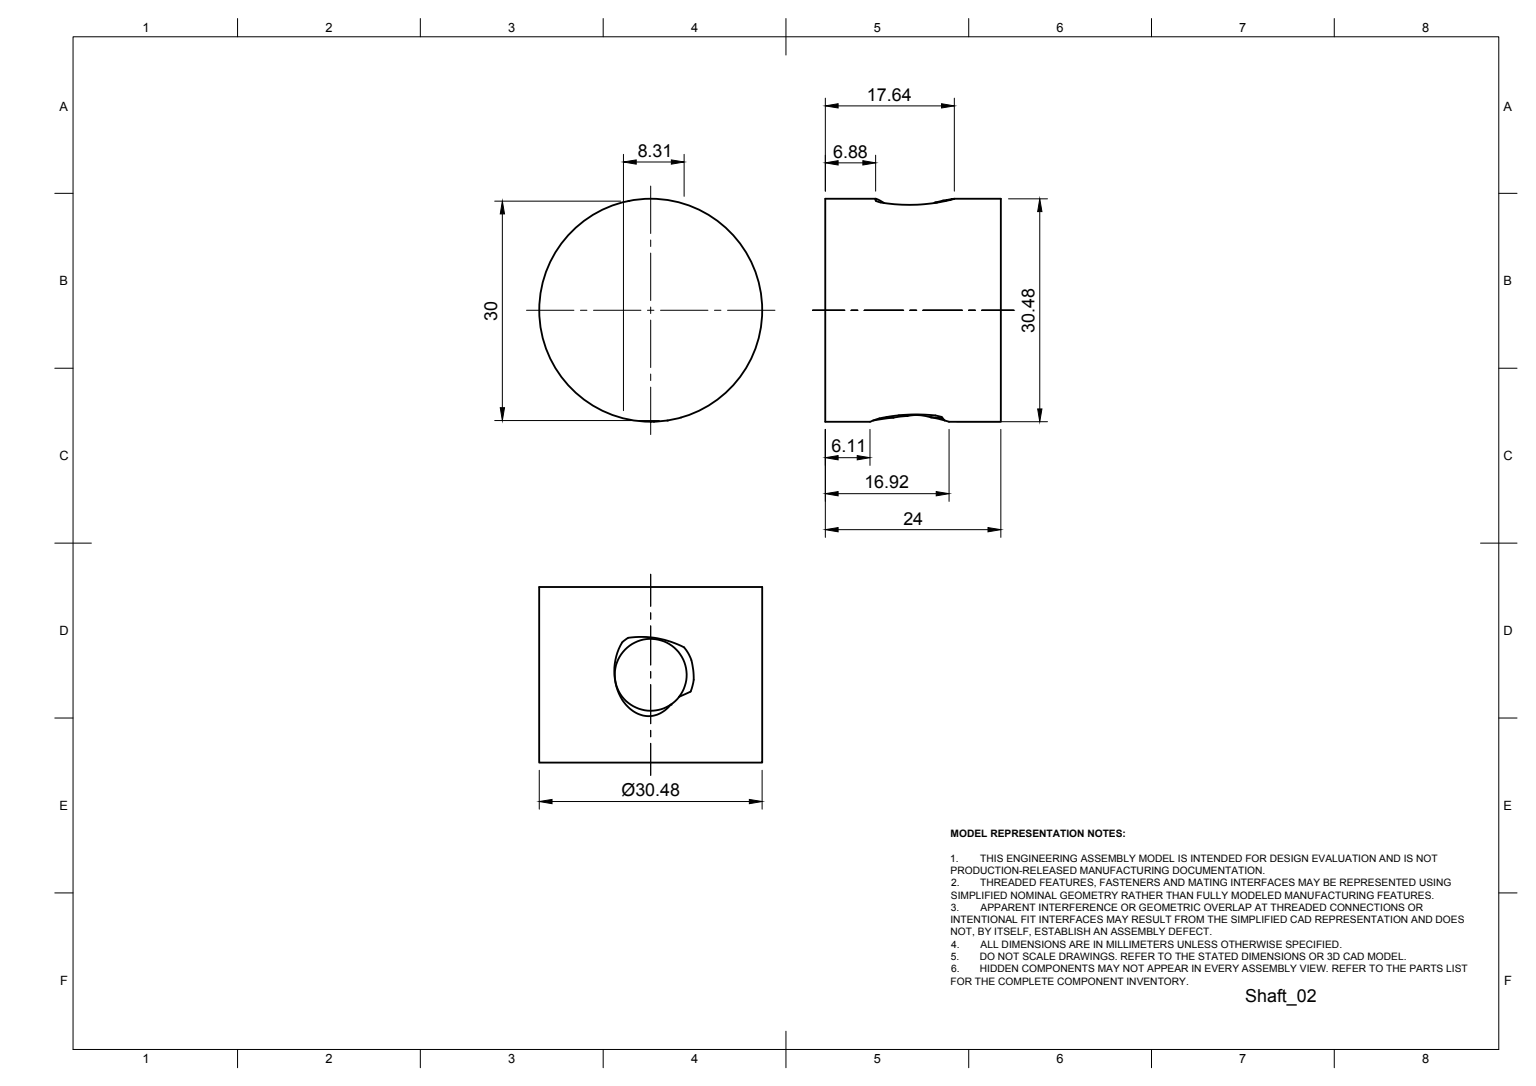
ISO-10303-21;
HEADER;
/* Generated by software containing ST-Developer
 * from STEP Tools, Inc. (www.steptools.com) 
 */

FILE_DESCRIPTION(
/* description */ (''),
/* implementation_level */ '2;1');

FILE_NAME(
/* name */ 'Shaft_02.step',
/* time_stamp */ '2026-10-06T13:41:14-07:00',
/* author */ (''),
/* organization */ (''),
/* preprocessor_version */ 'ST-DEVELOPER v20.2',
/* originating_system */ 'Autodesk Translation Framework v15.15.0.0',
/* authorisation */ '');

FILE_SCHEMA (('AUTOMOTIVE_DESIGN { 1 0 10303 214 3 1 1 }'));
ENDSEC;

DATA;
#10=MECHANICAL_DESIGN_GEOMETRIC_PRESENTATION_REPRESENTATION('',(#1967),#279266);
#53=B_SPLINE_SURFACE_WITH_KNOTS('',3,3,((#247756,#247757,#247758,#247759,
#247760,#247761,#247762,#247763,#247764,#247765,#247766,#247767,#247768,
#247769,#247770,#247771,#247772,#247773,#247774,#247775,#247776,#247777,
#247778,#247779,#247780,#247781,#247782,#247783,#247784,#247785,#247786,
#247787,#247788,#247789,#247790,#247791,#247792,#247793,#247794,#247795,
#247796,#247797,#247798,#247799,#247800,#247801,#247802,#247803,#247804,
#247805,#247806,#247807,#247808,#247809,#247810,#247811,#247812,#247813,
#247814,#247815,#247816,#247817,#247818,#247819,#247820,#247821,#247822,
#247823,#247824,#247825,#247826,#247827,#247828,#247829,#247830,#247831,
#247832,#247833,#247834,#247835,#247836,#247837,#247838,#247839,#247840,
#247841,#247842,#247843,#247844,#247845,#247846,#247847,#247848,#247849,
#247850,#247851,#247852,#247853,#247854,#247855,#247856,#247857,#247858,
#247859,#247860,#247861,#247862,#247863,#247864,#247865,#247866,#247867,
#247868,#247869,#247870,#247871,#247872,#247873,#247874,#247875,#247876,
#247877,#247878,#247879,#247880,#247881,#247882,#247883,#247884,#247885,
#247886,#247887,#247888,#247889,#247890,#247891,#247892,#247893,#247894,
#247895,#247896,#247897,#247898,#247899,#247900,#247901,#247902,#247903,
#247904,#247905,#247906,#247907,#247908,#247909,#247910,#247911,#247912,
#247913,#247914,#247915,#247916,#247917,#247918,#247919,#247920,#247921,
#247922,#247923,#247924,#247925,#247926,#247927,#247928,#247929,#247930,
#247931,#247932,#247933,#247934,#247935,#247936,#247937,#247938,#247939,
#247940,#247941,#247942,#247943,#247944,#247945,#247946,#247947,#247948,
#247949,#247950,#247951,#247952,#247953,#247954,#247955,#247956,#247957,
#247958,#247959,#247960,#247961,#247962,#247963,#247964,#247965,#247966,
#247967,#247968,#247969,#247970,#247971,#247972,#247973,#247974,#247975,
#247976,#247977,#247978,#247979,#247980,#247981,#247982,#247983,#247984,
#247985,#247986,#247987,#247988,#247989,#247990,#247991,#247992,#247993,
#247994,#247995,#247996,#247997,#247998,#247999,#248000,#248001,#248002,
#248003,#248004,#248005,#248006,#248007,#248008,#248009,#248010,#248011,
#248012,#248013,#248014,#248015,#248016,#248017,#248018,#248019,#248020,
#248021,#248022,#248023,#248024,#248025,#248026,#248027,#248028,#248029,
#248030,#248031,#248032,#248033,#248034,#248035,#248036,#248037,#248038,
#248039,#248040,#248041,#248042,#248043,#248044,#248045,#248046,#248047,
#248048,#248049,#248050,#248051,#248052,#248053,#248054,#248055,#248056,
#248057,#248058,#248059,#248060,#248061,#248062,#248063,#248064,#248065,
#248066,#248067,#248068,#248069,#248070,#248071,#248072,#248073,#248074,
#248075,#248076,#248077,#248078,#248079,#248080,#248081,#248082,#248083,
#248084,#248085,#248086,#248087,#248088,#248089,#248090,#248091,#248092,
#248093,#248094,#248095,#248096,#248097,#248098,#248099,#248100,#248101,
#248102,#248103,#248104,#248105,#248106,#248107,#248108,#248109,#248110,
#248111,#248112,#248113,#248114,#248115,#248116,#248117,#248118,#248119,
#248120,#248121,#248122,#248123,#248124,#248125,#248126,#248127,#248128,
#248129,#248130,#248131,#248132,#248133,#248134,#248135,#248136,#248137,
#248138,#248139,#248140,#248141,#248142,#248143,#248144,#248145,#248146,
#248147,#248148,#248149,#248150,#248151,#248152,#248153,#248154,#248155,
#248156,#248157,#248158,#248159,#248160,#248161,#248162,#248163,#248164,
#248165,#248166,#248167,#248168,#248169,#248170,#248171,#248172,#248173,
#248174,#248175,#248176,#248177,#248178,#248179,#248180,#248181,#248182,
#248183,#248184,#248185,#248186,#248187,#248188,#248189,#248190,#248191,
#248192,#248193,#248194,#248195,#248196,#248197,#248198,#248199,#248200,
#248201,#248202,#248203,#248204,#248205,#248206,#248207,#248208,#248209,
#248210,#248211,#248212,#248213,#248214,#248215,#248216,#248217,#248218,
#248219,#248220,#248221,#248222,#248223,#248224,#248225,#248226,#248227,
#248228,#248229,#248230,#248231,#248232,#248233,#248234,#248235,#248236,
#248237,#248238,#248239,#248240,#248241,#248242,#248243,#248244,#248245,
#248246,#248247,#248248,#248249,#248250,#248251,#248252,#248253,#248254,
#248255,#248256,#248257,#248258,#248259,#248260,#248261,#248262,#248263,
#248264,#248265,#248266,#248267,#248268,#248269,#248270,#248271,#248272,
#248273,#248274,#248275,#248276,#248277,#248278,#248279,#248280,#248281,
#248282,#248283,#248284,#248285,#248286,#248287,#248288,#248289,#248290,
#248291,#248292,#248293,#248294,#248295,#248296,#248297,#248298,#248299,
#248300,#248301,#248302,#248303,#248304,#248305,#248306,#248307,#248308,
#248309,#248310,#248311,#248312,#248313,#248314,#248315,#248316,#248317,
#248318,#248319,#248320,#248321,#248322,#248323,#248324,#248325,#248326,
#248327,#248328,#248329,#248330,#248331,#248332,#248333,#248334,#248335,
#248336,#248337,#248338,#248339,#248340,#248341,#248342,#248343,#248344,
#248345,#248346,#248347,#248348,#248349,#248350,#248351,#248352,#248353,
#248354,#248355,#248356,#248357,#248358,#248359,#248360,#248361,#248362,
#248363,#248364,#248365,#248366,#248367,#248368,#248369,#248370,#248371,
#248372,#248373,#248374,#248375,#248376,#248377,#248378,#248379,#248380,
#248381,#248382,#248383,#248384,#248385,#248386,#248387,#248388,#248389,
#248390,#248391,#248392,#248393,#248394,#248395,#248396,#248397,#248398,
#248399,#248400,#248401,#248402,#248403,#248404,#248405,#248406,#248407,
#248408,#248409,#248410,#248411,#248412,#248413,#248414,#248415,#248416,
#248417,#248418,#248419,#248420,#248421,#248422,#248423,#248424,#248425,
#248426,#248427,#248428,#248429,#248430,#248431,#248432,#248433,#248434,
#248435,#248436,#248437,#248438,#248439,#248440,#248441,#248442,#248443,
#248444,#248445,#248446,#248447,#248448,#248449,#248450,#248451,#248452,
#248453,#248454,#248455,#248456,#248457,#248458,#248459,#248460,#248461,
#248462,#248463,#248464,#248465,#248466,#248467,#248468,#248469,#248470,
#248471,#248472,#248473,#248474,#248475,#248476,#248477,#248478,#248479,
#248480,#248481,#248482,#248483,#248484,#248485,#248486,#248487,#248488,
#248489,#248490,#248491,#248492,#248493,#248494,#248495,#248496,#248497,
#248498,#248499,#248500,#248501,#248502,#248503,#248504,#248505,#248506,
#248507,#248508,#248509,#248510,#248511,#248512,#248513,#248514,#248515,
#248516,#248517,#248518,#248519,#248520,#248521,#248522,#248523,#248524,
#248525,#248526,#248527,#248528,#248529,#248530,#248531,#248532,#248533,
#248534,#248535,#248536,#248537,#248538,#248539,#248540,#248541,#248542,
#248543,#248544,#248545,#248546,#248547,#248548,#248549,#248550,#248551,
#248552,#248553,#248554,#248555,#248556,#248557,#248558,#248559,#248560,
#248561,#248562,#248563,#248564,#248565,#248566,#248567,#248568,#248569,
#248570,#248571,#248572,#248573,#248574,#248575,#248576,#248577,#248578,
#248579,#248580,#248581,#248582,#248583,#248584,#248585,#248586,#248587,
#248588,#248589,#248590,#248591,#248592,#248593,#248594,#248595,#248596,
#248597,#248598,#248599,#248600,#248601,#248602,#248603,#248604,#248605,
#248606,#248607,#248608,#248609,#248610,#248611,#248612,#248613,#248614,
#248615,#248616,#248617,#248618,#248619,#248620,#248621,#248622,#248623,
#248624,#248625,#248626,#248627,#248628,#248629,#248630,#248631,#248632,
#248633,#248634,#248635,#248636,#248637,#248638,#248639,#248640,#248641,
#248642,#248643,#248644,#248645,#248646,#248647,#248648,#248649,#248650,
#248651,#248652,#248653,#248654,#248655,#248656,#248657,#248658,#248659,
#248660,#248661,#248662,#248663,#248664,#248665,#248666,#248667,#248668,
#248669,#248670,#248671,#248672,#248673,#248674,#248675,#248676,#248677,
#248678,#248679,#248680,#248681,#248682,#248683,#248684,#248685,#248686,
#248687,#248688,#248689,#248690,#248691,#248692,#248693,#248694,#248695,
#248696,#248697,#248698,#248699,#248700,#248701,#248702,#248703,#248704,
#248705,#248706,#248707,#248708,#248709,#248710,#248711,#248712,#248713,
#248714,#248715,#248716,#248717,#248718,#248719,#248720,#248721,#248722,
#248723,#248724,#248725,#248726,#248727,#248728,#248729,#248730,#248731,
#248732,#248733,#248734,#248735,#248736,#248737,#248738,#248739,#248740,
#248741,#248742,#248743,#248744,#248745,#248746,#248747,#248748,#248749,
#248750,#248751,#248752,#248753,#248754,#248755,#248756,#248757,#248758,
#248759,#248760,#248761,#248762,#248763,#248764,#248765,#248766,#248767,
#248768,#248769,#248770,#248771,#248772,#248773,#248774,#248775,#248776,
#248777,#248778,#248779,#248780,#248781,#248782,#248783,#248784,#248785,
#248786,#248787,#248788,#248789,#248790,#248791,#248792,#248793,#248794,
#248795,#248796,#248797,#248798,#248799,#248800,#248801,#248802,#248803,
#248804,#248805,#248806,#248807,#248808,#248809,#248810,#248811,#248812,
#248813,#248814,#248815,#248816,#248817,#248818,#248819,#248820,#248821,
#248822,#248823,#248824,#248825,#248826,#248827,#248828,#248829,#248830,
#248831,#248832,#248833,#248834,#248835,#248836,#248837,#248838,#248839,
#248840,#248841,#248842,#248843,#248844,#248845,#248846,#248847,#248848,
#248849,#248850,#248851,#248852,#248853,#248854,#248855,#248856,#248857,
#248858,#248859,#248860,#248861,#248862,#248863,#248864,#248865,#248866,
#248867,#248868,#248869,#248870,#248871,#248872,#248873,#248874,#248875,
#248876,#248877,#248878,#248879,#248880,#248881,#248882,#248883,#248884,
#248885,#248886,#248887,#248888,#248889,#248890,#248891,#248892,#248893,
#248894,#248895,#248896,#248897,#248898,#248899,#248900,#248901,#248902,
#248903,#248904,#248905,#248906,#248907,#248908,#248909,#248910,#248911,
#248912,#248913,#248914,#248915,#248916,#248917,#248918,#248919,#248920,
#248921,#248922,#248923,#248924,#248925,#248926,#248927,#248928,#248929,
#248930,#248931,#248932,#248933,#248934,#248935,#248936,#248937,#248938,
#248939,#248940,#248941,#248942,#248943,#248944,#248945,#248946,#248947,
#248948,#248949,#248950,#248951,#248952,#248953,#248954,#248955,#248956,
#248957,#248958,#248959,#248960,#248961,#248962,#248963,#248964,#248965,
#248966,#248967,#248968,#248969,#248970,#248971,#248972,#248973,#248974,
#248975,#248976,#248977,#248978,#248979,#248980,#248981,#248982,#248983,
#248984,#248985,#248986,#248987,#248988,#248989,#248990,#248991,#248992,
#248993,#248994,#248995,#248996,#248997,#248998,#248999,#249000,#249001,
#249002,#249003,#249004,#249005,#249006,#249007,#249008,#249009,#249010,
#249011,#249012,#249013,#249014,#249015,#249016,#249017,#249018,#249019,
#249020,#249021,#249022,#249023,#249024,#249025,#249026,#249027,#249028,
#249029,#249030,#249031,#249032,#249033,#249034,#249035,#249036,#249037,
#249038,#249039,#249040,#249041,#249042,#249043,#249044,#249045,#249046,
#249047,#249048,#249049,#249050,#249051,#249052,#249053,#249054,#249055,
#249056,#249057,#249058,#249059,#249060,#249061,#249062,#249063,#249064,
#249065,#249066,#249067,#249068,#249069,#249070,#249071,#249072,#249073,
#249074,#249075,#249076,#249077,#249078,#249079,#249080,#249081,#249082,
#249083,#249084,#249085,#249086,#249087,#249088,#249089,#249090,#249091,
#249092,#249093,#249094,#249095,#249096,#249097,#249098,#249099,#249100,
#249101,#249102,#249103,#249104,#249105,#249106,#249107,#249108,#249109,
#249110,#249111,#249112,#249113,#249114,#249115,#249116,#249117,#249118,
#249119,#249120,#249121,#249122,#249123,#249124,#249125,#249126,#249127,
#249128,#249129,#249130,#249131,#249132,#249133,#249134,#249135,#249136,
#249137,#249138,#249139,#249140,#249141,#249142,#249143,#249144,#249145,
#249146,#249147,#249148,#249149,#249150,#249151,#249152,#249153,#249154,
#249155,#249156,#249157,#249158,#249159,#249160,#249161,#249162,#249163,
#249164,#249165,#249166,#249167,#249168,#249169,#249170,#249171,#249172,
#249173,#249174,#249175,#249176,#249177,#249178,#249179,#249180,#249181,
#249182,#249183,#249184,#249185,#249186,#249187,#249188,#249189,#249190,
#249191,#249192,#249193,#249194,#249195,#249196,#249197,#249198,#249199,
#249200,#249201,#249202,#249203,#249204,#249205,#249206,#249207,#249208,
#249209,#249210,#249211,#249212,#249213,#249214,#249215,#249216,#249217,
#249218,#249219,#249220,#249221,#249222,#249223,#249224,#249225,#249226,
#249227,#249228,#249229,#249230,#249231,#249232,#249233,#249234,#249235,
#249236,#249237,#249238,#249239,#249240,#249241,#249242,#249243,#249244,
#249245,#249246,#249247,#249248,#249249,#249250,#249251,#249252,#249253,
#249254,#249255,#249256,#249257,#249258,#249259,#249260,#249261,#249262,
#249263,#249264,#249265,#249266,#249267,#249268,#249269,#249270,#249271,
#249272,#249273,#249274,#249275,#249276,#249277,#249278,#249279,#249280,
#249281,#249282,#249283,#249284,#249285,#249286,#249287,#249288,#249289,
#249290,#249291,#249292,#249293,#249294,#249295,#249296,#249297,#249298,
#249299,#249300,#249301,#249302,#249303,#249304,#249305,#249306,#249307,
#249308,#249309,#249310,#249311,#249312,#249313,#249314,#249315,#249316,
#249317,#249318,#249319,#249320,#249321,#249322,#249323,#249324,#249325,
#249326,#249327,#249328,#249329,#249330,#249331,#249332,#249333,#249334,
#249335,#249336,#249337,#249338,#249339,#249340,#249341,#249342,#249343,
#249344,#249345,#249346,#249347,#249348,#249349,#249350,#249351,#249352,
#249353,#249354,#249355,#249356,#249357,#249358,#249359,#249360,#249361,
#249362,#249363,#249364,#249365,#249366,#249367,#249368,#249369,#249370,
#249371,#249372,#249373,#249374,#249375,#249376,#249377,#249378,#249379,
#249380,#249381,#249382,#249383,#249384,#249385,#249386,#249387,#249388,
#249389,#249390,#249391,#249392,#249393,#249394,#249395,#249396,#249397,
#249398,#249399,#249400,#249401,#249402,#249403,#249404,#249405,#249406,
#249407,#249408,#249409,#249410,#249411,#249412,#249413,#249414,#249415,
#249416,#249417,#249418,#249419,#249420,#249421,#249422,#249423,#249424,
#249425,#249426,#249427,#249428,#249429,#249430,#249431,#249432,#249433,
#249434,#249435,#249436,#249437,#249438,#249439,#249440,#249441,#249442,
#249443,#249444,#249445,#249446,#249447,#249448,#249449,#249450),(#249451,
#249452,#249453,#249454,#249455,#249456,#249457,#249458,#249459,#249460,
#249461,#249462,#249463,#249464,#249465,#249466,#249467,#249468,#249469,
#249470,#249471,#249472,#249473,#249474,#249475,#249476,#249477,#249478,
#249479,#249480,#249481,#249482,#249483,#249484,#249485,#249486,#249487,
#249488,#249489,#249490,#249491,#249492,#249493,#249494,#249495,#249496,
#249497,#249498,#249499,#249500,#249501,#249502,#249503,#249504,#249505,
#249506,#249507,#249508,#249509,#249510,#249511,#249512,#249513,#249514,
#249515,#249516,#249517,#249518,#249519,#249520,#249521,#249522,#249523,
#249524,#249525,#249526,#249527,#249528,#249529,#249530,#249531,#249532,
#249533,#249534,#249535,#249536,#249537,#249538,#249539,#249540,#249541,
#249542,#249543,#249544,#249545,#249546,#249547,#249548,#249549,#249550,
#249551,#249552,#249553,#249554,#249555,#249556,#249557,#249558,#249559,
#249560,#249561,#249562,#249563,#249564,#249565,#249566,#249567,#249568,
#249569,#249570,#249571,#249572,#249573,#249574,#249575,#249576,#249577,
#249578,#249579,#249580,#249581,#249582,#249583,#249584,#249585,#249586,
#249587,#249588,#249589,#249590,#249591,#249592,#249593,#249594,#249595,
#249596,#249597,#249598,#249599,#249600,#249601,#249602,#249603,#249604,
#249605,#249606,#249607,#249608,#249609,#249610,#249611,#249612,#249613,
#249614,#249615,#249616,#249617,#249618,#249619,#249620,#249621,#249622,
#249623,#249624,#249625,#249626,#249627,#249628,#249629,#249630,#249631,
#249632,#249633,#249634,#249635,#249636,#249637,#249638,#249639,#249640,
#249641,#249642,#249643,#249644,#249645,#249646,#249647,#249648,#249649,
#249650,#249651,#249652,#249653,#249654,#249655,#249656,#249657,#249658,
#249659,#249660,#249661,#249662,#249663,#249664,#249665,#249666,#249667,
#249668,#249669,#249670,#249671,#249672,#249673,#249674,#249675,#249676,
#249677,#249678,#249679,#249680,#249681,#249682,#249683,#249684,#249685,
#249686,#249687,#249688,#249689,#249690,#249691,#249692,#249693,#249694,
#249695,#249696,#249697,#249698,#249699,#249700,#249701,#249702,#249703,
#249704,#249705,#249706,#249707,#249708,#249709,#249710,#249711,#249712,
#249713,#249714,#249715,#249716,#249717,#249718,#249719,#249720,#249721,
#249722,#249723,#249724,#249725,#249726,#249727,#249728,#249729,#249730,
#249731,#249732,#249733,#249734,#249735,#249736,#249737,#249738,#249739,
#249740,#249741,#249742,#249743,#249744,#249745,#249746,#249747,#249748,
#249749,#249750,#249751,#249752,#249753,#249754,#249755,#249756,#249757,
#249758,#249759,#249760,#249761,#249762,#249763,#249764,#249765,#249766,
#249767,#249768,#249769,#249770,#249771,#249772,#249773,#249774,#249775,
#249776,#249777,#249778,#249779,#249780,#249781,#249782,#249783,#249784,
#249785,#249786,#249787,#249788,#249789,#249790,#249791,#249792,#249793,
#249794,#249795,#249796,#249797,#249798,#249799,#249800,#249801,#249802,
#249803,#249804,#249805,#249806,#249807,#249808,#249809,#249810,#249811,
#249812,#249813,#249814,#249815,#249816,#249817,#249818,#249819,#249820,
#249821,#249822,#249823,#249824,#249825,#249826,#249827,#249828,#249829,
#249830,#249831,#249832,#249833,#249834,#249835,#249836,#249837,#249838,
#249839,#249840,#249841,#249842,#249843,#249844,#249845,#249846,#249847,
#249848,#249849,#249850,#249851,#249852,#249853,#249854,#249855,#249856,
#249857,#249858,#249859,#249860,#249861,#249862,#249863,#249864,#249865,
#249866,#249867,#249868,#249869,#249870,#249871,#249872,#249873,#249874,
#249875,#249876,#249877,#249878,#249879,#249880,#249881,#249882,#249883,
#249884,#249885,#249886,#249887,#249888,#249889,#249890,#249891,#249892,
#249893,#249894,#249895,#249896,#249897,#249898,#249899,#249900,#249901,
#249902,#249903,#249904,#249905,#249906,#249907,#249908,#249909,#249910,
#249911,#249912,#249913,#249914,#249915,#249916,#249917,#249918,#249919,
#249920,#249921,#249922,#249923,#249924,#249925,#249926,#249927,#249928,
#249929,#249930,#249931,#249932,#249933,#249934,#249935,#249936,#249937,
#249938,#249939,#249940,#249941,#249942,#249943,#249944,#249945,#249946,
#249947,#249948,#249949,#249950,#249951,#249952,#249953,#249954,#249955,
#249956,#249957,#249958,#249959,#249960,#249961,#249962,#249963,#249964,
#249965,#249966,#249967,#249968,#249969,#249970,#249971,#249972,#249973,
#249974,#249975,#249976,#249977,#249978,#249979,#249980,#249981,#249982,
#249983,#249984,#249985,#249986,#249987,#249988,#249989,#249990,#249991,
#249992,#249993,#249994,#249995,#249996,#249997,#249998,#249999,#250000,
#250001,#250002,#250003,#250004,#250005,#250006,#250007,#250008,#250009,
#250010,#250011,#250012,#250013,#250014,#250015,#250016,#250017,#250018,
#250019,#250020,#250021,#250022,#250023,#250024,#250025,#250026,#250027,
#250028,#250029,#250030,#250031,#250032,#250033,#250034,#250035,#250036,
#250037,#250038,#250039,#250040,#250041,#250042,#250043,#250044,#250045,
#250046,#250047,#250048,#250049,#250050,#250051,#250052,#250053,#250054,
#250055,#250056,#250057,#250058,#250059,#250060,#250061,#250062,#250063,
#250064,#250065,#250066,#250067,#250068,#250069,#250070,#250071,#250072,
#250073,#250074,#250075,#250076,#250077,#250078,#250079,#250080,#250081,
#250082,#250083,#250084,#250085,#250086,#250087,#250088,#250089,#250090,
#250091,#250092,#250093,#250094,#250095,#250096,#250097,#250098,#250099,
#250100,#250101,#250102,#250103,#250104,#250105,#250106,#250107,#250108,
#250109,#250110,#250111,#250112,#250113,#250114,#250115,#250116,#250117,
#250118,#250119,#250120,#250121,#250122,#250123,#250124,#250125,#250126,
#250127,#250128,#250129,#250130,#250131,#250132,#250133,#250134,#250135,
#250136,#250137,#250138,#250139,#250140,#250141,#250142,#250143,#250144,
#250145,#250146,#250147,#250148,#250149,#250150,#250151,#250152,#250153,
#250154,#250155,#250156,#250157,#250158,#250159,#250160,#250161,#250162,
#250163,#250164,#250165,#250166,#250167,#250168,#250169,#250170,#250171,
#250172,#250173,#250174,#250175,#250176,#250177,#250178,#250179,#250180,
#250181,#250182,#250183,#250184,#250185,#250186,#250187,#250188,#250189,
#250190,#250191,#250192,#250193,#250194,#250195,#250196,#250197,#250198,
#250199,#250200,#250201,#250202,#250203,#250204,#250205,#250206,#250207,
#250208,#250209,#250210,#250211,#250212,#250213,#250214,#250215,#250216,
#250217,#250218,#250219,#250220,#250221,#250222,#250223,#250224,#250225,
#250226,#250227,#250228,#250229,#250230,#250231,#250232,#250233,#250234,
#250235,#250236,#250237,#250238,#250239,#250240,#250241,#250242,#250243,
#250244,#250245,#250246,#250247,#250248,#250249,#250250,#250251,#250252,
#250253,#250254,#250255,#250256,#250257,#250258,#250259,#250260,#250261,
#250262,#250263,#250264,#250265,#250266,#250267,#250268,#250269,#250270,
#250271,#250272,#250273,#250274,#250275,#250276,#250277,#250278,#250279,
#250280,#250281,#250282,#250283,#250284,#250285,#250286,#250287,#250288,
#250289,#250290,#250291,#250292,#250293,#250294,#250295,#250296,#250297,
#250298,#250299,#250300,#250301,#250302,#250303,#250304,#250305,#250306,
#250307,#250308,#250309,#250310,#250311,#250312,#250313,#250314,#250315,
#250316,#250317,#250318,#250319,#250320,#250321,#250322,#250323,#250324,
#250325,#250326,#250327,#250328,#250329,#250330,#250331,#250332,#250333,
#250334,#250335,#250336,#250337,#250338,#250339,#250340,#250341,#250342,
#250343,#250344,#250345,#250346,#250347,#250348,#250349,#250350,#250351,
#250352,#250353,#250354,#250355,#250356,#250357,#250358,#250359,#250360,
#250361,#250362,#250363,#250364,#250365,#250366,#250367,#250368,#250369,
#250370,#250371,#250372,#250373,#250374,#250375,#250376,#250377,#250378,
#250379,#250380,#250381,#250382,#250383,#250384,#250385,#250386,#250387,
#250388,#250389,#250390,#250391,#250392,#250393,#250394,#250395,#250396,
#250397,#250398,#250399,#250400,#250401,#250402,#250403,#250404,#250405,
#250406,#250407,#250408,#250409,#250410,#250411,#250412,#250413,#250414,
#250415,#250416,#250417,#250418,#250419,#250420,#250421,#250422,#250423,
#250424,#250425,#250426,#250427,#250428,#250429,#250430,#250431,#250432,
#250433,#250434,#250435,#250436,#250437,#250438,#250439,#250440,#250441,
#250442,#250443,#250444,#250445,#250446,#250447,#250448,#250449,#250450,
#250451,#250452,#250453,#250454,#250455,#250456,#250457,#250458,#250459,
#250460,#250461,#250462,#250463,#250464,#250465,#250466,#250467,#250468,
#250469,#250470,#250471,#250472,#250473,#250474,#250475,#250476,#250477,
#250478,#250479,#250480,#250481,#250482,#250483,#250484,#250485,#250486,
#250487,#250488,#250489,#250490,#250491,#250492,#250493,#250494,#250495,
#250496,#250497,#250498,#250499,#250500,#250501,#250502,#250503,#250504,
#250505,#250506,#250507,#250508,#250509,#250510,#250511,#250512,#250513,
#250514,#250515,#250516,#250517,#250518,#250519,#250520,#250521,#250522,
#250523,#250524,#250525,#250526,#250527,#250528,#250529,#250530,#250531,
#250532,#250533,#250534,#250535,#250536,#250537,#250538,#250539,#250540,
#250541,#250542,#250543,#250544,#250545,#250546,#250547,#250548,#250549,
#250550,#250551,#250552,#250553,#250554,#250555,#250556,#250557,#250558,
#250559,#250560,#250561,#250562,#250563,#250564,#250565,#250566,#250567,
#250568,#250569,#250570,#250571,#250572,#250573,#250574,#250575,#250576,
#250577,#250578,#250579,#250580,#250581,#250582,#250583,#250584,#250585,
#250586,#250587,#250588,#250589,#250590,#250591,#250592,#250593,#250594,
#250595,#250596,#250597,#250598,#250599,#250600,#250601,#250602,#250603,
#250604,#250605,#250606,#250607,#250608,#250609,#250610,#250611,#250612,
#250613,#250614,#250615,#250616,#250617,#250618,#250619,#250620,#250621,
#250622,#250623,#250624,#250625,#250626,#250627,#250628,#250629,#250630,
#250631,#250632,#250633,#250634,#250635,#250636,#250637,#250638,#250639,
#250640,#250641,#250642,#250643,#250644,#250645,#250646,#250647,#250648,
#250649,#250650,#250651,#250652,#250653,#250654,#250655,#250656,#250657,
#250658,#250659,#250660,#250661,#250662,#250663,#250664,#250665,#250666,
#250667,#250668,#250669,#250670,#250671,#250672,#250673,#250674,#250675,
#250676,#250677,#250678,#250679,#250680,#250681,#250682,#250683,#250684,
#250685,#250686,#250687,#250688,#250689,#250690,#250691,#250692,#250693,
#250694,#250695,#250696,#250697,#250698,#250699,#250700,#250701,#250702,
#250703,#250704,#250705,#250706,#250707,#250708,#250709,#250710,#250711,
#250712,#250713,#250714,#250715,#250716,#250717,#250718,#250719,#250720,
#250721,#250722,#250723,#250724,#250725,#250726,#250727,#250728,#250729,
#250730,#250731,#250732,#250733,#250734,#250735,#250736,#250737,#250738,
#250739,#250740,#250741,#250742,#250743,#250744,#250745,#250746,#250747,
#250748,#250749,#250750,#250751,#250752,#250753,#250754,#250755,#250756,
#250757,#250758,#250759,#250760,#250761,#250762,#250763,#250764,#250765,
#250766,#250767,#250768,#250769,#250770,#250771,#250772,#250773,#250774,
#250775,#250776,#250777,#250778,#250779,#250780,#250781,#250782,#250783,
#250784,#250785,#250786,#250787,#250788,#250789,#250790,#250791,#250792,
#250793,#250794,#250795,#250796,#250797,#250798,#250799,#250800,#250801,
#250802,#250803,#250804,#250805,#250806,#250807,#250808,#250809,#250810,
#250811,#250812,#250813,#250814,#250815,#250816,#250817,#250818,#250819,
#250820,#250821,#250822,#250823,#250824,#250825,#250826,#250827,#250828,
#250829,#250830,#250831,#250832,#250833,#250834,#250835,#250836,#250837,
#250838,#250839,#250840,#250841,#250842,#250843,#250844,#250845,#250846,
#250847,#250848,#250849,#250850,#250851,#250852,#250853,#250854,#250855,
#250856,#250857,#250858,#250859,#250860,#250861,#250862,#250863,#250864,
#250865,#250866,#250867,#250868,#250869,#250870,#250871,#250872,#250873,
#250874,#250875,#250876,#250877,#250878,#250879,#250880,#250881,#250882,
#250883,#250884,#250885,#250886,#250887,#250888,#250889,#250890,#250891,
#250892,#250893,#250894,#250895,#250896,#250897,#250898,#250899,#250900,
#250901,#250902,#250903,#250904,#250905,#250906,#250907,#250908,#250909,
#250910,#250911,#250912,#250913,#250914,#250915,#250916,#250917,#250918,
#250919,#250920,#250921,#250922,#250923,#250924,#250925,#250926,#250927,
#250928,#250929,#250930,#250931,#250932,#250933,#250934,#250935,#250936,
#250937,#250938,#250939,#250940,#250941,#250942,#250943,#250944,#250945,
#250946,#250947,#250948,#250949,#250950,#250951,#250952,#250953,#250954,
#250955,#250956,#250957,#250958,#250959,#250960,#250961,#250962,#250963,
#250964,#250965,#250966,#250967,#250968,#250969,#250970,#250971,#250972,
#250973,#250974,#250975,#250976,#250977,#250978,#250979,#250980,#250981,
#250982,#250983,#250984,#250985,#250986,#250987,#250988,#250989,#250990,
#250991,#250992,#250993,#250994,#250995,#250996,#250997,#250998,#250999,
#251000,#251001,#251002,#251003,#251004,#251005,#251006,#251007,#251008,
#251009,#251010,#251011,#251012,#251013,#251014,#251015,#251016,#251017,
#251018,#251019,#251020,#251021,#251022,#251023,#251024,#251025,#251026,
#251027,#251028,#251029,#251030,#251031,#251032,#251033,#251034,#251035,
#251036,#251037,#251038,#251039,#251040,#251041,#251042,#251043,#251044,
#251045,#251046,#251047,#251048,#251049,#251050,#251051,#251052,#251053,
#251054,#251055,#251056,#251057,#251058,#251059,#251060,#251061,#251062,
#251063,#251064,#251065,#251066,#251067,#251068,#251069,#251070,#251071,
#251072,#251073,#251074,#251075,#251076,#251077,#251078,#251079,#251080,
#251081,#251082,#251083,#251084,#251085,#251086,#251087,#251088,#251089,
#251090,#251091,#251092,#251093,#251094,#251095,#251096,#251097,#251098,
#251099,#251100,#251101,#251102,#251103,#251104,#251105,#251106,#251107,
#251108,#251109,#251110,#251111,#251112,#251113,#251114,#251115,#251116,
#251117,#251118,#251119,#251120,#251121,#251122,#251123,#251124,#251125,
#251126,#251127,#251128,#251129,#251130,#251131,#251132,#251133,#251134,
#251135,#251136,#251137,#251138,#251139,#251140,#251141,#251142,#251143,
#251144,#251145),(#251146,#251147,#251148,#251149,#251150,#251151,#251152,
#251153,#251154,#251155,#251156,#251157,#251158,#251159,#251160,#251161,
#251162,#251163,#251164,#251165,#251166,#251167,#251168,#251169,#251170,
#251171,#251172,#251173,#251174,#251175,#251176,#251177,#251178,#251179,
#251180,#251181,#251182,#251183,#251184,#251185,#251186,#251187,#251188,
#251189,#251190,#251191,#251192,#251193,#251194,#251195,#251196,#251197,
#251198,#251199,#251200,#251201,#251202,#251203,#251204,#251205,#251206,
#251207,#251208,#251209,#251210,#251211,#251212,#251213,#251214,#251215,
#251216,#251217,#251218,#251219,#251220,#251221,#251222,#251223,#251224,
#251225,#251226,#251227,#251228,#251229,#251230,#251231,#251232,#251233,
#251234,#251235,#251236,#251237,#251238,#251239,#251240,#251241,#251242,
#251243,#251244,#251245,#251246,#251247,#251248,#251249,#251250,#251251,
#251252,#251253,#251254,#251255,#251256,#251257,#251258,#251259,#251260,
#251261,#251262,#251263,#251264,#251265,#251266,#251267,#251268,#251269,
#251270,#251271,#251272,#251273,#251274,#251275,#251276,#251277,#251278,
#251279,#251280,#251281,#251282,#251283,#251284,#251285,#251286,#251287,
#251288,#251289,#251290,#251291,#251292,#251293,#251294,#251295,#251296,
#251297,#251298,#251299,#251300,#251301,#251302,#251303,#251304,#251305,
#251306,#251307,#251308,#251309,#251310,#251311,#251312,#251313,#251314,
#251315,#251316,#251317,#251318,#251319,#251320,#251321,#251322,#251323,
#251324,#251325,#251326,#251327,#251328,#251329,#251330,#251331,#251332,
#251333,#251334,#251335,#251336,#251337,#251338,#251339,#251340,#251341,
#251342,#251343,#251344,#251345,#251346,#251347,#251348,#251349,#251350,
#251351,#251352,#251353,#251354,#251355,#251356,#251357,#251358,#251359,
#251360,#251361,#251362,#251363,#251364,#251365,#251366,#251367,#251368,
#251369,#251370,#251371,#251372,#251373,#251374,#251375,#251376,#251377,
#251378,#251379,#251380,#251381,#251382,#251383,#251384,#251385,#251386,
#251387,#251388,#251389,#251390,#251391,#251392,#251393,#251394,#251395,
#251396,#251397,#251398,#251399,#251400,#251401,#251402,#251403,#251404,
#251405,#251406,#251407,#251408,#251409,#251410,#251411,#251412,#251413,
#251414,#251415,#251416,#251417,#251418,#251419,#251420,#251421,#251422,
#251423,#251424,#251425,#251426,#251427,#251428,#251429,#251430,#251431,
#251432,#251433,#251434,#251435,#251436,#251437,#251438,#251439,#251440,
#251441,#251442,#251443,#251444,#251445,#251446,#251447,#251448,#251449,
#251450,#251451,#251452,#251453,#251454,#251455,#251456,#251457,#251458,
#251459,#251460,#251461,#251462,#251463,#251464,#251465,#251466,#251467,
#251468,#251469,#251470,#251471,#251472,#251473,#251474,#251475,#251476,
#251477,#251478,#251479,#251480,#251481,#251482,#251483,#251484,#251485,
#251486,#251487,#251488,#251489,#251490,#251491,#251492,#251493,#251494,
#251495,#251496,#251497,#251498,#251499,#251500,#251501,#251502,#251503,
#251504,#251505,#251506,#251507,#251508,#251509,#251510,#251511,#251512,
#251513,#251514,#251515,#251516,#251517,#251518,#251519,#251520,#251521,
#251522,#251523,#251524,#251525,#251526,#251527,#251528,#251529,#251530,
#251531,#251532,#251533,#251534,#251535,#251536,#251537,#251538,#251539,
#251540,#251541,#251542,#251543,#251544,#251545,#251546,#251547,#251548,
#251549,#251550,#251551,#251552,#251553,#251554,#251555,#251556,#251557,
#251558,#251559,#251560,#251561,#251562,#251563,#251564,#251565,#251566,
#251567,#251568,#251569,#251570,#251571,#251572,#251573,#251574,#251575,
#251576,#251577,#251578,#251579,#251580,#251581,#251582,#251583,#251584,
#251585,#251586,#251587,#251588,#251589,#251590,#251591,#251592,#251593,
#251594,#251595,#251596,#251597,#251598,#251599,#251600,#251601,#251602,
#251603,#251604,#251605,#251606,#251607,#251608,#251609,#251610,#251611,
#251612,#251613,#251614,#251615,#251616,#251617,#251618,#251619,#251620,
#251621,#251622,#251623,#251624,#251625,#251626,#251627,#251628,#251629,
#251630,#251631,#251632,#251633,#251634,#251635,#251636,#251637,#251638,
#251639,#251640,#251641,#251642,#251643,#251644,#251645,#251646,#251647,
#251648,#251649,#251650,#251651,#251652,#251653,#251654,#251655,#251656,
#251657,#251658,#251659,#251660,#251661,#251662,#251663,#251664,#251665,
#251666,#251667,#251668,#251669,#251670,#251671,#251672,#251673,#251674,
#251675,#251676,#251677,#251678,#251679,#251680,#251681,#251682,#251683,
#251684,#251685,#251686,#251687,#251688,#251689,#251690,#251691,#251692,
#251693,#251694,#251695,#251696,#251697,#251698,#251699,#251700,#251701,
#251702,#251703,#251704,#251705,#251706,#251707,#251708,#251709,#251710,
#251711,#251712,#251713,#251714,#251715,#251716,#251717,#251718,#251719,
#251720,#251721,#251722,#251723,#251724,#251725,#251726,#251727,#251728,
#251729,#251730,#251731,#251732,#251733,#251734,#251735,#251736,#251737,
#251738,#251739,#251740,#251741,#251742,#251743,#251744,#251745,#251746,
#251747,#251748,#251749,#251750,#251751,#251752,#251753,#251754,#251755,
#251756,#251757,#251758,#251759,#251760,#251761,#251762,#251763,#251764,
#251765,#251766,#251767,#251768,#251769,#251770,#251771,#251772,#251773,
#251774,#251775,#251776,#251777,#251778,#251779,#251780,#251781,#251782,
#251783,#251784,#251785,#251786,#251787,#251788,#251789,#251790,#251791,
#251792,#251793,#251794,#251795,#251796,#251797,#251798,#251799,#251800,
#251801,#251802,#251803,#251804,#251805,#251806,#251807,#251808,#251809,
#251810,#251811,#251812,#251813,#251814,#251815,#251816,#251817,#251818,
#251819,#251820,#251821,#251822,#251823,#251824,#251825,#251826,#251827,
#251828,#251829,#251830,#251831,#251832,#251833,#251834,#251835,#251836,
#251837,#251838,#251839,#251840,#251841,#251842,#251843,#251844,#251845,
#251846,#251847,#251848,#251849,#251850,#251851,#251852,#251853,#251854,
#251855,#251856,#251857,#251858,#251859,#251860,#251861,#251862,#251863,
#251864,#251865,#251866,#251867,#251868,#251869,#251870,#251871,#251872,
#251873,#251874,#251875,#251876,#251877,#251878,#251879,#251880,#251881,
#251882,#251883,#251884,#251885,#251886,#251887,#251888,#251889,#251890,
#251891,#251892,#251893,#251894,#251895,#251896,#251897,#251898,#251899,
#251900,#251901,#251902,#251903,#251904,#251905,#251906,#251907,#251908,
#251909,#251910,#251911,#251912,#251913,#251914,#251915,#251916,#251917,
#251918,#251919,#251920,#251921,#251922,#251923,#251924,#251925,#251926,
#251927,#251928,#251929,#251930,#251931,#251932,#251933,#251934,#251935,
#251936,#251937,#251938,#251939,#251940,#251941,#251942,#251943,#251944,
#251945,#251946,#251947,#251948,#251949,#251950,#251951,#251952,#251953,
#251954,#251955,#251956,#251957,#251958,#251959,#251960,#251961,#251962,
#251963,#251964,#251965,#251966,#251967,#251968,#251969,#251970,#251971,
#251972,#251973,#251974,#251975,#251976,#251977,#251978,#251979,#251980,
#251981,#251982,#251983,#251984,#251985,#251986,#251987,#251988,#251989,
#251990,#251991,#251992,#251993,#251994,#251995,#251996,#251997,#251998,
#251999,#252000,#252001,#252002,#252003,#252004,#252005,#252006,#252007,
#252008,#252009,#252010,#252011,#252012,#252013,#252014,#252015,#252016,
#252017,#252018,#252019,#252020,#252021,#252022,#252023,#252024,#252025,
#252026,#252027,#252028,#252029,#252030,#252031,#252032,#252033,#252034,
#252035,#252036,#252037,#252038,#252039,#252040,#252041,#252042,#252043,
#252044,#252045,#252046,#252047,#252048,#252049,#252050,#252051,#252052,
#252053,#252054,#252055,#252056,#252057,#252058,#252059,#252060,#252061,
#252062,#252063,#252064,#252065,#252066,#252067,#252068,#252069,#252070,
#252071,#252072,#252073,#252074,#252075,#252076,#252077,#252078,#252079,
#252080,#252081,#252082,#252083,#252084,#252085,#252086,#252087,#252088,
#252089,#252090,#252091,#252092,#252093,#252094,#252095,#252096,#252097,
#252098,#252099,#252100,#252101,#252102,#252103,#252104,#252105,#252106,
#252107,#252108,#252109,#252110,#252111,#252112,#252113,#252114,#252115,
#252116,#252117,#252118,#252119,#252120,#252121,#252122,#252123,#252124,
#252125,#252126,#252127,#252128,#252129,#252130,#252131,#252132,#252133,
#252134,#252135,#252136,#252137,#252138,#252139,#252140,#252141,#252142,
#252143,#252144,#252145,#252146,#252147,#252148,#252149,#252150,#252151,
#252152,#252153,#252154,#252155,#252156,#252157,#252158,#252159,#252160,
#252161,#252162,#252163,#252164,#252165,#252166,#252167,#252168,#252169,
#252170,#252171,#252172,#252173,#252174,#252175,#252176,#252177,#252178,
#252179,#252180,#252181,#252182,#252183,#252184,#252185,#252186,#252187,
#252188,#252189,#252190,#252191,#252192,#252193,#252194,#252195,#252196,
#252197,#252198,#252199,#252200,#252201,#252202,#252203,#252204,#252205,
#252206,#252207,#252208,#252209,#252210,#252211,#252212,#252213,#252214,
#252215,#252216,#252217,#252218,#252219,#252220,#252221,#252222,#252223,
#252224,#252225,#252226,#252227,#252228,#252229,#252230,#252231,#252232,
#252233,#252234,#252235,#252236,#252237,#252238,#252239,#252240,#252241,
#252242,#252243,#252244,#252245,#252246,#252247,#252248,#252249,#252250,
#252251,#252252,#252253,#252254,#252255,#252256,#252257,#252258,#252259,
#252260,#252261,#252262,#252263,#252264,#252265,#252266,#252267,#252268,
#252269,#252270,#252271,#252272,#252273,#252274,#252275,#252276,#252277,
#252278,#252279,#252280,#252281,#252282,#252283,#252284,#252285,#252286,
#252287,#252288,#252289,#252290,#252291,#252292,#252293,#252294,#252295,
#252296,#252297,#252298,#252299,#252300,#252301,#252302,#252303,#252304,
#252305,#252306,#252307,#252308,#252309,#252310,#252311,#252312,#252313,
#252314,#252315,#252316,#252317,#252318,#252319,#252320,#252321,#252322,
#252323,#252324,#252325,#252326,#252327,#252328,#252329,#252330,#252331,
#252332,#252333,#252334,#252335,#252336,#252337,#252338,#252339,#252340,
#252341,#252342,#252343,#252344,#252345,#252346,#252347,#252348,#252349,
#252350,#252351,#252352,#252353,#252354,#252355,#252356,#252357,#252358,
#252359,#252360,#252361,#252362,#252363,#252364,#252365,#252366,#252367,
#252368,#252369,#252370,#252371,#252372,#252373,#252374,#252375,#252376,
#252377,#252378,#252379,#252380,#252381,#252382,#252383,#252384,#252385,
#252386,#252387,#252388,#252389,#252390,#252391,#252392,#252393,#252394,
#252395,#252396,#252397,#252398,#252399,#252400,#252401,#252402,#252403,
#252404,#252405,#252406,#252407,#252408,#252409,#252410,#252411,#252412,
#252413,#252414,#252415,#252416,#252417,#252418,#252419,#252420,#252421,
#252422,#252423,#252424,#252425,#252426,#252427,#252428,#252429,#252430,
#252431,#252432,#252433,#252434,#252435,#252436,#252437,#252438,#252439,
#252440,#252441,#252442,#252443,#252444,#252445,#252446,#252447,#252448,
#252449,#252450,#252451,#252452,#252453,#252454,#252455,#252456,#252457,
#252458,#252459,#252460,#252461,#252462,#252463,#252464,#252465,#252466,
#252467,#252468,#252469,#252470,#252471,#252472,#252473,#252474,#252475,
#252476,#252477,#252478,#252479,#252480,#252481,#252482,#252483,#252484,
#252485,#252486,#252487,#252488,#252489,#252490,#252491,#252492,#252493,
#252494,#252495,#252496,#252497,#252498,#252499,#252500,#252501,#252502,
#252503,#252504,#252505,#252506,#252507,#252508,#252509,#252510,#252511,
#252512,#252513,#252514,#252515,#252516,#252517,#252518,#252519,#252520,
#252521,#252522,#252523,#252524,#252525,#252526,#252527,#252528,#252529,
#252530,#252531,#252532,#252533,#252534,#252535,#252536,#252537,#252538,
#252539,#252540,#252541,#252542,#252543,#252544,#252545,#252546,#252547,
#252548,#252549,#252550,#252551,#252552,#252553,#252554,#252555,#252556,
#252557,#252558,#252559,#252560,#252561,#252562,#252563,#252564,#252565,
#252566,#252567,#252568,#252569,#252570,#252571,#252572,#252573,#252574,
#252575,#252576,#252577,#252578,#252579,#252580,#252581,#252582,#252583,
#252584,#252585,#252586,#252587,#252588,#252589,#252590,#252591,#252592,
#252593,#252594,#252595,#252596,#252597,#252598,#252599,#252600,#252601,
#252602,#252603,#252604,#252605,#252606,#252607,#252608,#252609,#252610,
#252611,#252612,#252613,#252614,#252615,#252616,#252617,#252618,#252619,
#252620,#252621,#252622,#252623,#252624,#252625,#252626,#252627,#252628,
#252629,#252630,#252631,#252632,#252633,#252634,#252635,#252636,#252637,
#252638,#252639,#252640,#252641,#252642,#252643,#252644,#252645,#252646,
#252647,#252648,#252649,#252650,#252651,#252652,#252653,#252654,#252655,
#252656,#252657,#252658,#252659,#252660,#252661,#252662,#252663,#252664,
#252665,#252666,#252667,#252668,#252669,#252670,#252671,#252672,#252673,
#252674,#252675,#252676,#252677,#252678,#252679,#252680,#252681,#252682,
#252683,#252684,#252685,#252686,#252687,#252688,#252689,#252690,#252691,
#252692,#252693,#252694,#252695,#252696,#252697,#252698,#252699,#252700,
#252701,#252702,#252703,#252704,#252705,#252706,#252707,#252708,#252709,
#252710,#252711,#252712,#252713,#252714,#252715,#252716,#252717,#252718,
#252719,#252720,#252721,#252722,#252723,#252724,#252725,#252726,#252727,
#252728,#252729,#252730,#252731,#252732,#252733,#252734,#252735,#252736,
#252737,#252738,#252739,#252740,#252741,#252742,#252743,#252744,#252745,
#252746,#252747,#252748,#252749,#252750,#252751,#252752,#252753,#252754,
#252755,#252756,#252757,#252758,#252759,#252760,#252761,#252762,#252763,
#252764,#252765,#252766,#252767,#252768,#252769,#252770,#252771,#252772,
#252773,#252774,#252775,#252776,#252777,#252778,#252779,#252780,#252781,
#252782,#252783,#252784,#252785,#252786,#252787,#252788,#252789,#252790,
#252791,#252792,#252793,#252794,#252795,#252796,#252797,#252798,#252799,
#252800,#252801,#252802,#252803,#252804,#252805,#252806,#252807,#252808,
#252809,#252810,#252811,#252812,#252813,#252814,#252815,#252816,#252817,
#252818,#252819,#252820,#252821,#252822,#252823,#252824,#252825,#252826,
#252827,#252828,#252829,#252830,#252831,#252832,#252833,#252834,#252835,
#252836,#252837,#252838,#252839,#252840),(#252841,#252842,#252843,#252844,
#252845,#252846,#252847,#252848,#252849,#252850,#252851,#252852,#252853,
#252854,#252855,#252856,#252857,#252858,#252859,#252860,#252861,#252862,
#252863,#252864,#252865,#252866,#252867,#252868,#252869,#252870,#252871,
#252872,#252873,#252874,#252875,#252876,#252877,#252878,#252879,#252880,
#252881,#252882,#252883,#252884,#252885,#252886,#252887,#252888,#252889,
#252890,#252891,#252892,#252893,#252894,#252895,#252896,#252897,#252898,
#252899,#252900,#252901,#252902,#252903,#252904,#252905,#252906,#252907,
#252908,#252909,#252910,#252911,#252912,#252913,#252914,#252915,#252916,
#252917,#252918,#252919,#252920,#252921,#252922,#252923,#252924,#252925,
#252926,#252927,#252928,#252929,#252930,#252931,#252932,#252933,#252934,
#252935,#252936,#252937,#252938,#252939,#252940,#252941,#252942,#252943,
#252944,#252945,#252946,#252947,#252948,#252949,#252950,#252951,#252952,
#252953,#252954,#252955,#252956,#252957,#252958,#252959,#252960,#252961,
#252962,#252963,#252964,#252965,#252966,#252967,#252968,#252969,#252970,
#252971,#252972,#252973,#252974,#252975,#252976,#252977,#252978,#252979,
#252980,#252981,#252982,#252983,#252984,#252985,#252986,#252987,#252988,
#252989,#252990,#252991,#252992,#252993,#252994,#252995,#252996,#252997,
#252998,#252999,#253000,#253001,#253002,#253003,#253004,#253005,#253006,
#253007,#253008,#253009,#253010,#253011,#253012,#253013,#253014,#253015,
#253016,#253017,#253018,#253019,#253020,#253021,#253022,#253023,#253024,
#253025,#253026,#253027,#253028,#253029,#253030,#253031,#253032,#253033,
#253034,#253035,#253036,#253037,#253038,#253039,#253040,#253041,#253042,
#253043,#253044,#253045,#253046,#253047,#253048,#253049,#253050,#253051,
#253052,#253053,#253054,#253055,#253056,#253057,#253058,#253059,#253060,
#253061,#253062,#253063,#253064,#253065,#253066,#253067,#253068,#253069,
#253070,#253071,#253072,#253073,#253074,#253075,#253076,#253077,#253078,
#253079,#253080,#253081,#253082,#253083,#253084,#253085,#253086,#253087,
#253088,#253089,#253090,#253091,#253092,#253093,#253094,#253095,#253096,
#253097,#253098,#253099,#253100,#253101,#253102,#253103,#253104,#253105,
#253106,#253107,#253108,#253109,#253110,#253111,#253112,#253113,#253114,
#253115,#253116,#253117,#253118,#253119,#253120,#253121,#253122,#253123,
#253124,#253125,#253126,#253127,#253128,#253129,#253130,#253131,#253132,
#253133,#253134,#253135,#253136,#253137,#253138,#253139,#253140,#253141,
#253142,#253143,#253144,#253145,#253146,#253147,#253148,#253149,#253150,
#253151,#253152,#253153,#253154,#253155,#253156,#253157,#253158,#253159,
#253160,#253161,#253162,#253163,#253164,#253165,#253166,#253167,#253168,
#253169,#253170,#253171,#253172,#253173,#253174,#253175,#253176,#253177,
#253178,#253179,#253180,#253181,#253182,#253183,#253184,#253185,#253186,
#253187,#253188,#253189,#253190,#253191,#253192,#253193,#253194,#253195,
#253196,#253197,#253198,#253199,#253200,#253201,#253202,#253203,#253204,
#253205,#253206,#253207,#253208,#253209,#253210,#253211,#253212,#253213,
#253214,#253215,#253216,#253217,#253218,#253219,#253220,#253221,#253222,
#253223,#253224,#253225,#253226,#253227,#253228,#253229,#253230,#253231,
#253232,#253233,#253234,#253235,#253236,#253237,#253238,#253239,#253240,
#253241,#253242,#253243,#253244,#253245,#253246,#253247,#253248,#253249,
#253250,#253251,#253252,#253253,#253254,#253255,#253256,#253257,#253258,
#253259,#253260,#253261,#253262,#253263,#253264,#253265,#253266,#253267,
#253268,#253269,#253270,#253271,#253272,#253273,#253274,#253275,#253276,
#253277,#253278,#253279,#253280,#253281,#253282,#253283,#253284,#253285,
#253286,#253287,#253288,#253289,#253290,#253291,#253292,#253293,#253294,
#253295,#253296,#253297,#253298,#253299,#253300,#253301,#253302,#253303,
#253304,#253305,#253306,#253307,#253308,#253309,#253310,#253311,#253312,
#253313,#253314,#253315,#253316,#253317,#253318,#253319,#253320,#253321,
#253322,#253323,#253324,#253325,#253326,#253327,#253328,#253329,#253330,
#253331,#253332,#253333,#253334,#253335,#253336,#253337,#253338,#253339,
#253340,#253341,#253342,#253343,#253344,#253345,#253346,#253347,#253348,
#253349,#253350,#253351,#253352,#253353,#253354,#253355,#253356,#253357,
#253358,#253359,#253360,#253361,#253362,#253363,#253364,#253365,#253366,
#253367,#253368,#253369,#253370,#253371,#253372,#253373,#253374,#253375,
#253376,#253377,#253378,#253379,#253380,#253381,#253382,#253383,#253384,
#253385,#253386,#253387,#253388,#253389,#253390,#253391,#253392,#253393,
#253394,#253395,#253396,#253397,#253398,#253399,#253400,#253401,#253402,
#253403,#253404,#253405,#253406,#253407,#253408,#253409,#253410,#253411,
#253412,#253413,#253414,#253415,#253416,#253417,#253418,#253419,#253420,
#253421,#253422,#253423,#253424,#253425,#253426,#253427,#253428,#253429,
#253430,#253431,#253432,#253433,#253434,#253435,#253436,#253437,#253438,
#253439,#253440,#253441,#253442,#253443,#253444,#253445,#253446,#253447,
#253448,#253449,#253450,#253451,#253452,#253453,#253454,#253455,#253456,
#253457,#253458,#253459,#253460,#253461,#253462,#253463,#253464,#253465,
#253466,#253467,#253468,#253469,#253470,#253471,#253472,#253473,#253474,
#253475,#253476,#253477,#253478,#253479,#253480,#253481,#253482,#253483,
#253484,#253485,#253486,#253487,#253488,#253489,#253490,#253491,#253492,
#253493,#253494,#253495,#253496,#253497,#253498,#253499,#253500,#253501,
#253502,#253503,#253504,#253505,#253506,#253507,#253508,#253509,#253510,
#253511,#253512,#253513,#253514,#253515,#253516,#253517,#253518,#253519,
#253520,#253521,#253522,#253523,#253524,#253525,#253526,#253527,#253528,
#253529,#253530,#253531,#253532,#253533,#253534,#253535,#253536,#253537,
#253538,#253539,#253540,#253541,#253542,#253543,#253544,#253545,#253546,
#253547,#253548,#253549,#253550,#253551,#253552,#253553,#253554,#253555,
#253556,#253557,#253558,#253559,#253560,#253561,#253562,#253563,#253564,
#253565,#253566,#253567,#253568,#253569,#253570,#253571,#253572,#253573,
#253574,#253575,#253576,#253577,#253578,#253579,#253580,#253581,#253582,
#253583,#253584,#253585,#253586,#253587,#253588,#253589,#253590,#253591,
#253592,#253593,#253594,#253595,#253596,#253597,#253598,#253599,#253600,
#253601,#253602,#253603,#253604,#253605,#253606,#253607,#253608,#253609,
#253610,#253611,#253612,#253613,#253614,#253615,#253616,#253617,#253618,
#253619,#253620,#253621,#253622,#253623,#253624,#253625,#253626,#253627,
#253628,#253629,#253630,#253631,#253632,#253633,#253634,#253635,#253636,
#253637,#253638,#253639,#253640,#253641,#253642,#253643,#253644,#253645,
#253646,#253647,#253648,#253649,#253650,#253651,#253652,#253653,#253654,
#253655,#253656,#253657,#253658,#253659,#253660,#253661,#253662,#253663,
#253664,#253665,#253666,#253667,#253668,#253669,#253670,#253671,#253672,
#253673,#253674,#253675,#253676,#253677,#253678,#253679,#253680,#253681,
#253682,#253683,#253684,#253685,#253686,#253687,#253688,#253689,#253690,
#253691,#253692,#253693,#253694,#253695,#253696,#253697,#253698,#253699,
#253700,#253701,#253702,#253703,#253704,#253705,#253706,#253707,#253708,
#253709,#253710,#253711,#253712,#253713,#253714,#253715,#253716,#253717,
#253718,#253719,#253720,#253721,#253722,#253723,#253724,#253725,#253726,
#253727,#253728,#253729,#253730,#253731,#253732,#253733,#253734,#253735,
#253736,#253737,#253738,#253739,#253740,#253741,#253742,#253743,#253744,
#253745,#253746,#253747,#253748,#253749,#253750,#253751,#253752,#253753,
#253754,#253755,#253756,#253757,#253758,#253759,#253760,#253761,#253762,
#253763,#253764,#253765,#253766,#253767,#253768,#253769,#253770,#253771,
#253772,#253773,#253774,#253775,#253776,#253777,#253778,#253779,#253780,
#253781,#253782,#253783,#253784,#253785,#253786,#253787,#253788,#253789,
#253790,#253791,#253792,#253793,#253794,#253795,#253796,#253797,#253798,
#253799,#253800,#253801,#253802,#253803,#253804,#253805,#253806,#253807,
#253808,#253809,#253810,#253811,#253812,#253813,#253814,#253815,#253816,
#253817,#253818,#253819,#253820,#253821,#253822,#253823,#253824,#253825,
#253826,#253827,#253828,#253829,#253830,#253831,#253832,#253833,#253834,
#253835,#253836,#253837,#253838,#253839,#253840,#253841,#253842,#253843,
#253844,#253845,#253846,#253847,#253848,#253849,#253850,#253851,#253852,
#253853,#253854,#253855,#253856,#253857,#253858,#253859,#253860,#253861,
#253862,#253863,#253864,#253865,#253866,#253867,#253868,#253869,#253870,
#253871,#253872,#253873,#253874,#253875,#253876,#253877,#253878,#253879,
#253880,#253881,#253882,#253883,#253884,#253885,#253886,#253887,#253888,
#253889,#253890,#253891,#253892,#253893,#253894,#253895,#253896,#253897,
#253898,#253899,#253900,#253901,#253902,#253903,#253904,#253905,#253906,
#253907,#253908,#253909,#253910,#253911,#253912,#253913,#253914,#253915,
#253916,#253917,#253918,#253919,#253920,#253921,#253922,#253923,#253924,
#253925,#253926,#253927,#253928,#253929,#253930,#253931,#253932,#253933,
#253934,#253935,#253936,#253937,#253938,#253939,#253940,#253941,#253942,
#253943,#253944,#253945,#253946,#253947,#253948,#253949,#253950,#253951,
#253952,#253953,#253954,#253955,#253956,#253957,#253958,#253959,#253960,
#253961,#253962,#253963,#253964,#253965,#253966,#253967,#253968,#253969,
#253970,#253971,#253972,#253973,#253974,#253975,#253976,#253977,#253978,
#253979,#253980,#253981,#253982,#253983,#253984,#253985,#253986,#253987,
#253988,#253989,#253990,#253991,#253992,#253993,#253994,#253995,#253996,
#253997,#253998,#253999,#254000,#254001,#254002,#254003,#254004,#254005,
#254006,#254007,#254008,#254009,#254010,#254011,#254012,#254013,#254014,
#254015,#254016,#254017,#254018,#254019,#254020,#254021,#254022,#254023,
#254024,#254025,#254026,#254027,#254028,#254029,#254030,#254031,#254032,
#254033,#254034,#254035,#254036,#254037,#254038,#254039,#254040,#254041,
#254042,#254043,#254044,#254045,#254046,#254047,#254048,#254049,#254050,
#254051,#254052,#254053,#254054,#254055,#254056,#254057,#254058,#254059,
#254060,#254061,#254062,#254063,#254064,#254065,#254066,#254067,#254068,
#254069,#254070,#254071,#254072,#254073,#254074,#254075,#254076,#254077,
#254078,#254079,#254080,#254081,#254082,#254083,#254084,#254085,#254086,
#254087,#254088,#254089,#254090,#254091,#254092,#254093,#254094,#254095,
#254096,#254097,#254098,#254099,#254100,#254101,#254102,#254103,#254104,
#254105,#254106,#254107,#254108,#254109,#254110,#254111,#254112,#254113,
#254114,#254115,#254116,#254117,#254118,#254119,#254120,#254121,#254122,
#254123,#254124,#254125,#254126,#254127,#254128,#254129,#254130,#254131,
#254132,#254133,#254134,#254135,#254136,#254137,#254138,#254139,#254140,
#254141,#254142,#254143,#254144,#254145,#254146,#254147,#254148,#254149,
#254150,#254151,#254152,#254153,#254154,#254155,#254156,#254157,#254158,
#254159,#254160,#254161,#254162,#254163,#254164,#254165,#254166,#254167,
#254168,#254169,#254170,#254171,#254172,#254173,#254174,#254175,#254176,
#254177,#254178,#254179,#254180,#254181,#254182,#254183,#254184,#254185,
#254186,#254187,#254188,#254189,#254190,#254191,#254192,#254193,#254194,
#254195,#254196,#254197,#254198,#254199,#254200,#254201,#254202,#254203,
#254204,#254205,#254206,#254207,#254208,#254209,#254210,#254211,#254212,
#254213,#254214,#254215,#254216,#254217,#254218,#254219,#254220,#254221,
#254222,#254223,#254224,#254225,#254226,#254227,#254228,#254229,#254230,
#254231,#254232,#254233,#254234,#254235,#254236,#254237,#254238,#254239,
#254240,#254241,#254242,#254243,#254244,#254245,#254246,#254247,#254248,
#254249,#254250,#254251,#254252,#254253,#254254,#254255,#254256,#254257,
#254258,#254259,#254260,#254261,#254262,#254263,#254264,#254265,#254266,
#254267,#254268,#254269,#254270,#254271,#254272,#254273,#254274,#254275,
#254276,#254277,#254278,#254279,#254280,#254281,#254282,#254283,#254284,
#254285,#254286,#254287,#254288,#254289,#254290,#254291,#254292,#254293,
#254294,#254295,#254296,#254297,#254298,#254299,#254300,#254301,#254302,
#254303,#254304,#254305,#254306,#254307,#254308,#254309,#254310,#254311,
#254312,#254313,#254314,#254315,#254316,#254317,#254318,#254319,#254320,
#254321,#254322,#254323,#254324,#254325,#254326,#254327,#254328,#254329,
#254330,#254331,#254332,#254333,#254334,#254335,#254336,#254337,#254338,
#254339,#254340,#254341,#254342,#254343,#254344,#254345,#254346,#254347,
#254348,#254349,#254350,#254351,#254352,#254353,#254354,#254355,#254356,
#254357,#254358,#254359,#254360,#254361,#254362,#254363,#254364,#254365,
#254366,#254367,#254368,#254369,#254370,#254371,#254372,#254373,#254374,
#254375,#254376,#254377,#254378,#254379,#254380,#254381,#254382,#254383,
#254384,#254385,#254386,#254387,#254388,#254389,#254390,#254391,#254392,
#254393,#254394,#254395,#254396,#254397,#254398,#254399,#254400,#254401,
#254402,#254403,#254404,#254405,#254406,#254407,#254408,#254409,#254410,
#254411,#254412,#254413,#254414,#254415,#254416,#254417,#254418,#254419,
#254420,#254421,#254422,#254423,#254424,#254425,#254426,#254427,#254428,
#254429,#254430,#254431,#254432,#254433,#254434,#254435,#254436,#254437,
#254438,#254439,#254440,#254441,#254442,#254443,#254444,#254445,#254446,
#254447,#254448,#254449,#254450,#254451,#254452,#254453,#254454,#254455,
#254456,#254457,#254458,#254459,#254460,#254461,#254462,#254463,#254464,
#254465,#254466,#254467,#254468,#254469,#254470,#254471,#254472,#254473,
#254474,#254475,#254476,#254477,#254478,#254479,#254480,#254481,#254482,
#254483,#254484,#254485,#254486,#254487,#254488,#254489,#254490,#254491,
#254492,#254493,#254494,#254495,#254496,#254497,#254498,#254499,#254500,
#254501,#254502,#254503,#254504,#254505,#254506,#254507,#254508,#254509,
#254510,#254511,#254512,#254513,#254514,#254515,#254516,#254517,#254518,
#254519,#254520,#254521,#254522,#254523,#254524,#254525,#254526,#254527,
#254528,#254529,#254530,#254531,#254532,#254533,#254534,#254535)),
 .UNSPECIFIED.,.F.,.F.,.F.,(4,4),(4,1,1,1,1,1,1,1,1,1,1,1,1,1,1,1,1,1,1,
1,1,1,1,1,1,1,1,1,1,1,1,1,1,1,1,1,1,1,1,1,1,1,1,1,1,1,1,1,1,1,1,1,1,1,1,
1,1,1,1,1,1,1,1,1,1,1,1,1,1,1,1,1,1,1,1,1,1,1,1,1,1,1,1,1,1,1,1,1,1,1,1,
1,1,1,1,1,1,1,1,1,1,1,1,1,1,1,1,1,1,1,1,1,1,1,1,1,1,1,1,1,1,1,1,1,1,1,1,
1,1,1,1,1,1,1,1,1,1,1,1,1,1,1,1,1,1,1,1,1,1,1,1,1,1,1,1,1,1,1,1,1,1,1,1,
1,1,1,1,1,1,1,1,1,1,1,1,1,1,1,1,1,1,1,1,1,1,1,1,1,1,1,1,1,1,1,1,1,1,1,1,
1,1,1,1,1,1,1,1,1,1,1,1,1,1,1,1,1,1,1,1,1,1,1,1,1,1,1,1,1,1,1,1,1,1,1,1,
1,1,1,1,1,1,1,1,1,1,1,1,1,1,1,1,1,1,1,1,1,1,1,1,1,1,1,1,1,1,1,1,1,1,1,1,
1,1,1,1,1,1,1,1,1,1,1,1,1,1,1,1,1,1,1,1,1,1,1,1,1,1,1,1,1,1,1,1,1,1,1,1,
1,1,1,1,1,1,1,1,1,1,1,1,1,1,1,1,1,1,1,1,1,1,1,1,1,1,1,1,1,1,1,1,1,1,1,1,
1,1,1,1,1,1,1,1,1,1,1,1,1,1,1,1,1,1,1,1,1,1,1,1,1,1,1,1,1,1,1,1,1,1,1,1,
1,1,1,1,1,1,1,1,1,1,1,1,1,1,1,1,1,1,1,1,1,1,1,1,1,1,1,1,1,1,1,1,1,1,1,1,
1,1,1,1,1,1,1,1,1,1,1,1,1,1,1,1,1,1,1,1,1,1,1,1,1,1,1,1,1,1,1,1,1,1,1,1,
1,1,1,1,1,1,1,1,1,1,1,1,1,1,1,1,1,1,1,1,1,1,1,1,1,1,1,1,1,1,1,1,1,1,1,1,
1,1,1,1,1,1,1,1,1,1,1,1,1,1,1,1,1,1,1,1,1,1,1,1,1,1,1,1,1,1,1,1,1,1,1,1,
1,1,1,1,1,1,1,1,1,1,1,1,1,1,1,1,1,1,1,1,1,1,1,1,1,1,1,1,1,1,1,1,1,1,1,1,
1,1,1,1,1,1,1,1,1,1,1,1,1,1,1,1,1,1,1,1,1,1,1,1,1,1,1,1,1,1,1,1,1,1,1,1,
1,1,1,1,1,1,1,1,1,1,1,1,1,1,1,1,1,1,1,1,1,1,1,1,1,1,1,1,1,1,1,1,1,1,1,1,
1,1,1,1,1,1,1,1,1,1,1,1,1,1,1,1,1,1,1,1,1,1,1,1,1,1,1,1,1,1,1,1,1,1,1,1,
1,1,1,1,1,1,1,1,1,1,1,1,1,1,1,1,1,1,1,1,1,1,1,1,1,1,1,1,1,1,1,1,1,1,1,1,
1,1,1,1,1,1,1,1,1,1,1,1,1,1,1,1,1,1,1,1,1,1,1,1,1,1,1,1,1,1,1,1,1,1,1,1,
1,1,1,1,1,1,1,1,1,1,1,1,1,1,1,1,1,1,1,1,1,1,1,1,1,1,1,1,1,1,1,1,1,1,1,1,
1,1,1,1,1,1,1,1,1,1,1,1,1,1,1,1,1,1,1,1,1,1,1,1,1,1,1,1,1,1,1,1,1,1,1,1,
1,1,1,1,1,1,1,1,1,1,1,1,1,1,1,1,1,1,1,1,1,1,1,1,1,1,1,1,1,1,1,1,1,1,1,1,
1,1,1,1,1,1,1,1,1,1,1,1,1,1,1,1,1,1,1,1,1,1,1,1,1,1,1,1,1,1,1,1,1,1,1,1,
1,1,1,1,1,1,1,1,1,1,1,1,1,1,1,1,1,1,1,1,1,1,1,1,1,1,1,1,1,1,1,1,1,1,1,1,
1,1,1,1,1,1,1,1,1,1,1,1,1,1,1,1,1,1,1,1,1,1,1,1,1,1,1,1,1,1,1,1,1,1,1,1,
1,1,1,1,1,1,1,1,1,1,1,1,1,1,1,1,1,1,1,1,1,1,1,1,1,1,1,1,1,1,1,1,1,1,1,1,
1,1,1,1,1,1,1,1,1,1,1,1,1,1,1,1,1,1,1,1,1,1,1,1,1,1,1,1,1,1,1,1,1,1,1,1,
1,1,1,1,1,1,1,1,1,1,1,1,1,1,1,1,1,1,1,1,1,1,1,1,1,1,1,1,1,1,1,1,1,1,1,1,
1,1,1,1,1,1,1,1,1,1,1,1,1,1,1,1,1,1,1,1,1,1,1,1,1,1,1,1,1,1,1,1,1,1,1,1,
1,1,1,1,1,1,1,1,1,1,1,1,1,1,1,1,1,1,1,1,1,1,1,1,1,1,1,1,1,1,1,1,1,1,1,1,
1,1,1,1,1,1,1,1,1,1,1,1,1,1,1,1,1,1,1,1,1,1,1,1,1,1,1,1,1,1,1,1,1,1,1,1,
1,1,1,1,1,1,1,1,1,1,1,1,1,1,1,1,1,1,1,1,1,1,1,1,1,1,1,1,1,1,1,1,1,1,1,1,
1,1,1,1,1,1,1,1,1,1,1,1,1,1,1,1,1,1,1,1,1,1,1,1,1,1,1,1,1,1,1,1,1,1,1,1,
1,1,1,1,1,1,1,1,1,1,1,1,1,1,1,1,1,1,1,1,1,1,1,1,1,1,1,1,1,1,1,1,1,1,1,1,
1,1,1,1,1,1,1,1,1,1,1,1,1,1,1,1,1,1,1,1,1,1,1,1,1,1,1,1,1,1,1,1,1,1,1,1,
1,1,1,1,1,1,1,1,1,1,1,1,1,1,1,1,1,1,1,1,1,1,1,1,1,1,1,1,1,1,1,1,1,1,1,1,
1,1,1,1,1,1,1,1,1,1,1,1,1,1,1,1,1,1,1,1,1,1,1,1,1,1,1,1,1,1,1,1,1,1,1,1,
1,1,1,1,1,1,1,1,1,1,1,1,1,1,1,1,1,1,1,1,1,1,1,1,1,1,1,1,1,1,1,1,1,1,1,1,
1,1,1,1,1,1,1,1,1,1,1,1,1,1,1,1,1,1,1,1,1,1,1,1,1,1,1,1,1,1,1,1,1,1,1,1,
1,1,1,1,1,1,1,1,1,1,1,1,1,1,1,1,1,1,1,1,1,1,1,1,1,1,1,1,1,1,1,1,1,1,1,1,
1,1,1,1,1,1,1,1,1,1,1,1,1,1,1,1,1,1,1,1,1,1,1,1,1,1,1,1,1,1,1,1,1,1,1,1,
1,1,1,1,1,1,1,1,1,1,1,1,1,1,1,1,1,1,1,1,1,1,1,1,1,1,1,1,1,1,1,1,1,1,1,1,
1,1,1,1,1,1,1,1,1,1,1,1,1,1,1,1,1,1,1,1,1,1,1,1,1,1,1,1,1,1,1,1,1,1,1,1,
1,1,1,1,1,1,1,1,1,1,1,1,1,1,1,1,1,1,1,1,1,1,1,1,1,1,1,1,1,1,1,1,1,1,1,1,
1,1,1,1,1,1,1,1,1,1,1,1,1,1,1,1,1,1,1,1,1,1,1,1,1,1,1,1,1,1,1,1,1,1,1,1,
1,1,1,1,1,1,1,1,1,1,1,1,1,1,1,1,1,4),(-0.000587328099657093,0.1157205948422),
(8.30590413559005,8.80579087257276,9.30565887793282,10.305394888653,11.3051308993731,
12.3048669100932,13.3046029208133,14.3043389315335,15.3040749422536,16.3038109529737,
17.3035469636939,18.303282974414,19.3030189851341,20.3027549958542,21.3024910065744,
22.3022270172945,23.3019630280146,24.3016990387348,25.3014350494549,26.301171060175,
27.3009070708951,28.3006430816153,29.3003790923354,30.3001151030555,31.2998511137757,
32.2995871244958,33.2993231352159,34.299059145936,35.2987951566562,36.2985311673763,
37.2982671780964,38.2980031888166,39.2977391995367,40.2974752102568,41.2972112209769,
42.2969472316971,43.2966832424172,44.2964192531373,45.2961552638575,46.2958912745776,
47.2956272852977,48.2953632960178,49.295099306738,50.2948353174581,51.2945713281782,
52.2943073388984,53.2940433496185,54.2937793603386,55.2935153710587,56.2932513817789,
57.292987392499,58.2927234032191,59.2924594139393,60.2921954246594,61.2919314353795,
62.2916674460996,63.2914034568198,64.2911394675399,65.29087547826,66.2906114889802,
67.2903474997003,68.2900835104204,69.2898195211405,70.2895555318607,71.2892915425808,
72.2890275533009,73.2887635640211,74.2884995747412,75.2882355854613,76.2879715961814,
77.2877076069016,78.2874436176217,79.2871796283418,80.286915639062,81.2866516497821,
82.2863876605022,83.2861236712224,84.2858596819425,85.2855956926626,86.2853317033827,
87.2850677141029,88.284803724823,89.2845397355431,90.2842757462633,91.2840117569834,
92.2837477677035,93.2834837784236,94.2832197891438,95.2829557998639,96.282691810584,
97.2824278213041,98.2821638320243,99.2818998427444,100.281635853465,101.281371864185,
102.281107874905,103.280843885625,104.280579896345,105.280315907065,106.280051917785,
107.279787928505,108.279523939226,109.279259949946,110.278995960666,111.278731971386,
112.278467982106,113.278203992826,114.277940003546,115.277676014266,116.277412024987,
117.277148035707,118.276884046427,119.276620057147,120.276356067867,121.276092078587,
122.275828089307,123.275564100028,124.275300110748,125.275036121468,126.274772132188,
127.274508142908,128.274244153628,129.273980164348,130.273716175068,131.273452185789,
132.273188196509,133.272924207229,134.272660217949,135.272396228669,136.272132239389,
137.271868250109,138.271604260829,139.27134027155,140.27107628227,141.27081229299,
142.27054830371,143.27028431443,144.27002032515,145.26975633587,146.26949234659,
147.269228357311,148.268964368031,149.268700378751,150.268436389471,151.268172400191,
152.267908410911,153.267644421631,154.267380432352,155.267116443072,156.266852453792,
157.266588464512,158.266324475232,159.266060485952,160.265796496672,161.265532507392,
162.265268518113,163.265004528833,164.264740539553,165.264476550273,166.264212560993,
167.263948571713,168.263684582433,169.263420593153,170.263156603874,171.262892614594,
172.262628625314,173.262364636034,174.262100646754,175.261836657474,176.261572668194,
177.261308678914,178.261044689635,179.260780700355,180.260516711075,181.260252721795,
182.259988732515,183.259724743235,184.259460753955,185.259196764675,186.258932775396,
187.258668786116,188.258404796836,189.258140807556,190.257876818276,191.257612828996,
192.257348839716,193.257084850437,194.256820861157,195.256556871877,196.256292882597,
197.256028893317,198.255764904037,199.255500914757,200.255236925477,201.254972936198,
202.254708946918,203.254444957638,204.254180968358,205.253916979078,206.253652989798,
207.253389000518,208.253125011238,209.252861021959,210.252597032679,211.252333043399,
212.252069054119,213.251805064839,214.251541075559,215.251277086279,216.251013096999,
217.25074910772,218.25048511844,219.25022112916,220.24995713988,221.2496931506,
222.24942916132,223.24916517204,224.248901182761,225.248637193481,226.248373204201,
227.248109214921,228.247845225641,229.247581236361,230.247317247081,231.247053257801,
232.246789268522,233.246525279242,234.246261289962,235.245997300682,236.245733311402,
237.245469322122,238.245205332842,239.244941343562,240.244677354283,241.244413365003,
242.244149375723,243.243885386443,244.243621397163,245.243357407883,246.243093418603,
247.242829429323,248.242565440044,249.242301450764,250.242037461484,251.241773472204,
252.241509482924,253.241245493644,254.240981504364,255.240717515084,256.240453525805,
257.240189536525,258.239925547245,259.239661557965,260.239397568685,261.239133579405,
262.238869590125,263.238605600846,264.238341611566,265.238077622286,266.237813633006,
267.237549643726,268.237285654446,269.237021665166,270.236757675886,271.236493686607,
272.236229697327,273.235965708047,274.235701718767,275.235437729487,276.235173740207,
277.234909750927,278.234645761647,279.234381772368,280.234117783088,281.233853793808,
282.233589804528,283.233325815248,284.233061825968,285.232797836688,286.232533847408,
287.232269858129,288.232005868849,289.231741879569,290.231477890289,291.231213901009,
292.230949911729,293.230685922449,294.23042193317,295.23015794389,296.22989395461,
297.22962996533,298.22936597605,299.22910198677,300.22883799749,301.22857400821,
302.228310018931,303.228046029651,304.227782040371,305.227518051091,306.227254061811,
307.226990072531,308.226726083251,309.226462093971,310.226198104692,311.225934115412,
312.225670126132,313.225406136852,314.225142147572,315.224878158292,316.224614169012,
317.224350179732,318.224086190453,319.223822201173,320.223558211893,321.223294222613,
322.223030233333,323.222766244053,324.222502254773,325.222238265494,326.221974276214,
327.221710286934,328.221446297654,329.221182308374,330.220918319094,331.220654329814,
332.220390340534,333.220126351255,334.219862361975,335.219598372695,336.219334383415,
337.219070394135,338.218806404855,339.218542415575,340.218278426295,341.218014437016,
342.217750447736,343.217486458456,344.217222469176,345.216958479896,346.216694490616,
347.216430501336,348.216166512056,349.215902522777,350.215638533497,351.215374544217,
352.215110554937,353.214846565657,354.214582576377,355.214318587097,356.214054597817,
357.213790608538,358.213526619258,359.213262629978,360.212998640698,361.212734651418,
362.212470662138,363.212206672858,364.211942683579,365.211678694299,366.211414705019,
367.211150715739,368.210886726459,369.210622737179,370.210358747899,371.210094758619,
372.20983076934,373.20956678006,374.20930279078,375.2090388015,376.20877481222,
377.20851082294,378.20824683366,379.20798284438,380.207718855101,381.207454865821,
382.207190876541,383.206926887261,384.206662897981,385.206398908701,386.206134919421,
387.205870930141,388.205606940862,389.205342951582,390.205078962302,391.204814973022,
392.204550983742,393.204286994462,394.204023005182,395.203759015903,396.203495026623,
397.203231037343,398.202967048063,399.202703058783,400.202439069503,401.202175080223,
402.201911090943,403.201647101664,404.201383112384,405.201119123104,406.200855133824,
407.200591144544,408.200327155264,409.200063165984,410.199799176704,411.199535187425,
412.199271198145,413.199007208865,414.198743219585,415.198479230305,416.198215241025,
417.197951251745,418.197687262465,419.197423273186,420.197159283906,421.196895294626,
422.196631305346,423.196367316066,424.196103326786,425.195839337506,426.195575348226,
427.195311358947,428.195047369667,429.194783380387,430.194519391107,431.194255401827,
432.193991412547,433.193727423267,434.193463433988,435.193199444708,436.192935455428,
437.192671466148,438.192407476868,439.192143487588,440.191879498308,441.191615509028,
442.191351519749,443.191087530469,444.190823541189,445.190559551909,446.190295562629,
447.190031573349,448.189767584069,449.189503594789,450.18923960551,451.18897561623,
452.18871162695,453.18844763767,454.18818364839,455.18791965911,456.18765566983,
457.18739168055,458.187127691271,459.186863701991,460.186599712711,461.186335723431,
462.186071734151,463.185807744871,464.185543755591,465.185279766312,466.185015777032,
467.184751787752,468.184487798472,469.184223809192,470.183959819912,471.183695830632,
472.183431841352,473.183167852073,474.182903862793,475.182639873513,476.182375884233,
477.182111894953,478.181847905673,479.181583916393,480.181319927113,481.181055937834,
482.180791948554,483.180527959274,484.180263969994,485.179999980714,486.179735991434,
487.179472002154,488.179208012874,489.178944023595,490.178680034315,491.178416045035,
492.178152055755,493.177888066475,494.177624077195,495.177360087915,496.177096098636,
497.176832109356,498.176568120076,499.176304130796,500.176040141516,501.175776152236,
502.175512162956,503.175248173676,504.174984184397,505.174720195117,506.174456205837,
507.174192216557,508.173928227277,509.173664237997,510.173400248717,511.173136259437,
512.172872270158,513.172608280878,514.172344291598,515.172080302318,516.171816313038,
517.171552323758,518.171288334478,519.171024345198,520.170760355919,521.170496366639,
522.170232377359,523.169968388079,524.169704398799,525.169440409519,526.169176420239,
527.168912430959,528.16864844168,529.1683844524,530.16812046312,531.16785647384,
532.16759248456,533.16732849528,534.167064506,535.166800516721,536.166536527441,
537.166272538161,538.166008548881,539.165744559601,540.165480570321,541.165216581041,
542.164952591761,543.164688602482,544.164424613202,545.164160623922,546.163896634642,
547.163632645362,548.163368656082,549.163104666802,550.162840677522,551.162576688243,
552.162312698963,553.162048709683,554.161784720403,555.161520731123,556.161256741843,
557.160992752563,558.160728763283,559.160464774004,560.160200784724,561.159936795444,
562.159672806164,563.159408816884,564.159144827604,565.158880838324,566.158616849045,
567.158352859765,568.158088870485,569.157824881205,570.157560891925,571.157296902645,
572.157032913365,573.156768924085,574.156504934806,575.156240945526,576.155976956246,
577.155712966966,578.155448977686,579.155184988406,580.154920999126,581.154657009846,
582.154393020567,583.154129031287,584.153865042007,585.153601052727,586.153337063447,
587.153073074167,588.152809084887,589.152545095607,590.152281106328,591.152017117048,
592.151753127768,593.151489138488,594.151225149208,595.150961159928,596.150697170648,
597.150433181368,598.150169192089,599.149905202809,600.149641213529,601.149377224249,
602.149113234969,603.148849245689,604.148585256409,605.14832126713,606.14805727785,
607.14779328857,608.14752929929,609.14726531001,610.14700132073,611.14673733145,
612.14647334217,613.146209352891,614.145945363611,615.145681374331,616.145417385051,
617.145153395771,618.144889406491,619.144625417211,620.144361427931,621.144097438652,
622.143833449372,623.143569460092,624.143305470812,625.143041481532,626.142777492252,
627.142513502972,628.142249513692,629.141985524413,630.141721535133,631.141457545853,
632.141193556573,633.140929567293,634.140665578013,635.140401588733,636.140137599454,
637.139873610174,638.139609620894,639.139345631614,640.139081642334,641.138817653054,
642.138553663774,643.138289674494,644.138025685215,645.137761695935,646.137497706655,
647.137233717375,648.136969728095,649.136705738815,650.136441749535,651.136177760255,
652.135913770976,653.135649781696,654.135385792416,655.135121803136,656.134857813856,
657.134593824576,658.134329835296,659.134065846016,660.133801856737,661.133537867457,
662.133273878177,663.133009888897,664.132745899617,665.132481910337,666.132217921057,
667.131953931778,668.131689942498,669.131425953218,670.131161963938,671.130897974658,
672.130633985378,673.130369996098,674.130106006818,675.129842017539,676.129578028259,
677.129314038979,678.129050049699,679.128786060419,680.128522071139,681.128258081859,
682.127994092579,683.1277301033,684.12746611402,685.12720212474,686.12693813546,
687.12667414618,688.1264101569,689.12614616762,690.12588217834,691.125618189061,
692.125354199781,693.125090210501,694.124826221221,695.124562231941,696.124298242661,
697.124034253381,698.123770264101,699.123506274822,700.123242285542,701.122978296262,
702.122714306982,703.122450317702,704.122186328422,705.121922339142,706.121658349863,
707.121394360583,708.121130371303,709.120866382023,710.120602392743,711.120338403463,
712.120074414183,713.119810424903,714.119546435624,715.119282446344,716.119018457064,
717.118754467784,718.118490478504,719.118226489224,720.117962499944,721.117698510664,
722.117434521385,723.117170532105,724.116906542825,725.116642553545,726.116378564265,
727.116114574985,728.115850585705,729.115586596425,730.115322607146,731.115058617866,
732.114794628586,733.114530639306,734.114266650026,735.114002660746,736.113738671466,
737.113474682187,738.113210692907,739.112946703627,740.112682714347,741.112418725067,
742.112154735787,743.111890746507,744.111626757227,745.111362767948,746.111098778668,
747.110834789388,748.110570800108,749.110306810828,750.110042821548,751.109778832268,
752.109514842988,753.109250853709,754.108986864429,755.108722875149,756.108458885869,
757.108194896589,758.107930907309,759.107666918029,760.107402928749,761.10713893947,
762.10687495019,763.10661096091,764.10634697163,765.10608298235,766.10581899307,
767.10555500379,768.10529101451,769.105027025231,770.104763035951,771.104499046671,
772.104235057391,773.103971068111,774.103707078831,775.103443089551,776.103179100272,
777.102915110992,778.102651121712,779.102387132432,780.102123143152,781.101859153872,
782.101595164592,783.101331175312,784.101067186033,785.100803196753,786.100539207473,
787.100275218193,788.100011228913,789.099747239633,790.099483250353,791.099219261073,
792.098955271794,793.098691282514,794.098427293234,795.098163303954,796.097899314674,
797.097635325394,798.097371336114,799.097107346834,800.096843357555,801.096579368275,
802.096315378995,803.096051389715,804.095787400435,805.095523411155,806.095259421875,
807.094995432596,808.094731443316,809.094467454036,810.094203464756,811.093939475476,
812.093675486196,813.093411496916,814.093147507636,815.092883518357,816.092619529077,
817.092355539797,818.092091550517,819.091827561237,820.091563571957,821.091299582677,
822.091035593397,823.090771604118,824.090507614838,825.090243625558,826.089979636278,
827.089715646998,828.089451657718,829.089187668438,830.088923679158,831.088659689879,
832.088395700599,833.088131711319,834.087867722039,835.087603732759,836.087339743479,
837.087075754199,838.08681176492,839.08654777564,840.08628378636,841.08601979708,
842.0857558078,843.08549181852,844.08522782924,845.08496383996,846.084699850681,
847.084435861401,848.084171872121,849.083907882841,850.083643893561,851.083379904281,
852.083115915001,853.082851925721,854.082587936442,855.082323947162,856.082059957882,
857.081795968602,858.081531979322,859.081267990042,860.081004000762,861.080740011482,
862.080476022203,863.080212032923,864.079948043643,865.079684054363,866.079420065083,
867.079156075803,868.078892086523,869.078628097243,870.078364107964,871.078100118684,
872.077836129404,873.077572140124,874.077308150844,875.077044161564,876.076780172284,
877.076516183005,878.076252193725,879.075988204445,880.075724215165,881.075460225885,
882.075196236605,883.074932247325,884.074668258045,885.074404268766,886.074140279486,
887.073876290206,888.073612300926,889.073348311646,890.073084322366,891.072820333086,
892.072556343806,893.072292354527,894.072028365247,895.071764375967,896.071500386687,
897.071236397407,898.070972408127,899.070708418847,900.070444429567,901.070180440288,
902.069916451008,903.069652461728,904.069388472448,905.069124483168,906.068860493888,
907.068596504608,908.068332515329,909.068068526049,910.067804536769,911.067540547489,
912.067276558209,913.067012568929,914.066748579649,915.066484590369,916.06622060109,
917.06595661181,918.06569262253,919.06542863325,920.06516464397,921.06490065469,
922.06463666541,923.06437267613,924.064108686851,925.063844697571,926.063580708291,
927.063316719011,928.063052729731,929.062788740451,930.062524751171,931.062260761891,
932.061996772612,933.061732783332,934.061468794052,935.061204804772,936.060940815492,
937.060676826212,938.060412836932,939.060148847652,940.059884858373,941.059620869093,
942.059356879813,943.059092890533,944.058828901253,945.058564911973,946.058300922693,
947.058036933414,948.057772944134,949.057508954854,950.057244965574,951.056980976294,
952.056716987014,953.056452997734,954.056189008454,955.055925019175,956.055661029895,
957.055397040615,958.055133051335,959.054869062055,960.054605072775,961.054341083495,
962.054077094215,963.053813104936,964.053549115656,965.053285126376,966.053021137096,
967.052757147816,968.052493158536,969.052229169256,970.051965179976,971.051701190697,
972.051437201417,973.051173212137,974.050909222857,975.050645233577,976.050381244297,
977.050117255017,978.049853265738,979.049589276458,980.049325287178,981.049061297898,
982.048797308618,983.048533319338,984.048269330058,985.048005340778,986.047741351499,
987.047477362219,988.047213372939,989.046949383659,990.046685394379,991.046421405099,
992.046157415819,993.045893426539,994.04562943726,995.04536544798,996.0451014587,
997.04483746942,998.04457348014,999.04430949086,1000.04404550158,1001.0437815123,
1002.04351752302,1003.04325353374,1004.04298954446,1005.04272555518,1006.0424615659,
1007.04219757662,1008.04193358734,1009.04166959806,1010.04140560878,1011.0411416195,
1012.04087763022,1013.04061364094,1014.04034965166,1015.04008566238,1016.0398216731,
1017.03955768382,1018.03929369454,1019.03902970526,1020.03876571598,1021.0385017267,
1022.03823773742,1023.03797374814,1024.03770975886,1025.03744576958,1026.0371817803,
1027.03691779102,1028.03665380174,1029.03638981246,1030.03612582318,1031.0358618339,
1032.03559784462,1033.03533385534,1034.03506986606,1035.03480587678,1036.03454188751,
1037.03427789823,1038.03401390895,1039.03374991967,1040.03348593039,1041.03322194111,
1042.03295795183,1043.03269396255,1044.03242997327,1045.03216598399,1046.03190199471,
1047.03163800543,1048.03137401615,1049.03111002687,1050.03084603759,1051.03058204831,
1052.03031805903,1053.03005406975,1054.02979008047,1055.02952609119,1056.02926210191,
1057.02899811263,1058.02873412335,1059.02847013407,1060.02820614479,1061.02794215551,
1062.02767816623,1063.02741417695,1064.02715018767,1065.02688619839,1066.02662220911,
1067.02635821983,1068.02609423055,1069.02583024127,1070.02556625199,1071.02530226271,
1072.02503827343,1073.02477428415,1074.02451029487,1075.02424630559,1076.02398231631,
1077.02371832703,1078.02345433775,1079.02319034847,1080.02292635919,1081.02266236991,
1082.02239838063,1083.02213439135,1084.02187040207,1085.02160641279,1086.02134242351,
1087.02107843423,1088.02081444495,1089.02055045567,1090.02028646639,1091.02002247711,
1092.01975848783,1093.01949449855,1094.01923050927,1095.01896651999,1096.01870253071,
1097.01843854143,1098.01817455215,1099.01791056287,1100.01764657359,1101.01738258431,
1102.01711859503,1103.01685460575,1104.01659061647,1105.01632662719,1106.01606263791,
1107.01579864863,1108.01553465935,1109.01527067007,1110.01500668079,1111.01474269151,
1112.01447870223,1113.01421471295,1114.01395072368,1115.0136867344,1116.01342274512,
1117.01315875584,1118.01289476656,1119.01263077728,1120.012366788,1121.01210279872,
1122.01183880944,1123.01157482016,1124.01131083088,1125.0110468416,1126.01078285232,
1127.01051886304,1128.01025487376,1129.00999088448,1130.0097268952,1131.00946290592,
1132.00919891664,1133.00893492736,1134.00867093808,1135.0084069488,1136.00814295952,
1137.00787897024,1138.00761498096,1139.00735099168,1140.0070870024,1141.00682301312,
1142.00655902384,1143.00629503456,1144.00603104528,1145.005767056,1146.00550306672,
1147.00523907744,1148.00497508816,1149.00471109888,1150.0044471096,1151.00418312032,
1152.00391913104,1153.00365514176,1154.00339115248,1155.0031271632,1156.00286317392,
1157.00259918464,1158.00233519536,1159.00207120608,1160.0018072168,1161.00154322752,
1162.00127923824,1163.00101524896,1164.00075125968,1165.0004872704,1166.00022328112,
1166.99995929184,1167.99969530256,1168.99943131328,1169.999167324,1170.99890333472,
1171.99863934544,1172.99837535616,1173.99811136688,1174.9978473776,1175.99758338832,
1176.99731939904,1177.99705540976,1178.99679142048,1179.9965274312,1180.99626344192,
1181.99599945264,1182.99573546336,1183.99547147408,1184.9952074848,1185.99494349552,
1186.99467950624,1187.99441551696,1188.99415152768,1189.99388753841,1190.99362354913,
1191.99335955985,1192.99309557057,1193.99283158129,1194.99256759201,1195.99230360273,
1196.99203961345,1197.99177562417,1198.99151163489,1199.99124764561,1200.99098365633,
1201.99071966705,1202.99045567777,1203.99019168849,1204.98992769921,1205.98966370993,
1206.98939972065,1207.98913573137,1208.98887174209,1209.98860775281,1210.98834376353,
1211.98807977425,1212.98781578497,1213.98755179569,1214.98728780641,1215.98702381713,
1216.98675982785,1217.98649583857,1218.98623184929,1219.98596786001,1220.98570387073,
1221.98543988145,1222.98517589217,1223.98491190289,1224.98464791361,1225.98438392433,
1226.98411993505,1227.98385594577,1228.98359195649,1229.98332796721,1230.98306397793,
1231.98279998865,1232.98253599937,1233.98227201009,1234.98200802081,1235.98174403153,
1236.98148004225,1237.98121605297,1238.98095206369,1239.98068807441,1240.98042408513,
1241.98016009585,1242.97989610657,1243.97963211729,1244.97936812801,1245.97910413873,
1246.97884014945,1247.97857616017,1248.97831217089,1249.97804818161,1250.97778419233,
1251.97752020305,1252.97725621377,1253.97699222449,1254.97672823521,1255.97646424593,
1256.97620025665,1257.97593626737,1258.97567227809,1259.97540828881,1260.97514429953,
1261.97488031025,1262.97461632097,1263.97435233169,1264.97408834241,1265.97382435313,
1266.97356036385,1267.97329637458,1268.9730323853,1269.97276839602,1270.97250440674,
1271.97224041746,1272.97197642818,1273.9717124389,1274.97144844962,1275.97118446034,
1276.97092047106,1277.97065648178,1278.9703924925,1279.97012850322,1280.96986451394,
1281.96960052466,1282.96933653538,1283.9690725461,1284.96880855682,1285.96854456754,
1286.96828057826,1287.96801658898,1288.9677525997,1289.96748861042,1290.96722462114,
1291.96696063186,1292.96669664258,1293.9664326533,1294.96616866402,1295.96590467474,
1296.96564068546,1297.96537669618,1298.9651127069,1299.96484871762,1300.96458472834,
1301.96432073906,1302.96405674978,1303.9637927605,1304.96352877122,1305.96326478194,
1306.96300079266,1307.96273680338,1308.9624728141,1309.96220882482,1310.96194483554,
1311.96168084626,1312.96141685698,1313.9611528677,1314.96088887842,1315.96062488914,
1316.96036089986,1317.96009691058,1318.9598329213,1319.95956893202,1320.95930494274,
1321.95904095346,1322.95877696418,1323.9585129749,1324.95824898562,1325.95798499634,
1326.95772100706,1327.95745701778,1328.9571930285,1329.95692903922,1330.95666504994,
1331.95640106066,1332.95613707138,1333.9558730821,1334.95560909282,1335.95534510354,
1336.95508111426,1337.95481712498,1338.9545531357,1339.95428914642,1340.95402515714,
1341.95376116786,1342.95349717858,1343.9532331893,1344.95296920002,1345.95270521075,
1346.95244122147,1347.95217723219,1348.95191324291,1349.95164925363,1350.95138526435,
1351.95112127507,1352.95085728579,1353.95059329651,1354.95032930723,1355.95006531795,
1356.94980132867,1357.94953733939,1358.94927335011,1359.94900936083,1360.94874537155,
1361.94848138227,1362.94821739299,1363.94795340371,1364.94768941443,1365.94742542515,
1366.94716143587,1367.94689744659,1368.94663345731,1369.94636946803,1370.94610547875,
1371.94584148947,1372.94557750019,1373.94531351091,1374.94504952163,1375.94478553235,
1376.94452154307,1377.94425755379,1378.94399356451,1379.94372957523,1380.94346558595,
1381.94320159667,1382.94293760739,1383.94267361811,1384.94240962883,1385.94214563955,
1386.94188165027,1387.94161766099,1388.94135367171,1389.94108968243,1390.94082569315,
1391.94056170387,1392.94029771459,1393.94003372531,1394.93976973603,1395.93950574675,
1396.93924175747,1397.93897776819,1398.93871377891,1399.93844978963,1400.93818580035,
1401.93792181107,1402.93765782179,1403.93739383251,1404.93712984323,1405.93686585395,
1406.93660186467,1407.93633787539,1408.93607388611,1409.93580989683,1410.93554590755,
1411.93528191827,1412.93501792899,1413.93475393971,1414.93448995043,1415.93422596115,
1416.93396197187,1417.93369798259,1418.93343399331,1419.93317000403,1420.93290601475,
1421.93264202547,1422.93237803619,1423.93211404692,1424.93185005764,1425.93158606836,
1426.93132207908,1427.9310580898,1428.93079410052,1429.93053011124,1430.93026612196,
1431.93000213268,1432.9297381434,1433.92947415412,1434.92921016484,1435.92894617556,
1436.92868218628,1437.928418197,1438.92815420772,1439.92789021844,1440.92762622916,
1441.92736223988,1442.9270982506,1443.92683426132,1444.92657027204,1445.92630628276,
1446.92604229348,1447.9257783042,1448.92551431492,1449.92525032564,1450.92498633636,
1451.92472234708,1452.9244583578,1453.92419436852,1454.92393037924,1455.92366638996,
1456.92340240068,1457.9231384114,1458.92287442212,1459.92261043284,1460.92234644356,
1461.92208245428,1462.921818465,1463.92155447572,1464.92129048644,1465.92102649716,
1466.92076250788,1467.9204985186,1468.92023452932,1469.91997054004,1470.91970655076,
1471.91944256148,1472.9191785722,1473.91891458292,1474.91865059364,1475.91838660436,
1476.91812261508,1477.9178586258,1478.91759463652,1479.91733064724,1480.91706665796,
1481.91680266868,1482.9165386794,1483.91627469012,1484.91601070084,1485.91574671156,
1486.91548272228,1487.915218733,1488.91495474372,1489.91469075444,1490.91442676516,
1491.91416277588,1492.9138987866,1493.91363479732,1494.91337080804,1495.91310681876,
1496.91284282948,1497.9125788402,1498.91231485092,1499.91205086164,1500.91178687236,
1501.91152288309,1502.91125889381,1503.91099490453,1504.91073091525,1505.91046692597,
1506.91020293669,1507.90993894741,1508.90967495813,1509.90941096885,1510.90914697957,
1511.90888299029,1512.90861900101,1513.90835501173,1514.90809102245,1515.90782703317,
1516.90756304389,1517.90729905461,1518.90703506533,1519.90677107605,1520.90650708677,
1521.90624309749,1522.90597910821,1523.90571511893,1524.90545112965,1525.90518714037,
1526.90492315109,1527.90465916181,1528.90439517253,1529.90413118325,1530.90386719397,
1531.90360320469,1532.90333921541,1533.90307522613,1534.90281123685,1535.90254724757,
1536.90228325829,1537.90201926901,1538.90175527973,1539.90149129045,1540.90122730117,
1541.90096331189,1542.90069932261,1543.90043533333,1544.90017134405,1545.89990735477,
1546.89964336549,1547.89937937621,1548.89911538693,1549.89885139765,1550.89858740837,
1551.89832341909,1552.89805942981,1553.89779544053,1554.89753145125,1555.89726746197,
1556.89700347269,1557.89673948341,1558.89647549413,1559.89621150485,1560.89594751557,
1561.89568352629,1562.89541953701,1563.89515554773,1564.89489155845,1565.89462756917,
1566.89436357989,1567.89409959061,1568.89383560133,1569.89357161205,1570.89330762277,
1571.89304363349,1572.89277964421,1573.89251565493,1574.89225166565,1575.89198767637,
1576.89172368709,1577.89145969781,1578.89119570853,1579.89093171926,1580.89066772998,
1581.8904037407,1582.89013975142,1583.88987576214,1584.88961177286,1585.88934778358,
1586.8890837943,1587.88881980502,1588.88855581574,1589.88829182646,1590.88802783718,
1591.8877638479,1592.88749985862,1593.88723586934,1594.88697188006,1595.88670789078,
1596.8864439015,1597.88617991222,1598.88591592294,1599.88565193366,1600.88538794438,
1601.8851239551,1602.88485996582,1603.88459597654,1604.88433198726,1605.88406799798,
1606.8838040087,1607.88354001942,1608.88327603014,1609.88301204086,1610.88274805158,
1611.8824840623,1612.88222007302,1613.88195608374,1614.88169209446,1615.88142810518,
1616.8811641159,1617.88090012662,1618.88063613734,1619.88037214806,1620.88010815878,
1621.8798441695,1622.87958018022,1623.87931619094,1624.87905220166,1625.87878821238,
1626.8785242231,1627.87826023382,1628.87799624454,1629.87773225526,1630.87746826598,
1631.8772042767,1632.87694028742,1633.87667629814,1634.87641230886,1635.87614831958,
1636.8758843303,1637.87562034102,1638.87535635174,1639.87509236246,1640.87482837318,
1641.8745643839,1642.87430039462,1643.87403640534,1644.87377241606,1645.87350842678,
1646.8732444375,1647.87298044822,1648.87271645894,1649.87245246966,1650.87218848038,
1651.8719244911,1652.87166050182,1653.87139651254,1654.87113252326,1655.87086853399,
1656.8706045447,1657.87034055543,1658.87007656615,1659.86981257687,1660.86954858759,
1661.86928459831,1662.86902060903,1663.86875661975,1664.86849263047,1665.86822864119,
1666.86796465191,1667.86770066263,1668.86743667335,1669.86717268407,1670.86690869479,
1671.86664470551,1672.86638071623,1673.86611672695,1674.86585273767,1675.86558874839,
1676.86532475911,1677.86506076983,1678.86479678055,1679.86453279127,1680.86426880199,
1681.86400481271,1682.86374082343,1683.86347683415,1684.86321284487,1685.86294885559,
1686.86268486631,1687.86242087703,1688.86215688775,1689.86189289847,1690.86162890919,
1691.86136491991,1692.86110093063,1693.86083694135,1694.86057295207,1695.86030896279,
1696.86004497351,1697.35991297887,1697.85988790214),.UNSPECIFIED.);
#54=B_SPLINE_SURFACE_WITH_KNOTS('',3,3,((#254642,#254643,#254644,#254645,
#254646,#254647,#254648,#254649,#254650,#254651,#254652,#254653,#254654,
#254655,#254656,#254657,#254658,#254659,#254660,#254661,#254662,#254663,
#254664,#254665,#254666,#254667,#254668,#254669,#254670,#254671,#254672,
#254673,#254674,#254675,#254676,#254677,#254678,#254679,#254680,#254681,
#254682,#254683,#254684,#254685,#254686,#254687,#254688,#254689,#254690,
#254691,#254692,#254693,#254694,#254695,#254696,#254697,#254698,#254699,
#254700,#254701,#254702,#254703,#254704,#254705,#254706,#254707,#254708,
#254709,#254710,#254711,#254712,#254713,#254714,#254715,#254716,#254717,
#254718,#254719,#254720,#254721,#254722,#254723,#254724,#254725,#254726,
#254727,#254728,#254729,#254730,#254731,#254732,#254733,#254734,#254735,
#254736,#254737,#254738,#254739,#254740,#254741,#254742,#254743,#254744,
#254745,#254746,#254747,#254748,#254749,#254750,#254751,#254752,#254753,
#254754,#254755,#254756,#254757,#254758,#254759,#254760,#254761,#254762,
#254763,#254764,#254765,#254766,#254767,#254768,#254769,#254770,#254771,
#254772,#254773,#254774,#254775,#254776,#254777,#254778,#254779,#254780,
#254781,#254782,#254783,#254784,#254785,#254786,#254787,#254788,#254789,
#254790,#254791,#254792,#254793,#254794,#254795,#254796,#254797,#254798,
#254799,#254800,#254801,#254802,#254803,#254804,#254805,#254806,#254807,
#254808,#254809,#254810,#254811,#254812,#254813,#254814,#254815,#254816,
#254817,#254818,#254819,#254820,#254821,#254822,#254823,#254824,#254825,
#254826,#254827,#254828,#254829,#254830,#254831,#254832,#254833,#254834,
#254835,#254836,#254837,#254838,#254839,#254840,#254841,#254842,#254843,
#254844,#254845,#254846,#254847,#254848,#254849,#254850,#254851,#254852,
#254853,#254854,#254855,#254856,#254857,#254858,#254859,#254860,#254861,
#254862,#254863,#254864,#254865,#254866,#254867,#254868,#254869,#254870,
#254871,#254872,#254873,#254874,#254875,#254876,#254877,#254878,#254879,
#254880,#254881,#254882,#254883,#254884,#254885,#254886,#254887,#254888,
#254889,#254890,#254891,#254892,#254893,#254894,#254895,#254896,#254897,
#254898,#254899,#254900,#254901,#254902,#254903,#254904,#254905,#254906,
#254907,#254908,#254909,#254910,#254911,#254912,#254913,#254914,#254915,
#254916,#254917,#254918,#254919,#254920,#254921,#254922,#254923,#254924,
#254925,#254926,#254927,#254928,#254929,#254930,#254931,#254932,#254933,
#254934,#254935,#254936,#254937,#254938,#254939,#254940,#254941,#254942,
#254943,#254944,#254945,#254946,#254947,#254948,#254949,#254950,#254951,
#254952,#254953,#254954,#254955,#254956,#254957,#254958,#254959,#254960,
#254961,#254962,#254963,#254964,#254965,#254966,#254967,#254968,#254969,
#254970,#254971,#254972,#254973,#254974,#254975,#254976,#254977,#254978,
#254979,#254980,#254981,#254982,#254983,#254984,#254985,#254986,#254987,
#254988,#254989,#254990,#254991,#254992,#254993,#254994,#254995,#254996,
#254997,#254998,#254999,#255000,#255001,#255002,#255003,#255004,#255005,
#255006,#255007,#255008,#255009,#255010,#255011,#255012,#255013,#255014,
#255015,#255016,#255017,#255018,#255019,#255020,#255021,#255022,#255023,
#255024,#255025,#255026,#255027,#255028,#255029,#255030,#255031,#255032,
#255033,#255034,#255035,#255036,#255037,#255038,#255039,#255040,#255041,
#255042,#255043,#255044,#255045,#255046,#255047,#255048,#255049,#255050,
#255051,#255052,#255053,#255054,#255055,#255056,#255057,#255058,#255059,
#255060,#255061,#255062,#255063,#255064,#255065,#255066,#255067,#255068,
#255069,#255070,#255071,#255072,#255073,#255074,#255075,#255076,#255077,
#255078,#255079,#255080,#255081,#255082,#255083,#255084,#255085,#255086,
#255087,#255088,#255089,#255090,#255091,#255092,#255093,#255094,#255095,
#255096,#255097,#255098,#255099,#255100,#255101,#255102,#255103,#255104,
#255105,#255106,#255107,#255108,#255109,#255110,#255111,#255112,#255113,
#255114,#255115,#255116,#255117,#255118,#255119,#255120,#255121,#255122,
#255123,#255124,#255125,#255126,#255127,#255128,#255129,#255130,#255131,
#255132,#255133,#255134,#255135,#255136,#255137,#255138,#255139,#255140,
#255141,#255142,#255143,#255144,#255145,#255146,#255147,#255148,#255149,
#255150,#255151,#255152,#255153,#255154,#255155,#255156,#255157,#255158,
#255159,#255160,#255161,#255162,#255163,#255164,#255165,#255166,#255167,
#255168,#255169,#255170,#255171,#255172,#255173,#255174,#255175,#255176,
#255177,#255178,#255179,#255180,#255181,#255182,#255183,#255184,#255185,
#255186,#255187,#255188,#255189,#255190,#255191,#255192,#255193,#255194,
#255195,#255196,#255197,#255198,#255199,#255200,#255201,#255202,#255203,
#255204,#255205,#255206,#255207,#255208,#255209,#255210,#255211,#255212,
#255213,#255214,#255215,#255216,#255217,#255218,#255219,#255220,#255221,
#255222,#255223,#255224,#255225,#255226,#255227,#255228,#255229,#255230,
#255231,#255232,#255233,#255234,#255235,#255236,#255237,#255238,#255239,
#255240,#255241,#255242,#255243,#255244,#255245,#255246,#255247,#255248,
#255249,#255250,#255251,#255252,#255253,#255254,#255255,#255256,#255257,
#255258,#255259,#255260,#255261,#255262,#255263,#255264,#255265,#255266,
#255267,#255268,#255269,#255270,#255271,#255272,#255273,#255274,#255275,
#255276,#255277,#255278,#255279,#255280,#255281,#255282,#255283,#255284,
#255285,#255286,#255287,#255288,#255289,#255290,#255291,#255292,#255293,
#255294,#255295,#255296,#255297,#255298,#255299,#255300,#255301,#255302,
#255303,#255304,#255305,#255306,#255307,#255308,#255309,#255310,#255311,
#255312,#255313,#255314,#255315,#255316,#255317,#255318,#255319,#255320,
#255321,#255322,#255323,#255324,#255325,#255326,#255327,#255328,#255329,
#255330,#255331,#255332,#255333,#255334,#255335,#255336,#255337,#255338,
#255339,#255340,#255341,#255342,#255343,#255344,#255345,#255346,#255347,
#255348,#255349,#255350,#255351,#255352,#255353,#255354,#255355,#255356,
#255357,#255358,#255359,#255360,#255361,#255362,#255363,#255364,#255365,
#255366,#255367,#255368,#255369,#255370,#255371,#255372,#255373,#255374,
#255375,#255376,#255377,#255378,#255379,#255380,#255381,#255382,#255383,
#255384,#255385,#255386,#255387,#255388,#255389,#255390,#255391,#255392,
#255393,#255394,#255395,#255396,#255397,#255398,#255399,#255400,#255401,
#255402,#255403,#255404,#255405,#255406,#255407,#255408,#255409,#255410,
#255411,#255412,#255413,#255414,#255415,#255416,#255417,#255418,#255419,
#255420,#255421,#255422,#255423,#255424,#255425,#255426,#255427,#255428,
#255429,#255430,#255431,#255432,#255433,#255434,#255435,#255436,#255437,
#255438,#255439,#255440,#255441,#255442,#255443,#255444,#255445,#255446,
#255447,#255448,#255449,#255450,#255451,#255452,#255453,#255454,#255455,
#255456,#255457,#255458,#255459,#255460,#255461,#255462,#255463,#255464,
#255465,#255466,#255467,#255468,#255469,#255470,#255471,#255472,#255473,
#255474,#255475,#255476,#255477,#255478,#255479,#255480,#255481,#255482,
#255483,#255484,#255485,#255486,#255487,#255488,#255489,#255490,#255491,
#255492,#255493,#255494,#255495,#255496,#255497,#255498,#255499,#255500,
#255501,#255502,#255503,#255504,#255505,#255506,#255507,#255508,#255509,
#255510,#255511,#255512,#255513,#255514,#255515,#255516,#255517,#255518,
#255519,#255520,#255521,#255522,#255523,#255524,#255525,#255526,#255527,
#255528,#255529,#255530,#255531,#255532,#255533,#255534,#255535,#255536,
#255537,#255538,#255539,#255540,#255541,#255542,#255543,#255544,#255545,
#255546,#255547,#255548,#255549,#255550,#255551,#255552,#255553,#255554,
#255555,#255556,#255557,#255558,#255559,#255560,#255561,#255562,#255563,
#255564,#255565,#255566,#255567,#255568,#255569,#255570,#255571,#255572,
#255573,#255574,#255575,#255576,#255577,#255578,#255579,#255580,#255581,
#255582,#255583,#255584,#255585,#255586,#255587,#255588,#255589,#255590,
#255591,#255592,#255593,#255594,#255595,#255596,#255597,#255598,#255599,
#255600,#255601,#255602,#255603,#255604,#255605,#255606,#255607,#255608,
#255609,#255610,#255611,#255612,#255613,#255614,#255615,#255616,#255617,
#255618,#255619,#255620,#255621,#255622,#255623,#255624,#255625,#255626,
#255627,#255628,#255629,#255630,#255631,#255632,#255633,#255634,#255635,
#255636,#255637,#255638,#255639,#255640,#255641,#255642,#255643,#255644,
#255645,#255646,#255647,#255648,#255649,#255650,#255651,#255652,#255653,
#255654,#255655,#255656,#255657,#255658,#255659,#255660,#255661,#255662,
#255663,#255664,#255665,#255666,#255667,#255668,#255669,#255670,#255671,
#255672,#255673,#255674,#255675,#255676,#255677,#255678,#255679,#255680,
#255681,#255682,#255683,#255684,#255685,#255686,#255687,#255688,#255689,
#255690,#255691,#255692,#255693,#255694,#255695,#255696,#255697,#255698,
#255699,#255700,#255701,#255702,#255703,#255704,#255705,#255706,#255707,
#255708,#255709,#255710,#255711,#255712,#255713,#255714,#255715,#255716,
#255717,#255718,#255719,#255720,#255721,#255722,#255723,#255724,#255725,
#255726,#255727,#255728,#255729,#255730,#255731,#255732,#255733,#255734,
#255735,#255736,#255737,#255738,#255739,#255740,#255741,#255742,#255743,
#255744,#255745,#255746,#255747,#255748,#255749,#255750,#255751,#255752,
#255753,#255754,#255755,#255756,#255757,#255758,#255759,#255760,#255761,
#255762,#255763,#255764,#255765,#255766,#255767,#255768,#255769,#255770,
#255771,#255772,#255773,#255774,#255775,#255776,#255777,#255778,#255779,
#255780,#255781,#255782,#255783,#255784,#255785,#255786,#255787,#255788,
#255789,#255790,#255791,#255792,#255793,#255794,#255795,#255796,#255797,
#255798,#255799,#255800,#255801,#255802,#255803,#255804,#255805,#255806,
#255807,#255808,#255809,#255810,#255811,#255812,#255813,#255814,#255815,
#255816,#255817,#255818,#255819,#255820,#255821,#255822,#255823,#255824,
#255825,#255826,#255827,#255828,#255829,#255830,#255831,#255832,#255833,
#255834,#255835,#255836,#255837,#255838,#255839,#255840,#255841,#255842,
#255843,#255844,#255845,#255846,#255847,#255848,#255849,#255850,#255851,
#255852,#255853,#255854,#255855,#255856,#255857,#255858,#255859,#255860,
#255861,#255862,#255863,#255864,#255865,#255866,#255867,#255868,#255869,
#255870,#255871,#255872,#255873,#255874,#255875,#255876,#255877,#255878,
#255879,#255880,#255881,#255882,#255883,#255884,#255885,#255886,#255887,
#255888,#255889,#255890,#255891,#255892,#255893,#255894,#255895,#255896,
#255897,#255898,#255899,#255900,#255901,#255902,#255903,#255904,#255905,
#255906,#255907,#255908,#255909,#255910,#255911,#255912,#255913,#255914,
#255915,#255916,#255917,#255918,#255919,#255920,#255921,#255922,#255923,
#255924,#255925,#255926,#255927,#255928,#255929,#255930,#255931,#255932,
#255933,#255934,#255935,#255936,#255937,#255938,#255939,#255940,#255941,
#255942,#255943,#255944,#255945,#255946,#255947,#255948,#255949,#255950,
#255951,#255952,#255953,#255954,#255955,#255956,#255957,#255958,#255959,
#255960,#255961,#255962,#255963,#255964,#255965,#255966,#255967,#255968,
#255969,#255970,#255971,#255972,#255973,#255974,#255975,#255976,#255977,
#255978,#255979,#255980,#255981,#255982,#255983,#255984,#255985,#255986,
#255987,#255988,#255989,#255990,#255991,#255992,#255993,#255994,#255995,
#255996,#255997,#255998,#255999,#256000,#256001,#256002,#256003,#256004,
#256005,#256006,#256007,#256008,#256009,#256010,#256011,#256012,#256013,
#256014,#256015,#256016,#256017,#256018,#256019,#256020,#256021,#256022,
#256023,#256024,#256025,#256026,#256027,#256028,#256029,#256030,#256031,
#256032,#256033,#256034,#256035,#256036,#256037,#256038,#256039,#256040,
#256041,#256042,#256043,#256044,#256045,#256046,#256047,#256048,#256049,
#256050,#256051,#256052,#256053,#256054,#256055,#256056,#256057,#256058,
#256059,#256060,#256061,#256062,#256063,#256064,#256065,#256066,#256067,
#256068,#256069,#256070,#256071,#256072,#256073,#256074,#256075,#256076,
#256077,#256078,#256079,#256080,#256081,#256082,#256083,#256084,#256085,
#256086,#256087,#256088,#256089,#256090,#256091,#256092,#256093,#256094,
#256095,#256096,#256097,#256098,#256099,#256100,#256101,#256102,#256103,
#256104,#256105,#256106,#256107,#256108,#256109,#256110,#256111,#256112,
#256113,#256114,#256115,#256116,#256117,#256118,#256119,#256120,#256121,
#256122,#256123,#256124,#256125,#256126,#256127,#256128,#256129,#256130,
#256131,#256132,#256133,#256134,#256135,#256136,#256137,#256138,#256139,
#256140,#256141,#256142,#256143,#256144,#256145,#256146,#256147,#256148,
#256149,#256150,#256151,#256152,#256153,#256154,#256155,#256156,#256157,
#256158,#256159,#256160,#256161,#256162,#256163,#256164,#256165,#256166,
#256167,#256168,#256169,#256170,#256171,#256172,#256173,#256174,#256175,
#256176,#256177,#256178,#256179,#256180,#256181,#256182,#256183,#256184,
#256185,#256186,#256187,#256188,#256189,#256190,#256191,#256192,#256193,
#256194,#256195,#256196,#256197,#256198,#256199,#256200,#256201,#256202,
#256203,#256204,#256205,#256206,#256207,#256208,#256209,#256210,#256211,
#256212,#256213,#256214,#256215,#256216,#256217,#256218,#256219,#256220,
#256221,#256222,#256223,#256224,#256225,#256226,#256227,#256228,#256229,
#256230,#256231,#256232,#256233,#256234,#256235,#256236,#256237,#256238,
#256239,#256240,#256241,#256242,#256243,#256244,#256245,#256246,#256247,
#256248,#256249,#256250,#256251,#256252,#256253,#256254,#256255,#256256,
#256257,#256258,#256259,#256260,#256261,#256262,#256263,#256264,#256265,
#256266,#256267,#256268,#256269,#256270,#256271,#256272,#256273,#256274,
#256275,#256276,#256277,#256278,#256279,#256280,#256281,#256282,#256283,
#256284,#256285,#256286,#256287,#256288,#256289,#256290,#256291,#256292,
#256293,#256294,#256295,#256296,#256297,#256298,#256299,#256300,#256301,
#256302,#256303,#256304,#256305,#256306,#256307,#256308,#256309,#256310,
#256311,#256312,#256313,#256314,#256315,#256316,#256317,#256318,#256319,
#256320,#256321,#256322,#256323,#256324,#256325,#256326,#256327,#256328,
#256329,#256330,#256331,#256332,#256333,#256334,#256335,#256336),(#256337,
#256338,#256339,#256340,#256341,#256342,#256343,#256344,#256345,#256346,
#256347,#256348,#256349,#256350,#256351,#256352,#256353,#256354,#256355,
#256356,#256357,#256358,#256359,#256360,#256361,#256362,#256363,#256364,
#256365,#256366,#256367,#256368,#256369,#256370,#256371,#256372,#256373,
#256374,#256375,#256376,#256377,#256378,#256379,#256380,#256381,#256382,
#256383,#256384,#256385,#256386,#256387,#256388,#256389,#256390,#256391,
#256392,#256393,#256394,#256395,#256396,#256397,#256398,#256399,#256400,
#256401,#256402,#256403,#256404,#256405,#256406,#256407,#256408,#256409,
#256410,#256411,#256412,#256413,#256414,#256415,#256416,#256417,#256418,
#256419,#256420,#256421,#256422,#256423,#256424,#256425,#256426,#256427,
#256428,#256429,#256430,#256431,#256432,#256433,#256434,#256435,#256436,
#256437,#256438,#256439,#256440,#256441,#256442,#256443,#256444,#256445,
#256446,#256447,#256448,#256449,#256450,#256451,#256452,#256453,#256454,
#256455,#256456,#256457,#256458,#256459,#256460,#256461,#256462,#256463,
#256464,#256465,#256466,#256467,#256468,#256469,#256470,#256471,#256472,
#256473,#256474,#256475,#256476,#256477,#256478,#256479,#256480,#256481,
#256482,#256483,#256484,#256485,#256486,#256487,#256488,#256489,#256490,
#256491,#256492,#256493,#256494,#256495,#256496,#256497,#256498,#256499,
#256500,#256501,#256502,#256503,#256504,#256505,#256506,#256507,#256508,
#256509,#256510,#256511,#256512,#256513,#256514,#256515,#256516,#256517,
#256518,#256519,#256520,#256521,#256522,#256523,#256524,#256525,#256526,
#256527,#256528,#256529,#256530,#256531,#256532,#256533,#256534,#256535,
#256536,#256537,#256538,#256539,#256540,#256541,#256542,#256543,#256544,
#256545,#256546,#256547,#256548,#256549,#256550,#256551,#256552,#256553,
#256554,#256555,#256556,#256557,#256558,#256559,#256560,#256561,#256562,
#256563,#256564,#256565,#256566,#256567,#256568,#256569,#256570,#256571,
#256572,#256573,#256574,#256575,#256576,#256577,#256578,#256579,#256580,
#256581,#256582,#256583,#256584,#256585,#256586,#256587,#256588,#256589,
#256590,#256591,#256592,#256593,#256594,#256595,#256596,#256597,#256598,
#256599,#256600,#256601,#256602,#256603,#256604,#256605,#256606,#256607,
#256608,#256609,#256610,#256611,#256612,#256613,#256614,#256615,#256616,
#256617,#256618,#256619,#256620,#256621,#256622,#256623,#256624,#256625,
#256626,#256627,#256628,#256629,#256630,#256631,#256632,#256633,#256634,
#256635,#256636,#256637,#256638,#256639,#256640,#256641,#256642,#256643,
#256644,#256645,#256646,#256647,#256648,#256649,#256650,#256651,#256652,
#256653,#256654,#256655,#256656,#256657,#256658,#256659,#256660,#256661,
#256662,#256663,#256664,#256665,#256666,#256667,#256668,#256669,#256670,
#256671,#256672,#256673,#256674,#256675,#256676,#256677,#256678,#256679,
#256680,#256681,#256682,#256683,#256684,#256685,#256686,#256687,#256688,
#256689,#256690,#256691,#256692,#256693,#256694,#256695,#256696,#256697,
#256698,#256699,#256700,#256701,#256702,#256703,#256704,#256705,#256706,
#256707,#256708,#256709,#256710,#256711,#256712,#256713,#256714,#256715,
#256716,#256717,#256718,#256719,#256720,#256721,#256722,#256723,#256724,
#256725,#256726,#256727,#256728,#256729,#256730,#256731,#256732,#256733,
#256734,#256735,#256736,#256737,#256738,#256739,#256740,#256741,#256742,
#256743,#256744,#256745,#256746,#256747,#256748,#256749,#256750,#256751,
#256752,#256753,#256754,#256755,#256756,#256757,#256758,#256759,#256760,
#256761,#256762,#256763,#256764,#256765,#256766,#256767,#256768,#256769,
#256770,#256771,#256772,#256773,#256774,#256775,#256776,#256777,#256778,
#256779,#256780,#256781,#256782,#256783,#256784,#256785,#256786,#256787,
#256788,#256789,#256790,#256791,#256792,#256793,#256794,#256795,#256796,
#256797,#256798,#256799,#256800,#256801,#256802,#256803,#256804,#256805,
#256806,#256807,#256808,#256809,#256810,#256811,#256812,#256813,#256814,
#256815,#256816,#256817,#256818,#256819,#256820,#256821,#256822,#256823,
#256824,#256825,#256826,#256827,#256828,#256829,#256830,#256831,#256832,
#256833,#256834,#256835,#256836,#256837,#256838,#256839,#256840,#256841,
#256842,#256843,#256844,#256845,#256846,#256847,#256848,#256849,#256850,
#256851,#256852,#256853,#256854,#256855,#256856,#256857,#256858,#256859,
#256860,#256861,#256862,#256863,#256864,#256865,#256866,#256867,#256868,
#256869,#256870,#256871,#256872,#256873,#256874,#256875,#256876,#256877,
#256878,#256879,#256880,#256881,#256882,#256883,#256884,#256885,#256886,
#256887,#256888,#256889,#256890,#256891,#256892,#256893,#256894,#256895,
#256896,#256897,#256898,#256899,#256900,#256901,#256902,#256903,#256904,
#256905,#256906,#256907,#256908,#256909,#256910,#256911,#256912,#256913,
#256914,#256915,#256916,#256917,#256918,#256919,#256920,#256921,#256922,
#256923,#256924,#256925,#256926,#256927,#256928,#256929,#256930,#256931,
#256932,#256933,#256934,#256935,#256936,#256937,#256938,#256939,#256940,
#256941,#256942,#256943,#256944,#256945,#256946,#256947,#256948,#256949,
#256950,#256951,#256952,#256953,#256954,#256955,#256956,#256957,#256958,
#256959,#256960,#256961,#256962,#256963,#256964,#256965,#256966,#256967,
#256968,#256969,#256970,#256971,#256972,#256973,#256974,#256975,#256976,
#256977,#256978,#256979,#256980,#256981,#256982,#256983,#256984,#256985,
#256986,#256987,#256988,#256989,#256990,#256991,#256992,#256993,#256994,
#256995,#256996,#256997,#256998,#256999,#257000,#257001,#257002,#257003,
#257004,#257005,#257006,#257007,#257008,#257009,#257010,#257011,#257012,
#257013,#257014,#257015,#257016,#257017,#257018,#257019,#257020,#257021,
#257022,#257023,#257024,#257025,#257026,#257027,#257028,#257029,#257030,
#257031,#257032,#257033,#257034,#257035,#257036,#257037,#257038,#257039,
#257040,#257041,#257042,#257043,#257044,#257045,#257046,#257047,#257048,
#257049,#257050,#257051,#257052,#257053,#257054,#257055,#257056,#257057,
#257058,#257059,#257060,#257061,#257062,#257063,#257064,#257065,#257066,
#257067,#257068,#257069,#257070,#257071,#257072,#257073,#257074,#257075,
#257076,#257077,#257078,#257079,#257080,#257081,#257082,#257083,#257084,
#257085,#257086,#257087,#257088,#257089,#257090,#257091,#257092,#257093,
#257094,#257095,#257096,#257097,#257098,#257099,#257100,#257101,#257102,
#257103,#257104,#257105,#257106,#257107,#257108,#257109,#257110,#257111,
#257112,#257113,#257114,#257115,#257116,#257117,#257118,#257119,#257120,
#257121,#257122,#257123,#257124,#257125,#257126,#257127,#257128,#257129,
#257130,#257131,#257132,#257133,#257134,#257135,#257136,#257137,#257138,
#257139,#257140,#257141,#257142,#257143,#257144,#257145,#257146,#257147,
#257148,#257149,#257150,#257151,#257152,#257153,#257154,#257155,#257156,
#257157,#257158,#257159,#257160,#257161,#257162,#257163,#257164,#257165,
#257166,#257167,#257168,#257169,#257170,#257171,#257172,#257173,#257174,
#257175,#257176,#257177,#257178,#257179,#257180,#257181,#257182,#257183,
#257184,#257185,#257186,#257187,#257188,#257189,#257190,#257191,#257192,
#257193,#257194,#257195,#257196,#257197,#257198,#257199,#257200,#257201,
#257202,#257203,#257204,#257205,#257206,#257207,#257208,#257209,#257210,
#257211,#257212,#257213,#257214,#257215,#257216,#257217,#257218,#257219,
#257220,#257221,#257222,#257223,#257224,#257225,#257226,#257227,#257228,
#257229,#257230,#257231,#257232,#257233,#257234,#257235,#257236,#257237,
#257238,#257239,#257240,#257241,#257242,#257243,#257244,#257245,#257246,
#257247,#257248,#257249,#257250,#257251,#257252,#257253,#257254,#257255,
#257256,#257257,#257258,#257259,#257260,#257261,#257262,#257263,#257264,
#257265,#257266,#257267,#257268,#257269,#257270,#257271,#257272,#257273,
#257274,#257275,#257276,#257277,#257278,#257279,#257280,#257281,#257282,
#257283,#257284,#257285,#257286,#257287,#257288,#257289,#257290,#257291,
#257292,#257293,#257294,#257295,#257296,#257297,#257298,#257299,#257300,
#257301,#257302,#257303,#257304,#257305,#257306,#257307,#257308,#257309,
#257310,#257311,#257312,#257313,#257314,#257315,#257316,#257317,#257318,
#257319,#257320,#257321,#257322,#257323,#257324,#257325,#257326,#257327,
#257328,#257329,#257330,#257331,#257332,#257333,#257334,#257335,#257336,
#257337,#257338,#257339,#257340,#257341,#257342,#257343,#257344,#257345,
#257346,#257347,#257348,#257349,#257350,#257351,#257352,#257353,#257354,
#257355,#257356,#257357,#257358,#257359,#257360,#257361,#257362,#257363,
#257364,#257365,#257366,#257367,#257368,#257369,#257370,#257371,#257372,
#257373,#257374,#257375,#257376,#257377,#257378,#257379,#257380,#257381,
#257382,#257383,#257384,#257385,#257386,#257387,#257388,#257389,#257390,
#257391,#257392,#257393,#257394,#257395,#257396,#257397,#257398,#257399,
#257400,#257401,#257402,#257403,#257404,#257405,#257406,#257407,#257408,
#257409,#257410,#257411,#257412,#257413,#257414,#257415,#257416,#257417,
#257418,#257419,#257420,#257421,#257422,#257423,#257424,#257425,#257426,
#257427,#257428,#257429,#257430,#257431,#257432,#257433,#257434,#257435,
#257436,#257437,#257438,#257439,#257440,#257441,#257442,#257443,#257444,
#257445,#257446,#257447,#257448,#257449,#257450,#257451,#257452,#257453,
#257454,#257455,#257456,#257457,#257458,#257459,#257460,#257461,#257462,
#257463,#257464,#257465,#257466,#257467,#257468,#257469,#257470,#257471,
#257472,#257473,#257474,#257475,#257476,#257477,#257478,#257479,#257480,
#257481,#257482,#257483,#257484,#257485,#257486,#257487,#257488,#257489,
#257490,#257491,#257492,#257493,#257494,#257495,#257496,#257497,#257498,
#257499,#257500,#257501,#257502,#257503,#257504,#257505,#257506,#257507,
#257508,#257509,#257510,#257511,#257512,#257513,#257514,#257515,#257516,
#257517,#257518,#257519,#257520,#257521,#257522,#257523,#257524,#257525,
#257526,#257527,#257528,#257529,#257530,#257531,#257532,#257533,#257534,
#257535,#257536,#257537,#257538,#257539,#257540,#257541,#257542,#257543,
#257544,#257545,#257546,#257547,#257548,#257549,#257550,#257551,#257552,
#257553,#257554,#257555,#257556,#257557,#257558,#257559,#257560,#257561,
#257562,#257563,#257564,#257565,#257566,#257567,#257568,#257569,#257570,
#257571,#257572,#257573,#257574,#257575,#257576,#257577,#257578,#257579,
#257580,#257581,#257582,#257583,#257584,#257585,#257586,#257587,#257588,
#257589,#257590,#257591,#257592,#257593,#257594,#257595,#257596,#257597,
#257598,#257599,#257600,#257601,#257602,#257603,#257604,#257605,#257606,
#257607,#257608,#257609,#257610,#257611,#257612,#257613,#257614,#257615,
#257616,#257617,#257618,#257619,#257620,#257621,#257622,#257623,#257624,
#257625,#257626,#257627,#257628,#257629,#257630,#257631,#257632,#257633,
#257634,#257635,#257636,#257637,#257638,#257639,#257640,#257641,#257642,
#257643,#257644,#257645,#257646,#257647,#257648,#257649,#257650,#257651,
#257652,#257653,#257654,#257655,#257656,#257657,#257658,#257659,#257660,
#257661,#257662,#257663,#257664,#257665,#257666,#257667,#257668,#257669,
#257670,#257671,#257672,#257673,#257674,#257675,#257676,#257677,#257678,
#257679,#257680,#257681,#257682,#257683,#257684,#257685,#257686,#257687,
#257688,#257689,#257690,#257691,#257692,#257693,#257694,#257695,#257696,
#257697,#257698,#257699,#257700,#257701,#257702,#257703,#257704,#257705,
#257706,#257707,#257708,#257709,#257710,#257711,#257712,#257713,#257714,
#257715,#257716,#257717,#257718,#257719,#257720,#257721,#257722,#257723,
#257724,#257725,#257726,#257727,#257728,#257729,#257730,#257731,#257732,
#257733,#257734,#257735,#257736,#257737,#257738,#257739,#257740,#257741,
#257742,#257743,#257744,#257745,#257746,#257747,#257748,#257749,#257750,
#257751,#257752,#257753,#257754,#257755,#257756,#257757,#257758,#257759,
#257760,#257761,#257762,#257763,#257764,#257765,#257766,#257767,#257768,
#257769,#257770,#257771,#257772,#257773,#257774,#257775,#257776,#257777,
#257778,#257779,#257780,#257781,#257782,#257783,#257784,#257785,#257786,
#257787,#257788,#257789,#257790,#257791,#257792,#257793,#257794,#257795,
#257796,#257797,#257798,#257799,#257800,#257801,#257802,#257803,#257804,
#257805,#257806,#257807,#257808,#257809,#257810,#257811,#257812,#257813,
#257814,#257815,#257816,#257817,#257818,#257819,#257820,#257821,#257822,
#257823,#257824,#257825,#257826,#257827,#257828,#257829,#257830,#257831,
#257832,#257833,#257834,#257835,#257836,#257837,#257838,#257839,#257840,
#257841,#257842,#257843,#257844,#257845,#257846,#257847,#257848,#257849,
#257850,#257851,#257852,#257853,#257854,#257855,#257856,#257857,#257858,
#257859,#257860,#257861,#257862,#257863,#257864,#257865,#257866,#257867,
#257868,#257869,#257870,#257871,#257872,#257873,#257874,#257875,#257876,
#257877,#257878,#257879,#257880,#257881,#257882,#257883,#257884,#257885,
#257886,#257887,#257888,#257889,#257890,#257891,#257892,#257893,#257894,
#257895,#257896,#257897,#257898,#257899,#257900,#257901,#257902,#257903,
#257904,#257905,#257906,#257907,#257908,#257909,#257910,#257911,#257912,
#257913,#257914,#257915,#257916,#257917,#257918,#257919,#257920,#257921,
#257922,#257923,#257924,#257925,#257926,#257927,#257928,#257929,#257930,
#257931,#257932,#257933,#257934,#257935,#257936,#257937,#257938,#257939,
#257940,#257941,#257942,#257943,#257944,#257945,#257946,#257947,#257948,
#257949,#257950,#257951,#257952,#257953,#257954,#257955,#257956,#257957,
#257958,#257959,#257960,#257961,#257962,#257963,#257964,#257965,#257966,
#257967,#257968,#257969,#257970,#257971,#257972,#257973,#257974,#257975,
#257976,#257977,#257978,#257979,#257980,#257981,#257982,#257983,#257984,
#257985,#257986,#257987,#257988,#257989,#257990,#257991,#257992,#257993,
#257994,#257995,#257996,#257997,#257998,#257999,#258000,#258001,#258002,
#258003,#258004,#258005,#258006,#258007,#258008,#258009,#258010,#258011,
#258012,#258013,#258014,#258015,#258016,#258017,#258018,#258019,#258020,
#258021,#258022,#258023,#258024,#258025,#258026,#258027,#258028,#258029,
#258030,#258031),(#258032,#258033,#258034,#258035,#258036,#258037,#258038,
#258039,#258040,#258041,#258042,#258043,#258044,#258045,#258046,#258047,
#258048,#258049,#258050,#258051,#258052,#258053,#258054,#258055,#258056,
#258057,#258058,#258059,#258060,#258061,#258062,#258063,#258064,#258065,
#258066,#258067,#258068,#258069,#258070,#258071,#258072,#258073,#258074,
#258075,#258076,#258077,#258078,#258079,#258080,#258081,#258082,#258083,
#258084,#258085,#258086,#258087,#258088,#258089,#258090,#258091,#258092,
#258093,#258094,#258095,#258096,#258097,#258098,#258099,#258100,#258101,
#258102,#258103,#258104,#258105,#258106,#258107,#258108,#258109,#258110,
#258111,#258112,#258113,#258114,#258115,#258116,#258117,#258118,#258119,
#258120,#258121,#258122,#258123,#258124,#258125,#258126,#258127,#258128,
#258129,#258130,#258131,#258132,#258133,#258134,#258135,#258136,#258137,
#258138,#258139,#258140,#258141,#258142,#258143,#258144,#258145,#258146,
#258147,#258148,#258149,#258150,#258151,#258152,#258153,#258154,#258155,
#258156,#258157,#258158,#258159,#258160,#258161,#258162,#258163,#258164,
#258165,#258166,#258167,#258168,#258169,#258170,#258171,#258172,#258173,
#258174,#258175,#258176,#258177,#258178,#258179,#258180,#258181,#258182,
#258183,#258184,#258185,#258186,#258187,#258188,#258189,#258190,#258191,
#258192,#258193,#258194,#258195,#258196,#258197,#258198,#258199,#258200,
#258201,#258202,#258203,#258204,#258205,#258206,#258207,#258208,#258209,
#258210,#258211,#258212,#258213,#258214,#258215,#258216,#258217,#258218,
#258219,#258220,#258221,#258222,#258223,#258224,#258225,#258226,#258227,
#258228,#258229,#258230,#258231,#258232,#258233,#258234,#258235,#258236,
#258237,#258238,#258239,#258240,#258241,#258242,#258243,#258244,#258245,
#258246,#258247,#258248,#258249,#258250,#258251,#258252,#258253,#258254,
#258255,#258256,#258257,#258258,#258259,#258260,#258261,#258262,#258263,
#258264,#258265,#258266,#258267,#258268,#258269,#258270,#258271,#258272,
#258273,#258274,#258275,#258276,#258277,#258278,#258279,#258280,#258281,
#258282,#258283,#258284,#258285,#258286,#258287,#258288,#258289,#258290,
#258291,#258292,#258293,#258294,#258295,#258296,#258297,#258298,#258299,
#258300,#258301,#258302,#258303,#258304,#258305,#258306,#258307,#258308,
#258309,#258310,#258311,#258312,#258313,#258314,#258315,#258316,#258317,
#258318,#258319,#258320,#258321,#258322,#258323,#258324,#258325,#258326,
#258327,#258328,#258329,#258330,#258331,#258332,#258333,#258334,#258335,
#258336,#258337,#258338,#258339,#258340,#258341,#258342,#258343,#258344,
#258345,#258346,#258347,#258348,#258349,#258350,#258351,#258352,#258353,
#258354,#258355,#258356,#258357,#258358,#258359,#258360,#258361,#258362,
#258363,#258364,#258365,#258366,#258367,#258368,#258369,#258370,#258371,
#258372,#258373,#258374,#258375,#258376,#258377,#258378,#258379,#258380,
#258381,#258382,#258383,#258384,#258385,#258386,#258387,#258388,#258389,
#258390,#258391,#258392,#258393,#258394,#258395,#258396,#258397,#258398,
#258399,#258400,#258401,#258402,#258403,#258404,#258405,#258406,#258407,
#258408,#258409,#258410,#258411,#258412,#258413,#258414,#258415,#258416,
#258417,#258418,#258419,#258420,#258421,#258422,#258423,#258424,#258425,
#258426,#258427,#258428,#258429,#258430,#258431,#258432,#258433,#258434,
#258435,#258436,#258437,#258438,#258439,#258440,#258441,#258442,#258443,
#258444,#258445,#258446,#258447,#258448,#258449,#258450,#258451,#258452,
#258453,#258454,#258455,#258456,#258457,#258458,#258459,#258460,#258461,
#258462,#258463,#258464,#258465,#258466,#258467,#258468,#258469,#258470,
#258471,#258472,#258473,#258474,#258475,#258476,#258477,#258478,#258479,
#258480,#258481,#258482,#258483,#258484,#258485,#258486,#258487,#258488,
#258489,#258490,#258491,#258492,#258493,#258494,#258495,#258496,#258497,
#258498,#258499,#258500,#258501,#258502,#258503,#258504,#258505,#258506,
#258507,#258508,#258509,#258510,#258511,#258512,#258513,#258514,#258515,
#258516,#258517,#258518,#258519,#258520,#258521,#258522,#258523,#258524,
#258525,#258526,#258527,#258528,#258529,#258530,#258531,#258532,#258533,
#258534,#258535,#258536,#258537,#258538,#258539,#258540,#258541,#258542,
#258543,#258544,#258545,#258546,#258547,#258548,#258549,#258550,#258551,
#258552,#258553,#258554,#258555,#258556,#258557,#258558,#258559,#258560,
#258561,#258562,#258563,#258564,#258565,#258566,#258567,#258568,#258569,
#258570,#258571,#258572,#258573,#258574,#258575,#258576,#258577,#258578,
#258579,#258580,#258581,#258582,#258583,#258584,#258585,#258586,#258587,
#258588,#258589,#258590,#258591,#258592,#258593,#258594,#258595,#258596,
#258597,#258598,#258599,#258600,#258601,#258602,#258603,#258604,#258605,
#258606,#258607,#258608,#258609,#258610,#258611,#258612,#258613,#258614,
#258615,#258616,#258617,#258618,#258619,#258620,#258621,#258622,#258623,
#258624,#258625,#258626,#258627,#258628,#258629,#258630,#258631,#258632,
#258633,#258634,#258635,#258636,#258637,#258638,#258639,#258640,#258641,
#258642,#258643,#258644,#258645,#258646,#258647,#258648,#258649,#258650,
#258651,#258652,#258653,#258654,#258655,#258656,#258657,#258658,#258659,
#258660,#258661,#258662,#258663,#258664,#258665,#258666,#258667,#258668,
#258669,#258670,#258671,#258672,#258673,#258674,#258675,#258676,#258677,
#258678,#258679,#258680,#258681,#258682,#258683,#258684,#258685,#258686,
#258687,#258688,#258689,#258690,#258691,#258692,#258693,#258694,#258695,
#258696,#258697,#258698,#258699,#258700,#258701,#258702,#258703,#258704,
#258705,#258706,#258707,#258708,#258709,#258710,#258711,#258712,#258713,
#258714,#258715,#258716,#258717,#258718,#258719,#258720,#258721,#258722,
#258723,#258724,#258725,#258726,#258727,#258728,#258729,#258730,#258731,
#258732,#258733,#258734,#258735,#258736,#258737,#258738,#258739,#258740,
#258741,#258742,#258743,#258744,#258745,#258746,#258747,#258748,#258749,
#258750,#258751,#258752,#258753,#258754,#258755,#258756,#258757,#258758,
#258759,#258760,#258761,#258762,#258763,#258764,#258765,#258766,#258767,
#258768,#258769,#258770,#258771,#258772,#258773,#258774,#258775,#258776,
#258777,#258778,#258779,#258780,#258781,#258782,#258783,#258784,#258785,
#258786,#258787,#258788,#258789,#258790,#258791,#258792,#258793,#258794,
#258795,#258796,#258797,#258798,#258799,#258800,#258801,#258802,#258803,
#258804,#258805,#258806,#258807,#258808,#258809,#258810,#258811,#258812,
#258813,#258814,#258815,#258816,#258817,#258818,#258819,#258820,#258821,
#258822,#258823,#258824,#258825,#258826,#258827,#258828,#258829,#258830,
#258831,#258832,#258833,#258834,#258835,#258836,#258837,#258838,#258839,
#258840,#258841,#258842,#258843,#258844,#258845,#258846,#258847,#258848,
#258849,#258850,#258851,#258852,#258853,#258854,#258855,#258856,#258857,
#258858,#258859,#258860,#258861,#258862,#258863,#258864,#258865,#258866,
#258867,#258868,#258869,#258870,#258871,#258872,#258873,#258874,#258875,
#258876,#258877,#258878,#258879,#258880,#258881,#258882,#258883,#258884,
#258885,#258886,#258887,#258888,#258889,#258890,#258891,#258892,#258893,
#258894,#258895,#258896,#258897,#258898,#258899,#258900,#258901,#258902,
#258903,#258904,#258905,#258906,#258907,#258908,#258909,#258910,#258911,
#258912,#258913,#258914,#258915,#258916,#258917,#258918,#258919,#258920,
#258921,#258922,#258923,#258924,#258925,#258926,#258927,#258928,#258929,
#258930,#258931,#258932,#258933,#258934,#258935,#258936,#258937,#258938,
#258939,#258940,#258941,#258942,#258943,#258944,#258945,#258946,#258947,
#258948,#258949,#258950,#258951,#258952,#258953,#258954,#258955,#258956,
#258957,#258958,#258959,#258960,#258961,#258962,#258963,#258964,#258965,
#258966,#258967,#258968,#258969,#258970,#258971,#258972,#258973,#258974,
#258975,#258976,#258977,#258978,#258979,#258980,#258981,#258982,#258983,
#258984,#258985,#258986,#258987,#258988,#258989,#258990,#258991,#258992,
#258993,#258994,#258995,#258996,#258997,#258998,#258999,#259000,#259001,
#259002,#259003,#259004,#259005,#259006,#259007,#259008,#259009,#259010,
#259011,#259012,#259013,#259014,#259015,#259016,#259017,#259018,#259019,
#259020,#259021,#259022,#259023,#259024,#259025,#259026,#259027,#259028,
#259029,#259030,#259031,#259032,#259033,#259034,#259035,#259036,#259037,
#259038,#259039,#259040,#259041,#259042,#259043,#259044,#259045,#259046,
#259047,#259048,#259049,#259050,#259051,#259052,#259053,#259054,#259055,
#259056,#259057,#259058,#259059,#259060,#259061,#259062,#259063,#259064,
#259065,#259066,#259067,#259068,#259069,#259070,#259071,#259072,#259073,
#259074,#259075,#259076,#259077,#259078,#259079,#259080,#259081,#259082,
#259083,#259084,#259085,#259086,#259087,#259088,#259089,#259090,#259091,
#259092,#259093,#259094,#259095,#259096,#259097,#259098,#259099,#259100,
#259101,#259102,#259103,#259104,#259105,#259106,#259107,#259108,#259109,
#259110,#259111,#259112,#259113,#259114,#259115,#259116,#259117,#259118,
#259119,#259120,#259121,#259122,#259123,#259124,#259125,#259126,#259127,
#259128,#259129,#259130,#259131,#259132,#259133,#259134,#259135,#259136,
#259137,#259138,#259139,#259140,#259141,#259142,#259143,#259144,#259145,
#259146,#259147,#259148,#259149,#259150,#259151,#259152,#259153,#259154,
#259155,#259156,#259157,#259158,#259159,#259160,#259161,#259162,#259163,
#259164,#259165,#259166,#259167,#259168,#259169,#259170,#259171,#259172,
#259173,#259174,#259175,#259176,#259177,#259178,#259179,#259180,#259181,
#259182,#259183,#259184,#259185,#259186,#259187,#259188,#259189,#259190,
#259191,#259192,#259193,#259194,#259195,#259196,#259197,#259198,#259199,
#259200,#259201,#259202,#259203,#259204,#259205,#259206,#259207,#259208,
#259209,#259210,#259211,#259212,#259213,#259214,#259215,#259216,#259217,
#259218,#259219,#259220,#259221,#259222,#259223,#259224,#259225,#259226,
#259227,#259228,#259229,#259230,#259231,#259232,#259233,#259234,#259235,
#259236,#259237,#259238,#259239,#259240,#259241,#259242,#259243,#259244,
#259245,#259246,#259247,#259248,#259249,#259250,#259251,#259252,#259253,
#259254,#259255,#259256,#259257,#259258,#259259,#259260,#259261,#259262,
#259263,#259264,#259265,#259266,#259267,#259268,#259269,#259270,#259271,
#259272,#259273,#259274,#259275,#259276,#259277,#259278,#259279,#259280,
#259281,#259282,#259283,#259284,#259285,#259286,#259287,#259288,#259289,
#259290,#259291,#259292,#259293,#259294,#259295,#259296,#259297,#259298,
#259299,#259300,#259301,#259302,#259303,#259304,#259305,#259306,#259307,
#259308,#259309,#259310,#259311,#259312,#259313,#259314,#259315,#259316,
#259317,#259318,#259319,#259320,#259321,#259322,#259323,#259324,#259325,
#259326,#259327,#259328,#259329,#259330,#259331,#259332,#259333,#259334,
#259335,#259336,#259337,#259338,#259339,#259340,#259341,#259342,#259343,
#259344,#259345,#259346,#259347,#259348,#259349,#259350,#259351,#259352,
#259353,#259354,#259355,#259356,#259357,#259358,#259359,#259360,#259361,
#259362,#259363,#259364,#259365,#259366,#259367,#259368,#259369,#259370,
#259371,#259372,#259373,#259374,#259375,#259376,#259377,#259378,#259379,
#259380,#259381,#259382,#259383,#259384,#259385,#259386,#259387,#259388,
#259389,#259390,#259391,#259392,#259393,#259394,#259395,#259396,#259397,
#259398,#259399,#259400,#259401,#259402,#259403,#259404,#259405,#259406,
#259407,#259408,#259409,#259410,#259411,#259412,#259413,#259414,#259415,
#259416,#259417,#259418,#259419,#259420,#259421,#259422,#259423,#259424,
#259425,#259426,#259427,#259428,#259429,#259430,#259431,#259432,#259433,
#259434,#259435,#259436,#259437,#259438,#259439,#259440,#259441,#259442,
#259443,#259444,#259445,#259446,#259447,#259448,#259449,#259450,#259451,
#259452,#259453,#259454,#259455,#259456,#259457,#259458,#259459,#259460,
#259461,#259462,#259463,#259464,#259465,#259466,#259467,#259468,#259469,
#259470,#259471,#259472,#259473,#259474,#259475,#259476,#259477,#259478,
#259479,#259480,#259481,#259482,#259483,#259484,#259485,#259486,#259487,
#259488,#259489,#259490,#259491,#259492,#259493,#259494,#259495,#259496,
#259497,#259498,#259499,#259500,#259501,#259502,#259503,#259504,#259505,
#259506,#259507,#259508,#259509,#259510,#259511,#259512,#259513,#259514,
#259515,#259516,#259517,#259518,#259519,#259520,#259521,#259522,#259523,
#259524,#259525,#259526,#259527,#259528,#259529,#259530,#259531,#259532,
#259533,#259534,#259535,#259536,#259537,#259538,#259539,#259540,#259541,
#259542,#259543,#259544,#259545,#259546,#259547,#259548,#259549,#259550,
#259551,#259552,#259553,#259554,#259555,#259556,#259557,#259558,#259559,
#259560,#259561,#259562,#259563,#259564,#259565,#259566,#259567,#259568,
#259569,#259570,#259571,#259572,#259573,#259574,#259575,#259576,#259577,
#259578,#259579,#259580,#259581,#259582,#259583,#259584,#259585,#259586,
#259587,#259588,#259589,#259590,#259591,#259592,#259593,#259594,#259595,
#259596,#259597,#259598,#259599,#259600,#259601,#259602,#259603,#259604,
#259605,#259606,#259607,#259608,#259609,#259610,#259611,#259612,#259613,
#259614,#259615,#259616,#259617,#259618,#259619,#259620,#259621,#259622,
#259623,#259624,#259625,#259626,#259627,#259628,#259629,#259630,#259631,
#259632,#259633,#259634,#259635,#259636,#259637,#259638,#259639,#259640,
#259641,#259642,#259643,#259644,#259645,#259646,#259647,#259648,#259649,
#259650,#259651,#259652,#259653,#259654,#259655,#259656,#259657,#259658,
#259659,#259660,#259661,#259662,#259663,#259664,#259665,#259666,#259667,
#259668,#259669,#259670,#259671,#259672,#259673,#259674,#259675,#259676,
#259677,#259678,#259679,#259680,#259681,#259682,#259683,#259684,#259685,
#259686,#259687,#259688,#259689,#259690,#259691,#259692,#259693,#259694,
#259695,#259696,#259697,#259698,#259699,#259700,#259701,#259702,#259703,
#259704,#259705,#259706,#259707,#259708,#259709,#259710,#259711,#259712,
#259713,#259714,#259715,#259716,#259717,#259718,#259719,#259720,#259721,
#259722,#259723,#259724,#259725,#259726),(#259727,#259728,#259729,#259730,
#259731,#259732,#259733,#259734,#259735,#259736,#259737,#259738,#259739,
#259740,#259741,#259742,#259743,#259744,#259745,#259746,#259747,#259748,
#259749,#259750,#259751,#259752,#259753,#259754,#259755,#259756,#259757,
#259758,#259759,#259760,#259761,#259762,#259763,#259764,#259765,#259766,
#259767,#259768,#259769,#259770,#259771,#259772,#259773,#259774,#259775,
#259776,#259777,#259778,#259779,#259780,#259781,#259782,#259783,#259784,
#259785,#259786,#259787,#259788,#259789,#259790,#259791,#259792,#259793,
#259794,#259795,#259796,#259797,#259798,#259799,#259800,#259801,#259802,
#259803,#259804,#259805,#259806,#259807,#259808,#259809,#259810,#259811,
#259812,#259813,#259814,#259815,#259816,#259817,#259818,#259819,#259820,
#259821,#259822,#259823,#259824,#259825,#259826,#259827,#259828,#259829,
#259830,#259831,#259832,#259833,#259834,#259835,#259836,#259837,#259838,
#259839,#259840,#259841,#259842,#259843,#259844,#259845,#259846,#259847,
#259848,#259849,#259850,#259851,#259852,#259853,#259854,#259855,#259856,
#259857,#259858,#259859,#259860,#259861,#259862,#259863,#259864,#259865,
#259866,#259867,#259868,#259869,#259870,#259871,#259872,#259873,#259874,
#259875,#259876,#259877,#259878,#259879,#259880,#259881,#259882,#259883,
#259884,#259885,#259886,#259887,#259888,#259889,#259890,#259891,#259892,
#259893,#259894,#259895,#259896,#259897,#259898,#259899,#259900,#259901,
#259902,#259903,#259904,#259905,#259906,#259907,#259908,#259909,#259910,
#259911,#259912,#259913,#259914,#259915,#259916,#259917,#259918,#259919,
#259920,#259921,#259922,#259923,#259924,#259925,#259926,#259927,#259928,
#259929,#259930,#259931,#259932,#259933,#259934,#259935,#259936,#259937,
#259938,#259939,#259940,#259941,#259942,#259943,#259944,#259945,#259946,
#259947,#259948,#259949,#259950,#259951,#259952,#259953,#259954,#259955,
#259956,#259957,#259958,#259959,#259960,#259961,#259962,#259963,#259964,
#259965,#259966,#259967,#259968,#259969,#259970,#259971,#259972,#259973,
#259974,#259975,#259976,#259977,#259978,#259979,#259980,#259981,#259982,
#259983,#259984,#259985,#259986,#259987,#259988,#259989,#259990,#259991,
#259992,#259993,#259994,#259995,#259996,#259997,#259998,#259999,#260000,
#260001,#260002,#260003,#260004,#260005,#260006,#260007,#260008,#260009,
#260010,#260011,#260012,#260013,#260014,#260015,#260016,#260017,#260018,
#260019,#260020,#260021,#260022,#260023,#260024,#260025,#260026,#260027,
#260028,#260029,#260030,#260031,#260032,#260033,#260034,#260035,#260036,
#260037,#260038,#260039,#260040,#260041,#260042,#260043,#260044,#260045,
#260046,#260047,#260048,#260049,#260050,#260051,#260052,#260053,#260054,
#260055,#260056,#260057,#260058,#260059,#260060,#260061,#260062,#260063,
#260064,#260065,#260066,#260067,#260068,#260069,#260070,#260071,#260072,
#260073,#260074,#260075,#260076,#260077,#260078,#260079,#260080,#260081,
#260082,#260083,#260084,#260085,#260086,#260087,#260088,#260089,#260090,
#260091,#260092,#260093,#260094,#260095,#260096,#260097,#260098,#260099,
#260100,#260101,#260102,#260103,#260104,#260105,#260106,#260107,#260108,
#260109,#260110,#260111,#260112,#260113,#260114,#260115,#260116,#260117,
#260118,#260119,#260120,#260121,#260122,#260123,#260124,#260125,#260126,
#260127,#260128,#260129,#260130,#260131,#260132,#260133,#260134,#260135,
#260136,#260137,#260138,#260139,#260140,#260141,#260142,#260143,#260144,
#260145,#260146,#260147,#260148,#260149,#260150,#260151,#260152,#260153,
#260154,#260155,#260156,#260157,#260158,#260159,#260160,#260161,#260162,
#260163,#260164,#260165,#260166,#260167,#260168,#260169,#260170,#260171,
#260172,#260173,#260174,#260175,#260176,#260177,#260178,#260179,#260180,
#260181,#260182,#260183,#260184,#260185,#260186,#260187,#260188,#260189,
#260190,#260191,#260192,#260193,#260194,#260195,#260196,#260197,#260198,
#260199,#260200,#260201,#260202,#260203,#260204,#260205,#260206,#260207,
#260208,#260209,#260210,#260211,#260212,#260213,#260214,#260215,#260216,
#260217,#260218,#260219,#260220,#260221,#260222,#260223,#260224,#260225,
#260226,#260227,#260228,#260229,#260230,#260231,#260232,#260233,#260234,
#260235,#260236,#260237,#260238,#260239,#260240,#260241,#260242,#260243,
#260244,#260245,#260246,#260247,#260248,#260249,#260250,#260251,#260252,
#260253,#260254,#260255,#260256,#260257,#260258,#260259,#260260,#260261,
#260262,#260263,#260264,#260265,#260266,#260267,#260268,#260269,#260270,
#260271,#260272,#260273,#260274,#260275,#260276,#260277,#260278,#260279,
#260280,#260281,#260282,#260283,#260284,#260285,#260286,#260287,#260288,
#260289,#260290,#260291,#260292,#260293,#260294,#260295,#260296,#260297,
#260298,#260299,#260300,#260301,#260302,#260303,#260304,#260305,#260306,
#260307,#260308,#260309,#260310,#260311,#260312,#260313,#260314,#260315,
#260316,#260317,#260318,#260319,#260320,#260321,#260322,#260323,#260324,
#260325,#260326,#260327,#260328,#260329,#260330,#260331,#260332,#260333,
#260334,#260335,#260336,#260337,#260338,#260339,#260340,#260341,#260342,
#260343,#260344,#260345,#260346,#260347,#260348,#260349,#260350,#260351,
#260352,#260353,#260354,#260355,#260356,#260357,#260358,#260359,#260360,
#260361,#260362,#260363,#260364,#260365,#260366,#260367,#260368,#260369,
#260370,#260371,#260372,#260373,#260374,#260375,#260376,#260377,#260378,
#260379,#260380,#260381,#260382,#260383,#260384,#260385,#260386,#260387,
#260388,#260389,#260390,#260391,#260392,#260393,#260394,#260395,#260396,
#260397,#260398,#260399,#260400,#260401,#260402,#260403,#260404,#260405,
#260406,#260407,#260408,#260409,#260410,#260411,#260412,#260413,#260414,
#260415,#260416,#260417,#260418,#260419,#260420,#260421,#260422,#260423,
#260424,#260425,#260426,#260427,#260428,#260429,#260430,#260431,#260432,
#260433,#260434,#260435,#260436,#260437,#260438,#260439,#260440,#260441,
#260442,#260443,#260444,#260445,#260446,#260447,#260448,#260449,#260450,
#260451,#260452,#260453,#260454,#260455,#260456,#260457,#260458,#260459,
#260460,#260461,#260462,#260463,#260464,#260465,#260466,#260467,#260468,
#260469,#260470,#260471,#260472,#260473,#260474,#260475,#260476,#260477,
#260478,#260479,#260480,#260481,#260482,#260483,#260484,#260485,#260486,
#260487,#260488,#260489,#260490,#260491,#260492,#260493,#260494,#260495,
#260496,#260497,#260498,#260499,#260500,#260501,#260502,#260503,#260504,
#260505,#260506,#260507,#260508,#260509,#260510,#260511,#260512,#260513,
#260514,#260515,#260516,#260517,#260518,#260519,#260520,#260521,#260522,
#260523,#260524,#260525,#260526,#260527,#260528,#260529,#260530,#260531,
#260532,#260533,#260534,#260535,#260536,#260537,#260538,#260539,#260540,
#260541,#260542,#260543,#260544,#260545,#260546,#260547,#260548,#260549,
#260550,#260551,#260552,#260553,#260554,#260555,#260556,#260557,#260558,
#260559,#260560,#260561,#260562,#260563,#260564,#260565,#260566,#260567,
#260568,#260569,#260570,#260571,#260572,#260573,#260574,#260575,#260576,
#260577,#260578,#260579,#260580,#260581,#260582,#260583,#260584,#260585,
#260586,#260587,#260588,#260589,#260590,#260591,#260592,#260593,#260594,
#260595,#260596,#260597,#260598,#260599,#260600,#260601,#260602,#260603,
#260604,#260605,#260606,#260607,#260608,#260609,#260610,#260611,#260612,
#260613,#260614,#260615,#260616,#260617,#260618,#260619,#260620,#260621,
#260622,#260623,#260624,#260625,#260626,#260627,#260628,#260629,#260630,
#260631,#260632,#260633,#260634,#260635,#260636,#260637,#260638,#260639,
#260640,#260641,#260642,#260643,#260644,#260645,#260646,#260647,#260648,
#260649,#260650,#260651,#260652,#260653,#260654,#260655,#260656,#260657,
#260658,#260659,#260660,#260661,#260662,#260663,#260664,#260665,#260666,
#260667,#260668,#260669,#260670,#260671,#260672,#260673,#260674,#260675,
#260676,#260677,#260678,#260679,#260680,#260681,#260682,#260683,#260684,
#260685,#260686,#260687,#260688,#260689,#260690,#260691,#260692,#260693,
#260694,#260695,#260696,#260697,#260698,#260699,#260700,#260701,#260702,
#260703,#260704,#260705,#260706,#260707,#260708,#260709,#260710,#260711,
#260712,#260713,#260714,#260715,#260716,#260717,#260718,#260719,#260720,
#260721,#260722,#260723,#260724,#260725,#260726,#260727,#260728,#260729,
#260730,#260731,#260732,#260733,#260734,#260735,#260736,#260737,#260738,
#260739,#260740,#260741,#260742,#260743,#260744,#260745,#260746,#260747,
#260748,#260749,#260750,#260751,#260752,#260753,#260754,#260755,#260756,
#260757,#260758,#260759,#260760,#260761,#260762,#260763,#260764,#260765,
#260766,#260767,#260768,#260769,#260770,#260771,#260772,#260773,#260774,
#260775,#260776,#260777,#260778,#260779,#260780,#260781,#260782,#260783,
#260784,#260785,#260786,#260787,#260788,#260789,#260790,#260791,#260792,
#260793,#260794,#260795,#260796,#260797,#260798,#260799,#260800,#260801,
#260802,#260803,#260804,#260805,#260806,#260807,#260808,#260809,#260810,
#260811,#260812,#260813,#260814,#260815,#260816,#260817,#260818,#260819,
#260820,#260821,#260822,#260823,#260824,#260825,#260826,#260827,#260828,
#260829,#260830,#260831,#260832,#260833,#260834,#260835,#260836,#260837,
#260838,#260839,#260840,#260841,#260842,#260843,#260844,#260845,#260846,
#260847,#260848,#260849,#260850,#260851,#260852,#260853,#260854,#260855,
#260856,#260857,#260858,#260859,#260860,#260861,#260862,#260863,#260864,
#260865,#260866,#260867,#260868,#260869,#260870,#260871,#260872,#260873,
#260874,#260875,#260876,#260877,#260878,#260879,#260880,#260881,#260882,
#260883,#260884,#260885,#260886,#260887,#260888,#260889,#260890,#260891,
#260892,#260893,#260894,#260895,#260896,#260897,#260898,#260899,#260900,
#260901,#260902,#260903,#260904,#260905,#260906,#260907,#260908,#260909,
#260910,#260911,#260912,#260913,#260914,#260915,#260916,#260917,#260918,
#260919,#260920,#260921,#260922,#260923,#260924,#260925,#260926,#260927,
#260928,#260929,#260930,#260931,#260932,#260933,#260934,#260935,#260936,
#260937,#260938,#260939,#260940,#260941,#260942,#260943,#260944,#260945,
#260946,#260947,#260948,#260949,#260950,#260951,#260952,#260953,#260954,
#260955,#260956,#260957,#260958,#260959,#260960,#260961,#260962,#260963,
#260964,#260965,#260966,#260967,#260968,#260969,#260970,#260971,#260972,
#260973,#260974,#260975,#260976,#260977,#260978,#260979,#260980,#260981,
#260982,#260983,#260984,#260985,#260986,#260987,#260988,#260989,#260990,
#260991,#260992,#260993,#260994,#260995,#260996,#260997,#260998,#260999,
#261000,#261001,#261002,#261003,#261004,#261005,#261006,#261007,#261008,
#261009,#261010,#261011,#261012,#261013,#261014,#261015,#261016,#261017,
#261018,#261019,#261020,#261021,#261022,#261023,#261024,#261025,#261026,
#261027,#261028,#261029,#261030,#261031,#261032,#261033,#261034,#261035,
#261036,#261037,#261038,#261039,#261040,#261041,#261042,#261043,#261044,
#261045,#261046,#261047,#261048,#261049,#261050,#261051,#261052,#261053,
#261054,#261055,#261056,#261057,#261058,#261059,#261060,#261061,#261062,
#261063,#261064,#261065,#261066,#261067,#261068,#261069,#261070,#261071,
#261072,#261073,#261074,#261075,#261076,#261077,#261078,#261079,#261080,
#261081,#261082,#261083,#261084,#261085,#261086,#261087,#261088,#261089,
#261090,#261091,#261092,#261093,#261094,#261095,#261096,#261097,#261098,
#261099,#261100,#261101,#261102,#261103,#261104,#261105,#261106,#261107,
#261108,#261109,#261110,#261111,#261112,#261113,#261114,#261115,#261116,
#261117,#261118,#261119,#261120,#261121,#261122,#261123,#261124,#261125,
#261126,#261127,#261128,#261129,#261130,#261131,#261132,#261133,#261134,
#261135,#261136,#261137,#261138,#261139,#261140,#261141,#261142,#261143,
#261144,#261145,#261146,#261147,#261148,#261149,#261150,#261151,#261152,
#261153,#261154,#261155,#261156,#261157,#261158,#261159,#261160,#261161,
#261162,#261163,#261164,#261165,#261166,#261167,#261168,#261169,#261170,
#261171,#261172,#261173,#261174,#261175,#261176,#261177,#261178,#261179,
#261180,#261181,#261182,#261183,#261184,#261185,#261186,#261187,#261188,
#261189,#261190,#261191,#261192,#261193,#261194,#261195,#261196,#261197,
#261198,#261199,#261200,#261201,#261202,#261203,#261204,#261205,#261206,
#261207,#261208,#261209,#261210,#261211,#261212,#261213,#261214,#261215,
#261216,#261217,#261218,#261219,#261220,#261221,#261222,#261223,#261224,
#261225,#261226,#261227,#261228,#261229,#261230,#261231,#261232,#261233,
#261234,#261235,#261236,#261237,#261238,#261239,#261240,#261241,#261242,
#261243,#261244,#261245,#261246,#261247,#261248,#261249,#261250,#261251,
#261252,#261253,#261254,#261255,#261256,#261257,#261258,#261259,#261260,
#261261,#261262,#261263,#261264,#261265,#261266,#261267,#261268,#261269,
#261270,#261271,#261272,#261273,#261274,#261275,#261276,#261277,#261278,
#261279,#261280,#261281,#261282,#261283,#261284,#261285,#261286,#261287,
#261288,#261289,#261290,#261291,#261292,#261293,#261294,#261295,#261296,
#261297,#261298,#261299,#261300,#261301,#261302,#261303,#261304,#261305,
#261306,#261307,#261308,#261309,#261310,#261311,#261312,#261313,#261314,
#261315,#261316,#261317,#261318,#261319,#261320,#261321,#261322,#261323,
#261324,#261325,#261326,#261327,#261328,#261329,#261330,#261331,#261332,
#261333,#261334,#261335,#261336,#261337,#261338,#261339,#261340,#261341,
#261342,#261343,#261344,#261345,#261346,#261347,#261348,#261349,#261350,
#261351,#261352,#261353,#261354,#261355,#261356,#261357,#261358,#261359,
#261360,#261361,#261362,#261363,#261364,#261365,#261366,#261367,#261368,
#261369,#261370,#261371,#261372,#261373,#261374,#261375,#261376,#261377,
#261378,#261379,#261380,#261381,#261382,#261383,#261384,#261385,#261386,
#261387,#261388,#261389,#261390,#261391,#261392,#261393,#261394,#261395,
#261396,#261397,#261398,#261399,#261400,#261401,#261402,#261403,#261404,
#261405,#261406,#261407,#261408,#261409,#261410,#261411,#261412,#261413,
#261414,#261415,#261416,#261417,#261418,#261419,#261420,#261421)),
 .UNSPECIFIED.,.F.,.F.,.F.,(4,4),(4,1,1,1,1,1,1,1,1,1,1,1,1,1,1,1,1,1,1,
1,1,1,1,1,1,1,1,1,1,1,1,1,1,1,1,1,1,1,1,1,1,1,1,1,1,1,1,1,1,1,1,1,1,1,1,
1,1,1,1,1,1,1,1,1,1,1,1,1,1,1,1,1,1,1,1,1,1,1,1,1,1,1,1,1,1,1,1,1,1,1,1,
1,1,1,1,1,1,1,1,1,1,1,1,1,1,1,1,1,1,1,1,1,1,1,1,1,1,1,1,1,1,1,1,1,1,1,1,
1,1,1,1,1,1,1,1,1,1,1,1,1,1,1,1,1,1,1,1,1,1,1,1,1,1,1,1,1,1,1,1,1,1,1,1,
1,1,1,1,1,1,1,1,1,1,1,1,1,1,1,1,1,1,1,1,1,1,1,1,1,1,1,1,1,1,1,1,1,1,1,1,
1,1,1,1,1,1,1,1,1,1,1,1,1,1,1,1,1,1,1,1,1,1,1,1,1,1,1,1,1,1,1,1,1,1,1,1,
1,1,1,1,1,1,1,1,1,1,1,1,1,1,1,1,1,1,1,1,1,1,1,1,1,1,1,1,1,1,1,1,1,1,1,1,
1,1,1,1,1,1,1,1,1,1,1,1,1,1,1,1,1,1,1,1,1,1,1,1,1,1,1,1,1,1,1,1,1,1,1,1,
1,1,1,1,1,1,1,1,1,1,1,1,1,1,1,1,1,1,1,1,1,1,1,1,1,1,1,1,1,1,1,1,1,1,1,1,
1,1,1,1,1,1,1,1,1,1,1,1,1,1,1,1,1,1,1,1,1,1,1,1,1,1,1,1,1,1,1,1,1,1,1,1,
1,1,1,1,1,1,1,1,1,1,1,1,1,1,1,1,1,1,1,1,1,1,1,1,1,1,1,1,1,1,1,1,1,1,1,1,
1,1,1,1,1,1,1,1,1,1,1,1,1,1,1,1,1,1,1,1,1,1,1,1,1,1,1,1,1,1,1,1,1,1,1,1,
1,1,1,1,1,1,1,1,1,1,1,1,1,1,1,1,1,1,1,1,1,1,1,1,1,1,1,1,1,1,1,1,1,1,1,1,
1,1,1,1,1,1,1,1,1,1,1,1,1,1,1,1,1,1,1,1,1,1,1,1,1,1,1,1,1,1,1,1,1,1,1,1,
1,1,1,1,1,1,1,1,1,1,1,1,1,1,1,1,1,1,1,1,1,1,1,1,1,1,1,1,1,1,1,1,1,1,1,1,
1,1,1,1,1,1,1,1,1,1,1,1,1,1,1,1,1,1,1,1,1,1,1,1,1,1,1,1,1,1,1,1,1,1,1,1,
1,1,1,1,1,1,1,1,1,1,1,1,1,1,1,1,1,1,1,1,1,1,1,1,1,1,1,1,1,1,1,1,1,1,1,1,
1,1,1,1,1,1,1,1,1,1,1,1,1,1,1,1,1,1,1,1,1,1,1,1,1,1,1,1,1,1,1,1,1,1,1,1,
1,1,1,1,1,1,1,1,1,1,1,1,1,1,1,1,1,1,1,1,1,1,1,1,1,1,1,1,1,1,1,1,1,1,1,1,
1,1,1,1,1,1,1,1,1,1,1,1,1,1,1,1,1,1,1,1,1,1,1,1,1,1,1,1,1,1,1,1,1,1,1,1,
1,1,1,1,1,1,1,1,1,1,1,1,1,1,1,1,1,1,1,1,1,1,1,1,1,1,1,1,1,1,1,1,1,1,1,1,
1,1,1,1,1,1,1,1,1,1,1,1,1,1,1,1,1,1,1,1,1,1,1,1,1,1,1,1,1,1,1,1,1,1,1,1,
1,1,1,1,1,1,1,1,1,1,1,1,1,1,1,1,1,1,1,1,1,1,1,1,1,1,1,1,1,1,1,1,1,1,1,1,
1,1,1,1,1,1,1,1,1,1,1,1,1,1,1,1,1,1,1,1,1,1,1,1,1,1,1,1,1,1,1,1,1,1,1,1,
1,1,1,1,1,1,1,1,1,1,1,1,1,1,1,1,1,1,1,1,1,1,1,1,1,1,1,1,1,1,1,1,1,1,1,1,
1,1,1,1,1,1,1,1,1,1,1,1,1,1,1,1,1,1,1,1,1,1,1,1,1,1,1,1,1,1,1,1,1,1,1,1,
1,1,1,1,1,1,1,1,1,1,1,1,1,1,1,1,1,1,1,1,1,1,1,1,1,1,1,1,1,1,1,1,1,1,1,1,
1,1,1,1,1,1,1,1,1,1,1,1,1,1,1,1,1,1,1,1,1,1,1,1,1,1,1,1,1,1,1,1,1,1,1,1,
1,1,1,1,1,1,1,1,1,1,1,1,1,1,1,1,1,1,1,1,1,1,1,1,1,1,1,1,1,1,1,1,1,1,1,1,
1,1,1,1,1,1,1,1,1,1,1,1,1,1,1,1,1,1,1,1,1,1,1,1,1,1,1,1,1,1,1,1,1,1,1,1,
1,1,1,1,1,1,1,1,1,1,1,1,1,1,1,1,1,1,1,1,1,1,1,1,1,1,1,1,1,1,1,1,1,1,1,1,
1,1,1,1,1,1,1,1,1,1,1,1,1,1,1,1,1,1,1,1,1,1,1,1,1,1,1,1,1,1,1,1,1,1,1,1,
1,1,1,1,1,1,1,1,1,1,1,1,1,1,1,1,1,1,1,1,1,1,1,1,1,1,1,1,1,1,1,1,1,1,1,1,
1,1,1,1,1,1,1,1,1,1,1,1,1,1,1,1,1,1,1,1,1,1,1,1,1,1,1,1,1,1,1,1,1,1,1,1,
1,1,1,1,1,1,1,1,1,1,1,1,1,1,1,1,1,1,1,1,1,1,1,1,1,1,1,1,1,1,1,1,1,1,1,1,
1,1,1,1,1,1,1,1,1,1,1,1,1,1,1,1,1,1,1,1,1,1,1,1,1,1,1,1,1,1,1,1,1,1,1,1,
1,1,1,1,1,1,1,1,1,1,1,1,1,1,1,1,1,1,1,1,1,1,1,1,1,1,1,1,1,1,1,1,1,1,1,1,
1,1,1,1,1,1,1,1,1,1,1,1,1,1,1,1,1,1,1,1,1,1,1,1,1,1,1,1,1,1,1,1,1,1,1,1,
1,1,1,1,1,1,1,1,1,1,1,1,1,1,1,1,1,1,1,1,1,1,1,1,1,1,1,1,1,1,1,1,1,1,1,1,
1,1,1,1,1,1,1,1,1,1,1,1,1,1,1,1,1,1,1,1,1,1,1,1,1,1,1,1,1,1,1,1,1,1,1,1,
1,1,1,1,1,1,1,1,1,1,1,1,1,1,1,1,1,1,1,1,1,1,1,1,1,1,1,1,1,1,1,1,1,1,1,1,
1,1,1,1,1,1,1,1,1,1,1,1,1,1,1,1,1,1,1,1,1,1,1,1,1,1,1,1,1,1,1,1,1,1,1,1,
1,1,1,1,1,1,1,1,1,1,1,1,1,1,1,1,1,1,1,1,1,1,1,1,1,1,1,1,1,1,1,1,1,1,1,1,
1,1,1,1,1,1,1,1,1,1,1,1,1,1,1,1,1,1,1,1,1,1,1,1,1,1,1,1,1,1,1,1,1,1,1,1,
1,1,1,1,1,1,1,1,1,1,1,1,1,1,1,1,1,1,1,1,1,1,1,1,1,1,1,1,1,1,1,1,1,1,1,1,
1,1,1,1,1,1,1,1,1,1,1,1,1,1,1,1,1,1,1,1,1,1,1,1,1,1,1,1,1,1,1,1,1,1,1,1,
1,1,1,1,1,1,1,1,1,1,1,1,1,1,1,1,1,4),(-0.000587328099657093,0.1157205948422),
(8.30590413559005,8.80579087257276,9.30565887793282,10.305394888653,11.3051308993731,
12.3048669100932,13.3046029208133,14.3043389315335,15.3040749422536,16.3038109529737,
17.3035469636939,18.303282974414,19.3030189851341,20.3027549958542,21.3024910065744,
22.3022270172945,23.3019630280146,24.3016990387348,25.3014350494549,26.301171060175,
27.3009070708951,28.3006430816153,29.3003790923354,30.3001151030555,31.2998511137757,
32.2995871244958,33.2993231352159,34.299059145936,35.2987951566562,36.2985311673763,
37.2982671780964,38.2980031888166,39.2977391995367,40.2974752102568,41.2972112209769,
42.2969472316971,43.2966832424172,44.2964192531373,45.2961552638575,46.2958912745776,
47.2956272852977,48.2953632960178,49.295099306738,50.2948353174581,51.2945713281782,
52.2943073388984,53.2940433496185,54.2937793603386,55.2935153710587,56.2932513817789,
57.292987392499,58.2927234032191,59.2924594139393,60.2921954246594,61.2919314353795,
62.2916674460996,63.2914034568198,64.2911394675399,65.29087547826,66.2906114889802,
67.2903474997003,68.2900835104204,69.2898195211405,70.2895555318607,71.2892915425808,
72.2890275533009,73.2887635640211,74.2884995747412,75.2882355854613,76.2879715961814,
77.2877076069016,78.2874436176217,79.2871796283418,80.286915639062,81.2866516497821,
82.2863876605022,83.2861236712224,84.2858596819425,85.2855956926626,86.2853317033827,
87.2850677141029,88.284803724823,89.2845397355431,90.2842757462633,91.2840117569834,
92.2837477677035,93.2834837784236,94.2832197891438,95.2829557998639,96.282691810584,
97.2824278213041,98.2821638320243,99.2818998427444,100.281635853465,101.281371864185,
102.281107874905,103.280843885625,104.280579896345,105.280315907065,106.280051917785,
107.279787928505,108.279523939226,109.279259949946,110.278995960666,111.278731971386,
112.278467982106,113.278203992826,114.277940003546,115.277676014266,116.277412024987,
117.277148035707,118.276884046427,119.276620057147,120.276356067867,121.276092078587,
122.275828089307,123.275564100028,124.275300110748,125.275036121468,126.274772132188,
127.274508142908,128.274244153628,129.273980164348,130.273716175068,131.273452185789,
132.273188196509,133.272924207229,134.272660217949,135.272396228669,136.272132239389,
137.271868250109,138.271604260829,139.27134027155,140.27107628227,141.27081229299,
142.27054830371,143.27028431443,144.27002032515,145.26975633587,146.26949234659,
147.269228357311,148.268964368031,149.268700378751,150.268436389471,151.268172400191,
152.267908410911,153.267644421631,154.267380432352,155.267116443072,156.266852453792,
157.266588464512,158.266324475232,159.266060485952,160.265796496672,161.265532507392,
162.265268518113,163.265004528833,164.264740539553,165.264476550273,166.264212560993,
167.263948571713,168.263684582433,169.263420593153,170.263156603874,171.262892614594,
172.262628625314,173.262364636034,174.262100646754,175.261836657474,176.261572668194,
177.261308678914,178.261044689635,179.260780700355,180.260516711075,181.260252721795,
182.259988732515,183.259724743235,184.259460753955,185.259196764675,186.258932775396,
187.258668786116,188.258404796836,189.258140807556,190.257876818276,191.257612828996,
192.257348839716,193.257084850437,194.256820861157,195.256556871877,196.256292882597,
197.256028893317,198.255764904037,199.255500914757,200.255236925477,201.254972936198,
202.254708946918,203.254444957638,204.254180968358,205.253916979078,206.253652989798,
207.253389000518,208.253125011238,209.252861021959,210.252597032679,211.252333043399,
212.252069054119,213.251805064839,214.251541075559,215.251277086279,216.251013096999,
217.25074910772,218.25048511844,219.25022112916,220.24995713988,221.2496931506,
222.24942916132,223.24916517204,224.248901182761,225.248637193481,226.248373204201,
227.248109214921,228.247845225641,229.247581236361,230.247317247081,231.247053257801,
232.246789268522,233.246525279242,234.246261289962,235.245997300682,236.245733311402,
237.245469322122,238.245205332842,239.244941343562,240.244677354283,241.244413365003,
242.244149375723,243.243885386443,244.243621397163,245.243357407883,246.243093418603,
247.242829429323,248.242565440044,249.242301450764,250.242037461484,251.241773472204,
252.241509482924,253.241245493644,254.240981504364,255.240717515084,256.240453525805,
257.240189536525,258.239925547245,259.239661557965,260.239397568685,261.239133579405,
262.238869590125,263.238605600846,264.238341611566,265.238077622286,266.237813633006,
267.237549643726,268.237285654446,269.237021665166,270.236757675886,271.236493686607,
272.236229697327,273.235965708047,274.235701718767,275.235437729487,276.235173740207,
277.234909750927,278.234645761647,279.234381772368,280.234117783088,281.233853793808,
282.233589804528,283.233325815248,284.233061825968,285.232797836688,286.232533847408,
287.232269858129,288.232005868849,289.231741879569,290.231477890289,291.231213901009,
292.230949911729,293.230685922449,294.23042193317,295.23015794389,296.22989395461,
297.22962996533,298.22936597605,299.22910198677,300.22883799749,301.22857400821,
302.228310018931,303.228046029651,304.227782040371,305.227518051091,306.227254061811,
307.226990072531,308.226726083251,309.226462093971,310.226198104692,311.225934115412,
312.225670126132,313.225406136852,314.225142147572,315.224878158292,316.224614169012,
317.224350179732,318.224086190453,319.223822201173,320.223558211893,321.223294222613,
322.223030233333,323.222766244053,324.222502254773,325.222238265494,326.221974276214,
327.221710286934,328.221446297654,329.221182308374,330.220918319094,331.220654329814,
332.220390340534,333.220126351255,334.219862361975,335.219598372695,336.219334383415,
337.219070394135,338.218806404855,339.218542415575,340.218278426295,341.218014437016,
342.217750447736,343.217486458456,344.217222469176,345.216958479896,346.216694490616,
347.216430501336,348.216166512056,349.215902522777,350.215638533497,351.215374544217,
352.215110554937,353.214846565657,354.214582576377,355.214318587097,356.214054597817,
357.213790608538,358.213526619258,359.213262629978,360.212998640698,361.212734651418,
362.212470662138,363.212206672858,364.211942683579,365.211678694299,366.211414705019,
367.211150715739,368.210886726459,369.210622737179,370.210358747899,371.210094758619,
372.20983076934,373.20956678006,374.20930279078,375.2090388015,376.20877481222,
377.20851082294,378.20824683366,379.20798284438,380.207718855101,381.207454865821,
382.207190876541,383.206926887261,384.206662897981,385.206398908701,386.206134919421,
387.205870930141,388.205606940862,389.205342951582,390.205078962302,391.204814973022,
392.204550983742,393.204286994462,394.204023005182,395.203759015903,396.203495026623,
397.203231037343,398.202967048063,399.202703058783,400.202439069503,401.202175080223,
402.201911090943,403.201647101664,404.201383112384,405.201119123104,406.200855133824,
407.200591144544,408.200327155264,409.200063165984,410.199799176704,411.199535187425,
412.199271198145,413.199007208865,414.198743219585,415.198479230305,416.198215241025,
417.197951251745,418.197687262465,419.197423273186,420.197159283906,421.196895294626,
422.196631305346,423.196367316066,424.196103326786,425.195839337506,426.195575348226,
427.195311358947,428.195047369667,429.194783380387,430.194519391107,431.194255401827,
432.193991412547,433.193727423267,434.193463433988,435.193199444708,436.192935455428,
437.192671466148,438.192407476868,439.192143487588,440.191879498308,441.191615509028,
442.191351519749,443.191087530469,444.190823541189,445.190559551909,446.190295562629,
447.190031573349,448.189767584069,449.189503594789,450.18923960551,451.18897561623,
452.18871162695,453.18844763767,454.18818364839,455.18791965911,456.18765566983,
457.18739168055,458.187127691271,459.186863701991,460.186599712711,461.186335723431,
462.186071734151,463.185807744871,464.185543755591,465.185279766312,466.185015777032,
467.184751787752,468.184487798472,469.184223809192,470.183959819912,471.183695830632,
472.183431841352,473.183167852073,474.182903862793,475.182639873513,476.182375884233,
477.182111894953,478.181847905673,479.181583916393,480.181319927113,481.181055937834,
482.180791948554,483.180527959274,484.180263969994,485.179999980714,486.179735991434,
487.179472002154,488.179208012874,489.178944023595,490.178680034315,491.178416045035,
492.178152055755,493.177888066475,494.177624077195,495.177360087915,496.177096098636,
497.176832109356,498.176568120076,499.176304130796,500.176040141516,501.175776152236,
502.175512162956,503.175248173676,504.174984184397,505.174720195117,506.174456205837,
507.174192216557,508.173928227277,509.173664237997,510.173400248717,511.173136259437,
512.172872270158,513.172608280878,514.172344291598,515.172080302318,516.171816313038,
517.171552323758,518.171288334478,519.171024345198,520.170760355919,521.170496366639,
522.170232377359,523.169968388079,524.169704398799,525.169440409519,526.169176420239,
527.168912430959,528.16864844168,529.1683844524,530.16812046312,531.16785647384,
532.16759248456,533.16732849528,534.167064506,535.166800516721,536.166536527441,
537.166272538161,538.166008548881,539.165744559601,540.165480570321,541.165216581041,
542.164952591761,543.164688602482,544.164424613202,545.164160623922,546.163896634642,
547.163632645362,548.163368656082,549.163104666802,550.162840677522,551.162576688243,
552.162312698963,553.162048709683,554.161784720403,555.161520731123,556.161256741843,
557.160992752563,558.160728763283,559.160464774004,560.160200784724,561.159936795444,
562.159672806164,563.159408816884,564.159144827604,565.158880838324,566.158616849045,
567.158352859765,568.158088870485,569.157824881205,570.157560891925,571.157296902645,
572.157032913365,573.156768924085,574.156504934806,575.156240945526,576.155976956246,
577.155712966966,578.155448977686,579.155184988406,580.154920999126,581.154657009846,
582.154393020567,583.154129031287,584.153865042007,585.153601052727,586.153337063447,
587.153073074167,588.152809084887,589.152545095607,590.152281106328,591.152017117048,
592.151753127768,593.151489138488,594.151225149208,595.150961159928,596.150697170648,
597.150433181368,598.150169192089,599.149905202809,600.149641213529,601.149377224249,
602.149113234969,603.148849245689,604.148585256409,605.14832126713,606.14805727785,
607.14779328857,608.14752929929,609.14726531001,610.14700132073,611.14673733145,
612.14647334217,613.146209352891,614.145945363611,615.145681374331,616.145417385051,
617.145153395771,618.144889406491,619.144625417211,620.144361427931,621.144097438652,
622.143833449372,623.143569460092,624.143305470812,625.143041481532,626.142777492252,
627.142513502972,628.142249513692,629.141985524413,630.141721535133,631.141457545853,
632.141193556573,633.140929567293,634.140665578013,635.140401588733,636.140137599454,
637.139873610174,638.139609620894,639.139345631614,640.139081642334,641.138817653054,
642.138553663774,643.138289674494,644.138025685215,645.137761695935,646.137497706655,
647.137233717375,648.136969728095,649.136705738815,650.136441749535,651.136177760255,
652.135913770976,653.135649781696,654.135385792416,655.135121803136,656.134857813856,
657.134593824576,658.134329835296,659.134065846016,660.133801856737,661.133537867457,
662.133273878177,663.133009888897,664.132745899617,665.132481910337,666.132217921057,
667.131953931778,668.131689942498,669.131425953218,670.131161963938,671.130897974658,
672.130633985378,673.130369996098,674.130106006818,675.129842017539,676.129578028259,
677.129314038979,678.129050049699,679.128786060419,680.128522071139,681.128258081859,
682.127994092579,683.1277301033,684.12746611402,685.12720212474,686.12693813546,
687.12667414618,688.1264101569,689.12614616762,690.12588217834,691.125618189061,
692.125354199781,693.125090210501,694.124826221221,695.124562231941,696.124298242661,
697.124034253381,698.123770264101,699.123506274822,700.123242285542,701.122978296262,
702.122714306982,703.122450317702,704.122186328422,705.121922339142,706.121658349863,
707.121394360583,708.121130371303,709.120866382023,710.120602392743,711.120338403463,
712.120074414183,713.119810424903,714.119546435624,715.119282446344,716.119018457064,
717.118754467784,718.118490478504,719.118226489224,720.117962499944,721.117698510664,
722.117434521385,723.117170532105,724.116906542825,725.116642553545,726.116378564265,
727.116114574985,728.115850585705,729.115586596425,730.115322607146,731.115058617866,
732.114794628586,733.114530639306,734.114266650026,735.114002660746,736.113738671466,
737.113474682187,738.113210692907,739.112946703627,740.112682714347,741.112418725067,
742.112154735787,743.111890746507,744.111626757227,745.111362767948,746.111098778668,
747.110834789388,748.110570800108,749.110306810828,750.110042821548,751.109778832268,
752.109514842988,753.109250853709,754.108986864429,755.108722875149,756.108458885869,
757.108194896589,758.107930907309,759.107666918029,760.107402928749,761.10713893947,
762.10687495019,763.10661096091,764.10634697163,765.10608298235,766.10581899307,
767.10555500379,768.10529101451,769.105027025231,770.104763035951,771.104499046671,
772.104235057391,773.103971068111,774.103707078831,775.103443089551,776.103179100272,
777.102915110992,778.102651121712,779.102387132432,780.102123143152,781.101859153872,
782.101595164592,783.101331175312,784.101067186033,785.100803196753,786.100539207473,
787.100275218193,788.100011228913,789.099747239633,790.099483250353,791.099219261073,
792.098955271794,793.098691282514,794.098427293234,795.098163303954,796.097899314674,
797.097635325394,798.097371336114,799.097107346834,800.096843357555,801.096579368275,
802.096315378995,803.096051389715,804.095787400435,805.095523411155,806.095259421875,
807.094995432596,808.094731443316,809.094467454036,810.094203464756,811.093939475476,
812.093675486196,813.093411496916,814.093147507636,815.092883518357,816.092619529077,
817.092355539797,818.092091550517,819.091827561237,820.091563571957,821.091299582677,
822.091035593397,823.090771604118,824.090507614838,825.090243625558,826.089979636278,
827.089715646998,828.089451657718,829.089187668438,830.088923679158,831.088659689879,
832.088395700599,833.088131711319,834.087867722039,835.087603732759,836.087339743479,
837.087075754199,838.08681176492,839.08654777564,840.08628378636,841.08601979708,
842.0857558078,843.08549181852,844.08522782924,845.08496383996,846.084699850681,
847.084435861401,848.084171872121,849.083907882841,850.083643893561,851.083379904281,
852.083115915001,853.082851925721,854.082587936442,855.082323947162,856.082059957882,
857.081795968602,858.081531979322,859.081267990042,860.081004000762,861.080740011482,
862.080476022203,863.080212032923,864.079948043643,865.079684054363,866.079420065083,
867.079156075803,868.078892086523,869.078628097243,870.078364107964,871.078100118684,
872.077836129404,873.077572140124,874.077308150844,875.077044161564,876.076780172284,
877.076516183005,878.076252193725,879.075988204445,880.075724215165,881.075460225885,
882.075196236605,883.074932247325,884.074668258045,885.074404268766,886.074140279486,
887.073876290206,888.073612300926,889.073348311646,890.073084322366,891.072820333086,
892.072556343806,893.072292354527,894.072028365247,895.071764375967,896.071500386687,
897.071236397407,898.070972408127,899.070708418847,900.070444429567,901.070180440288,
902.069916451008,903.069652461728,904.069388472448,905.069124483168,906.068860493888,
907.068596504608,908.068332515329,909.068068526049,910.067804536769,911.067540547489,
912.067276558209,913.067012568929,914.066748579649,915.066484590369,916.06622060109,
917.06595661181,918.06569262253,919.06542863325,920.06516464397,921.06490065469,
922.06463666541,923.06437267613,924.064108686851,925.063844697571,926.063580708291,
927.063316719011,928.063052729731,929.062788740451,930.062524751171,931.062260761891,
932.061996772612,933.061732783332,934.061468794052,935.061204804772,936.060940815492,
937.060676826212,938.060412836932,939.060148847652,940.059884858373,941.059620869093,
942.059356879813,943.059092890533,944.058828901253,945.058564911973,946.058300922693,
947.058036933414,948.057772944134,949.057508954854,950.057244965574,951.056980976294,
952.056716987014,953.056452997734,954.056189008454,955.055925019175,956.055661029895,
957.055397040615,958.055133051335,959.054869062055,960.054605072775,961.054341083495,
962.054077094215,963.053813104936,964.053549115656,965.053285126376,966.053021137096,
967.052757147816,968.052493158536,969.052229169256,970.051965179976,971.051701190697,
972.051437201417,973.051173212137,974.050909222857,975.050645233577,976.050381244297,
977.050117255017,978.049853265738,979.049589276458,980.049325287178,981.049061297898,
982.048797308618,983.048533319338,984.048269330058,985.048005340778,986.047741351499,
987.047477362219,988.047213372939,989.046949383659,990.046685394379,991.046421405099,
992.046157415819,993.045893426539,994.04562943726,995.04536544798,996.0451014587,
997.04483746942,998.04457348014,999.04430949086,1000.04404550158,1001.0437815123,
1002.04351752302,1003.04325353374,1004.04298954446,1005.04272555518,1006.0424615659,
1007.04219757662,1008.04193358734,1009.04166959806,1010.04140560878,1011.0411416195,
1012.04087763022,1013.04061364094,1014.04034965166,1015.04008566238,1016.0398216731,
1017.03955768382,1018.03929369454,1019.03902970526,1020.03876571598,1021.0385017267,
1022.03823773742,1023.03797374814,1024.03770975886,1025.03744576958,1026.0371817803,
1027.03691779102,1028.03665380174,1029.03638981246,1030.03612582318,1031.0358618339,
1032.03559784462,1033.03533385534,1034.03506986606,1035.03480587678,1036.03454188751,
1037.03427789823,1038.03401390895,1039.03374991967,1040.03348593039,1041.03322194111,
1042.03295795183,1043.03269396255,1044.03242997327,1045.03216598399,1046.03190199471,
1047.03163800543,1048.03137401615,1049.03111002687,1050.03084603759,1051.03058204831,
1052.03031805903,1053.03005406975,1054.02979008047,1055.02952609119,1056.02926210191,
1057.02899811263,1058.02873412335,1059.02847013407,1060.02820614479,1061.02794215551,
1062.02767816623,1063.02741417695,1064.02715018767,1065.02688619839,1066.02662220911,
1067.02635821983,1068.02609423055,1069.02583024127,1070.02556625199,1071.02530226271,
1072.02503827343,1073.02477428415,1074.02451029487,1075.02424630559,1076.02398231631,
1077.02371832703,1078.02345433775,1079.02319034847,1080.02292635919,1081.02266236991,
1082.02239838063,1083.02213439135,1084.02187040207,1085.02160641279,1086.02134242351,
1087.02107843423,1088.02081444495,1089.02055045567,1090.02028646639,1091.02002247711,
1092.01975848783,1093.01949449855,1094.01923050927,1095.01896651999,1096.01870253071,
1097.01843854143,1098.01817455215,1099.01791056287,1100.01764657359,1101.01738258431,
1102.01711859503,1103.01685460575,1104.01659061647,1105.01632662719,1106.01606263791,
1107.01579864863,1108.01553465935,1109.01527067007,1110.01500668079,1111.01474269151,
1112.01447870223,1113.01421471295,1114.01395072368,1115.0136867344,1116.01342274512,
1117.01315875584,1118.01289476656,1119.01263077728,1120.012366788,1121.01210279872,
1122.01183880944,1123.01157482016,1124.01131083088,1125.0110468416,1126.01078285232,
1127.01051886304,1128.01025487376,1129.00999088448,1130.0097268952,1131.00946290592,
1132.00919891664,1133.00893492736,1134.00867093808,1135.0084069488,1136.00814295952,
1137.00787897024,1138.00761498096,1139.00735099168,1140.0070870024,1141.00682301312,
1142.00655902384,1143.00629503456,1144.00603104528,1145.005767056,1146.00550306672,
1147.00523907744,1148.00497508816,1149.00471109888,1150.0044471096,1151.00418312032,
1152.00391913104,1153.00365514176,1154.00339115248,1155.0031271632,1156.00286317392,
1157.00259918464,1158.00233519536,1159.00207120608,1160.0018072168,1161.00154322752,
1162.00127923824,1163.00101524896,1164.00075125968,1165.0004872704,1166.00022328112,
1166.99995929184,1167.99969530256,1168.99943131328,1169.999167324,1170.99890333472,
1171.99863934544,1172.99837535616,1173.99811136688,1174.9978473776,1175.99758338832,
1176.99731939904,1177.99705540976,1178.99679142048,1179.9965274312,1180.99626344192,
1181.99599945264,1182.99573546336,1183.99547147408,1184.9952074848,1185.99494349552,
1186.99467950624,1187.99441551696,1188.99415152768,1189.99388753841,1190.99362354913,
1191.99335955985,1192.99309557057,1193.99283158129,1194.99256759201,1195.99230360273,
1196.99203961345,1197.99177562417,1198.99151163489,1199.99124764561,1200.99098365633,
1201.99071966705,1202.99045567777,1203.99019168849,1204.98992769921,1205.98966370993,
1206.98939972065,1207.98913573137,1208.98887174209,1209.98860775281,1210.98834376353,
1211.98807977425,1212.98781578497,1213.98755179569,1214.98728780641,1215.98702381713,
1216.98675982785,1217.98649583857,1218.98623184929,1219.98596786001,1220.98570387073,
1221.98543988145,1222.98517589217,1223.98491190289,1224.98464791361,1225.98438392433,
1226.98411993505,1227.98385594577,1228.98359195649,1229.98332796721,1230.98306397793,
1231.98279998865,1232.98253599937,1233.98227201009,1234.98200802081,1235.98174403153,
1236.98148004225,1237.98121605297,1238.98095206369,1239.98068807441,1240.98042408513,
1241.98016009585,1242.97989610657,1243.97963211729,1244.97936812801,1245.97910413873,
1246.97884014945,1247.97857616017,1248.97831217089,1249.97804818161,1250.97778419233,
1251.97752020305,1252.97725621377,1253.97699222449,1254.97672823521,1255.97646424593,
1256.97620025665,1257.97593626737,1258.97567227809,1259.97540828881,1260.97514429953,
1261.97488031025,1262.97461632097,1263.97435233169,1264.97408834241,1265.97382435313,
1266.97356036385,1267.97329637458,1268.9730323853,1269.97276839602,1270.97250440674,
1271.97224041746,1272.97197642818,1273.9717124389,1274.97144844962,1275.97118446034,
1276.97092047106,1277.97065648178,1278.9703924925,1279.97012850322,1280.96986451394,
1281.96960052466,1282.96933653538,1283.9690725461,1284.96880855682,1285.96854456754,
1286.96828057826,1287.96801658898,1288.9677525997,1289.96748861042,1290.96722462114,
1291.96696063186,1292.96669664258,1293.9664326533,1294.96616866402,1295.96590467474,
1296.96564068546,1297.96537669618,1298.9651127069,1299.96484871762,1300.96458472834,
1301.96432073906,1302.96405674978,1303.9637927605,1304.96352877122,1305.96326478194,
1306.96300079266,1307.96273680338,1308.9624728141,1309.96220882482,1310.96194483554,
1311.96168084626,1312.96141685698,1313.9611528677,1314.96088887842,1315.96062488914,
1316.96036089986,1317.96009691058,1318.9598329213,1319.95956893202,1320.95930494274,
1321.95904095346,1322.95877696418,1323.9585129749,1324.95824898562,1325.95798499634,
1326.95772100706,1327.95745701778,1328.9571930285,1329.95692903922,1330.95666504994,
1331.95640106066,1332.95613707138,1333.9558730821,1334.95560909282,1335.95534510354,
1336.95508111426,1337.95481712498,1338.9545531357,1339.95428914642,1340.95402515714,
1341.95376116786,1342.95349717858,1343.9532331893,1344.95296920002,1345.95270521075,
1346.95244122147,1347.95217723219,1348.95191324291,1349.95164925363,1350.95138526435,
1351.95112127507,1352.95085728579,1353.95059329651,1354.95032930723,1355.95006531795,
1356.94980132867,1357.94953733939,1358.94927335011,1359.94900936083,1360.94874537155,
1361.94848138227,1362.94821739299,1363.94795340371,1364.94768941443,1365.94742542515,
1366.94716143587,1367.94689744659,1368.94663345731,1369.94636946803,1370.94610547875,
1371.94584148947,1372.94557750019,1373.94531351091,1374.94504952163,1375.94478553235,
1376.94452154307,1377.94425755379,1378.94399356451,1379.94372957523,1380.94346558595,
1381.94320159667,1382.94293760739,1383.94267361811,1384.94240962883,1385.94214563955,
1386.94188165027,1387.94161766099,1388.94135367171,1389.94108968243,1390.94082569315,
1391.94056170387,1392.94029771459,1393.94003372531,1394.93976973603,1395.93950574675,
1396.93924175747,1397.93897776819,1398.93871377891,1399.93844978963,1400.93818580035,
1401.93792181107,1402.93765782179,1403.93739383251,1404.93712984323,1405.93686585395,
1406.93660186467,1407.93633787539,1408.93607388611,1409.93580989683,1410.93554590755,
1411.93528191827,1412.93501792899,1413.93475393971,1414.93448995043,1415.93422596115,
1416.93396197187,1417.93369798259,1418.93343399331,1419.93317000403,1420.93290601475,
1421.93264202547,1422.93237803619,1423.93211404692,1424.93185005764,1425.93158606836,
1426.93132207908,1427.9310580898,1428.93079410052,1429.93053011124,1430.93026612196,
1431.93000213268,1432.9297381434,1433.92947415412,1434.92921016484,1435.92894617556,
1436.92868218628,1437.928418197,1438.92815420772,1439.92789021844,1440.92762622916,
1441.92736223988,1442.9270982506,1443.92683426132,1444.92657027204,1445.92630628276,
1446.92604229348,1447.9257783042,1448.92551431492,1449.92525032564,1450.92498633636,
1451.92472234708,1452.9244583578,1453.92419436852,1454.92393037924,1455.92366638996,
1456.92340240068,1457.9231384114,1458.92287442212,1459.92261043284,1460.92234644356,
1461.92208245428,1462.921818465,1463.92155447572,1464.92129048644,1465.92102649716,
1466.92076250788,1467.9204985186,1468.92023452932,1469.91997054004,1470.91970655076,
1471.91944256148,1472.9191785722,1473.91891458292,1474.91865059364,1475.91838660436,
1476.91812261508,1477.9178586258,1478.91759463652,1479.91733064724,1480.91706665796,
1481.91680266868,1482.9165386794,1483.91627469012,1484.91601070084,1485.91574671156,
1486.91548272228,1487.915218733,1488.91495474372,1489.91469075444,1490.91442676516,
1491.91416277588,1492.9138987866,1493.91363479732,1494.91337080804,1495.91310681876,
1496.91284282948,1497.9125788402,1498.91231485092,1499.91205086164,1500.91178687236,
1501.91152288309,1502.91125889381,1503.91099490453,1504.91073091525,1505.91046692597,
1506.91020293669,1507.90993894741,1508.90967495813,1509.90941096885,1510.90914697957,
1511.90888299029,1512.90861900101,1513.90835501173,1514.90809102245,1515.90782703317,
1516.90756304389,1517.90729905461,1518.90703506533,1519.90677107605,1520.90650708677,
1521.90624309749,1522.90597910821,1523.90571511893,1524.90545112965,1525.90518714037,
1526.90492315109,1527.90465916181,1528.90439517253,1529.90413118325,1530.90386719397,
1531.90360320469,1532.90333921541,1533.90307522613,1534.90281123685,1535.90254724757,
1536.90228325829,1537.90201926901,1538.90175527973,1539.90149129045,1540.90122730117,
1541.90096331189,1542.90069932261,1543.90043533333,1544.90017134405,1545.89990735477,
1546.89964336549,1547.89937937621,1548.89911538693,1549.89885139765,1550.89858740837,
1551.89832341909,1552.89805942981,1553.89779544053,1554.89753145125,1555.89726746197,
1556.89700347269,1557.89673948341,1558.89647549413,1559.89621150485,1560.89594751557,
1561.89568352629,1562.89541953701,1563.89515554773,1564.89489155845,1565.89462756917,
1566.89436357989,1567.89409959061,1568.89383560133,1569.89357161205,1570.89330762277,
1571.89304363349,1572.89277964421,1573.89251565493,1574.89225166565,1575.89198767637,
1576.89172368709,1577.89145969781,1578.89119570853,1579.89093171926,1580.89066772998,
1581.8904037407,1582.89013975142,1583.88987576214,1584.88961177286,1585.88934778358,
1586.8890837943,1587.88881980502,1588.88855581574,1589.88829182646,1590.88802783718,
1591.8877638479,1592.88749985862,1593.88723586934,1594.88697188006,1595.88670789078,
1596.8864439015,1597.88617991222,1598.88591592294,1599.88565193366,1600.88538794438,
1601.8851239551,1602.88485996582,1603.88459597654,1604.88433198726,1605.88406799798,
1606.8838040087,1607.88354001942,1608.88327603014,1609.88301204086,1610.88274805158,
1611.8824840623,1612.88222007302,1613.88195608374,1614.88169209446,1615.88142810518,
1616.8811641159,1617.88090012662,1618.88063613734,1619.88037214806,1620.88010815878,
1621.8798441695,1622.87958018022,1623.87931619094,1624.87905220166,1625.87878821238,
1626.8785242231,1627.87826023382,1628.87799624454,1629.87773225526,1630.87746826598,
1631.8772042767,1632.87694028742,1633.87667629814,1634.87641230886,1635.87614831958,
1636.8758843303,1637.87562034102,1638.87535635174,1639.87509236246,1640.87482837318,
1641.8745643839,1642.87430039462,1643.87403640534,1644.87377241606,1645.87350842678,
1646.8732444375,1647.87298044822,1648.87271645894,1649.87245246966,1650.87218848038,
1651.8719244911,1652.87166050182,1653.87139651254,1654.87113252326,1655.87086853399,
1656.8706045447,1657.87034055543,1658.87007656615,1659.86981257687,1660.86954858759,
1661.86928459831,1662.86902060903,1663.86875661975,1664.86849263047,1665.86822864119,
1666.86796465191,1667.86770066263,1668.86743667335,1669.86717268407,1670.86690869479,
1671.86664470551,1672.86638071623,1673.86611672695,1674.86585273767,1675.86558874839,
1676.86532475911,1677.86506076983,1678.86479678055,1679.86453279127,1680.86426880199,
1681.86400481271,1682.86374082343,1683.86347683415,1684.86321284487,1685.86294885559,
1686.86268486631,1687.86242087703,1688.86215688775,1689.86189289847,1690.86162890919,
1691.86136491991,1692.86110093063,1693.86083694135,1694.86057295207,1695.86030896279,
1696.86004497351,1697.35991297887,1697.85988790214),.UNSPECIFIED.);
#55=B_SPLINE_SURFACE_WITH_KNOTS('',3,3,((#265391,#265392,#265393,#265394,
#265395,#265396,#265397,#265398,#265399,#265400,#265401,#265402,#265403,
#265404,#265405,#265406,#265407,#265408,#265409,#265410,#265411,#265412,
#265413,#265414,#265415,#265416,#265417,#265418,#265419,#265420,#265421,
#265422,#265423,#265424,#265425,#265426,#265427,#265428,#265429,#265430,
#265431,#265432,#265433,#265434,#265435,#265436,#265437,#265438,#265439,
#265440,#265441,#265442,#265443,#265444,#265445,#265446,#265447,#265448,
#265449,#265450,#265451,#265452,#265453,#265454,#265455,#265456,#265457,
#265458,#265459,#265460,#265461,#265462,#265463,#265464,#265465,#265466,
#265467,#265468,#265469,#265470,#265471,#265472,#265473,#265474,#265475,
#265476,#265477,#265478,#265479,#265480,#265481,#265482,#265483,#265484,
#265485,#265486,#265487,#265488,#265489,#265490,#265491,#265492,#265493,
#265494,#265495,#265496,#265497,#265498,#265499,#265500,#265501,#265502,
#265503,#265504,#265505,#265506,#265507,#265508,#265509,#265510,#265511,
#265512,#265513,#265514,#265515,#265516,#265517,#265518,#265519,#265520,
#265521,#265522,#265523,#265524,#265525,#265526,#265527,#265528,#265529,
#265530,#265531,#265532,#265533,#265534,#265535,#265536,#265537,#265538,
#265539,#265540,#265541,#265542,#265543,#265544,#265545,#265546,#265547,
#265548,#265549,#265550,#265551,#265552,#265553,#265554,#265555,#265556,
#265557,#265558,#265559,#265560,#265561,#265562,#265563,#265564,#265565,
#265566,#265567,#265568,#265569,#265570,#265571,#265572,#265573,#265574,
#265575,#265576,#265577,#265578,#265579,#265580,#265581,#265582,#265583,
#265584,#265585,#265586,#265587,#265588,#265589,#265590,#265591,#265592,
#265593,#265594,#265595,#265596,#265597,#265598,#265599,#265600,#265601,
#265602,#265603,#265604,#265605,#265606,#265607,#265608,#265609,#265610,
#265611,#265612,#265613,#265614,#265615,#265616,#265617,#265618,#265619,
#265620,#265621,#265622,#265623,#265624,#265625,#265626,#265627,#265628,
#265629,#265630,#265631,#265632,#265633,#265634,#265635,#265636,#265637,
#265638,#265639,#265640,#265641,#265642,#265643,#265644,#265645,#265646,
#265647,#265648,#265649,#265650,#265651,#265652,#265653,#265654,#265655,
#265656,#265657,#265658,#265659,#265660,#265661,#265662,#265663,#265664,
#265665,#265666,#265667,#265668,#265669,#265670,#265671,#265672,#265673,
#265674,#265675,#265676,#265677,#265678,#265679,#265680,#265681,#265682,
#265683,#265684,#265685,#265686,#265687,#265688,#265689,#265690,#265691,
#265692,#265693,#265694,#265695,#265696,#265697,#265698,#265699,#265700,
#265701,#265702,#265703,#265704,#265705,#265706,#265707,#265708,#265709,
#265710,#265711,#265712,#265713,#265714,#265715,#265716,#265717,#265718,
#265719,#265720,#265721,#265722,#265723,#265724,#265725,#265726,#265727,
#265728,#265729,#265730,#265731,#265732,#265733,#265734,#265735,#265736,
#265737,#265738,#265739,#265740,#265741,#265742,#265743,#265744,#265745,
#265746,#265747,#265748,#265749,#265750,#265751,#265752,#265753,#265754,
#265755,#265756,#265757,#265758,#265759,#265760,#265761,#265762,#265763,
#265764,#265765,#265766,#265767,#265768,#265769,#265770,#265771,#265772,
#265773,#265774,#265775,#265776,#265777,#265778,#265779,#265780,#265781,
#265782,#265783,#265784,#265785,#265786,#265787,#265788,#265789,#265790,
#265791,#265792,#265793,#265794,#265795,#265796,#265797,#265798,#265799,
#265800,#265801,#265802,#265803,#265804,#265805,#265806,#265807,#265808,
#265809,#265810,#265811,#265812,#265813,#265814,#265815,#265816,#265817,
#265818,#265819,#265820,#265821,#265822,#265823,#265824,#265825,#265826,
#265827,#265828,#265829,#265830,#265831,#265832,#265833,#265834,#265835,
#265836,#265837,#265838,#265839,#265840,#265841,#265842,#265843,#265844,
#265845,#265846,#265847,#265848,#265849,#265850,#265851,#265852,#265853,
#265854,#265855,#265856,#265857,#265858,#265859,#265860,#265861,#265862,
#265863,#265864,#265865,#265866,#265867,#265868,#265869,#265870,#265871,
#265872,#265873,#265874,#265875,#265876,#265877,#265878,#265879,#265880,
#265881,#265882,#265883,#265884,#265885,#265886,#265887,#265888,#265889,
#265890,#265891,#265892,#265893,#265894,#265895,#265896,#265897,#265898,
#265899,#265900,#265901,#265902,#265903,#265904,#265905,#265906,#265907,
#265908,#265909,#265910,#265911,#265912,#265913,#265914,#265915,#265916,
#265917,#265918,#265919,#265920,#265921,#265922,#265923,#265924,#265925,
#265926,#265927,#265928,#265929,#265930,#265931,#265932,#265933,#265934,
#265935,#265936,#265937,#265938,#265939,#265940,#265941,#265942,#265943,
#265944,#265945,#265946,#265947,#265948,#265949,#265950,#265951,#265952,
#265953,#265954,#265955,#265956,#265957,#265958,#265959,#265960,#265961,
#265962,#265963,#265964,#265965,#265966,#265967,#265968,#265969,#265970,
#265971,#265972,#265973,#265974,#265975,#265976,#265977,#265978,#265979,
#265980,#265981,#265982,#265983,#265984,#265985,#265986,#265987,#265988,
#265989,#265990,#265991,#265992,#265993,#265994,#265995,#265996,#265997,
#265998,#265999,#266000,#266001,#266002,#266003,#266004,#266005,#266006,
#266007,#266008,#266009,#266010,#266011,#266012,#266013,#266014,#266015,
#266016,#266017,#266018,#266019,#266020,#266021,#266022,#266023,#266024,
#266025,#266026,#266027,#266028,#266029,#266030,#266031,#266032,#266033,
#266034,#266035,#266036,#266037,#266038,#266039,#266040,#266041,#266042,
#266043,#266044,#266045,#266046,#266047,#266048,#266049,#266050,#266051,
#266052,#266053,#266054,#266055,#266056,#266057,#266058,#266059,#266060,
#266061,#266062,#266063,#266064,#266065,#266066,#266067,#266068,#266069,
#266070,#266071,#266072,#266073,#266074,#266075,#266076,#266077,#266078,
#266079,#266080,#266081,#266082,#266083,#266084,#266085,#266086,#266087,
#266088,#266089,#266090,#266091,#266092,#266093,#266094,#266095,#266096,
#266097,#266098,#266099,#266100,#266101,#266102,#266103,#266104,#266105,
#266106,#266107,#266108,#266109,#266110,#266111,#266112,#266113,#266114,
#266115,#266116,#266117,#266118,#266119,#266120,#266121,#266122,#266123,
#266124,#266125,#266126,#266127,#266128,#266129,#266130,#266131,#266132,
#266133,#266134,#266135,#266136,#266137,#266138,#266139,#266140,#266141,
#266142,#266143,#266144,#266145,#266146,#266147,#266148,#266149,#266150,
#266151,#266152,#266153,#266154,#266155,#266156,#266157,#266158,#266159,
#266160,#266161,#266162,#266163,#266164,#266165,#266166,#266167,#266168,
#266169,#266170,#266171,#266172,#266173,#266174,#266175,#266176,#266177,
#266178,#266179,#266180,#266181,#266182,#266183,#266184,#266185,#266186,
#266187,#266188,#266189,#266190,#266191,#266192,#266193,#266194,#266195,
#266196,#266197,#266198,#266199,#266200,#266201,#266202,#266203,#266204,
#266205,#266206,#266207,#266208,#266209,#266210,#266211,#266212,#266213,
#266214,#266215,#266216,#266217,#266218,#266219,#266220,#266221,#266222,
#266223,#266224,#266225,#266226,#266227,#266228,#266229,#266230,#266231,
#266232,#266233,#266234,#266235,#266236,#266237,#266238,#266239,#266240,
#266241,#266242,#266243,#266244,#266245,#266246,#266247,#266248,#266249,
#266250,#266251,#266252,#266253,#266254,#266255,#266256,#266257,#266258,
#266259,#266260,#266261,#266262,#266263,#266264,#266265,#266266,#266267,
#266268,#266269,#266270,#266271,#266272,#266273,#266274,#266275,#266276,
#266277,#266278,#266279,#266280,#266281,#266282,#266283,#266284,#266285,
#266286,#266287,#266288,#266289,#266290,#266291,#266292,#266293,#266294,
#266295,#266296,#266297,#266298,#266299,#266300,#266301,#266302,#266303,
#266304,#266305,#266306,#266307,#266308,#266309,#266310,#266311,#266312,
#266313,#266314,#266315,#266316,#266317,#266318,#266319,#266320,#266321,
#266322,#266323,#266324,#266325,#266326,#266327,#266328,#266329,#266330,
#266331,#266332,#266333,#266334,#266335,#266336,#266337,#266338,#266339,
#266340,#266341,#266342,#266343,#266344,#266345,#266346,#266347,#266348,
#266349,#266350,#266351,#266352,#266353,#266354,#266355,#266356,#266357,
#266358,#266359,#266360,#266361,#266362,#266363,#266364,#266365,#266366,
#266367,#266368,#266369,#266370,#266371,#266372,#266373,#266374,#266375,
#266376,#266377,#266378,#266379,#266380,#266381,#266382,#266383,#266384,
#266385,#266386,#266387,#266388,#266389,#266390,#266391,#266392,#266393,
#266394,#266395,#266396,#266397,#266398,#266399,#266400,#266401,#266402,
#266403,#266404,#266405,#266406,#266407,#266408,#266409,#266410,#266411,
#266412,#266413,#266414,#266415,#266416,#266417,#266418,#266419,#266420,
#266421,#266422,#266423,#266424,#266425,#266426,#266427,#266428,#266429,
#266430,#266431,#266432,#266433,#266434,#266435,#266436,#266437,#266438,
#266439,#266440,#266441,#266442,#266443,#266444,#266445,#266446,#266447,
#266448,#266449,#266450,#266451,#266452,#266453,#266454,#266455,#266456,
#266457,#266458,#266459,#266460,#266461,#266462,#266463,#266464,#266465,
#266466,#266467,#266468,#266469,#266470,#266471,#266472,#266473,#266474,
#266475,#266476,#266477,#266478,#266479,#266480,#266481,#266482,#266483,
#266484,#266485,#266486,#266487,#266488,#266489,#266490,#266491,#266492,
#266493,#266494,#266495,#266496,#266497,#266498,#266499,#266500,#266501,
#266502,#266503,#266504,#266505,#266506,#266507,#266508,#266509,#266510,
#266511,#266512,#266513,#266514,#266515,#266516,#266517,#266518,#266519,
#266520,#266521,#266522,#266523,#266524,#266525,#266526,#266527,#266528,
#266529,#266530,#266531,#266532,#266533,#266534,#266535,#266536,#266537,
#266538,#266539,#266540,#266541,#266542,#266543,#266544,#266545,#266546,
#266547,#266548,#266549,#266550,#266551,#266552,#266553,#266554,#266555,
#266556,#266557,#266558,#266559,#266560,#266561,#266562,#266563,#266564,
#266565,#266566,#266567,#266568,#266569,#266570,#266571,#266572,#266573,
#266574,#266575,#266576,#266577,#266578,#266579,#266580,#266581,#266582,
#266583,#266584,#266585,#266586,#266587,#266588,#266589,#266590,#266591,
#266592,#266593,#266594,#266595,#266596,#266597,#266598,#266599,#266600,
#266601,#266602,#266603,#266604,#266605,#266606,#266607,#266608,#266609,
#266610,#266611,#266612,#266613,#266614,#266615,#266616,#266617,#266618,
#266619,#266620,#266621,#266622,#266623,#266624,#266625,#266626,#266627,
#266628,#266629,#266630,#266631,#266632,#266633,#266634,#266635,#266636,
#266637,#266638,#266639,#266640,#266641,#266642,#266643,#266644,#266645,
#266646,#266647,#266648,#266649,#266650,#266651,#266652,#266653,#266654,
#266655,#266656,#266657,#266658,#266659,#266660,#266661,#266662,#266663,
#266664,#266665,#266666,#266667,#266668,#266669,#266670,#266671,#266672,
#266673,#266674,#266675,#266676,#266677,#266678,#266679,#266680,#266681,
#266682,#266683,#266684,#266685,#266686,#266687,#266688,#266689,#266690,
#266691,#266692,#266693,#266694,#266695,#266696,#266697,#266698,#266699,
#266700,#266701,#266702,#266703,#266704,#266705,#266706,#266707,#266708,
#266709,#266710,#266711,#266712,#266713,#266714,#266715,#266716,#266717,
#266718,#266719,#266720,#266721,#266722,#266723,#266724,#266725,#266726,
#266727,#266728,#266729,#266730,#266731,#266732,#266733,#266734,#266735,
#266736,#266737,#266738,#266739,#266740,#266741,#266742,#266743,#266744,
#266745,#266746,#266747,#266748,#266749,#266750,#266751,#266752,#266753,
#266754,#266755,#266756,#266757,#266758,#266759,#266760,#266761,#266762,
#266763,#266764,#266765,#266766,#266767,#266768,#266769,#266770,#266771,
#266772,#266773,#266774,#266775,#266776,#266777,#266778,#266779,#266780,
#266781,#266782,#266783,#266784,#266785,#266786,#266787,#266788,#266789,
#266790,#266791,#266792,#266793,#266794,#266795,#266796,#266797,#266798,
#266799,#266800,#266801,#266802,#266803,#266804,#266805,#266806,#266807,
#266808,#266809,#266810,#266811,#266812,#266813,#266814,#266815,#266816,
#266817,#266818,#266819,#266820,#266821,#266822,#266823,#266824,#266825,
#266826,#266827,#266828,#266829,#266830,#266831,#266832,#266833,#266834,
#266835,#266836,#266837,#266838,#266839,#266840,#266841,#266842,#266843,
#266844,#266845,#266846,#266847,#266848,#266849,#266850,#266851,#266852,
#266853,#266854,#266855,#266856,#266857,#266858,#266859,#266860,#266861,
#266862,#266863,#266864,#266865,#266866,#266867,#266868,#266869,#266870,
#266871,#266872,#266873,#266874,#266875,#266876,#266877,#266878,#266879,
#266880,#266881,#266882,#266883,#266884,#266885,#266886,#266887,#266888,
#266889,#266890,#266891,#266892,#266893,#266894,#266895,#266896,#266897,
#266898,#266899,#266900,#266901,#266902,#266903,#266904,#266905,#266906,
#266907,#266908,#266909,#266910,#266911,#266912,#266913,#266914,#266915,
#266916,#266917,#266918,#266919,#266920,#266921,#266922,#266923,#266924,
#266925,#266926,#266927,#266928,#266929,#266930,#266931,#266932,#266933,
#266934,#266935,#266936,#266937,#266938,#266939,#266940,#266941,#266942,
#266943,#266944,#266945,#266946,#266947,#266948,#266949,#266950,#266951,
#266952,#266953,#266954,#266955,#266956,#266957,#266958,#266959,#266960,
#266961,#266962,#266963,#266964,#266965,#266966,#266967,#266968,#266969,
#266970,#266971,#266972,#266973,#266974,#266975,#266976,#266977,#266978,
#266979,#266980,#266981,#266982,#266983,#266984,#266985,#266986,#266987,
#266988,#266989,#266990,#266991,#266992,#266993,#266994,#266995,#266996,
#266997,#266998,#266999,#267000,#267001,#267002,#267003,#267004,#267005,
#267006,#267007,#267008,#267009,#267010,#267011,#267012,#267013,#267014,
#267015,#267016,#267017,#267018,#267019,#267020,#267021,#267022,#267023,
#267024,#267025,#267026,#267027,#267028,#267029,#267030,#267031,#267032,
#267033,#267034,#267035,#267036,#267037,#267038,#267039,#267040,#267041,
#267042,#267043,#267044,#267045,#267046,#267047,#267048,#267049,#267050,
#267051,#267052,#267053,#267054,#267055,#267056,#267057,#267058,#267059,
#267060,#267061,#267062,#267063,#267064,#267065,#267066,#267067,#267068,
#267069,#267070,#267071,#267072,#267073,#267074,#267075,#267076,#267077,
#267078,#267079,#267080,#267081,#267082,#267083,#267084,#267085),(#267086,
#267087,#267088,#267089,#267090,#267091,#267092,#267093,#267094,#267095,
#267096,#267097,#267098,#267099,#267100,#267101,#267102,#267103,#267104,
#267105,#267106,#267107,#267108,#267109,#267110,#267111,#267112,#267113,
#267114,#267115,#267116,#267117,#267118,#267119,#267120,#267121,#267122,
#267123,#267124,#267125,#267126,#267127,#267128,#267129,#267130,#267131,
#267132,#267133,#267134,#267135,#267136,#267137,#267138,#267139,#267140,
#267141,#267142,#267143,#267144,#267145,#267146,#267147,#267148,#267149,
#267150,#267151,#267152,#267153,#267154,#267155,#267156,#267157,#267158,
#267159,#267160,#267161,#267162,#267163,#267164,#267165,#267166,#267167,
#267168,#267169,#267170,#267171,#267172,#267173,#267174,#267175,#267176,
#267177,#267178,#267179,#267180,#267181,#267182,#267183,#267184,#267185,
#267186,#267187,#267188,#267189,#267190,#267191,#267192,#267193,#267194,
#267195,#267196,#267197,#267198,#267199,#267200,#267201,#267202,#267203,
#267204,#267205,#267206,#267207,#267208,#267209,#267210,#267211,#267212,
#267213,#267214,#267215,#267216,#267217,#267218,#267219,#267220,#267221,
#267222,#267223,#267224,#267225,#267226,#267227,#267228,#267229,#267230,
#267231,#267232,#267233,#267234,#267235,#267236,#267237,#267238,#267239,
#267240,#267241,#267242,#267243,#267244,#267245,#267246,#267247,#267248,
#267249,#267250,#267251,#267252,#267253,#267254,#267255,#267256,#267257,
#267258,#267259,#267260,#267261,#267262,#267263,#267264,#267265,#267266,
#267267,#267268,#267269,#267270,#267271,#267272,#267273,#267274,#267275,
#267276,#267277,#267278,#267279,#267280,#267281,#267282,#267283,#267284,
#267285,#267286,#267287,#267288,#267289,#267290,#267291,#267292,#267293,
#267294,#267295,#267296,#267297,#267298,#267299,#267300,#267301,#267302,
#267303,#267304,#267305,#267306,#267307,#267308,#267309,#267310,#267311,
#267312,#267313,#267314,#267315,#267316,#267317,#267318,#267319,#267320,
#267321,#267322,#267323,#267324,#267325,#267326,#267327,#267328,#267329,
#267330,#267331,#267332,#267333,#267334,#267335,#267336,#267337,#267338,
#267339,#267340,#267341,#267342,#267343,#267344,#267345,#267346,#267347,
#267348,#267349,#267350,#267351,#267352,#267353,#267354,#267355,#267356,
#267357,#267358,#267359,#267360,#267361,#267362,#267363,#267364,#267365,
#267366,#267367,#267368,#267369,#267370,#267371,#267372,#267373,#267374,
#267375,#267376,#267377,#267378,#267379,#267380,#267381,#267382,#267383,
#267384,#267385,#267386,#267387,#267388,#267389,#267390,#267391,#267392,
#267393,#267394,#267395,#267396,#267397,#267398,#267399,#267400,#267401,
#267402,#267403,#267404,#267405,#267406,#267407,#267408,#267409,#267410,
#267411,#267412,#267413,#267414,#267415,#267416,#267417,#267418,#267419,
#267420,#267421,#267422,#267423,#267424,#267425,#267426,#267427,#267428,
#267429,#267430,#267431,#267432,#267433,#267434,#267435,#267436,#267437,
#267438,#267439,#267440,#267441,#267442,#267443,#267444,#267445,#267446,
#267447,#267448,#267449,#267450,#267451,#267452,#267453,#267454,#267455,
#267456,#267457,#267458,#267459,#267460,#267461,#267462,#267463,#267464,
#267465,#267466,#267467,#267468,#267469,#267470,#267471,#267472,#267473,
#267474,#267475,#267476,#267477,#267478,#267479,#267480,#267481,#267482,
#267483,#267484,#267485,#267486,#267487,#267488,#267489,#267490,#267491,
#267492,#267493,#267494,#267495,#267496,#267497,#267498,#267499,#267500,
#267501,#267502,#267503,#267504,#267505,#267506,#267507,#267508,#267509,
#267510,#267511,#267512,#267513,#267514,#267515,#267516,#267517,#267518,
#267519,#267520,#267521,#267522,#267523,#267524,#267525,#267526,#267527,
#267528,#267529,#267530,#267531,#267532,#267533,#267534,#267535,#267536,
#267537,#267538,#267539,#267540,#267541,#267542,#267543,#267544,#267545,
#267546,#267547,#267548,#267549,#267550,#267551,#267552,#267553,#267554,
#267555,#267556,#267557,#267558,#267559,#267560,#267561,#267562,#267563,
#267564,#267565,#267566,#267567,#267568,#267569,#267570,#267571,#267572,
#267573,#267574,#267575,#267576,#267577,#267578,#267579,#267580,#267581,
#267582,#267583,#267584,#267585,#267586,#267587,#267588,#267589,#267590,
#267591,#267592,#267593,#267594,#267595,#267596,#267597,#267598,#267599,
#267600,#267601,#267602,#267603,#267604,#267605,#267606,#267607,#267608,
#267609,#267610,#267611,#267612,#267613,#267614,#267615,#267616,#267617,
#267618,#267619,#267620,#267621,#267622,#267623,#267624,#267625,#267626,
#267627,#267628,#267629,#267630,#267631,#267632,#267633,#267634,#267635,
#267636,#267637,#267638,#267639,#267640,#267641,#267642,#267643,#267644,
#267645,#267646,#267647,#267648,#267649,#267650,#267651,#267652,#267653,
#267654,#267655,#267656,#267657,#267658,#267659,#267660,#267661,#267662,
#267663,#267664,#267665,#267666,#267667,#267668,#267669,#267670,#267671,
#267672,#267673,#267674,#267675,#267676,#267677,#267678,#267679,#267680,
#267681,#267682,#267683,#267684,#267685,#267686,#267687,#267688,#267689,
#267690,#267691,#267692,#267693,#267694,#267695,#267696,#267697,#267698,
#267699,#267700,#267701,#267702,#267703,#267704,#267705,#267706,#267707,
#267708,#267709,#267710,#267711,#267712,#267713,#267714,#267715,#267716,
#267717,#267718,#267719,#267720,#267721,#267722,#267723,#267724,#267725,
#267726,#267727,#267728,#267729,#267730,#267731,#267732,#267733,#267734,
#267735,#267736,#267737,#267738,#267739,#267740,#267741,#267742,#267743,
#267744,#267745,#267746,#267747,#267748,#267749,#267750,#267751,#267752,
#267753,#267754,#267755,#267756,#267757,#267758,#267759,#267760,#267761,
#267762,#267763,#267764,#267765,#267766,#267767,#267768,#267769,#267770,
#267771,#267772,#267773,#267774,#267775,#267776,#267777,#267778,#267779,
#267780,#267781,#267782,#267783,#267784,#267785,#267786,#267787,#267788,
#267789,#267790,#267791,#267792,#267793,#267794,#267795,#267796,#267797,
#267798,#267799,#267800,#267801,#267802,#267803,#267804,#267805,#267806,
#267807,#267808,#267809,#267810,#267811,#267812,#267813,#267814,#267815,
#267816,#267817,#267818,#267819,#267820,#267821,#267822,#267823,#267824,
#267825,#267826,#267827,#267828,#267829,#267830,#267831,#267832,#267833,
#267834,#267835,#267836,#267837,#267838,#267839,#267840,#267841,#267842,
#267843,#267844,#267845,#267846,#267847,#267848,#267849,#267850,#267851,
#267852,#267853,#267854,#267855,#267856,#267857,#267858,#267859,#267860,
#267861,#267862,#267863,#267864,#267865,#267866,#267867,#267868,#267869,
#267870,#267871,#267872,#267873,#267874,#267875,#267876,#267877,#267878,
#267879,#267880,#267881,#267882,#267883,#267884,#267885,#267886,#267887,
#267888,#267889,#267890,#267891,#267892,#267893,#267894,#267895,#267896,
#267897,#267898,#267899,#267900,#267901,#267902,#267903,#267904,#267905,
#267906,#267907,#267908,#267909,#267910,#267911,#267912,#267913,#267914,
#267915,#267916,#267917,#267918,#267919,#267920,#267921,#267922,#267923,
#267924,#267925,#267926,#267927,#267928,#267929,#267930,#267931,#267932,
#267933,#267934,#267935,#267936,#267937,#267938,#267939,#267940,#267941,
#267942,#267943,#267944,#267945,#267946,#267947,#267948,#267949,#267950,
#267951,#267952,#267953,#267954,#267955,#267956,#267957,#267958,#267959,
#267960,#267961,#267962,#267963,#267964,#267965,#267966,#267967,#267968,
#267969,#267970,#267971,#267972,#267973,#267974,#267975,#267976,#267977,
#267978,#267979,#267980,#267981,#267982,#267983,#267984,#267985,#267986,
#267987,#267988,#267989,#267990,#267991,#267992,#267993,#267994,#267995,
#267996,#267997,#267998,#267999,#268000,#268001,#268002,#268003,#268004,
#268005,#268006,#268007,#268008,#268009,#268010,#268011,#268012,#268013,
#268014,#268015,#268016,#268017,#268018,#268019,#268020,#268021,#268022,
#268023,#268024,#268025,#268026,#268027,#268028,#268029,#268030,#268031,
#268032,#268033,#268034,#268035,#268036,#268037,#268038,#268039,#268040,
#268041,#268042,#268043,#268044,#268045,#268046,#268047,#268048,#268049,
#268050,#268051,#268052,#268053,#268054,#268055,#268056,#268057,#268058,
#268059,#268060,#268061,#268062,#268063,#268064,#268065,#268066,#268067,
#268068,#268069,#268070,#268071,#268072,#268073,#268074,#268075,#268076,
#268077,#268078,#268079,#268080,#268081,#268082,#268083,#268084,#268085,
#268086,#268087,#268088,#268089,#268090,#268091,#268092,#268093,#268094,
#268095,#268096,#268097,#268098,#268099,#268100,#268101,#268102,#268103,
#268104,#268105,#268106,#268107,#268108,#268109,#268110,#268111,#268112,
#268113,#268114,#268115,#268116,#268117,#268118,#268119,#268120,#268121,
#268122,#268123,#268124,#268125,#268126,#268127,#268128,#268129,#268130,
#268131,#268132,#268133,#268134,#268135,#268136,#268137,#268138,#268139,
#268140,#268141,#268142,#268143,#268144,#268145,#268146,#268147,#268148,
#268149,#268150,#268151,#268152,#268153,#268154,#268155,#268156,#268157,
#268158,#268159,#268160,#268161,#268162,#268163,#268164,#268165,#268166,
#268167,#268168,#268169,#268170,#268171,#268172,#268173,#268174,#268175,
#268176,#268177,#268178,#268179,#268180,#268181,#268182,#268183,#268184,
#268185,#268186,#268187,#268188,#268189,#268190,#268191,#268192,#268193,
#268194,#268195,#268196,#268197,#268198,#268199,#268200,#268201,#268202,
#268203,#268204,#268205,#268206,#268207,#268208,#268209,#268210,#268211,
#268212,#268213,#268214,#268215,#268216,#268217,#268218,#268219,#268220,
#268221,#268222,#268223,#268224,#268225,#268226,#268227,#268228,#268229,
#268230,#268231,#268232,#268233,#268234,#268235,#268236,#268237,#268238,
#268239,#268240,#268241,#268242,#268243,#268244,#268245,#268246,#268247,
#268248,#268249,#268250,#268251,#268252,#268253,#268254,#268255,#268256,
#268257,#268258,#268259,#268260,#268261,#268262,#268263,#268264,#268265,
#268266,#268267,#268268,#268269,#268270,#268271,#268272,#268273,#268274,
#268275,#268276,#268277,#268278,#268279,#268280,#268281,#268282,#268283,
#268284,#268285,#268286,#268287,#268288,#268289,#268290,#268291,#268292,
#268293,#268294,#268295,#268296,#268297,#268298,#268299,#268300,#268301,
#268302,#268303,#268304,#268305,#268306,#268307,#268308,#268309,#268310,
#268311,#268312,#268313,#268314,#268315,#268316,#268317,#268318,#268319,
#268320,#268321,#268322,#268323,#268324,#268325,#268326,#268327,#268328,
#268329,#268330,#268331,#268332,#268333,#268334,#268335,#268336,#268337,
#268338,#268339,#268340,#268341,#268342,#268343,#268344,#268345,#268346,
#268347,#268348,#268349,#268350,#268351,#268352,#268353,#268354,#268355,
#268356,#268357,#268358,#268359,#268360,#268361,#268362,#268363,#268364,
#268365,#268366,#268367,#268368,#268369,#268370,#268371,#268372,#268373,
#268374,#268375,#268376,#268377,#268378,#268379,#268380,#268381,#268382,
#268383,#268384,#268385,#268386,#268387,#268388,#268389,#268390,#268391,
#268392,#268393,#268394,#268395,#268396,#268397,#268398,#268399,#268400,
#268401,#268402,#268403,#268404,#268405,#268406,#268407,#268408,#268409,
#268410,#268411,#268412,#268413,#268414,#268415,#268416,#268417,#268418,
#268419,#268420,#268421,#268422,#268423,#268424,#268425,#268426,#268427,
#268428,#268429,#268430,#268431,#268432,#268433,#268434,#268435,#268436,
#268437,#268438,#268439,#268440,#268441,#268442,#268443,#268444,#268445,
#268446,#268447,#268448,#268449,#268450,#268451,#268452,#268453,#268454,
#268455,#268456,#268457,#268458,#268459,#268460,#268461,#268462,#268463,
#268464,#268465,#268466,#268467,#268468,#268469,#268470,#268471,#268472,
#268473,#268474,#268475,#268476,#268477,#268478,#268479,#268480,#268481,
#268482,#268483,#268484,#268485,#268486,#268487,#268488,#268489,#268490,
#268491,#268492,#268493,#268494,#268495,#268496,#268497,#268498,#268499,
#268500,#268501,#268502,#268503,#268504,#268505,#268506,#268507,#268508,
#268509,#268510,#268511,#268512,#268513,#268514,#268515,#268516,#268517,
#268518,#268519,#268520,#268521,#268522,#268523,#268524,#268525,#268526,
#268527,#268528,#268529,#268530,#268531,#268532,#268533,#268534,#268535,
#268536,#268537,#268538,#268539,#268540,#268541,#268542,#268543,#268544,
#268545,#268546,#268547,#268548,#268549,#268550,#268551,#268552,#268553,
#268554,#268555,#268556,#268557,#268558,#268559,#268560,#268561,#268562,
#268563,#268564,#268565,#268566,#268567,#268568,#268569,#268570,#268571,
#268572,#268573,#268574,#268575,#268576,#268577,#268578,#268579,#268580,
#268581,#268582,#268583,#268584,#268585,#268586,#268587,#268588,#268589,
#268590,#268591,#268592,#268593,#268594,#268595,#268596,#268597,#268598,
#268599,#268600,#268601,#268602,#268603,#268604,#268605,#268606,#268607,
#268608,#268609,#268610,#268611,#268612,#268613,#268614,#268615,#268616,
#268617,#268618,#268619,#268620,#268621,#268622,#268623,#268624,#268625,
#268626,#268627,#268628,#268629,#268630,#268631,#268632,#268633,#268634,
#268635,#268636,#268637,#268638,#268639,#268640,#268641,#268642,#268643,
#268644,#268645,#268646,#268647,#268648,#268649,#268650,#268651,#268652,
#268653,#268654,#268655,#268656,#268657,#268658,#268659,#268660,#268661,
#268662,#268663,#268664,#268665,#268666,#268667,#268668,#268669,#268670,
#268671,#268672,#268673,#268674,#268675,#268676,#268677,#268678,#268679,
#268680,#268681,#268682,#268683,#268684,#268685,#268686,#268687,#268688,
#268689,#268690,#268691,#268692,#268693,#268694,#268695,#268696,#268697,
#268698,#268699,#268700,#268701,#268702,#268703,#268704,#268705,#268706,
#268707,#268708,#268709,#268710,#268711,#268712,#268713,#268714,#268715,
#268716,#268717,#268718,#268719,#268720,#268721,#268722,#268723,#268724,
#268725,#268726,#268727,#268728,#268729,#268730,#268731,#268732,#268733,
#268734,#268735,#268736,#268737,#268738,#268739,#268740,#268741,#268742,
#268743,#268744,#268745,#268746,#268747,#268748,#268749,#268750,#268751,
#268752,#268753,#268754,#268755,#268756,#268757,#268758,#268759,#268760,
#268761,#268762,#268763,#268764,#268765,#268766,#268767,#268768,#268769,
#268770,#268771,#268772,#268773,#268774,#268775,#268776,#268777,#268778,
#268779,#268780),(#268781,#268782,#268783,#268784,#268785,#268786,#268787,
#268788,#268789,#268790,#268791,#268792,#268793,#268794,#268795,#268796,
#268797,#268798,#268799,#268800,#268801,#268802,#268803,#268804,#268805,
#268806,#268807,#268808,#268809,#268810,#268811,#268812,#268813,#268814,
#268815,#268816,#268817,#268818,#268819,#268820,#268821,#268822,#268823,
#268824,#268825,#268826,#268827,#268828,#268829,#268830,#268831,#268832,
#268833,#268834,#268835,#268836,#268837,#268838,#268839,#268840,#268841,
#268842,#268843,#268844,#268845,#268846,#268847,#268848,#268849,#268850,
#268851,#268852,#268853,#268854,#268855,#268856,#268857,#268858,#268859,
#268860,#268861,#268862,#268863,#268864,#268865,#268866,#268867,#268868,
#268869,#268870,#268871,#268872,#268873,#268874,#268875,#268876,#268877,
#268878,#268879,#268880,#268881,#268882,#268883,#268884,#268885,#268886,
#268887,#268888,#268889,#268890,#268891,#268892,#268893,#268894,#268895,
#268896,#268897,#268898,#268899,#268900,#268901,#268902,#268903,#268904,
#268905,#268906,#268907,#268908,#268909,#268910,#268911,#268912,#268913,
#268914,#268915,#268916,#268917,#268918,#268919,#268920,#268921,#268922,
#268923,#268924,#268925,#268926,#268927,#268928,#268929,#268930,#268931,
#268932,#268933,#268934,#268935,#268936,#268937,#268938,#268939,#268940,
#268941,#268942,#268943,#268944,#268945,#268946,#268947,#268948,#268949,
#268950,#268951,#268952,#268953,#268954,#268955,#268956,#268957,#268958,
#268959,#268960,#268961,#268962,#268963,#268964,#268965,#268966,#268967,
#268968,#268969,#268970,#268971,#268972,#268973,#268974,#268975,#268976,
#268977,#268978,#268979,#268980,#268981,#268982,#268983,#268984,#268985,
#268986,#268987,#268988,#268989,#268990,#268991,#268992,#268993,#268994,
#268995,#268996,#268997,#268998,#268999,#269000,#269001,#269002,#269003,
#269004,#269005,#269006,#269007,#269008,#269009,#269010,#269011,#269012,
#269013,#269014,#269015,#269016,#269017,#269018,#269019,#269020,#269021,
#269022,#269023,#269024,#269025,#269026,#269027,#269028,#269029,#269030,
#269031,#269032,#269033,#269034,#269035,#269036,#269037,#269038,#269039,
#269040,#269041,#269042,#269043,#269044,#269045,#269046,#269047,#269048,
#269049,#269050,#269051,#269052,#269053,#269054,#269055,#269056,#269057,
#269058,#269059,#269060,#269061,#269062,#269063,#269064,#269065,#269066,
#269067,#269068,#269069,#269070,#269071,#269072,#269073,#269074,#269075,
#269076,#269077,#269078,#269079,#269080,#269081,#269082,#269083,#269084,
#269085,#269086,#269087,#269088,#269089,#269090,#269091,#269092,#269093,
#269094,#269095,#269096,#269097,#269098,#269099,#269100,#269101,#269102,
#269103,#269104,#269105,#269106,#269107,#269108,#269109,#269110,#269111,
#269112,#269113,#269114,#269115,#269116,#269117,#269118,#269119,#269120,
#269121,#269122,#269123,#269124,#269125,#269126,#269127,#269128,#269129,
#269130,#269131,#269132,#269133,#269134,#269135,#269136,#269137,#269138,
#269139,#269140,#269141,#269142,#269143,#269144,#269145,#269146,#269147,
#269148,#269149,#269150,#269151,#269152,#269153,#269154,#269155,#269156,
#269157,#269158,#269159,#269160,#269161,#269162,#269163,#269164,#269165,
#269166,#269167,#269168,#269169,#269170,#269171,#269172,#269173,#269174,
#269175,#269176,#269177,#269178,#269179,#269180,#269181,#269182,#269183,
#269184,#269185,#269186,#269187,#269188,#269189,#269190,#269191,#269192,
#269193,#269194,#269195,#269196,#269197,#269198,#269199,#269200,#269201,
#269202,#269203,#269204,#269205,#269206,#269207,#269208,#269209,#269210,
#269211,#269212,#269213,#269214,#269215,#269216,#269217,#269218,#269219,
#269220,#269221,#269222,#269223,#269224,#269225,#269226,#269227,#269228,
#269229,#269230,#269231,#269232,#269233,#269234,#269235,#269236,#269237,
#269238,#269239,#269240,#269241,#269242,#269243,#269244,#269245,#269246,
#269247,#269248,#269249,#269250,#269251,#269252,#269253,#269254,#269255,
#269256,#269257,#269258,#269259,#269260,#269261,#269262,#269263,#269264,
#269265,#269266,#269267,#269268,#269269,#269270,#269271,#269272,#269273,
#269274,#269275,#269276,#269277,#269278,#269279,#269280,#269281,#269282,
#269283,#269284,#269285,#269286,#269287,#269288,#269289,#269290,#269291,
#269292,#269293,#269294,#269295,#269296,#269297,#269298,#269299,#269300,
#269301,#269302,#269303,#269304,#269305,#269306,#269307,#269308,#269309,
#269310,#269311,#269312,#269313,#269314,#269315,#269316,#269317,#269318,
#269319,#269320,#269321,#269322,#269323,#269324,#269325,#269326,#269327,
#269328,#269329,#269330,#269331,#269332,#269333,#269334,#269335,#269336,
#269337,#269338,#269339,#269340,#269341,#269342,#269343,#269344,#269345,
#269346,#269347,#269348,#269349,#269350,#269351,#269352,#269353,#269354,
#269355,#269356,#269357,#269358,#269359,#269360,#269361,#269362,#269363,
#269364,#269365,#269366,#269367,#269368,#269369,#269370,#269371,#269372,
#269373,#269374,#269375,#269376,#269377,#269378,#269379,#269380,#269381,
#269382,#269383,#269384,#269385,#269386,#269387,#269388,#269389,#269390,
#269391,#269392,#269393,#269394,#269395,#269396,#269397,#269398,#269399,
#269400,#269401,#269402,#269403,#269404,#269405,#269406,#269407,#269408,
#269409,#269410,#269411,#269412,#269413,#269414,#269415,#269416,#269417,
#269418,#269419,#269420,#269421,#269422,#269423,#269424,#269425,#269426,
#269427,#269428,#269429,#269430,#269431,#269432,#269433,#269434,#269435,
#269436,#269437,#269438,#269439,#269440,#269441,#269442,#269443,#269444,
#269445,#269446,#269447,#269448,#269449,#269450,#269451,#269452,#269453,
#269454,#269455,#269456,#269457,#269458,#269459,#269460,#269461,#269462,
#269463,#269464,#269465,#269466,#269467,#269468,#269469,#269470,#269471,
#269472,#269473,#269474,#269475,#269476,#269477,#269478,#269479,#269480,
#269481,#269482,#269483,#269484,#269485,#269486,#269487,#269488,#269489,
#269490,#269491,#269492,#269493,#269494,#269495,#269496,#269497,#269498,
#269499,#269500,#269501,#269502,#269503,#269504,#269505,#269506,#269507,
#269508,#269509,#269510,#269511,#269512,#269513,#269514,#269515,#269516,
#269517,#269518,#269519,#269520,#269521,#269522,#269523,#269524,#269525,
#269526,#269527,#269528,#269529,#269530,#269531,#269532,#269533,#269534,
#269535,#269536,#269537,#269538,#269539,#269540,#269541,#269542,#269543,
#269544,#269545,#269546,#269547,#269548,#269549,#269550,#269551,#269552,
#269553,#269554,#269555,#269556,#269557,#269558,#269559,#269560,#269561,
#269562,#269563,#269564,#269565,#269566,#269567,#269568,#269569,#269570,
#269571,#269572,#269573,#269574,#269575,#269576,#269577,#269578,#269579,
#269580,#269581,#269582,#269583,#269584,#269585,#269586,#269587,#269588,
#269589,#269590,#269591,#269592,#269593,#269594,#269595,#269596,#269597,
#269598,#269599,#269600,#269601,#269602,#269603,#269604,#269605,#269606,
#269607,#269608,#269609,#269610,#269611,#269612,#269613,#269614,#269615,
#269616,#269617,#269618,#269619,#269620,#269621,#269622,#269623,#269624,
#269625,#269626,#269627,#269628,#269629,#269630,#269631,#269632,#269633,
#269634,#269635,#269636,#269637,#269638,#269639,#269640,#269641,#269642,
#269643,#269644,#269645,#269646,#269647,#269648,#269649,#269650,#269651,
#269652,#269653,#269654,#269655,#269656,#269657,#269658,#269659,#269660,
#269661,#269662,#269663,#269664,#269665,#269666,#269667,#269668,#269669,
#269670,#269671,#269672,#269673,#269674,#269675,#269676,#269677,#269678,
#269679,#269680,#269681,#269682,#269683,#269684,#269685,#269686,#269687,
#269688,#269689,#269690,#269691,#269692,#269693,#269694,#269695,#269696,
#269697,#269698,#269699,#269700,#269701,#269702,#269703,#269704,#269705,
#269706,#269707,#269708,#269709,#269710,#269711,#269712,#269713,#269714,
#269715,#269716,#269717,#269718,#269719,#269720,#269721,#269722,#269723,
#269724,#269725,#269726,#269727,#269728,#269729,#269730,#269731,#269732,
#269733,#269734,#269735,#269736,#269737,#269738,#269739,#269740,#269741,
#269742,#269743,#269744,#269745,#269746,#269747,#269748,#269749,#269750,
#269751,#269752,#269753,#269754,#269755,#269756,#269757,#269758,#269759,
#269760,#269761,#269762,#269763,#269764,#269765,#269766,#269767,#269768,
#269769,#269770,#269771,#269772,#269773,#269774,#269775,#269776,#269777,
#269778,#269779,#269780,#269781,#269782,#269783,#269784,#269785,#269786,
#269787,#269788,#269789,#269790,#269791,#269792,#269793,#269794,#269795,
#269796,#269797,#269798,#269799,#269800,#269801,#269802,#269803,#269804,
#269805,#269806,#269807,#269808,#269809,#269810,#269811,#269812,#269813,
#269814,#269815,#269816,#269817,#269818,#269819,#269820,#269821,#269822,
#269823,#269824,#269825,#269826,#269827,#269828,#269829,#269830,#269831,
#269832,#269833,#269834,#269835,#269836,#269837,#269838,#269839,#269840,
#269841,#269842,#269843,#269844,#269845,#269846,#269847,#269848,#269849,
#269850,#269851,#269852,#269853,#269854,#269855,#269856,#269857,#269858,
#269859,#269860,#269861,#269862,#269863,#269864,#269865,#269866,#269867,
#269868,#269869,#269870,#269871,#269872,#269873,#269874,#269875,#269876,
#269877,#269878,#269879,#269880,#269881,#269882,#269883,#269884,#269885,
#269886,#269887,#269888,#269889,#269890,#269891,#269892,#269893,#269894,
#269895,#269896,#269897,#269898,#269899,#269900,#269901,#269902,#269903,
#269904,#269905,#269906,#269907,#269908,#269909,#269910,#269911,#269912,
#269913,#269914,#269915,#269916,#269917,#269918,#269919,#269920,#269921,
#269922,#269923,#269924,#269925,#269926,#269927,#269928,#269929,#269930,
#269931,#269932,#269933,#269934,#269935,#269936,#269937,#269938,#269939,
#269940,#269941,#269942,#269943,#269944,#269945,#269946,#269947,#269948,
#269949,#269950,#269951,#269952,#269953,#269954,#269955,#269956,#269957,
#269958,#269959,#269960,#269961,#269962,#269963,#269964,#269965,#269966,
#269967,#269968,#269969,#269970,#269971,#269972,#269973,#269974,#269975,
#269976,#269977,#269978,#269979,#269980,#269981,#269982,#269983,#269984,
#269985,#269986,#269987,#269988,#269989,#269990,#269991,#269992,#269993,
#269994,#269995,#269996,#269997,#269998,#269999,#270000,#270001,#270002,
#270003,#270004,#270005,#270006,#270007,#270008,#270009,#270010,#270011,
#270012,#270013,#270014,#270015,#270016,#270017,#270018,#270019,#270020,
#270021,#270022,#270023,#270024,#270025,#270026,#270027,#270028,#270029,
#270030,#270031,#270032,#270033,#270034,#270035,#270036,#270037,#270038,
#270039,#270040,#270041,#270042,#270043,#270044,#270045,#270046,#270047,
#270048,#270049,#270050,#270051,#270052,#270053,#270054,#270055,#270056,
#270057,#270058,#270059,#270060,#270061,#270062,#270063,#270064,#270065,
#270066,#270067,#270068,#270069,#270070,#270071,#270072,#270073,#270074,
#270075,#270076,#270077,#270078,#270079,#270080,#270081,#270082,#270083,
#270084,#270085,#270086,#270087,#270088,#270089,#270090,#270091,#270092,
#270093,#270094,#270095,#270096,#270097,#270098,#270099,#270100,#270101,
#270102,#270103,#270104,#270105,#270106,#270107,#270108,#270109,#270110,
#270111,#270112,#270113,#270114,#270115,#270116,#270117,#270118,#270119,
#270120,#270121,#270122,#270123,#270124,#270125,#270126,#270127,#270128,
#270129,#270130,#270131,#270132,#270133,#270134,#270135,#270136,#270137,
#270138,#270139,#270140,#270141,#270142,#270143,#270144,#270145,#270146,
#270147,#270148,#270149,#270150,#270151,#270152,#270153,#270154,#270155,
#270156,#270157,#270158,#270159,#270160,#270161,#270162,#270163,#270164,
#270165,#270166,#270167,#270168,#270169,#270170,#270171,#270172,#270173,
#270174,#270175,#270176,#270177,#270178,#270179,#270180,#270181,#270182,
#270183,#270184,#270185,#270186,#270187,#270188,#270189,#270190,#270191,
#270192,#270193,#270194,#270195,#270196,#270197,#270198,#270199,#270200,
#270201,#270202,#270203,#270204,#270205,#270206,#270207,#270208,#270209,
#270210,#270211,#270212,#270213,#270214,#270215,#270216,#270217,#270218,
#270219,#270220,#270221,#270222,#270223,#270224,#270225,#270226,#270227,
#270228,#270229,#270230,#270231,#270232,#270233,#270234,#270235,#270236,
#270237,#270238,#270239,#270240,#270241,#270242,#270243,#270244,#270245,
#270246,#270247,#270248,#270249,#270250,#270251,#270252,#270253,#270254,
#270255,#270256,#270257,#270258,#270259,#270260,#270261,#270262,#270263,
#270264,#270265,#270266,#270267,#270268,#270269,#270270,#270271,#270272,
#270273,#270274,#270275,#270276,#270277,#270278,#270279,#270280,#270281,
#270282,#270283,#270284,#270285,#270286,#270287,#270288,#270289,#270290,
#270291,#270292,#270293,#270294,#270295,#270296,#270297,#270298,#270299,
#270300,#270301,#270302,#270303,#270304,#270305,#270306,#270307,#270308,
#270309,#270310,#270311,#270312,#270313,#270314,#270315,#270316,#270317,
#270318,#270319,#270320,#270321,#270322,#270323,#270324,#270325,#270326,
#270327,#270328,#270329,#270330,#270331,#270332,#270333,#270334,#270335,
#270336,#270337,#270338,#270339,#270340,#270341,#270342,#270343,#270344,
#270345,#270346,#270347,#270348,#270349,#270350,#270351,#270352,#270353,
#270354,#270355,#270356,#270357,#270358,#270359,#270360,#270361,#270362,
#270363,#270364,#270365,#270366,#270367,#270368,#270369,#270370,#270371,
#270372,#270373,#270374,#270375,#270376,#270377,#270378,#270379,#270380,
#270381,#270382,#270383,#270384,#270385,#270386,#270387,#270388,#270389,
#270390,#270391,#270392,#270393,#270394,#270395,#270396,#270397,#270398,
#270399,#270400,#270401,#270402,#270403,#270404,#270405,#270406,#270407,
#270408,#270409,#270410,#270411,#270412,#270413,#270414,#270415,#270416,
#270417,#270418,#270419,#270420,#270421,#270422,#270423,#270424,#270425,
#270426,#270427,#270428,#270429,#270430,#270431,#270432,#270433,#270434,
#270435,#270436,#270437,#270438,#270439,#270440,#270441,#270442,#270443,
#270444,#270445,#270446,#270447,#270448,#270449,#270450,#270451,#270452,
#270453,#270454,#270455,#270456,#270457,#270458,#270459,#270460,#270461,
#270462,#270463,#270464,#270465,#270466,#270467,#270468,#270469,#270470,
#270471,#270472,#270473,#270474,#270475),(#270476,#270477,#270478,#270479,
#270480,#270481,#270482,#270483,#270484,#270485,#270486,#270487,#270488,
#270489,#270490,#270491,#270492,#270493,#270494,#270495,#270496,#270497,
#270498,#270499,#270500,#270501,#270502,#270503,#270504,#270505,#270506,
#270507,#270508,#270509,#270510,#270511,#270512,#270513,#270514,#270515,
#270516,#270517,#270518,#270519,#270520,#270521,#270522,#270523,#270524,
#270525,#270526,#270527,#270528,#270529,#270530,#270531,#270532,#270533,
#270534,#270535,#270536,#270537,#270538,#270539,#270540,#270541,#270542,
#270543,#270544,#270545,#270546,#270547,#270548,#270549,#270550,#270551,
#270552,#270553,#270554,#270555,#270556,#270557,#270558,#270559,#270560,
#270561,#270562,#270563,#270564,#270565,#270566,#270567,#270568,#270569,
#270570,#270571,#270572,#270573,#270574,#270575,#270576,#270577,#270578,
#270579,#270580,#270581,#270582,#270583,#270584,#270585,#270586,#270587,
#270588,#270589,#270590,#270591,#270592,#270593,#270594,#270595,#270596,
#270597,#270598,#270599,#270600,#270601,#270602,#270603,#270604,#270605,
#270606,#270607,#270608,#270609,#270610,#270611,#270612,#270613,#270614,
#270615,#270616,#270617,#270618,#270619,#270620,#270621,#270622,#270623,
#270624,#270625,#270626,#270627,#270628,#270629,#270630,#270631,#270632,
#270633,#270634,#270635,#270636,#270637,#270638,#270639,#270640,#270641,
#270642,#270643,#270644,#270645,#270646,#270647,#270648,#270649,#270650,
#270651,#270652,#270653,#270654,#270655,#270656,#270657,#270658,#270659,
#270660,#270661,#270662,#270663,#270664,#270665,#270666,#270667,#270668,
#270669,#270670,#270671,#270672,#270673,#270674,#270675,#270676,#270677,
#270678,#270679,#270680,#270681,#270682,#270683,#270684,#270685,#270686,
#270687,#270688,#270689,#270690,#270691,#270692,#270693,#270694,#270695,
#270696,#270697,#270698,#270699,#270700,#270701,#270702,#270703,#270704,
#270705,#270706,#270707,#270708,#270709,#270710,#270711,#270712,#270713,
#270714,#270715,#270716,#270717,#270718,#270719,#270720,#270721,#270722,
#270723,#270724,#270725,#270726,#270727,#270728,#270729,#270730,#270731,
#270732,#270733,#270734,#270735,#270736,#270737,#270738,#270739,#270740,
#270741,#270742,#270743,#270744,#270745,#270746,#270747,#270748,#270749,
#270750,#270751,#270752,#270753,#270754,#270755,#270756,#270757,#270758,
#270759,#270760,#270761,#270762,#270763,#270764,#270765,#270766,#270767,
#270768,#270769,#270770,#270771,#270772,#270773,#270774,#270775,#270776,
#270777,#270778,#270779,#270780,#270781,#270782,#270783,#270784,#270785,
#270786,#270787,#270788,#270789,#270790,#270791,#270792,#270793,#270794,
#270795,#270796,#270797,#270798,#270799,#270800,#270801,#270802,#270803,
#270804,#270805,#270806,#270807,#270808,#270809,#270810,#270811,#270812,
#270813,#270814,#270815,#270816,#270817,#270818,#270819,#270820,#270821,
#270822,#270823,#270824,#270825,#270826,#270827,#270828,#270829,#270830,
#270831,#270832,#270833,#270834,#270835,#270836,#270837,#270838,#270839,
#270840,#270841,#270842,#270843,#270844,#270845,#270846,#270847,#270848,
#270849,#270850,#270851,#270852,#270853,#270854,#270855,#270856,#270857,
#270858,#270859,#270860,#270861,#270862,#270863,#270864,#270865,#270866,
#270867,#270868,#270869,#270870,#270871,#270872,#270873,#270874,#270875,
#270876,#270877,#270878,#270879,#270880,#270881,#270882,#270883,#270884,
#270885,#270886,#270887,#270888,#270889,#270890,#270891,#270892,#270893,
#270894,#270895,#270896,#270897,#270898,#270899,#270900,#270901,#270902,
#270903,#270904,#270905,#270906,#270907,#270908,#270909,#270910,#270911,
#270912,#270913,#270914,#270915,#270916,#270917,#270918,#270919,#270920,
#270921,#270922,#270923,#270924,#270925,#270926,#270927,#270928,#270929,
#270930,#270931,#270932,#270933,#270934,#270935,#270936,#270937,#270938,
#270939,#270940,#270941,#270942,#270943,#270944,#270945,#270946,#270947,
#270948,#270949,#270950,#270951,#270952,#270953,#270954,#270955,#270956,
#270957,#270958,#270959,#270960,#270961,#270962,#270963,#270964,#270965,
#270966,#270967,#270968,#270969,#270970,#270971,#270972,#270973,#270974,
#270975,#270976,#270977,#270978,#270979,#270980,#270981,#270982,#270983,
#270984,#270985,#270986,#270987,#270988,#270989,#270990,#270991,#270992,
#270993,#270994,#270995,#270996,#270997,#270998,#270999,#271000,#271001,
#271002,#271003,#271004,#271005,#271006,#271007,#271008,#271009,#271010,
#271011,#271012,#271013,#271014,#271015,#271016,#271017,#271018,#271019,
#271020,#271021,#271022,#271023,#271024,#271025,#271026,#271027,#271028,
#271029,#271030,#271031,#271032,#271033,#271034,#271035,#271036,#271037,
#271038,#271039,#271040,#271041,#271042,#271043,#271044,#271045,#271046,
#271047,#271048,#271049,#271050,#271051,#271052,#271053,#271054,#271055,
#271056,#271057,#271058,#271059,#271060,#271061,#271062,#271063,#271064,
#271065,#271066,#271067,#271068,#271069,#271070,#271071,#271072,#271073,
#271074,#271075,#271076,#271077,#271078,#271079,#271080,#271081,#271082,
#271083,#271084,#271085,#271086,#271087,#271088,#271089,#271090,#271091,
#271092,#271093,#271094,#271095,#271096,#271097,#271098,#271099,#271100,
#271101,#271102,#271103,#271104,#271105,#271106,#271107,#271108,#271109,
#271110,#271111,#271112,#271113,#271114,#271115,#271116,#271117,#271118,
#271119,#271120,#271121,#271122,#271123,#271124,#271125,#271126,#271127,
#271128,#271129,#271130,#271131,#271132,#271133,#271134,#271135,#271136,
#271137,#271138,#271139,#271140,#271141,#271142,#271143,#271144,#271145,
#271146,#271147,#271148,#271149,#271150,#271151,#271152,#271153,#271154,
#271155,#271156,#271157,#271158,#271159,#271160,#271161,#271162,#271163,
#271164,#271165,#271166,#271167,#271168,#271169,#271170,#271171,#271172,
#271173,#271174,#271175,#271176,#271177,#271178,#271179,#271180,#271181,
#271182,#271183,#271184,#271185,#271186,#271187,#271188,#271189,#271190,
#271191,#271192,#271193,#271194,#271195,#271196,#271197,#271198,#271199,
#271200,#271201,#271202,#271203,#271204,#271205,#271206,#271207,#271208,
#271209,#271210,#271211,#271212,#271213,#271214,#271215,#271216,#271217,
#271218,#271219,#271220,#271221,#271222,#271223,#271224,#271225,#271226,
#271227,#271228,#271229,#271230,#271231,#271232,#271233,#271234,#271235,
#271236,#271237,#271238,#271239,#271240,#271241,#271242,#271243,#271244,
#271245,#271246,#271247,#271248,#271249,#271250,#271251,#271252,#271253,
#271254,#271255,#271256,#271257,#271258,#271259,#271260,#271261,#271262,
#271263,#271264,#271265,#271266,#271267,#271268,#271269,#271270,#271271,
#271272,#271273,#271274,#271275,#271276,#271277,#271278,#271279,#271280,
#271281,#271282,#271283,#271284,#271285,#271286,#271287,#271288,#271289,
#271290,#271291,#271292,#271293,#271294,#271295,#271296,#271297,#271298,
#271299,#271300,#271301,#271302,#271303,#271304,#271305,#271306,#271307,
#271308,#271309,#271310,#271311,#271312,#271313,#271314,#271315,#271316,
#271317,#271318,#271319,#271320,#271321,#271322,#271323,#271324,#271325,
#271326,#271327,#271328,#271329,#271330,#271331,#271332,#271333,#271334,
#271335,#271336,#271337,#271338,#271339,#271340,#271341,#271342,#271343,
#271344,#271345,#271346,#271347,#271348,#271349,#271350,#271351,#271352,
#271353,#271354,#271355,#271356,#271357,#271358,#271359,#271360,#271361,
#271362,#271363,#271364,#271365,#271366,#271367,#271368,#271369,#271370,
#271371,#271372,#271373,#271374,#271375,#271376,#271377,#271378,#271379,
#271380,#271381,#271382,#271383,#271384,#271385,#271386,#271387,#271388,
#271389,#271390,#271391,#271392,#271393,#271394,#271395,#271396,#271397,
#271398,#271399,#271400,#271401,#271402,#271403,#271404,#271405,#271406,
#271407,#271408,#271409,#271410,#271411,#271412,#271413,#271414,#271415,
#271416,#271417,#271418,#271419,#271420,#271421,#271422,#271423,#271424,
#271425,#271426,#271427,#271428,#271429,#271430,#271431,#271432,#271433,
#271434,#271435,#271436,#271437,#271438,#271439,#271440,#271441,#271442,
#271443,#271444,#271445,#271446,#271447,#271448,#271449,#271450,#271451,
#271452,#271453,#271454,#271455,#271456,#271457,#271458,#271459,#271460,
#271461,#271462,#271463,#271464,#271465,#271466,#271467,#271468,#271469,
#271470,#271471,#271472,#271473,#271474,#271475,#271476,#271477,#271478,
#271479,#271480,#271481,#271482,#271483,#271484,#271485,#271486,#271487,
#271488,#271489,#271490,#271491,#271492,#271493,#271494,#271495,#271496,
#271497,#271498,#271499,#271500,#271501,#271502,#271503,#271504,#271505,
#271506,#271507,#271508,#271509,#271510,#271511,#271512,#271513,#271514,
#271515,#271516,#271517,#271518,#271519,#271520,#271521,#271522,#271523,
#271524,#271525,#271526,#271527,#271528,#271529,#271530,#271531,#271532,
#271533,#271534,#271535,#271536,#271537,#271538,#271539,#271540,#271541,
#271542,#271543,#271544,#271545,#271546,#271547,#271548,#271549,#271550,
#271551,#271552,#271553,#271554,#271555,#271556,#271557,#271558,#271559,
#271560,#271561,#271562,#271563,#271564,#271565,#271566,#271567,#271568,
#271569,#271570,#271571,#271572,#271573,#271574,#271575,#271576,#271577,
#271578,#271579,#271580,#271581,#271582,#271583,#271584,#271585,#271586,
#271587,#271588,#271589,#271590,#271591,#271592,#271593,#271594,#271595,
#271596,#271597,#271598,#271599,#271600,#271601,#271602,#271603,#271604,
#271605,#271606,#271607,#271608,#271609,#271610,#271611,#271612,#271613,
#271614,#271615,#271616,#271617,#271618,#271619,#271620,#271621,#271622,
#271623,#271624,#271625,#271626,#271627,#271628,#271629,#271630,#271631,
#271632,#271633,#271634,#271635,#271636,#271637,#271638,#271639,#271640,
#271641,#271642,#271643,#271644,#271645,#271646,#271647,#271648,#271649,
#271650,#271651,#271652,#271653,#271654,#271655,#271656,#271657,#271658,
#271659,#271660,#271661,#271662,#271663,#271664,#271665,#271666,#271667,
#271668,#271669,#271670,#271671,#271672,#271673,#271674,#271675,#271676,
#271677,#271678,#271679,#271680,#271681,#271682,#271683,#271684,#271685,
#271686,#271687,#271688,#271689,#271690,#271691,#271692,#271693,#271694,
#271695,#271696,#271697,#271698,#271699,#271700,#271701,#271702,#271703,
#271704,#271705,#271706,#271707,#271708,#271709,#271710,#271711,#271712,
#271713,#271714,#271715,#271716,#271717,#271718,#271719,#271720,#271721,
#271722,#271723,#271724,#271725,#271726,#271727,#271728,#271729,#271730,
#271731,#271732,#271733,#271734,#271735,#271736,#271737,#271738,#271739,
#271740,#271741,#271742,#271743,#271744,#271745,#271746,#271747,#271748,
#271749,#271750,#271751,#271752,#271753,#271754,#271755,#271756,#271757,
#271758,#271759,#271760,#271761,#271762,#271763,#271764,#271765,#271766,
#271767,#271768,#271769,#271770,#271771,#271772,#271773,#271774,#271775,
#271776,#271777,#271778,#271779,#271780,#271781,#271782,#271783,#271784,
#271785,#271786,#271787,#271788,#271789,#271790,#271791,#271792,#271793,
#271794,#271795,#271796,#271797,#271798,#271799,#271800,#271801,#271802,
#271803,#271804,#271805,#271806,#271807,#271808,#271809,#271810,#271811,
#271812,#271813,#271814,#271815,#271816,#271817,#271818,#271819,#271820,
#271821,#271822,#271823,#271824,#271825,#271826,#271827,#271828,#271829,
#271830,#271831,#271832,#271833,#271834,#271835,#271836,#271837,#271838,
#271839,#271840,#271841,#271842,#271843,#271844,#271845,#271846,#271847,
#271848,#271849,#271850,#271851,#271852,#271853,#271854,#271855,#271856,
#271857,#271858,#271859,#271860,#271861,#271862,#271863,#271864,#271865,
#271866,#271867,#271868,#271869,#271870,#271871,#271872,#271873,#271874,
#271875,#271876,#271877,#271878,#271879,#271880,#271881,#271882,#271883,
#271884,#271885,#271886,#271887,#271888,#271889,#271890,#271891,#271892,
#271893,#271894,#271895,#271896,#271897,#271898,#271899,#271900,#271901,
#271902,#271903,#271904,#271905,#271906,#271907,#271908,#271909,#271910,
#271911,#271912,#271913,#271914,#271915,#271916,#271917,#271918,#271919,
#271920,#271921,#271922,#271923,#271924,#271925,#271926,#271927,#271928,
#271929,#271930,#271931,#271932,#271933,#271934,#271935,#271936,#271937,
#271938,#271939,#271940,#271941,#271942,#271943,#271944,#271945,#271946,
#271947,#271948,#271949,#271950,#271951,#271952,#271953,#271954,#271955,
#271956,#271957,#271958,#271959,#271960,#271961,#271962,#271963,#271964,
#271965,#271966,#271967,#271968,#271969,#271970,#271971,#271972,#271973,
#271974,#271975,#271976,#271977,#271978,#271979,#271980,#271981,#271982,
#271983,#271984,#271985,#271986,#271987,#271988,#271989,#271990,#271991,
#271992,#271993,#271994,#271995,#271996,#271997,#271998,#271999,#272000,
#272001,#272002,#272003,#272004,#272005,#272006,#272007,#272008,#272009,
#272010,#272011,#272012,#272013,#272014,#272015,#272016,#272017,#272018,
#272019,#272020,#272021,#272022,#272023,#272024,#272025,#272026,#272027,
#272028,#272029,#272030,#272031,#272032,#272033,#272034,#272035,#272036,
#272037,#272038,#272039,#272040,#272041,#272042,#272043,#272044,#272045,
#272046,#272047,#272048,#272049,#272050,#272051,#272052,#272053,#272054,
#272055,#272056,#272057,#272058,#272059,#272060,#272061,#272062,#272063,
#272064,#272065,#272066,#272067,#272068,#272069,#272070,#272071,#272072,
#272073,#272074,#272075,#272076,#272077,#272078,#272079,#272080,#272081,
#272082,#272083,#272084,#272085,#272086,#272087,#272088,#272089,#272090,
#272091,#272092,#272093,#272094,#272095,#272096,#272097,#272098,#272099,
#272100,#272101,#272102,#272103,#272104,#272105,#272106,#272107,#272108,
#272109,#272110,#272111,#272112,#272113,#272114,#272115,#272116,#272117,
#272118,#272119,#272120,#272121,#272122,#272123,#272124,#272125,#272126,
#272127,#272128,#272129,#272130,#272131,#272132,#272133,#272134,#272135,
#272136,#272137,#272138,#272139,#272140,#272141,#272142,#272143,#272144,
#272145,#272146,#272147,#272148,#272149,#272150,#272151,#272152,#272153,
#272154,#272155,#272156,#272157,#272158,#272159,#272160,#272161,#272162,
#272163,#272164,#272165,#272166,#272167,#272168,#272169,#272170)),
 .UNSPECIFIED.,.F.,.F.,.F.,(4,4),(4,1,1,1,1,1,1,1,1,1,1,1,1,1,1,1,1,1,1,
1,1,1,1,1,1,1,1,1,1,1,1,1,1,1,1,1,1,1,1,1,1,1,1,1,1,1,1,1,1,1,1,1,1,1,1,
1,1,1,1,1,1,1,1,1,1,1,1,1,1,1,1,1,1,1,1,1,1,1,1,1,1,1,1,1,1,1,1,1,1,1,1,
1,1,1,1,1,1,1,1,1,1,1,1,1,1,1,1,1,1,1,1,1,1,1,1,1,1,1,1,1,1,1,1,1,1,1,1,
1,1,1,1,1,1,1,1,1,1,1,1,1,1,1,1,1,1,1,1,1,1,1,1,1,1,1,1,1,1,1,1,1,1,1,1,
1,1,1,1,1,1,1,1,1,1,1,1,1,1,1,1,1,1,1,1,1,1,1,1,1,1,1,1,1,1,1,1,1,1,1,1,
1,1,1,1,1,1,1,1,1,1,1,1,1,1,1,1,1,1,1,1,1,1,1,1,1,1,1,1,1,1,1,1,1,1,1,1,
1,1,1,1,1,1,1,1,1,1,1,1,1,1,1,1,1,1,1,1,1,1,1,1,1,1,1,1,1,1,1,1,1,1,1,1,
1,1,1,1,1,1,1,1,1,1,1,1,1,1,1,1,1,1,1,1,1,1,1,1,1,1,1,1,1,1,1,1,1,1,1,1,
1,1,1,1,1,1,1,1,1,1,1,1,1,1,1,1,1,1,1,1,1,1,1,1,1,1,1,1,1,1,1,1,1,1,1,1,
1,1,1,1,1,1,1,1,1,1,1,1,1,1,1,1,1,1,1,1,1,1,1,1,1,1,1,1,1,1,1,1,1,1,1,1,
1,1,1,1,1,1,1,1,1,1,1,1,1,1,1,1,1,1,1,1,1,1,1,1,1,1,1,1,1,1,1,1,1,1,1,1,
1,1,1,1,1,1,1,1,1,1,1,1,1,1,1,1,1,1,1,1,1,1,1,1,1,1,1,1,1,1,1,1,1,1,1,1,
1,1,1,1,1,1,1,1,1,1,1,1,1,1,1,1,1,1,1,1,1,1,1,1,1,1,1,1,1,1,1,1,1,1,1,1,
1,1,1,1,1,1,1,1,1,1,1,1,1,1,1,1,1,1,1,1,1,1,1,1,1,1,1,1,1,1,1,1,1,1,1,1,
1,1,1,1,1,1,1,1,1,1,1,1,1,1,1,1,1,1,1,1,1,1,1,1,1,1,1,1,1,1,1,1,1,1,1,1,
1,1,1,1,1,1,1,1,1,1,1,1,1,1,1,1,1,1,1,1,1,1,1,1,1,1,1,1,1,1,1,1,1,1,1,1,
1,1,1,1,1,1,1,1,1,1,1,1,1,1,1,1,1,1,1,1,1,1,1,1,1,1,1,1,1,1,1,1,1,1,1,1,
1,1,1,1,1,1,1,1,1,1,1,1,1,1,1,1,1,1,1,1,1,1,1,1,1,1,1,1,1,1,1,1,1,1,1,1,
1,1,1,1,1,1,1,1,1,1,1,1,1,1,1,1,1,1,1,1,1,1,1,1,1,1,1,1,1,1,1,1,1,1,1,1,
1,1,1,1,1,1,1,1,1,1,1,1,1,1,1,1,1,1,1,1,1,1,1,1,1,1,1,1,1,1,1,1,1,1,1,1,
1,1,1,1,1,1,1,1,1,1,1,1,1,1,1,1,1,1,1,1,1,1,1,1,1,1,1,1,1,1,1,1,1,1,1,1,
1,1,1,1,1,1,1,1,1,1,1,1,1,1,1,1,1,1,1,1,1,1,1,1,1,1,1,1,1,1,1,1,1,1,1,1,
1,1,1,1,1,1,1,1,1,1,1,1,1,1,1,1,1,1,1,1,1,1,1,1,1,1,1,1,1,1,1,1,1,1,1,1,
1,1,1,1,1,1,1,1,1,1,1,1,1,1,1,1,1,1,1,1,1,1,1,1,1,1,1,1,1,1,1,1,1,1,1,1,
1,1,1,1,1,1,1,1,1,1,1,1,1,1,1,1,1,1,1,1,1,1,1,1,1,1,1,1,1,1,1,1,1,1,1,1,
1,1,1,1,1,1,1,1,1,1,1,1,1,1,1,1,1,1,1,1,1,1,1,1,1,1,1,1,1,1,1,1,1,1,1,1,
1,1,1,1,1,1,1,1,1,1,1,1,1,1,1,1,1,1,1,1,1,1,1,1,1,1,1,1,1,1,1,1,1,1,1,1,
1,1,1,1,1,1,1,1,1,1,1,1,1,1,1,1,1,1,1,1,1,1,1,1,1,1,1,1,1,1,1,1,1,1,1,1,
1,1,1,1,1,1,1,1,1,1,1,1,1,1,1,1,1,1,1,1,1,1,1,1,1,1,1,1,1,1,1,1,1,1,1,1,
1,1,1,1,1,1,1,1,1,1,1,1,1,1,1,1,1,1,1,1,1,1,1,1,1,1,1,1,1,1,1,1,1,1,1,1,
1,1,1,1,1,1,1,1,1,1,1,1,1,1,1,1,1,1,1,1,1,1,1,1,1,1,1,1,1,1,1,1,1,1,1,1,
1,1,1,1,1,1,1,1,1,1,1,1,1,1,1,1,1,1,1,1,1,1,1,1,1,1,1,1,1,1,1,1,1,1,1,1,
1,1,1,1,1,1,1,1,1,1,1,1,1,1,1,1,1,1,1,1,1,1,1,1,1,1,1,1,1,1,1,1,1,1,1,1,
1,1,1,1,1,1,1,1,1,1,1,1,1,1,1,1,1,1,1,1,1,1,1,1,1,1,1,1,1,1,1,1,1,1,1,1,
1,1,1,1,1,1,1,1,1,1,1,1,1,1,1,1,1,1,1,1,1,1,1,1,1,1,1,1,1,1,1,1,1,1,1,1,
1,1,1,1,1,1,1,1,1,1,1,1,1,1,1,1,1,1,1,1,1,1,1,1,1,1,1,1,1,1,1,1,1,1,1,1,
1,1,1,1,1,1,1,1,1,1,1,1,1,1,1,1,1,1,1,1,1,1,1,1,1,1,1,1,1,1,1,1,1,1,1,1,
1,1,1,1,1,1,1,1,1,1,1,1,1,1,1,1,1,1,1,1,1,1,1,1,1,1,1,1,1,1,1,1,1,1,1,1,
1,1,1,1,1,1,1,1,1,1,1,1,1,1,1,1,1,1,1,1,1,1,1,1,1,1,1,1,1,1,1,1,1,1,1,1,
1,1,1,1,1,1,1,1,1,1,1,1,1,1,1,1,1,1,1,1,1,1,1,1,1,1,1,1,1,1,1,1,1,1,1,1,
1,1,1,1,1,1,1,1,1,1,1,1,1,1,1,1,1,1,1,1,1,1,1,1,1,1,1,1,1,1,1,1,1,1,1,1,
1,1,1,1,1,1,1,1,1,1,1,1,1,1,1,1,1,1,1,1,1,1,1,1,1,1,1,1,1,1,1,1,1,1,1,1,
1,1,1,1,1,1,1,1,1,1,1,1,1,1,1,1,1,1,1,1,1,1,1,1,1,1,1,1,1,1,1,1,1,1,1,1,
1,1,1,1,1,1,1,1,1,1,1,1,1,1,1,1,1,1,1,1,1,1,1,1,1,1,1,1,1,1,1,1,1,1,1,1,
1,1,1,1,1,1,1,1,1,1,1,1,1,1,1,1,1,1,1,1,1,1,1,1,1,1,1,1,1,1,1,1,1,1,1,1,
1,1,1,1,1,1,1,1,1,1,1,1,1,1,1,1,1,1,1,1,1,1,1,1,1,1,1,1,1,1,1,1,1,1,1,1,
1,1,1,1,1,1,1,1,1,1,1,1,1,1,1,1,1,4),(-0.000423095957202541,0.115881565465356),
(11.6153146011728,12.1152895244478,12.6151575298078,13.614893540528,14.6146295512481,
15.6143655619682,16.6141015726884,17.6138375834085,18.6135735941286,19.6133096048488,
20.6130456155689,21.612781626289,22.6125176370092,23.6122536477293,24.6119896584494,
25.6117256691696,26.6114616798897,27.6111976906098,28.6109337013299,29.6106697120501,
30.6104057227702,31.6101417334903,32.6098777442105,33.6096137549306,34.6093497656507,
35.6090857763709,36.608821787091,37.6085577978111,38.6082938085313,39.6080298192514,
40.6077658299715,41.6075018406916,42.6072378514118,43.6069738621319,44.606709872852,
45.6064458835722,46.6061818942923,47.6059179050124,48.6056539157326,49.6053899264527,
50.6051259371728,51.604861947893,52.6045979586131,53.6043339693332,54.6040699800534,
55.6038059907735,56.6035420014936,57.6032780122137,58.6030140229339,59.602750033654,
60.6024860443741,61.6022220550943,62.6019580658144,63.6016940765345,64.6014300872547,
65.6011660979748,66.6009021086949,67.6006381194151,68.6003741301352,69.6001101408553,
70.5998461515754,71.5995821622956,72.5993181730157,73.5990541837358,74.598790194456,
75.5985262051761,76.5982622158962,77.5979982266164,78.5977342373365,79.5974702480566,
80.5972062587768,81.5969422694969,82.596678280217,83.5964142909372,84.5961503016573,
85.5958863123774,86.5956223230975,87.5953583338177,88.5950943445378,89.5948303552579,
90.5945663659781,91.5943023766982,92.5940383874183,93.5937743981385,94.5935104088586,
95.5932464195787,96.5929824302989,97.592718441019,98.5924544517391,99.5921904624593,
100.591926473179,101.5916624839,102.59139849462,103.59113450534,104.59087051606,
105.59060652678,106.5903425375,107.59007854822,108.58981455894,109.589550569661,
110.589286580381,111.589022591101,112.588758601821,113.588494612541,114.588230623261,
115.587966633981,116.587702644701,117.587438655422,118.587174666142,119.586910676862,
120.586646687582,121.586382698302,122.586118709022,123.585854719742,124.585590730463,
125.585326741183,126.585062751903,127.584798762623,128.584534773343,129.584270784063,
130.584006794783,131.583742805503,132.583478816224,133.583214826944,134.582950837664,
135.582686848384,136.582422859104,137.582158869824,138.581894880544,139.581630891264,
140.581366901985,141.581102912705,142.580838923425,143.580574934145,144.580310944865,
145.580046955585,146.579782966305,147.579518977026,148.579254987746,149.578990998466,
150.578727009186,151.578463019906,152.578199030626,153.577935041346,154.577671052066,
155.577407062787,156.577143073507,157.576879084227,158.576615094947,159.576351105667,
160.576087116387,161.575823127107,162.575559137827,163.575295148548,164.575031159268,
165.574767169988,166.574503180708,167.574239191428,168.573975202148,169.573711212868,
170.573447223589,171.573183234309,172.572919245029,173.572655255749,174.572391266469,
175.572127277189,176.571863287909,177.571599298629,178.57133530935,179.57107132007,
180.57080733079,181.57054334151,182.57027935223,183.57001536295,184.56975137367,
185.56948738439,186.569223395111,187.568959405831,188.568695416551,189.568431427271,
190.568167437991,191.567903448711,192.567639459431,193.567375470152,194.567111480872,
195.566847491592,196.566583502312,197.566319513032,198.566055523752,199.565791534472,
200.565527545192,201.565263555913,202.564999566633,203.564735577353,204.564471588073,
205.564207598793,206.563943609513,207.563679620233,208.563415630954,209.563151641674,
210.562887652394,211.562623663114,212.562359673834,213.562095684554,214.561831695274,
215.561567705994,216.561303716715,217.561039727435,218.560775738155,219.560511748875,
220.560247759595,221.559983770315,222.559719781035,223.559455791755,224.559191802476,
225.558927813196,226.558663823916,227.558399834636,228.558135845356,229.557871856076,
230.557607866796,231.557343877517,232.557079888237,233.556815898957,234.556551909677,
235.556287920397,236.556023931117,237.555759941837,238.555495952557,239.555231963278,
240.554967973998,241.554703984718,242.554439995438,243.554176006158,244.553912016878,
245.553648027598,246.553384038319,247.553120049039,248.552856059759,249.552592070479,
250.552328081199,251.552064091919,252.551800102639,253.551536113359,254.55127212408,
255.5510081348,256.55074414552,257.55048015624,258.55021616696,259.54995217768,
260.5496881884,261.54942419912,262.549160209841,263.548896220561,264.548632231281,
265.548368242001,266.548104252721,267.547840263441,268.547576274161,269.547312284882,
270.547048295602,271.546784306322,272.546520317042,273.546256327762,274.545992338482,
275.545728349202,276.545464359922,277.545200370643,278.544936381363,279.544672392083,
280.544408402803,281.544144413523,282.543880424243,283.543616434963,284.543352445683,
285.543088456404,286.542824467124,287.542560477844,288.542296488564,289.542032499284,
290.541768510004,291.541504520724,292.541240531445,293.540976542165,294.540712552885,
295.540448563605,296.540184574325,297.539920585045,298.539656595765,299.539392606485,
300.539128617206,301.538864627926,302.538600638646,303.538336649366,304.538072660086,
305.537808670806,306.537544681526,307.537280692246,308.537016702967,309.536752713687,
310.536488724407,311.536224735127,312.535960745847,313.535696756567,314.535432767287,
315.535168778008,316.534904788728,317.534640799448,318.534376810168,319.534112820888,
320.533848831608,321.533584842328,322.533320853048,323.533056863769,324.532792874489,
325.532528885209,326.532264895929,327.532000906649,328.531736917369,329.531472928089,
330.53120893881,331.53094494953,332.53068096025,333.53041697097,334.53015298169,
335.52988899241,336.52962500313,337.52936101385,338.529097024571,339.528833035291,
340.528569046011,341.528305056731,342.528041067451,343.527777078171,344.527513088891,
345.527249099611,346.526985110332,347.526721121052,348.526457131772,349.526193142492,
350.525929153212,351.525665163932,352.525401174652,353.525137185373,354.524873196093,
355.524609206813,356.524345217533,357.524081228253,358.523817238973,359.523553249693,
360.523289260413,361.523025271134,362.522761281854,363.522497292574,364.522233303294,
365.521969314014,366.521705324734,367.521441335454,368.521177346175,369.520913356895,
370.520649367615,371.520385378335,372.520121389055,373.519857399775,374.519593410495,
375.519329421215,376.519065431936,377.518801442656,378.518537453376,379.518273464096,
380.518009474816,381.517745485536,382.517481496256,383.517217506976,384.516953517697,
385.516689528417,386.516425539137,387.516161549857,388.515897560577,389.515633571297,
390.515369582017,391.515105592737,392.514841603458,393.514577614178,394.514313624898,
395.514049635618,396.513785646338,397.513521657058,398.513257667778,399.512993678499,
400.512729689219,401.512465699939,402.512201710659,403.511937721379,404.511673732099,
405.511409742819,406.511145753539,407.51088176426,408.51061777498,409.5103537857,
410.51008979642,411.50982580714,412.50956181786,413.50929782858,414.509033839301,
415.508769850021,416.508505860741,417.508241871461,418.507977882181,419.507713892901,
420.507449903621,421.507185914341,422.506921925062,423.506657935782,424.506393946502,
425.506129957222,426.505865967942,427.505601978662,428.505337989382,429.505074000102,
430.504810010823,431.504546021543,432.504282032263,433.504018042983,434.503754053703,
435.503490064423,436.503226075143,437.502962085864,438.502698096584,439.502434107304,
440.502170118024,441.501906128744,442.501642139464,443.501378150184,444.501114160904,
445.500850171625,446.500586182345,447.500322193065,448.500058203785,449.499794214505,
450.499530225225,451.499266235945,452.499002246665,453.498738257386,454.498474268106,
455.498210278826,456.497946289546,457.497682300266,458.497418310986,459.497154321706,
460.496890332427,461.496626343147,462.496362353867,463.496098364587,464.495834375307,
465.495570386027,466.495306396747,467.495042407467,468.494778418188,469.494514428908,
470.494250439628,471.493986450348,472.493722461068,473.493458471788,474.493194482508,
475.492930493229,476.492666503949,477.492402514669,478.492138525389,479.491874536109,
480.491610546829,481.491346557549,482.491082568269,483.49081857899,484.49055458971,
485.49029060043,486.49002661115,487.48976262187,488.48949863259,489.48923464331,
490.48897065403,491.488706664751,492.488442675471,493.488178686191,494.487914696911,
495.487650707631,496.487386718351,497.487122729071,498.486858739792,499.486594750512,
500.486330761232,501.486066771952,502.485802782672,503.485538793392,504.485274804112,
505.485010814832,506.484746825553,507.484482836273,508.484218846993,509.483954857713,
510.483690868433,511.483426879153,512.483162889873,513.482898900594,514.482634911314,
515.482370922034,516.482106932754,517.481842943474,518.481578954194,519.481314964914,
520.481050975635,521.480786986355,522.480522997075,523.480259007795,524.479995018515,
525.479731029235,526.479467039955,527.479203050675,528.478939061396,529.478675072116,
530.478411082836,531.478147093556,532.477883104276,533.477619114996,534.477355125716,
535.477091136436,536.476827147157,537.476563157877,538.476299168597,539.476035179317,
540.475771190037,541.475507200757,542.475243211477,543.474979222197,544.474715232918,
545.474451243638,546.474187254358,547.473923265078,548.473659275798,549.473395286518,
550.473131297238,551.472867307958,552.472603318679,553.472339329399,554.472075340119,
555.471811350839,556.471547361559,557.471283372279,558.471019382999,559.47075539372,
560.47049140444,561.47022741516,562.46996342588,563.4696994366,564.46943544732,
565.46917145804,566.46890746876,567.468643479481,568.468379490201,569.468115500921,
570.467851511641,571.467587522361,572.467323533081,573.467059543801,574.466795554521,
575.466531565242,576.466267575962,577.466003586682,578.465739597402,579.465475608122,
580.465211618842,581.464947629562,582.464683640283,583.464419651003,584.464155661723,
585.463891672443,586.463627683163,587.463363693883,588.463099704603,589.462835715323,
590.462571726044,591.462307736764,592.462043747484,593.461779758204,594.461515768924,
595.461251779644,596.460987790364,597.460723801085,598.460459811805,599.460195822525,
600.459931833245,601.459667843965,602.459403854685,603.459139865405,604.458875876125,
605.458611886846,606.458347897566,607.458083908286,608.457819919006,609.457555929726,
610.457291940446,611.457027951166,612.456763961887,613.456499972607,614.456235983327,
615.455971994047,616.455708004767,617.455444015487,618.455180026207,619.454916036927,
620.454652047648,621.454388058368,622.454124069088,623.453860079808,624.453596090528,
625.453332101248,626.453068111968,627.452804122688,628.452540133409,629.452276144129,
630.452012154849,631.451748165569,632.451484176289,633.451220187009,634.450956197729,
635.450692208449,636.45042821917,637.45016422989,638.44990024061,639.44963625133,
640.44937226205,641.44910827277,642.44884428349,643.448580294211,644.448316304931,
645.448052315651,646.447788326371,647.447524337091,648.447260347811,649.446996358531,
650.446732369251,651.446468379972,652.446204390692,653.445940401412,654.445676412132,
655.445412422852,656.445148433572,657.444884444292,658.444620455012,659.444356465733,
660.444092476453,661.443828487173,662.443564497893,663.443300508613,664.443036519333,
665.442772530053,666.442508540774,667.442244551494,668.441980562214,669.441716572934,
670.441452583654,671.441188594374,672.440924605094,673.440660615815,674.440396626535,
675.440132637255,676.439868647975,677.439604658695,678.439340669415,679.439076680135,
680.438812690855,681.438548701576,682.438284712296,683.438020723016,684.437756733736,
685.437492744456,686.437228755176,687.436964765896,688.436700776616,689.436436787337,
690.436172798057,691.435908808777,692.435644819497,693.435380830217,694.435116840937,
695.434852851657,696.434588862377,697.434324873098,698.434060883818,699.433796894538,
700.433532905258,701.433268915978,702.433004926698,703.432740937418,704.432476948139,
705.432212958859,706.431948969579,707.431684980299,708.431420991019,709.431157001739,
710.430893012459,711.430629023179,712.4303650339,713.43010104462,714.42983705534,
715.42957306606,716.42930907678,717.4290450875,718.42878109822,719.42851710894,
720.428253119661,721.427989130381,722.427725141101,723.427461151821,724.427197162541,
725.426933173261,726.426669183981,727.426405194702,728.426141205422,729.425877216142,
730.425613226862,731.425349237582,732.425085248302,733.424821259022,734.424557269742,
735.424293280463,736.424029291183,737.423765301903,738.423501312623,739.423237323343,
740.422973334063,741.422709344783,742.422445355504,743.422181366224,744.421917376944,
745.421653387664,746.421389398384,747.421125409104,748.420861419824,749.420597430544,
750.420333441265,751.420069451985,752.419805462705,753.419541473425,754.419277484145,
755.419013494865,756.418749505585,757.418485516306,758.418221527026,759.417957537746,
760.417693548466,761.417429559186,762.417165569906,763.416901580626,764.416637591346,
765.416373602067,766.416109612787,767.415845623507,768.415581634227,769.415317644947,
770.415053655667,771.414789666387,772.414525677107,773.414261687828,774.413997698548,
775.413733709268,776.413469719988,777.413205730708,778.412941741428,779.412677752148,
780.412413762868,781.412149773589,782.411885784309,783.411621795029,784.411357805749,
785.411093816469,786.410829827189,787.410565837909,788.41030184863,789.41003785935,
790.40977387007,791.40950988079,792.40924589151,793.40898190223,794.40871791295,
795.40845392367,796.408189934391,797.407925945111,798.407661955831,799.407397966551,
800.407133977271,801.406869987991,802.406605998711,803.406342009432,804.406078020152,
805.405814030872,806.405550041592,807.405286052312,808.405022063032,809.404758073752,
810.404494084472,811.404230095193,812.403966105913,813.403702116633,814.403438127353,
815.403174138073,816.402910148793,817.402646159513,818.402382170234,819.402118180954,
820.401854191674,821.401590202394,822.401326213114,823.401062223834,824.400798234554,
825.400534245274,826.400270255995,827.400006266715,828.399742277435,829.399478288155,
830.399214298875,831.398950309595,832.398686320315,833.398422331035,834.398158341756,
835.397894352476,836.397630363196,837.397366373916,838.397102384636,839.396838395356,
840.396574406076,841.396310416796,842.396046427517,843.395782438237,844.395518448957,
845.395254459677,846.394990470397,847.394726481117,848.394462491837,849.394198502558,
850.393934513278,851.393670523998,852.393406534718,853.393142545438,854.392878556158,
855.392614566878,856.392350577598,857.392086588319,858.391822599039,859.391558609759,
860.391294620479,861.391030631199,862.390766641919,863.390502652639,864.390238663359,
865.38997467408,866.3897106848,867.38944669552,868.38918270624,869.38891871696,
870.38865472768,871.3883907384,872.388126749121,873.387862759841,874.387598770561,
875.387334781281,876.387070792001,877.386806802721,878.386542813441,879.386278824161,
880.386014834882,881.385750845602,882.385486856322,883.385222867042,884.384958877762,
885.384694888482,886.384430899202,887.384166909923,888.383902920643,889.383638931363,
890.383374942083,891.383110952803,892.382846963523,893.382582974243,894.382318984963,
895.382054995684,896.381791006404,897.381527017124,898.381263027844,899.380999038564,
900.380735049284,901.380471060004,902.380207070725,903.379943081445,904.379679092165,
905.379415102885,906.379151113605,907.378887124325,908.378623135045,909.378359145765,
910.378095156486,911.377831167206,912.377567177926,913.377303188646,914.377039199366,
915.376775210086,916.376511220806,917.376247231526,918.375983242247,919.375719252967,
920.375455263687,921.375191274407,922.374927285127,923.374663295847,924.374399306567,
925.374135317287,926.373871328008,927.373607338728,928.373343349448,929.373079360168,
930.372815370888,931.372551381608,932.372287392328,933.372023403049,934.371759413769,
935.371495424489,936.371231435209,937.370967445929,938.370703456649,939.370439467369,
940.370175478089,941.36991148881,942.36964749953,943.36938351025,944.36911952097,
945.36885553169,946.36859154241,947.36832755313,948.368063563851,949.367799574571,
950.367535585291,951.367271596011,952.367007606731,953.366743617451,954.366479628171,
955.366215638891,956.365951649612,957.365687660332,958.365423671052,959.365159681772,
960.364895692492,961.364631703212,962.364367713932,963.364103724653,964.363839735373,
965.363575746093,966.363311756813,967.363047767533,968.362783778253,969.362519788973,
970.362255799693,971.361991810414,972.361727821134,973.361463831854,974.361199842574,
975.360935853294,976.360671864014,977.360407874734,978.360143885454,979.359879896175,
980.359615906895,981.359351917615,982.359087928335,983.358823939055,984.358559949775,
985.358295960495,986.358031971215,987.357767981936,988.357503992656,989.357240003376,
990.356976014096,991.356712024816,992.356448035536,993.356184046256,994.355920056977,
995.355656067697,996.355392078417,997.355128089137,998.354864099857,999.354600110577,
1000.3543361213,1001.35407213202,1002.35380814274,1003.35354415346,1004.35328016418,
1005.3530161749,1006.35275218562,1007.35248819634,1008.35222420706,1009.35196021778,
1010.3516962285,1011.35143223922,1012.35116824994,1013.35090426066,1014.35064027138,
1015.3503762821,1016.35011229282,1017.34984830354,1018.34958431426,1019.34932032498,
1020.3490563357,1021.34879234642,1022.34852835714,1023.34826436786,1024.34800037858,
1025.3477363893,1026.34747240002,1027.34720841074,1028.34694442146,1029.34668043218,
1030.3464164429,1031.34615245362,1032.34588846434,1033.34562447506,1034.34536048578,
1035.3450964965,1036.34483250722,1037.34456851794,1038.34430452866,1039.34404053938,
1040.3437765501,1041.34351256082,1042.34324857154,1043.34298458226,1044.34272059298,
1045.3424566037,1046.34219261442,1047.34192862514,1048.34166463586,1049.34140064658,
1050.3411366573,1051.34087266802,1052.34060867874,1053.34034468946,1054.34008070018,
1055.3398167109,1056.33955272162,1057.33928873234,1058.33902474307,1059.33876075378,
1060.33849676451,1061.33823277523,1062.33796878595,1063.33770479667,1064.33744080739,
1065.33717681811,1066.33691282883,1067.33664883955,1068.33638485027,1069.33612086099,
1070.33585687171,1071.33559288243,1072.33532889315,1073.33506490387,1074.33480091459,
1075.33453692531,1076.33427293603,1077.33400894675,1078.33374495747,1079.33348096819,
1080.33321697891,1081.33295298963,1082.33268900035,1083.33242501107,1084.33216102179,
1085.33189703251,1086.33163304323,1087.33136905395,1088.33110506467,1089.33084107539,
1090.33057708611,1091.33031309683,1092.33004910755,1093.32978511827,1094.32952112899,
1095.32925713971,1096.32899315043,1097.32872916115,1098.32846517187,1099.32820118259,
1100.32793719331,1101.32767320403,1102.32740921475,1103.32714522547,1104.32688123619,
1105.32661724691,1106.32635325763,1107.32608926835,1108.32582527907,1109.32556128979,
1110.32529730051,1111.32503331123,1112.32476932195,1113.32450533267,1114.32424134339,
1115.32397735411,1116.32371336483,1117.32344937555,1118.32318538627,1119.32292139699,
1120.32265740771,1121.32239341843,1122.32212942915,1123.32186543987,1124.32160145059,
1125.32133746131,1126.32107347203,1127.32080948275,1128.32054549347,1129.32028150419,
1130.32001751491,1131.31975352563,1132.31948953635,1133.31922554707,1134.31896155779,
1135.31869756852,1136.31843357924,1137.31816958996,1138.31790560068,1139.3176416114,
1140.31737762212,1141.31711363284,1142.31684964356,1143.31658565428,1144.316321665,
1145.31605767572,1146.31579368644,1147.31552969716,1148.31526570788,1149.3150017186,
1150.31473772932,1151.31447374004,1152.31420975076,1153.31394576148,1154.3136817722,
1155.31341778292,1156.31315379364,1157.31288980436,1158.31262581508,1159.3123618258,
1160.31209783652,1161.31183384724,1162.31156985796,1163.31130586868,1164.3110418794,
1165.31077789012,1166.31051390084,1167.31024991156,1168.30998592228,1169.309721933,
1170.30945794372,1171.30919395444,1172.30892996516,1173.30866597588,1174.3084019866,
1175.30813799732,1176.30787400804,1177.30761001876,1178.30734602948,1179.3070820402,
1180.30681805092,1181.30655406164,1182.30629007236,1183.30602608308,1184.3057620938,
1185.30549810452,1186.30523411524,1187.30497012596,1188.30470613668,1189.3044421474,
1190.30417815812,1191.30391416884,1192.30365017956,1193.30338619028,1194.303122201,
1195.30285821172,1196.30259422244,1197.30233023316,1198.30206624388,1199.3018022546,
1200.30153826532,1201.30127427604,1202.30101028676,1203.30074629748,1204.3004823082,
1205.30021831892,1206.29995432964,1207.29969034036,1208.29942635108,1209.2991623618,
1210.29889837252,1211.29863438324,1212.29837039397,1213.29810640469,1214.29784241541,
1215.29757842613,1216.29731443685,1217.29705044757,1218.29678645829,1219.29652246901,
1220.29625847973,1221.29599449045,1222.29573050117,1223.29546651189,1224.29520252261,
1225.29493853333,1226.29467454405,1227.29441055477,1228.29414656549,1229.29388257621,
1230.29361858693,1231.29335459765,1232.29309060837,1233.29282661909,1234.29256262981,
1235.29229864053,1236.29203465125,1237.29177066197,1238.29150667269,1239.29124268341,
1240.29097869413,1241.29071470485,1242.29045071557,1243.29018672629,1244.28992273701,
1245.28965874773,1246.28939475845,1247.28913076917,1248.28886677989,1249.28860279061,
1250.28833880133,1251.28807481205,1252.28781082277,1253.28754683349,1254.28728284421,
1255.28701885493,1256.28675486565,1257.28649087637,1258.28622688709,1259.28596289781,
1260.28569890853,1261.28543491925,1262.28517092997,1263.28490694069,1264.28464295141,
1265.28437896213,1266.28411497285,1267.28385098357,1268.28358699429,1269.28332300501,
1270.28305901573,1271.28279502645,1272.28253103717,1273.28226704789,1274.28200305861,
1275.28173906933,1276.28147508005,1277.28121109077,1278.28094710149,1279.28068311221,
1280.28041912293,1281.28015513365,1282.27989114437,1283.27962715509,1284.27936316581,
1285.27909917653,1286.27883518725,1287.27857119797,1288.2783072087,1289.27804321942,
1290.27777923014,1291.27751524086,1292.27725125158,1293.2769872623,1294.27672327302,
1295.27645928374,1296.27619529446,1297.27593130518,1298.2756673159,1299.27540332662,
1300.27513933734,1301.27487534806,1302.27461135878,1303.2743473695,1304.27408338022,
1305.27381939094,1306.27355540166,1307.27329141238,1308.2730274231,1309.27276343382,
1310.27249944454,1311.27223545526,1312.27197146598,1313.2717074767,1314.27144348742,
1315.27117949814,1316.27091550886,1317.27065151958,1318.2703875303,1319.27012354102,
1320.26985955174,1321.26959556246,1322.26933157318,1323.2690675839,1324.26880359462,
1325.26853960534,1326.26827561606,1327.26801162678,1328.2677476375,1329.26748364822,
1330.26721965894,1331.26695566966,1332.26669168038,1333.2664276911,1334.26616370182,
1335.26589971254,1336.26563572326,1337.26537173398,1338.2651077447,1339.26484375542,
1340.26457976614,1341.26431577686,1342.26405178758,1343.2637877983,1344.26352380902,
1345.26325981974,1346.26299583046,1347.26273184118,1348.2624678519,1349.26220386262,
1350.26193987334,1351.26167588406,1352.26141189478,1353.2611479055,1354.26088391622,
1355.26061992694,1356.26035593766,1357.26009194838,1358.2598279591,1359.25956396982,
1360.25929998054,1361.25903599126,1362.25877200198,1363.2585080127,1364.25824402343,
1365.25798003415,1366.25771604487,1367.25745205559,1368.25718806631,1369.25692407703,
1370.25666008775,1371.25639609847,1372.25613210919,1373.25586811991,1374.25560413063,
1375.25534014135,1376.25507615207,1377.25481216279,1378.25454817351,1379.25428418423,
1380.25402019495,1381.25375620567,1382.25349221639,1383.25322822711,1384.25296423783,
1385.25270024855,1386.25243625927,1387.25217226999,1388.25190828071,1389.25164429143,
1390.25138030215,1391.25111631287,1392.25085232359,1393.25058833431,1394.25032434503,
1395.25006035575,1396.24979636647,1397.24953237719,1398.24926838791,1399.24900439863,
1400.24874040935,1401.24847642007,1402.24821243079,1403.24794844151,1404.24768445223,
1405.24742046295,1406.24715647367,1407.24689248439,1408.24662849511,1409.24636450583,
1410.24610051655,1411.24583652727,1412.24557253799,1413.24530854871,1414.24504455943,
1415.24478057015,1416.24451658087,1417.24425259159,1418.24398860231,1419.24372461303,
1420.24346062375,1421.24319663447,1422.24293264519,1423.24266865591,1424.24240466663,
1425.24214067735,1426.24187668807,1427.24161269879,1428.24134870951,1429.24108472023,
1430.24082073095,1431.24055674167,1432.24029275239,1433.24002876311,1434.23976477383,
1435.23950078455,1436.23923679527,1437.23897280599,1438.23870881671,1439.23844482743,
1440.23818083815,1441.23791684888,1442.2376528596,1443.23738887032,1444.23712488104,
1445.23686089176,1446.23659690248,1447.2363329132,1448.23606892392,1449.23580493464,
1450.23554094536,1451.23527695608,1452.2350129668,1453.23474897752,1454.23448498824,
1455.23422099896,1456.23395700968,1457.2336930204,1458.23342903112,1459.23316504184,
1460.23290105256,1461.23263706328,1462.232373074,1463.23210908472,1464.23184509544,
1465.23158110616,1466.23131711688,1467.2310531276,1468.23078913832,1469.23052514904,
1470.23026115976,1471.22999717048,1472.2297331812,1473.22946919192,1474.22920520264,
1475.22894121336,1476.22867722408,1477.2284132348,1478.22814924552,1479.22788525624,
1480.22762126696,1481.22735727768,1482.2270932884,1483.22682929912,1484.22656530984,
1485.22630132056,1486.22603733128,1487.225773342,1488.22550935272,1489.22524536344,
1490.22498137416,1491.22471738488,1492.2244533956,1493.22418940632,1494.22392541704,
1495.22366142776,1496.22339743848,1497.2231334492,1498.22286945992,1499.22260547064,
1500.22234148136,1501.22207749208,1502.2218135028,1503.22154951352,1504.22128552424,
1505.22102153496,1506.22075754568,1507.2204935564,1508.22022956712,1509.21996557784,
1510.21970158856,1511.21943759928,1512.21917361,1513.21890962072,1514.21864563144,
1515.21838164216,1516.21811765288,1517.21785366361,1518.21758967433,1519.21732568505,
1520.21706169577,1521.21679770649,1522.21653371721,1523.21626972793,1524.21600573865,
1525.21574174937,1526.21547776009,1527.21521377081,1528.21494978153,1529.21468579225,
1530.21442180297,1531.21415781369,1532.21389382441,1533.21362983513,1534.21336584585,
1535.21310185657,1536.21283786729,1537.21257387801,1538.21230988873,1539.21204589945,
1540.21178191017,1541.21151792089,1542.21125393161,1543.21098994233,1544.21072595305,
1545.21046196377,1546.21019797449,1547.20993398521,1548.20966999593,1549.20940600665,
1550.20914201737,1551.20887802809,1552.20861403881,1553.20835004953,1554.20808606025,
1555.20782207097,1556.20755808169,1557.20729409241,1558.20703010313,1559.20676611385,
1560.20650212457,1561.20623813529,1562.20597414601,1563.20571015673,1564.20544616745,
1565.20518217817,1566.20491818889,1567.20465419961,1568.20439021033,1569.20412622105,
1570.20386223177,1571.20359824249,1572.20333425321,1573.20307026393,1574.20280627465,
1575.20254228537,1576.20227829609,1577.20201430681,1578.20175031753,1579.20148632825,
1580.20122233897,1581.20095834969,1582.20069436041,1583.20043037113,1584.20016638185,
1585.19990239257,1586.19963840329,1587.19937441401,1588.19911042473,1589.19884643545,
1590.19858244617,1591.19831845689,1592.19805446761,1593.19779047834,1594.19752648906,
1595.19726249978,1596.1969985105,1597.19673452122,1598.19647053194,1599.19620654266,
1600.19594255338,1601.1956785641,1602.19541457482,1603.19515058554,1604.19488659626,
1605.19462260698,1606.1943586177,1607.19409462842,1608.19383063914,1609.19356664986,
1610.19330266058,1611.1930386713,1612.19277468202,1613.19251069274,1614.19224670346,
1615.19198271418,1616.1917187249,1617.19145473562,1618.19119074634,1619.19092675706,
1620.19066276778,1621.1903987785,1622.19013478922,1623.18987079994,1624.18960681066,
1625.18934282138,1626.1890788321,1627.18881484282,1628.18855085354,1629.18828686426,
1630.18802287498,1631.1877588857,1632.18749489642,1633.18723090714,1634.18696691786,
1635.18670292858,1636.1864389393,1637.18617495002,1638.18591096074,1639.18564697146,
1640.18538298218,1641.1851189929,1642.18485500362,1643.18459101434,1644.18432702506,
1645.18406303578,1646.1837990465,1647.18353505722,1648.18327106794,1649.18300707866,
1650.18274308938,1651.1824791001,1652.18221511082,1653.18195112154,1654.18168713226,
1655.18142314298,1656.1811591537,1657.18089516442,1658.18063117514,1659.18036718586,
1660.18010319658,1661.1798392073,1662.17957521802,1663.17931122874,1664.17904723946,
1665.17878325018,1666.1785192609,1667.17825527162,1668.17799128234,1669.17772729307,
1670.17746330379,1671.17719931451,1672.17693532523,1673.17667133595,1674.17640734667,
1675.17614335739,1676.17587936811,1677.17561537883,1678.17535138955,1679.17508740027,
1680.17482341099,1681.17455942171,1682.17429543243,1683.17403144315,1684.17376745387,
1685.17350346459,1686.17323947531,1687.17297548603,1688.17271149675,1689.17244750747,
1690.17218351819,1691.17191952891,1692.17165553963,1693.17139155035,1694.17112756107,
1695.17086357179,1696.17059958251,1697.17033559323,1698.17007160395,1699.16980761467,
1700.16954362539,1700.66941163075,1701.16959429301),.UNSPECIFIED.);
#56=B_SPLINE_SURFACE_WITH_KNOTS('',3,3,((#272352,#272353,#272354,#272355,
#272356,#272357,#272358,#272359,#272360,#272361,#272362,#272363,#272364,
#272365,#272366,#272367,#272368,#272369,#272370,#272371,#272372,#272373,
#272374,#272375,#272376,#272377,#272378,#272379,#272380,#272381,#272382,
#272383,#272384,#272385,#272386,#272387,#272388,#272389,#272390,#272391,
#272392,#272393,#272394,#272395,#272396,#272397,#272398,#272399,#272400,
#272401,#272402,#272403,#272404,#272405,#272406,#272407,#272408,#272409,
#272410,#272411,#272412,#272413,#272414,#272415,#272416,#272417,#272418,
#272419,#272420,#272421,#272422,#272423,#272424,#272425,#272426,#272427,
#272428,#272429,#272430,#272431,#272432,#272433,#272434,#272435,#272436,
#272437,#272438,#272439,#272440,#272441,#272442,#272443,#272444,#272445,
#272446,#272447,#272448,#272449,#272450,#272451,#272452,#272453,#272454,
#272455,#272456,#272457,#272458,#272459,#272460,#272461,#272462,#272463,
#272464,#272465,#272466,#272467,#272468,#272469,#272470,#272471,#272472,
#272473,#272474,#272475,#272476,#272477,#272478,#272479,#272480,#272481,
#272482,#272483,#272484,#272485,#272486,#272487,#272488,#272489,#272490,
#272491,#272492,#272493,#272494,#272495,#272496,#272497,#272498,#272499,
#272500,#272501,#272502,#272503,#272504,#272505,#272506,#272507,#272508,
#272509,#272510,#272511,#272512,#272513,#272514,#272515,#272516,#272517,
#272518,#272519,#272520,#272521,#272522,#272523,#272524,#272525,#272526,
#272527,#272528,#272529,#272530,#272531,#272532,#272533,#272534,#272535,
#272536,#272537,#272538,#272539,#272540,#272541,#272542,#272543,#272544,
#272545,#272546,#272547,#272548,#272549,#272550,#272551,#272552,#272553,
#272554,#272555,#272556,#272557,#272558,#272559,#272560,#272561,#272562,
#272563,#272564,#272565,#272566,#272567,#272568,#272569,#272570,#272571,
#272572,#272573,#272574,#272575,#272576,#272577,#272578,#272579,#272580,
#272581,#272582,#272583,#272584,#272585,#272586,#272587,#272588,#272589,
#272590,#272591,#272592,#272593,#272594,#272595,#272596,#272597,#272598,
#272599,#272600,#272601,#272602,#272603,#272604,#272605,#272606,#272607,
#272608,#272609,#272610,#272611,#272612,#272613,#272614,#272615,#272616,
#272617,#272618,#272619,#272620,#272621,#272622,#272623,#272624,#272625,
#272626,#272627,#272628,#272629,#272630,#272631,#272632,#272633,#272634,
#272635,#272636,#272637,#272638,#272639,#272640,#272641,#272642,#272643,
#272644,#272645,#272646,#272647,#272648,#272649,#272650,#272651,#272652,
#272653,#272654,#272655,#272656,#272657,#272658,#272659,#272660,#272661,
#272662,#272663,#272664,#272665,#272666,#272667,#272668,#272669,#272670,
#272671,#272672,#272673,#272674,#272675,#272676,#272677,#272678,#272679,
#272680,#272681,#272682,#272683,#272684,#272685,#272686,#272687,#272688,
#272689,#272690,#272691,#272692,#272693,#272694,#272695,#272696,#272697,
#272698,#272699,#272700,#272701,#272702,#272703,#272704,#272705,#272706,
#272707,#272708,#272709,#272710,#272711,#272712,#272713,#272714,#272715,
#272716,#272717,#272718,#272719,#272720,#272721,#272722,#272723,#272724,
#272725,#272726,#272727,#272728,#272729,#272730,#272731,#272732,#272733,
#272734,#272735,#272736,#272737,#272738,#272739,#272740,#272741,#272742,
#272743,#272744,#272745,#272746,#272747,#272748,#272749,#272750,#272751,
#272752,#272753,#272754,#272755,#272756,#272757,#272758,#272759,#272760,
#272761,#272762,#272763,#272764,#272765,#272766,#272767,#272768,#272769,
#272770,#272771,#272772,#272773,#272774,#272775,#272776,#272777,#272778,
#272779,#272780,#272781,#272782,#272783,#272784,#272785,#272786,#272787,
#272788,#272789,#272790,#272791,#272792,#272793,#272794,#272795,#272796,
#272797,#272798,#272799,#272800,#272801,#272802,#272803,#272804,#272805,
#272806,#272807,#272808,#272809,#272810,#272811,#272812,#272813,#272814,
#272815,#272816,#272817,#272818,#272819,#272820,#272821,#272822,#272823,
#272824,#272825,#272826,#272827,#272828,#272829,#272830,#272831,#272832,
#272833,#272834,#272835,#272836,#272837,#272838,#272839,#272840,#272841,
#272842,#272843,#272844,#272845,#272846,#272847,#272848,#272849,#272850,
#272851,#272852,#272853,#272854,#272855,#272856,#272857,#272858,#272859,
#272860,#272861,#272862,#272863,#272864,#272865,#272866,#272867,#272868,
#272869,#272870,#272871,#272872,#272873,#272874,#272875,#272876,#272877,
#272878,#272879,#272880,#272881,#272882,#272883,#272884,#272885,#272886,
#272887,#272888,#272889,#272890,#272891,#272892,#272893,#272894,#272895,
#272896,#272897,#272898,#272899,#272900,#272901,#272902,#272903,#272904,
#272905,#272906,#272907,#272908,#272909,#272910,#272911,#272912,#272913,
#272914,#272915,#272916,#272917,#272918,#272919,#272920,#272921,#272922,
#272923,#272924,#272925,#272926,#272927,#272928,#272929,#272930,#272931,
#272932,#272933,#272934,#272935,#272936,#272937,#272938,#272939,#272940,
#272941,#272942,#272943,#272944,#272945,#272946,#272947,#272948,#272949,
#272950,#272951,#272952,#272953,#272954,#272955,#272956,#272957,#272958,
#272959,#272960,#272961,#272962,#272963,#272964,#272965,#272966,#272967,
#272968,#272969,#272970,#272971,#272972,#272973,#272974,#272975,#272976,
#272977,#272978,#272979,#272980,#272981,#272982,#272983,#272984,#272985,
#272986,#272987,#272988,#272989,#272990,#272991,#272992,#272993,#272994,
#272995,#272996,#272997,#272998,#272999,#273000,#273001,#273002,#273003,
#273004,#273005,#273006,#273007,#273008,#273009,#273010,#273011,#273012,
#273013,#273014,#273015,#273016,#273017,#273018,#273019,#273020,#273021,
#273022,#273023,#273024,#273025,#273026,#273027,#273028,#273029,#273030,
#273031,#273032,#273033,#273034,#273035,#273036,#273037,#273038,#273039,
#273040,#273041,#273042,#273043,#273044,#273045,#273046,#273047,#273048,
#273049,#273050,#273051,#273052,#273053,#273054,#273055,#273056,#273057,
#273058,#273059,#273060,#273061,#273062,#273063,#273064,#273065,#273066,
#273067,#273068,#273069,#273070,#273071,#273072,#273073,#273074,#273075,
#273076,#273077,#273078,#273079,#273080,#273081,#273082,#273083,#273084,
#273085,#273086,#273087,#273088,#273089,#273090,#273091,#273092,#273093,
#273094,#273095,#273096,#273097,#273098,#273099,#273100,#273101,#273102,
#273103,#273104,#273105,#273106,#273107,#273108,#273109,#273110,#273111,
#273112,#273113,#273114,#273115,#273116,#273117,#273118,#273119,#273120,
#273121,#273122,#273123,#273124,#273125,#273126,#273127,#273128,#273129,
#273130,#273131,#273132,#273133,#273134,#273135,#273136,#273137,#273138,
#273139,#273140,#273141,#273142,#273143,#273144,#273145,#273146,#273147,
#273148,#273149,#273150,#273151,#273152,#273153,#273154,#273155,#273156,
#273157,#273158,#273159,#273160,#273161,#273162,#273163,#273164,#273165,
#273166,#273167,#273168,#273169,#273170,#273171,#273172,#273173,#273174,
#273175,#273176,#273177,#273178,#273179,#273180,#273181,#273182,#273183,
#273184,#273185,#273186,#273187,#273188,#273189,#273190,#273191,#273192,
#273193,#273194,#273195,#273196,#273197,#273198,#273199,#273200,#273201,
#273202,#273203,#273204,#273205,#273206,#273207,#273208,#273209,#273210,
#273211,#273212,#273213,#273214,#273215,#273216,#273217,#273218,#273219,
#273220,#273221,#273222,#273223,#273224,#273225,#273226,#273227,#273228,
#273229,#273230,#273231,#273232,#273233,#273234,#273235,#273236,#273237,
#273238,#273239,#273240,#273241,#273242,#273243,#273244,#273245,#273246,
#273247,#273248,#273249,#273250,#273251,#273252,#273253,#273254,#273255,
#273256,#273257,#273258,#273259,#273260,#273261,#273262,#273263,#273264,
#273265,#273266,#273267,#273268,#273269,#273270,#273271,#273272,#273273,
#273274,#273275,#273276,#273277,#273278,#273279,#273280,#273281,#273282,
#273283,#273284,#273285,#273286,#273287,#273288,#273289,#273290,#273291,
#273292,#273293,#273294,#273295,#273296,#273297,#273298,#273299,#273300,
#273301,#273302,#273303,#273304,#273305,#273306,#273307,#273308,#273309,
#273310,#273311,#273312,#273313,#273314,#273315,#273316,#273317,#273318,
#273319,#273320,#273321,#273322,#273323,#273324,#273325,#273326,#273327,
#273328,#273329,#273330,#273331,#273332,#273333,#273334,#273335,#273336,
#273337,#273338,#273339,#273340,#273341,#273342,#273343,#273344,#273345,
#273346,#273347,#273348,#273349,#273350,#273351,#273352,#273353,#273354,
#273355,#273356,#273357,#273358,#273359,#273360,#273361,#273362,#273363,
#273364,#273365,#273366,#273367,#273368,#273369,#273370,#273371,#273372,
#273373,#273374,#273375,#273376,#273377,#273378,#273379,#273380,#273381,
#273382,#273383,#273384,#273385,#273386,#273387,#273388,#273389,#273390,
#273391,#273392,#273393,#273394,#273395,#273396,#273397,#273398,#273399,
#273400,#273401,#273402,#273403,#273404,#273405,#273406,#273407,#273408,
#273409,#273410,#273411,#273412,#273413,#273414,#273415,#273416,#273417,
#273418,#273419,#273420,#273421,#273422,#273423,#273424,#273425,#273426,
#273427,#273428,#273429,#273430,#273431,#273432,#273433,#273434,#273435,
#273436,#273437,#273438,#273439,#273440,#273441,#273442,#273443,#273444,
#273445,#273446,#273447,#273448,#273449,#273450,#273451,#273452,#273453,
#273454,#273455,#273456,#273457,#273458,#273459,#273460,#273461,#273462,
#273463,#273464,#273465,#273466,#273467,#273468,#273469,#273470,#273471,
#273472,#273473,#273474,#273475,#273476,#273477,#273478,#273479,#273480,
#273481,#273482,#273483,#273484,#273485,#273486,#273487,#273488,#273489,
#273490,#273491,#273492,#273493,#273494,#273495,#273496,#273497,#273498,
#273499,#273500,#273501,#273502,#273503,#273504,#273505,#273506,#273507,
#273508,#273509,#273510,#273511,#273512,#273513,#273514,#273515,#273516,
#273517,#273518,#273519,#273520,#273521,#273522,#273523,#273524,#273525,
#273526,#273527,#273528,#273529,#273530,#273531,#273532,#273533,#273534,
#273535,#273536,#273537,#273538,#273539,#273540,#273541,#273542,#273543,
#273544,#273545,#273546,#273547,#273548,#273549,#273550,#273551,#273552,
#273553,#273554,#273555,#273556,#273557,#273558,#273559,#273560,#273561,
#273562,#273563,#273564,#273565,#273566,#273567,#273568,#273569,#273570,
#273571,#273572,#273573,#273574,#273575,#273576,#273577,#273578,#273579,
#273580,#273581,#273582,#273583,#273584,#273585,#273586,#273587,#273588,
#273589,#273590,#273591,#273592,#273593,#273594,#273595,#273596,#273597,
#273598,#273599,#273600,#273601,#273602,#273603,#273604,#273605,#273606,
#273607,#273608,#273609,#273610,#273611,#273612,#273613,#273614,#273615,
#273616,#273617,#273618,#273619,#273620,#273621,#273622,#273623,#273624,
#273625,#273626,#273627,#273628,#273629,#273630,#273631,#273632,#273633,
#273634,#273635,#273636,#273637,#273638,#273639,#273640,#273641,#273642,
#273643,#273644,#273645,#273646,#273647,#273648,#273649,#273650,#273651,
#273652,#273653,#273654,#273655,#273656,#273657,#273658,#273659,#273660,
#273661,#273662,#273663,#273664,#273665,#273666,#273667,#273668,#273669,
#273670,#273671,#273672,#273673,#273674,#273675,#273676,#273677,#273678,
#273679,#273680,#273681,#273682,#273683,#273684,#273685,#273686,#273687,
#273688,#273689,#273690,#273691,#273692,#273693,#273694,#273695,#273696,
#273697,#273698,#273699,#273700,#273701,#273702,#273703,#273704,#273705,
#273706,#273707,#273708,#273709,#273710,#273711,#273712,#273713,#273714,
#273715,#273716,#273717,#273718,#273719,#273720,#273721,#273722,#273723,
#273724,#273725,#273726,#273727,#273728,#273729,#273730,#273731,#273732,
#273733,#273734,#273735,#273736,#273737,#273738,#273739,#273740,#273741,
#273742,#273743,#273744,#273745,#273746,#273747,#273748,#273749,#273750,
#273751,#273752,#273753,#273754,#273755,#273756,#273757,#273758,#273759,
#273760,#273761,#273762,#273763,#273764,#273765,#273766,#273767,#273768,
#273769,#273770,#273771,#273772,#273773,#273774,#273775,#273776,#273777,
#273778,#273779,#273780,#273781,#273782,#273783,#273784,#273785,#273786,
#273787,#273788,#273789,#273790,#273791,#273792,#273793,#273794,#273795,
#273796,#273797,#273798,#273799,#273800,#273801,#273802,#273803,#273804,
#273805,#273806,#273807,#273808,#273809,#273810,#273811,#273812,#273813,
#273814,#273815,#273816,#273817,#273818,#273819,#273820,#273821,#273822,
#273823,#273824,#273825,#273826,#273827,#273828,#273829,#273830,#273831,
#273832,#273833,#273834,#273835,#273836,#273837,#273838,#273839,#273840,
#273841,#273842,#273843,#273844,#273845,#273846,#273847,#273848,#273849,
#273850,#273851,#273852,#273853,#273854,#273855,#273856,#273857,#273858,
#273859,#273860,#273861,#273862,#273863,#273864,#273865,#273866,#273867,
#273868,#273869,#273870,#273871,#273872,#273873,#273874,#273875,#273876,
#273877,#273878,#273879,#273880,#273881,#273882,#273883,#273884,#273885,
#273886,#273887,#273888,#273889,#273890,#273891,#273892,#273893,#273894,
#273895,#273896,#273897,#273898,#273899,#273900,#273901,#273902,#273903,
#273904,#273905,#273906,#273907,#273908,#273909,#273910,#273911,#273912,
#273913,#273914,#273915,#273916,#273917,#273918,#273919,#273920,#273921,
#273922,#273923,#273924,#273925,#273926,#273927,#273928,#273929,#273930,
#273931,#273932,#273933,#273934,#273935,#273936,#273937,#273938,#273939,
#273940,#273941,#273942,#273943,#273944,#273945,#273946,#273947,#273948,
#273949,#273950,#273951,#273952,#273953,#273954,#273955,#273956,#273957,
#273958,#273959,#273960,#273961,#273962,#273963,#273964,#273965,#273966,
#273967,#273968,#273969,#273970,#273971,#273972,#273973,#273974,#273975,
#273976,#273977,#273978,#273979,#273980,#273981,#273982,#273983,#273984,
#273985,#273986,#273987,#273988,#273989,#273990,#273991,#273992,#273993,
#273994,#273995,#273996,#273997,#273998,#273999,#274000,#274001,#274002,
#274003,#274004,#274005,#274006,#274007,#274008,#274009,#274010,#274011,
#274012,#274013,#274014,#274015,#274016,#274017,#274018,#274019,#274020,
#274021,#274022,#274023,#274024,#274025,#274026,#274027,#274028,#274029,
#274030,#274031,#274032,#274033,#274034,#274035,#274036,#274037,#274038,
#274039,#274040,#274041,#274042,#274043,#274044,#274045,#274046),(#274047,
#274048,#274049,#274050,#274051,#274052,#274053,#274054,#274055,#274056,
#274057,#274058,#274059,#274060,#274061,#274062,#274063,#274064,#274065,
#274066,#274067,#274068,#274069,#274070,#274071,#274072,#274073,#274074,
#274075,#274076,#274077,#274078,#274079,#274080,#274081,#274082,#274083,
#274084,#274085,#274086,#274087,#274088,#274089,#274090,#274091,#274092,
#274093,#274094,#274095,#274096,#274097,#274098,#274099,#274100,#274101,
#274102,#274103,#274104,#274105,#274106,#274107,#274108,#274109,#274110,
#274111,#274112,#274113,#274114,#274115,#274116,#274117,#274118,#274119,
#274120,#274121,#274122,#274123,#274124,#274125,#274126,#274127,#274128,
#274129,#274130,#274131,#274132,#274133,#274134,#274135,#274136,#274137,
#274138,#274139,#274140,#274141,#274142,#274143,#274144,#274145,#274146,
#274147,#274148,#274149,#274150,#274151,#274152,#274153,#274154,#274155,
#274156,#274157,#274158,#274159,#274160,#274161,#274162,#274163,#274164,
#274165,#274166,#274167,#274168,#274169,#274170,#274171,#274172,#274173,
#274174,#274175,#274176,#274177,#274178,#274179,#274180,#274181,#274182,
#274183,#274184,#274185,#274186,#274187,#274188,#274189,#274190,#274191,
#274192,#274193,#274194,#274195,#274196,#274197,#274198,#274199,#274200,
#274201,#274202,#274203,#274204,#274205,#274206,#274207,#274208,#274209,
#274210,#274211,#274212,#274213,#274214,#274215,#274216,#274217,#274218,
#274219,#274220,#274221,#274222,#274223,#274224,#274225,#274226,#274227,
#274228,#274229,#274230,#274231,#274232,#274233,#274234,#274235,#274236,
#274237,#274238,#274239,#274240,#274241,#274242,#274243,#274244,#274245,
#274246,#274247,#274248,#274249,#274250,#274251,#274252,#274253,#274254,
#274255,#274256,#274257,#274258,#274259,#274260,#274261,#274262,#274263,
#274264,#274265,#274266,#274267,#274268,#274269,#274270,#274271,#274272,
#274273,#274274,#274275,#274276,#274277,#274278,#274279,#274280,#274281,
#274282,#274283,#274284,#274285,#274286,#274287,#274288,#274289,#274290,
#274291,#274292,#274293,#274294,#274295,#274296,#274297,#274298,#274299,
#274300,#274301,#274302,#274303,#274304,#274305,#274306,#274307,#274308,
#274309,#274310,#274311,#274312,#274313,#274314,#274315,#274316,#274317,
#274318,#274319,#274320,#274321,#274322,#274323,#274324,#274325,#274326,
#274327,#274328,#274329,#274330,#274331,#274332,#274333,#274334,#274335,
#274336,#274337,#274338,#274339,#274340,#274341,#274342,#274343,#274344,
#274345,#274346,#274347,#274348,#274349,#274350,#274351,#274352,#274353,
#274354,#274355,#274356,#274357,#274358,#274359,#274360,#274361,#274362,
#274363,#274364,#274365,#274366,#274367,#274368,#274369,#274370,#274371,
#274372,#274373,#274374,#274375,#274376,#274377,#274378,#274379,#274380,
#274381,#274382,#274383,#274384,#274385,#274386,#274387,#274388,#274389,
#274390,#274391,#274392,#274393,#274394,#274395,#274396,#274397,#274398,
#274399,#274400,#274401,#274402,#274403,#274404,#274405,#274406,#274407,
#274408,#274409,#274410,#274411,#274412,#274413,#274414,#274415,#274416,
#274417,#274418,#274419,#274420,#274421,#274422,#274423,#274424,#274425,
#274426,#274427,#274428,#274429,#274430,#274431,#274432,#274433,#274434,
#274435,#274436,#274437,#274438,#274439,#274440,#274441,#274442,#274443,
#274444,#274445,#274446,#274447,#274448,#274449,#274450,#274451,#274452,
#274453,#274454,#274455,#274456,#274457,#274458,#274459,#274460,#274461,
#274462,#274463,#274464,#274465,#274466,#274467,#274468,#274469,#274470,
#274471,#274472,#274473,#274474,#274475,#274476,#274477,#274478,#274479,
#274480,#274481,#274482,#274483,#274484,#274485,#274486,#274487,#274488,
#274489,#274490,#274491,#274492,#274493,#274494,#274495,#274496,#274497,
#274498,#274499,#274500,#274501,#274502,#274503,#274504,#274505,#274506,
#274507,#274508,#274509,#274510,#274511,#274512,#274513,#274514,#274515,
#274516,#274517,#274518,#274519,#274520,#274521,#274522,#274523,#274524,
#274525,#274526,#274527,#274528,#274529,#274530,#274531,#274532,#274533,
#274534,#274535,#274536,#274537,#274538,#274539,#274540,#274541,#274542,
#274543,#274544,#274545,#274546,#274547,#274548,#274549,#274550,#274551,
#274552,#274553,#274554,#274555,#274556,#274557,#274558,#274559,#274560,
#274561,#274562,#274563,#274564,#274565,#274566,#274567,#274568,#274569,
#274570,#274571,#274572,#274573,#274574,#274575,#274576,#274577,#274578,
#274579,#274580,#274581,#274582,#274583,#274584,#274585,#274586,#274587,
#274588,#274589,#274590,#274591,#274592,#274593,#274594,#274595,#274596,
#274597,#274598,#274599,#274600,#274601,#274602,#274603,#274604,#274605,
#274606,#274607,#274608,#274609,#274610,#274611,#274612,#274613,#274614,
#274615,#274616,#274617,#274618,#274619,#274620,#274621,#274622,#274623,
#274624,#274625,#274626,#274627,#274628,#274629,#274630,#274631,#274632,
#274633,#274634,#274635,#274636,#274637,#274638,#274639,#274640,#274641,
#274642,#274643,#274644,#274645,#274646,#274647,#274648,#274649,#274650,
#274651,#274652,#274653,#274654,#274655,#274656,#274657,#274658,#274659,
#274660,#274661,#274662,#274663,#274664,#274665,#274666,#274667,#274668,
#274669,#274670,#274671,#274672,#274673,#274674,#274675,#274676,#274677,
#274678,#274679,#274680,#274681,#274682,#274683,#274684,#274685,#274686,
#274687,#274688,#274689,#274690,#274691,#274692,#274693,#274694,#274695,
#274696,#274697,#274698,#274699,#274700,#274701,#274702,#274703,#274704,
#274705,#274706,#274707,#274708,#274709,#274710,#274711,#274712,#274713,
#274714,#274715,#274716,#274717,#274718,#274719,#274720,#274721,#274722,
#274723,#274724,#274725,#274726,#274727,#274728,#274729,#274730,#274731,
#274732,#274733,#274734,#274735,#274736,#274737,#274738,#274739,#274740,
#274741,#274742,#274743,#274744,#274745,#274746,#274747,#274748,#274749,
#274750,#274751,#274752,#274753,#274754,#274755,#274756,#274757,#274758,
#274759,#274760,#274761,#274762,#274763,#274764,#274765,#274766,#274767,
#274768,#274769,#274770,#274771,#274772,#274773,#274774,#274775,#274776,
#274777,#274778,#274779,#274780,#274781,#274782,#274783,#274784,#274785,
#274786,#274787,#274788,#274789,#274790,#274791,#274792,#274793,#274794,
#274795,#274796,#274797,#274798,#274799,#274800,#274801,#274802,#274803,
#274804,#274805,#274806,#274807,#274808,#274809,#274810,#274811,#274812,
#274813,#274814,#274815,#274816,#274817,#274818,#274819,#274820,#274821,
#274822,#274823,#274824,#274825,#274826,#274827,#274828,#274829,#274830,
#274831,#274832,#274833,#274834,#274835,#274836,#274837,#274838,#274839,
#274840,#274841,#274842,#274843,#274844,#274845,#274846,#274847,#274848,
#274849,#274850,#274851,#274852,#274853,#274854,#274855,#274856,#274857,
#274858,#274859,#274860,#274861,#274862,#274863,#274864,#274865,#274866,
#274867,#274868,#274869,#274870,#274871,#274872,#274873,#274874,#274875,
#274876,#274877,#274878,#274879,#274880,#274881,#274882,#274883,#274884,
#274885,#274886,#274887,#274888,#274889,#274890,#274891,#274892,#274893,
#274894,#274895,#274896,#274897,#274898,#274899,#274900,#274901,#274902,
#274903,#274904,#274905,#274906,#274907,#274908,#274909,#274910,#274911,
#274912,#274913,#274914,#274915,#274916,#274917,#274918,#274919,#274920,
#274921,#274922,#274923,#274924,#274925,#274926,#274927,#274928,#274929,
#274930,#274931,#274932,#274933,#274934,#274935,#274936,#274937,#274938,
#274939,#274940,#274941,#274942,#274943,#274944,#274945,#274946,#274947,
#274948,#274949,#274950,#274951,#274952,#274953,#274954,#274955,#274956,
#274957,#274958,#274959,#274960,#274961,#274962,#274963,#274964,#274965,
#274966,#274967,#274968,#274969,#274970,#274971,#274972,#274973,#274974,
#274975,#274976,#274977,#274978,#274979,#274980,#274981,#274982,#274983,
#274984,#274985,#274986,#274987,#274988,#274989,#274990,#274991,#274992,
#274993,#274994,#274995,#274996,#274997,#274998,#274999,#275000,#275001,
#275002,#275003,#275004,#275005,#275006,#275007,#275008,#275009,#275010,
#275011,#275012,#275013,#275014,#275015,#275016,#275017,#275018,#275019,
#275020,#275021,#275022,#275023,#275024,#275025,#275026,#275027,#275028,
#275029,#275030,#275031,#275032,#275033,#275034,#275035,#275036,#275037,
#275038,#275039,#275040,#275041,#275042,#275043,#275044,#275045,#275046,
#275047,#275048,#275049,#275050,#275051,#275052,#275053,#275054,#275055,
#275056,#275057,#275058,#275059,#275060,#275061,#275062,#275063,#275064,
#275065,#275066,#275067,#275068,#275069,#275070,#275071,#275072,#275073,
#275074,#275075,#275076,#275077,#275078,#275079,#275080,#275081,#275082,
#275083,#275084,#275085,#275086,#275087,#275088,#275089,#275090,#275091,
#275092,#275093,#275094,#275095,#275096,#275097,#275098,#275099,#275100,
#275101,#275102,#275103,#275104,#275105,#275106,#275107,#275108,#275109,
#275110,#275111,#275112,#275113,#275114,#275115,#275116,#275117,#275118,
#275119,#275120,#275121,#275122,#275123,#275124,#275125,#275126,#275127,
#275128,#275129,#275130,#275131,#275132,#275133,#275134,#275135,#275136,
#275137,#275138,#275139,#275140,#275141,#275142,#275143,#275144,#275145,
#275146,#275147,#275148,#275149,#275150,#275151,#275152,#275153,#275154,
#275155,#275156,#275157,#275158,#275159,#275160,#275161,#275162,#275163,
#275164,#275165,#275166,#275167,#275168,#275169,#275170,#275171,#275172,
#275173,#275174,#275175,#275176,#275177,#275178,#275179,#275180,#275181,
#275182,#275183,#275184,#275185,#275186,#275187,#275188,#275189,#275190,
#275191,#275192,#275193,#275194,#275195,#275196,#275197,#275198,#275199,
#275200,#275201,#275202,#275203,#275204,#275205,#275206,#275207,#275208,
#275209,#275210,#275211,#275212,#275213,#275214,#275215,#275216,#275217,
#275218,#275219,#275220,#275221,#275222,#275223,#275224,#275225,#275226,
#275227,#275228,#275229,#275230,#275231,#275232,#275233,#275234,#275235,
#275236,#275237,#275238,#275239,#275240,#275241,#275242,#275243,#275244,
#275245,#275246,#275247,#275248,#275249,#275250,#275251,#275252,#275253,
#275254,#275255,#275256,#275257,#275258,#275259,#275260,#275261,#275262,
#275263,#275264,#275265,#275266,#275267,#275268,#275269,#275270,#275271,
#275272,#275273,#275274,#275275,#275276,#275277,#275278,#275279,#275280,
#275281,#275282,#275283,#275284,#275285,#275286,#275287,#275288,#275289,
#275290,#275291,#275292,#275293,#275294,#275295,#275296,#275297,#275298,
#275299,#275300,#275301,#275302,#275303,#275304,#275305,#275306,#275307,
#275308,#275309,#275310,#275311,#275312,#275313,#275314,#275315,#275316,
#275317,#275318,#275319,#275320,#275321,#275322,#275323,#275324,#275325,
#275326,#275327,#275328,#275329,#275330,#275331,#275332,#275333,#275334,
#275335,#275336,#275337,#275338,#275339,#275340,#275341,#275342,#275343,
#275344,#275345,#275346,#275347,#275348,#275349,#275350,#275351,#275352,
#275353,#275354,#275355,#275356,#275357,#275358,#275359,#275360,#275361,
#275362,#275363,#275364,#275365,#275366,#275367,#275368,#275369,#275370,
#275371,#275372,#275373,#275374,#275375,#275376,#275377,#275378,#275379,
#275380,#275381,#275382,#275383,#275384,#275385,#275386,#275387,#275388,
#275389,#275390,#275391,#275392,#275393,#275394,#275395,#275396,#275397,
#275398,#275399,#275400,#275401,#275402,#275403,#275404,#275405,#275406,
#275407,#275408,#275409,#275410,#275411,#275412,#275413,#275414,#275415,
#275416,#275417,#275418,#275419,#275420,#275421,#275422,#275423,#275424,
#275425,#275426,#275427,#275428,#275429,#275430,#275431,#275432,#275433,
#275434,#275435,#275436,#275437,#275438,#275439,#275440,#275441,#275442,
#275443,#275444,#275445,#275446,#275447,#275448,#275449,#275450,#275451,
#275452,#275453,#275454,#275455,#275456,#275457,#275458,#275459,#275460,
#275461,#275462,#275463,#275464,#275465,#275466,#275467,#275468,#275469,
#275470,#275471,#275472,#275473,#275474,#275475,#275476,#275477,#275478,
#275479,#275480,#275481,#275482,#275483,#275484,#275485,#275486,#275487,
#275488,#275489,#275490,#275491,#275492,#275493,#275494,#275495,#275496,
#275497,#275498,#275499,#275500,#275501,#275502,#275503,#275504,#275505,
#275506,#275507,#275508,#275509,#275510,#275511,#275512,#275513,#275514,
#275515,#275516,#275517,#275518,#275519,#275520,#275521,#275522,#275523,
#275524,#275525,#275526,#275527,#275528,#275529,#275530,#275531,#275532,
#275533,#275534,#275535,#275536,#275537,#275538,#275539,#275540,#275541,
#275542,#275543,#275544,#275545,#275546,#275547,#275548,#275549,#275550,
#275551,#275552,#275553,#275554,#275555,#275556,#275557,#275558,#275559,
#275560,#275561,#275562,#275563,#275564,#275565,#275566,#275567,#275568,
#275569,#275570,#275571,#275572,#275573,#275574,#275575,#275576,#275577,
#275578,#275579,#275580,#275581,#275582,#275583,#275584,#275585,#275586,
#275587,#275588,#275589,#275590,#275591,#275592,#275593,#275594,#275595,
#275596,#275597,#275598,#275599,#275600,#275601,#275602,#275603,#275604,
#275605,#275606,#275607,#275608,#275609,#275610,#275611,#275612,#275613,
#275614,#275615,#275616,#275617,#275618,#275619,#275620,#275621,#275622,
#275623,#275624,#275625,#275626,#275627,#275628,#275629,#275630,#275631,
#275632,#275633,#275634,#275635,#275636,#275637,#275638,#275639,#275640,
#275641,#275642,#275643,#275644,#275645,#275646,#275647,#275648,#275649,
#275650,#275651,#275652,#275653,#275654,#275655,#275656,#275657,#275658,
#275659,#275660,#275661,#275662,#275663,#275664,#275665,#275666,#275667,
#275668,#275669,#275670,#275671,#275672,#275673,#275674,#275675,#275676,
#275677,#275678,#275679,#275680,#275681,#275682,#275683,#275684,#275685,
#275686,#275687,#275688,#275689,#275690,#275691,#275692,#275693,#275694,
#275695,#275696,#275697,#275698,#275699,#275700,#275701,#275702,#275703,
#275704,#275705,#275706,#275707,#275708,#275709,#275710,#275711,#275712,
#275713,#275714,#275715,#275716,#275717,#275718,#275719,#275720,#275721,
#275722,#275723,#275724,#275725,#275726,#275727,#275728,#275729,#275730,
#275731,#275732,#275733,#275734,#275735,#275736,#275737,#275738,#275739,
#275740,#275741),(#275742,#275743,#275744,#275745,#275746,#275747,#275748,
#275749,#275750,#275751,#275752,#275753,#275754,#275755,#275756,#275757,
#275758,#275759,#275760,#275761,#275762,#275763,#275764,#275765,#275766,
#275767,#275768,#275769,#275770,#275771,#275772,#275773,#275774,#275775,
#275776,#275777,#275778,#275779,#275780,#275781,#275782,#275783,#275784,
#275785,#275786,#275787,#275788,#275789,#275790,#275791,#275792,#275793,
#275794,#275795,#275796,#275797,#275798,#275799,#275800,#275801,#275802,
#275803,#275804,#275805,#275806,#275807,#275808,#275809,#275810,#275811,
#275812,#275813,#275814,#275815,#275816,#275817,#275818,#275819,#275820,
#275821,#275822,#275823,#275824,#275825,#275826,#275827,#275828,#275829,
#275830,#275831,#275832,#275833,#275834,#275835,#275836,#275837,#275838,
#275839,#275840,#275841,#275842,#275843,#275844,#275845,#275846,#275847,
#275848,#275849,#275850,#275851,#275852,#275853,#275854,#275855,#275856,
#275857,#275858,#275859,#275860,#275861,#275862,#275863,#275864,#275865,
#275866,#275867,#275868,#275869,#275870,#275871,#275872,#275873,#275874,
#275875,#275876,#275877,#275878,#275879,#275880,#275881,#275882,#275883,
#275884,#275885,#275886,#275887,#275888,#275889,#275890,#275891,#275892,
#275893,#275894,#275895,#275896,#275897,#275898,#275899,#275900,#275901,
#275902,#275903,#275904,#275905,#275906,#275907,#275908,#275909,#275910,
#275911,#275912,#275913,#275914,#275915,#275916,#275917,#275918,#275919,
#275920,#275921,#275922,#275923,#275924,#275925,#275926,#275927,#275928,
#275929,#275930,#275931,#275932,#275933,#275934,#275935,#275936,#275937,
#275938,#275939,#275940,#275941,#275942,#275943,#275944,#275945,#275946,
#275947,#275948,#275949,#275950,#275951,#275952,#275953,#275954,#275955,
#275956,#275957,#275958,#275959,#275960,#275961,#275962,#275963,#275964,
#275965,#275966,#275967,#275968,#275969,#275970,#275971,#275972,#275973,
#275974,#275975,#275976,#275977,#275978,#275979,#275980,#275981,#275982,
#275983,#275984,#275985,#275986,#275987,#275988,#275989,#275990,#275991,
#275992,#275993,#275994,#275995,#275996,#275997,#275998,#275999,#276000,
#276001,#276002,#276003,#276004,#276005,#276006,#276007,#276008,#276009,
#276010,#276011,#276012,#276013,#276014,#276015,#276016,#276017,#276018,
#276019,#276020,#276021,#276022,#276023,#276024,#276025,#276026,#276027,
#276028,#276029,#276030,#276031,#276032,#276033,#276034,#276035,#276036,
#276037,#276038,#276039,#276040,#276041,#276042,#276043,#276044,#276045,
#276046,#276047,#276048,#276049,#276050,#276051,#276052,#276053,#276054,
#276055,#276056,#276057,#276058,#276059,#276060,#276061,#276062,#276063,
#276064,#276065,#276066,#276067,#276068,#276069,#276070,#276071,#276072,
#276073,#276074,#276075,#276076,#276077,#276078,#276079,#276080,#276081,
#276082,#276083,#276084,#276085,#276086,#276087,#276088,#276089,#276090,
#276091,#276092,#276093,#276094,#276095,#276096,#276097,#276098,#276099,
#276100,#276101,#276102,#276103,#276104,#276105,#276106,#276107,#276108,
#276109,#276110,#276111,#276112,#276113,#276114,#276115,#276116,#276117,
#276118,#276119,#276120,#276121,#276122,#276123,#276124,#276125,#276126,
#276127,#276128,#276129,#276130,#276131,#276132,#276133,#276134,#276135,
#276136,#276137,#276138,#276139,#276140,#276141,#276142,#276143,#276144,
#276145,#276146,#276147,#276148,#276149,#276150,#276151,#276152,#276153,
#276154,#276155,#276156,#276157,#276158,#276159,#276160,#276161,#276162,
#276163,#276164,#276165,#276166,#276167,#276168,#276169,#276170,#276171,
#276172,#276173,#276174,#276175,#276176,#276177,#276178,#276179,#276180,
#276181,#276182,#276183,#276184,#276185,#276186,#276187,#276188,#276189,
#276190,#276191,#276192,#276193,#276194,#276195,#276196,#276197,#276198,
#276199,#276200,#276201,#276202,#276203,#276204,#276205,#276206,#276207,
#276208,#276209,#276210,#276211,#276212,#276213,#276214,#276215,#276216,
#276217,#276218,#276219,#276220,#276221,#276222,#276223,#276224,#276225,
#276226,#276227,#276228,#276229,#276230,#276231,#276232,#276233,#276234,
#276235,#276236,#276237,#276238,#276239,#276240,#276241,#276242,#276243,
#276244,#276245,#276246,#276247,#276248,#276249,#276250,#276251,#276252,
#276253,#276254,#276255,#276256,#276257,#276258,#276259,#276260,#276261,
#276262,#276263,#276264,#276265,#276266,#276267,#276268,#276269,#276270,
#276271,#276272,#276273,#276274,#276275,#276276,#276277,#276278,#276279,
#276280,#276281,#276282,#276283,#276284,#276285,#276286,#276287,#276288,
#276289,#276290,#276291,#276292,#276293,#276294,#276295,#276296,#276297,
#276298,#276299,#276300,#276301,#276302,#276303,#276304,#276305,#276306,
#276307,#276308,#276309,#276310,#276311,#276312,#276313,#276314,#276315,
#276316,#276317,#276318,#276319,#276320,#276321,#276322,#276323,#276324,
#276325,#276326,#276327,#276328,#276329,#276330,#276331,#276332,#276333,
#276334,#276335,#276336,#276337,#276338,#276339,#276340,#276341,#276342,
#276343,#276344,#276345,#276346,#276347,#276348,#276349,#276350,#276351,
#276352,#276353,#276354,#276355,#276356,#276357,#276358,#276359,#276360,
#276361,#276362,#276363,#276364,#276365,#276366,#276367,#276368,#276369,
#276370,#276371,#276372,#276373,#276374,#276375,#276376,#276377,#276378,
#276379,#276380,#276381,#276382,#276383,#276384,#276385,#276386,#276387,
#276388,#276389,#276390,#276391,#276392,#276393,#276394,#276395,#276396,
#276397,#276398,#276399,#276400,#276401,#276402,#276403,#276404,#276405,
#276406,#276407,#276408,#276409,#276410,#276411,#276412,#276413,#276414,
#276415,#276416,#276417,#276418,#276419,#276420,#276421,#276422,#276423,
#276424,#276425,#276426,#276427,#276428,#276429,#276430,#276431,#276432,
#276433,#276434,#276435,#276436,#276437,#276438,#276439,#276440,#276441,
#276442,#276443,#276444,#276445,#276446,#276447,#276448,#276449,#276450,
#276451,#276452,#276453,#276454,#276455,#276456,#276457,#276458,#276459,
#276460,#276461,#276462,#276463,#276464,#276465,#276466,#276467,#276468,
#276469,#276470,#276471,#276472,#276473,#276474,#276475,#276476,#276477,
#276478,#276479,#276480,#276481,#276482,#276483,#276484,#276485,#276486,
#276487,#276488,#276489,#276490,#276491,#276492,#276493,#276494,#276495,
#276496,#276497,#276498,#276499,#276500,#276501,#276502,#276503,#276504,
#276505,#276506,#276507,#276508,#276509,#276510,#276511,#276512,#276513,
#276514,#276515,#276516,#276517,#276518,#276519,#276520,#276521,#276522,
#276523,#276524,#276525,#276526,#276527,#276528,#276529,#276530,#276531,
#276532,#276533,#276534,#276535,#276536,#276537,#276538,#276539,#276540,
#276541,#276542,#276543,#276544,#276545,#276546,#276547,#276548,#276549,
#276550,#276551,#276552,#276553,#276554,#276555,#276556,#276557,#276558,
#276559,#276560,#276561,#276562,#276563,#276564,#276565,#276566,#276567,
#276568,#276569,#276570,#276571,#276572,#276573,#276574,#276575,#276576,
#276577,#276578,#276579,#276580,#276581,#276582,#276583,#276584,#276585,
#276586,#276587,#276588,#276589,#276590,#276591,#276592,#276593,#276594,
#276595,#276596,#276597,#276598,#276599,#276600,#276601,#276602,#276603,
#276604,#276605,#276606,#276607,#276608,#276609,#276610,#276611,#276612,
#276613,#276614,#276615,#276616,#276617,#276618,#276619,#276620,#276621,
#276622,#276623,#276624,#276625,#276626,#276627,#276628,#276629,#276630,
#276631,#276632,#276633,#276634,#276635,#276636,#276637,#276638,#276639,
#276640,#276641,#276642,#276643,#276644,#276645,#276646,#276647,#276648,
#276649,#276650,#276651,#276652,#276653,#276654,#276655,#276656,#276657,
#276658,#276659,#276660,#276661,#276662,#276663,#276664,#276665,#276666,
#276667,#276668,#276669,#276670,#276671,#276672,#276673,#276674,#276675,
#276676,#276677,#276678,#276679,#276680,#276681,#276682,#276683,#276684,
#276685,#276686,#276687,#276688,#276689,#276690,#276691,#276692,#276693,
#276694,#276695,#276696,#276697,#276698,#276699,#276700,#276701,#276702,
#276703,#276704,#276705,#276706,#276707,#276708,#276709,#276710,#276711,
#276712,#276713,#276714,#276715,#276716,#276717,#276718,#276719,#276720,
#276721,#276722,#276723,#276724,#276725,#276726,#276727,#276728,#276729,
#276730,#276731,#276732,#276733,#276734,#276735,#276736,#276737,#276738,
#276739,#276740,#276741,#276742,#276743,#276744,#276745,#276746,#276747,
#276748,#276749,#276750,#276751,#276752,#276753,#276754,#276755,#276756,
#276757,#276758,#276759,#276760,#276761,#276762,#276763,#276764,#276765,
#276766,#276767,#276768,#276769,#276770,#276771,#276772,#276773,#276774,
#276775,#276776,#276777,#276778,#276779,#276780,#276781,#276782,#276783,
#276784,#276785,#276786,#276787,#276788,#276789,#276790,#276791,#276792,
#276793,#276794,#276795,#276796,#276797,#276798,#276799,#276800,#276801,
#276802,#276803,#276804,#276805,#276806,#276807,#276808,#276809,#276810,
#276811,#276812,#276813,#276814,#276815,#276816,#276817,#276818,#276819,
#276820,#276821,#276822,#276823,#276824,#276825,#276826,#276827,#276828,
#276829,#276830,#276831,#276832,#276833,#276834,#276835,#276836,#276837,
#276838,#276839,#276840,#276841,#276842,#276843,#276844,#276845,#276846,
#276847,#276848,#276849,#276850,#276851,#276852,#276853,#276854,#276855,
#276856,#276857,#276858,#276859,#276860,#276861,#276862,#276863,#276864,
#276865,#276866,#276867,#276868,#276869,#276870,#276871,#276872,#276873,
#276874,#276875,#276876,#276877,#276878,#276879,#276880,#276881,#276882,
#276883,#276884,#276885,#276886,#276887,#276888,#276889,#276890,#276891,
#276892,#276893,#276894,#276895,#276896,#276897,#276898,#276899,#276900,
#276901,#276902,#276903,#276904,#276905,#276906,#276907,#276908,#276909,
#276910,#276911,#276912,#276913,#276914,#276915,#276916,#276917,#276918,
#276919,#276920,#276921,#276922,#276923,#276924,#276925,#276926,#276927,
#276928,#276929,#276930,#276931,#276932,#276933,#276934,#276935,#276936,
#276937,#276938,#276939,#276940,#276941,#276942,#276943,#276944,#276945,
#276946,#276947,#276948,#276949,#276950,#276951,#276952,#276953,#276954,
#276955,#276956,#276957,#276958,#276959,#276960,#276961,#276962,#276963,
#276964,#276965,#276966,#276967,#276968,#276969,#276970,#276971,#276972,
#276973,#276974,#276975,#276976,#276977,#276978,#276979,#276980,#276981,
#276982,#276983,#276984,#276985,#276986,#276987,#276988,#276989,#276990,
#276991,#276992,#276993,#276994,#276995,#276996,#276997,#276998,#276999,
#277000,#277001,#277002,#277003,#277004,#277005,#277006,#277007,#277008,
#277009,#277010,#277011,#277012,#277013,#277014,#277015,#277016,#277017,
#277018,#277019,#277020,#277021,#277022,#277023,#277024,#277025,#277026,
#277027,#277028,#277029,#277030,#277031,#277032,#277033,#277034,#277035,
#277036,#277037,#277038,#277039,#277040,#277041,#277042,#277043,#277044,
#277045,#277046,#277047,#277048,#277049,#277050,#277051,#277052,#277053,
#277054,#277055,#277056,#277057,#277058,#277059,#277060,#277061,#277062,
#277063,#277064,#277065,#277066,#277067,#277068,#277069,#277070,#277071,
#277072,#277073,#277074,#277075,#277076,#277077,#277078,#277079,#277080,
#277081,#277082,#277083,#277084,#277085,#277086,#277087,#277088,#277089,
#277090,#277091,#277092,#277093,#277094,#277095,#277096,#277097,#277098,
#277099,#277100,#277101,#277102,#277103,#277104,#277105,#277106,#277107,
#277108,#277109,#277110,#277111,#277112,#277113,#277114,#277115,#277116,
#277117,#277118,#277119,#277120,#277121,#277122,#277123,#277124,#277125,
#277126,#277127,#277128,#277129,#277130,#277131,#277132,#277133,#277134,
#277135,#277136,#277137,#277138,#277139,#277140,#277141,#277142,#277143,
#277144,#277145,#277146,#277147,#277148,#277149,#277150,#277151,#277152,
#277153,#277154,#277155,#277156,#277157,#277158,#277159,#277160,#277161,
#277162,#277163,#277164,#277165,#277166,#277167,#277168,#277169,#277170,
#277171,#277172,#277173,#277174,#277175,#277176,#277177,#277178,#277179,
#277180,#277181,#277182,#277183,#277184,#277185,#277186,#277187,#277188,
#277189,#277190,#277191,#277192,#277193,#277194,#277195,#277196,#277197,
#277198,#277199,#277200,#277201,#277202,#277203,#277204,#277205,#277206,
#277207,#277208,#277209,#277210,#277211,#277212,#277213,#277214,#277215,
#277216,#277217,#277218,#277219,#277220,#277221,#277222,#277223,#277224,
#277225,#277226,#277227,#277228,#277229,#277230,#277231,#277232,#277233,
#277234,#277235,#277236,#277237,#277238,#277239,#277240,#277241,#277242,
#277243,#277244,#277245,#277246,#277247,#277248,#277249,#277250,#277251,
#277252,#277253,#277254,#277255,#277256,#277257,#277258,#277259,#277260,
#277261,#277262,#277263,#277264,#277265,#277266,#277267,#277268,#277269,
#277270,#277271,#277272,#277273,#277274,#277275,#277276,#277277,#277278,
#277279,#277280,#277281,#277282,#277283,#277284,#277285,#277286,#277287,
#277288,#277289,#277290,#277291,#277292,#277293,#277294,#277295,#277296,
#277297,#277298,#277299,#277300,#277301,#277302,#277303,#277304,#277305,
#277306,#277307,#277308,#277309,#277310,#277311,#277312,#277313,#277314,
#277315,#277316,#277317,#277318,#277319,#277320,#277321,#277322,#277323,
#277324,#277325,#277326,#277327,#277328,#277329,#277330,#277331,#277332,
#277333,#277334,#277335,#277336,#277337,#277338,#277339,#277340,#277341,
#277342,#277343,#277344,#277345,#277346,#277347,#277348,#277349,#277350,
#277351,#277352,#277353,#277354,#277355,#277356,#277357,#277358,#277359,
#277360,#277361,#277362,#277363,#277364,#277365,#277366,#277367,#277368,
#277369,#277370,#277371,#277372,#277373,#277374,#277375,#277376,#277377,
#277378,#277379,#277380,#277381,#277382,#277383,#277384,#277385,#277386,
#277387,#277388,#277389,#277390,#277391,#277392,#277393,#277394,#277395,
#277396,#277397,#277398,#277399,#277400,#277401,#277402,#277403,#277404,
#277405,#277406,#277407,#277408,#277409,#277410,#277411,#277412,#277413,
#277414,#277415,#277416,#277417,#277418,#277419,#277420,#277421,#277422,
#277423,#277424,#277425,#277426,#277427,#277428,#277429,#277430,#277431,
#277432,#277433,#277434,#277435,#277436),(#277437,#277438,#277439,#277440,
#277441,#277442,#277443,#277444,#277445,#277446,#277447,#277448,#277449,
#277450,#277451,#277452,#277453,#277454,#277455,#277456,#277457,#277458,
#277459,#277460,#277461,#277462,#277463,#277464,#277465,#277466,#277467,
#277468,#277469,#277470,#277471,#277472,#277473,#277474,#277475,#277476,
#277477,#277478,#277479,#277480,#277481,#277482,#277483,#277484,#277485,
#277486,#277487,#277488,#277489,#277490,#277491,#277492,#277493,#277494,
#277495,#277496,#277497,#277498,#277499,#277500,#277501,#277502,#277503,
#277504,#277505,#277506,#277507,#277508,#277509,#277510,#277511,#277512,
#277513,#277514,#277515,#277516,#277517,#277518,#277519,#277520,#277521,
#277522,#277523,#277524,#277525,#277526,#277527,#277528,#277529,#277530,
#277531,#277532,#277533,#277534,#277535,#277536,#277537,#277538,#277539,
#277540,#277541,#277542,#277543,#277544,#277545,#277546,#277547,#277548,
#277549,#277550,#277551,#277552,#277553,#277554,#277555,#277556,#277557,
#277558,#277559,#277560,#277561,#277562,#277563,#277564,#277565,#277566,
#277567,#277568,#277569,#277570,#277571,#277572,#277573,#277574,#277575,
#277576,#277577,#277578,#277579,#277580,#277581,#277582,#277583,#277584,
#277585,#277586,#277587,#277588,#277589,#277590,#277591,#277592,#277593,
#277594,#277595,#277596,#277597,#277598,#277599,#277600,#277601,#277602,
#277603,#277604,#277605,#277606,#277607,#277608,#277609,#277610,#277611,
#277612,#277613,#277614,#277615,#277616,#277617,#277618,#277619,#277620,
#277621,#277622,#277623,#277624,#277625,#277626,#277627,#277628,#277629,
#277630,#277631,#277632,#277633,#277634,#277635,#277636,#277637,#277638,
#277639,#277640,#277641,#277642,#277643,#277644,#277645,#277646,#277647,
#277648,#277649,#277650,#277651,#277652,#277653,#277654,#277655,#277656,
#277657,#277658,#277659,#277660,#277661,#277662,#277663,#277664,#277665,
#277666,#277667,#277668,#277669,#277670,#277671,#277672,#277673,#277674,
#277675,#277676,#277677,#277678,#277679,#277680,#277681,#277682,#277683,
#277684,#277685,#277686,#277687,#277688,#277689,#277690,#277691,#277692,
#277693,#277694,#277695,#277696,#277697,#277698,#277699,#277700,#277701,
#277702,#277703,#277704,#277705,#277706,#277707,#277708,#277709,#277710,
#277711,#277712,#277713,#277714,#277715,#277716,#277717,#277718,#277719,
#277720,#277721,#277722,#277723,#277724,#277725,#277726,#277727,#277728,
#277729,#277730,#277731,#277732,#277733,#277734,#277735,#277736,#277737,
#277738,#277739,#277740,#277741,#277742,#277743,#277744,#277745,#277746,
#277747,#277748,#277749,#277750,#277751,#277752,#277753,#277754,#277755,
#277756,#277757,#277758,#277759,#277760,#277761,#277762,#277763,#277764,
#277765,#277766,#277767,#277768,#277769,#277770,#277771,#277772,#277773,
#277774,#277775,#277776,#277777,#277778,#277779,#277780,#277781,#277782,
#277783,#277784,#277785,#277786,#277787,#277788,#277789,#277790,#277791,
#277792,#277793,#277794,#277795,#277796,#277797,#277798,#277799,#277800,
#277801,#277802,#277803,#277804,#277805,#277806,#277807,#277808,#277809,
#277810,#277811,#277812,#277813,#277814,#277815,#277816,#277817,#277818,
#277819,#277820,#277821,#277822,#277823,#277824,#277825,#277826,#277827,
#277828,#277829,#277830,#277831,#277832,#277833,#277834,#277835,#277836,
#277837,#277838,#277839,#277840,#277841,#277842,#277843,#277844,#277845,
#277846,#277847,#277848,#277849,#277850,#277851,#277852,#277853,#277854,
#277855,#277856,#277857,#277858,#277859,#277860,#277861,#277862,#277863,
#277864,#277865,#277866,#277867,#277868,#277869,#277870,#277871,#277872,
#277873,#277874,#277875,#277876,#277877,#277878,#277879,#277880,#277881,
#277882,#277883,#277884,#277885,#277886,#277887,#277888,#277889,#277890,
#277891,#277892,#277893,#277894,#277895,#277896,#277897,#277898,#277899,
#277900,#277901,#277902,#277903,#277904,#277905,#277906,#277907,#277908,
#277909,#277910,#277911,#277912,#277913,#277914,#277915,#277916,#277917,
#277918,#277919,#277920,#277921,#277922,#277923,#277924,#277925,#277926,
#277927,#277928,#277929,#277930,#277931,#277932,#277933,#277934,#277935,
#277936,#277937,#277938,#277939,#277940,#277941,#277942,#277943,#277944,
#277945,#277946,#277947,#277948,#277949,#277950,#277951,#277952,#277953,
#277954,#277955,#277956,#277957,#277958,#277959,#277960,#277961,#277962,
#277963,#277964,#277965,#277966,#277967,#277968,#277969,#277970,#277971,
#277972,#277973,#277974,#277975,#277976,#277977,#277978,#277979,#277980,
#277981,#277982,#277983,#277984,#277985,#277986,#277987,#277988,#277989,
#277990,#277991,#277992,#277993,#277994,#277995,#277996,#277997,#277998,
#277999,#278000,#278001,#278002,#278003,#278004,#278005,#278006,#278007,
#278008,#278009,#278010,#278011,#278012,#278013,#278014,#278015,#278016,
#278017,#278018,#278019,#278020,#278021,#278022,#278023,#278024,#278025,
#278026,#278027,#278028,#278029,#278030,#278031,#278032,#278033,#278034,
#278035,#278036,#278037,#278038,#278039,#278040,#278041,#278042,#278043,
#278044,#278045,#278046,#278047,#278048,#278049,#278050,#278051,#278052,
#278053,#278054,#278055,#278056,#278057,#278058,#278059,#278060,#278061,
#278062,#278063,#278064,#278065,#278066,#278067,#278068,#278069,#278070,
#278071,#278072,#278073,#278074,#278075,#278076,#278077,#278078,#278079,
#278080,#278081,#278082,#278083,#278084,#278085,#278086,#278087,#278088,
#278089,#278090,#278091,#278092,#278093,#278094,#278095,#278096,#278097,
#278098,#278099,#278100,#278101,#278102,#278103,#278104,#278105,#278106,
#278107,#278108,#278109,#278110,#278111,#278112,#278113,#278114,#278115,
#278116,#278117,#278118,#278119,#278120,#278121,#278122,#278123,#278124,
#278125,#278126,#278127,#278128,#278129,#278130,#278131,#278132,#278133,
#278134,#278135,#278136,#278137,#278138,#278139,#278140,#278141,#278142,
#278143,#278144,#278145,#278146,#278147,#278148,#278149,#278150,#278151,
#278152,#278153,#278154,#278155,#278156,#278157,#278158,#278159,#278160,
#278161,#278162,#278163,#278164,#278165,#278166,#278167,#278168,#278169,
#278170,#278171,#278172,#278173,#278174,#278175,#278176,#278177,#278178,
#278179,#278180,#278181,#278182,#278183,#278184,#278185,#278186,#278187,
#278188,#278189,#278190,#278191,#278192,#278193,#278194,#278195,#278196,
#278197,#278198,#278199,#278200,#278201,#278202,#278203,#278204,#278205,
#278206,#278207,#278208,#278209,#278210,#278211,#278212,#278213,#278214,
#278215,#278216,#278217,#278218,#278219,#278220,#278221,#278222,#278223,
#278224,#278225,#278226,#278227,#278228,#278229,#278230,#278231,#278232,
#278233,#278234,#278235,#278236,#278237,#278238,#278239,#278240,#278241,
#278242,#278243,#278244,#278245,#278246,#278247,#278248,#278249,#278250,
#278251,#278252,#278253,#278254,#278255,#278256,#278257,#278258,#278259,
#278260,#278261,#278262,#278263,#278264,#278265,#278266,#278267,#278268,
#278269,#278270,#278271,#278272,#278273,#278274,#278275,#278276,#278277,
#278278,#278279,#278280,#278281,#278282,#278283,#278284,#278285,#278286,
#278287,#278288,#278289,#278290,#278291,#278292,#278293,#278294,#278295,
#278296,#278297,#278298,#278299,#278300,#278301,#278302,#278303,#278304,
#278305,#278306,#278307,#278308,#278309,#278310,#278311,#278312,#278313,
#278314,#278315,#278316,#278317,#278318,#278319,#278320,#278321,#278322,
#278323,#278324,#278325,#278326,#278327,#278328,#278329,#278330,#278331,
#278332,#278333,#278334,#278335,#278336,#278337,#278338,#278339,#278340,
#278341,#278342,#278343,#278344,#278345,#278346,#278347,#278348,#278349,
#278350,#278351,#278352,#278353,#278354,#278355,#278356,#278357,#278358,
#278359,#278360,#278361,#278362,#278363,#278364,#278365,#278366,#278367,
#278368,#278369,#278370,#278371,#278372,#278373,#278374,#278375,#278376,
#278377,#278378,#278379,#278380,#278381,#278382,#278383,#278384,#278385,
#278386,#278387,#278388,#278389,#278390,#278391,#278392,#278393,#278394,
#278395,#278396,#278397,#278398,#278399,#278400,#278401,#278402,#278403,
#278404,#278405,#278406,#278407,#278408,#278409,#278410,#278411,#278412,
#278413,#278414,#278415,#278416,#278417,#278418,#278419,#278420,#278421,
#278422,#278423,#278424,#278425,#278426,#278427,#278428,#278429,#278430,
#278431,#278432,#278433,#278434,#278435,#278436,#278437,#278438,#278439,
#278440,#278441,#278442,#278443,#278444,#278445,#278446,#278447,#278448,
#278449,#278450,#278451,#278452,#278453,#278454,#278455,#278456,#278457,
#278458,#278459,#278460,#278461,#278462,#278463,#278464,#278465,#278466,
#278467,#278468,#278469,#278470,#278471,#278472,#278473,#278474,#278475,
#278476,#278477,#278478,#278479,#278480,#278481,#278482,#278483,#278484,
#278485,#278486,#278487,#278488,#278489,#278490,#278491,#278492,#278493,
#278494,#278495,#278496,#278497,#278498,#278499,#278500,#278501,#278502,
#278503,#278504,#278505,#278506,#278507,#278508,#278509,#278510,#278511,
#278512,#278513,#278514,#278515,#278516,#278517,#278518,#278519,#278520,
#278521,#278522,#278523,#278524,#278525,#278526,#278527,#278528,#278529,
#278530,#278531,#278532,#278533,#278534,#278535,#278536,#278537,#278538,
#278539,#278540,#278541,#278542,#278543,#278544,#278545,#278546,#278547,
#278548,#278549,#278550,#278551,#278552,#278553,#278554,#278555,#278556,
#278557,#278558,#278559,#278560,#278561,#278562,#278563,#278564,#278565,
#278566,#278567,#278568,#278569,#278570,#278571,#278572,#278573,#278574,
#278575,#278576,#278577,#278578,#278579,#278580,#278581,#278582,#278583,
#278584,#278585,#278586,#278587,#278588,#278589,#278590,#278591,#278592,
#278593,#278594,#278595,#278596,#278597,#278598,#278599,#278600,#278601,
#278602,#278603,#278604,#278605,#278606,#278607,#278608,#278609,#278610,
#278611,#278612,#278613,#278614,#278615,#278616,#278617,#278618,#278619,
#278620,#278621,#278622,#278623,#278624,#278625,#278626,#278627,#278628,
#278629,#278630,#278631,#278632,#278633,#278634,#278635,#278636,#278637,
#278638,#278639,#278640,#278641,#278642,#278643,#278644,#278645,#278646,
#278647,#278648,#278649,#278650,#278651,#278652,#278653,#278654,#278655,
#278656,#278657,#278658,#278659,#278660,#278661,#278662,#278663,#278664,
#278665,#278666,#278667,#278668,#278669,#278670,#278671,#278672,#278673,
#278674,#278675,#278676,#278677,#278678,#278679,#278680,#278681,#278682,
#278683,#278684,#278685,#278686,#278687,#278688,#278689,#278690,#278691,
#278692,#278693,#278694,#278695,#278696,#278697,#278698,#278699,#278700,
#278701,#278702,#278703,#278704,#278705,#278706,#278707,#278708,#278709,
#278710,#278711,#278712,#278713,#278714,#278715,#278716,#278717,#278718,
#278719,#278720,#278721,#278722,#278723,#278724,#278725,#278726,#278727,
#278728,#278729,#278730,#278731,#278732,#278733,#278734,#278735,#278736,
#278737,#278738,#278739,#278740,#278741,#278742,#278743,#278744,#278745,
#278746,#278747,#278748,#278749,#278750,#278751,#278752,#278753,#278754,
#278755,#278756,#278757,#278758,#278759,#278760,#278761,#278762,#278763,
#278764,#278765,#278766,#278767,#278768,#278769,#278770,#278771,#278772,
#278773,#278774,#278775,#278776,#278777,#278778,#278779,#278780,#278781,
#278782,#278783,#278784,#278785,#278786,#278787,#278788,#278789,#278790,
#278791,#278792,#278793,#278794,#278795,#278796,#278797,#278798,#278799,
#278800,#278801,#278802,#278803,#278804,#278805,#278806,#278807,#278808,
#278809,#278810,#278811,#278812,#278813,#278814,#278815,#278816,#278817,
#278818,#278819,#278820,#278821,#278822,#278823,#278824,#278825,#278826,
#278827,#278828,#278829,#278830,#278831,#278832,#278833,#278834,#278835,
#278836,#278837,#278838,#278839,#278840,#278841,#278842,#278843,#278844,
#278845,#278846,#278847,#278848,#278849,#278850,#278851,#278852,#278853,
#278854,#278855,#278856,#278857,#278858,#278859,#278860,#278861,#278862,
#278863,#278864,#278865,#278866,#278867,#278868,#278869,#278870,#278871,
#278872,#278873,#278874,#278875,#278876,#278877,#278878,#278879,#278880,
#278881,#278882,#278883,#278884,#278885,#278886,#278887,#278888,#278889,
#278890,#278891,#278892,#278893,#278894,#278895,#278896,#278897,#278898,
#278899,#278900,#278901,#278902,#278903,#278904,#278905,#278906,#278907,
#278908,#278909,#278910,#278911,#278912,#278913,#278914,#278915,#278916,
#278917,#278918,#278919,#278920,#278921,#278922,#278923,#278924,#278925,
#278926,#278927,#278928,#278929,#278930,#278931,#278932,#278933,#278934,
#278935,#278936,#278937,#278938,#278939,#278940,#278941,#278942,#278943,
#278944,#278945,#278946,#278947,#278948,#278949,#278950,#278951,#278952,
#278953,#278954,#278955,#278956,#278957,#278958,#278959,#278960,#278961,
#278962,#278963,#278964,#278965,#278966,#278967,#278968,#278969,#278970,
#278971,#278972,#278973,#278974,#278975,#278976,#278977,#278978,#278979,
#278980,#278981,#278982,#278983,#278984,#278985,#278986,#278987,#278988,
#278989,#278990,#278991,#278992,#278993,#278994,#278995,#278996,#278997,
#278998,#278999,#279000,#279001,#279002,#279003,#279004,#279005,#279006,
#279007,#279008,#279009,#279010,#279011,#279012,#279013,#279014,#279015,
#279016,#279017,#279018,#279019,#279020,#279021,#279022,#279023,#279024,
#279025,#279026,#279027,#279028,#279029,#279030,#279031,#279032,#279033,
#279034,#279035,#279036,#279037,#279038,#279039,#279040,#279041,#279042,
#279043,#279044,#279045,#279046,#279047,#279048,#279049,#279050,#279051,
#279052,#279053,#279054,#279055,#279056,#279057,#279058,#279059,#279060,
#279061,#279062,#279063,#279064,#279065,#279066,#279067,#279068,#279069,
#279070,#279071,#279072,#279073,#279074,#279075,#279076,#279077,#279078,
#279079,#279080,#279081,#279082,#279083,#279084,#279085,#279086,#279087,
#279088,#279089,#279090,#279091,#279092,#279093,#279094,#279095,#279096,
#279097,#279098,#279099,#279100,#279101,#279102,#279103,#279104,#279105,
#279106,#279107,#279108,#279109,#279110,#279111,#279112,#279113,#279114,
#279115,#279116,#279117,#279118,#279119,#279120,#279121,#279122,#279123,
#279124,#279125,#279126,#279127,#279128,#279129,#279130,#279131)),
 .UNSPECIFIED.,.F.,.F.,.F.,(4,4),(4,1,1,1,1,1,1,1,1,1,1,1,1,1,1,1,1,1,1,
1,1,1,1,1,1,1,1,1,1,1,1,1,1,1,1,1,1,1,1,1,1,1,1,1,1,1,1,1,1,1,1,1,1,1,1,
1,1,1,1,1,1,1,1,1,1,1,1,1,1,1,1,1,1,1,1,1,1,1,1,1,1,1,1,1,1,1,1,1,1,1,1,
1,1,1,1,1,1,1,1,1,1,1,1,1,1,1,1,1,1,1,1,1,1,1,1,1,1,1,1,1,1,1,1,1,1,1,1,
1,1,1,1,1,1,1,1,1,1,1,1,1,1,1,1,1,1,1,1,1,1,1,1,1,1,1,1,1,1,1,1,1,1,1,1,
1,1,1,1,1,1,1,1,1,1,1,1,1,1,1,1,1,1,1,1,1,1,1,1,1,1,1,1,1,1,1,1,1,1,1,1,
1,1,1,1,1,1,1,1,1,1,1,1,1,1,1,1,1,1,1,1,1,1,1,1,1,1,1,1,1,1,1,1,1,1,1,1,
1,1,1,1,1,1,1,1,1,1,1,1,1,1,1,1,1,1,1,1,1,1,1,1,1,1,1,1,1,1,1,1,1,1,1,1,
1,1,1,1,1,1,1,1,1,1,1,1,1,1,1,1,1,1,1,1,1,1,1,1,1,1,1,1,1,1,1,1,1,1,1,1,
1,1,1,1,1,1,1,1,1,1,1,1,1,1,1,1,1,1,1,1,1,1,1,1,1,1,1,1,1,1,1,1,1,1,1,1,
1,1,1,1,1,1,1,1,1,1,1,1,1,1,1,1,1,1,1,1,1,1,1,1,1,1,1,1,1,1,1,1,1,1,1,1,
1,1,1,1,1,1,1,1,1,1,1,1,1,1,1,1,1,1,1,1,1,1,1,1,1,1,1,1,1,1,1,1,1,1,1,1,
1,1,1,1,1,1,1,1,1,1,1,1,1,1,1,1,1,1,1,1,1,1,1,1,1,1,1,1,1,1,1,1,1,1,1,1,
1,1,1,1,1,1,1,1,1,1,1,1,1,1,1,1,1,1,1,1,1,1,1,1,1,1,1,1,1,1,1,1,1,1,1,1,
1,1,1,1,1,1,1,1,1,1,1,1,1,1,1,1,1,1,1,1,1,1,1,1,1,1,1,1,1,1,1,1,1,1,1,1,
1,1,1,1,1,1,1,1,1,1,1,1,1,1,1,1,1,1,1,1,1,1,1,1,1,1,1,1,1,1,1,1,1,1,1,1,
1,1,1,1,1,1,1,1,1,1,1,1,1,1,1,1,1,1,1,1,1,1,1,1,1,1,1,1,1,1,1,1,1,1,1,1,
1,1,1,1,1,1,1,1,1,1,1,1,1,1,1,1,1,1,1,1,1,1,1,1,1,1,1,1,1,1,1,1,1,1,1,1,
1,1,1,1,1,1,1,1,1,1,1,1,1,1,1,1,1,1,1,1,1,1,1,1,1,1,1,1,1,1,1,1,1,1,1,1,
1,1,1,1,1,1,1,1,1,1,1,1,1,1,1,1,1,1,1,1,1,1,1,1,1,1,1,1,1,1,1,1,1,1,1,1,
1,1,1,1,1,1,1,1,1,1,1,1,1,1,1,1,1,1,1,1,1,1,1,1,1,1,1,1,1,1,1,1,1,1,1,1,
1,1,1,1,1,1,1,1,1,1,1,1,1,1,1,1,1,1,1,1,1,1,1,1,1,1,1,1,1,1,1,1,1,1,1,1,
1,1,1,1,1,1,1,1,1,1,1,1,1,1,1,1,1,1,1,1,1,1,1,1,1,1,1,1,1,1,1,1,1,1,1,1,
1,1,1,1,1,1,1,1,1,1,1,1,1,1,1,1,1,1,1,1,1,1,1,1,1,1,1,1,1,1,1,1,1,1,1,1,
1,1,1,1,1,1,1,1,1,1,1,1,1,1,1,1,1,1,1,1,1,1,1,1,1,1,1,1,1,1,1,1,1,1,1,1,
1,1,1,1,1,1,1,1,1,1,1,1,1,1,1,1,1,1,1,1,1,1,1,1,1,1,1,1,1,1,1,1,1,1,1,1,
1,1,1,1,1,1,1,1,1,1,1,1,1,1,1,1,1,1,1,1,1,1,1,1,1,1,1,1,1,1,1,1,1,1,1,1,
1,1,1,1,1,1,1,1,1,1,1,1,1,1,1,1,1,1,1,1,1,1,1,1,1,1,1,1,1,1,1,1,1,1,1,1,
1,1,1,1,1,1,1,1,1,1,1,1,1,1,1,1,1,1,1,1,1,1,1,1,1,1,1,1,1,1,1,1,1,1,1,1,
1,1,1,1,1,1,1,1,1,1,1,1,1,1,1,1,1,1,1,1,1,1,1,1,1,1,1,1,1,1,1,1,1,1,1,1,
1,1,1,1,1,1,1,1,1,1,1,1,1,1,1,1,1,1,1,1,1,1,1,1,1,1,1,1,1,1,1,1,1,1,1,1,
1,1,1,1,1,1,1,1,1,1,1,1,1,1,1,1,1,1,1,1,1,1,1,1,1,1,1,1,1,1,1,1,1,1,1,1,
1,1,1,1,1,1,1,1,1,1,1,1,1,1,1,1,1,1,1,1,1,1,1,1,1,1,1,1,1,1,1,1,1,1,1,1,
1,1,1,1,1,1,1,1,1,1,1,1,1,1,1,1,1,1,1,1,1,1,1,1,1,1,1,1,1,1,1,1,1,1,1,1,
1,1,1,1,1,1,1,1,1,1,1,1,1,1,1,1,1,1,1,1,1,1,1,1,1,1,1,1,1,1,1,1,1,1,1,1,
1,1,1,1,1,1,1,1,1,1,1,1,1,1,1,1,1,1,1,1,1,1,1,1,1,1,1,1,1,1,1,1,1,1,1,1,
1,1,1,1,1,1,1,1,1,1,1,1,1,1,1,1,1,1,1,1,1,1,1,1,1,1,1,1,1,1,1,1,1,1,1,1,
1,1,1,1,1,1,1,1,1,1,1,1,1,1,1,1,1,1,1,1,1,1,1,1,1,1,1,1,1,1,1,1,1,1,1,1,
1,1,1,1,1,1,1,1,1,1,1,1,1,1,1,1,1,1,1,1,1,1,1,1,1,1,1,1,1,1,1,1,1,1,1,1,
1,1,1,1,1,1,1,1,1,1,1,1,1,1,1,1,1,1,1,1,1,1,1,1,1,1,1,1,1,1,1,1,1,1,1,1,
1,1,1,1,1,1,1,1,1,1,1,1,1,1,1,1,1,1,1,1,1,1,1,1,1,1,1,1,1,1,1,1,1,1,1,1,
1,1,1,1,1,1,1,1,1,1,1,1,1,1,1,1,1,1,1,1,1,1,1,1,1,1,1,1,1,1,1,1,1,1,1,1,
1,1,1,1,1,1,1,1,1,1,1,1,1,1,1,1,1,1,1,1,1,1,1,1,1,1,1,1,1,1,1,1,1,1,1,1,
1,1,1,1,1,1,1,1,1,1,1,1,1,1,1,1,1,1,1,1,1,1,1,1,1,1,1,1,1,1,1,1,1,1,1,1,
1,1,1,1,1,1,1,1,1,1,1,1,1,1,1,1,1,1,1,1,1,1,1,1,1,1,1,1,1,1,1,1,1,1,1,1,
1,1,1,1,1,1,1,1,1,1,1,1,1,1,1,1,1,1,1,1,1,1,1,1,1,1,1,1,1,1,1,1,1,1,1,1,
1,1,1,1,1,1,1,1,1,1,1,1,1,1,1,1,1,1,1,1,1,1,1,1,1,1,1,1,1,1,1,1,1,1,1,1,
1,1,1,1,1,1,1,1,1,1,1,1,1,1,1,1,1,4),(-0.000423095957202541,0.115881565465356),
(11.6153146011728,12.1152895244478,12.6151575298078,13.614893540528,14.6146295512481,
15.6143655619682,16.6141015726884,17.6138375834085,18.6135735941286,19.6133096048488,
20.6130456155689,21.612781626289,22.6125176370092,23.6122536477293,24.6119896584494,
25.6117256691696,26.6114616798897,27.6111976906098,28.6109337013299,29.6106697120501,
30.6104057227702,31.6101417334903,32.6098777442105,33.6096137549306,34.6093497656507,
35.6090857763709,36.608821787091,37.6085577978111,38.6082938085313,39.6080298192514,
40.6077658299715,41.6075018406916,42.6072378514118,43.6069738621319,44.606709872852,
45.6064458835722,46.6061818942923,47.6059179050124,48.6056539157326,49.6053899264527,
50.6051259371728,51.604861947893,52.6045979586131,53.6043339693332,54.6040699800534,
55.6038059907735,56.6035420014936,57.6032780122137,58.6030140229339,59.602750033654,
60.6024860443741,61.6022220550943,62.6019580658144,63.6016940765345,64.6014300872547,
65.6011660979748,66.6009021086949,67.6006381194151,68.6003741301352,69.6001101408553,
70.5998461515754,71.5995821622956,72.5993181730157,73.5990541837358,74.598790194456,
75.5985262051761,76.5982622158962,77.5979982266164,78.5977342373365,79.5974702480566,
80.5972062587768,81.5969422694969,82.596678280217,83.5964142909372,84.5961503016573,
85.5958863123774,86.5956223230975,87.5953583338177,88.5950943445378,89.5948303552579,
90.5945663659781,91.5943023766982,92.5940383874183,93.5937743981385,94.5935104088586,
95.5932464195787,96.5929824302989,97.592718441019,98.5924544517391,99.5921904624593,
100.591926473179,101.5916624839,102.59139849462,103.59113450534,104.59087051606,
105.59060652678,106.5903425375,107.59007854822,108.58981455894,109.589550569661,
110.589286580381,111.589022591101,112.588758601821,113.588494612541,114.588230623261,
115.587966633981,116.587702644701,117.587438655422,118.587174666142,119.586910676862,
120.586646687582,121.586382698302,122.586118709022,123.585854719742,124.585590730463,
125.585326741183,126.585062751903,127.584798762623,128.584534773343,129.584270784063,
130.584006794783,131.583742805503,132.583478816224,133.583214826944,134.582950837664,
135.582686848384,136.582422859104,137.582158869824,138.581894880544,139.581630891264,
140.581366901985,141.581102912705,142.580838923425,143.580574934145,144.580310944865,
145.580046955585,146.579782966305,147.579518977026,148.579254987746,149.578990998466,
150.578727009186,151.578463019906,152.578199030626,153.577935041346,154.577671052066,
155.577407062787,156.577143073507,157.576879084227,158.576615094947,159.576351105667,
160.576087116387,161.575823127107,162.575559137827,163.575295148548,164.575031159268,
165.574767169988,166.574503180708,167.574239191428,168.573975202148,169.573711212868,
170.573447223589,171.573183234309,172.572919245029,173.572655255749,174.572391266469,
175.572127277189,176.571863287909,177.571599298629,178.57133530935,179.57107132007,
180.57080733079,181.57054334151,182.57027935223,183.57001536295,184.56975137367,
185.56948738439,186.569223395111,187.568959405831,188.568695416551,189.568431427271,
190.568167437991,191.567903448711,192.567639459431,193.567375470152,194.567111480872,
195.566847491592,196.566583502312,197.566319513032,198.566055523752,199.565791534472,
200.565527545192,201.565263555913,202.564999566633,203.564735577353,204.564471588073,
205.564207598793,206.563943609513,207.563679620233,208.563415630954,209.563151641674,
210.562887652394,211.562623663114,212.562359673834,213.562095684554,214.561831695274,
215.561567705994,216.561303716715,217.561039727435,218.560775738155,219.560511748875,
220.560247759595,221.559983770315,222.559719781035,223.559455791755,224.559191802476,
225.558927813196,226.558663823916,227.558399834636,228.558135845356,229.557871856076,
230.557607866796,231.557343877517,232.557079888237,233.556815898957,234.556551909677,
235.556287920397,236.556023931117,237.555759941837,238.555495952557,239.555231963278,
240.554967973998,241.554703984718,242.554439995438,243.554176006158,244.553912016878,
245.553648027598,246.553384038319,247.553120049039,248.552856059759,249.552592070479,
250.552328081199,251.552064091919,252.551800102639,253.551536113359,254.55127212408,
255.5510081348,256.55074414552,257.55048015624,258.55021616696,259.54995217768,
260.5496881884,261.54942419912,262.549160209841,263.548896220561,264.548632231281,
265.548368242001,266.548104252721,267.547840263441,268.547576274161,269.547312284882,
270.547048295602,271.546784306322,272.546520317042,273.546256327762,274.545992338482,
275.545728349202,276.545464359922,277.545200370643,278.544936381363,279.544672392083,
280.544408402803,281.544144413523,282.543880424243,283.543616434963,284.543352445683,
285.543088456404,286.542824467124,287.542560477844,288.542296488564,289.542032499284,
290.541768510004,291.541504520724,292.541240531445,293.540976542165,294.540712552885,
295.540448563605,296.540184574325,297.539920585045,298.539656595765,299.539392606485,
300.539128617206,301.538864627926,302.538600638646,303.538336649366,304.538072660086,
305.537808670806,306.537544681526,307.537280692246,308.537016702967,309.536752713687,
310.536488724407,311.536224735127,312.535960745847,313.535696756567,314.535432767287,
315.535168778008,316.534904788728,317.534640799448,318.534376810168,319.534112820888,
320.533848831608,321.533584842328,322.533320853048,323.533056863769,324.532792874489,
325.532528885209,326.532264895929,327.532000906649,328.531736917369,329.531472928089,
330.53120893881,331.53094494953,332.53068096025,333.53041697097,334.53015298169,
335.52988899241,336.52962500313,337.52936101385,338.529097024571,339.528833035291,
340.528569046011,341.528305056731,342.528041067451,343.527777078171,344.527513088891,
345.527249099611,346.526985110332,347.526721121052,348.526457131772,349.526193142492,
350.525929153212,351.525665163932,352.525401174652,353.525137185373,354.524873196093,
355.524609206813,356.524345217533,357.524081228253,358.523817238973,359.523553249693,
360.523289260413,361.523025271134,362.522761281854,363.522497292574,364.522233303294,
365.521969314014,366.521705324734,367.521441335454,368.521177346175,369.520913356895,
370.520649367615,371.520385378335,372.520121389055,373.519857399775,374.519593410495,
375.519329421215,376.519065431936,377.518801442656,378.518537453376,379.518273464096,
380.518009474816,381.517745485536,382.517481496256,383.517217506976,384.516953517697,
385.516689528417,386.516425539137,387.516161549857,388.515897560577,389.515633571297,
390.515369582017,391.515105592737,392.514841603458,393.514577614178,394.514313624898,
395.514049635618,396.513785646338,397.513521657058,398.513257667778,399.512993678499,
400.512729689219,401.512465699939,402.512201710659,403.511937721379,404.511673732099,
405.511409742819,406.511145753539,407.51088176426,408.51061777498,409.5103537857,
410.51008979642,411.50982580714,412.50956181786,413.50929782858,414.509033839301,
415.508769850021,416.508505860741,417.508241871461,418.507977882181,419.507713892901,
420.507449903621,421.507185914341,422.506921925062,423.506657935782,424.506393946502,
425.506129957222,426.505865967942,427.505601978662,428.505337989382,429.505074000102,
430.504810010823,431.504546021543,432.504282032263,433.504018042983,434.503754053703,
435.503490064423,436.503226075143,437.502962085864,438.502698096584,439.502434107304,
440.502170118024,441.501906128744,442.501642139464,443.501378150184,444.501114160904,
445.500850171625,446.500586182345,447.500322193065,448.500058203785,449.499794214505,
450.499530225225,451.499266235945,452.499002246665,453.498738257386,454.498474268106,
455.498210278826,456.497946289546,457.497682300266,458.497418310986,459.497154321706,
460.496890332427,461.496626343147,462.496362353867,463.496098364587,464.495834375307,
465.495570386027,466.495306396747,467.495042407467,468.494778418188,469.494514428908,
470.494250439628,471.493986450348,472.493722461068,473.493458471788,474.493194482508,
475.492930493229,476.492666503949,477.492402514669,478.492138525389,479.491874536109,
480.491610546829,481.491346557549,482.491082568269,483.49081857899,484.49055458971,
485.49029060043,486.49002661115,487.48976262187,488.48949863259,489.48923464331,
490.48897065403,491.488706664751,492.488442675471,493.488178686191,494.487914696911,
495.487650707631,496.487386718351,497.487122729071,498.486858739792,499.486594750512,
500.486330761232,501.486066771952,502.485802782672,503.485538793392,504.485274804112,
505.485010814832,506.484746825553,507.484482836273,508.484218846993,509.483954857713,
510.483690868433,511.483426879153,512.483162889873,513.482898900594,514.482634911314,
515.482370922034,516.482106932754,517.481842943474,518.481578954194,519.481314964914,
520.481050975635,521.480786986355,522.480522997075,523.480259007795,524.479995018515,
525.479731029235,526.479467039955,527.479203050675,528.478939061396,529.478675072116,
530.478411082836,531.478147093556,532.477883104276,533.477619114996,534.477355125716,
535.477091136436,536.476827147157,537.476563157877,538.476299168597,539.476035179317,
540.475771190037,541.475507200757,542.475243211477,543.474979222197,544.474715232918,
545.474451243638,546.474187254358,547.473923265078,548.473659275798,549.473395286518,
550.473131297238,551.472867307958,552.472603318679,553.472339329399,554.472075340119,
555.471811350839,556.471547361559,557.471283372279,558.471019382999,559.47075539372,
560.47049140444,561.47022741516,562.46996342588,563.4696994366,564.46943544732,
565.46917145804,566.46890746876,567.468643479481,568.468379490201,569.468115500921,
570.467851511641,571.467587522361,572.467323533081,573.467059543801,574.466795554521,
575.466531565242,576.466267575962,577.466003586682,578.465739597402,579.465475608122,
580.465211618842,581.464947629562,582.464683640283,583.464419651003,584.464155661723,
585.463891672443,586.463627683163,587.463363693883,588.463099704603,589.462835715323,
590.462571726044,591.462307736764,592.462043747484,593.461779758204,594.461515768924,
595.461251779644,596.460987790364,597.460723801085,598.460459811805,599.460195822525,
600.459931833245,601.459667843965,602.459403854685,603.459139865405,604.458875876125,
605.458611886846,606.458347897566,607.458083908286,608.457819919006,609.457555929726,
610.457291940446,611.457027951166,612.456763961887,613.456499972607,614.456235983327,
615.455971994047,616.455708004767,617.455444015487,618.455180026207,619.454916036927,
620.454652047648,621.454388058368,622.454124069088,623.453860079808,624.453596090528,
625.453332101248,626.453068111968,627.452804122688,628.452540133409,629.452276144129,
630.452012154849,631.451748165569,632.451484176289,633.451220187009,634.450956197729,
635.450692208449,636.45042821917,637.45016422989,638.44990024061,639.44963625133,
640.44937226205,641.44910827277,642.44884428349,643.448580294211,644.448316304931,
645.448052315651,646.447788326371,647.447524337091,648.447260347811,649.446996358531,
650.446732369251,651.446468379972,652.446204390692,653.445940401412,654.445676412132,
655.445412422852,656.445148433572,657.444884444292,658.444620455012,659.444356465733,
660.444092476453,661.443828487173,662.443564497893,663.443300508613,664.443036519333,
665.442772530053,666.442508540774,667.442244551494,668.441980562214,669.441716572934,
670.441452583654,671.441188594374,672.440924605094,673.440660615815,674.440396626535,
675.440132637255,676.439868647975,677.439604658695,678.439340669415,679.439076680135,
680.438812690855,681.438548701576,682.438284712296,683.438020723016,684.437756733736,
685.437492744456,686.437228755176,687.436964765896,688.436700776616,689.436436787337,
690.436172798057,691.435908808777,692.435644819497,693.435380830217,694.435116840937,
695.434852851657,696.434588862377,697.434324873098,698.434060883818,699.433796894538,
700.433532905258,701.433268915978,702.433004926698,703.432740937418,704.432476948139,
705.432212958859,706.431948969579,707.431684980299,708.431420991019,709.431157001739,
710.430893012459,711.430629023179,712.4303650339,713.43010104462,714.42983705534,
715.42957306606,716.42930907678,717.4290450875,718.42878109822,719.42851710894,
720.428253119661,721.427989130381,722.427725141101,723.427461151821,724.427197162541,
725.426933173261,726.426669183981,727.426405194702,728.426141205422,729.425877216142,
730.425613226862,731.425349237582,732.425085248302,733.424821259022,734.424557269742,
735.424293280463,736.424029291183,737.423765301903,738.423501312623,739.423237323343,
740.422973334063,741.422709344783,742.422445355504,743.422181366224,744.421917376944,
745.421653387664,746.421389398384,747.421125409104,748.420861419824,749.420597430544,
750.420333441265,751.420069451985,752.419805462705,753.419541473425,754.419277484145,
755.419013494865,756.418749505585,757.418485516306,758.418221527026,759.417957537746,
760.417693548466,761.417429559186,762.417165569906,763.416901580626,764.416637591346,
765.416373602067,766.416109612787,767.415845623507,768.415581634227,769.415317644947,
770.415053655667,771.414789666387,772.414525677107,773.414261687828,774.413997698548,
775.413733709268,776.413469719988,777.413205730708,778.412941741428,779.412677752148,
780.412413762868,781.412149773589,782.411885784309,783.411621795029,784.411357805749,
785.411093816469,786.410829827189,787.410565837909,788.41030184863,789.41003785935,
790.40977387007,791.40950988079,792.40924589151,793.40898190223,794.40871791295,
795.40845392367,796.408189934391,797.407925945111,798.407661955831,799.407397966551,
800.407133977271,801.406869987991,802.406605998711,803.406342009432,804.406078020152,
805.405814030872,806.405550041592,807.405286052312,808.405022063032,809.404758073752,
810.404494084472,811.404230095193,812.403966105913,813.403702116633,814.403438127353,
815.403174138073,816.402910148793,817.402646159513,818.402382170234,819.402118180954,
820.401854191674,821.401590202394,822.401326213114,823.401062223834,824.400798234554,
825.400534245274,826.400270255995,827.400006266715,828.399742277435,829.399478288155,
830.399214298875,831.398950309595,832.398686320315,833.398422331035,834.398158341756,
835.397894352476,836.397630363196,837.397366373916,838.397102384636,839.396838395356,
840.396574406076,841.396310416796,842.396046427517,843.395782438237,844.395518448957,
845.395254459677,846.394990470397,847.394726481117,848.394462491837,849.394198502558,
850.393934513278,851.393670523998,852.393406534718,853.393142545438,854.392878556158,
855.392614566878,856.392350577598,857.392086588319,858.391822599039,859.391558609759,
860.391294620479,861.391030631199,862.390766641919,863.390502652639,864.390238663359,
865.38997467408,866.3897106848,867.38944669552,868.38918270624,869.38891871696,
870.38865472768,871.3883907384,872.388126749121,873.387862759841,874.387598770561,
875.387334781281,876.387070792001,877.386806802721,878.386542813441,879.386278824161,
880.386014834882,881.385750845602,882.385486856322,883.385222867042,884.384958877762,
885.384694888482,886.384430899202,887.384166909923,888.383902920643,889.383638931363,
890.383374942083,891.383110952803,892.382846963523,893.382582974243,894.382318984963,
895.382054995684,896.381791006404,897.381527017124,898.381263027844,899.380999038564,
900.380735049284,901.380471060004,902.380207070725,903.379943081445,904.379679092165,
905.379415102885,906.379151113605,907.378887124325,908.378623135045,909.378359145765,
910.378095156486,911.377831167206,912.377567177926,913.377303188646,914.377039199366,
915.376775210086,916.376511220806,917.376247231526,918.375983242247,919.375719252967,
920.375455263687,921.375191274407,922.374927285127,923.374663295847,924.374399306567,
925.374135317287,926.373871328008,927.373607338728,928.373343349448,929.373079360168,
930.372815370888,931.372551381608,932.372287392328,933.372023403049,934.371759413769,
935.371495424489,936.371231435209,937.370967445929,938.370703456649,939.370439467369,
940.370175478089,941.36991148881,942.36964749953,943.36938351025,944.36911952097,
945.36885553169,946.36859154241,947.36832755313,948.368063563851,949.367799574571,
950.367535585291,951.367271596011,952.367007606731,953.366743617451,954.366479628171,
955.366215638891,956.365951649612,957.365687660332,958.365423671052,959.365159681772,
960.364895692492,961.364631703212,962.364367713932,963.364103724653,964.363839735373,
965.363575746093,966.363311756813,967.363047767533,968.362783778253,969.362519788973,
970.362255799693,971.361991810414,972.361727821134,973.361463831854,974.361199842574,
975.360935853294,976.360671864014,977.360407874734,978.360143885454,979.359879896175,
980.359615906895,981.359351917615,982.359087928335,983.358823939055,984.358559949775,
985.358295960495,986.358031971215,987.357767981936,988.357503992656,989.357240003376,
990.356976014096,991.356712024816,992.356448035536,993.356184046256,994.355920056977,
995.355656067697,996.355392078417,997.355128089137,998.354864099857,999.354600110577,
1000.3543361213,1001.35407213202,1002.35380814274,1003.35354415346,1004.35328016418,
1005.3530161749,1006.35275218562,1007.35248819634,1008.35222420706,1009.35196021778,
1010.3516962285,1011.35143223922,1012.35116824994,1013.35090426066,1014.35064027138,
1015.3503762821,1016.35011229282,1017.34984830354,1018.34958431426,1019.34932032498,
1020.3490563357,1021.34879234642,1022.34852835714,1023.34826436786,1024.34800037858,
1025.3477363893,1026.34747240002,1027.34720841074,1028.34694442146,1029.34668043218,
1030.3464164429,1031.34615245362,1032.34588846434,1033.34562447506,1034.34536048578,
1035.3450964965,1036.34483250722,1037.34456851794,1038.34430452866,1039.34404053938,
1040.3437765501,1041.34351256082,1042.34324857154,1043.34298458226,1044.34272059298,
1045.3424566037,1046.34219261442,1047.34192862514,1048.34166463586,1049.34140064658,
1050.3411366573,1051.34087266802,1052.34060867874,1053.34034468946,1054.34008070018,
1055.3398167109,1056.33955272162,1057.33928873234,1058.33902474307,1059.33876075378,
1060.33849676451,1061.33823277523,1062.33796878595,1063.33770479667,1064.33744080739,
1065.33717681811,1066.33691282883,1067.33664883955,1068.33638485027,1069.33612086099,
1070.33585687171,1071.33559288243,1072.33532889315,1073.33506490387,1074.33480091459,
1075.33453692531,1076.33427293603,1077.33400894675,1078.33374495747,1079.33348096819,
1080.33321697891,1081.33295298963,1082.33268900035,1083.33242501107,1084.33216102179,
1085.33189703251,1086.33163304323,1087.33136905395,1088.33110506467,1089.33084107539,
1090.33057708611,1091.33031309683,1092.33004910755,1093.32978511827,1094.32952112899,
1095.32925713971,1096.32899315043,1097.32872916115,1098.32846517187,1099.32820118259,
1100.32793719331,1101.32767320403,1102.32740921475,1103.32714522547,1104.32688123619,
1105.32661724691,1106.32635325763,1107.32608926835,1108.32582527907,1109.32556128979,
1110.32529730051,1111.32503331123,1112.32476932195,1113.32450533267,1114.32424134339,
1115.32397735411,1116.32371336483,1117.32344937555,1118.32318538627,1119.32292139699,
1120.32265740771,1121.32239341843,1122.32212942915,1123.32186543987,1124.32160145059,
1125.32133746131,1126.32107347203,1127.32080948275,1128.32054549347,1129.32028150419,
1130.32001751491,1131.31975352563,1132.31948953635,1133.31922554707,1134.31896155779,
1135.31869756852,1136.31843357924,1137.31816958996,1138.31790560068,1139.3176416114,
1140.31737762212,1141.31711363284,1142.31684964356,1143.31658565428,1144.316321665,
1145.31605767572,1146.31579368644,1147.31552969716,1148.31526570788,1149.3150017186,
1150.31473772932,1151.31447374004,1152.31420975076,1153.31394576148,1154.3136817722,
1155.31341778292,1156.31315379364,1157.31288980436,1158.31262581508,1159.3123618258,
1160.31209783652,1161.31183384724,1162.31156985796,1163.31130586868,1164.3110418794,
1165.31077789012,1166.31051390084,1167.31024991156,1168.30998592228,1169.309721933,
1170.30945794372,1171.30919395444,1172.30892996516,1173.30866597588,1174.3084019866,
1175.30813799732,1176.30787400804,1177.30761001876,1178.30734602948,1179.3070820402,
1180.30681805092,1181.30655406164,1182.30629007236,1183.30602608308,1184.3057620938,
1185.30549810452,1186.30523411524,1187.30497012596,1188.30470613668,1189.3044421474,
1190.30417815812,1191.30391416884,1192.30365017956,1193.30338619028,1194.303122201,
1195.30285821172,1196.30259422244,1197.30233023316,1198.30206624388,1199.3018022546,
1200.30153826532,1201.30127427604,1202.30101028676,1203.30074629748,1204.3004823082,
1205.30021831892,1206.29995432964,1207.29969034036,1208.29942635108,1209.2991623618,
1210.29889837252,1211.29863438324,1212.29837039397,1213.29810640469,1214.29784241541,
1215.29757842613,1216.29731443685,1217.29705044757,1218.29678645829,1219.29652246901,
1220.29625847973,1221.29599449045,1222.29573050117,1223.29546651189,1224.29520252261,
1225.29493853333,1226.29467454405,1227.29441055477,1228.29414656549,1229.29388257621,
1230.29361858693,1231.29335459765,1232.29309060837,1233.29282661909,1234.29256262981,
1235.29229864053,1236.29203465125,1237.29177066197,1238.29150667269,1239.29124268341,
1240.29097869413,1241.29071470485,1242.29045071557,1243.29018672629,1244.28992273701,
1245.28965874773,1246.28939475845,1247.28913076917,1248.28886677989,1249.28860279061,
1250.28833880133,1251.28807481205,1252.28781082277,1253.28754683349,1254.28728284421,
1255.28701885493,1256.28675486565,1257.28649087637,1258.28622688709,1259.28596289781,
1260.28569890853,1261.28543491925,1262.28517092997,1263.28490694069,1264.28464295141,
1265.28437896213,1266.28411497285,1267.28385098357,1268.28358699429,1269.28332300501,
1270.28305901573,1271.28279502645,1272.28253103717,1273.28226704789,1274.28200305861,
1275.28173906933,1276.28147508005,1277.28121109077,1278.28094710149,1279.28068311221,
1280.28041912293,1281.28015513365,1282.27989114437,1283.27962715509,1284.27936316581,
1285.27909917653,1286.27883518725,1287.27857119797,1288.2783072087,1289.27804321942,
1290.27777923014,1291.27751524086,1292.27725125158,1293.2769872623,1294.27672327302,
1295.27645928374,1296.27619529446,1297.27593130518,1298.2756673159,1299.27540332662,
1300.27513933734,1301.27487534806,1302.27461135878,1303.2743473695,1304.27408338022,
1305.27381939094,1306.27355540166,1307.27329141238,1308.2730274231,1309.27276343382,
1310.27249944454,1311.27223545526,1312.27197146598,1313.2717074767,1314.27144348742,
1315.27117949814,1316.27091550886,1317.27065151958,1318.2703875303,1319.27012354102,
1320.26985955174,1321.26959556246,1322.26933157318,1323.2690675839,1324.26880359462,
1325.26853960534,1326.26827561606,1327.26801162678,1328.2677476375,1329.26748364822,
1330.26721965894,1331.26695566966,1332.26669168038,1333.2664276911,1334.26616370182,
1335.26589971254,1336.26563572326,1337.26537173398,1338.2651077447,1339.26484375542,
1340.26457976614,1341.26431577686,1342.26405178758,1343.2637877983,1344.26352380902,
1345.26325981974,1346.26299583046,1347.26273184118,1348.2624678519,1349.26220386262,
1350.26193987334,1351.26167588406,1352.26141189478,1353.2611479055,1354.26088391622,
1355.26061992694,1356.26035593766,1357.26009194838,1358.2598279591,1359.25956396982,
1360.25929998054,1361.25903599126,1362.25877200198,1363.2585080127,1364.25824402343,
1365.25798003415,1366.25771604487,1367.25745205559,1368.25718806631,1369.25692407703,
1370.25666008775,1371.25639609847,1372.25613210919,1373.25586811991,1374.25560413063,
1375.25534014135,1376.25507615207,1377.25481216279,1378.25454817351,1379.25428418423,
1380.25402019495,1381.25375620567,1382.25349221639,1383.25322822711,1384.25296423783,
1385.25270024855,1386.25243625927,1387.25217226999,1388.25190828071,1389.25164429143,
1390.25138030215,1391.25111631287,1392.25085232359,1393.25058833431,1394.25032434503,
1395.25006035575,1396.24979636647,1397.24953237719,1398.24926838791,1399.24900439863,
1400.24874040935,1401.24847642007,1402.24821243079,1403.24794844151,1404.24768445223,
1405.24742046295,1406.24715647367,1407.24689248439,1408.24662849511,1409.24636450583,
1410.24610051655,1411.24583652727,1412.24557253799,1413.24530854871,1414.24504455943,
1415.24478057015,1416.24451658087,1417.24425259159,1418.24398860231,1419.24372461303,
1420.24346062375,1421.24319663447,1422.24293264519,1423.24266865591,1424.24240466663,
1425.24214067735,1426.24187668807,1427.24161269879,1428.24134870951,1429.24108472023,
1430.24082073095,1431.24055674167,1432.24029275239,1433.24002876311,1434.23976477383,
1435.23950078455,1436.23923679527,1437.23897280599,1438.23870881671,1439.23844482743,
1440.23818083815,1441.23791684888,1442.2376528596,1443.23738887032,1444.23712488104,
1445.23686089176,1446.23659690248,1447.2363329132,1448.23606892392,1449.23580493464,
1450.23554094536,1451.23527695608,1452.2350129668,1453.23474897752,1454.23448498824,
1455.23422099896,1456.23395700968,1457.2336930204,1458.23342903112,1459.23316504184,
1460.23290105256,1461.23263706328,1462.232373074,1463.23210908472,1464.23184509544,
1465.23158110616,1466.23131711688,1467.2310531276,1468.23078913832,1469.23052514904,
1470.23026115976,1471.22999717048,1472.2297331812,1473.22946919192,1474.22920520264,
1475.22894121336,1476.22867722408,1477.2284132348,1478.22814924552,1479.22788525624,
1480.22762126696,1481.22735727768,1482.2270932884,1483.22682929912,1484.22656530984,
1485.22630132056,1486.22603733128,1487.225773342,1488.22550935272,1489.22524536344,
1490.22498137416,1491.22471738488,1492.2244533956,1493.22418940632,1494.22392541704,
1495.22366142776,1496.22339743848,1497.2231334492,1498.22286945992,1499.22260547064,
1500.22234148136,1501.22207749208,1502.2218135028,1503.22154951352,1504.22128552424,
1505.22102153496,1506.22075754568,1507.2204935564,1508.22022956712,1509.21996557784,
1510.21970158856,1511.21943759928,1512.21917361,1513.21890962072,1514.21864563144,
1515.21838164216,1516.21811765288,1517.21785366361,1518.21758967433,1519.21732568505,
1520.21706169577,1521.21679770649,1522.21653371721,1523.21626972793,1524.21600573865,
1525.21574174937,1526.21547776009,1527.21521377081,1528.21494978153,1529.21468579225,
1530.21442180297,1531.21415781369,1532.21389382441,1533.21362983513,1534.21336584585,
1535.21310185657,1536.21283786729,1537.21257387801,1538.21230988873,1539.21204589945,
1540.21178191017,1541.21151792089,1542.21125393161,1543.21098994233,1544.21072595305,
1545.21046196377,1546.21019797449,1547.20993398521,1548.20966999593,1549.20940600665,
1550.20914201737,1551.20887802809,1552.20861403881,1553.20835004953,1554.20808606025,
1555.20782207097,1556.20755808169,1557.20729409241,1558.20703010313,1559.20676611385,
1560.20650212457,1561.20623813529,1562.20597414601,1563.20571015673,1564.20544616745,
1565.20518217817,1566.20491818889,1567.20465419961,1568.20439021033,1569.20412622105,
1570.20386223177,1571.20359824249,1572.20333425321,1573.20307026393,1574.20280627465,
1575.20254228537,1576.20227829609,1577.20201430681,1578.20175031753,1579.20148632825,
1580.20122233897,1581.20095834969,1582.20069436041,1583.20043037113,1584.20016638185,
1585.19990239257,1586.19963840329,1587.19937441401,1588.19911042473,1589.19884643545,
1590.19858244617,1591.19831845689,1592.19805446761,1593.19779047834,1594.19752648906,
1595.19726249978,1596.1969985105,1597.19673452122,1598.19647053194,1599.19620654266,
1600.19594255338,1601.1956785641,1602.19541457482,1603.19515058554,1604.19488659626,
1605.19462260698,1606.1943586177,1607.19409462842,1608.19383063914,1609.19356664986,
1610.19330266058,1611.1930386713,1612.19277468202,1613.19251069274,1614.19224670346,
1615.19198271418,1616.1917187249,1617.19145473562,1618.19119074634,1619.19092675706,
1620.19066276778,1621.1903987785,1622.19013478922,1623.18987079994,1624.18960681066,
1625.18934282138,1626.1890788321,1627.18881484282,1628.18855085354,1629.18828686426,
1630.18802287498,1631.1877588857,1632.18749489642,1633.18723090714,1634.18696691786,
1635.18670292858,1636.1864389393,1637.18617495002,1638.18591096074,1639.18564697146,
1640.18538298218,1641.1851189929,1642.18485500362,1643.18459101434,1644.18432702506,
1645.18406303578,1646.1837990465,1647.18353505722,1648.18327106794,1649.18300707866,
1650.18274308938,1651.1824791001,1652.18221511082,1653.18195112154,1654.18168713226,
1655.18142314298,1656.1811591537,1657.18089516442,1658.18063117514,1659.18036718586,
1660.18010319658,1661.1798392073,1662.17957521802,1663.17931122874,1664.17904723946,
1665.17878325018,1666.1785192609,1667.17825527162,1668.17799128234,1669.17772729307,
1670.17746330379,1671.17719931451,1672.17693532523,1673.17667133595,1674.17640734667,
1675.17614335739,1676.17587936811,1677.17561537883,1678.17535138955,1679.17508740027,
1680.17482341099,1681.17455942171,1682.17429543243,1683.17403144315,1684.17376745387,
1685.17350346459,1686.17323947531,1687.17297548603,1688.17271149675,1689.17244750747,
1690.17218351819,1691.17191952891,1692.17165553963,1693.17139155035,1694.17112756107,
1695.17086357179,1696.17059958251,1697.17033559323,1698.17007160395,1699.16980761467,
1700.16954362539,1700.66941163075,1701.16959429301),.UNSPECIFIED.);
#1809=B_SPLINE_CURVE_WITH_KNOTS('',3,(#240811,#240812,#240813,#240814,#240815,
#240816,#240817,#240818,#240819,#240820),.UNSPECIFIED.,.F.,.F.,(4,3,3,4),
(1504.57104348731,1504.65363118549,1504.73825612743,1504.82288106937),
 .UNSPECIFIED.);
#1810=B_SPLINE_CURVE_WITH_KNOTS('',3,(#240822,#240823,#240824,#240825,#240826,
#240827,#240828,#240829,#240830,#240831,#240832,#240833,#240834,#240835,
#240836,#240837,#240838,#240839,#240840,#240841,#240842,#240843,#240844,
#240845,#240846,#240847,#240848,#240849,#240850,#240851,#240852,#240853,
#240854,#240855,#240856,#240857,#240858,#240859,#240860,#240861,#240862,
#240863,#240864,#240865,#240866,#240867,#240868,#240869,#240870,#240871,
#240872,#240873,#240874,#240875,#240876,#240877,#240878,#240879,#240880,
#240881,#240882,#240883,#240884,#240885,#240886,#240887,#240888,#240889,
#240890,#240891,#240892,#240893,#240894,#240895,#240896,#240897,#240898,
#240899,#240900,#240901,#240902,#240903,#240904,#240905,#240906,#240907,
#240908,#240909,#240910,#240911,#240912,#240913,#240914,#240915,#240916,
#240917,#240918,#240919,#240920,#240921,#240922,#240923,#240924,#240925,
#240926,#240927,#240928,#240929,#240930,#240931,#240932,#240933,#240934,
#240935,#240936,#240937,#240938,#240939,#240940,#240941,#240942,#240943,
#240944,#240945,#240946,#240947,#240948,#240949,#240950,#240951,#240952,
#240953,#240954,#240955,#240956,#240957,#240958,#240959,#240960,#240961,
#240962,#240963,#240964,#240965,#240966,#240967,#240968,#240969,#240970,
#240971,#240972),.UNSPECIFIED.,.F.,.F.,(4,3,3,3,3,3,3,3,3,3,3,3,3,3,3,3,
3,3,3,3,3,3,3,3,3,3,3,3,3,3,3,3,3,3,3,3,3,3,3,3,3,3,3,3,3,3,3,3,3,3,4),
(1504.8228810695,1504.91073091525,1504.9944696271,1505.07810513846,1505.16165758186,
1505.24514701771,1505.32860096832,1505.41203746217,1505.49547457192,1505.57893036684,
1505.66247485957,1505.74606394251,1505.82978721006,1505.91046692597,1505.99420563782,
1506.07784114918,1506.16139359258,1506.24488302843,1506.32833697905,1506.41177347289,
1506.49521058265,1506.57866637757,1506.6622108703,1506.74579995324,1506.82952322079,
1506.91020293669,1506.99394164854,1507.0775771599,1507.1611296033,1507.24461903915,
1507.32807298977,1507.41150948361,1507.49494659337,1507.57840238829,1507.66194688102,
1507.74553596396,1507.82925923151,1507.90993894741,1507.99367765926,1508.07731317062,
1508.16086561402,1508.24435504987,1508.32780900049,1508.41124549433,1508.49468260409,
1508.57813839901,1508.66168289173,1508.74527197468,1508.82899524223,1508.90967495813,
1508.96603014687),.UNSPECIFIED.);
#1811=B_SPLINE_CURVE_WITH_KNOTS('',3,(#240974,#240975,#240976,#240977,#240978,
#240979),.UNSPECIFIED.,.F.,.F.,(4,2,4),(1.56320921069321,1.68048617233251,
1.7638474477127),.UNSPECIFIED.);
#1812=B_SPLINE_CURVE_WITH_KNOTS('',3,(#240981,#240982,#240983,#240984,#240985,
#240986,#240987,#240988,#240989,#240990,#240991,#240992,#240993,#240994,
#240995,#240996,#240997,#240998,#240999,#241000,#241001,#241002,#241003,
#241004,#241005,#241006,#241007,#241008,#241009,#241010,#241011,#241012,
#241013,#241014,#241015,#241016,#241017,#241018,#241019,#241020,#241021,
#241022,#241023,#241024,#241025,#241026,#241027,#241028,#241029,#241030,
#241031,#241032,#241033,#241034,#241035,#241036,#241037,#241038,#241039,
#241040,#241041,#241042,#241043,#241044,#241045,#241046,#241047,#241048,
#241049,#241050,#241051,#241052,#241053,#241054,#241055,#241056,#241057,
#241058,#241059,#241060,#241061,#241062,#241063,#241064,#241065,#241066,
#241067,#241068,#241069,#241070,#241071,#241072,#241073,#241074,#241075,
#241076,#241077,#241078,#241079,#241080,#241081,#241082,#241083,#241084,
#241085,#241086,#241087,#241088,#241089,#241090,#241091,#241092,#241093,
#241094,#241095,#241096,#241097,#241098,#241099,#241100,#241101,#241102,
#241103,#241104,#241105,#241106,#241107,#241108,#241109,#241110,#241111,
#241112,#241113,#241114,#241115,#241116,#241117,#241118,#241119,#241120,
#241121,#241122,#241123,#241124,#241125,#241126,#241127,#241128,#241129,
#241130,#241131,#241132,#241133,#241134,#241135,#241136,#241137,#241138,
#241139,#241140,#241141,#241142,#241143,#241144,#241145,#241146),
 .UNSPECIFIED.,.F.,.F.,(4,3,3,3,3,3,3,3,3,3,3,3,3,3,3,3,3,3,3,3,3,3,3,3,
3,3,3,3,3,3,3,3,3,3,3,3,3,3,3,3,3,3,3,3,3,3,3,3,3,3,3,3,3,3,3,4),(1504.82288106969,
1504.91507842316,1505.00777905537,1505.1007403094,1505.19403937815,1505.22102153496,
1505.30476024681,1505.38839575818,1505.47194820158,1505.55543763743,1505.63889158805,
1505.7223280819,1505.80576519166,1505.88922098658,1505.97276547931,1506.05635456225,
1506.14007782982,1506.22075754568,1506.30449625753,1506.38813176889,1506.47168421229,
1506.55517364814,1506.63862759876,1506.7220640926,1506.80550120236,1506.88895699728,
1506.97250149001,1507.05609057295,1507.13981384051,1507.2204935564,1507.30423226825,
1507.38786777961,1507.47142022301,1507.55490965886,1507.63836360947,1507.72180010332,
1507.80523721307,1507.88869300799,1507.97223750072,1508.05582658366,1508.13954985122,
1508.22022956712,1508.30396827897,1508.38760379033,1508.47115623373,1508.55464566958,
1508.6380996202,1508.72153611404,1508.8049732238,1508.88842901872,1508.97197351145,
1509.05556259439,1509.13928586195,1509.21996557784,1509.30425789109,1509.38855020433),
 .UNSPECIFIED.);
#1813=B_SPLINE_CURVE_WITH_KNOTS('',3,(#241147,#241148,#241149,#241150,#241151,
#241152,#241153,#241154,#241155,#241156),.UNSPECIFIED.,.F.,.F.,(4,3,3,4),
(1504.57225479568,1504.65682073549,1504.74135303069,1504.82288106951),
 .UNSPECIFIED.);
#1814=B_SPLINE_CURVE_WITH_KNOTS('',3,(#241162,#241163,#241164,#241165),
 .UNSPECIFIED.,.F.,.F.,(4,4),(1498.28924643674,1498.53969576232),
 .UNSPECIFIED.);
#1815=B_SPLINE_CURVE_WITH_KNOTS('',3,(#241166,#241167,#241168,#241169,#241170,
#241171,#241172,#241173,#241174,#241175,#241176,#241177,#241178,#241179,
#241180,#241181,#241182,#241183,#241184,#241185,#241186,#241187,#241188,
#241189,#241190,#241191,#241192,#241193,#241194,#241195,#241196,#241197,
#241198,#241199,#241200,#241201,#241202,#241203,#241204,#241205,#241206,
#241207,#241208,#241209,#241210,#241211,#241212,#241213,#241214,#241215,
#241216,#241217,#241218,#241219,#241220,#241221,#241222,#241223,#241224,
#241225,#241226,#241227,#241228,#241229,#241230,#241231,#241232,#241233,
#241234,#241235,#241236,#241237,#241238,#241239,#241240,#241241,#241242,
#241243,#241244,#241245,#241246,#241247,#241248,#241249,#241250,#241251,
#241252,#241253,#241254,#241255,#241256,#241257,#241258,#241259,#241260,
#241261,#241262,#241263,#241264,#241265,#241266,#241267,#241268,#241269,
#241270,#241271,#241272,#241273,#241274,#241275,#241276,#241277,#241278,
#241279,#241280,#241281,#241282,#241283,#241284,#241285,#241286,#241287,
#241288,#241289,#241290,#241291,#241292,#241293,#241294,#241295,#241296,
#241297,#241298,#241299,#241300,#241301,#241302,#241303,#241304,#241305,
#241306,#241307,#241308,#241309,#241310,#241311,#241312,#241313,#241314,
#241315,#241316,#241317,#241318,#241319,#241320,#241321,#241322,#241323,
#241324,#241325,#241326,#241327,#241328,#241329,#241330,#241331,#241332,
#241333,#241334,#241335,#241336,#241337,#241338,#241339,#241340,#241341,
#241342,#241343,#241344,#241345,#241346,#241347,#241348,#241349,#241350,
#241351,#241352,#241353,#241354,#241355,#241356,#241357,#241358,#241359,
#241360,#241361,#241362,#241363,#241364,#241365,#241366,#241367,#241368,
#241369,#241370,#241371,#241372,#241373,#241374,#241375,#241376,#241377,
#241378,#241379,#241380,#241381,#241382),.UNSPECIFIED.,.F.,.F.,(4,3,3,3,
3,3,3,3,3,3,3,3,3,3,3,3,3,3,3,3,3,3,3,3,3,3,3,3,3,3,3,3,3,3,3,3,3,3,3,3,
3,3,3,3,3,3,3,3,3,3,3,3,3,3,3,3,3,3,3,3,3,3,3,3,3,3,3,3,3,3,3,3,4),(1498.53969576232,
1498.63380533641,1498.72828492247,1498.82328898073,1498.91231485092,1498.99605356277,
1499.07968907413,1499.16324151753,1499.24673095338,1499.33018490399,1499.41362139784,
1499.4970585076,1499.58051430251,1499.66405879524,1499.74764787818,1499.83137114574,
1499.91205086164,1499.99578957349,1500.07942508486,1500.16297752826,1500.24646696411,
1500.32992091473,1500.41335740858,1500.49679451833,1500.58025031325,1500.66379480598,
1500.74738388893,1500.83110715649,1500.91178687237,1500.99552558422,1501.07916109558,
1501.16271353898,1501.24620297483,1501.32965692545,1501.41309341929,1501.49653052905,
1501.57998632397,1501.6635308167,1501.74711989964,1501.8308431672,1501.91152288309,
1501.99526159493,1502.0788971063,1502.1624495497,1502.24593898555,1502.32939293616,
1502.41282943001,1502.49626653976,1502.57972233468,1502.66326682741,1502.74685591035,
1502.8305791779,1502.91125889381,1502.99499760566,1503.07863311703,1503.16218556043,
1503.24567499628,1503.32912894689,1503.41256544074,1503.4960025505,1503.57945834542,
1503.66300283815,1503.74659192109,1503.83031518865,1503.91099490453,1503.99374376682,
1504.0763980856,1504.15897688734,1504.24149913172,1504.32399495184,1504.4064721317,
1504.48898209449,1504.57104348731),.UNSPECIFIED.);
#1816=B_SPLINE_CURVE_WITH_KNOTS('',3,(#241384,#241385,#241386,#241387,#241388,
#241389,#241390,#241391,#241392,#241393,#241394,#241395,#241396,#241397,
#241398,#241399,#241400,#241401,#241402,#241403,#241404,#241405,#241406,
#241407,#241408,#241409,#241410,#241411,#241412,#241413,#241414,#241415,
#241416,#241417,#241418,#241419,#241420,#241421,#241422,#241423,#241424,
#241425,#241426,#241427,#241428,#241429,#241430,#241431,#241432,#241433,
#241434,#241435,#241436,#241437,#241438,#241439,#241440,#241441,#241442,
#241443,#241444,#241445,#241446,#241447,#241448,#241449,#241450,#241451,
#241452,#241453,#241454,#241455,#241456,#241457,#241458,#241459,#241460,
#241461,#241462,#241463,#241464,#241465,#241466,#241467,#241468,#241469,
#241470,#241471,#241472,#241473,#241474,#241475,#241476,#241477,#241478,
#241479,#241480,#241481,#241482,#241483,#241484,#241485,#241486,#241487,
#241488,#241489,#241490,#241491,#241492,#241493,#241494,#241495,#241496,
#241497,#241498,#241499,#241500,#241501,#241502,#241503,#241504,#241505,
#241506,#241507,#241508,#241509,#241510,#241511,#241512,#241513,#241514,
#241515,#241516,#241517,#241518,#241519,#241520,#241521,#241522,#241523,
#241524,#241525,#241526,#241527,#241528,#241529,#241530,#241531,#241532,
#241533,#241534,#241535,#241536,#241537,#241538,#241539,#241540,#241541,
#241542,#241543,#241544,#241545,#241546,#241547,#241548,#241549,#241550,
#241551,#241552,#241553,#241554,#241555,#241556,#241557,#241558,#241559,
#241560,#241561,#241562,#241563,#241564,#241565,#241566,#241567,#241568,
#241569,#241570,#241571,#241572,#241573,#241574,#241575,#241576,#241577,
#241578,#241579,#241580,#241581,#241582,#241583,#241584,#241585,#241586,
#241587,#241588,#241589,#241590,#241591,#241592,#241593,#241594,#241595,
#241596,#241597,#241598,#241599,#241600,#241601,#241602,#241603,#241604,
#241605,#241606),.UNSPECIFIED.,.F.,.F.,(4,3,3,3,3,3,3,3,3,3,3,3,3,3,3,3,
3,3,3,3,3,3,3,3,3,3,3,3,3,3,3,3,3,3,3,3,3,3,3,3,3,3,3,3,3,3,3,3,3,3,3,3,
3,3,3,3,3,3,3,3,3,3,3,3,3,3,3,3,3,3,3,3,3,3,4),(1498.53969576233,1498.62505947587,
1498.70820805334,1498.79135490896,1498.87451833665,1498.96154012015,1499.04483918337,
1499.12819845884,1499.21167592631,1499.22260547064,1499.30634418249,1499.38997969385,
1499.47353213725,1499.55702157311,1499.64047552372,1499.72391201757,1499.80734912732,
1499.89080492224,1499.97434941497,1500.05793849791,1500.14166176547,1500.22234148136,
1500.30608019321,1500.38971570457,1500.47326814797,1500.55675758382,1500.64021153444,
1500.72364802828,1500.80708513804,1500.89054093296,1500.97408542569,1501.05767450863,
1501.14139777619,1501.22207749208,1501.30581620393,1501.38945171529,1501.47300415869,
1501.55649359454,1501.63994754516,1501.723384039,1501.80682114876,1501.89027694367,
1501.9738214364,1502.05741051934,1502.1411337869,1502.2218135028,1502.30555221465,
1502.38918772601,1502.47274016941,1502.55622960526,1502.63968355588,1502.72312004972,
1502.80655715948,1502.8900129544,1502.97355744713,1503.05714653007,1503.14086979762,
1503.22154951352,1503.30528822537,1503.38892373673,1503.47247618013,1503.55596561598,
1503.63941956659,1503.72285606044,1503.80629317019,1503.88974896511,1503.97329345784,
1504.05688254078,1504.14060580834,1504.22128552424,1504.3090278421,1504.39384146299,
1504.47856831567,1504.56320793387,1504.57225479568),.UNSPECIFIED.);
#1817=B_SPLINE_CURVE_WITH_KNOTS('',3,(#241607,#241608,#241609,#241610,#241611,
#241612,#241613,#241614,#241615,#241616),.UNSPECIFIED.,.F.,.F.,(4,3,3,4),
(1498.28900992258,1498.38879043601,1498.48754282435,1498.53969576216),
 .UNSPECIFIED.);
#1818=B_SPLINE_CURVE_WITH_KNOTS('',3,(#241622,#241623,#241624,#241625),
 .UNSPECIFIED.,.F.,.F.,(4,4),(1492.00598701905,1492.25651045514),
 .UNSPECIFIED.);
#1819=B_SPLINE_CURVE_WITH_KNOTS('',3,(#241626,#241627,#241628,#241629,#241630,
#241631,#241632,#241633,#241634,#241635),.UNSPECIFIED.,.F.,.F.,(4,1,1,1,
1,1,1,4),(1492.25651045514,1492.9138987866,1493.91363479732,1494.91337080804,
1495.91310681876,1496.91284282948,1497.9125788402,1498.28924643674),
 .UNSPECIFIED.);
#1820=B_SPLINE_CURVE_WITH_KNOTS('',3,(#241637,#241638,#241639,#241640,#241641,
#241642,#241643,#241644,#241645,#241646,#241647,#241648,#241649,#241650,
#241651,#241652,#241653,#241654,#241655,#241656,#241657,#241658,#241659,
#241660,#241661,#241662,#241663,#241664,#241665,#241666,#241667,#241668,
#241669,#241670,#241671,#241672,#241673,#241674,#241675,#241676,#241677,
#241678,#241679,#241680,#241681,#241682,#241683,#241684,#241685,#241686,
#241687,#241688,#241689,#241690,#241691,#241692,#241693,#241694,#241695,
#241696,#241697,#241698,#241699,#241700,#241701,#241702,#241703,#241704,
#241705,#241706,#241707,#241708,#241709,#241710,#241711,#241712,#241713,
#241714,#241715,#241716,#241717,#241718,#241719,#241720,#241721,#241722,
#241723,#241724,#241725,#241726,#241727,#241728,#241729,#241730,#241731,
#241732,#241733,#241734,#241735,#241736,#241737,#241738,#241739,#241740,
#241741,#241742,#241743,#241744,#241745,#241746,#241747,#241748,#241749,
#241750,#241751,#241752,#241753,#241754,#241755,#241756,#241757,#241758,
#241759,#241760,#241761,#241762,#241763,#241764,#241765,#241766,#241767,
#241768,#241769,#241770,#241771,#241772,#241773,#241774,#241775,#241776,
#241777,#241778,#241779,#241780,#241781,#241782,#241783,#241784,#241785,
#241786,#241787,#241788,#241789,#241790,#241791,#241792,#241793,#241794,
#241795,#241796,#241797,#241798,#241799,#241800,#241801,#241802,#241803,
#241804,#241805,#241806,#241807,#241808,#241809,#241810,#241811,#241812,
#241813,#241814,#241815,#241816,#241817,#241818,#241819,#241820,#241821,
#241822,#241823,#241824,#241825,#241826,#241827,#241828,#241829,#241830,
#241831,#241832,#241833,#241834,#241835,#241836,#241837,#241838,#241839,
#241840,#241841,#241842,#241843,#241844,#241845,#241846,#241847,#241848,
#241849,#241850,#241851,#241852,#241853,#241854,#241855,#241856),
 .UNSPECIFIED.,.F.,.F.,(4,3,3,3,3,3,3,3,3,3,3,3,3,3,3,3,3,3,3,3,3,3,3,3,
3,3,3,3,3,3,3,3,3,3,3,3,3,3,3,3,3,3,3,3,3,3,3,3,3,3,3,3,3,3,3,3,3,3,3,3,
3,3,3,3,3,3,3,3,3,3,3,3,3,4),(1492.25651045529,1492.33980475775,1492.42299730472,
1492.50610866675,1492.58915933873,1492.67217794586,1492.75518199317,1492.83818994494,
1492.92122026463,1493.00433983238,1493.08750804642,1493.1708018184,1493.22418940632,
1493.30792811817,1493.39156362953,1493.47511607293,1493.55860550878,1493.6420594594,
1493.72549595324,1493.808933063,1493.89238885792,1493.97593335065,1494.05952243359,
1494.14324570114,1494.22392541704,1494.30766412889,1494.39129964025,1494.47485208365,
1494.5583415195,1494.64179547012,1494.72523196396,1494.80866907372,1494.89212486864,
1494.97566936137,1495.05925844431,1495.14298171187,1495.22366142776,1495.30740013961,
1495.39103565097,1495.47458809437,1495.55807753022,1495.64153148084,1495.72496797468,
1495.80840508444,1495.89186087936,1495.97540537209,1496.05899445503,1496.14271772258,
1496.22339743848,1496.30713615033,1496.39077166169,1496.47432410509,1496.55781354094,
1496.64126749156,1496.7247039854,1496.80814109516,1496.89159689008,1496.9751413828,
1497.05873046575,1497.1424537333,1497.2231334492,1497.30687216105,1497.39050767241,
1497.47406011581,1497.55754955166,1497.64100350227,1497.72443999612,1497.80787710587,
1497.89133290079,1497.97487739352,1498.05846647646,1498.14218974402,1498.22286945992,
1498.28900992258),.UNSPECIFIED.);
#1821=B_SPLINE_CURVE_WITH_KNOTS('',3,(#241857,#241858,#241859,#241860,#241861,
#241862,#241863,#241864,#241865,#241866,#241867,#241868,#241869),
 .UNSPECIFIED.,.F.,.F.,(4,3,3,3,4),(1492.00484482495,1492.08845275128,1492.17218669413,
1492.2244533956,1492.25651045515),.UNSPECIFIED.);
#1822=B_SPLINE_CURVE_WITH_KNOTS('',3,(#241875,#241876,#241877,#241878,#241879,
#241880,#241881,#241882,#241883,#241884,#241885,#241886,#241887),
 .UNSPECIFIED.,.F.,.F.,(4,3,3,3,4),(1485.72166203219,1485.80528850285,1485.88903401518,
1485.91574671156,1485.97332514797),.UNSPECIFIED.);
#1823=B_SPLINE_CURVE_WITH_KNOTS('',3,(#241888,#241889,#241890,#241891,#241892,
#241893,#241894,#241895,#241896,#241897),.UNSPECIFIED.,.F.,.F.,(4,1,1,1,
1,1,1,4),(1485.97333225685,1486.91548272228,1487.915218733,1488.91495474372,
1489.91469075444,1490.91442676516,1491.91416277588,1492.00598701905),
 .UNSPECIFIED.);
#1824=B_SPLINE_CURVE_WITH_KNOTS('',3,(#241899,#241900,#241901,#241902,#241903,
#241904,#241905,#241906,#241907,#241908,#241909,#241910,#241911,#241912,
#241913,#241914,#241915,#241916,#241917,#241918,#241919,#241920,#241921,
#241922,#241923,#241924,#241925,#241926,#241927,#241928,#241929,#241930,
#241931,#241932,#241933,#241934,#241935,#241936,#241937,#241938,#241939,
#241940,#241941,#241942,#241943,#241944,#241945,#241946,#241947,#241948,
#241949,#241950,#241951,#241952,#241953,#241954,#241955,#241956,#241957,
#241958,#241959,#241960,#241961,#241962,#241963,#241964,#241965,#241966,
#241967,#241968,#241969,#241970,#241971,#241972,#241973,#241974,#241975,
#241976,#241977,#241978,#241979,#241980,#241981,#241982,#241983,#241984,
#241985,#241986,#241987,#241988,#241989,#241990,#241991,#241992,#241993,
#241994,#241995,#241996,#241997,#241998,#241999,#242000,#242001,#242002,
#242003,#242004,#242005,#242006,#242007,#242008,#242009,#242010,#242011,
#242012,#242013,#242014,#242015,#242016,#242017,#242018,#242019,#242020,
#242021,#242022,#242023,#242024,#242025,#242026,#242027,#242028,#242029,
#242030,#242031,#242032,#242033,#242034,#242035,#242036,#242037,#242038,
#242039,#242040,#242041,#242042,#242043,#242044,#242045,#242046,#242047,
#242048,#242049,#242050,#242051,#242052,#242053,#242054,#242055,#242056,
#242057,#242058,#242059,#242060,#242061,#242062,#242063,#242064,#242065,
#242066,#242067,#242068,#242069,#242070,#242071,#242072,#242073,#242074,
#242075,#242076,#242077,#242078,#242079,#242080,#242081,#242082,#242083,
#242084,#242085,#242086,#242087,#242088,#242089,#242090,#242091,#242092,
#242093,#242094,#242095,#242096,#242097,#242098,#242099,#242100,#242101,
#242102,#242103,#242104,#242105,#242106,#242107,#242108,#242109,#242110,
#242111,#242112,#242113,#242114,#242115,#242116,#242117,#242118),
 .UNSPECIFIED.,.F.,.F.,(4,3,3,3,3,3,3,3,3,3,3,3,3,3,3,3,3,3,3,3,3,3,3,3,
3,3,3,3,3,3,3,3,3,3,3,3,3,3,3,3,3,3,3,3,3,3,3,3,3,3,3,3,3,3,3,3,3,3,3,3,
3,3,3,3,3,3,3,3,3,3,3,3,3,4),(1485.97332514817,1486.08013280166,1486.18927155072,
1486.22603733128,1486.30977604313,1486.39341155449,1486.47696399789,1486.56045343374,
1486.64390738436,1486.7273438782,1486.81078098796,1486.89423678288,1486.97778127561,
1487.06137035855,1487.1450936261,1487.225773342,1487.30951205385,1487.39314756521,
1487.47670000861,1487.56018944446,1487.64364339508,1487.72707988892,1487.81051699868,
1487.8939727936,1487.97751728633,1488.06110636927,1488.14482963682,1488.22550935272,
1488.30924806457,1488.39288357593,1488.47643601933,1488.55992545518,1488.6433794058,
1488.72681589964,1488.8102530094,1488.89370880432,1488.97725329705,1489.06084237999,
1489.14456564755,1489.22524536344,1489.30898407529,1489.39261958665,1489.47617203005,
1489.5596614659,1489.64311541652,1489.72655191036,1489.80998902012,1489.89344481504,
1489.97698930776,1490.06057839071,1490.14430165826,1490.22498137416,1490.30872008601,
1490.39235559737,1490.47590804077,1490.55939747662,1490.64285142724,1490.72628792108,
1490.80972503084,1490.89318082576,1490.97672531848,1491.06031440143,1491.14403766898,
1491.22471738488,1491.30846947086,1491.39551639012,1491.47905786342,1491.56254230654,
1491.64598783891,1491.72941254974,1491.81285539563,1491.89630938701,1491.97981837138,
1492.00484482495),.UNSPECIFIED.);
#1825=B_SPLINE_CURVE_WITH_KNOTS('',3,(#242119,#242120,#242121,#242122,#242123,
#242124,#242125,#242126,#242127,#242128),.UNSPECIFIED.,.F.,.F.,(4,3,3,4),
(1485.72197536628,1485.80448560964,1485.8889053788,1485.97332514797),
 .UNSPECIFIED.);
#1826=B_SPLINE_CURVE_WITH_KNOTS('',3,(#242134,#242135,#242136,#242137,#242138,
#242139,#242140,#242141,#242142,#242143),.UNSPECIFIED.,.F.,.F.,(4,3,3,4),
(1479.43866858093,1479.52103553806,1479.60558768936,1479.69013984066),
 .UNSPECIFIED.);
#1827=B_SPLINE_CURVE_WITH_KNOTS('',3,(#242144,#242145,#242146,#242147,#242148,
#242149,#242150,#242151,#242152,#242153,#242154,#242155,#242156,#242157,
#242158,#242159,#242160,#242161,#242162,#242163,#242164,#242165,#242166,
#242167,#242168,#242169,#242170,#242171,#242172,#242173,#242174,#242175,
#242176,#242177,#242178,#242179,#242180,#242181,#242182,#242183,#242184,
#242185,#242186,#242187,#242188,#242189,#242190,#242191,#242192,#242193,
#242194,#242195,#242196,#242197,#242198,#242199,#242200,#242201,#242202,
#242203,#242204,#242205,#242206,#242207,#242208,#242209,#242210,#242211,
#242212,#242213,#242214,#242215,#242216,#242217,#242218,#242219,#242220,
#242221,#242222,#242223,#242224,#242225,#242226,#242227,#242228,#242229,
#242230,#242231,#242232,#242233,#242234,#242235,#242236,#242237,#242238,
#242239,#242240,#242241,#242242,#242243,#242244,#242245,#242246,#242247,
#242248,#242249,#242250,#242251,#242252,#242253,#242254,#242255,#242256,
#242257,#242258,#242259,#242260,#242261,#242262,#242263,#242264,#242265,
#242266,#242267,#242268,#242269,#242270,#242271,#242272,#242273,#242274,
#242275,#242276,#242277,#242278,#242279,#242280,#242281,#242282,#242283,
#242284,#242285,#242286,#242287,#242288,#242289,#242290,#242291,#242292,
#242293,#242294,#242295,#242296,#242297,#242298,#242299,#242300,#242301,
#242302,#242303,#242304,#242305,#242306,#242307,#242308,#242309,#242310,
#242311,#242312,#242313,#242314,#242315,#242316,#242317,#242318,#242319,
#242320,#242321,#242322,#242323,#242324,#242325,#242326,#242327,#242328,
#242329,#242330,#242331,#242332,#242333,#242334,#242335,#242336,#242337,
#242338,#242339,#242340,#242341,#242342,#242343,#242344,#242345,#242346,
#242347,#242348,#242349,#242350,#242351,#242352,#242353,#242354,#242355,
#242356,#242357,#242358,#242359,#242360),.UNSPECIFIED.,.F.,.F.,(4,3,3,3,
3,3,3,3,3,3,3,3,3,3,3,3,3,3,3,3,3,3,3,3,3,3,3,3,3,3,3,3,3,3,3,3,3,3,3,3,
3,3,3,3,3,3,3,3,3,3,3,3,3,3,3,3,3,3,3,3,3,3,3,3,3,3,3,3,3,3,3,3,4),(1479.69013984079,
1479.80373524402,1479.91733064724,1480.00106935909,1480.08470487045,1480.16825731385,
1480.2517467497,1480.33520070032,1480.41863719416,1480.50207430392,1480.58553009884,
1480.66907459157,1480.75266367451,1480.83638694206,1480.91706665796,1481.00080536981,
1481.08444088117,1481.16799332457,1481.25148276042,1481.33493671104,1481.41837320488,
1481.50181031464,1481.58526610956,1481.66881060229,1481.75239968523,1481.83612295279,
1481.91680266868,1482.00054138053,1482.08417689189,1482.16772933529,1482.25121877114,
1482.33467272176,1482.4181092156,1482.50154632536,1482.58500212028,1482.66854661301,
1482.75213569595,1482.8358589635,1482.9165386794,1483.00027739125,1483.08391290261,
1483.16746534601,1483.25095478186,1483.33440873248,1483.41784522632,1483.50128233608,
1483.584738131,1483.66828262373,1483.75187170667,1483.83559497422,1483.91627469012,
1484.00001340197,1484.08364891333,1484.16720135673,1484.25069079258,1484.33414474319,
1484.41758123704,1484.5010183468,1484.58447414171,1484.66801863444,1484.75160771738,
1484.83533098494,1484.91601070084,1484.99976112188,1485.08340578193,1485.16694939894,
1485.25043572519,1485.33388288075,1485.41730895535,1485.50075704418,1485.58421581109,
1485.66774035371,1485.72166203219),.UNSPECIFIED.);
#1828=B_SPLINE_CURVE_WITH_KNOTS('',3,(#242362,#242363,#242364,#242365,#242366,
#242367,#242368,#242369,#242370,#242371,#242372,#242373,#242374,#242375,
#242376,#242377,#242378,#242379,#242380,#242381,#242382,#242383,#242384,
#242385,#242386,#242387,#242388,#242389,#242390,#242391,#242392,#242393,
#242394,#242395,#242396,#242397,#242398,#242399,#242400,#242401,#242402,
#242403,#242404,#242405,#242406,#242407,#242408,#242409,#242410,#242411,
#242412,#242413,#242414,#242415,#242416,#242417,#242418,#242419,#242420,
#242421,#242422,#242423,#242424,#242425,#242426,#242427,#242428,#242429,
#242430,#242431,#242432,#242433,#242434,#242435,#242436,#242437,#242438,
#242439,#242440,#242441,#242442,#242443,#242444,#242445,#242446,#242447,
#242448,#242449,#242450,#242451,#242452,#242453,#242454,#242455,#242456,
#242457,#242458,#242459,#242460,#242461,#242462,#242463,#242464,#242465,
#242466,#242467,#242468,#242469,#242470,#242471,#242472,#242473,#242474,
#242475,#242476,#242477,#242478,#242479,#242480,#242481,#242482,#242483,
#242484,#242485,#242486,#242487,#242488,#242489,#242490,#242491,#242492,
#242493,#242494,#242495,#242496,#242497,#242498,#242499,#242500,#242501,
#242502,#242503,#242504,#242505,#242506,#242507,#242508,#242509,#242510,
#242511,#242512,#242513,#242514,#242515,#242516,#242517,#242518,#242519,
#242520,#242521,#242522,#242523,#242524,#242525,#242526,#242527,#242528,
#242529,#242530,#242531,#242532,#242533,#242534,#242535,#242536,#242537,
#242538,#242539,#242540,#242541,#242542,#242543,#242544,#242545,#242546,
#242547,#242548,#242549,#242550,#242551,#242552,#242553,#242554,#242555,
#242556,#242557,#242558,#242559,#242560,#242561,#242562,#242563,#242564,
#242565,#242566,#242567,#242568,#242569,#242570,#242571,#242572,#242573,
#242574,#242575,#242576,#242577,#242578,#242579,#242580,#242581),
 .UNSPECIFIED.,.F.,.F.,(4,3,3,3,3,3,3,3,3,3,3,3,3,3,3,3,3,3,3,3,3,3,3,3,
3,3,3,3,3,3,3,3,3,3,3,3,3,3,3,3,3,3,3,3,3,3,3,3,3,3,3,3,3,3,3,3,3,3,3,3,
3,3,3,3,3,3,3,3,3,3,3,3,3,4),(1479.69013984079,1479.77630058833,1479.86253318071,
1479.94885023975,1480.03532621794,1480.1218940574,1480.20861921668,1480.22762126696,
1480.31135997881,1480.39499549017,1480.47854793357,1480.56203736942,1480.64549132004,
1480.72892781388,1480.81236492364,1480.89582071856,1480.97936521129,1481.06295429423,
1481.14667756178,1481.22735727768,1481.31109598953,1481.39473150089,1481.47828394429,
1481.56177338014,1481.64522733076,1481.7286638246,1481.81210093436,1481.89555672928,
1481.97910122201,1482.06269030495,1482.1464135725,1482.2270932884,1482.31083200025,
1482.39446751161,1482.47801995501,1482.56150939086,1482.64496334148,1482.72839983532,
1482.81183694508,1482.89529274,1482.97883723273,1483.06242631567,1483.14614958322,
1483.22682929912,1483.31056801097,1483.39420352233,1483.47775596573,1483.56124540158,
1483.6446993522,1483.72813584604,1483.8115729558,1483.89502875072,1483.97857324344,
1484.06216232639,1484.14588559394,1484.22656530984,1484.31030402169,1484.39393953305,
1484.47749197645,1484.5609814123,1484.64443536292,1484.72787185676,1484.81130896652,
1484.89476476144,1484.97830925417,1485.06189833711,1485.14562160467,1485.22630132056,
1485.3090888973,1485.39177806216,1485.47437529998,1485.5569182117,1485.63944678899,
1485.72197536628),.UNSPECIFIED.);
#1829=B_SPLINE_CURVE_WITH_KNOTS('',3,(#242582,#242583,#242584,#242585,#242586,
#242587,#242588,#242589,#242590,#242591),.UNSPECIFIED.,.F.,.F.,(4,3,3,4),
(1479.43983851051,1479.52903735213,1479.61799758571,1479.69013984063),
 .UNSPECIFIED.);
#1830=B_SPLINE_CURVE_WITH_KNOTS('',3,(#242597,#242598,#242599,#242600,#242601,
#242602,#242603,#242604,#242605,#242606),.UNSPECIFIED.,.F.,.F.,(4,3,3,4),
(1473.15664071279,1473.24472264985,1473.3326204829,1473.40695453349),
 .UNSPECIFIED.);
#1831=B_SPLINE_CURVE_WITH_KNOTS('',3,(#242607,#242608,#242609,#242610,#242611,
#242612,#242613,#242614,#242615,#242616,#242617,#242618,#242619,#242620,
#242621,#242622,#242623,#242624,#242625,#242626,#242627,#242628,#242629,
#242630,#242631,#242632,#242633,#242634,#242635,#242636,#242637,#242638,
#242639,#242640,#242641,#242642,#242643,#242644,#242645,#242646,#242647,
#242648,#242649,#242650,#242651,#242652,#242653,#242654,#242655,#242656,
#242657,#242658,#242659,#242660,#242661,#242662,#242663,#242664,#242665,
#242666,#242667,#242668,#242669,#242670,#242671,#242672,#242673,#242674,
#242675,#242676,#242677,#242678,#242679,#242680,#242681,#242682,#242683,
#242684,#242685,#242686,#242687,#242688,#242689,#242690,#242691,#242692,
#242693,#242694,#242695,#242696,#242697,#242698,#242699,#242700,#242701,
#242702,#242703,#242704,#242705,#242706,#242707,#242708,#242709,#242710,
#242711,#242712,#242713,#242714,#242715,#242716,#242717,#242718,#242719,
#242720,#242721,#242722,#242723,#242724,#242725,#242726,#242727,#242728,
#242729,#242730,#242731,#242732,#242733,#242734,#242735,#242736,#242737,
#242738,#242739,#242740,#242741,#242742,#242743,#242744,#242745,#242746,
#242747,#242748,#242749,#242750,#242751,#242752,#242753,#242754,#242755,
#242756,#242757,#242758,#242759,#242760,#242761,#242762,#242763,#242764,
#242765,#242766,#242767,#242768,#242769,#242770,#242771,#242772,#242773,
#242774,#242775,#242776,#242777,#242778,#242779,#242780,#242781,#242782,
#242783,#242784,#242785,#242786,#242787,#242788,#242789,#242790,#242791,
#242792,#242793,#242794,#242795,#242796,#242797,#242798,#242799,#242800,
#242801,#242802,#242803,#242804,#242805,#242806,#242807,#242808,#242809,
#242810,#242811,#242812,#242813,#242814,#242815,#242816,#242817,#242818,
#242819,#242820,#242821,#242822,#242823,#242824,#242825,#242826),
 .UNSPECIFIED.,.F.,.F.,(4,3,3,3,3,3,3,3,3,3,3,3,3,3,3,3,3,3,3,3,3,3,3,3,
3,3,3,3,3,3,3,3,3,3,3,3,3,3,3,3,3,3,3,3,3,3,3,3,3,3,3,3,3,3,3,3,3,3,3,3,
3,3,3,3,3,3,3,3,3,3,3,3,3,4),(1473.40695453361,1473.49393313965,1473.5810114473,
1473.66828127154,1473.75565011186,1473.8432173964,1473.91891458292,1474.00265329477,
1474.08628880613,1474.16984124953,1474.25333068538,1474.336784636,1474.42022112984,
1474.5036582396,1474.58711403452,1474.67065852724,1474.75424761019,1474.83797087774,
1474.91865059364,1475.00238930549,1475.08602481685,1475.16957726025,1475.2530666961,
1475.33652064672,1475.41995714056,1475.50339425032,1475.58685004524,1475.67039453797,
1475.75398362091,1475.83770688847,1475.91838660436,1476.00212531621,1476.08576082757,
1476.16931327097,1476.25280270682,1476.33625665744,1476.41969315128,1476.50313026104,
1476.58658605596,1476.67013054869,1476.75371963163,1476.83744289918,1476.91812261508,
1477.00186132693,1477.08549683829,1477.16904928169,1477.25253871754,1477.33599266816,
1477.419429162,1477.50286627176,1477.58632206667,1477.6698665594,1477.75345564234,
1477.8371789099,1477.9178586258,1478.00159733765,1478.08523284901,1478.16878529241,
1478.25227472826,1478.33572867888,1478.41916517272,1478.50260228248,1478.5860580774,
1478.66960257013,1478.75319165307,1478.83691492063,1478.91759463652,1479.00021914845,
1479.08274652633,1479.16519590404,1479.24758186863,1479.32993154163,1479.41227038175,
1479.43866858093),.UNSPECIFIED.);
#1832=B_SPLINE_CURVE_WITH_KNOTS('',3,(#242828,#242829,#242830,#242831,#242832,
#242833,#242834,#242835,#242836,#242837,#242838,#242839,#242840,#242841,
#242842,#242843,#242844,#242845,#242846,#242847,#242848,#242849,#242850,
#242851,#242852,#242853,#242854,#242855,#242856,#242857,#242858,#242859,
#242860,#242861,#242862,#242863,#242864,#242865,#242866,#242867,#242868,
#242869,#242870,#242871,#242872,#242873,#242874,#242875,#242876,#242877,
#242878,#242879,#242880,#242881,#242882,#242883,#242884,#242885,#242886,
#242887,#242888,#242889,#242890,#242891,#242892,#242893,#242894,#242895,
#242896,#242897,#242898,#242899,#242900,#242901,#242902,#242903,#242904,
#242905,#242906,#242907,#242908,#242909,#242910,#242911,#242912,#242913,
#242914,#242915,#242916,#242917,#242918,#242919,#242920,#242921,#242922,
#242923,#242924,#242925,#242926,#242927,#242928,#242929,#242930,#242931,
#242932,#242933,#242934,#242935,#242936,#242937,#242938,#242939,#242940,
#242941,#242942,#242943,#242944,#242945,#242946,#242947,#242948,#242949,
#242950,#242951,#242952,#242953,#242954,#242955,#242956,#242957,#242958,
#242959,#242960,#242961,#242962,#242963,#242964,#242965,#242966,#242967,
#242968,#242969,#242970,#242971,#242972,#242973,#242974,#242975,#242976,
#242977,#242978,#242979,#242980,#242981,#242982,#242983,#242984,#242985,
#242986,#242987,#242988,#242989,#242990,#242991,#242992,#242993,#242994,
#242995,#242996,#242997,#242998,#242999,#243000,#243001,#243002,#243003,
#243004,#243005,#243006,#243007,#243008,#243009,#243010,#243011,#243012,
#243013,#243014,#243015,#243016,#243017,#243018,#243019,#243020,#243021,
#243022,#243023,#243024,#243025,#243026,#243027,#243028,#243029,#243030,
#243031,#243032,#243033,#243034,#243035,#243036,#243037,#243038,#243039,
#243040,#243041,#243042,#243043,#243044,#243045,#243046,#243047),
 .UNSPECIFIED.,.F.,.F.,(4,3,3,3,3,3,3,3,3,3,3,3,3,3,3,3,3,3,3,3,3,3,3,3,
3,3,3,3,3,3,3,3,3,3,3,3,3,3,3,3,3,3,3,3,3,3,3,3,3,3,3,3,3,3,3,3,3,3,3,3,
3,3,3,3,3,3,3,3,3,3,3,3,3,4),(1473.40695453377,1473.4893182278,1473.57160671137,
1473.65384440038,1473.73605555324,1473.81825920997,1473.90047440225,1473.98277068985,
1474.06510696983,1474.14757432633,1474.22920520264,1474.31294391449,1474.39657942585,
1474.48013186925,1474.5636213051,1474.64707525572,1474.73051174956,1474.81394885932,
1474.89740465424,1474.98094914697,1475.06453822991,1475.14826149746,1475.22894121336,
1475.31267992521,1475.39631543657,1475.47986787997,1475.56335731582,1475.64681126644,
1475.73024776028,1475.81368487004,1475.89714066496,1475.98068515769,1476.06427424063,
1476.14799750818,1476.22867722408,1476.31241593593,1476.39605144729,1476.47960389069,
1476.56309332654,1476.64654727716,1476.729983771,1476.81342088076,1476.89687667568,
1476.98042116841,1477.06401025135,1477.1477335189,1477.2284132348,1477.31215194665,
1477.39578745801,1477.47933990141,1477.56282933726,1477.64628328788,1477.72971978172,
1477.81315689148,1477.8966126864,1477.98015717913,1478.06374626207,1478.14746952962,
1478.22814924552,1478.31188795737,1478.39552346873,1478.47907591213,1478.56256534798,
1478.6460192986,1478.72945579244,1478.8128929022,1478.89634869712,1478.97989318985,
1479.06348227279,1479.14720554034,1479.22788525624,1479.31758500425,1479.40706476103,
1479.43983851051),.UNSPECIFIED.);
#1833=B_SPLINE_CURVE_WITH_KNOTS('',3,(#243048,#243049,#243050,#243051,#243052,
#243053,#243054,#243055,#243056,#243057),.UNSPECIFIED.,.F.,.F.,(4,3,3,4),
(1473.15552466501,1473.22946919192,1473.35769273628,1473.40695453361),
 .UNSPECIFIED.);
#1834=B_SPLINE_CURVE_WITH_KNOTS('',3,(#243063,#243064,#243065,#243066,#243067,
#243068,#243069,#243070,#243071,#243072),.UNSPECIFIED.,.F.,.F.,(4,3,3,4),
(1466.87244437141,1466.92076250788,1467.04006077289,1467.12376922643),
 .UNSPECIFIED.);
#1835=B_SPLINE_CURVE_WITH_KNOTS('',3,(#243073,#243074,#243075,#243076,#243077,
#243078,#243079,#243080,#243081,#243082,#243083,#243084,#243085,#243086,
#243087,#243088,#243089,#243090,#243091,#243092,#243093,#243094,#243095,
#243096,#243097,#243098,#243099,#243100,#243101,#243102,#243103,#243104,
#243105,#243106,#243107,#243108,#243109,#243110,#243111,#243112,#243113,
#243114,#243115,#243116,#243117,#243118,#243119,#243120,#243121,#243122,
#243123,#243124,#243125,#243126,#243127,#243128,#243129,#243130,#243131,
#243132,#243133,#243134,#243135,#243136,#243137,#243138,#243139,#243140,
#243141,#243142,#243143,#243144,#243145,#243146,#243147,#243148,#243149,
#243150,#243151,#243152,#243153,#243154,#243155,#243156,#243157,#243158,
#243159,#243160,#243161,#243162,#243163,#243164,#243165,#243166,#243167,
#243168,#243169,#243170,#243171,#243172,#243173,#243174,#243175,#243176,
#243177,#243178,#243179,#243180,#243181,#243182,#243183,#243184,#243185,
#243186,#243187,#243188,#243189,#243190,#243191,#243192,#243193,#243194,
#243195,#243196,#243197,#243198,#243199,#243200,#243201,#243202,#243203,
#243204,#243205,#243206,#243207,#243208,#243209,#243210,#243211,#243212,
#243213,#243214,#243215,#243216,#243217,#243218,#243219,#243220,#243221,
#243222,#243223,#243224,#243225,#243226,#243227,#243228,#243229,#243230,
#243231,#243232,#243233,#243234,#243235,#243236,#243237,#243238,#243239,
#243240,#243241,#243242,#243243,#243244,#243245,#243246,#243247,#243248,
#243249,#243250,#243251,#243252,#243253,#243254,#243255,#243256,#243257,
#243258,#243259,#243260,#243261,#243262,#243263,#243264,#243265,#243266,
#243267,#243268,#243269,#243270,#243271,#243272,#243273,#243274,#243275,
#243276,#243277,#243278,#243279,#243280,#243281,#243282,#243283,#243284,
#243285,#243286,#243287,#243288,#243289,#243290,#243291,#243292),
 .UNSPECIFIED.,.F.,.F.,(4,3,3,3,3,3,3,3,3,3,3,3,3,3,3,3,3,3,3,3,3,3,3,3,
3,3,3,3,3,3,3,3,3,3,3,3,3,3,3,3,3,3,3,3,3,3,3,3,3,3,3,3,3,3,3,3,3,3,3,3,
3,3,3,3,3,3,3,3,3,3,3,3,3,4),(1467.12376922661,1467.20615137202,1467.28846542945,
1467.37073818782,1467.45299077312,1467.53524219248,1467.61751144987,1467.69986534415,
1467.78226484149,1467.86478835703,1467.9204985186,1468.00423723045,1468.08787274181,
1468.17142518521,1468.25491462106,1468.33836857168,1468.42180506552,1468.50524217528,
1468.5886979702,1468.67224246292,1468.75583154587,1468.83955481342,1468.92023452932,
1469.00397324117,1469.08760875253,1469.17116119593,1469.25465063178,1469.3381045824,
1469.42154107624,1469.504978186,1469.58843398092,1469.67197847365,1469.75556755659,
1469.83929082415,1469.91997054004,1470.00370925189,1470.08734476325,1470.17089720665,
1470.2543866425,1470.33784059312,1470.42127708696,1470.50471419672,1470.58816999164,
1470.67171448437,1470.75530356731,1470.83902683487,1470.91970655076,1471.00344526261,
1471.08708077397,1471.17063321737,1471.25412265322,1471.33757660384,1471.42101309768,
1471.50445020744,1471.58790600235,1471.67145049508,1471.75503957802,1471.83876284558,
1471.91944256148,1472.00318127333,1472.08681678469,1472.17036922809,1472.25385866394,
1472.33731261456,1472.4207491084,1472.50418621816,1472.58764201308,1472.67118650581,
1472.75477558875,1472.83849885631,1472.9191785722,1473.00772889966,1473.09607576719,
1473.15664071279),.UNSPECIFIED.);
#1836=B_SPLINE_CURVE_WITH_KNOTS('',3,(#243294,#243295,#243296,#243297,#243298,
#243299,#243300,#243301,#243302,#243303,#243304,#243305,#243306,#243307,
#243308,#243309,#243310,#243311,#243312,#243313,#243314,#243315,#243316,
#243317,#243318,#243319,#243320,#243321,#243322,#243323,#243324,#243325,
#243326,#243327,#243328,#243329,#243330,#243331,#243332,#243333,#243334,
#243335,#243336,#243337,#243338,#243339,#243340,#243341,#243342,#243343,
#243344,#243345,#243346,#243347,#243348,#243349,#243350,#243351,#243352,
#243353,#243354,#243355,#243356,#243357,#243358,#243359,#243360,#243361,
#243362,#243363,#243364,#243365,#243366,#243367,#243368,#243369,#243370,
#243371,#243372,#243373,#243374,#243375,#243376,#243377,#243378,#243379,
#243380,#243381,#243382,#243383,#243384,#243385,#243386,#243387,#243388,
#243389,#243390,#243391,#243392,#243393,#243394,#243395,#243396,#243397,
#243398,#243399,#243400,#243401,#243402,#243403,#243404,#243405,#243406,
#243407,#243408,#243409,#243410,#243411,#243412,#243413,#243414,#243415,
#243416,#243417,#243418,#243419,#243420,#243421,#243422,#243423,#243424,
#243425,#243426,#243427,#243428,#243429,#243430,#243431,#243432,#243433,
#243434,#243435,#243436,#243437,#243438,#243439,#243440,#243441,#243442,
#243443,#243444,#243445,#243446,#243447,#243448,#243449,#243450,#243451,
#243452,#243453,#243454,#243455,#243456,#243457,#243458,#243459,#243460,
#243461,#243462,#243463,#243464,#243465,#243466,#243467,#243468,#243469,
#243470,#243471,#243472,#243473,#243474,#243475,#243476,#243477,#243478,
#243479,#243480,#243481,#243482,#243483,#243484,#243485,#243486,#243487,
#243488,#243489,#243490,#243491,#243492,#243493,#243494,#243495,#243496,
#243497,#243498,#243499,#243500,#243501,#243502,#243503,#243504,#243505,
#243506,#243507,#243508,#243509,#243510),.UNSPECIFIED.,.F.,.F.,(4,3,3,3,
3,3,3,3,3,3,3,3,3,3,3,3,3,3,3,3,3,3,3,3,3,3,3,3,3,3,3,3,3,3,3,3,3,3,3,3,
3,3,3,3,3,3,3,3,3,3,3,3,3,3,3,3,3,3,3,3,3,3,3,3,3,3,3,3,3,3,3,3,4),(1467.12376922643,
1467.2310531276,1467.31479183945,1467.39842735081,1467.48197979421,1467.56546923006,
1467.64892318068,1467.73235967452,1467.81579678428,1467.8992525792,1467.98279707193,
1468.06638615487,1468.15010942242,1468.23078913832,1468.31452785017,1468.39816336153,
1468.48171580493,1468.56520524078,1468.6486591914,1468.73209568524,1468.815532795,
1468.89898858992,1468.98253308265,1469.06612216559,1469.14984543314,1469.23052514904,
1469.31426386089,1469.39789937225,1469.48145181565,1469.5649412515,1469.64839520212,
1469.73183169596,1469.81526880572,1469.89872460064,1469.98226909337,1470.06585817631,
1470.14958144386,1470.23026115976,1470.31399987161,1470.39763538297,1470.48118782637,
1470.56467726222,1470.64813121284,1470.73156770668,1470.81500481644,1470.89846061136,
1470.98200510409,1471.06559418703,1471.14931745458,1471.22999717048,1471.31373588233,
1471.39737139369,1471.48092383709,1471.56441327294,1471.64786722356,1471.7313037174,
1471.81474082716,1471.89819662208,1471.98174111481,1472.06533019775,1472.1490534653,
1472.2297331812,1472.31347615588,1472.39711495474,1472.48066971443,1472.56502658325,
1472.64847685927,1472.73190848728,1472.81533953906,1472.90038582054,1472.98390578302,
1473.06971522401,1473.15552466501),.UNSPECIFIED.);
#1837=B_SPLINE_CURVE_WITH_KNOTS('',3,(#243511,#243512,#243513,#243514,#243515,
#243516,#243517,#243518,#243519,#243520),.UNSPECIFIED.,.F.,.F.,(4,3,3,4),
(1466.8719408414,1466.9543981102,1467.03908366825,1467.12376922629),
 .UNSPECIFIED.);
#1838=B_SPLINE_CURVE_WITH_KNOTS('',3,(#243526,#243527,#243528,#243529,#243530,
#243531,#243532,#243533,#243534,#243535),.UNSPECIFIED.,.F.,.F.,(4,3,3,4),
(1460.5887469457,1460.67138214754,1460.75598303333,1460.84058391912),
 .UNSPECIFIED.);
#1839=B_SPLINE_CURVE_WITH_KNOTS('',3,(#243536,#243537,#243538,#243539,#243540,
#243541,#243542,#243543,#243544,#243545,#243546,#243547,#243548,#243549,
#243550,#243551,#243552,#243553,#243554,#243555,#243556,#243557,#243558,
#243559,#243560,#243561,#243562,#243563,#243564,#243565,#243566,#243567,
#243568,#243569,#243570,#243571,#243572,#243573,#243574,#243575,#243576,
#243577,#243578,#243579,#243580,#243581,#243582,#243583,#243584,#243585,
#243586,#243587,#243588,#243589,#243590,#243591,#243592,#243593,#243594,
#243595,#243596,#243597,#243598,#243599,#243600,#243601,#243602,#243603,
#243604,#243605,#243606,#243607,#243608,#243609,#243610,#243611,#243612,
#243613,#243614,#243615,#243616,#243617,#243618,#243619,#243620,#243621,
#243622,#243623,#243624,#243625,#243626,#243627,#243628,#243629,#243630,
#243631,#243632,#243633,#243634,#243635,#243636,#243637,#243638,#243639,
#243640,#243641,#243642,#243643,#243644,#243645,#243646,#243647,#243648,
#243649,#243650,#243651,#243652,#243653,#243654,#243655,#243656,#243657,
#243658,#243659,#243660,#243661,#243662,#243663,#243664,#243665,#243666,
#243667,#243668,#243669,#243670,#243671,#243672,#243673,#243674,#243675,
#243676,#243677,#243678,#243679,#243680,#243681,#243682,#243683,#243684,
#243685,#243686,#243687,#243688,#243689,#243690,#243691,#243692,#243693,
#243694,#243695,#243696,#243697,#243698,#243699,#243700,#243701,#243702,
#243703,#243704,#243705,#243706,#243707,#243708,#243709,#243710,#243711,
#243712,#243713,#243714,#243715,#243716,#243717,#243718,#243719,#243720,
#243721,#243722,#243723,#243724,#243725,#243726,#243727,#243728,#243729,
#243730,#243731,#243732,#243733,#243734,#243735,#243736,#243737,#243738,
#243739,#243740,#243741,#243742,#243743,#243744,#243745,#243746,#243747,
#243748,#243749,#243750,#243751,#243752,#243753,#243754,#243755),
 .UNSPECIFIED.,.F.,.F.,(4,3,3,3,3,3,3,3,3,3,3,3,3,3,3,3,3,3,3,3,3,3,3,3,
3,3,3,3,3,3,3,3,3,3,3,3,3,3,3,3,3,3,3,3,3,3,3,3,3,3,3,3,3,3,3,3,3,3,3,3,
3,3,3,3,3,3,3,3,3,3,3,3,3,4),(1460.84058391925,1460.92234644356,1461.00608515541,
1461.08972066677,1461.17327311017,1461.25676254602,1461.34021649664,1461.42365299048,
1461.50709010024,1461.59054589516,1461.67409038789,1461.75767947083,1461.84140273838,
1461.92208245428,1462.00582116613,1462.08945667749,1462.17300912089,1462.25649855674,
1462.33995250736,1462.4233890012,1462.50682611096,1462.59028190588,1462.67382639861,
1462.75741548155,1462.84113874911,1462.921818465,1463.00555717685,1463.08919268821,
1463.17274513161,1463.25623456746,1463.33968851808,1463.42312501192,1463.50656212168,
1463.5900179166,1463.67356240933,1463.75715149227,1463.84087475982,1463.92155447572,
1464.00529318757,1464.08892869893,1464.17248114233,1464.25597057818,1464.3394245288,
1464.42286102264,1464.5062981324,1464.58975392732,1464.67329842005,1464.75688750299,
1464.84061077054,1464.92129048644,1465.00502919829,1465.08866470965,1465.17221715305,
1465.2557065889,1465.33916053952,1465.42259703336,1465.50603414312,1465.58948993803,
1465.67303443076,1465.7566235137,1465.84034678126,1465.92102649716,1466.00476796687,
1466.08840559879,1466.17195952814,1466.25952013355,1466.34297044609,1466.42640328248,
1466.50983671436,1466.59328880972,1466.67681791279,1466.76039202568,1466.84407147563,
1466.87244437141),.UNSPECIFIED.);
#1840=B_SPLINE_CURVE_WITH_KNOTS('',3,(#243757,#243758,#243759,#243760,#243761,
#243762,#243763,#243764,#243765,#243766,#243767,#243768,#243769,#243770,
#243771,#243772,#243773,#243774,#243775,#243776,#243777,#243778,#243779,
#243780,#243781,#243782,#243783,#243784,#243785,#243786,#243787,#243788,
#243789,#243790,#243791,#243792,#243793,#243794,#243795,#243796,#243797,
#243798,#243799,#243800,#243801,#243802,#243803,#243804,#243805,#243806,
#243807,#243808,#243809,#243810,#243811,#243812,#243813,#243814,#243815,
#243816,#243817,#243818,#243819,#243820,#243821,#243822,#243823,#243824,
#243825,#243826,#243827,#243828,#243829,#243830,#243831,#243832,#243833,
#243834,#243835,#243836,#243837,#243838,#243839,#243840,#243841,#243842,
#243843,#243844,#243845,#243846,#243847,#243848,#243849,#243850,#243851,
#243852,#243853,#243854,#243855,#243856,#243857,#243858,#243859,#243860,
#243861,#243862,#243863,#243864,#243865,#243866,#243867,#243868,#243869,
#243870,#243871,#243872,#243873,#243874,#243875,#243876,#243877,#243878,
#243879,#243880,#243881,#243882,#243883,#243884,#243885,#243886,#243887,
#243888,#243889,#243890,#243891,#243892,#243893,#243894,#243895,#243896,
#243897,#243898,#243899,#243900,#243901,#243902,#243903,#243904,#243905,
#243906,#243907,#243908,#243909,#243910,#243911,#243912,#243913,#243914,
#243915,#243916,#243917,#243918,#243919,#243920,#243921,#243922,#243923,
#243924,#243925,#243926,#243927,#243928,#243929,#243930,#243931,#243932,
#243933,#243934,#243935,#243936,#243937,#243938,#243939,#243940,#243941,
#243942,#243943,#243944,#243945,#243946,#243947,#243948,#243949,#243950,
#243951,#243952,#243953,#243954,#243955,#243956,#243957,#243958,#243959,
#243960,#243961,#243962,#243963,#243964,#243965,#243966,#243967,#243968,
#243969,#243970,#243971,#243972,#243973,#243974,#243975,#243976),
 .UNSPECIFIED.,.F.,.F.,(4,3,3,3,3,3,3,3,3,3,3,3,3,3,3,3,3,3,3,3,3,3,3,3,
3,3,3,3,3,3,3,3,3,3,3,3,3,3,3,3,3,3,3,3,3,3,3,3,3,3,3,3,3,3,3,3,3,3,3,3,
3,3,3,3,3,3,3,3,3,3,3,3,3,4),(1460.84058391944,1460.93315405195,1461.02625537987,
1461.11963264212,1461.21335570444,1461.23263706328,1461.31637577513,1461.40001128649,
1461.48356372989,1461.56705316574,1461.65050711636,1461.7339436102,1461.81738071996,
1461.90083651488,1461.98438100761,1462.06797009055,1462.1516933581,1462.232373074,
1462.31611178585,1462.39974729721,1462.48329974061,1462.56678917646,1462.65024312708,
1462.73367962092,1462.81711673068,1462.9005725256,1462.98411701832,1463.06770610127,
1463.15142936882,1463.23210908472,1463.31584779657,1463.39948330793,1463.48303575133,
1463.56652518718,1463.6499791378,1463.73341563164,1463.8168527414,1463.90030853632,
1463.98385302905,1464.06744211199,1464.15116537954,1464.23184509544,1464.31558380729,
1464.39921931865,1464.48277176205,1464.5662611979,1464.64971514852,1464.73315164236,
1464.81658875212,1464.90004454704,1464.98358903977,1465.06717812271,1465.15090139026,
1465.23158110616,1465.31531981801,1465.39895532937,1465.48250777277,1465.56599720862,
1465.64945115924,1465.73288765308,1465.81632476284,1465.89978055776,1465.98332505049,
1466.06691413343,1466.15063740098,1466.23131711688,1466.31394700638,1466.39648229565,
1466.47894209376,1466.56134544058,1466.64372069725,1466.72607768958,1466.80846141686,
1466.8719408414),.UNSPECIFIED.);
#1841=B_SPLINE_CURVE_WITH_KNOTS('',3,(#243977,#243978,#243979,#243980,#243981,
#243982,#243983,#243984,#243985,#243986),.UNSPECIFIED.,.F.,.F.,(4,3,3,4),
(1460.58993146501,1460.67436365968,1460.75876766208,1460.84058391925),
 .UNSPECIFIED.);
#1842=B_SPLINE_CURVE_WITH_KNOTS('',3,(#243992,#243993,#243994,#243995,#243996,
#243997,#243998,#243999,#244000,#244001),.UNSPECIFIED.,.F.,.F.,(4,3,3,4),
(1454.30662927058,1454.3905507352,1454.47446510851,1454.55739861207),
 .UNSPECIFIED.);
#1843=B_SPLINE_CURVE_WITH_KNOTS('',3,(#244002,#244003,#244004,#244005,#244006,
#244007,#244008,#244009,#244010,#244011,#244012,#244013,#244014,#244015,
#244016,#244017,#244018,#244019,#244020,#244021,#244022,#244023,#244024,
#244025,#244026,#244027,#244028,#244029,#244030,#244031,#244032,#244033,
#244034,#244035,#244036,#244037,#244038,#244039,#244040,#244041,#244042,
#244043,#244044,#244045,#244046,#244047,#244048,#244049,#244050,#244051,
#244052,#244053,#244054,#244055,#244056,#244057,#244058,#244059,#244060,
#244061,#244062,#244063,#244064,#244065,#244066,#244067,#244068,#244069,
#244070,#244071,#244072,#244073,#244074,#244075,#244076,#244077,#244078,
#244079,#244080,#244081,#244082,#244083,#244084,#244085,#244086,#244087,
#244088,#244089,#244090,#244091,#244092,#244093,#244094,#244095,#244096,
#244097,#244098,#244099,#244100,#244101,#244102,#244103,#244104,#244105,
#244106,#244107,#244108,#244109,#244110,#244111,#244112,#244113,#244114,
#244115,#244116,#244117,#244118,#244119,#244120,#244121,#244122,#244123,
#244124,#244125,#244126,#244127,#244128,#244129,#244130,#244131,#244132,
#244133,#244134,#244135,#244136,#244137,#244138,#244139,#244140,#244141,
#244142,#244143,#244144,#244145,#244146,#244147,#244148,#244149,#244150,
#244151,#244152,#244153,#244154,#244155,#244156,#244157,#244158,#244159,
#244160,#244161,#244162,#244163,#244164,#244165,#244166,#244167,#244168,
#244169,#244170,#244171,#244172,#244173,#244174,#244175,#244176,#244177,
#244178,#244179,#244180,#244181,#244182,#244183,#244184,#244185,#244186,
#244187,#244188,#244189,#244190,#244191,#244192,#244193,#244194,#244195,
#244196,#244197,#244198,#244199,#244200,#244201,#244202,#244203,#244204,
#244205,#244206,#244207,#244208,#244209,#244210,#244211,#244212,#244213,
#244214,#244215,#244216,#244217,#244218),.UNSPECIFIED.,.F.,.F.,(4,3,3,3,
3,3,3,3,3,3,3,3,3,3,3,3,3,3,3,3,3,3,3,3,3,3,3,3,3,3,3,3,3,3,3,3,3,3,3,3,
3,3,3,3,3,3,3,3,3,3,3,3,3,3,3,3,3,3,3,3,3,3,3,3,3,3,3,3,3,3,3,3,4),(1454.55739861227,
1454.65194746431,1454.74689204477,1454.84238116431,1454.92393037924,1455.00766909109,
1455.09130460245,1455.17485704585,1455.2583464817,1455.34180043232,1455.42523692616,
1455.50867403592,1455.59212983084,1455.67567432356,1455.75926340651,1455.84298667406,
1455.92366638996,1456.00740510181,1456.09104061317,1456.17459305657,1456.25808249242,
1456.34153644304,1456.42497293688,1456.50841004664,1456.59186584156,1456.67541033429,
1456.75899941723,1456.84272268479,1456.92340240068,1457.00714111253,1457.09077662389,
1457.17432906729,1457.25781850314,1457.34127245376,1457.4247089476,1457.50814605736,
1457.59160185228,1457.67514634501,1457.75873542795,1457.8424586955,1457.9231384114,
1458.00687712325,1458.09051263461,1458.17406507801,1458.25755451386,1458.34100846448,
1458.42444495832,1458.50788206808,1458.591337863,1458.67488235572,1458.75847143867,
1458.84219470622,1458.92287442212,1459.00661313397,1459.09024864533,1459.17380108873,
1459.25729052458,1459.3407444752,1459.42418096904,1459.5076180788,1459.59107387372,
1459.67461836645,1459.75820744939,1459.84193071695,1459.92261043284,1460.00587749695,
1460.08857547718,1460.17119802281,1460.25376406267,1460.33750978343,1460.4200311627,
1460.5043890542,1460.5887469457),.UNSPECIFIED.);
#1844=B_SPLINE_CURVE_WITH_KNOTS('',3,(#244220,#244221,#244222,#244223,#244224,
#244225,#244226,#244227,#244228,#244229,#244230,#244231,#244232,#244233,
#244234,#244235,#244236,#244237,#244238,#244239,#244240,#244241,#244242,
#244243,#244244,#244245,#244246,#244247,#244248,#244249,#244250,#244251,
#244252,#244253,#244254,#244255,#244256,#244257,#244258,#244259,#244260,
#244261,#244262,#244263,#244264,#244265,#244266,#244267,#244268,#244269,
#244270,#244271,#244272,#244273,#244274,#244275,#244276,#244277,#244278,
#244279,#244280,#244281,#244282,#244283,#244284,#244285,#244286,#244287,
#244288,#244289,#244290,#244291,#244292,#244293,#244294,#244295,#244296,
#244297,#244298,#244299,#244300,#244301,#244302,#244303,#244304,#244305,
#244306,#244307,#244308,#244309,#244310,#244311,#244312,#244313,#244314,
#244315,#244316,#244317,#244318,#244319,#244320,#244321,#244322,#244323,
#244324,#244325,#244326,#244327,#244328,#244329,#244330,#244331,#244332,
#244333,#244334,#244335,#244336,#244337,#244338,#244339,#244340,#244341,
#244342,#244343,#244344,#244345,#244346,#244347,#244348,#244349,#244350,
#244351,#244352,#244353,#244354,#244355,#244356,#244357,#244358,#244359,
#244360,#244361,#244362,#244363,#244364,#244365,#244366,#244367,#244368,
#244369,#244370,#244371,#244372,#244373,#244374,#244375,#244376,#244377,
#244378,#244379,#244380,#244381,#244382,#244383,#244384,#244385,#244386,
#244387,#244388,#244389,#244390,#244391,#244392,#244393,#244394,#244395,
#244396,#244397,#244398,#244399,#244400,#244401,#244402,#244403,#244404,
#244405,#244406,#244407,#244408,#244409,#244410,#244411,#244412,#244413,
#244414,#244415,#244416,#244417,#244418,#244419,#244420,#244421,#244422,
#244423,#244424,#244425,#244426,#244427,#244428,#244429,#244430,#244431,
#244432,#244433,#244434,#244435,#244436,#244437,#244438,#244439),
 .UNSPECIFIED.,.F.,.F.,(4,3,3,3,3,3,3,3,3,3,3,3,3,3,3,3,3,3,3,3,3,3,3,3,
3,3,3,3,3,3,3,3,3,3,3,3,3,3,3,3,3,3,3,3,3,3,3,3,3,3,3,3,3,3,3,3,3,3,3,3,
3,3,3,3,3,3,3,3,3,3,3,3,3,4),(1454.55739861207,1454.64200141043,1454.72522978866,
1454.80845873658,1454.89170646772,1454.97733510053,1455.06072123565,1455.1474711173,
1455.23422099896,1455.31795971081,1455.40159522217,1455.48514766557,1455.56863710142,
1455.65209105204,1455.73552754588,1455.81896465564,1455.90242045056,1455.98596494329,
1456.06955402623,1456.15327729378,1456.23395700968,1456.31769572153,1456.40133123289,
1456.48488367629,1456.56837311214,1456.65182706276,1456.7352635566,1456.81870066636,
1456.90215646127,1456.985700954,1457.06929003695,1457.1530133045,1457.2336930204,
1457.31743173225,1457.40106724361,1457.48461968701,1457.56810912286,1457.65156307348,
1457.73499956732,1457.81843667708,1457.901892472,1457.98543696473,1458.06902604767,
1458.15274931522,1458.23342903112,1458.31716774297,1458.40080325433,1458.48435569773,
1458.56784513358,1458.6512990842,1458.73473557804,1458.8181726878,1458.90162848272,
1458.98517297545,1459.06876205839,1459.15248532595,1459.23316504184,1459.31690375369,
1459.40053926505,1459.48409170845,1459.5675811443,1459.65103509492,1459.73447158876,
1459.81790869852,1459.90136449344,1459.98490898617,1460.06849806911,1460.15222133666,
1460.23290105256,1460.32215865567,1460.40683272219,1460.49142158211,1460.57592537746,
1460.58993146501),.UNSPECIFIED.);
#1845=B_SPLINE_CURVE_WITH_KNOTS('',3,(#244440,#244441,#244442,#244443,#244444,
#244445,#244446,#244447,#244448,#244449),.UNSPECIFIED.,.F.,.F.,(4,3,3,4),
(1454.30674307549,1454.40585639479,1454.50400867407,1454.55739861189),
 .UNSPECIFIED.);
#1846=B_SPLINE_CURVE_WITH_KNOTS('',3,(#244455,#244456,#244457,#244458,#244459,
#244460,#244461,#244462,#244463,#244464),.UNSPECIFIED.,.F.,.F.,(4,3,3,4),
(1448.0236730871,1448.12028229969,1448.21615954937,1448.27421330469),
 .UNSPECIFIED.);
#1847=B_SPLINE_CURVE_WITH_KNOTS('',3,(#244465,#244466,#244467,#244468,#244469,
#244470,#244471,#244472,#244473,#244474,#244475,#244476,#244477,#244478,
#244479,#244480,#244481,#244482,#244483,#244484,#244485,#244486,#244487,
#244488,#244489,#244490,#244491,#244492,#244493,#244494,#244495,#244496,
#244497,#244498,#244499,#244500,#244501,#244502,#244503,#244504,#244505,
#244506,#244507,#244508,#244509,#244510,#244511,#244512,#244513,#244514,
#244515,#244516,#244517,#244518,#244519,#244520,#244521,#244522,#244523,
#244524,#244525,#244526,#244527,#244528,#244529,#244530,#244531,#244532,
#244533,#244534,#244535,#244536,#244537,#244538,#244539,#244540,#244541,
#244542,#244543,#244544,#244545,#244546,#244547,#244548,#244549,#244550,
#244551,#244552,#244553,#244554,#244555,#244556,#244557,#244558,#244559,
#244560,#244561,#244562,#244563,#244564,#244565,#244566,#244567,#244568,
#244569,#244570,#244571,#244572,#244573,#244574,#244575,#244576,#244577,
#244578,#244579,#244580,#244581,#244582,#244583,#244584,#244585,#244586,
#244587,#244588,#244589,#244590,#244591,#244592,#244593,#244594,#244595,
#244596,#244597,#244598,#244599,#244600,#244601,#244602,#244603,#244604,
#244605,#244606,#244607,#244608,#244609,#244610,#244611,#244612,#244613,
#244614,#244615,#244616,#244617,#244618,#244619,#244620,#244621,#244622,
#244623,#244624,#244625,#244626,#244627,#244628,#244629,#244630,#244631,
#244632,#244633,#244634,#244635,#244636,#244637,#244638,#244639,#244640,
#244641,#244642,#244643,#244644,#244645,#244646,#244647,#244648,#244649,
#244650,#244651,#244652,#244653,#244654,#244655,#244656,#244657,#244658,
#244659,#244660,#244661,#244662,#244663,#244664,#244665,#244666,#244667,
#244668,#244669,#244670,#244671,#244672,#244673,#244674,#244675,#244676,
#244677,#244678,#244679,#244680,#244681,#244682,#244683,#244684),
 .UNSPECIFIED.,.F.,.F.,(4,3,3,3,3,3,3,3,3,3,3,3,3,3,3,3,3,3,3,3,3,3,3,3,
3,3,3,3,3,3,3,3,3,3,3,3,3,3,3,3,3,3,3,3,3,3,3,3,3,3,3,3,3,3,3,3,3,3,3,3,
3,3,3,3,3,3,3,3,3,3,3,3,3,4),(1448.27421330489,1448.35782433656,1448.44142899155,
1448.52504506398,1448.60869035153,1448.69243622458,1448.77623540817,1448.8601726709,
1448.92551431492,1449.00925302677,1449.09288853813,1449.17644098153,1449.25993041738,
1449.343384368,1449.42682086184,1449.5102579716,1449.59371376652,1449.67725825924,
1449.76084734219,1449.84457060974,1449.92525032564,1450.00898903749,1450.09262454885,
1450.17617699225,1450.2596664281,1450.34312037872,1450.42655687256,1450.50999398232,
1450.59344977724,1450.67699426997,1450.76058335291,1450.84430662046,1450.92498633636,
1451.00872504821,1451.09236055957,1451.17591300297,1451.25940243882,1451.34285638944,
1451.42629288328,1451.50972999304,1451.59318578796,1451.67673028069,1451.76031936363,
1451.84404263118,1451.92472234708,1452.00846105893,1452.09209657029,1452.17564901369,
1452.25913844954,1452.34259240016,1452.426028894,1452.50946600376,1452.59292179867,
1452.6764662914,1452.76005537434,1452.8437786419,1452.9244583578,1453.00819706965,
1453.09183258101,1453.17538502441,1453.25887446026,1453.34232841088,1453.42576490472,
1453.50920201448,1453.5926578094,1453.67620230213,1453.75979138507,1453.84351465263,
1453.92419436852,1454.00848723102,1454.09263873748,1454.17670875473,1454.26070005874,
1454.30662927058),.UNSPECIFIED.);
#1848=B_SPLINE_CURVE_WITH_KNOTS('',3,(#244686,#244687,#244688,#244689,#244690,
#244691,#244692,#244693,#244694,#244695,#244696,#244697,#244698,#244699,
#244700,#244701,#244702,#244703,#244704,#244705,#244706,#244707,#244708,
#244709,#244710,#244711,#244712,#244713,#244714,#244715,#244716,#244717,
#244718,#244719,#244720,#244721,#244722,#244723,#244724,#244725,#244726,
#244727,#244728,#244729,#244730,#244731,#244732,#244733,#244734,#244735,
#244736,#244737,#244738,#244739,#244740,#244741,#244742,#244743,#244744,
#244745,#244746,#244747,#244748,#244749,#244750,#244751,#244752,#244753,
#244754,#244755,#244756,#244757,#244758,#244759,#244760,#244761,#244762,
#244763,#244764,#244765,#244766,#244767,#244768,#244769,#244770,#244771,
#244772,#244773,#244774,#244775,#244776,#244777,#244778,#244779,#244780,
#244781,#244782,#244783,#244784,#244785,#244786,#244787,#244788,#244789,
#244790,#244791,#244792,#244793,#244794,#244795,#244796,#244797,#244798,
#244799,#244800,#244801,#244802,#244803,#244804,#244805,#244806,#244807,
#244808,#244809,#244810,#244811,#244812,#244813,#244814,#244815,#244816,
#244817,#244818,#244819,#244820,#244821,#244822,#244823,#244824,#244825,
#244826,#244827,#244828,#244829,#244830,#244831,#244832,#244833,#244834,
#244835,#244836,#244837,#244838,#244839,#244840,#244841,#244842,#244843,
#244844,#244845,#244846,#244847,#244848,#244849,#244850,#244851,#244852,
#244853,#244854,#244855,#244856,#244857,#244858,#244859,#244860,#244861,
#244862,#244863,#244864,#244865,#244866,#244867,#244868,#244869,#244870,
#244871,#244872,#244873,#244874,#244875,#244876,#244877,#244878,#244879,
#244880,#244881,#244882,#244883,#244884,#244885,#244886,#244887,#244888,
#244889,#244890,#244891,#244892,#244893,#244894,#244895,#244896,#244897,
#244898,#244899,#244900,#244901,#244902,#244903,#244904,#244905),
 .UNSPECIFIED.,.F.,.F.,(4,3,3,3,3,3,3,3,3,3,3,3,3,3,3,3,3,3,3,3,3,3,3,3,
3,3,3,3,3,3,3,3,3,3,3,3,3,3,3,3,3,3,3,3,3,3,3,3,3,3,3,3,3,3,3,3,3,3,3,3,
3,3,3,3,3,3,3,3,3,3,3,3,3,4),(1448.27421330505,1448.35743318097,1448.4405518179,
1448.52358985075,1448.60656783825,1448.68951465084,1448.77244760275,1448.85538521634,
1448.93834601377,1449.02139624031,1449.10449595701,1449.18771960852,1449.23580493464,
1449.31954364649,1449.40317915785,1449.48673160125,1449.5702210371,1449.65367498772,
1449.73711148156,1449.82054859132,1449.90400438624,1449.98754887897,1450.07113796191,
1450.15486122947,1450.23554094536,1450.31927965721,1450.40291516857,1450.48646761197,
1450.56995704782,1450.65341099844,1450.73684749228,1450.82028460204,1450.90374039696,
1450.98728488969,1451.07087397263,1451.15459724018,1451.23527695608,1451.31901566793,
1451.40265117929,1451.48620362269,1451.56969305854,1451.65314700916,1451.736583503,
1451.82002061276,1451.90347640768,1451.98702090041,1452.07060998335,1452.1543332509,
1452.2350129668,1452.31875167865,1452.40238719001,1452.48593963341,1452.56942906926,
1452.65288301988,1452.73631951372,1452.81975662348,1452.9032124184,1452.98675691113,
1453.07034599407,1453.15406926163,1453.23474897752,1453.31848768937,1453.40212320073,
1453.48567564413,1453.56916507998,1453.6526190306,1453.73605552444,1453.8194926342,
1453.90294842912,1453.98649292185,1454.07008200479,1454.15380527234,1454.23448498824,
1454.30674307549),.UNSPECIFIED.);
#1849=B_SPLINE_CURVE_WITH_KNOTS('',3,(#244906,#244907,#244908,#244909,#244910,
#244911,#244912,#244913,#244914,#244915,#244916,#244917,#244918),
 .UNSPECIFIED.,.F.,.F.,(4,3,3,3,4),(1448.02254698393,1448.10615919498,1448.18989572745,
1448.23606892392,1448.27421330489),.UNSPECIFIED.);
#1850=B_SPLINE_CURVE_WITH_KNOTS('',3,(#244924,#244925,#244926,#244927,#244928,
#244929,#244930,#244931,#244932,#244933,#244934,#244935,#244936),
 .UNSPECIFIED.,.F.,.F.,(4,3,3,3,4),(1441.73936764326,1441.82299876243,1441.9067473108,
1441.92736223988,1441.99102799771),.UNSPECIFIED.);
#1851=B_SPLINE_CURVE_WITH_KNOTS('',3,(#244937,#244938,#244939,#244940,#244941,
#244942,#244943,#244944,#244945,#244946,#244947,#244948,#244949,#244950,
#244951,#244952,#244953,#244954,#244955,#244956,#244957,#244958,#244959,
#244960,#244961,#244962,#244963,#244964,#244965,#244966,#244967,#244968,
#244969,#244970,#244971,#244972,#244973,#244974,#244975,#244976,#244977,
#244978,#244979,#244980,#244981,#244982,#244983,#244984,#244985,#244986,
#244987,#244988,#244989,#244990,#244991,#244992,#244993,#244994,#244995,
#244996,#244997,#244998,#244999,#245000,#245001,#245002,#245003,#245004,
#245005,#245006,#245007,#245008,#245009,#245010,#245011,#245012,#245013,
#245014,#245015,#245016,#245017,#245018,#245019,#245020,#245021,#245022,
#245023,#245024,#245025,#245026,#245027,#245028,#245029,#245030,#245031,
#245032,#245033,#245034,#245035,#245036,#245037,#245038,#245039,#245040,
#245041,#245042,#245043,#245044,#245045,#245046,#245047,#245048,#245049,
#245050,#245051,#245052,#245053,#245054,#245055,#245056,#245057,#245058,
#245059,#245060,#245061,#245062,#245063,#245064,#245065,#245066,#245067,
#245068,#245069,#245070,#245071,#245072,#245073,#245074,#245075,#245076,
#245077,#245078,#245079,#245080,#245081,#245082,#245083,#245084,#245085,
#245086,#245087,#245088,#245089,#245090,#245091,#245092,#245093,#245094,
#245095,#245096,#245097,#245098,#245099,#245100,#245101,#245102,#245103,
#245104,#245105,#245106,#245107,#245108,#245109,#245110,#245111,#245112,
#245113,#245114,#245115,#245116,#245117,#245118,#245119,#245120,#245121,
#245122,#245123,#245124,#245125,#245126,#245127,#245128,#245129,#245130,
#245131,#245132,#245133,#245134,#245135,#245136,#245137,#245138,#245139,
#245140,#245141,#245142,#245143,#245144,#245145,#245146,#245147,#245148,
#245149,#245150,#245151,#245152,#245153,#245154,#245155,#245156),
 .UNSPECIFIED.,.F.,.F.,(4,3,3,3,3,3,3,3,3,3,3,3,3,3,3,3,3,3,3,3,3,3,3,3,
3,3,3,3,3,3,3,3,3,3,3,3,3,3,3,3,3,3,3,3,3,3,3,3,3,3,3,3,3,3,3,3,3,3,3,3,
3,3,3,3,3,3,3,3,3,3,3,3,3,4),(1441.99102799783,1442.07397001655,1442.15681366223,
1442.23957978767,1442.32551959554,1442.40820144904,1442.49087354865,1442.5735546158,
1442.65626337548,1442.73906287441,1442.82191629707,1442.90488611973,1442.9270982506,
1443.01083696245,1443.09447247381,1443.17802491721,1443.26151435306,1443.34496830368,
1443.42840479752,1443.51184190728,1443.5952977022,1443.67884219493,1443.76243127787,
1443.84615454542,1443.92683426132,1444.01057297317,1444.09420848453,1444.17776092793,
1444.26125036378,1444.3447043144,1444.42814080824,1444.511577918,1444.59503371292,
1444.67857820565,1444.76216728859,1444.84589055615,1444.92657027204,1445.01030898389,
1445.09394449525,1445.17749693865,1445.2609863745,1445.34444032512,1445.42787681896,
1445.51131392872,1445.59476972363,1445.67831421636,1445.7619032993,1445.84562656686,
1445.92630628276,1446.01004499461,1446.09368050597,1446.17723294937,1446.26072238522,
1446.34417633584,1446.42761282968,1446.51104993944,1446.59450573436,1446.67805022709,
1446.76163931003,1446.84536257758,1446.92604229348,1447.00978100533,1447.09341651669,
1447.17696896009,1447.26045839594,1447.34391234655,1447.4273488404,1447.51078595016,
1447.59424174507,1447.6777862378,1447.76137532074,1447.8450985883,1447.9257783042,
1448.0236730871),.UNSPECIFIED.);
#1852=B_SPLINE_CURVE_WITH_KNOTS('',3,(#245158,#245159,#245160,#245161,#245162,
#245163,#245164,#245165,#245166,#245167,#245168,#245169,#245170,#245171,
#245172,#245173,#245174,#245175,#245176,#245177,#245178,#245179,#245180,
#245181,#245182,#245183,#245184,#245185,#245186,#245187,#245188,#245189,
#245190,#245191,#245192,#245193,#245194,#245195,#245196,#245197,#245198,
#245199,#245200,#245201,#245202,#245203,#245204,#245205,#245206,#245207,
#245208,#245209,#245210,#245211,#245212,#245213,#245214,#245215,#245216,
#245217,#245218,#245219,#245220,#245221,#245222,#245223,#245224,#245225,
#245226,#245227,#245228,#245229,#245230,#245231,#245232,#245233,#245234,
#245235,#245236,#245237,#245238,#245239,#245240,#245241,#245242,#245243,
#245244,#245245,#245246,#245247,#245248,#245249,#245250,#245251,#245252,
#245253,#245254,#245255,#245256,#245257,#245258,#245259,#245260,#245261,
#245262,#245263,#245264,#245265,#245266,#245267,#245268,#245269,#245270,
#245271,#245272,#245273,#245274,#245275,#245276,#245277,#245278,#245279,
#245280,#245281,#245282,#245283,#245284,#245285,#245286,#245287,#245288,
#245289,#245290,#245291,#245292,#245293,#245294,#245295,#245296,#245297,
#245298,#245299,#245300,#245301,#245302,#245303,#245304,#245305,#245306,
#245307,#245308,#245309,#245310,#245311,#245312,#245313,#245314,#245315,
#245316,#245317,#245318,#245319,#245320,#245321,#245322,#245323,#245324,
#245325,#245326,#245327,#245328,#245329,#245330,#245331,#245332,#245333,
#245334,#245335,#245336,#245337,#245338,#245339,#245340,#245341,#245342,
#245343,#245344,#245345,#245346,#245347,#245348,#245349,#245350,#245351,
#245352,#245353,#245354,#245355,#245356,#245357,#245358,#245359,#245360,
#245361,#245362,#245363,#245364,#245365,#245366,#245367,#245368,#245369,
#245370,#245371,#245372,#245373,#245374,#245375,#245376,#245377),
 .UNSPECIFIED.,.F.,.F.,(4,3,3,3,3,3,3,3,3,3,3,3,3,3,3,3,3,3,3,3,3,3,3,3,
3,3,3,3,3,3,3,3,3,3,3,3,3,3,3,3,3,3,3,3,3,3,3,3,3,3,3,3,3,3,3,3,3,3,3,3,
3,3,3,3,3,3,3,3,3,3,3,3,3,4),(1441.99102799785,1442.09882248263,1442.20915371554,
1442.2376528596,1442.32139157145,1442.40502708281,1442.48857952621,1442.57206896206,
1442.65552291267,1442.73895940652,1442.82239651628,1442.90585231119,1442.98939680392,
1443.07298588686,1443.15670915442,1443.23738887032,1443.32112758217,1443.40476309353,
1443.48831553693,1443.57180497278,1443.6552589234,1443.73869541724,1443.822132527,
1443.90558832192,1443.98913281465,1444.07272189759,1444.15644516514,1444.23712488104,
1444.32086359289,1444.40449910425,1444.48805154765,1444.5715409835,1444.65499493412,
1444.73843142796,1444.82186853772,1444.90532433264,1444.98886882536,1445.07245790831,
1445.15618117586,1445.23686089176,1445.32059960361,1445.40423511497,1445.48778755837,
1445.57127699422,1445.65473094484,1445.73816743868,1445.82160454844,1445.90506034336,
1445.98860483609,1446.07219391903,1446.15591718658,1446.23659690248,1446.32033561433,
1446.40397112569,1446.48752356909,1446.57101300494,1446.65446695556,1446.7379034494,
1446.82134055916,1446.90479635408,1446.98834084681,1447.07192992975,1447.1556531973,
1447.2363329132,1447.32008459951,1447.40789239756,1447.49143313082,1447.57491711298,
1447.65836246294,1447.74178726958,1447.82523138041,1447.90868683001,1447.99219954226,
1448.02254698393),.UNSPECIFIED.);
#1853=B_SPLINE_CURVE_WITH_KNOTS('',3,(#245378,#245379,#245380,#245381,#245382,
#245383,#245384,#245385,#245386,#245387),.UNSPECIFIED.,.F.,.F.,(4,3,3,4),
(1441.73964840693,1441.82211908339,1441.90657354055,1441.99102799771),
 .UNSPECIFIED.);
#1854=B_SPLINE_CURVE_WITH_KNOTS('',3,(#245393,#245394,#245395,#245396,#245397,
#245398,#245399,#245400,#245401,#245402),.UNSPECIFIED.,.F.,.F.,(4,3,3,4),
(1435.45634400191,1435.53868546224,1435.62326407632,1435.70784269039),
 .UNSPECIFIED.);
#1855=B_SPLINE_CURVE_WITH_KNOTS('',3,(#245403,#245404,#245405,#245406,#245407,
#245408,#245409,#245410,#245411,#245412,#245413,#245414,#245415,#245416,
#245417,#245418,#245419,#245420,#245421,#245422,#245423,#245424,#245425,
#245426,#245427,#245428,#245429,#245430,#245431,#245432,#245433,#245434,
#245435,#245436,#245437,#245438,#245439,#245440,#245441,#245442,#245443,
#245444,#245445,#245446,#245447,#245448,#245449,#245450,#245451,#245452,
#245453,#245454,#245455,#245456,#245457,#245458,#245459,#245460,#245461,
#245462,#245463,#245464,#245465,#245466,#245467,#245468,#245469,#245470,
#245471,#245472,#245473,#245474,#245475,#245476,#245477,#245478,#245479,
#245480,#245481,#245482,#245483,#245484,#245485,#245486,#245487,#245488,
#245489,#245490,#245491,#245492,#245493,#245494,#245495,#245496,#245497,
#245498,#245499,#245500,#245501,#245502,#245503,#245504,#245505,#245506,
#245507,#245508,#245509,#245510,#245511,#245512,#245513,#245514,#245515,
#245516,#245517,#245518,#245519,#245520,#245521,#245522,#245523,#245524,
#245525,#245526,#245527,#245528,#245529,#245530,#245531,#245532,#245533,
#245534,#245535,#245536,#245537,#245538,#245539,#245540,#245541,#245542,
#245543,#245544,#245545,#245546,#245547,#245548,#245549,#245550,#245551,
#245552,#245553,#245554,#245555,#245556,#245557,#245558,#245559,#245560,
#245561,#245562,#245563,#245564,#245565,#245566,#245567,#245568,#245569,
#245570,#245571,#245572,#245573,#245574,#245575,#245576,#245577,#245578,
#245579,#245580,#245581,#245582,#245583,#245584,#245585,#245586,#245587,
#245588,#245589,#245590,#245591,#245592,#245593,#245594,#245595,#245596,
#245597,#245598,#245599,#245600,#245601,#245602,#245603,#245604,#245605,
#245606,#245607,#245608,#245609,#245610,#245611,#245612,#245613,#245614,
#245615,#245616,#245617,#245618,#245619),.UNSPECIFIED.,.F.,.F.,(4,3,3,3,
3,3,3,3,3,3,3,3,3,3,3,3,3,3,3,3,3,3,3,3,3,3,3,3,3,3,3,3,3,3,3,3,3,3,3,3,
3,3,3,3,3,3,3,3,3,3,3,3,3,3,3,3,3,3,3,3,3,3,3,3,3,3,3,3,3,3,3,3,4),(1435.70784269053,
1435.82235604207,1435.92894617556,1436.01268488741,1436.09632039877,1436.17987284217,
1436.26336227802,1436.34681622863,1436.43025272248,1436.51368983223,1436.59714562715,
1436.68069011988,1436.76427920282,1436.84800247038,1436.92868218628,1437.01242089813,
1437.09605640949,1437.17960885289,1437.26309828874,1437.34655223936,1437.4299887332,
1437.51342584296,1437.59688163788,1437.68042613061,1437.76401521355,1437.8477384811,
1437.928418197,1438.01215690885,1438.09579242021,1438.17934486361,1438.26283429946,
1438.34628825008,1438.42972474392,1438.51316185368,1438.5966176486,1438.68016214133,
1438.76375122427,1438.84747449183,1438.92815420772,1439.01189291957,1439.09552843093,
1439.17908087433,1439.26257031018,1439.3460242608,1439.42946075464,1439.5128978644,
1439.59635365932,1439.67989815205,1439.76348723499,1439.84721050254,1439.92789021844,
1440.01162893029,1440.09526444165,1440.17881688505,1440.2623063209,1440.34576027152,
1440.42919676536,1440.51263387512,1440.59608967004,1440.67963416277,1440.76322324571,
1440.84694651326,1440.92762622916,1441.01137625723,1441.09502060469,1441.17856410501,
1441.26205042852,1441.34549769506,1441.42892399429,1441.51237342932,1441.59583358817,
1441.67936222842,1441.73936764326),.UNSPECIFIED.);
#1856=B_SPLINE_CURVE_WITH_KNOTS('',3,(#245621,#245622,#245623,#245624,#245625,
#245626,#245627,#245628,#245629,#245630,#245631,#245632,#245633,#245634,
#245635,#245636,#245637,#245638,#245639,#245640,#245641,#245642,#245643,
#245644,#245645,#245646,#245647,#245648,#245649,#245650,#245651,#245652,
#245653,#245654,#245655,#245656,#245657,#245658,#245659,#245660,#245661,
#245662,#245663,#245664,#245665,#245666,#245667,#245668,#245669,#245670,
#245671,#245672,#245673,#245674,#245675,#245676,#245677,#245678,#245679,
#245680,#245681,#245682,#245683,#245684,#245685,#245686,#245687,#245688,
#245689,#245690,#245691,#245692,#245693,#245694,#245695,#245696,#245697,
#245698,#245699,#245700,#245701,#245702,#245703,#245704,#245705,#245706,
#245707,#245708,#245709,#245710,#245711,#245712,#245713,#245714,#245715,
#245716,#245717,#245718,#245719,#245720,#245721,#245722,#245723,#245724,
#245725,#245726,#245727,#245728,#245729,#245730,#245731,#245732,#245733,
#245734,#245735,#245736,#245737,#245738,#245739,#245740,#245741,#245742,
#245743,#245744,#245745,#245746,#245747,#245748,#245749,#245750,#245751,
#245752,#245753,#245754,#245755,#245756,#245757,#245758,#245759,#245760,
#245761,#245762,#245763,#245764,#245765,#245766,#245767,#245768,#245769,
#245770,#245771,#245772,#245773,#245774,#245775,#245776,#245777,#245778,
#245779,#245780,#245781,#245782,#245783,#245784,#245785,#245786,#245787,
#245788,#245789,#245790,#245791,#245792,#245793,#245794,#245795,#245796,
#245797,#245798,#245799,#245800,#245801,#245802,#245803,#245804,#245805,
#245806,#245807,#245808,#245809,#245810,#245811,#245812,#245813,#245814,
#245815,#245816,#245817,#245818,#245819,#245820,#245821,#245822,#245823,
#245824,#245825,#245826,#245827,#245828,#245829,#245830,#245831,#245832,
#245833,#245834,#245835,#245836,#245837),.UNSPECIFIED.,.F.,.F.,(4,3,3,3,
3,3,3,3,3,3,3,3,3,3,3,3,3,3,3,3,3,3,3,3,3,3,3,3,3,3,3,3,3,3,3,3,3,3,3,3,
3,3,3,3,3,3,3,3,3,3,3,3,3,3,3,3,3,3,3,3,3,3,3,3,3,3,3,3,3,3,3,3,4),(1435.70784269053,
1435.79418909534,1435.8806134886,1435.97026931526,1436.05695086,1436.14809382764,
1436.23923679527,1436.32297550712,1436.40661101849,1436.49016346189,1436.57365289774,
1436.65710684835,1436.7405433422,1436.82398045196,1436.90743624688,1436.99098073961,
1437.07456982255,1437.15829309011,1437.23897280599,1437.32271151783,1437.4063470292,
1437.4898994726,1437.57338890845,1437.65684285906,1437.74027935291,1437.82371646266,
1437.90717225758,1437.99071675031,1438.07430583325,1438.15802910081,1438.23870881671,
1438.32244752856,1438.40608303993,1438.48963548333,1438.57312491918,1438.6565788698,
1438.74001536364,1438.8234524734,1438.90690826832,1438.99045276105,1439.07404184399,
1439.15776511155,1439.23844482744,1439.32218353929,1439.40581905065,1439.48937149405,
1439.57286092991,1439.65631488052,1439.73975137437,1439.82318848412,1439.90664427904,
1439.99018877177,1440.07377785471,1440.15750112227,1440.23818083816,1440.32191955001,
1440.40555506137,1440.48910750477,1440.57259694062,1440.65605089123,1440.73948738508,
1440.82292449483,1440.90638028975,1440.98992478248,1441.07351386542,1441.15723713298,
1441.23791684888,1441.32066010468,1441.40330528578,1441.48739106607,1441.56989035993,
1441.65476938343,1441.73964840693),.UNSPECIFIED.);
#1857=B_SPLINE_CURVE_WITH_KNOTS('',3,(#245838,#245839,#245840,#245841,#245842,
#245843,#245844,#245845,#245846,#245847),.UNSPECIFIED.,.F.,.F.,(4,3,3,4),
(1435.45754054782,1435.54645941689,1435.63515374008,1435.7078426904),
 .UNSPECIFIED.);
#1858=B_SPLINE_CURVE_WITH_KNOTS('',3,(#245853,#245854,#245855,#245856,#245857,
#245858,#245859,#245860,#245861,#245862),.UNSPECIFIED.,.F.,.F.,(4,3,3,4),
(1429.17433711171,1429.26217368456,1429.3498375818,1429.42465738322),
 .UNSPECIFIED.);
#1859=B_SPLINE_CURVE_WITH_KNOTS('',3,(#245863,#245864,#245865,#245866,#245867,
#245868,#245869,#245870,#245871,#245872,#245873,#245874,#245875,#245876,
#245877,#245878,#245879,#245880,#245881,#245882,#245883,#245884,#245885,
#245886,#245887,#245888,#245889,#245890,#245891,#245892,#245893,#245894,
#245895,#245896,#245897,#245898,#245899,#245900,#245901,#245902,#245903,
#245904,#245905,#245906,#245907,#245908,#245909,#245910,#245911,#245912,
#245913,#245914,#245915,#245916,#245917,#245918,#245919,#245920,#245921,
#245922,#245923,#245924,#245925,#245926,#245927,#245928,#245929,#245930,
#245931,#245932,#245933,#245934,#245935,#245936,#245937,#245938,#245939,
#245940,#245941,#245942,#245943,#245944,#245945,#245946,#245947,#245948,
#245949,#245950,#245951,#245952,#245953,#245954,#245955,#245956,#245957,
#245958,#245959,#245960,#245961,#245962,#245963,#245964,#245965,#245966,
#245967,#245968,#245969,#245970,#245971,#245972,#245973,#245974,#245975,
#245976,#245977,#245978,#245979,#245980,#245981,#245982,#245983,#245984,
#245985,#245986,#245987,#245988,#245989,#245990,#245991,#245992,#245993,
#245994,#245995,#245996,#245997,#245998,#245999,#246000,#246001,#246002,
#246003,#246004,#246005,#246006,#246007,#246008,#246009,#246010,#246011,
#246012,#246013,#246014,#246015,#246016,#246017,#246018,#246019,#246020,
#246021,#246022,#246023,#246024,#246025,#246026,#246027,#246028,#246029,
#246030,#246031,#246032,#246033,#246034,#246035,#246036,#246037,#246038,
#246039,#246040,#246041,#246042,#246043,#246044,#246045,#246046,#246047,
#246048,#246049,#246050,#246051,#246052,#246053,#246054,#246055,#246056,
#246057,#246058,#246059,#246060,#246061,#246062,#246063,#246064,#246065,
#246066,#246067,#246068,#246069,#246070,#246071,#246072,#246073,#246074,
#246075,#246076,#246077,#246078,#246079,#246080,#246081,#246082),
 .UNSPECIFIED.,.F.,.F.,(4,3,3,3,3,3,3,3,3,3,3,3,3,3,3,3,3,3,3,3,3,3,3,3,
3,3,3,3,3,3,3,3,3,3,3,3,3,3,3,3,3,3,3,3,3,3,3,3,3,3,3,3,3,3,3,3,3,3,3,3,
3,3,3,3,3,3,3,3,3,3,3,3,3,4),(1429.42465738335,1429.51184693731,1429.59914373417,
1429.6866395601,1429.77423939675,1429.86203908662,1429.93053011124,1430.01426882309,
1430.09790433445,1430.18145677785,1430.2649462137,1430.34840016431,1430.43183665816,
1430.51527376791,1430.59872956283,1430.68227405556,1430.7658631385,1430.84958640606,
1430.93026612196,1431.01400483381,1431.09764034517,1431.18119278857,1431.26468222442,
1431.34813617504,1431.43157266888,1431.51500977864,1431.59846557356,1431.68201006629,
1431.76559914923,1431.84932241678,1431.93000213268,1432.01374084453,1432.09737635589,
1432.18092879929,1432.26441823514,1432.34787218576,1432.4313086796,1432.51474578936,
1432.59820158428,1432.68174607701,1432.76533515995,1432.84905842751,1432.9297381434,
1433.01347685525,1433.09711236661,1433.18066481001,1433.26415424586,1433.34760819648,
1433.43104469032,1433.51448180008,1433.597937595,1433.68148208772,1433.76507117067,
1433.84879443822,1433.92947415412,1434.01321286597,1434.09684837733,1434.18040082073,
1434.26389025658,1434.3473442072,1434.43078070104,1434.5142178108,1434.59767360572,
1434.68121809845,1434.76480718139,1434.84853044895,1434.92921016484,1435.01180452316,
1435.09430200276,1435.17672175617,1435.25907889747,1435.34139995451,1435.42371181849,
1435.45634400191),.UNSPECIFIED.);
#1860=B_SPLINE_CURVE_WITH_KNOTS('',3,(#246084,#246085,#246086,#246087,#246088,
#246089,#246090,#246091,#246092,#246093,#246094,#246095,#246096,#246097,
#246098,#246099,#246100,#246101,#246102,#246103,#246104,#246105,#246106,
#246107,#246108,#246109,#246110,#246111,#246112,#246113,#246114,#246115,
#246116,#246117,#246118,#246119,#246120,#246121,#246122,#246123,#246124,
#246125,#246126,#246127,#246128,#246129,#246130,#246131,#246132,#246133,
#246134,#246135,#246136,#246137,#246138,#246139,#246140,#246141,#246142,
#246143,#246144,#246145,#246146,#246147,#246148,#246149,#246150,#246151,
#246152,#246153,#246154,#246155,#246156,#246157,#246158,#246159,#246160,
#246161,#246162,#246163,#246164,#246165,#246166,#246167,#246168,#246169,
#246170,#246171,#246172,#246173,#246174,#246175,#246176,#246177,#246178,
#246179,#246180,#246181,#246182,#246183,#246184,#246185,#246186,#246187,
#246188,#246189,#246190,#246191,#246192,#246193,#246194,#246195,#246196,
#246197,#246198,#246199,#246200,#246201,#246202,#246203,#246204,#246205,
#246206,#246207,#246208,#246209,#246210,#246211,#246212,#246213,#246214,
#246215,#246216,#246217,#246218,#246219,#246220,#246221,#246222,#246223,
#246224,#246225,#246226,#246227,#246228,#246229,#246230,#246231,#246232,
#246233,#246234,#246235,#246236,#246237,#246238,#246239,#246240,#246241,
#246242,#246243,#246244,#246245,#246246,#246247,#246248,#246249,#246250,
#246251,#246252,#246253,#246254,#246255,#246256,#246257,#246258,#246259,
#246260,#246261,#246262,#246263,#246264,#246265,#246266,#246267,#246268,
#246269,#246270,#246271,#246272,#246273,#246274,#246275,#246276,#246277,
#246278,#246279,#246280,#246281,#246282,#246283,#246284,#246285,#246286,
#246287,#246288,#246289,#246290,#246291,#246292,#246293,#246294,#246295,
#246296,#246297,#246298,#246299,#246300,#246301,#246302,#246303),
 .UNSPECIFIED.,.F.,.F.,(4,3,3,3,3,3,3,3,3,3,3,3,3,3,3,3,3,3,3,3,3,3,3,3,
3,3,3,3,3,3,3,3,3,3,3,3,3,3,3,3,3,3,3,3,3,3,3,3,3,3,3,3,3,3,3,3,3,3,3,3,
3,3,3,3,3,3,3,3,3,3,3,3,3,4),(1429.4246573835,1429.50702048783,1429.58931001852,
1429.67155095664,1429.75376682562,1429.83597666066,1429.91819948982,1430.0005042299,
1430.08285026655,1430.16532564741,1430.24082073095,1430.3245594428,1430.40819495416,
1430.49174739756,1430.57523683341,1430.65869078403,1430.74212727787,1430.82556438763,
1430.90902018255,1430.99256467528,1431.07615375822,1431.15987702578,1431.24055674167,
1431.32429545352,1431.40793096488,1431.49148340828,1431.57497284413,1431.65842679475,
1431.74186328859,1431.82530039835,1431.90875619327,1431.992300686,1432.07588976894,
1432.1596130365,1432.24029275239,1432.32403146424,1432.4076669756,1432.491219419,
1432.57470885485,1432.65816280547,1432.74159929931,1432.82503640907,1432.90849220399,
1432.99203669672,1433.07562577966,1433.15934904721,1433.24002876311,1433.32376747496,
1433.40740298632,1433.49095542972,1433.57444486557,1433.65789881619,1433.74133531003,
1433.82477241979,1433.90822821471,1433.99177270744,1434.07536179038,1434.15908505794,
1434.23976477383,1434.32350348568,1434.40713899704,1434.49069144044,1434.57418087629,
1434.6576348269,1434.74107132075,1434.8245084305,1434.90796422542,1434.99150871815,
1435.07509780109,1435.15882106865,1435.23950078455,1435.32891254343,1435.41810836263,
1435.45754054782),.UNSPECIFIED.);
#1861=B_SPLINE_CURVE_WITH_KNOTS('',3,(#246304,#246305,#246306,#246307,#246308,
#246309,#246310,#246311,#246312,#246313),.UNSPECIFIED.,.F.,.F.,(4,3,3,4),
(1429.17325060202,1429.24108472023,1429.36688712493,1429.42465738335),
 .UNSPECIFIED.);
#1862=B_SPLINE_CURVE_WITH_KNOTS('',3,(#246319,#246320,#246321,#246322,#246323,
#246324,#246325,#246326,#246327,#246328),.UNSPECIFIED.,.F.,.F.,(4,3,3,4),
(1422.89017552255,1422.93237803619,1423.04995135785,1423.14147207617),
 .UNSPECIFIED.);
#1863=B_SPLINE_CURVE_WITH_KNOTS('',3,(#246329,#246330,#246331,#246332,#246333,
#246334,#246335,#246336,#246337,#246338,#246339,#246340,#246341,#246342,
#246343,#246344,#246345,#246346,#246347,#246348,#246349,#246350,#246351,
#246352,#246353,#246354,#246355,#246356,#246357,#246358,#246359,#246360,
#246361,#246362,#246363,#246364,#246365,#246366,#246367,#246368,#246369,
#246370,#246371,#246372,#246373,#246374,#246375,#246376,#246377,#246378,
#246379,#246380,#246381,#246382,#246383,#246384,#246385,#246386,#246387,
#246388,#246389,#246390,#246391,#246392,#246393,#246394,#246395,#246396,
#246397,#246398,#246399,#246400,#246401,#246402,#246403,#246404,#246405,
#246406,#246407,#246408,#246409,#246410,#246411,#246412,#246413,#246414,
#246415,#246416,#246417,#246418,#246419,#246420,#246421,#246422,#246423,
#246424,#246425,#246426,#246427,#246428,#246429,#246430,#246431,#246432,
#246433,#246434,#246435,#246436,#246437,#246438,#246439,#246440,#246441,
#246442,#246443,#246444,#246445,#246446,#246447,#246448,#246449,#246450,
#246451,#246452,#246453,#246454,#246455,#246456,#246457,#246458,#246459,
#246460,#246461,#246462,#246463,#246464,#246465,#246466,#246467,#246468,
#246469,#246470,#246471,#246472,#246473,#246474,#246475,#246476,#246477,
#246478,#246479,#246480,#246481,#246482,#246483,#246484,#246485,#246486,
#246487,#246488,#246489,#246490,#246491,#246492,#246493,#246494,#246495,
#246496,#246497,#246498,#246499,#246500,#246501,#246502,#246503,#246504,
#246505,#246506,#246507,#246508,#246509,#246510,#246511,#246512,#246513,
#246514,#246515,#246516,#246517,#246518,#246519,#246520,#246521,#246522,
#246523,#246524,#246525,#246526,#246527,#246528,#246529,#246530,#246531,
#246532,#246533,#246534,#246535,#246536,#246537,#246538,#246539,#246540,
#246541,#246542,#246543,#246544,#246545,#246546,#246547,#246548),
 .UNSPECIFIED.,.F.,.F.,(4,3,3,3,3,3,3,3,3,3,3,3,3,3,3,3,3,3,3,3,3,3,3,3,
3,3,3,3,3,3,3,3,3,3,3,3,3,3,3,3,3,3,3,3,3,3,3,3,3,3,3,3,3,3,3,3,3,3,3,3,
3,3,3,3,3,3,3,3,3,3,3,3,3,4),(1423.14147207631,1423.22386678623,1423.30619520945,
1423.38848470131,1423.47075562151,1423.55302696428,1423.63531772196,1423.71769400858,
1423.80011729223,1423.88266299128,1423.93211404692,1424.01585275877,1424.09948827013,
1424.18304071353,1424.26653014938,1424.3499841,1424.43342059384,1424.5168577036,
1424.60031349852,1424.68385799124,1424.76744707419,1424.85117034174,1424.93185005764,
1425.01558876949,1425.09922428085,1425.18277672425,1425.2662661601,1425.34972011072,
1425.43315660456,1425.51659371432,1425.60004950923,1425.68359400196,1425.7671830849,
1425.85090635246,1425.93158606836,1426.01532478021,1426.09896029157,1426.18251273497,
1426.26600217082,1426.34945612144,1426.43289261528,1426.51632972504,1426.59978551996,
1426.68333001269,1426.76691909563,1426.85064236319,1426.93132207908,1427.01506079093,
1427.09869630229,1427.18224874569,1427.26573818154,1427.34919213216,1427.432628626,
1427.51606573576,1427.59952153068,1427.68306602341,1427.76665510635,1427.85037837391,
1427.9310580898,1428.01479680165,1428.09843231301,1428.18198475641,1428.26547419226,
1428.34892814288,1428.43236463672,1428.51580174648,1428.5992575414,1428.68280203413,
1428.76639111707,1428.85011438462,1428.93079410052,1429.01909172383,1429.10718968499,
1429.17433711171),.UNSPECIFIED.);
#1864=B_SPLINE_CURVE_WITH_KNOTS('',3,(#246550,#246551,#246552,#246553,#246554,
#246555,#246556,#246557,#246558,#246559,#246560,#246561,#246562,#246563,
#246564,#246565,#246566,#246567,#246568,#246569,#246570,#246571,#246572,
#246573,#246574,#246575,#246576,#246577,#246578,#246579,#246580,#246581,
#246582,#246583,#246584,#246585,#246586,#246587,#246588,#246589,#246590,
#246591,#246592,#246593,#246594,#246595,#246596,#246597,#246598,#246599,
#246600,#246601,#246602,#246603,#246604,#246605,#246606,#246607,#246608,
#246609,#246610,#246611,#246612,#246613,#246614,#246615,#246616,#246617,
#246618,#246619,#246620,#246621,#246622,#246623,#246624,#246625,#246626,
#246627,#246628,#246629,#246630,#246631,#246632,#246633,#246634,#246635,
#246636,#246637,#246638,#246639,#246640,#246641,#246642,#246643,#246644,
#246645,#246646,#246647,#246648,#246649,#246650,#246651,#246652,#246653,
#246654,#246655,#246656,#246657,#246658,#246659,#246660,#246661,#246662,
#246663,#246664,#246665,#246666,#246667,#246668,#246669,#246670,#246671,
#246672,#246673,#246674,#246675,#246676,#246677,#246678,#246679,#246680,
#246681,#246682,#246683,#246684,#246685,#246686,#246687,#246688,#246689,
#246690,#246691,#246692,#246693,#246694,#246695,#246696,#246697,#246698,
#246699,#246700,#246701,#246702,#246703,#246704,#246705,#246706,#246707,
#246708,#246709,#246710,#246711,#246712,#246713,#246714,#246715,#246716,
#246717,#246718,#246719,#246720,#246721,#246722,#246723,#246724,#246725,
#246726,#246727,#246728,#246729,#246730,#246731,#246732,#246733,#246734,
#246735,#246736,#246737,#246738,#246739,#246740,#246741,#246742,#246743,
#246744,#246745,#246746,#246747,#246748,#246749,#246750,#246751,#246752,
#246753,#246754,#246755,#246756,#246757,#246758,#246759,#246760,#246761,
#246762,#246763,#246764,#246765,#246766),.UNSPECIFIED.,.F.,.F.,(4,3,3,3,
3,3,3,3,3,3,3,3,3,3,3,3,3,3,3,3,3,3,3,3,3,3,3,3,3,3,3,3,3,3,3,3,3,3,3,3,
3,3,3,3,3,3,3,3,3,3,3,3,3,3,3,3,3,3,3,3,3,3,3,3,3,3,3,3,3,3,3,3,4),(1423.14147207617,
1423.24266865591,1423.32640736776,1423.41004287912,1423.49359532252,1423.57708475837,
1423.66053870899,1423.74397520283,1423.82741231259,1423.91086810751,1423.99441260024,
1424.07800168318,1424.16172495074,1424.24240466663,1424.32614337848,1424.40977888984,
1424.49333133324,1424.57682076909,1424.66027471971,1424.74371121355,1424.82714832331,
1424.91060411823,1424.99414861096,1425.0777376939,1425.16146096146,1425.24214067735,
1425.3258793892,1425.40951490056,1425.49306734396,1425.57655677981,1425.66001073043,
1425.74344722427,1425.82688433403,1425.91034012894,1425.99388462167,1426.07747370462,
1426.16119697217,1426.24187668807,1426.32561539992,1426.40925091128,1426.49280335468,
1426.57629279053,1426.65974674115,1426.74318323499,1426.82662034475,1426.91007613967,
1426.9936206324,1427.07720971534,1427.1609329829,1427.24161269879,1427.32535141064,
1427.408986922,1427.4925393654,1427.57602880125,1427.65948275187,1427.74291924571,
1427.82635635547,1427.90981215039,1427.99335664312,1428.07694572606,1428.16066899361,
1428.24134870951,1428.32509132268,1428.40872984063,1428.49228439967,1428.57740517497,
1428.66085544328,1428.74428734301,1428.82771894588,1428.91410185992,1428.9976247119,
1429.08543765696,1429.17325060202),.UNSPECIFIED.);
#1865=B_SPLINE_CURVE_WITH_KNOTS('',3,(#246767,#246768,#246769,#246770,#246771,
#246772,#246773,#246774,#246775,#246776),.UNSPECIFIED.,.F.,.F.,(4,3,3,4),
(1422.88963902832,1422.97213368162,1423.05680287883,1423.14147207603),
 .UNSPECIFIED.);
#1866=B_SPLINE_CURVE_WITH_KNOTS('',3,(#246782,#246783,#246784,#246785,#246786,
#246787,#246788,#246789,#246790,#246791),.UNSPECIFIED.,.F.,.F.,(4,3,3,4),
(1416.60645213015,1416.68913802073,1416.7737123948,1416.85828676886),
 .UNSPECIFIED.);
#1867=B_SPLINE_CURVE_WITH_KNOTS('',3,(#246792,#246793,#246794,#246795,#246796,
#246797,#246798,#246799,#246800,#246801,#246802,#246803,#246804,#246805,
#246806,#246807,#246808,#246809,#246810,#246811,#246812,#246813,#246814,
#246815,#246816,#246817,#246818,#246819,#246820,#246821,#246822,#246823,
#246824,#246825,#246826,#246827,#246828,#246829,#246830,#246831,#246832,
#246833,#246834,#246835,#246836,#246837,#246838,#246839,#246840,#246841,
#246842,#246843,#246844,#246845,#246846,#246847,#246848,#246849,#246850,
#246851,#246852,#246853,#246854,#246855,#246856,#246857,#246858,#246859,
#246860,#246861,#246862,#246863,#246864,#246865,#246866,#246867,#246868,
#246869,#246870,#246871,#246872,#246873,#246874,#246875,#246876,#246877,
#246878,#246879,#246880,#246881,#246882,#246883,#246884,#246885,#246886,
#246887,#246888,#246889,#246890,#246891,#246892,#246893,#246894,#246895,
#246896,#246897,#246898,#246899,#246900,#246901,#246902,#246903,#246904,
#246905,#246906,#246907,#246908,#246909,#246910,#246911,#246912,#246913,
#246914,#246915,#246916,#246917,#246918,#246919,#246920,#246921,#246922,
#246923,#246924,#246925,#246926,#246927,#246928,#246929,#246930,#246931,
#246932,#246933,#246934,#246935,#246936,#246937,#246938,#246939,#246940,
#246941,#246942,#246943,#246944,#246945,#246946,#246947,#246948,#246949,
#246950,#246951,#246952,#246953,#246954,#246955,#246956,#246957,#246958,
#246959,#246960,#246961,#246962,#246963,#246964,#246965,#246966,#246967,
#246968,#246969,#246970,#246971,#246972,#246973,#246974,#246975,#246976,
#246977,#246978,#246979,#246980,#246981,#246982,#246983,#246984,#246985,
#246986,#246987,#246988,#246989,#246990,#246991,#246992,#246993,#246994,
#246995,#246996,#246997,#246998,#246999,#247000,#247001,#247002,#247003,
#247004,#247005,#247006,#247007,#247008,#247009,#247010,#247011),
 .UNSPECIFIED.,.F.,.F.,(4,3,3,3,3,3,3,3,3,3,3,3,3,3,3,3,3,3,3,3,3,3,3,3,
3,3,3,3,3,3,3,3,3,3,3,3,3,3,3,3,3,3,3,3,3,3,3,3,3,3,3,3,3,3,3,3,3,3,3,3,
3,3,3,3,3,3,3,3,3,3,3,3,3,4),(1416.85828676899,1416.93396197187,1417.01770068372,
1417.10133619508,1417.18488863848,1417.26837807433,1417.35183202495,1417.43526851879,
1417.51870562855,1417.60216142347,1417.6857059162,1417.76929499914,1417.8530182667,
1417.93369798259,1418.01743669444,1418.1010722058,1418.1846246492,1418.26811408505,
1418.35156803567,1418.43500452951,1418.51844163927,1418.60189743419,1418.68544192692,
1418.76903100986,1418.85275427742,1418.93343399331,1419.01717270516,1419.10080821652,
1419.18436065992,1419.26785009577,1419.35130404639,1419.43474054023,1419.51817764999,
1419.60163344491,1419.68517793764,1419.76876702058,1419.85249028813,1419.93317000403,
1420.01690871588,1420.10054422724,1420.18409667064,1420.26758610649,1420.35104005711,
1420.43447655095,1420.51791366071,1420.60136945563,1420.68491394836,1420.7685030313,
1420.85222629885,1420.93290601475,1421.0166447266,1421.10028023796,1421.18383268136,
1421.26732211721,1421.35077606783,1421.43421256167,1421.51764967143,1421.60110546634,
1421.68464995907,1421.76823904201,1421.85196230957,1421.93264202547,1422.01638314035,
1422.10002049812,1422.18357423364,1422.26706440912,1422.35051630726,1422.4339499617,
1422.51738344462,1422.60083482409,1422.68436422929,1422.76793789954,1422.85162109986,
1422.89017552255),.UNSPECIFIED.);
#1868=B_SPLINE_CURVE_WITH_KNOTS('',3,(#247013,#247014,#247015,#247016,#247017,
#247018,#247019,#247020,#247021,#247022,#247023,#247024,#247025,#247026,
#247027,#247028,#247029,#247030,#247031,#247032,#247033,#247034,#247035,
#247036,#247037,#247038,#247039,#247040,#247041,#247042,#247043,#247044,
#247045,#247046,#247047,#247048,#247049,#247050,#247051,#247052,#247053,
#247054,#247055,#247056,#247057,#247058,#247059,#247060,#247061,#247062,
#247063,#247064,#247065,#247066,#247067,#247068,#247069,#247070,#247071,
#247072,#247073,#247074,#247075,#247076,#247077,#247078,#247079,#247080,
#247081,#247082,#247083,#247084,#247085,#247086,#247087,#247088,#247089,
#247090,#247091,#247092,#247093,#247094,#247095,#247096,#247097,#247098,
#247099,#247100,#247101,#247102,#247103,#247104,#247105,#247106,#247107,
#247108,#247109,#247110,#247111,#247112,#247113,#247114,#247115,#247116,
#247117,#247118,#247119,#247120,#247121,#247122,#247123,#247124,#247125,
#247126,#247127,#247128,#247129,#247130,#247131,#247132,#247133,#247134,
#247135,#247136,#247137,#247138,#247139,#247140,#247141,#247142,#247143,
#247144,#247145,#247146,#247147,#247148,#247149,#247150,#247151,#247152,
#247153,#247154,#247155,#247156,#247157,#247158,#247159,#247160,#247161,
#247162,#247163,#247164,#247165,#247166,#247167,#247168,#247169,#247170,
#247171,#247172,#247173,#247174,#247175,#247176,#247177,#247178,#247179,
#247180,#247181,#247182,#247183,#247184,#247185,#247186,#247187,#247188,
#247189,#247190,#247191,#247192,#247193,#247194,#247195,#247196,#247197,
#247198,#247199,#247200,#247201,#247202,#247203,#247204,#247205,#247206,
#247207,#247208,#247209,#247210,#247211,#247212,#247213,#247214,#247215,
#247216,#247217,#247218,#247219,#247220,#247221,#247222,#247223,#247224,
#247225,#247226,#247227,#247228,#247229),.UNSPECIFIED.,.F.,.F.,(4,3,3,3,
3,3,3,3,3,3,3,3,3,3,3,3,3,3,3,3,3,3,3,3,3,3,3,3,3,3,3,3,3,3,3,3,3,3,3,3,
3,3,3,3,3,3,3,3,3,3,3,3,3,3,3,3,3,3,3,3,3,3,3,3,3,3,3,3,3,3,3,3,4),(1416.85828676918,
1416.95477822478,1417.04830595778,1417.14627927468,1417.24425259159,1417.32799130344,
1417.4116268148,1417.4951792582,1417.57866869405,1417.66212264467,1417.74555913851,
1417.82899624827,1417.91245204319,1417.99599653592,1418.07958561886,1418.16330888641,
1418.24398860231,1418.32772731416,1418.41136282552,1418.49491526892,1418.57840470477,
1418.66185865539,1418.74529514923,1418.82873225899,1418.91218805391,1418.99573254664,
1419.07932162958,1419.16304489713,1419.24372461303,1419.32746332488,1419.41109883624,
1419.49465127964,1419.57814071549,1419.66159466611,1419.74503115995,1419.82846826971,
1419.91192406463,1419.99546855736,1420.0790576403,1420.16278090785,1420.24346062375,
1420.3271993356,1420.41083484696,1420.49438729036,1420.57787672621,1420.66133067683,
1420.74476717067,1420.82820428043,1420.91166007535,1420.99520456808,1421.07879365102,
1421.16251691857,1421.24319663447,1421.32693534632,1421.41057085768,1421.49412330108,
1421.57761273693,1421.66106668755,1421.74450318139,1421.82794029115,1421.91139608607,
1421.9949405788,1422.07852966174,1422.16225292929,1422.24293264519,1422.32559622083,
1422.40816522113,1422.490658732,1422.57309577088,1422.6555052585,1422.73789637857,
1422.82031610301,1422.88963902832),.UNSPECIFIED.);
#1869=B_SPLINE_CURVE_WITH_KNOTS('',3,(#247230,#247231,#247232,#247233,#247234,
#247235,#247236,#247237,#247238,#247239),.UNSPECIFIED.,.F.,.F.,(4,3,3,4),
(1416.60760743314,1416.69191056942,1416.77619079502,1416.85828676899),
 .UNSPECIFIED.);
#1870=B_SPLINE_CURVE_WITH_KNOTS('',3,(#247245,#247246,#247247,#247248,#247249,
#247250,#247251,#247252,#247253,#247254),.UNSPECIFIED.,.F.,.F.,(4,3,3,4),
(1410.32430278068,1410.40811390766,1410.49192260022,1410.57510146181),
 .UNSPECIFIED.);
#1871=B_SPLINE_CURVE_WITH_KNOTS('',3,(#247255,#247256,#247257,#247258,#247259,
#247260,#247261,#247262,#247263,#247264,#247265,#247266,#247267,#247268,
#247269,#247270,#247271,#247272,#247273,#247274,#247275,#247276,#247277,
#247278,#247279,#247280,#247281,#247282,#247283,#247284,#247285,#247286,
#247287,#247288,#247289,#247290,#247291,#247292,#247293,#247294,#247295,
#247296,#247297,#247298,#247299,#247300,#247301,#247302,#247303,#247304,
#247305,#247306,#247307,#247308,#247309,#247310,#247311,#247312,#247313,
#247314,#247315,#247316,#247317,#247318,#247319,#247320,#247321,#247322,
#247323,#247324,#247325,#247326,#247327,#247328,#247329,#247330,#247331,
#247332,#247333,#247334,#247335,#247336,#247337,#247338,#247339,#247340,
#247341,#247342,#247343,#247344,#247345,#247346,#247347,#247348,#247349,
#247350,#247351,#247352,#247353,#247354,#247355,#247356,#247357,#247358,
#247359,#247360,#247361,#247362,#247363,#247364,#247365,#247366,#247367,
#247368,#247369,#247370,#247371,#247372,#247373,#247374,#247375,#247376,
#247377,#247378,#247379,#247380,#247381,#247382,#247383,#247384,#247385,
#247386,#247387,#247388,#247389,#247390,#247391,#247392,#247393,#247394,
#247395,#247396,#247397,#247398,#247399,#247400,#247401,#247402,#247403,
#247404,#247405,#247406,#247407,#247408,#247409,#247410,#247411,#247412,
#247413,#247414,#247415,#247416,#247417,#247418,#247419,#247420,#247421,
#247422,#247423,#247424,#247425,#247426,#247427,#247428,#247429,#247430,
#247431,#247432,#247433,#247434,#247435,#247436,#247437,#247438,#247439,
#247440,#247441,#247442,#247443,#247444,#247445,#247446,#247447,#247448,
#247449,#247450,#247451,#247452,#247453,#247454,#247455,#247456,#247457,
#247458,#247459,#247460,#247461,#247462,#247463,#247464,#247465,#247466,
#247467,#247468,#247469,#247470,#247471),.UNSPECIFIED.,.F.,.F.,(4,3,3,3,
3,3,3,3,3,3,3,3,3,3,3,3,3,3,3,3,3,3,3,3,3,3,3,3,3,3,3,3,3,3,3,3,3,3,3,3,
3,3,3,3,3,3,3,3,3,3,3,3,3,3,3,3,3,3,3,3,3,3,3,3,3,3,3,3,3,3,3,3,4),(1410.57510146201,
1410.67010500045,1410.76553206136,1410.86152504162,1410.93554590755,1411.0192846194,
1411.10292013076,1411.18647257416,1411.26996201001,1411.35341596063,1411.43685245447,
1411.52028956423,1411.60374535915,1411.68728985187,1411.77087893482,1411.85460220237,
1411.93528191827,1412.01902063012,1412.10265614148,1412.18620858488,1412.26969802073,
1412.35315197135,1412.43658846519,1412.52002557495,1412.60348136987,1412.6870258626,
1412.77061494554,1412.8543382131,1412.93501792899,1413.01875664084,1413.1023921522,
1413.1859445956,1413.26943403145,1413.35288798207,1413.43632447591,1413.51976158567,
1413.60321738059,1413.68676187332,1413.77035095626,1413.85407422381,1413.93475393971,
1414.01849265156,1414.10212816292,1414.18568060632,1414.26917004217,1414.35262399279,
1414.43606048663,1414.51949759639,1414.6029533913,1414.68649788403,1414.77008696697,
1414.85381023453,1414.93448995043,1415.01822866228,1415.10186417364,1415.18541661704,
1415.26890605289,1415.35236000351,1415.43579649735,1415.51923360711,1415.60268940203,
1415.68623389476,1415.7698229777,1415.85354624526,1415.93422596115,1416.01825423227,
1416.10099893318,1416.18366832812,1416.26628131214,1416.35132401664,1416.43389281429,
1416.52017247222,1416.60645213015),.UNSPECIFIED.);
#1872=B_SPLINE_CURVE_WITH_KNOTS('',3,(#247473,#247474,#247475,#247476,#247477,
#247478,#247479,#247480,#247481,#247482,#247483,#247484,#247485,#247486,
#247487,#247488,#247489,#247490,#247491,#247492,#247493,#247494,#247495,
#247496,#247497,#247498,#247499,#247500,#247501,#247502,#247503,#247504,
#247505,#247506,#247507,#247508,#247509,#247510,#247511,#247512,#247513,
#247514,#247515,#247516,#247517,#247518,#247519,#247520,#247521,#247522,
#247523,#247524,#247525,#247526,#247527,#247528,#247529,#247530,#247531,
#247532,#247533,#247534,#247535,#247536,#247537,#247538,#247539,#247540,
#247541,#247542,#247543,#247544,#247545,#247546,#247547,#247548,#247549,
#247550,#247551,#247552,#247553,#247554,#247555,#247556,#247557,#247558,
#247559,#247560,#247561,#247562,#247563,#247564,#247565,#247566,#247567,
#247568,#247569,#247570,#247571,#247572,#247573,#247574,#247575,#247576,
#247577,#247578,#247579,#247580,#247581,#247582,#247583,#247584,#247585,
#247586,#247587,#247588,#247589,#247590,#247591,#247592,#247593,#247594,
#247595,#247596,#247597,#247598,#247599,#247600,#247601,#247602,#247603,
#247604,#247605,#247606,#247607,#247608,#247609,#247610,#247611,#247612,
#247613,#247614,#247615,#247616,#247617,#247618,#247619,#247620,#247621,
#247622,#247623,#247624,#247625,#247626,#247627,#247628,#247629,#247630,
#247631,#247632,#247633,#247634,#247635,#247636,#247637,#247638,#247639,
#247640,#247641,#247642,#247643,#247644,#247645,#247646,#247647,#247648,
#247649,#247650,#247651,#247652,#247653,#247654,#247655,#247656,#247657,
#247658,#247659,#247660,#247661,#247662,#247663,#247664,#247665,#247666,
#247667,#247668,#247669,#247670,#247671,#247672,#247673,#247674,#247675,
#247676,#247677,#247678,#247679,#247680,#247681,#247682,#247683,#247684,
#247685,#247686,#247687,#247688,#247689,#247690,#247691,#247692),
 .UNSPECIFIED.,.F.,.F.,(4,3,3,3,3,3,3,3,3,3,3,3,3,3,3,3,3,3,3,3,3,3,3,3,
3,3,3,3,3,3,3,3,3,3,3,3,3,3,3,3,3,3,3,3,3,3,3,3,3,3,3,3,3,3,3,3,3,3,3,3,
3,3,3,3,3,3,3,3,3,3,3,3,3,4),(1410.57510146181,1410.65894334499,1410.74225529584,
1410.82557017512,1410.9089061093,1410.9931387138,1411.07661585494,1411.1612261911,
1411.24583652727,1411.32957523912,1411.41321075048,1411.49676319388,1411.58025262973,
1411.66370658035,1411.74714307419,1411.83058018395,1411.91403597887,1411.9975804716,
1412.08116955454,1412.16489282209,1412.24557253799,1412.32931124984,1412.4129467612,
1412.4964992046,1412.57998864045,1412.66344259107,1412.74687908491,1412.83031619467,
1412.91377198959,1412.99731648232,1413.08090556526,1413.16462883281,1413.24530854871,
1413.32904726056,1413.41268277192,1413.49623521532,1413.57972465117,1413.66317860179,
1413.74661509563,1413.83005220539,1413.91350800031,1413.99705249304,1414.08064157598,
1414.16436484353,1414.24504455943,1414.32878327128,1414.41241878264,1414.49597122604,
1414.57946066189,1414.66291461251,1414.74635110635,1414.82978821611,1414.91324401103,
1414.99678850376,1415.0803775867,1415.16410085425,1415.24478057015,1415.328519282,
1415.41215479336,1415.49570723676,1415.57919667261,1415.66265062323,1415.74608711707,
1415.82952422683,1415.91298002175,1415.99652451447,1416.08011359742,1416.16383686497,
1416.24451658087,1416.32920862088,1416.41375449164,1416.49821554759,1416.5825919458,
1416.60760743314),.UNSPECIFIED.);
#1873=B_SPLINE_CURVE_WITH_KNOTS('',3,(#247693,#247694,#247695,#247696,#247697,
#247698,#247699,#247700,#247701,#247702),.UNSPECIFIED.,.F.,.F.,(4,3,3,4),
(1410.3244751935,1410.42295017058,1410.52052586119,1410.57510146163),
 .UNSPECIFIED.);
#1874=B_SPLINE_CURVE_WITH_KNOTS('',3,(#247708,#247709,#247710,#247711,#247712,
#247713,#247714,#247715,#247716,#247717,#247718,#247719,#247720),
 .UNSPECIFIED.,.F.,.F.,(4,3,3,3,4),(1403.7003517852,1403.78532632359,1403.86877413941,
1403.95451203908,1404.04024993874),.UNSPECIFIED.);
#1875=B_SPLINE_CURVE_WITH_KNOTS('',3,(#247722,#247723,#247724,#247725,#247726,
#247727),.UNSPECIFIED.,.F.,.F.,(4,2,4),(1.8052198339721,1.86724042443728,
1.96119997683881),.UNSPECIFIED.);
#1876=B_SPLINE_CURVE_WITH_KNOTS('',3,(#247728,#247729,#247730,#247731,#247732,
#247733,#247734,#247735,#247736,#247737,#247738,#247739,#247740,#247741,
#247742,#247743,#247744,#247745,#247746,#247747,#247748,#247749,#247750,
#247751,#247752,#247753,#247754,#247755),.UNSPECIFIED.,.F.,.F.,(4,3,3,3,
3,3,3,3,3,4),(1403.37979373757,1403.46322854723,1403.54666922749,1403.63013384884,
1403.71368962522,1403.79729471688,1403.88102697689,1403.93739383251,1404.03402820369,
1404.04140044517),.UNSPECIFIED.);
#1877=B_SPLINE_CURVE_WITH_KNOTS('',3,(#254538,#254539,#254540,#254541,#254542,
#254543,#254544,#254545,#254546,#254547),.UNSPECIFIED.,.F.,.F.,(4,2,2,2,
4),(0.000477622210521881,0.0654985715592456,0.146298798970954,0.27193450855757,
0.311339098434402),.UNSPECIFIED.);
#1878=B_SPLINE_CURVE_WITH_KNOTS('',3,(#254549,#254550,#254551,#254552,#254553,
#254554,#254555,#254556,#254557,#254558,#254559,#254560,#254561,#254562,
#254563,#254564,#254565,#254566,#254567,#254568,#254569,#254570,#254571,
#254572,#254573,#254574,#254575,#254576,#254577,#254578,#254579,#254580,
#254581,#254582,#254583,#254584,#254585,#254586,#254587,#254588,#254589,
#254590,#254591,#254592,#254593,#254594,#254595,#254596,#254597,#254598,
#254599,#254600,#254601,#254602,#254603,#254604,#254605,#254606,#254607,
#254608,#254609),.UNSPECIFIED.,.F.,.F.,(4,3,3,3,3,3,3,3,3,3,3,3,3,3,3,3,
3,3,3,3,4),(1392.30062248289,1392.38353259545,1392.46334657938,1392.54321558283,
1392.62319000748,1392.63226293314,1392.71222023327,1392.79208303051,1392.87186885299,
1392.95159516818,1393.03127939648,1393.1109503827,1393.19061783622,1393.27029748704,
1393.35000506944,1393.42980029851,1393.50964464022,1393.58960306727,1393.63199894386,
1393.71196956209,1393.72842800165),.UNSPECIFIED.);
#1879=B_SPLINE_CURVE_WITH_KNOTS('',3,(#254610,#254611,#254612,#254613,#254614,
#254615,#254616,#254617,#254618,#254619,#254620,#254621,#254622,#254623,
#254624,#254625,#254626,#254627,#254628,#254629,#254630,#254631,#254632,
#254633,#254634,#254635,#254636,#254637,#254638,#254639,#254640,#254641),
 .UNSPECIFIED.,.F.,.F.,(4,2,2,2,2,2,2,2,2,2,2,2,2,2,2,4),(0.311339098434402,
0.384933689166427,0.397094845809577,0.39736868756705,0.397450522008619,
0.397499655154026,0.397543081273146,0.397597345360711,0.397702470611355,
0.398379451119274,0.399871523283459,0.425219733962204,0.476781426924293,
0.631008672365873,0.720388372997854,0.803428429579855),.UNSPECIFIED.);
#1880=B_SPLINE_CURVE_WITH_KNOTS('',3,(#261424,#261425,#261426,#261427,#261428,
#261429,#261430,#261431,#261432,#261433,#261434,#261435,#261436,#261437,
#261438,#261439,#261440,#261441,#261442,#261443,#261444,#261445,#261446,
#261447,#261448,#261449,#261450,#261451,#261452,#261453,#261454,#261455,
#261456,#261457,#261458,#261459,#261460,#261461),.UNSPECIFIED.,.F.,.F.,
(4,2,2,2,2,2,2,2,2,2,2,2,2,2,2,2,2,2,4),(0.00239242256924691,0.134902032668107,
0.296770312006015,0.324000698094346,0.326552911280465,0.326929349600861,
0.327178375312593,0.327616377021976,0.32773031959246,0.327805417519109,
0.327847482964747,0.327882907829789,0.327925026518018,0.328000448551939,
0.328349673398392,0.328987017831634,0.347385760741725,0.39081477612345,
0.517465670307461),.UNSPECIFIED.);
#1881=B_SPLINE_CURVE_WITH_KNOTS('',3,(#261463,#261464,#261465,#261466,#261467,
#261468,#261469,#261470,#261471,#261472,#261473,#261474,#261475,#261476,
#261477,#261478,#261479,#261480,#261481,#261482,#261483,#261484,#261485,
#261486,#261487,#261488,#261489,#261490,#261491,#261492,#261493,#261494,
#261495,#261496,#261497,#261498,#261499,#261500,#261501,#261502,#261503,
#261504,#261505),.UNSPECIFIED.,.F.,.F.,(4,3,3,3,3,3,3,3,3,3,3,3,3,3,4),
(1498.97655487521,1499.05623057304,1499.1358974584,1499.21557126196,1499.2952677155,
1499.3750496428,1499.45487593369,1499.53482369084,1499.60401608019,1499.68397970309,
1499.76385130304,1499.84363027147,1499.92335568368,1500.00304021085,1500.04731086453),
 .UNSPECIFIED.);
#1882=B_SPLINE_CURVE_WITH_KNOTS('',3,(#261506,#261507,#261508,#261509,#261510,
#261511,#261512,#261513,#261514,#261515),.UNSPECIFIED.,.F.,.F.,(4,2,2,2,
4),(6.24789745713582E-5,0.0249353959329077,0.115784953094516,0.19994556386008,
0.348086239184528),.UNSPECIFIED.);
#1883=B_SPLINE_CURVE_WITH_KNOTS('',3,(#261517,#261518,#261519,#261520,#261521,
#261522,#261523,#261524,#261525,#261526,#261527,#261528,#261529,#261530,
#261531,#261532,#261533,#261534,#261535,#261536,#261537,#261538,#261539,
#261540,#261541,#261542,#261543,#261544,#261545,#261546,#261547,#261548,
#261549,#261550,#261551,#261552,#261553,#261554,#261555,#261556,#261557,
#261558,#261559,#261560,#261561,#261562,#261563,#261564,#261565,#261566,
#261567,#261568,#261569,#261570,#261571,#261572,#261573,#261574,#261575,
#261576,#261577,#261578,#261579,#261580,#261581,#261582,#261583,#261584,
#261585,#261586,#261587,#261588,#261589,#261590,#261591,#261592,#261593,
#261594,#261595,#261596,#261597,#261598,#261599,#261600,#261601,#261602,
#261603,#261604,#261605,#261606,#261607,#261608,#261609,#261610,#261611,
#261612,#261613,#261614,#261615,#261616,#261617,#261618,#261619,#261620,
#261621,#261622,#261623,#261624,#261625,#261626,#261627,#261628,#261629,
#261630,#261631,#261632,#261633,#261634,#261635,#261636,#261637,#261638,
#261639,#261640,#261641,#261642,#261643,#261644,#261645,#261646,#261647,
#261648,#261649,#261650,#261651,#261652,#261653,#261654,#261655,#261656,
#261657,#261658,#261659,#261660,#261661,#261662,#261663,#261664,#261665,
#261666,#261667,#261668,#261669,#261670,#261671,#261672,#261673,#261674,
#261675,#261676,#261677,#261678,#261679,#261680,#261681,#261682,#261683,
#261684,#261685,#261686,#261687,#261688,#261689,#261690,#261691,#261692,
#261693,#261694,#261695,#261696,#261697,#261698,#261699,#261700,#261701,
#261702,#261703,#261704,#261705,#261706,#261707,#261708,#261709,#261710,
#261711,#261712,#261713,#261714,#261715,#261716,#261717,#261718,#261719,
#261720,#261721,#261722,#261723,#261724,#261725,#261726,#261727,#261728,
#261729,#261730,#261731,#261732,#261733,#261734,#261735,#261736),
 .UNSPECIFIED.,.F.,.F.,(4,3,3,3,3,3,3,3,3,3,3,3,3,3,3,3,3,3,3,3,3,3,3,3,
3,3,3,3,3,3,3,3,3,3,3,3,3,3,3,3,3,3,3,3,3,3,3,3,3,3,3,3,3,3,3,3,3,3,3,3,
3,3,3,3,3,3,3,3,3,3,3,3,3,4),(1404.29191615463,1404.37562428831,1404.4593290263,
1404.54304803957,1404.62679900449,1404.7106527483,1404.79456200366,1404.87860831265,
1404.93712984323,1405.02086855508,1405.10450406644,1405.18805650984,1405.27154594569,
1405.35499989631,1405.43843639015,1405.52187349991,1405.60532929482,1405.68887378755,
1405.7724628705,1405.85618613805,1405.93686585395,1406.0206045658,1406.10424007716,
1406.18779252056,1406.27128195641,1406.35473590703,1406.43817240087,1406.52160951063,
1406.60506530555,1406.68860979828,1406.77219888122,1406.85592214878,1406.93660186467,
1407.02034057652,1407.10397608788,1407.18752853128,1407.27101796713,1407.35447191775,
1407.43790841159,1407.52134552135,1407.60480131627,1407.688345809,1407.77193489194,
1407.85565815949,1407.93633787539,1408.02007658724,1408.1037120986,1408.187264542,
1408.27075397785,1408.35420792847,1408.43764442231,1408.52108153207,1408.60453732698,
1408.68808181971,1408.77167090265,1408.85539417021,1408.93607388611,1409.01981259796,
1409.10344810932,1409.18700055272,1409.27048998857,1409.35394393919,1409.43738043303,
1409.52081754279,1409.60427333771,1409.68781783044,1409.77140691338,1409.85513018094,
1409.93580989683,1410.01998705489,1410.10402428112,1410.18798093152,1410.2718608454,
1410.32430278068),.UNSPECIFIED.);
#1884=B_SPLINE_CURVE_WITH_KNOTS('',3,(#261737,#261738,#261739,#261740,#261741,
#261742,#261743,#261744,#261745,#261746),.UNSPECIFIED.,.F.,.F.,(4,3,3,4),
(1404.04140044517,1404.13747352714,1404.23285921852,1404.29191615443),
 .UNSPECIFIED.);
#1885=B_SPLINE_CURVE_WITH_KNOTS('',3,(#261748,#261749,#261750,#261751,#261752,
#261753,#261754,#261755,#261756,#261757),.UNSPECIFIED.,.F.,.F.,(4,2,2,2,
4),(0.0014226223468972,0.0413177149723191,0.0846967743397222,0.130628866228341,
0.178453317484416),.UNSPECIFIED.);
#1886=B_SPLINE_CURVE_WITH_KNOTS('',3,(#261759,#261760,#261761,#261762,#261763,
#261764,#261765,#261766,#261767,#261768,#261769,#261770,#261771,#261772,
#261773,#261774,#261775,#261776,#261777,#261778,#261779,#261780,#261781,
#261782,#261783,#261784,#261785,#261786,#261787,#261788,#261789,#261790,
#261791,#261792,#261793,#261794,#261795,#261796,#261797,#261798,#261799,
#261800,#261801,#261802,#261803,#261804),.UNSPECIFIED.,.F.,.F.,(4,3,3,3,
3,3,3,3,3,3,3,3,3,3,3,4),(1394.81425368482,1394.89402080788,1394.97373338235,
1395.05595058022,1395.13561874826,1395.21528835869,1395.29497514184,1395.37469483532,
1395.45450405754,1395.53436687025,1395.61433714781,1395.6314709653,1395.72358358603,
1395.8153650835,1395.90649484727,1395.98599303994),.UNSPECIFIED.);
#1887=B_SPLINE_CURVE_WITH_KNOTS('',3,(#261806,#261807,#261808,#261809,#261810,
#261811,#261812,#261813,#261814,#261815),.UNSPECIFIED.,.F.,.F.,(4,1,1,1,
1,1,1,4),(1395.98599328739,1396.63120697602,1397.63094298674,1398.63067899746,
1399.63041500818,1400.6301510189,1401.62988702962,1402.26917859457),
 .UNSPECIFIED.);
#1888=B_SPLINE_CURVE_WITH_KNOTS('',3,(#261817,#261818,#261819,#261820,#261821,
#261822,#261823,#261824,#261825,#261826),.UNSPECIFIED.,.F.,.F.,(4,1,1,1,
1,1,1,4),(1402.26917859457,1402.62962304034,1403.62935905106,1404.62909506178,
1405.6288310725,1406.62856708322,1407.62830309394,1408.55236390175),
 .UNSPECIFIED.);
#1889=B_SPLINE_CURVE_WITH_KNOTS('',3,(#261828,#261829,#261830,#261831,#261832,
#261833,#261834,#261835,#261836,#261837,#261838,#261839),.UNSPECIFIED.,
 .F.,.F.,(4,2,1,1,1,1,1,1,4),(1408.55236390175,1408.62803910466,1409.62777511538,
1410.6275111261,1411.62724713682,1412.62698314754,1413.62671915826,1414.62645516898,
1414.83554920893),.UNSPECIFIED.);
#1890=B_SPLINE_CURVE_WITH_KNOTS('',3,(#261841,#261842,#261843,#261844,#261845,
#261846,#261847,#261848,#261849,#261850,#261851,#261852,#261853,#261854,
#261855,#261856,#261857,#261858,#261859,#261860,#261861,#261862,#261863,
#261864,#261865,#261866,#261867,#261868,#261869,#261870,#261871,#261872,
#261873,#261874,#261875,#261876,#261877,#261878,#261879,#261880,#261881,
#261882,#261883,#261884,#261885,#261886,#261887,#261888,#261889,#261890,
#261891,#261892,#261893,#261894,#261895,#261896,#261897,#261898,#261899,
#261900,#261901,#261902,#261903,#261904,#261905,#261906,#261907,#261908,
#261909,#261910,#261911,#261912,#261913,#261914,#261915,#261916,#261917,
#261918,#261919,#261920,#261921,#261922,#261923,#261924,#261925,#261926,
#261927,#261928,#261929,#261930,#261931,#261932,#261933,#261934,#261935,
#261936,#261937,#261938,#261939,#261940,#261941,#261942,#261943,#261944,
#261945,#261946,#261947,#261948,#261949,#261950,#261951,#261952,#261953,
#261954,#261955,#261956,#261957,#261958,#261959,#261960,#261961,#261962,
#261963,#261964,#261965,#261966,#261967,#261968,#261969,#261970,#261971,
#261972,#261973,#261974,#261975,#261976,#261977,#261978,#261979,#261980,
#261981,#261982,#261983,#261984,#261985,#261986,#261987,#261988,#261989,
#261990,#261991,#261992,#261993,#261994,#261995,#261996,#261997,#261998,
#261999,#262000,#262001,#262002,#262003,#262004,#262005,#262006,#262007,
#262008,#262009,#262010,#262011,#262012,#262013,#262014,#262015,#262016,
#262017,#262018,#262019,#262020,#262021,#262022,#262023,#262024,#262025,
#262026,#262027,#262028,#262029,#262030,#262031,#262032,#262033,#262034,
#262035,#262036,#262037,#262038,#262039,#262040,#262041,#262042,#262043,
#262044,#262045,#262046,#262047,#262048,#262049,#262050,#262051,#262052,
#262053,#262054,#262055,#262056,#262057,#262058,#262059,#262060,#262061,
#262062,#262063,#262064,#262065,#262066,#262067,#262068,#262069,#262070,
#262071,#262072,#262073,#262074,#262075,#262076,#262077,#262078,#262079,
#262080,#262081,#262082,#262083,#262084),.UNSPECIFIED.,.F.,.F.,(4,3,3,3,
3,3,3,3,3,3,3,3,3,3,3,3,3,3,3,3,3,3,3,3,3,3,3,3,3,3,3,3,3,3,3,3,3,3,3,3,
3,3,3,3,3,3,3,3,3,3,3,3,3,3,3,3,3,3,3,3,3,3,3,3,3,3,3,3,3,3,3,3,3,3,3,3,
3,3,3,3,3,4),(1414.83554920893,1414.91422319859,1414.99283632039,1415.0720056778,
1415.15056272849,1415.22911755209,1415.3076866817,1415.3873128062,1415.46599905401,
1415.54609511686,1415.6261911797,1415.70614847983,1415.78601127707,1415.86579709955,
1415.94552341474,1416.02520764304,1416.10487862926,1416.18454608278,1416.2642257336,
1416.34393331599,1416.42372854507,1416.50357288678,1416.58353131382,1416.62592719042,
1416.70588449055,1416.78574728779,1416.86553311027,1416.94525942546,1417.02494365375,
1417.10461463998,1417.1842820935,1417.26396174432,1417.34366932671,1417.42346455579,
1417.5033088975,1417.58326732454,1417.62566320114,1417.70562050127,1417.78548329851,
1417.86526912099,1417.94499543618,1418.02467966447,1418.1043506507,1418.18401810422,
1418.26369775504,1418.34340533743,1418.42320056651,1418.50304490822,1418.58300333526,
1418.62539921186,1418.70535651199,1418.78521930923,1418.86500513171,1418.9447314469,
1419.0244156752,1419.10408666142,1419.18375411494,1419.26343376576,1419.34314134815,
1419.42293657723,1419.50278091894,1419.58273934598,1419.62513522258,1419.70509252271,
1419.78495531995,1419.86474114243,1419.94446745762,1420.02415168591,1420.10382267214,
1420.18349012566,1420.26316977648,1420.34287735887,1420.42267258795,1420.50251692965,
1420.5824753567,1420.6248712333,1420.70918020921,1420.79334694167,1420.8773195318,
1420.96117782697,1421.0448782206,1421.11873451598),.UNSPECIFIED.);
#1891=B_SPLINE_CURVE_WITH_KNOTS('',3,(#262086,#262087,#262088,#262089,#262090,
#262091,#262092,#262093,#262094,#262095,#262096,#262097,#262098,#262099,
#262100,#262101,#262102,#262103,#262104,#262105,#262106,#262107,#262108,
#262109,#262110,#262111,#262112,#262113,#262114,#262115,#262116,#262117,
#262118,#262119,#262120,#262121,#262122,#262123,#262124,#262125,#262126,
#262127,#262128,#262129,#262130,#262131,#262132,#262133,#262134,#262135,
#262136,#262137,#262138,#262139,#262140,#262141,#262142,#262143,#262144,
#262145,#262146,#262147,#262148,#262149,#262150,#262151,#262152,#262153,
#262154,#262155,#262156,#262157,#262158,#262159,#262160,#262161,#262162,
#262163,#262164,#262165,#262166,#262167,#262168,#262169,#262170,#262171,
#262172,#262173,#262174,#262175,#262176,#262177,#262178,#262179,#262180,
#262181,#262182,#262183,#262184,#262185,#262186,#262187,#262188,#262189,
#262190,#262191,#262192,#262193,#262194,#262195,#262196,#262197,#262198,
#262199,#262200,#262201,#262202,#262203,#262204,#262205,#262206,#262207,
#262208,#262209,#262210,#262211,#262212,#262213,#262214,#262215,#262216,
#262217,#262218,#262219,#262220,#262221,#262222,#262223,#262224,#262225,
#262226,#262227,#262228,#262229,#262230,#262231,#262232,#262233,#262234,
#262235,#262236,#262237,#262238,#262239,#262240,#262241,#262242,#262243,
#262244,#262245,#262246,#262247,#262248,#262249,#262250,#262251,#262252,
#262253,#262254,#262255,#262256,#262257,#262258,#262259,#262260,#262261,
#262262,#262263,#262264,#262265,#262266,#262267,#262268,#262269,#262270,
#262271,#262272,#262273,#262274,#262275,#262276,#262277,#262278,#262279,
#262280,#262281,#262282,#262283,#262284,#262285,#262286,#262287,#262288,
#262289,#262290,#262291,#262292,#262293,#262294,#262295,#262296,#262297,
#262298,#262299,#262300,#262301,#262302,#262303,#262304,#262305,#262306,
#262307,#262308,#262309,#262310,#262311,#262312,#262313,#262314,#262315,
#262316,#262317,#262318,#262319,#262320,#262321,#262322,#262323,#262324,
#262325,#262326,#262327,#262328,#262329),.UNSPECIFIED.,.F.,.F.,(4,3,3,3,
3,3,3,3,3,3,3,3,3,3,3,3,3,3,3,3,3,3,3,3,3,3,3,3,3,3,3,3,3,3,3,3,3,3,3,3,
3,3,3,3,3,3,3,3,3,3,3,3,3,3,3,3,3,3,3,3,3,3,3,3,3,3,3,3,3,3,3,3,3,3,3,3,
3,3,3,3,3,4),(1421.11873451611,1421.20198682774,1421.28533673185,1421.37015435989,
1421.45378598796,1421.53919661599,1421.62460724402,1421.70456454415,1421.78442734139,
1421.86421316387,1421.94393947906,1422.02362370736,1422.10329469358,1422.1829621471,
1422.26264179792,1422.34234938032,1422.42214460939,1422.5019889511,1422.58194737815,
1422.62434325474,1422.70430055487,1422.78416335211,1422.86394917459,1422.94367548978,
1423.02335971808,1423.1030307043,1423.18269815782,1423.26237780864,1423.34208539104,
1423.42188062011,1423.50172496182,1423.58168338887,1423.62407926546,1423.70403656559,
1423.78389936283,1423.8636851853,1423.9434115005,1424.02309572879,1424.10276671501,
1424.18243416854,1424.26211381936,1424.34182140175,1424.42161663083,1424.50146097253,
1424.58141939958,1424.62381527618,1424.70377257631,1424.78363537355,1424.86342119603,
1424.94314751122,1425.02283173951,1425.10250272574,1425.18217017926,1425.26184983008,
1425.34155741247,1425.42135264155,1425.50119698326,1425.5811554103,1425.6235512869,
1425.70350858703,1425.78337138427,1425.86315720674,1425.94288352194,1426.02256775023,
1426.10223873645,1426.18190618998,1426.2615858408,1426.34129342319,1426.42108865227,
1426.50093299397,1426.58089142102,1426.62328729762,1426.7021669801,1426.78095145909,
1426.85964601321,1426.93828972882,1427.01689915789,1427.09549082411,1427.17410791049,
1427.2527358973,1427.33143433151,1427.40191982329),.UNSPECIFIED.);
#1892=B_SPLINE_CURVE_WITH_KNOTS('',3,(#262331,#262332,#262333,#262334,#262335,
#262336,#262337,#262338,#262339,#262340,#262341),.UNSPECIFIED.,.F.,.F.,
(4,1,1,1,1,1,1,1,4),(1427.40191982329,1427.62302330834,1428.62275931906,
1429.62249532978,1430.6222313405,1431.62196735122,1432.62170336194,1433.62143937266,
1433.68510513047),.UNSPECIFIED.);
#1893=B_SPLINE_CURVE_WITH_KNOTS('',3,(#262343,#262344,#262345,#262346,#262347,
#262348,#262349,#262350,#262351,#262352,#262353,#262354,#262355,#262356,
#262357,#262358,#262359,#262360,#262361,#262362,#262363,#262364,#262365,
#262366,#262367,#262368,#262369,#262370,#262371,#262372,#262373,#262374,
#262375,#262376,#262377,#262378,#262379,#262380,#262381,#262382,#262383,
#262384,#262385,#262386,#262387,#262388,#262389,#262390,#262391,#262392,
#262393,#262394,#262395,#262396,#262397,#262398,#262399,#262400,#262401,
#262402,#262403,#262404,#262405,#262406,#262407,#262408,#262409,#262410,
#262411,#262412,#262413,#262414,#262415,#262416,#262417,#262418,#262419,
#262420,#262421,#262422,#262423,#262424,#262425,#262426,#262427,#262428,
#262429,#262430,#262431,#262432,#262433,#262434,#262435,#262436,#262437,
#262438,#262439,#262440,#262441,#262442,#262443,#262444,#262445,#262446,
#262447,#262448,#262449,#262450,#262451,#262452,#262453,#262454,#262455,
#262456,#262457,#262458,#262459,#262460,#262461,#262462,#262463,#262464,
#262465,#262466,#262467,#262468,#262469,#262470,#262471,#262472,#262473,
#262474,#262475,#262476,#262477,#262478,#262479,#262480,#262481,#262482,
#262483,#262484,#262485,#262486,#262487,#262488,#262489,#262490,#262491,
#262492,#262493,#262494,#262495,#262496,#262497,#262498,#262499,#262500,
#262501,#262502,#262503,#262504,#262505,#262506,#262507,#262508,#262509,
#262510,#262511,#262512,#262513,#262514,#262515,#262516,#262517,#262518,
#262519,#262520,#262521,#262522,#262523,#262524,#262525,#262526,#262527,
#262528,#262529,#262530,#262531,#262532,#262533,#262534,#262535,#262536,
#262537,#262538,#262539,#262540,#262541,#262542,#262543,#262544,#262545,
#262546,#262547,#262548,#262549,#262550,#262551,#262552,#262553,#262554,
#262555,#262556,#262557,#262558,#262559,#262560,#262561,#262562,#262563,
#262564,#262565,#262566,#262567,#262568,#262569,#262570,#262571,#262572,
#262573,#262574,#262575,#262576,#262577,#262578,#262579,#262580,#262581,
#262582,#262583,#262584,#262585,#262586),.UNSPECIFIED.,.F.,.F.,(4,3,3,3,
3,3,3,3,3,3,3,3,3,3,3,3,3,3,3,3,3,3,3,3,3,3,3,3,3,3,3,3,3,3,3,3,3,3,3,3,
3,3,3,3,3,3,3,3,3,3,3,3,3,3,3,3,3,3,3,3,3,3,3,3,3,3,3,3,3,3,3,3,3,3,3,3,
3,3,3,3,3,4),(1433.68510513047,1433.76430171396,1433.84340818076,1433.92244268633,
1434.00142332046,1434.08037593041,1434.1593155102,1434.23825835883,1434.31722077516,
1434.3962651774,1434.47535225123,1434.55455861227,1434.62117538338,1434.70113268351,
1434.78099548076,1434.86078130323,1434.94050761843,1435.02019184673,1435.09986283295,
1435.17953028648,1435.2592099373,1435.33891751969,1435.41871274877,1435.49855709048,
1435.57851551753,1435.62091139411,1435.70086869424,1435.78073149149,1435.86051731396,
1435.94024362915,1436.01992785745,1436.09959884367,1436.1792662972,1436.25894594801,
1436.33865353041,1436.41844875948,1436.49829310119,1436.57825152824,1436.62064740483,
1436.70060470496,1436.7804675022,1436.86025332467,1436.93997963987,1437.01966386816,
1437.09933485438,1437.1790023079,1437.25868195872,1437.33838954111,1437.41818477019,
1437.49802911189,1437.57798753894,1437.62038341555,1437.70034071568,1437.78020351292,
1437.8599893354,1437.93971565059,1438.01939987889,1438.09907086511,1438.17873831863,
1438.25841796945,1438.33812555185,1438.41792078092,1438.49776512263,1438.57772354968,
1438.62011942627,1438.7000767264,1438.77993952365,1438.85972534612,1438.93945166132,
1439.01913588961,1439.09880687583,1439.17847432936,1439.25815398018,1439.33786156257,
1439.41765679165,1439.49750113336,1439.57745956041,1439.61985543699,1439.71247622588,
1439.80474479726,1439.89632503004,1439.96829031496),.UNSPECIFIED.);
#1894=B_SPLINE_CURVE_WITH_KNOTS('',3,(#262588,#262589,#262590,#262591,#262592,
#262593,#262594,#262595,#262596,#262597),.UNSPECIFIED.,.F.,.F.,(4,1,1,1,
1,1,1,4),(1439.96829043765,1440.61959144771,1441.61932745843,1442.61906346915,
1443.61879947987,1444.61853549059,1445.61827150131,1446.25147574483),
 .UNSPECIFIED.);
#1895=B_SPLINE_CURVE_WITH_KNOTS('',3,(#262599,#262600,#262601,#262602,#262603,
#262604,#262605,#262606,#262607,#262608),.UNSPECIFIED.,.F.,.F.,(4,1,1,1,
1,1,1,4),(1446.25147574483,1446.61800751203,1447.61774352275,1448.61747953347,
1449.61721554419,1450.61695155491,1451.61668756563,1452.53466105201),
 .UNSPECIFIED.);
#1896=B_SPLINE_CURVE_WITH_KNOTS('',3,(#262610,#262611,#262612,#262613,#262614,
#262615,#262616,#262617,#262618,#262619,#262620,#262621),.UNSPECIFIED.,
 .F.,.F.,(4,2,1,1,1,1,1,1,4),(1452.53466105201,1452.61642357635,1453.61615958707,
1454.61589559779,1455.61563160851,1456.61536761923,1457.61510362995,1458.61483964067,
1458.81784635919),.UNSPECIFIED.);
#1897=B_SPLINE_CURVE_WITH_KNOTS('',3,(#262623,#262624,#262625,#262626,#262627,
#262628,#262629,#262630,#262631,#262632,#262633,#262634,#262635,#262636,
#262637,#262638,#262639,#262640,#262641,#262642,#262643,#262644,#262645,
#262646,#262647,#262648,#262649,#262650,#262651,#262652,#262653,#262654,
#262655,#262656,#262657,#262658,#262659,#262660,#262661,#262662,#262663,
#262664,#262665,#262666,#262667,#262668,#262669,#262670,#262671,#262672,
#262673,#262674,#262675,#262676,#262677,#262678,#262679,#262680,#262681,
#262682,#262683,#262684,#262685,#262686,#262687,#262688,#262689,#262690,
#262691,#262692,#262693,#262694,#262695,#262696,#262697,#262698,#262699,
#262700,#262701,#262702,#262703,#262704,#262705,#262706,#262707,#262708,
#262709,#262710,#262711,#262712,#262713,#262714,#262715,#262716,#262717,
#262718,#262719,#262720,#262721,#262722,#262723,#262724,#262725,#262726,
#262727,#262728,#262729,#262730,#262731,#262732,#262733,#262734,#262735,
#262736,#262737,#262738,#262739,#262740,#262741,#262742,#262743,#262744,
#262745,#262746,#262747,#262748,#262749,#262750,#262751,#262752,#262753,
#262754,#262755,#262756,#262757,#262758,#262759,#262760,#262761,#262762,
#262763,#262764,#262765,#262766,#262767,#262768,#262769,#262770,#262771,
#262772,#262773,#262774,#262775,#262776,#262777,#262778,#262779,#262780,
#262781,#262782,#262783,#262784,#262785,#262786,#262787,#262788,#262789,
#262790,#262791,#262792,#262793,#262794,#262795,#262796,#262797,#262798,
#262799,#262800,#262801,#262802,#262803,#262804,#262805,#262806,#262807,
#262808,#262809,#262810,#262811,#262812,#262813,#262814,#262815,#262816,
#262817,#262818,#262819,#262820,#262821,#262822,#262823,#262824,#262825,
#262826,#262827,#262828,#262829,#262830,#262831,#262832,#262833,#262834,
#262835,#262836,#262837,#262838,#262839,#262840,#262841,#262842,#262843,
#262844,#262845,#262846,#262847,#262848,#262849,#262850,#262851,#262852,
#262853,#262854,#262855,#262856,#262857,#262858,#262859,#262860,#262861,
#262862,#262863,#262864,#262865,#262866),.UNSPECIFIED.,.F.,.F.,(4,3,3,3,
3,3,3,3,3,3,3,3,3,3,3,3,3,3,3,3,3,3,3,3,3,3,3,3,3,3,3,3,3,3,3,3,3,3,3,3,
3,3,3,3,3,3,3,3,3,3,3,3,3,3,3,3,3,3,3,3,3,3,3,3,3,3,3,3,3,3,3,3,3,3,3,3,
3,3,3,3,3,4),(1458.81784635919,1458.89650835172,1458.97510783377,1459.05504131097,
1459.13358093235,1459.21211704093,1459.29066618012,1459.37164354793,1459.45030870812,
1459.53244217975,1459.61457565139,1459.69453295152,1459.77439574876,1459.85418157123,
1459.93390788643,1460.01359211472,1460.09326310094,1460.17293055447,1460.25261020528,
1460.33231778768,1460.41211301675,1460.49195735846,1460.57191578551,1460.61431166211,
1460.69426896224,1460.77413175948,1460.85391758195,1460.93364389715,1461.01332812544,
1461.09299911166,1461.17266656519,1461.25234621601,1461.3320537984,1461.41184902748,
1461.49169336918,1461.57165179623,1461.61404767283,1461.69400497296,1461.7738677702,
1461.85365359268,1461.93337990787,1462.01306413617,1462.09273512239,1462.17240257591,
1462.25208222673,1462.33178980913,1462.4115850382,1462.49142937991,1462.57138780696,
1462.61378368355,1462.69374098368,1462.77360378092,1462.8533896034,1462.93311591859,
1463.01280014688,1463.09247113311,1463.17213858663,1463.25181823745,1463.33152581984,
1463.41132104892,1463.49116539063,1463.57112381767,1463.61351969427,1463.6934769944,
1463.77333979164,1463.85312561412,1463.93285192931,1464.01253615761,1464.09220714383,
1464.17187459735,1464.25155424817,1464.33126183057,1464.41105705964,1464.49090140135,
1464.5708598284,1464.61325570499,1464.69780465656,1464.7822076085,1464.86640944893,
1464.95049205445,1465.03440868174,1465.10103166624),.UNSPECIFIED.);
#1898=B_SPLINE_CURVE_WITH_KNOTS('',3,(#262868,#262869,#262870,#262871,#262872,
#262873,#262874,#262875,#262876,#262877,#262878,#262879,#262880,#262881,
#262882,#262883,#262884,#262885,#262886,#262887,#262888,#262889,#262890,
#262891,#262892,#262893,#262894,#262895,#262896,#262897,#262898,#262899,
#262900,#262901,#262902,#262903,#262904,#262905,#262906,#262907,#262908,
#262909,#262910,#262911,#262912,#262913,#262914,#262915,#262916,#262917,
#262918,#262919,#262920,#262921,#262922,#262923,#262924,#262925,#262926,
#262927,#262928,#262929,#262930,#262931,#262932,#262933,#262934,#262935,
#262936,#262937,#262938,#262939,#262940,#262941,#262942,#262943,#262944,
#262945,#262946,#262947,#262948,#262949,#262950,#262951,#262952,#262953,
#262954,#262955,#262956,#262957,#262958,#262959,#262960,#262961,#262962,
#262963,#262964,#262965,#262966,#262967,#262968,#262969,#262970,#262971,
#262972,#262973,#262974,#262975,#262976,#262977,#262978,#262979,#262980,
#262981,#262982,#262983,#262984,#262985,#262986,#262987,#262988,#262989,
#262990,#262991,#262992,#262993,#262994,#262995,#262996,#262997,#262998,
#262999,#263000,#263001,#263002,#263003,#263004,#263005,#263006,#263007,
#263008,#263009,#263010,#263011,#263012,#263013,#263014,#263015,#263016,
#263017,#263018,#263019,#263020,#263021,#263022,#263023,#263024,#263025,
#263026,#263027,#263028,#263029,#263030,#263031,#263032,#263033,#263034,
#263035,#263036,#263037,#263038,#263039,#263040,#263041,#263042,#263043,
#263044,#263045,#263046,#263047,#263048,#263049,#263050,#263051,#263052,
#263053,#263054,#263055,#263056,#263057,#263058,#263059,#263060,#263061,
#263062,#263063,#263064,#263065,#263066,#263067,#263068,#263069,#263070,
#263071,#263072,#263073,#263074,#263075,#263076,#263077,#263078,#263079,
#263080,#263081,#263082,#263083,#263084,#263085,#263086,#263087,#263088,
#263089,#263090,#263091,#263092,#263093,#263094,#263095,#263096,#263097,
#263098,#263099,#263100,#263101,#263102,#263103,#263104,#263105,#263106,
#263107,#263108,#263109,#263110,#263111,#263112,#263113,#263114),
 .UNSPECIFIED.,.F.,.F.,(4,3,3,3,3,3,3,3,3,3,3,3,3,3,3,3,3,3,3,3,3,3,3,3,
3,3,3,3,3,3,3,3,3,3,3,3,3,3,3,3,3,3,3,3,3,3,3,3,3,3,3,3,3,3,3,3,3,3,3,3,
3,3,3,3,3,3,3,3,3,3,3,3,3,3,3,3,3,3,3,3,3,3,4),(1465.10103166637,1465.18408255591,
1465.26722414529,1465.3536660379,1465.43707971455,1465.52059140623,1465.60425622782,
1465.61299171571,1465.69294901584,1465.77281181308,1465.85259763555,1465.93232395075,
1466.01200817904,1466.09167916526,1466.17134661879,1466.25102626961,1466.330733852,
1466.41052908107,1466.49037342278,1466.57033184983,1466.61272772643,1466.69268502656,
1466.7725478238,1466.85233364628,1466.93205996147,1467.01174418976,1467.09141517599,
1467.17108262951,1467.25076228033,1467.33046986272,1467.4102650918,1467.49010943351,
1467.57006786055,1467.61246373715,1467.69242103728,1467.77228383452,1467.852069657,
1467.93179597219,1468.01148020049,1468.09115118671,1468.17081864023,1468.25049829105,
1468.33020587345,1468.41000110252,1468.48984544423,1468.56980387128,1468.61219974787,
1468.692157048,1468.77201984524,1468.85180566772,1468.93153198291,1469.01121621121,
1469.09088719743,1469.17055465095,1469.25023430177,1469.32994188416,1469.40973711324,
1469.48958145495,1469.56953988199,1469.61193575859,1469.69189305872,1469.77175585596,
1469.85154167844,1469.93126799363,1470.01095222192,1470.09062320815,1470.17029066167,
1470.24997031249,1470.32967789488,1470.40947312396,1470.48931746567,1470.56927589271,
1470.61167176931,1470.69058006137,1470.76939294258,1470.84811543483,1470.92678681762,
1471.00542362705,1471.08404237083,1471.16268499734,1471.24133829156,1471.32005872964,
1471.38421697355),.UNSPECIFIED.);
#1899=B_SPLINE_CURVE_WITH_KNOTS('',3,(#263116,#263117,#263118,#263119,#263120,
#263121,#263122,#263123,#263124,#263125,#263126),.UNSPECIFIED.,.F.,.F.,
(4,1,1,1,1,1,1,1,4),(1471.38421697355,1471.61140778003,1472.61114379075,
1473.61087980147,1474.61061581219,1475.61035182291,1476.61008783363,1477.60982384435,
1477.66740228073),.UNSPECIFIED.);
#1900=B_SPLINE_CURVE_WITH_KNOTS('',3,(#263128,#263129,#263130,#263131,#263132,
#263133,#263134,#263135,#263136,#263137,#263138,#263139,#263140,#263141,
#263142,#263143,#263144,#263145,#263146,#263147,#263148,#263149,#263150,
#263151,#263152,#263153,#263154,#263155,#263156,#263157,#263158,#263159,
#263160,#263161,#263162,#263163,#263164,#263165,#263166,#263167,#263168,
#263169,#263170,#263171,#263172,#263173,#263174,#263175,#263176,#263177,
#263178,#263179,#263180,#263181,#263182,#263183,#263184,#263185,#263186,
#263187,#263188,#263189,#263190,#263191,#263192,#263193,#263194,#263195,
#263196,#263197,#263198,#263199,#263200,#263201,#263202,#263203,#263204,
#263205,#263206,#263207,#263208,#263209,#263210,#263211,#263212,#263213,
#263214,#263215,#263216,#263217,#263218,#263219,#263220,#263221,#263222,
#263223,#263224,#263225,#263226,#263227,#263228,#263229,#263230,#263231,
#263232,#263233,#263234,#263235,#263236,#263237,#263238,#263239,#263240,
#263241,#263242,#263243,#263244,#263245,#263246,#263247,#263248,#263249,
#263250,#263251,#263252,#263253,#263254,#263255,#263256,#263257,#263258,
#263259,#263260,#263261,#263262,#263263,#263264,#263265,#263266,#263267,
#263268,#263269,#263270,#263271,#263272,#263273,#263274,#263275,#263276,
#263277,#263278,#263279,#263280,#263281,#263282,#263283,#263284,#263285,
#263286,#263287,#263288,#263289,#263290,#263291,#263292,#263293,#263294,
#263295,#263296,#263297,#263298,#263299,#263300,#263301,#263302,#263303,
#263304,#263305,#263306,#263307,#263308,#263309,#263310,#263311,#263312,
#263313,#263314,#263315,#263316,#263317,#263318,#263319,#263320,#263321,
#263322,#263323,#263324,#263325,#263326,#263327,#263328,#263329,#263330,
#263331,#263332,#263333,#263334,#263335,#263336,#263337,#263338,#263339,
#263340,#263341,#263342,#263343,#263344,#263345,#263346,#263347,#263348,
#263349,#263350,#263351,#263352,#263353,#263354,#263355,#263356,#263357,
#263358,#263359,#263360,#263361,#263362,#263363,#263364,#263365,#263366,
#263367,#263368,#263369,#263370,#263371),.UNSPECIFIED.,.F.,.F.,(4,3,3,3,
3,3,3,3,3,3,3,3,3,3,3,3,3,3,3,3,3,3,3,3,3,3,3,3,3,3,3,3,3,3,3,3,3,3,3,3,
3,3,3,3,3,3,3,3,3,3,3,3,3,3,3,3,3,3,3,3,3,3,3,3,3,3,3,3,3,3,3,3,3,3,3,3,
3,3,3,3,3,4),(1477.66740228073,1477.74665738145,1477.82582165558,1477.90491321944,
1477.98395012394,1478.06295794255,1478.14195194843,1478.22094840445,1478.29996357275,
1478.37906049634,1478.45819925348,1478.53745897297,1478.60955985507,1478.6895171552,
1478.76937995244,1478.84916577492,1478.92889209011,1479.00857631841,1479.08824730463,
1479.16791475815,1479.24759440897,1479.32730199136,1479.40709722044,1479.48694156215,
1479.5668999892,1479.60929586579,1479.68925316592,1479.76911596316,1479.84890178564,
1479.92862810083,1480.00831232913,1480.08798331535,1480.16765076887,1480.24733041969,
1480.32703800208,1480.40683323116,1480.48667757287,1480.56663599991,1480.60903187651,
1480.68898917664,1480.76885197388,1480.84863779636,1480.92836411155,1481.00804833985,
1481.08771932607,1481.16738677959,1481.24706643041,1481.3267740128,1481.40656924188,
1481.48641358358,1481.56637201063,1481.60876788723,1481.68872518736,1481.7685879846,
1481.84837380708,1481.92810012227,1482.00778435057,1482.08745533679,1482.16712279031,
1482.24680244113,1482.32651002352,1482.4063052526,1482.48614959431,1482.56610802135,
1482.60850389795,1482.68846119808,1482.76832399532,1482.8481098178,1482.92783613299,
1483.00752036128,1483.0871913475,1483.16685880103,1483.24653845185,1483.32624603424,
1483.40604126332,1483.48588560502,1483.56584403207,1483.60823990867,1483.70138884274,
1483.79416232008,1483.8862079791,1483.9505875878),.UNSPECIFIED.);
#1901=B_SPLINE_CURVE_WITH_KNOTS('',3,(#263373,#263374,#263375,#263376,#263377,
#263378,#263379,#263380,#263381,#263382,#263383,#263384,#263385,#263386,
#263387,#263388,#263389,#263390,#263391,#263392,#263393,#263394,#263395,
#263396,#263397,#263398,#263399,#263400,#263401,#263402,#263403,#263404,
#263405,#263406,#263407,#263408,#263409,#263410,#263411,#263412,#263413,
#263414,#263415,#263416,#263417,#263418,#263419,#263420,#263421,#263422,
#263423,#263424,#263425,#263426,#263427,#263428,#263429,#263430,#263431,
#263432,#263433,#263434,#263435,#263436,#263437,#263438,#263439,#263440,
#263441,#263442,#263443,#263444,#263445,#263446,#263447,#263448,#263449,
#263450,#263451,#263452,#263453,#263454,#263455,#263456,#263457,#263458,
#263459,#263460,#263461,#263462,#263463,#263464,#263465,#263466,#263467,
#263468,#263469,#263470,#263471,#263472,#263473,#263474,#263475,#263476,
#263477,#263478,#263479,#263480,#263481,#263482,#263483,#263484,#263485,
#263486,#263487,#263488,#263489,#263490,#263491,#263492,#263493,#263494,
#263495,#263496,#263497,#263498,#263499,#263500,#263501,#263502,#263503,
#263504,#263505,#263506,#263507,#263508,#263509,#263510,#263511,#263512,
#263513,#263514,#263515,#263516,#263517,#263518,#263519,#263520,#263521,
#263522,#263523,#263524,#263525,#263526,#263527,#263528,#263529,#263530,
#263531,#263532,#263533,#263534,#263535,#263536,#263537,#263538,#263539,
#263540,#263541,#263542,#263543,#263544,#263545,#263546,#263547,#263548,
#263549,#263550,#263551,#263552,#263553,#263554,#263555,#263556,#263557,
#263558,#263559,#263560,#263561,#263562,#263563,#263564,#263565,#263566,
#263567,#263568,#263569,#263570,#263571,#263572,#263573,#263574,#263575,
#263576,#263577,#263578,#263579,#263580,#263581,#263582,#263583,#263584,
#263585,#263586,#263587,#263588,#263589,#263590,#263591,#263592,#263593,
#263594,#263595,#263596,#263597,#263598,#263599,#263600,#263601,#263602,
#263603,#263604,#263605,#263606,#263607,#263608,#263609,#263610,#263611,
#263612,#263613,#263614,#263615,#263616,#263617,#263618,#263619),
 .UNSPECIFIED.,.F.,.F.,(4,3,3,3,3,3,3,3,3,3,3,3,3,3,3,3,3,3,3,3,3,3,3,3,
3,3,3,3,3,3,3,3,3,3,3,3,3,3,3,3,3,3,3,3,3,3,3,3,3,3,3,3,3,3,3,3,3,3,3,3,
3,3,3,3,3,3,3,3,3,3,3,3,3,3,3,3,3,3,3,3,3,3,4),(1483.95058758791,1484.03276112934,
1484.11249874285,1484.19224360271,1484.27201130001,1484.35600245486,1484.43590835349,
1484.5158731071,1484.59594982076,1484.60797591939,1484.68793321952,1484.76779601676,
1484.84758183924,1484.92730815443,1485.00699238273,1485.08666336895,1485.16633082247,
1485.24601047329,1485.32571805569,1485.40551328476,1485.48535762647,1485.56531605352,
1485.60771193011,1485.68766923024,1485.76753202748,1485.84731784996,1485.92704416515,
1486.00672839345,1486.08639937967,1486.16606683319,1486.24574648401,1486.3254540664,
1486.40524929548,1486.48509363719,1486.56505206424,1486.60744794083,1486.68740524096,
1486.7672680382,1486.84705386067,1486.92678017587,1487.00646440416,1487.08613539038,
1487.16580284391,1487.24548249473,1487.32519007712,1487.40498530619,1487.4848296479,
1487.56478807495,1487.60718395155,1487.68714125168,1487.76700404892,1487.8467898714,
1487.92651618659,1488.00620041488,1488.08587140111,1488.16553885463,1488.24521850545,
1488.32492608784,1488.40472131692,1488.48456565863,1488.56452408567,1488.60691996227,
1488.6868772624,1488.76674005964,1488.84652588211,1488.92625219731,1489.0059364256,
1489.08560741182,1489.16527486535,1489.24495451617,1489.32466209856,1489.40445732764,
1489.48430166934,1489.56426009639,1489.60665597299,1489.68722612258,1489.7676985561,
1489.84808846144,1489.92841097225,1490.00867685395,1490.08890876417,1490.16913181602,
1490.23377289509),.UNSPECIFIED.);
#1902=B_SPLINE_CURVE_WITH_KNOTS('',3,(#263621,#263622,#263623,#263624,#263625,
#263626,#263627,#263628,#263629,#263630),.UNSPECIFIED.,.F.,.F.,(4,1,1,1,
1,1,1,4),(1490.233780566,1490.60639198371,1491.60612799443,1492.60586400515,
1493.60560001587,1494.60533602659,1495.60507203731,1496.5169494552),
 .UNSPECIFIED.);
#1903=B_SPLINE_CURVE_WITH_KNOTS('',3,(#263631,#263632,#263633,#263634,#263635,
#263636,#263637,#263638,#263639,#263640,#263641,#263642,#263643,#263644,
#263645,#263646,#263647,#263648,#263649,#263650,#263651,#263652,#263653,
#263654,#263655,#263656,#263657,#263658,#263659,#263660,#263661,#263662,
#263663,#263664,#263665,#263666,#263667,#263668,#263669,#263670),
 .UNSPECIFIED.,.F.,.F.,(4,3,3,3,3,3,3,3,3,3,3,3,3,4),(1496.51695820227,
1496.60480804803,1496.68476866345,1496.76463404788,1496.84442173243,1496.92414918687,
1497.00383691716,1497.08350435156,1497.16316722471,1497.24284126536,1497.32258142435,
1497.40235613046,1497.48223246019,1497.54400219811),.UNSPECIFIED.);
#1904=B_SPLINE_CURVE_WITH_KNOTS('',3,(#263673,#263674,#263675,#263676,#263677,
#263678),.UNSPECIFIED.,.F.,.F.,(4,2,4),(1.41357350471954,1.57818585554697,
1.60627031745981),.UNSPECIFIED.);
#1905=B_SPLINE_CURVE_WITH_KNOTS('',3,(#263680,#263681,#263682,#263683),
 .UNSPECIFIED.,.F.,.F.,(4,4),(0.488654425026599,0.592941394652162),
 .UNSPECIFIED.);
#1906=B_SPLINE_CURVE_WITH_KNOTS('',3,(#263684,#263685,#263686,#263687,#263688,
#263689),.UNSPECIFIED.,.F.,.F.,(4,1,1,4),(-1397.04440853625,-1396.63120697602,
-1395.6314709653,-1395.09571822406),.UNSPECIFIED.);
#1907=B_SPLINE_CURVE_WITH_KNOTS('',3,(#263692,#263693,#263694,#263695),
 .UNSPECIFIED.,.F.,.F.,(4,4),(0.311200159847851,0.413415476057656),
 .UNSPECIFIED.);
#1908=B_SPLINE_CURVE_WITH_KNOTS('',3,(#263697,#263698,#263699,#263700,#263701,
#263702),.UNSPECIFIED.,.F.,.F.,(4,2,4),(1.8681568300393,2.02932516755897,
2.03144978473733),.UNSPECIFIED.);
#1909=B_SPLINE_CURVE_WITH_KNOTS('',3,(#263704,#263705,#263706,#263707,#263708,
#263709),.UNSPECIFIED.,.F.,.F.,(4,1,1,4),(-1398.9596726741,-1398.63067899746,
-1397.63094298674,-1397.50325618979),.UNSPECIFIED.);
#1910=B_SPLINE_CURVE_WITH_KNOTS('',3,(#263711,#263712,#263713,#263714,#263715,
#263716,#263717,#263718,#263719,#263720,#263721,#263722,#263723,#263724,
#263725,#263726,#263727,#263728,#263729,#263730,#263731,#263732,#263733,
#263734,#263735,#263736,#263737,#263738,#263739,#263740,#263741,#263742,
#263743,#263744,#263745,#263746,#263747,#263748,#263749,#263750,#263751,
#263752,#263753,#263754,#263755,#263756,#263757,#263758,#263759,#263760,
#263761,#263762,#263763,#263764,#263765,#263766,#263767,#263768,#263769,
#263770,#263771,#263772,#263773,#263774,#263775,#263776,#263777,#263778,
#263779,#263780,#263781,#263782,#263783,#263784,#263785,#263786,#263787,
#263788,#263789,#263790,#263791,#263792,#263793,#263794,#263795,#263796,
#263797,#263798,#263799,#263800,#263801,#263802,#263803,#263804,#263805,
#263806,#263807,#263808,#263809,#263810,#263811,#263812,#263813,#263814,
#263815,#263816,#263817,#263818,#263819,#263820,#263821,#263822,#263823,
#263824,#263825,#263826,#263827,#263828,#263829,#263830,#263831,#263832,
#263833,#263834,#263835,#263836,#263837,#263838,#263839,#263840,#263841,
#263842,#263843,#263844,#263845,#263846,#263847,#263848,#263849,#263850,
#263851,#263852,#263853,#263854,#263855,#263856,#263857,#263858,#263859,
#263860,#263861,#263862,#263863,#263864,#263865,#263866,#263867,#263868,
#263869,#263870,#263871,#263872,#263873,#263874,#263875,#263876,#263877,
#263878,#263879,#263880,#263881,#263882,#263883,#263884,#263885,#263886,
#263887,#263888,#263889,#263890,#263891,#263892,#263893,#263894,#263895,
#263896,#263897,#263898,#263899,#263900,#263901,#263902,#263903,#263904,
#263905,#263906,#263907,#263908,#263909,#263910,#263911,#263912,#263913,
#263914,#263915,#263916,#263917,#263918,#263919,#263920,#263921,#263922,
#263923,#263924,#263925,#263926,#263927,#263928,#263929,#263930,#263931,
#263932,#263933,#263934,#263935,#263936,#263937,#263938,#263939,#263940,
#263941,#263942,#263943,#263944,#263945,#263946,#263947,#263948,#263949,
#263950,#263951,#263952,#263953,#263954,#263955,#263956,#263957),
 .UNSPECIFIED.,.F.,.F.,(4,3,3,3,3,3,3,3,3,3,3,3,3,3,3,3,3,3,3,3,3,3,3,3,
3,3,3,3,3,3,3,3,3,3,3,3,3,3,3,3,3,3,3,3,3,3,3,3,3,3,3,3,3,3,3,3,3,3,3,3,
3,3,3,3,3,3,3,3,3,3,3,3,3,3,3,3,3,3,3,3,3,3,4),(-1405.2428652499,-1405.16239569195,
-1405.08191404014,-1405.00140562355,-1404.92085575786,-1404.840199036,-1404.75948345872,
-1404.67863759454,-1404.62909506178,-1404.54913776165,-1404.46927496441,
-1404.38948914194,-1404.30976282674,-1404.23007859845,-1404.15040761223,
-1404.0707401587,-1403.99106050789,-1403.9113529255,-1403.83155769642,-1403.75171335471,
-1403.67175492767,-1403.62935905106,-1403.54940175093,-1403.46953895369,
-1403.38975313121,-1403.31002681602,-1403.23034258773,-1403.1506716015,
-1403.07100414798,-1402.99132449716,-1402.91161691477,-1402.83182168569,
-1402.75197734399,-1402.67201891694,-1402.62962304034,-1402.54966574021,
-1402.46980294297,-1402.39001712049,-1402.3102908053,-1402.230606577,-1402.15093559078,
-1402.07126813726,-1401.99158848644,-1401.91188090405,-1401.83208567497,
-1401.75224133326,-1401.67228290621,-1401.62988702962,-1401.54992972949,
-1401.47006693225,-1401.39028110977,-1401.31055479458,-1401.23087056629,
-1401.15119958006,-1401.07153212654,-1400.99185247572,-1400.91214489333,
-1400.83234966425,-1400.75250532255,-1400.6725468955,-1400.6301510189,-1400.55019371877,
-1400.47033092153,-1400.39054509905,-1400.31081878386,-1400.23113455556,
-1400.15146356934,-1400.07179611582,-1399.992116465,-1399.9124088826,-1399.83261365353,
-1399.75276931182,-1399.67281088477,-1399.63041500818,-1399.546573125,-1399.46682601498,
-1399.38715383661,-1399.30754071169,-1399.22797080243,-1399.14842137439,
-1399.0688836793,-1398.98932729873,-1398.95967994272),.UNSPECIFIED.);
#1911=B_SPLINE_CURVE_WITH_KNOTS('',3,(#263959,#263960,#263961,#263962,#263963,
#263964,#263965,#263966,#263967,#263968),.UNSPECIFIED.,.F.,.F.,(4,1,1,1,
1,1,1,4),(-1411.52604145674,-1410.62751112611,-1409.62777511538,-1408.62803910466,
-1407.62830309394,-1406.62856708322,-1405.6288310725,-1405.24287268663),
 .UNSPECIFIED.);
#1912=B_SPLINE_CURVE_WITH_KNOTS('',3,(#263970,#263971,#263972,#263973,#263974,
#263975,#263976,#263977,#263978,#263979,#263980,#263981,#263982,#263983,
#263984,#263985,#263986,#263987,#263988,#263989,#263990,#263991,#263992,
#263993,#263994,#263995,#263996,#263997,#263998,#263999,#264000,#264001,
#264002,#264003,#264004,#264005,#264006,#264007,#264008,#264009,#264010,
#264011,#264012,#264013,#264014,#264015,#264016,#264017,#264018,#264019,
#264020,#264021,#264022,#264023,#264024,#264025,#264026,#264027,#264028,
#264029,#264030,#264031,#264032,#264033,#264034,#264035,#264036,#264037,
#264038,#264039,#264040,#264041,#264042,#264043,#264044,#264045,#264046,
#264047,#264048,#264049,#264050,#264051,#264052,#264053,#264054,#264055,
#264056,#264057,#264058,#264059,#264060,#264061,#264062,#264063,#264064,
#264065,#264066,#264067,#264068,#264069,#264070,#264071,#264072,#264073,
#264074,#264075,#264076,#264077,#264078,#264079,#264080,#264081,#264082,
#264083,#264084,#264085,#264086,#264087,#264088,#264089,#264090,#264091,
#264092,#264093,#264094,#264095,#264096,#264097,#264098,#264099,#264100,
#264101,#264102,#264103,#264104,#264105,#264106,#264107,#264108,#264109,
#264110,#264111,#264112,#264113,#264114,#264115,#264116,#264117,#264118,
#264119,#264120,#264121,#264122,#264123,#264124,#264125,#264126,#264127,
#264128,#264129,#264130,#264131,#264132,#264133,#264134,#264135,#264136,
#264137,#264138,#264139,#264140,#264141,#264142,#264143,#264144,#264145,
#264146,#264147,#264148,#264149,#264150,#264151,#264152,#264153,#264154,
#264155,#264156,#264157,#264158,#264159,#264160,#264161,#264162,#264163,
#264164,#264165,#264166,#264167,#264168,#264169,#264170,#264171,#264172,
#264173,#264174,#264175,#264176,#264177,#264178,#264179,#264180,#264181,
#264182,#264183,#264184,#264185,#264186,#264187,#264188,#264189,#264190,
#264191,#264192,#264193,#264194,#264195,#264196,#264197,#264198,#264199,
#264200,#264201,#264202,#264203,#264204,#264205,#264206,#264207,#264208,
#264209,#264210,#264211,#264212,#264213),.UNSPECIFIED.,.F.,.F.,(4,3,3,3,
3,3,3,3,3,3,3,3,3,3,3,3,3,3,3,3,3,3,3,3,3,3,3,3,3,3,3,3,3,3,3,3,3,3,3,3,
3,3,3,3,3,3,3,3,3,3,3,3,3,3,3,3,3,3,3,3,3,3,3,3,3,3,3,3,3,3,3,3,3,3,3,3,
3,3,3,3,3,4),(-1417.80923586426,-1417.689114353,-1417.62566320115,-1417.54570590102,
-1417.46584310378,-1417.3860572813,-1417.30633096611,-1417.22664673781,
-1417.14697575159,-1417.06730829807,-1416.98762864725,-1416.90792106486,
-1416.82812583578,-1416.74828149407,-1416.66832306702,-1416.62592719043,
-1416.5459698903,-1416.46610709306,-1416.38632127058,-1416.30659495539,
-1416.22691072709,-1416.14723974087,-1416.06757228735,-1415.98789263653,
-1415.90818505414,-1415.82838982506,-1415.74854548335,-1415.66858705631,
-1415.62619117971,-1415.54623387958,-1415.46637108234,-1415.38658525986,
-1415.30685894467,-1415.22717471637,-1415.14750373015,-1415.06783627663,
-1414.98815662581,-1414.90844904342,-1414.82865381434,-1414.74880947263,
-1414.66885104559,-1414.62645516899,-1414.54649786886,-1414.46663507162,
-1414.38684924914,-1414.30712293395,-1414.22743870566,-1414.14776771943,
-1414.06810026591,-1413.98842061509,-1413.9087130327,-1413.82891780362,
-1413.74907346191,-1413.66911503487,-1413.62671915827,-1413.54676185814,
-1413.4668990609,-1413.38711323842,-1413.30738692323,-1413.22770269494,
-1413.14803170871,-1413.06836425519,-1412.98868460437,-1412.90897702198,
-1412.8291817929,-1412.74933745119,-1412.66937902415,-1412.62698314755,
-1412.54702584742,-1412.46716305018,-1412.38737722771,-1412.30765091251,
-1412.22796668422,-1412.148295698,-1412.06862824447,-1411.98894859366,-1411.90924101126,
-1411.82944578219,-1411.74960144048,-1411.66964301343,-1411.62724713683,
-1411.52605055708),.UNSPECIFIED.);
#1913=B_SPLINE_CURVE_WITH_KNOTS('',3,(#264215,#264216,#264217,#264218,#264219,
#264220,#264221,#264222,#264223,#264224),.UNSPECIFIED.,.F.,.F.,(4,1,1,1,
1,1,1,4),(-1424.09242117144,-1423.62407926547,-1422.62434325475,-1421.62460724403,
-1420.62487123331,-1419.62513522259,-1418.62539921187,-1417.80924068802),
 .UNSPECIFIED.);
#1914=B_SPLINE_CURVE_WITH_KNOTS('',3,(#264226,#264227,#264228,#264229,#264230,
#264231,#264232,#264233,#264234,#264235),.UNSPECIFIED.,.F.,.F.,(4,1,1,1,
1,1,1,4),(-1430.37560647862,-1429.62249532979,-1428.62275931907,-1427.62302330835,
-1426.62328729763,-1425.62355128691,-1424.62381527619,-1424.09242117144),
 .UNSPECIFIED.);
#1915=B_SPLINE_CURVE_WITH_KNOTS('',3,(#264237,#264238,#264239,#264240,#264241,
#264242,#264243,#264244,#264245,#264246,#264247,#264248,#264249,#264250,
#264251,#264252,#264253,#264254,#264255,#264256,#264257,#264258,#264259,
#264260,#264261,#264262,#264263,#264264,#264265,#264266,#264267,#264268,
#264269,#264270,#264271,#264272,#264273,#264274,#264275,#264276,#264277,
#264278,#264279,#264280,#264281,#264282,#264283,#264284,#264285,#264286,
#264287,#264288,#264289,#264290,#264291,#264292,#264293,#264294,#264295,
#264296,#264297,#264298,#264299,#264300,#264301,#264302,#264303,#264304,
#264305,#264306,#264307,#264308,#264309,#264310,#264311,#264312,#264313,
#264314,#264315,#264316,#264317,#264318,#264319,#264320,#264321,#264322,
#264323,#264324,#264325,#264326,#264327,#264328,#264329,#264330,#264331,
#264332,#264333,#264334,#264335,#264336,#264337,#264338,#264339,#264340,
#264341,#264342,#264343,#264344,#264345,#264346,#264347,#264348,#264349,
#264350,#264351,#264352,#264353,#264354,#264355,#264356,#264357,#264358,
#264359,#264360,#264361,#264362,#264363,#264364,#264365,#264366,#264367,
#264368,#264369,#264370,#264371,#264372,#264373,#264374,#264375,#264376,
#264377,#264378,#264379,#264380,#264381,#264382,#264383,#264384,#264385,
#264386,#264387,#264388,#264389,#264390,#264391,#264392,#264393,#264394,
#264395,#264396,#264397,#264398,#264399,#264400,#264401,#264402,#264403,
#264404,#264405,#264406,#264407,#264408,#264409,#264410,#264411,#264412,
#264413,#264414,#264415,#264416,#264417,#264418,#264419,#264420,#264421,
#264422,#264423,#264424,#264425,#264426,#264427,#264428,#264429,#264430,
#264431,#264432,#264433,#264434,#264435,#264436,#264437,#264438,#264439,
#264440,#264441,#264442,#264443,#264444,#264445,#264446,#264447,#264448,
#264449,#264450,#264451,#264452,#264453,#264454,#264455,#264456,#264457,
#264458,#264459,#264460,#264461,#264462,#264463,#264464,#264465,#264466,
#264467,#264468,#264469,#264470,#264471,#264472,#264473,#264474,#264475,
#264476,#264477,#264478,#264479,#264480,#264481,#264482,#264483),
 .UNSPECIFIED.,.F.,.F.,(4,3,3,3,3,3,3,3,3,3,3,3,3,3,3,3,3,3,3,3,3,3,3,3,
3,3,3,3,3,3,3,3,3,3,3,3,3,3,3,3,3,3,3,3,3,3,3,3,3,3,3,3,3,3,3,3,3,3,3,3,
3,3,3,3,3,3,3,3,3,3,3,3,3,3,3,3,3,3,3,3,3,3,4),(-1436.6587917858,-1436.62064740483,
-1436.5406901047,-1436.46082730746,-1436.38104148498,-1436.30131516979,
-1436.22163094149,-1436.14195995527,-1436.06229250175,-1435.98261285093,
-1435.90290526854,-1435.82311003946,-1435.74326569775,-1435.66330727071,
-1435.62091139411,-1435.54095409398,-1435.46109129674,-1435.38130547426,
-1435.30157915907,-1435.22189493077,-1435.14222394455,-1435.06255649103,
-1434.98287684021,-1434.90316925782,-1434.82337402874,-1434.74352968703,
-1434.66357125999,-1434.62117538339,-1434.54121808326,-1434.46135528602,
-1434.38156946354,-1434.30184314835,-1434.22215892005,-1434.14248793383,
-1434.06282048031,-1433.98314082949,-1433.9034332471,-1433.82363801802,
-1433.74379367631,-1433.66383524926,-1433.62143937267,-1433.54148207254,
-1433.4616192753,-1433.38183345282,-1433.30210713763,-1433.22242290934,
-1433.14275192312,-1433.06308446959,-1432.98340481877,-1432.90369723638,
-1432.8239020073,-1432.7440576656,-1432.66409923855,-1432.62170336195,-1432.54174606182,
-1432.46188326458,-1432.3820974421,-1432.30237112691,-1432.22268689861,
-1432.14301591239,-1432.06334845887,-1431.98366880805,-1431.90396122566,
-1431.82416599658,-1431.74432165487,-1431.66436322783,-1431.62196735123,
-1431.5420100511,-1431.46214725386,-1431.38236143138,-1431.30263511619,
-1431.2229508879,-1431.14327990167,-1431.06361244815,-1430.98393279733,
-1430.90422521494,-1430.82442998586,-1430.74458564415,-1430.66462721711,
-1430.62223134051,-1430.51675163816,-1430.41361228529,-1430.37560656682),
 .UNSPECIFIED.);
#1916=B_SPLINE_CURVE_WITH_KNOTS('',3,(#264485,#264486,#264487,#264488,#264489,
#264490,#264491,#264492,#264493,#264494),.UNSPECIFIED.,.F.,.F.,(4,1,1,1,
1,1,1,4),(-1442.94197709298,-1442.61906346915,-1441.61932745843,-1440.61959144771,
-1439.61985543699,-1438.62011942627,-1437.62038341555,-1436.65879704426),
 .UNSPECIFIED.);
#1917=B_SPLINE_CURVE_WITH_KNOTS('',3,(#264496,#264497,#264498,#264499,#264500,
#264501,#264502,#264503,#264504,#264505),.UNSPECIFIED.,.F.,.F.,(4,1,1,1,
1,1,1,4),(-1449.22516240016,-1448.61747953347,-1447.61774352275,-1446.61800751203,
-1445.61827150131,-1444.61853549059,-1443.61879947987,-1442.94197709298),
 .UNSPECIFIED.);
#1918=B_SPLINE_CURVE_WITH_KNOTS('',3,(#264507,#264508,#264509,#264510,#264511,
#264512,#264513,#264514,#264515,#264516),.UNSPECIFIED.,.F.,.F.,(4,1,1,1,
1,1,1,4),(-1455.50834770734,-1454.61589559779,-1453.61615958707,-1452.61642357635,
-1451.61668756563,-1450.61695155491,-1449.61721554419,-1449.22516240016),
 .UNSPECIFIED.);
#1919=B_SPLINE_CURVE_WITH_KNOTS('',3,(#264518,#264519,#264520,#264521,#264522,
#264523,#264524,#264525,#264526,#264527,#264528,#264529),.UNSPECIFIED.,
 .F.,.F.,(4,2,1,1,1,1,1,1,4),(-1461.79153301452,-1461.61404767283,-1460.61431166211,
-1459.61457565139,-1458.61483964067,-1457.61510362995,-1456.61536761923,
-1455.61563160851,-1455.50834770734),.UNSPECIFIED.);
#1920=B_SPLINE_CURVE_WITH_KNOTS('',3,(#264531,#264532,#264533,#264534,#264535,
#264536,#264537,#264538,#264539,#264540,#264541,#264542,#264543,#264544,
#264545,#264546,#264547,#264548,#264549,#264550,#264551,#264552,#264553,
#264554,#264555,#264556,#264557,#264558,#264559,#264560,#264561,#264562,
#264563,#264564,#264565,#264566,#264567,#264568,#264569,#264570,#264571,
#264572,#264573,#264574,#264575,#264576,#264577,#264578,#264579,#264580,
#264581,#264582,#264583,#264584,#264585,#264586,#264587,#264588,#264589,
#264590,#264591,#264592,#264593,#264594,#264595,#264596,#264597,#264598,
#264599,#264600,#264601,#264602,#264603,#264604,#264605,#264606,#264607,
#264608,#264609,#264610,#264611,#264612,#264613,#264614,#264615,#264616,
#264617,#264618,#264619,#264620,#264621,#264622,#264623,#264624,#264625,
#264626,#264627,#264628,#264629,#264630,#264631,#264632,#264633,#264634,
#264635,#264636,#264637,#264638,#264639,#264640,#264641,#264642,#264643,
#264644,#264645,#264646,#264647,#264648,#264649,#264650,#264651,#264652,
#264653,#264654,#264655,#264656,#264657,#264658,#264659,#264660,#264661,
#264662,#264663,#264664,#264665,#264666,#264667,#264668,#264669,#264670,
#264671,#264672,#264673,#264674,#264675,#264676,#264677,#264678,#264679,
#264680,#264681,#264682,#264683,#264684,#264685,#264686,#264687,#264688,
#264689,#264690,#264691,#264692,#264693,#264694,#264695,#264696,#264697,
#264698,#264699,#264700,#264701,#264702,#264703,#264704,#264705,#264706,
#264707,#264708,#264709,#264710,#264711,#264712,#264713,#264714,#264715,
#264716,#264717,#264718,#264719,#264720,#264721,#264722,#264723,#264724,
#264725,#264726,#264727,#264728,#264729,#264730,#264731,#264732,#264733,
#264734,#264735,#264736,#264737,#264738,#264739,#264740,#264741,#264742,
#264743,#264744,#264745,#264746,#264747,#264748,#264749,#264750,#264751,
#264752,#264753,#264754,#264755,#264756,#264757,#264758,#264759,#264760,
#264761,#264762,#264763,#264764,#264765,#264766,#264767,#264768,#264769,
#264770,#264771,#264772,#264773,#264774,#264775,#264776,#264777),
 .UNSPECIFIED.,.F.,.F.,(4,3,3,3,3,3,3,3,3,3,3,3,3,3,3,3,3,3,3,3,3,3,3,3,
3,3,3,3,3,3,3,3,3,3,3,3,3,3,3,3,3,3,3,3,3,3,3,3,3,3,3,3,3,3,3,3,3,3,3,3,
3,3,3,3,3,3,3,3,3,3,3,3,3,3,3,3,3,3,3,3,3,3,4),(-1468.07471811664,-1467.98983128614,
-1467.9047850356,-1467.81949107158,-1467.73406381551,-1467.64842972939,
-1467.61246373715,-1467.53250643702,-1467.45264363978,-1467.37285781731,
-1467.29313150212,-1467.21344727382,-1467.1337762876,-1467.05410883408,
-1466.97442918327,-1466.89472160087,-1466.8149263718,-1466.73508203009,
-1466.65512360305,-1466.61272772643,-1466.5327704263,-1466.45290762906,
-1466.37312180658,-1466.29339549139,-1466.2137112631,-1466.13404027688,
-1466.05437282335,-1465.97469317253,-1465.89498559014,-1465.81519036106,
-1465.73534601936,-1465.65538759231,-1465.61299171571,-1465.53303441558,
-1465.45317161834,-1465.37338579586,-1465.29365948067,-1465.21397525237,
-1465.13430426615,-1465.05463681262,-1464.97495716181,-1464.89524957941,
-1464.81545435034,-1464.73561000863,-1464.65565158158,-1464.61325570499,
-1464.53329840486,-1464.45343560762,-1464.37364978514,-1464.29392346995,
-1464.21423924166,-1464.13456825544,-1464.05490080191,-1463.97522115109,
-1463.8955135687,-1463.81571833962,-1463.73587399792,-1463.65591557087,
-1463.61351969427,-1463.53356239414,-1463.4536995969,-1463.37391377442,
-1463.29418745923,-1463.21450323093,-1463.13483224471,-1463.05516479119,
-1462.97548514037,-1462.89577755797,-1462.8159823289,-1462.73613798719,
-1462.65617956014,-1462.61378368355,-1462.53501718464,-1462.45634485605,
-1462.37774820447,-1462.29921262633,-1462.22070988667,-1462.14222340191,
-1462.06373660319,-1461.98520236571,-1461.90664134508,-1461.82800041734,
-1461.79153301452),.UNSPECIFIED.);
#1921=B_SPLINE_CURVE_WITH_KNOTS('',3,(#264779,#264780,#264781,#264782,#264783,
#264784,#264785,#264786,#264787,#264788),.UNSPECIFIED.,.F.,.F.,(4,1,1,1,
1,1,1,4),(-1474.35790362888,-1473.61087980147,-1472.61114379075,-1471.61140778003,
-1470.61167176931,-1469.61193575859,-1468.61219974787,-1468.0747183217),
 .UNSPECIFIED.);
#1922=B_SPLINE_CURVE_WITH_KNOTS('',3,(#264790,#264791,#264792,#264793,#264794,
#264795,#264796,#264797,#264798,#264799,#264800,#264801,#264802,#264803,
#264804,#264805,#264806,#264807,#264808,#264809,#264810,#264811,#264812,
#264813,#264814,#264815,#264816,#264817,#264818,#264819,#264820,#264821,
#264822,#264823,#264824,#264825,#264826,#264827,#264828,#264829,#264830,
#264831,#264832,#264833,#264834,#264835,#264836,#264837,#264838,#264839,
#264840,#264841,#264842,#264843,#264844,#264845,#264846,#264847,#264848,
#264849,#264850,#264851,#264852,#264853,#264854,#264855,#264856,#264857,
#264858,#264859,#264860,#264861,#264862,#264863,#264864,#264865,#264866,
#264867,#264868,#264869,#264870,#264871,#264872,#264873,#264874,#264875,
#264876,#264877,#264878,#264879,#264880,#264881,#264882,#264883,#264884,
#264885,#264886,#264887,#264888,#264889,#264890,#264891,#264892,#264893,
#264894,#264895,#264896,#264897,#264898,#264899,#264900,#264901,#264902,
#264903,#264904,#264905,#264906,#264907,#264908,#264909,#264910,#264911,
#264912,#264913,#264914,#264915,#264916,#264917,#264918,#264919,#264920,
#264921,#264922,#264923,#264924,#264925,#264926,#264927,#264928,#264929,
#264930,#264931,#264932,#264933,#264934,#264935,#264936,#264937,#264938,
#264939,#264940,#264941,#264942,#264943,#264944,#264945,#264946,#264947,
#264948,#264949,#264950,#264951,#264952,#264953,#264954,#264955,#264956,
#264957,#264958,#264959,#264960,#264961,#264962,#264963,#264964,#264965,
#264966,#264967,#264968,#264969,#264970,#264971,#264972,#264973,#264974,
#264975,#264976,#264977,#264978,#264979,#264980,#264981,#264982,#264983,
#264984,#264985,#264986,#264987,#264988,#264989,#264990,#264991,#264992,
#264993,#264994,#264995,#264996,#264997,#264998,#264999,#265000,#265001,
#265002,#265003,#265004,#265005,#265006,#265007,#265008,#265009,#265010,
#265011,#265012,#265013,#265014,#265015,#265016,#265017,#265018,#265019,
#265020,#265021,#265022,#265023,#265024,#265025,#265026,#265027,#265028,
#265029,#265030,#265031,#265032,#265033,#265034,#265035,#265036),
 .UNSPECIFIED.,.F.,.F.,(4,3,3,3,3,3,3,3,3,3,3,3,3,3,3,3,3,3,3,3,3,3,3,3,
3,3,3,3,3,3,3,3,3,3,3,3,3,3,3,3,3,3,3,3,3,3,3,3,3,3,3,3,3,3,3,3,3,3,3,3,
3,3,3,3,3,3,3,3,3,3,3,3,3,3,3,3,3,3,3,3,3,3,4),(-1480.64108893606,-1480.60903187651,
-1480.52907457638,-1480.44921177914,-1480.36942595667,-1480.28969964147,
-1480.21001541318,-1480.13034442696,-1480.05067697343,-1479.97099732262,
-1479.89128974022,-1479.81149451115,-1479.73165016944,-1479.6516917424,
-1479.60929586579,-1479.52933856566,-1479.44947576842,-1479.36968994594,
-1479.28996363075,-1479.21027940245,-1479.13060841623,-1479.05094096271,
-1478.97126131189,-1478.8915537295,-1478.81175850042,-1478.73191415871,
-1478.65195573167,-1478.60955985507,-1478.52960255494,-1478.4497397577,
-1478.36995393522,-1478.29022762003,-1478.21054339173,-1478.13087240551,
-1478.05120495199,-1477.97152530117,-1477.89181771878,-1477.8120224897,
-1477.73217814799,-1477.65221972095,-1477.60982384435,-1477.52986654422,
-1477.45000374698,-1477.3702179245,-1477.29049160931,-1477.21080738102,
-1477.13113639479,-1477.05146894127,-1476.97178929045,-1476.89208170806,
-1476.81228647898,-1476.73244213728,-1476.65248371023,-1476.61008783363,
-1476.5301305335,-1476.45026773626,-1476.37048191378,-1476.29075559859,
-1476.21107137029,-1476.13140038407,-1476.05173293055,-1475.97205327973,
-1475.89234569734,-1475.81255046826,-1475.73270612655,-1475.65274769951,
-1475.61035182291,-1475.53039452278,-1475.45053172553,-1475.37074590306,
-1475.29101958787,-1475.21133535957,-1475.13166437335,-1475.05199691982,
-1474.972317269,-1474.89260968661,-1474.81281445753,-1474.73297011582,-1474.65301168878,
-1474.61061581219,-1474.50625453886,-1474.40403233292,-1474.3579036915),
 .UNSPECIFIED.);
#1923=B_SPLINE_CURVE_WITH_KNOTS('',3,(#265038,#265039,#265040,#265041,#265042,
#265043,#265044,#265045,#265046,#265047,#265048),.UNSPECIFIED.,.F.,.F.,
(4,2,1,1,1,1,1,4),(-1486.92427424324,-1486.60744794083,-1485.60771193012,
-1484.60797591939,-1483.60823990867,-1482.60850389795,-1481.60876788723,
-1480.64109334394),.UNSPECIFIED.);
#1924=B_SPLINE_CURVE_WITH_KNOTS('',3,(#265050,#265051,#265052,#265053,#265054,
#265055,#265056,#265057,#265058,#265059),.UNSPECIFIED.,.F.,.F.,(4,1,1,1,
1,1,1,4),(-1493.20745955042,-1492.60586400516,-1491.60612799444,-1490.60639198372,
-1489.606655973,-1488.60691996228,-1487.60718395156,-1486.92427424324),
 .UNSPECIFIED.);
#1925=B_SPLINE_CURVE_WITH_KNOTS('',3,(#265061,#265062,#265063,#265064,#265065,
#265066,#265067,#265068,#265069,#265070),.UNSPECIFIED.,.F.,.F.,(4,1,1,1,
1,1,1,4),(-1499.4906448576,-1498.60428006948,-1497.60454405876,-1496.60480804804,
-1495.60507203732,-1494.6053360266,-1493.60560001588,-1493.20745955042),
 .UNSPECIFIED.);
#1926=B_SPLINE_CURVE_WITH_KNOTS('',3,(#265071,#265072,#265073,#265074,#265075),
 .UNSPECIFIED.,.F.,.F.,(4,1,4),(-1500.33866773228,-1499.6040160802,-1499.4906448576),
 .UNSPECIFIED.);
#1927=B_SPLINE_CURVE_WITH_KNOTS('',3,(#265078,#265079,#265080,#265081,#265082,
#265083,#265084,#265085,#265086,#265087,#265088,#265089,#265090,#265091,
#265092,#265093,#265094,#265095,#265096,#265097,#265098,#265099,#265100,
#265101,#265102,#265103,#265104,#265105,#265106,#265107,#265108,#265109,
#265110,#265111,#265112,#265113,#265114,#265115,#265116,#265117,#265118,
#265119,#265120,#265121,#265122,#265123,#265124,#265125,#265126,#265127,
#265128,#265129,#265130,#265131,#265132,#265133,#265134,#265135,#265136,
#265137,#265138,#265139,#265140,#265141,#265142,#265143,#265144,#265145,
#265146,#265147,#265148,#265149,#265150,#265151,#265152,#265153,#265154,
#265155,#265156,#265157,#265158,#265159,#265160,#265161,#265162,#265163,
#265164,#265165,#265166,#265167,#265168,#265169,#265170,#265171,#265172,
#265173,#265174,#265175,#265176,#265177,#265178,#265179,#265180,#265181,
#265182,#265183,#265184,#265185,#265186,#265187,#265188,#265189,#265190,
#265191,#265192,#265193,#265194,#265195,#265196,#265197,#265198,#265199,
#265200,#265201,#265202,#265203,#265204,#265205,#265206,#265207,#265208,
#265209,#265210,#265211,#265212,#265213,#265214,#265215,#265216,#265217,
#265218,#265219,#265220,#265221,#265222,#265223,#265224,#265225,#265226,
#265227,#265228,#265229,#265230,#265231,#265232,#265233,#265234,#265235,
#265236,#265237,#265238,#265239,#265240,#265241,#265242,#265243,#265244,
#265245,#265246,#265247,#265248,#265249,#265250,#265251,#265252,#265253,
#265254,#265255,#265256,#265257,#265258,#265259,#265260,#265261,#265262,
#265263,#265264,#265265,#265266,#265267,#265268,#265269,#265270,#265271,
#265272,#265273,#265274,#265275,#265276,#265277,#265278,#265279,#265280,
#265281,#265282,#265283,#265284,#265285,#265286,#265287,#265288,#265289,
#265290,#265291,#265292,#265293,#265294,#265295,#265296,#265297),
 .UNSPECIFIED.,.F.,.F.,(4,3,3,3,3,3,3,3,3,3,3,3,3,3,3,3,3,3,3,3,3,3,3,3,
3,3,3,3,3,3,3,3,3,3,3,3,3,3,3,3,3,3,3,3,3,3,3,3,3,3,3,3,3,3,3,3,3,3,3,3,
3,3,3,3,3,3,3,3,3,3,3,3,3,4),(1404.29191615481,1404.37506475554,1404.45811270144,
1404.54108068674,1404.62398932894,1404.70686775223,1404.78973305654,1404.87260381792,
1404.95549861295,1405.03848303953,1405.1215178224,1405.20467492572,1405.24742046295,
1405.3311591748,1405.41479468616,1405.49834712956,1405.58183656541,1405.66529051603,
1405.74872700987,1405.83216411963,1405.91561991455,1405.99916440728,1406.08275349022,
1406.16647675777,1406.24715647367,1406.33089518552,1406.41453069688,1406.49808314028,
1406.58157257613,1406.66502652675,1406.74846302059,1406.83190013035,1406.91535592527,
1406.998900418,1407.08248950094,1407.16621276849,1407.24689248439,1407.33063119624,
1407.4142667076,1407.497819151,1407.58130858685,1407.66476253747,1407.74819903131,
1407.83163614107,1407.91509193599,1407.99863642872,1408.08222551166,1408.16594877921,
1408.24662849511,1408.33036720696,1408.41400271832,1408.49755516172,1408.58104459757,
1408.66449854819,1408.74793504203,1408.83137215179,1408.91482794671,1408.99837243944,
1409.08196152238,1409.16568478993,1409.24636450583,1409.33010321768,1409.41373872904,
1409.49729117244,1409.58078060829,1409.66423455891,1409.74767105275,1409.83110816251,
1409.91456395743,1409.99810845016,1410.0816975331,1410.16542080065,1410.24610051655,
1410.3244751935),.UNSPECIFIED.);
#1928=B_SPLINE_CURVE_WITH_KNOTS('',3,(#265298,#265299,#265300,#265301,#265302,
#265303,#265304,#265305,#265306,#265307,#265308,#265309,#265310),
 .UNSPECIFIED.,.F.,.F.,(4,3,3,3,4),(1404.04024993874,1404.12386652121,1404.20760574971,
1404.24768445223,1404.29191615463),.UNSPECIFIED.);
#1929=B_SPLINE_CURVE_WITH_KNOTS('',3,(#265314,#265315,#265316,#265317,#265318,
#265319,#265320,#265321),.UNSPECIFIED.,.F.,.F.,(4,2,2,4),(0.511738111681904,
0.560187232161708,0.746865960113868,0.833421149073491),.UNSPECIFIED.);
#1930=B_SPLINE_CURVE_WITH_KNOTS('',3,(#265323,#265324,#265325,#265326,#265327,
#265328,#265329,#265330,#265331,#265332,#265333,#265334,#265335,#265336,
#265337,#265338,#265339,#265340,#265341),.UNSPECIFIED.,.F.,.F.,(4,3,3,3,
3,3,4),(1511.10606637669,1511.21943759928,1511.30319040684,1511.38681542686,
1511.47036680961,1511.55385319882,1511.60403841566),.UNSPECIFIED.);
#1931=B_SPLINE_CURVE_WITH_KNOTS('',3,(#265343,#265344,#265345,#265346,#265347,
#265348,#265349,#265350,#265351,#265352,#265353,#265354,#265355,#265356,
#265357,#265358,#265359,#265360,#265361,#265362,#265363,#265364,#265365,
#265366,#265367,#265368,#265369,#265370,#265371,#265372,#265373,#265374,
#265375,#265376,#265377,#265378,#265379,#265380,#265381,#265382),
 .UNSPECIFIED.,.F.,.F.,(4,3,3,3,3,3,3,3,3,3,3,3,3,4),(1510.04626900307,
1510.13298529582,1510.21970158856,1510.30231995216,1510.38483597174,1510.46727079007,
1510.54964461587,1510.63198603367,1510.71431401009,1510.79664749822,1510.8790479625,
1510.96148328965,1511.04402920436,1511.10606637655),.UNSPECIFIED.);
#1932=B_SPLINE_CURVE_WITH_KNOTS('',3,(#265383,#265384,#265385,#265386,#265387,
#265388,#265389,#265390),.UNSPECIFIED.,.F.,.F.,(4,2,2,4),(0.833421149073491,
0.933544688066027,1.12022341601819,1.25194814216481),.UNSPECIFIED.);
#1933=B_SPLINE_CURVE_WITH_KNOTS('',3,(#272171,#272172,#272173,#272174,#272175,
#272176,#272177,#272178,#272179,#272180),.UNSPECIFIED.,.F.,.F.,(4,2,2,2,
4),(0.000658062556380468,0.0111047509489515,0.0590298249892507,0.111505910077716,
0.21897564774011),.UNSPECIFIED.);
#1934=B_SPLINE_CURVE_WITH_KNOTS('',3,(#272181,#272182,#272183,#272184,#272185,
#272186,#272187,#272188,#272189,#272190,#272191,#272192,#272193,#272194,
#272195,#272196,#272197,#272198,#272199,#272200,#272201,#272202,#272203,
#272204,#272205,#272206,#272207,#272208,#272209,#272210),.UNSPECIFIED.,
 .F.,.F.,(4,2,2,2,2,2,2,2,2,2,2,2,2,2,4),(0.00421488007861112,0.126209593249118,
0.138553986655518,0.139238723759837,0.139494495774474,0.139701646022053,
0.139825836912464,0.139896118986021,0.139956803150512,0.140030152514862,
0.140167078926622,0.140893495700786,0.142281953339915,0.175403086699887,
0.271081612417309),.UNSPECIFIED.);
#1935=B_SPLINE_CURVE_WITH_KNOTS('',3,(#272212,#272213,#272214,#272215,#272216,
#272217,#272218,#272219,#272220,#272221,#272222,#272223,#272224,#272225,
#272226,#272227,#272228,#272229,#272230,#272231,#272232,#272233,#272234,
#272235,#272236,#272237,#272238,#272239,#272240,#272241,#272242,#272243,
#272244,#272245,#272246,#272247,#272248,#272249,#272250,#272251,#272252,
#272253,#272254,#272255,#272256,#272257,#272258,#272259,#272260,#272261,
#272262,#272263,#272264,#272265,#272266,#272267,#272268,#272269,#272270,
#272271,#272272,#272273,#272274,#272275,#272276,#272277),.UNSPECIFIED.,
 .F.,.F.,(4,2,2,2,2,2,2,2,2,2,2,2,2,2,2,2,2,2,2,2,2,2,2,2,2,2,2,2,2,2,2,
2,4),(0.327283840054511,0.396783892533185,0.398753154793215,0.39883104940972,
0.398913914893828,0.398957630479319,0.398993023019997,0.399033143424731,
0.399101184070818,0.399358824404068,0.425945100779195,0.48786691587727,
0.590116051707203,0.728147561875147,0.915995373334799,1.00257399236972,
1.01107722098825,1.01145699741804,1.01152254445187,1.01160528707227,1.01187936515956,
1.01198328823823,1.01205251272225,1.01211868643199,1.01220807494068,1.01240984189626,
1.01682708804678,1.04338539683548,1.10926355513005,1.20121102692353,1.32043543719856,
1.40835082600552,1.50774934918788),.UNSPECIFIED.);
#1936=B_SPLINE_CURVE_WITH_KNOTS('',3,(#272278,#272279,#272280,#272281,#272282,
#272283,#272284,#272285,#272286,#272287),.UNSPECIFIED.,.F.,.F.,(4,2,2,2,
4),(0.0020693068779551,0.0883072267821443,0.189117057255197,0.276553971900186,
0.327283840054511),.UNSPECIFIED.);
#1937=B_SPLINE_CURVE_WITH_KNOTS('',3,(#272288,#272289,#272290,#272291,#272292,
#272293,#272294,#272295,#272296,#272297,#272298,#272299,#272300,#272301,
#272302,#272303,#272304,#272305,#272306,#272307,#272308,#272309,#272310,
#272311,#272312,#272313,#272314,#272315,#272316,#272317,#272318,#272319,
#272320,#272321,#272322,#272323,#272324,#272325,#272326,#272327,#272328,
#272329,#272330,#272331,#272332,#272333),.UNSPECIFIED.,.F.,.F.,(4,2,2,2,
2,2,2,2,2,2,2,2,2,2,2,2,2,2,2,2,2,2,4),(0.000477110384091791,0.110358824121838,
0.172331397524916,0.183780301788713,0.187764976788729,0.191717661689663,
0.192789629652419,0.194532929434185,0.195126939526276,0.195487384399954,
0.195561053638385,0.195617377487698,0.195648423799949,0.195666662922991,
0.195682536300503,0.195701880767454,0.195738461322392,0.195943378897047,
0.196314700337278,0.212692416929255,0.248840090507569,0.30101993643223,
0.351147893655916),.UNSPECIFIED.);
#1938=B_SPLINE_CURVE_WITH_KNOTS('',3,(#272336,#272337,#272338,#272339,#272340,
#272341),.UNSPECIFIED.,.F.,.F.,(4,2,4),(2.88515402066428,2.93100248921169,
3.09523639416926),.UNSPECIFIED.);
#1939=B_SPLINE_CURVE_WITH_KNOTS('',3,(#272343,#272344,#272345,#272346,#272347),
 .UNSPECIFIED.,.F.,.F.,(4,1,4),(-1502.69543409617,-1502.60322411236,-1502.3180309781),
 .UNSPECIFIED.);
#1940=B_SPLINE_CURVE_WITH_KNOTS('',3,(#272348,#272349,#272350,#272351),
 .UNSPECIFIED.,.F.,.F.,(4,4),(2.48381435072133,2.66889972571145),
 .UNSPECIFIED.);
#1941=B_SPLINE_CURVE_WITH_KNOTS('',3,(#279132,#279133,#279134,#279135,#279136,
#279137,#279138,#279139,#279140,#279141,#279142,#279143,#279144,#279145,
#279146,#279147,#279148,#279149,#279150,#279151,#279152,#279153,#279154,
#279155),.UNSPECIFIED.,.F.,.F.,(4,2,2,2,2,2,2,2,2,2,2,4),(0.00293506500743818,
0.102989889801783,0.114060948170188,0.114147673612461,0.114232131538629,
0.11427719251539,0.11431393964835,0.114355889157666,0.114427166018751,0.114704271772878,
0.148089581915078,0.224846674886138),.UNSPECIFIED.);
#1949=SHAPE_REPRESENTATION_RELATIONSHIP('SRR','None',#279308,#1958);
#1958=ADVANCED_BREP_SHAPE_REPRESENTATION('',(#1976),#279264);
#1967=STYLED_ITEM('',(#279355),#1976);
#1976=MANIFOLD_SOLID_BREP('Body1',#14945);
#2017=FACE_BOUND('',#3073,.T.);
#2100=PLANE('',#15634);
#2101=PLANE('',#15635);
#2537=FACE_OUTER_BOUND('',#3046,.T.);
#2538=FACE_OUTER_BOUND('',#3047,.T.);
#2539=FACE_OUTER_BOUND('',#3048,.T.);
#2540=FACE_OUTER_BOUND('',#3049,.T.);
#2541=FACE_OUTER_BOUND('',#3050,.T.);
#2542=FACE_OUTER_BOUND('',#3051,.T.);
#2543=FACE_OUTER_BOUND('',#3052,.T.);
#2544=FACE_OUTER_BOUND('',#3053,.T.);
#2545=FACE_OUTER_BOUND('',#3054,.T.);
#2546=FACE_OUTER_BOUND('',#3055,.T.);
#2547=FACE_OUTER_BOUND('',#3056,.T.);
#2548=FACE_OUTER_BOUND('',#3057,.T.);
#2549=FACE_OUTER_BOUND('',#3058,.T.);
#2550=FACE_OUTER_BOUND('',#3059,.T.);
#2551=FACE_OUTER_BOUND('',#3060,.T.);
#2552=FACE_OUTER_BOUND('',#3061,.T.);
#2553=FACE_OUTER_BOUND('',#3062,.T.);
#2554=FACE_OUTER_BOUND('',#3063,.T.);
#2555=FACE_OUTER_BOUND('',#3064,.T.);
#2556=FACE_OUTER_BOUND('',#3065,.T.);
#2557=FACE_OUTER_BOUND('',#3066,.T.);
#2558=FACE_OUTER_BOUND('',#3067,.T.);
#2559=FACE_OUTER_BOUND('',#3068,.T.);
#2560=FACE_OUTER_BOUND('',#3069,.T.);
#2561=FACE_OUTER_BOUND('',#3070,.T.);
#2562=FACE_OUTER_BOUND('',#3071,.T.);
#2563=FACE_OUTER_BOUND('',#3072,.T.);
#2564=FACE_OUTER_BOUND('',#3074,.T.);
#2565=FACE_OUTER_BOUND('',#3075,.T.);
#3046=EDGE_LOOP('',(#13718,#13719,#13720,#13721,#13722,#13723));
#3047=EDGE_LOOP('',(#13724,#13725,#13726,#13727,#13728,#13729));
#3048=EDGE_LOOP('',(#13730,#13731,#13732,#13733,#13734,#13735));
#3049=EDGE_LOOP('',(#13736,#13737,#13738,#13739,#13740,#13741));
#3050=EDGE_LOOP('',(#13742,#13743,#13744,#13745,#13746,#13747));
#3051=EDGE_LOOP('',(#13748,#13749,#13750,#13751,#13752,#13753));
#3052=EDGE_LOOP('',(#13754,#13755,#13756,#13757,#13758,#13759));
#3053=EDGE_LOOP('',(#13760,#13761,#13762,#13763,#13764,#13765));
#3054=EDGE_LOOP('',(#13766,#13767,#13768,#13769,#13770,#13771));
#3055=EDGE_LOOP('',(#13772,#13773,#13774,#13775,#13776,#13777));
#3056=EDGE_LOOP('',(#13778,#13779,#13780,#13781,#13782,#13783));
#3057=EDGE_LOOP('',(#13784,#13785,#13786,#13787,#13788,#13789));
#3058=EDGE_LOOP('',(#13790,#13791,#13792,#13793,#13794,#13795));
#3059=EDGE_LOOP('',(#13796,#13797,#13798,#13799,#13800,#13801));
#3060=EDGE_LOOP('',(#13802,#13803,#13804,#13805,#13806,#13807));
#3061=EDGE_LOOP('',(#13808,#13809,#13810,#13811,#13812,#13813));
#3062=EDGE_LOOP('',(#13814,#13815,#13816,#13817));
#3063=EDGE_LOOP('',(#13818,#13819,#13820));
#3064=EDGE_LOOP('',(#13821,#13822,#13823,#13824,#13825,#13826,#13827,#13828,
#13829,#13830,#13831,#13832,#13833,#13834,#13835,#13836,#13837,#13838,#13839,
#13840,#13841,#13842,#13843,#13844,#13845,#13846,#13847,#13848,#13849,#13850,
#13851,#13852,#13853,#13854,#13855,#13856,#13857,#13858,#13859,#13860,#13861,
#13862,#13863,#13864,#13865,#13866,#13867,#13868,#13869,#13870,#13871,#13872,
#13873,#13874,#13875,#13876,#13877));
#3065=EDGE_LOOP('',(#13878,#13879,#13880,#13881));
#3066=EDGE_LOOP('',(#13882,#13883,#13884,#13885,#13886,#13887,#13888,#13889,
#13890,#13891,#13892,#13893,#13894,#13895,#13896,#13897,#13898,#13899,#13900,
#13901,#13902,#13903,#13904,#13905,#13906,#13907,#13908,#13909,#13910,#13911,
#13912,#13913,#13914,#13915,#13916,#13917,#13918,#13919));
#3067=EDGE_LOOP('',(#13920,#13921,#13922,#13923,#13924,#13925));
#3068=EDGE_LOOP('',(#13926,#13927,#13928,#13929));
#3069=EDGE_LOOP('',(#13930,#13931,#13932,#13933,#13934,#13935,#13936,#13937,
#13938,#13939,#13940,#13941,#13942,#13943,#13944,#13945,#13946,#13947,#13948,
#13949,#13950,#13951,#13952,#13953,#13954,#13955,#13956,#13957,#13958,#13959,
#13960,#13961,#13962,#13963,#13964,#13965,#13966,#13967,#13968,#13969,#13970,
#13971,#13972,#13973,#13974,#13975,#13976,#13977,#13978,#13979,#13980,#13981,
#13982,#13983,#13984,#13985,#13986,#13987,#13988,#13989,#13990));
#3070=EDGE_LOOP('',(#13991,#13992,#13993,#13994));
#3071=EDGE_LOOP('',(#13995,#13996));
#3072=EDGE_LOOP('',(#13997,#13998,#13999,#14000,#14001,#14002,#14003,#14004,
#14005,#14006,#14007,#14008,#14009,#14010,#14011,#14012));
#3073=EDGE_LOOP('',(#14013,#14014,#14015,#14016,#14017,#14018,#14019,#14020,
#14021,#14022,#14023));
#3074=EDGE_LOOP('',(#14024));
#3075=EDGE_LOOP('',(#14025));
#3585=LINE('',#240809,#4113);
#3586=LINE('',#241160,#4114);
#3587=LINE('',#241620,#4115);
#3588=LINE('',#241873,#4116);
#3589=LINE('',#242132,#4117);
#3590=LINE('',#242595,#4118);
#3591=LINE('',#243061,#4119);
#3592=LINE('',#243524,#4120);
#3593=LINE('',#243990,#4121);
#3594=LINE('',#244453,#4122);
#3595=LINE('',#244922,#4123);
#3596=LINE('',#245391,#4124);
#3597=LINE('',#245851,#4125);
#3598=LINE('',#246317,#4126);
#3599=LINE('',#246780,#4127);
#3600=LINE('',#247243,#4128);
#3601=LINE('',#247706,#4129);
#3602=LINE('',#279159,#4130);
#3603=LINE('',#279161,#4131);
#4113=VECTOR('',#17289,4.91825);
#4114=VECTOR('',#17292,4.91825);
#4115=VECTOR('',#17295,4.91825);
#4116=VECTOR('',#17298,4.91825);
#4117=VECTOR('',#17301,4.91825);
#4118=VECTOR('',#17304,4.91825);
#4119=VECTOR('',#17307,4.91825);
#4120=VECTOR('',#17310,4.91825);
#4121=VECTOR('',#17313,4.91825);
#4122=VECTOR('',#17316,4.91825);
#4123=VECTOR('',#17319,4.91825);
#4124=VECTOR('',#17322,4.91825);
#4125=VECTOR('',#17325,4.91825);
#4126=VECTOR('',#17328,4.91825);
#4127=VECTOR('',#17331,4.91825);
#4128=VECTOR('',#17334,4.91825);
#4129=VECTOR('',#17337,4.91825);
#4130=VECTOR('',#17352,15.2420394990918);
#4131=VECTOR('',#17353,15.2420394990918);
#4284=CIRCLE('',#15632,15.2420394990918);
#4285=CIRCLE('',#15633,15.2420394990918);
#6263=VERTEX_POINT('',#240807);
#6264=VERTEX_POINT('',#240808);
#6265=VERTEX_POINT('',#240810);
#6266=VERTEX_POINT('',#240821);
#6267=VERTEX_POINT('',#240973);
#6268=VERTEX_POINT('',#240980);
#6269=VERTEX_POINT('',#241158);
#6270=VERTEX_POINT('',#241159);
#6271=VERTEX_POINT('',#241161);
#6272=VERTEX_POINT('',#241383);
#6273=VERTEX_POINT('',#241618);
#6274=VERTEX_POINT('',#241619);
#6275=VERTEX_POINT('',#241621);
#6276=VERTEX_POINT('',#241636);
#6277=VERTEX_POINT('',#241871);
#6278=VERTEX_POINT('',#241872);
#6279=VERTEX_POINT('',#241874);
#6280=VERTEX_POINT('',#241898);
#6281=VERTEX_POINT('',#242130);
#6282=VERTEX_POINT('',#242131);
#6283=VERTEX_POINT('',#242133);
#6284=VERTEX_POINT('',#242361);
#6285=VERTEX_POINT('',#242593);
#6286=VERTEX_POINT('',#242594);
#6287=VERTEX_POINT('',#242596);
#6288=VERTEX_POINT('',#242827);
#6289=VERTEX_POINT('',#243059);
#6290=VERTEX_POINT('',#243060);
#6291=VERTEX_POINT('',#243062);
#6292=VERTEX_POINT('',#243293);
#6293=VERTEX_POINT('',#243522);
#6294=VERTEX_POINT('',#243523);
#6295=VERTEX_POINT('',#243525);
#6296=VERTEX_POINT('',#243756);
#6297=VERTEX_POINT('',#243988);
#6298=VERTEX_POINT('',#243989);
#6299=VERTEX_POINT('',#243991);
#6300=VERTEX_POINT('',#244219);
#6301=VERTEX_POINT('',#244451);
#6302=VERTEX_POINT('',#244452);
#6303=VERTEX_POINT('',#244454);
#6304=VERTEX_POINT('',#244685);
#6305=VERTEX_POINT('',#244920);
#6306=VERTEX_POINT('',#244921);
#6307=VERTEX_POINT('',#244923);
#6308=VERTEX_POINT('',#245157);
#6309=VERTEX_POINT('',#245389);
#6310=VERTEX_POINT('',#245390);
#6311=VERTEX_POINT('',#245392);
#6312=VERTEX_POINT('',#245620);
#6313=VERTEX_POINT('',#245849);
#6314=VERTEX_POINT('',#245850);
#6315=VERTEX_POINT('',#245852);
#6316=VERTEX_POINT('',#246083);
#6317=VERTEX_POINT('',#246315);
#6318=VERTEX_POINT('',#246316);
#6319=VERTEX_POINT('',#246318);
#6320=VERTEX_POINT('',#246549);
#6321=VERTEX_POINT('',#246778);
#6322=VERTEX_POINT('',#246779);
#6323=VERTEX_POINT('',#246781);
#6324=VERTEX_POINT('',#247012);
#6325=VERTEX_POINT('',#247241);
#6326=VERTEX_POINT('',#247242);
#6327=VERTEX_POINT('',#247244);
#6328=VERTEX_POINT('',#247472);
#6329=VERTEX_POINT('',#247704);
#6330=VERTEX_POINT('',#247705);
#6331=VERTEX_POINT('',#247707);
#6332=VERTEX_POINT('',#247721);
#6333=VERTEX_POINT('',#254536);
#6334=VERTEX_POINT('',#254537);
#6335=VERTEX_POINT('',#254548);
#6336=VERTEX_POINT('',#261422);
#6337=VERTEX_POINT('',#261423);
#6338=VERTEX_POINT('',#261462);
#6339=VERTEX_POINT('',#261516);
#6340=VERTEX_POINT('',#261747);
#6341=VERTEX_POINT('',#261758);
#6342=VERTEX_POINT('',#261805);
#6343=VERTEX_POINT('',#261816);
#6344=VERTEX_POINT('',#261827);
#6345=VERTEX_POINT('',#261840);
#6346=VERTEX_POINT('',#262085);
#6347=VERTEX_POINT('',#262330);
#6348=VERTEX_POINT('',#262342);
#6349=VERTEX_POINT('',#262587);
#6350=VERTEX_POINT('',#262598);
#6351=VERTEX_POINT('',#262609);
#6352=VERTEX_POINT('',#262622);
#6353=VERTEX_POINT('',#262867);
#6354=VERTEX_POINT('',#263115);
#6355=VERTEX_POINT('',#263127);
#6356=VERTEX_POINT('',#263372);
#6357=VERTEX_POINT('',#263620);
#6358=VERTEX_POINT('',#263672);
#6359=VERTEX_POINT('',#263679);
#6360=VERTEX_POINT('',#263691);
#6361=VERTEX_POINT('',#263696);
#6362=VERTEX_POINT('',#263703);
#6363=VERTEX_POINT('',#263710);
#6364=VERTEX_POINT('',#263958);
#6365=VERTEX_POINT('',#263969);
#6366=VERTEX_POINT('',#264214);
#6367=VERTEX_POINT('',#264225);
#6368=VERTEX_POINT('',#264236);
#6369=VERTEX_POINT('',#264484);
#6370=VERTEX_POINT('',#264495);
#6371=VERTEX_POINT('',#264506);
#6372=VERTEX_POINT('',#264517);
#6373=VERTEX_POINT('',#264530);
#6374=VERTEX_POINT('',#264778);
#6375=VERTEX_POINT('',#264789);
#6376=VERTEX_POINT('',#265037);
#6377=VERTEX_POINT('',#265049);
#6378=VERTEX_POINT('',#265060);
#6379=VERTEX_POINT('',#265077);
#6380=VERTEX_POINT('',#265312);
#6381=VERTEX_POINT('',#265313);
#6382=VERTEX_POINT('',#265322);
#6383=VERTEX_POINT('',#265342);
#6384=VERTEX_POINT('',#272211);
#6385=VERTEX_POINT('',#272335);
#6386=VERTEX_POINT('',#272342);
#6387=VERTEX_POINT('',#279157);
#6388=VERTEX_POINT('',#279160);
#8784=EDGE_CURVE('',#6263,#6264,#3585,.T.);
#8785=EDGE_CURVE('',#6264,#6265,#1809,.T.);
#8786=EDGE_CURVE('',#6265,#6266,#1810,.T.);
#8787=EDGE_CURVE('',#6267,#6266,#1811,.T.);
#8788=EDGE_CURVE('',#6268,#6267,#1812,.T.);
#8789=EDGE_CURVE('',#6263,#6268,#1813,.T.);
#8790=EDGE_CURVE('',#6269,#6270,#3586,.T.);
#8791=EDGE_CURVE('',#6270,#6271,#1814,.T.);
#8792=EDGE_CURVE('',#6271,#6264,#1815,.T.);
#8793=EDGE_CURVE('',#6272,#6263,#1816,.T.);
#8794=EDGE_CURVE('',#6269,#6272,#1817,.T.);
#8795=EDGE_CURVE('',#6273,#6274,#3587,.T.);
#8796=EDGE_CURVE('',#6274,#6275,#1818,.T.);
#8797=EDGE_CURVE('',#6275,#6270,#1819,.T.);
#8798=EDGE_CURVE('',#6276,#6269,#1820,.T.);
#8799=EDGE_CURVE('',#6273,#6276,#1821,.T.);
#8800=EDGE_CURVE('',#6277,#6278,#3588,.T.);
#8801=EDGE_CURVE('',#6278,#6279,#1822,.T.);
#8802=EDGE_CURVE('',#6279,#6274,#1823,.T.);
#8803=EDGE_CURVE('',#6280,#6273,#1824,.T.);
#8804=EDGE_CURVE('',#6277,#6280,#1825,.T.);
#8805=EDGE_CURVE('',#6281,#6282,#3589,.T.);
#8806=EDGE_CURVE('',#6282,#6283,#1826,.T.);
#8807=EDGE_CURVE('',#6283,#6278,#1827,.T.);
#8808=EDGE_CURVE('',#6284,#6277,#1828,.T.);
#8809=EDGE_CURVE('',#6281,#6284,#1829,.T.);
#8810=EDGE_CURVE('',#6285,#6286,#3590,.T.);
#8811=EDGE_CURVE('',#6286,#6287,#1830,.T.);
#8812=EDGE_CURVE('',#6287,#6282,#1831,.T.);
#8813=EDGE_CURVE('',#6288,#6281,#1832,.T.);
#8814=EDGE_CURVE('',#6285,#6288,#1833,.T.);
#8815=EDGE_CURVE('',#6289,#6290,#3591,.T.);
#8816=EDGE_CURVE('',#6290,#6291,#1834,.T.);
#8817=EDGE_CURVE('',#6291,#6286,#1835,.T.);
#8818=EDGE_CURVE('',#6292,#6285,#1836,.T.);
#8819=EDGE_CURVE('',#6289,#6292,#1837,.T.);
#8820=EDGE_CURVE('',#6293,#6294,#3592,.T.);
#8821=EDGE_CURVE('',#6294,#6295,#1838,.T.);
#8822=EDGE_CURVE('',#6295,#6290,#1839,.T.);
#8823=EDGE_CURVE('',#6296,#6289,#1840,.T.);
#8824=EDGE_CURVE('',#6293,#6296,#1841,.T.);
#8825=EDGE_CURVE('',#6297,#6298,#3593,.T.);
#8826=EDGE_CURVE('',#6298,#6299,#1842,.T.);
#8827=EDGE_CURVE('',#6299,#6294,#1843,.T.);
#8828=EDGE_CURVE('',#6300,#6293,#1844,.T.);
#8829=EDGE_CURVE('',#6297,#6300,#1845,.T.);
#8830=EDGE_CURVE('',#6301,#6302,#3594,.T.);
#8831=EDGE_CURVE('',#6302,#6303,#1846,.T.);
#8832=EDGE_CURVE('',#6303,#6298,#1847,.T.);
#8833=EDGE_CURVE('',#6304,#6297,#1848,.T.);
#8834=EDGE_CURVE('',#6301,#6304,#1849,.T.);
#8835=EDGE_CURVE('',#6305,#6306,#3595,.T.);
#8836=EDGE_CURVE('',#6306,#6307,#1850,.T.);
#8837=EDGE_CURVE('',#6307,#6302,#1851,.T.);
#8838=EDGE_CURVE('',#6308,#6301,#1852,.T.);
#8839=EDGE_CURVE('',#6305,#6308,#1853,.T.);
#8840=EDGE_CURVE('',#6309,#6310,#3596,.T.);
#8841=EDGE_CURVE('',#6310,#6311,#1854,.T.);
#8842=EDGE_CURVE('',#6311,#6306,#1855,.T.);
#8843=EDGE_CURVE('',#6312,#6305,#1856,.T.);
#8844=EDGE_CURVE('',#6309,#6312,#1857,.T.);
#8845=EDGE_CURVE('',#6313,#6314,#3597,.T.);
#8846=EDGE_CURVE('',#6314,#6315,#1858,.T.);
#8847=EDGE_CURVE('',#6315,#6310,#1859,.T.);
#8848=EDGE_CURVE('',#6316,#6309,#1860,.T.);
#8849=EDGE_CURVE('',#6313,#6316,#1861,.T.);
#8850=EDGE_CURVE('',#6317,#6318,#3598,.T.);
#8851=EDGE_CURVE('',#6318,#6319,#1862,.T.);
#8852=EDGE_CURVE('',#6319,#6314,#1863,.T.);
#8853=EDGE_CURVE('',#6320,#6313,#1864,.T.);
#8854=EDGE_CURVE('',#6317,#6320,#1865,.T.);
#8855=EDGE_CURVE('',#6321,#6322,#3599,.T.);
#8856=EDGE_CURVE('',#6322,#6323,#1866,.T.);
#8857=EDGE_CURVE('',#6323,#6318,#1867,.T.);
#8858=EDGE_CURVE('',#6324,#6317,#1868,.T.);
#8859=EDGE_CURVE('',#6321,#6324,#1869,.T.);
#8860=EDGE_CURVE('',#6325,#6326,#3600,.T.);
#8861=EDGE_CURVE('',#6326,#6327,#1870,.T.);
#8862=EDGE_CURVE('',#6327,#6322,#1871,.T.);
#8863=EDGE_CURVE('',#6328,#6321,#1872,.T.);
#8864=EDGE_CURVE('',#6325,#6328,#1873,.T.);
#8865=EDGE_CURVE('',#6329,#6330,#3601,.T.);
#8866=EDGE_CURVE('',#6331,#6329,#1874,.T.);
#8867=EDGE_CURVE('',#6332,#6331,#1875,.T.);
#8868=EDGE_CURVE('',#6332,#6330,#1876,.T.);
#8869=EDGE_CURVE('',#6333,#6334,#1877,.T.);
#8870=EDGE_CURVE('',#6333,#6335,#1878,.T.);
#8871=EDGE_CURVE('',#6334,#6335,#1879,.T.);
#8872=EDGE_CURVE('',#6336,#6337,#1880,.T.);
#8873=EDGE_CURVE('',#6336,#6338,#1881,.T.);
#8874=EDGE_CURVE('',#6266,#6338,#1882,.T.);
#8875=EDGE_CURVE('',#6339,#6326,#1883,.T.);
#8876=EDGE_CURVE('',#6330,#6339,#1884,.T.);
#8877=EDGE_CURVE('',#6340,#6332,#1885,.T.);
#8878=EDGE_CURVE('',#6340,#6341,#1886,.T.);
#8879=EDGE_CURVE('',#6341,#6342,#1887,.T.);
#8880=EDGE_CURVE('',#6342,#6343,#1888,.T.);
#8881=EDGE_CURVE('',#6343,#6344,#1889,.T.);
#8882=EDGE_CURVE('',#6344,#6345,#1890,.T.);
#8883=EDGE_CURVE('',#6345,#6346,#1891,.T.);
#8884=EDGE_CURVE('',#6346,#6347,#1892,.T.);
#8885=EDGE_CURVE('',#6347,#6348,#1893,.T.);
#8886=EDGE_CURVE('',#6348,#6349,#1894,.T.);
#8887=EDGE_CURVE('',#6349,#6350,#1895,.T.);
#8888=EDGE_CURVE('',#6350,#6351,#1896,.T.);
#8889=EDGE_CURVE('',#6351,#6352,#1897,.T.);
#8890=EDGE_CURVE('',#6352,#6353,#1898,.T.);
#8891=EDGE_CURVE('',#6353,#6354,#1899,.T.);
#8892=EDGE_CURVE('',#6354,#6355,#1900,.T.);
#8893=EDGE_CURVE('',#6355,#6356,#1901,.T.);
#8894=EDGE_CURVE('',#6356,#6357,#1902,.T.);
#8895=EDGE_CURVE('',#6357,#6337,#1903,.T.);
#8896=EDGE_CURVE('',#6335,#6358,#1904,.T.);
#8897=EDGE_CURVE('',#6359,#6333,#1905,.T.);
#8898=EDGE_CURVE('',#6358,#6359,#1906,.T.);
#8899=EDGE_CURVE('',#6337,#6360,#1907,.T.);
#8900=EDGE_CURVE('',#6361,#6340,#1908,.T.);
#8901=EDGE_CURVE('',#6362,#6361,#1909,.T.);
#8902=EDGE_CURVE('',#6363,#6362,#1910,.T.);
#8903=EDGE_CURVE('',#6364,#6363,#1911,.T.);
#8904=EDGE_CURVE('',#6365,#6364,#1912,.T.);
#8905=EDGE_CURVE('',#6366,#6365,#1913,.T.);
#8906=EDGE_CURVE('',#6367,#6366,#1914,.T.);
#8907=EDGE_CURVE('',#6368,#6367,#1915,.T.);
#8908=EDGE_CURVE('',#6369,#6368,#1916,.T.);
#8909=EDGE_CURVE('',#6370,#6369,#1917,.T.);
#8910=EDGE_CURVE('',#6371,#6370,#1918,.T.);
#8911=EDGE_CURVE('',#6372,#6371,#1919,.T.);
#8912=EDGE_CURVE('',#6373,#6372,#1920,.T.);
#8913=EDGE_CURVE('',#6374,#6373,#1921,.T.);
#8914=EDGE_CURVE('',#6375,#6374,#1922,.T.);
#8915=EDGE_CURVE('',#6376,#6375,#1923,.T.);
#8916=EDGE_CURVE('',#6377,#6376,#1924,.T.);
#8917=EDGE_CURVE('',#6378,#6377,#1925,.T.);
#8918=EDGE_CURVE('',#6360,#6378,#1926,.T.);
#8919=EDGE_CURVE('',#6379,#6325,#1927,.T.);
#8920=EDGE_CURVE('',#6329,#6379,#1928,.T.);
#8921=EDGE_CURVE('',#6380,#6381,#1929,.T.);
#8922=EDGE_CURVE('',#6382,#6380,#1930,.T.);
#8923=EDGE_CURVE('',#6383,#6382,#1931,.T.);
#8924=EDGE_CURVE('',#6381,#6383,#1932,.T.);
#8925=EDGE_CURVE('',#6360,#6380,#1933,.T.);
#8926=EDGE_CURVE('',#6358,#6361,#1934,.T.);
#8927=EDGE_CURVE('',#6384,#6359,#1935,.T.);
#8928=EDGE_CURVE('',#6331,#6384,#1936,.T.);
#8929=EDGE_CURVE('',#6383,#6267,#1937,.T.);
#8930=EDGE_CURVE('',#6385,#6336,#1938,.T.);
#8931=EDGE_CURVE('',#6386,#6385,#1939,.T.);
#8932=EDGE_CURVE('',#6338,#6386,#1940,.T.);
#8933=EDGE_CURVE('',#6386,#6385,#1941,.T.);
#8934=EDGE_CURVE('',#6387,#6387,#4284,.T.);
#8935=EDGE_CURVE('',#6387,#6334,#3602,.T.);
#8936=EDGE_CURVE('',#6384,#6388,#3603,.T.);
#8937=EDGE_CURVE('',#6388,#6388,#4285,.T.);
#13718=ORIENTED_EDGE('',*,*,#8784,.T.);
#13719=ORIENTED_EDGE('',*,*,#8785,.T.);
#13720=ORIENTED_EDGE('',*,*,#8786,.T.);
#13721=ORIENTED_EDGE('',*,*,#8787,.F.);
#13722=ORIENTED_EDGE('',*,*,#8788,.F.);
#13723=ORIENTED_EDGE('',*,*,#8789,.F.);
#13724=ORIENTED_EDGE('',*,*,#8790,.T.);
#13725=ORIENTED_EDGE('',*,*,#8791,.T.);
#13726=ORIENTED_EDGE('',*,*,#8792,.T.);
#13727=ORIENTED_EDGE('',*,*,#8784,.F.);
#13728=ORIENTED_EDGE('',*,*,#8793,.F.);
#13729=ORIENTED_EDGE('',*,*,#8794,.F.);
#13730=ORIENTED_EDGE('',*,*,#8795,.T.);
#13731=ORIENTED_EDGE('',*,*,#8796,.T.);
#13732=ORIENTED_EDGE('',*,*,#8797,.T.);
#13733=ORIENTED_EDGE('',*,*,#8790,.F.);
#13734=ORIENTED_EDGE('',*,*,#8798,.F.);
#13735=ORIENTED_EDGE('',*,*,#8799,.F.);
#13736=ORIENTED_EDGE('',*,*,#8800,.T.);
#13737=ORIENTED_EDGE('',*,*,#8801,.T.);
#13738=ORIENTED_EDGE('',*,*,#8802,.T.);
#13739=ORIENTED_EDGE('',*,*,#8795,.F.);
#13740=ORIENTED_EDGE('',*,*,#8803,.F.);
#13741=ORIENTED_EDGE('',*,*,#8804,.F.);
#13742=ORIENTED_EDGE('',*,*,#8805,.T.);
#13743=ORIENTED_EDGE('',*,*,#8806,.T.);
#13744=ORIENTED_EDGE('',*,*,#8807,.T.);
#13745=ORIENTED_EDGE('',*,*,#8800,.F.);
#13746=ORIENTED_EDGE('',*,*,#8808,.F.);
#13747=ORIENTED_EDGE('',*,*,#8809,.F.);
#13748=ORIENTED_EDGE('',*,*,#8810,.T.);
#13749=ORIENTED_EDGE('',*,*,#8811,.T.);
#13750=ORIENTED_EDGE('',*,*,#8812,.T.);
#13751=ORIENTED_EDGE('',*,*,#8805,.F.);
#13752=ORIENTED_EDGE('',*,*,#8813,.F.);
#13753=ORIENTED_EDGE('',*,*,#8814,.F.);
#13754=ORIENTED_EDGE('',*,*,#8815,.T.);
#13755=ORIENTED_EDGE('',*,*,#8816,.T.);
#13756=ORIENTED_EDGE('',*,*,#8817,.T.);
#13757=ORIENTED_EDGE('',*,*,#8810,.F.);
#13758=ORIENTED_EDGE('',*,*,#8818,.F.);
#13759=ORIENTED_EDGE('',*,*,#8819,.F.);
#13760=ORIENTED_EDGE('',*,*,#8820,.T.);
#13761=ORIENTED_EDGE('',*,*,#8821,.T.);
#13762=ORIENTED_EDGE('',*,*,#8822,.T.);
#13763=ORIENTED_EDGE('',*,*,#8815,.F.);
#13764=ORIENTED_EDGE('',*,*,#8823,.F.);
#13765=ORIENTED_EDGE('',*,*,#8824,.F.);
#13766=ORIENTED_EDGE('',*,*,#8825,.T.);
#13767=ORIENTED_EDGE('',*,*,#8826,.T.);
#13768=ORIENTED_EDGE('',*,*,#8827,.T.);
#13769=ORIENTED_EDGE('',*,*,#8820,.F.);
#13770=ORIENTED_EDGE('',*,*,#8828,.F.);
#13771=ORIENTED_EDGE('',*,*,#8829,.F.);
#13772=ORIENTED_EDGE('',*,*,#8830,.T.);
#13773=ORIENTED_EDGE('',*,*,#8831,.T.);
#13774=ORIENTED_EDGE('',*,*,#8832,.T.);
#13775=ORIENTED_EDGE('',*,*,#8825,.F.);
#13776=ORIENTED_EDGE('',*,*,#8833,.F.);
#13777=ORIENTED_EDGE('',*,*,#8834,.F.);
#13778=ORIENTED_EDGE('',*,*,#8835,.T.);
#13779=ORIENTED_EDGE('',*,*,#8836,.T.);
#13780=ORIENTED_EDGE('',*,*,#8837,.T.);
#13781=ORIENTED_EDGE('',*,*,#8830,.F.);
#13782=ORIENTED_EDGE('',*,*,#8838,.F.);
#13783=ORIENTED_EDGE('',*,*,#8839,.F.);
#13784=ORIENTED_EDGE('',*,*,#8840,.T.);
#13785=ORIENTED_EDGE('',*,*,#8841,.T.);
#13786=ORIENTED_EDGE('',*,*,#8842,.T.);
#13787=ORIENTED_EDGE('',*,*,#8835,.F.);
#13788=ORIENTED_EDGE('',*,*,#8843,.F.);
#13789=ORIENTED_EDGE('',*,*,#8844,.F.);
#13790=ORIENTED_EDGE('',*,*,#8845,.T.);
#13791=ORIENTED_EDGE('',*,*,#8846,.T.);
#13792=ORIENTED_EDGE('',*,*,#8847,.T.);
#13793=ORIENTED_EDGE('',*,*,#8840,.F.);
#13794=ORIENTED_EDGE('',*,*,#8848,.F.);
#13795=ORIENTED_EDGE('',*,*,#8849,.F.);
#13796=ORIENTED_EDGE('',*,*,#8850,.T.);
#13797=ORIENTED_EDGE('',*,*,#8851,.T.);
#13798=ORIENTED_EDGE('',*,*,#8852,.T.);
#13799=ORIENTED_EDGE('',*,*,#8845,.F.);
#13800=ORIENTED_EDGE('',*,*,#8853,.F.);
#13801=ORIENTED_EDGE('',*,*,#8854,.F.);
#13802=ORIENTED_EDGE('',*,*,#8855,.T.);
#13803=ORIENTED_EDGE('',*,*,#8856,.T.);
#13804=ORIENTED_EDGE('',*,*,#8857,.T.);
#13805=ORIENTED_EDGE('',*,*,#8850,.F.);
#13806=ORIENTED_EDGE('',*,*,#8858,.F.);
#13807=ORIENTED_EDGE('',*,*,#8859,.F.);
#13808=ORIENTED_EDGE('',*,*,#8860,.T.);
#13809=ORIENTED_EDGE('',*,*,#8861,.T.);
#13810=ORIENTED_EDGE('',*,*,#8862,.T.);
#13811=ORIENTED_EDGE('',*,*,#8855,.F.);
#13812=ORIENTED_EDGE('',*,*,#8863,.F.);
#13813=ORIENTED_EDGE('',*,*,#8864,.F.);
#13814=ORIENTED_EDGE('',*,*,#8865,.F.);
#13815=ORIENTED_EDGE('',*,*,#8866,.F.);
#13816=ORIENTED_EDGE('',*,*,#8867,.F.);
#13817=ORIENTED_EDGE('',*,*,#8868,.T.);
#13818=ORIENTED_EDGE('',*,*,#8869,.F.);
#13819=ORIENTED_EDGE('',*,*,#8870,.T.);
#13820=ORIENTED_EDGE('',*,*,#8871,.F.);
#13821=ORIENTED_EDGE('',*,*,#8872,.F.);
#13822=ORIENTED_EDGE('',*,*,#8873,.T.);
#13823=ORIENTED_EDGE('',*,*,#8874,.F.);
#13824=ORIENTED_EDGE('',*,*,#8786,.F.);
#13825=ORIENTED_EDGE('',*,*,#8785,.F.);
#13826=ORIENTED_EDGE('',*,*,#8792,.F.);
#13827=ORIENTED_EDGE('',*,*,#8791,.F.);
#13828=ORIENTED_EDGE('',*,*,#8797,.F.);
#13829=ORIENTED_EDGE('',*,*,#8796,.F.);
#13830=ORIENTED_EDGE('',*,*,#8802,.F.);
#13831=ORIENTED_EDGE('',*,*,#8801,.F.);
#13832=ORIENTED_EDGE('',*,*,#8807,.F.);
#13833=ORIENTED_EDGE('',*,*,#8806,.F.);
#13834=ORIENTED_EDGE('',*,*,#8812,.F.);
#13835=ORIENTED_EDGE('',*,*,#8811,.F.);
#13836=ORIENTED_EDGE('',*,*,#8817,.F.);
#13837=ORIENTED_EDGE('',*,*,#8816,.F.);
#13838=ORIENTED_EDGE('',*,*,#8822,.F.);
#13839=ORIENTED_EDGE('',*,*,#8821,.F.);
#13840=ORIENTED_EDGE('',*,*,#8827,.F.);
#13841=ORIENTED_EDGE('',*,*,#8826,.F.);
#13842=ORIENTED_EDGE('',*,*,#8832,.F.);
#13843=ORIENTED_EDGE('',*,*,#8831,.F.);
#13844=ORIENTED_EDGE('',*,*,#8837,.F.);
#13845=ORIENTED_EDGE('',*,*,#8836,.F.);
#13846=ORIENTED_EDGE('',*,*,#8842,.F.);
#13847=ORIENTED_EDGE('',*,*,#8841,.F.);
#13848=ORIENTED_EDGE('',*,*,#8847,.F.);
#13849=ORIENTED_EDGE('',*,*,#8846,.F.);
#13850=ORIENTED_EDGE('',*,*,#8852,.F.);
#13851=ORIENTED_EDGE('',*,*,#8851,.F.);
#13852=ORIENTED_EDGE('',*,*,#8857,.F.);
#13853=ORIENTED_EDGE('',*,*,#8856,.F.);
#13854=ORIENTED_EDGE('',*,*,#8862,.F.);
#13855=ORIENTED_EDGE('',*,*,#8861,.F.);
#13856=ORIENTED_EDGE('',*,*,#8875,.F.);
#13857=ORIENTED_EDGE('',*,*,#8876,.F.);
#13858=ORIENTED_EDGE('',*,*,#8868,.F.);
#13859=ORIENTED_EDGE('',*,*,#8877,.F.);
#13860=ORIENTED_EDGE('',*,*,#8878,.T.);
#13861=ORIENTED_EDGE('',*,*,#8879,.T.);
#13862=ORIENTED_EDGE('',*,*,#8880,.T.);
#13863=ORIENTED_EDGE('',*,*,#8881,.T.);
#13864=ORIENTED_EDGE('',*,*,#8882,.T.);
#13865=ORIENTED_EDGE('',*,*,#8883,.T.);
#13866=ORIENTED_EDGE('',*,*,#8884,.T.);
#13867=ORIENTED_EDGE('',*,*,#8885,.T.);
#13868=ORIENTED_EDGE('',*,*,#8886,.T.);
#13869=ORIENTED_EDGE('',*,*,#8887,.T.);
#13870=ORIENTED_EDGE('',*,*,#8888,.T.);
#13871=ORIENTED_EDGE('',*,*,#8889,.T.);
#13872=ORIENTED_EDGE('',*,*,#8890,.T.);
#13873=ORIENTED_EDGE('',*,*,#8891,.T.);
#13874=ORIENTED_EDGE('',*,*,#8892,.T.);
#13875=ORIENTED_EDGE('',*,*,#8893,.T.);
#13876=ORIENTED_EDGE('',*,*,#8894,.T.);
#13877=ORIENTED_EDGE('',*,*,#8895,.T.);
#13878=ORIENTED_EDGE('',*,*,#8896,.F.);
#13879=ORIENTED_EDGE('',*,*,#8870,.F.);
#13880=ORIENTED_EDGE('',*,*,#8897,.F.);
#13881=ORIENTED_EDGE('',*,*,#8898,.F.);
#13882=ORIENTED_EDGE('',*,*,#8899,.F.);
#13883=ORIENTED_EDGE('',*,*,#8895,.F.);
#13884=ORIENTED_EDGE('',*,*,#8894,.F.);
#13885=ORIENTED_EDGE('',*,*,#8893,.F.);
#13886=ORIENTED_EDGE('',*,*,#8892,.F.);
#13887=ORIENTED_EDGE('',*,*,#8891,.F.);
#13888=ORIENTED_EDGE('',*,*,#8890,.F.);
#13889=ORIENTED_EDGE('',*,*,#8889,.F.);
#13890=ORIENTED_EDGE('',*,*,#8888,.F.);
#13891=ORIENTED_EDGE('',*,*,#8887,.F.);
#13892=ORIENTED_EDGE('',*,*,#8886,.F.);
#13893=ORIENTED_EDGE('',*,*,#8885,.F.);
#13894=ORIENTED_EDGE('',*,*,#8884,.F.);
#13895=ORIENTED_EDGE('',*,*,#8883,.F.);
#13896=ORIENTED_EDGE('',*,*,#8882,.F.);
#13897=ORIENTED_EDGE('',*,*,#8881,.F.);
#13898=ORIENTED_EDGE('',*,*,#8880,.F.);
#13899=ORIENTED_EDGE('',*,*,#8879,.F.);
#13900=ORIENTED_EDGE('',*,*,#8878,.F.);
#13901=ORIENTED_EDGE('',*,*,#8900,.F.);
#13902=ORIENTED_EDGE('',*,*,#8901,.F.);
#13903=ORIENTED_EDGE('',*,*,#8902,.F.);
#13904=ORIENTED_EDGE('',*,*,#8903,.F.);
#13905=ORIENTED_EDGE('',*,*,#8904,.F.);
#13906=ORIENTED_EDGE('',*,*,#8905,.F.);
#13907=ORIENTED_EDGE('',*,*,#8906,.F.);
#13908=ORIENTED_EDGE('',*,*,#8907,.F.);
#13909=ORIENTED_EDGE('',*,*,#8908,.F.);
#13910=ORIENTED_EDGE('',*,*,#8909,.F.);
#13911=ORIENTED_EDGE('',*,*,#8910,.F.);
#13912=ORIENTED_EDGE('',*,*,#8911,.F.);
#13913=ORIENTED_EDGE('',*,*,#8912,.F.);
#13914=ORIENTED_EDGE('',*,*,#8913,.F.);
#13915=ORIENTED_EDGE('',*,*,#8914,.F.);
#13916=ORIENTED_EDGE('',*,*,#8915,.F.);
#13917=ORIENTED_EDGE('',*,*,#8916,.F.);
#13918=ORIENTED_EDGE('',*,*,#8917,.F.);
#13919=ORIENTED_EDGE('',*,*,#8918,.F.);
#13920=ORIENTED_EDGE('',*,*,#8865,.T.);
#13921=ORIENTED_EDGE('',*,*,#8876,.T.);
#13922=ORIENTED_EDGE('',*,*,#8875,.T.);
#13923=ORIENTED_EDGE('',*,*,#8860,.F.);
#13924=ORIENTED_EDGE('',*,*,#8919,.F.);
#13925=ORIENTED_EDGE('',*,*,#8920,.F.);
#13926=ORIENTED_EDGE('',*,*,#8921,.F.);
#13927=ORIENTED_EDGE('',*,*,#8922,.F.);
#13928=ORIENTED_EDGE('',*,*,#8923,.F.);
#13929=ORIENTED_EDGE('',*,*,#8924,.F.);
#13930=ORIENTED_EDGE('',*,*,#8925,.F.);
#13931=ORIENTED_EDGE('',*,*,#8918,.T.);
#13932=ORIENTED_EDGE('',*,*,#8917,.T.);
#13933=ORIENTED_EDGE('',*,*,#8916,.T.);
#13934=ORIENTED_EDGE('',*,*,#8915,.T.);
#13935=ORIENTED_EDGE('',*,*,#8914,.T.);
#13936=ORIENTED_EDGE('',*,*,#8913,.T.);
#13937=ORIENTED_EDGE('',*,*,#8912,.T.);
#13938=ORIENTED_EDGE('',*,*,#8911,.T.);
#13939=ORIENTED_EDGE('',*,*,#8910,.T.);
#13940=ORIENTED_EDGE('',*,*,#8909,.T.);
#13941=ORIENTED_EDGE('',*,*,#8908,.T.);
#13942=ORIENTED_EDGE('',*,*,#8907,.T.);
#13943=ORIENTED_EDGE('',*,*,#8906,.T.);
#13944=ORIENTED_EDGE('',*,*,#8905,.T.);
#13945=ORIENTED_EDGE('',*,*,#8904,.T.);
#13946=ORIENTED_EDGE('',*,*,#8903,.T.);
#13947=ORIENTED_EDGE('',*,*,#8902,.T.);
#13948=ORIENTED_EDGE('',*,*,#8901,.T.);
#13949=ORIENTED_EDGE('',*,*,#8926,.F.);
#13950=ORIENTED_EDGE('',*,*,#8898,.T.);
#13951=ORIENTED_EDGE('',*,*,#8927,.F.);
#13952=ORIENTED_EDGE('',*,*,#8928,.F.);
#13953=ORIENTED_EDGE('',*,*,#8866,.T.);
#13954=ORIENTED_EDGE('',*,*,#8920,.T.);
#13955=ORIENTED_EDGE('',*,*,#8919,.T.);
#13956=ORIENTED_EDGE('',*,*,#8864,.T.);
#13957=ORIENTED_EDGE('',*,*,#8863,.T.);
#13958=ORIENTED_EDGE('',*,*,#8859,.T.);
#13959=ORIENTED_EDGE('',*,*,#8858,.T.);
#13960=ORIENTED_EDGE('',*,*,#8854,.T.);
#13961=ORIENTED_EDGE('',*,*,#8853,.T.);
#13962=ORIENTED_EDGE('',*,*,#8849,.T.);
#13963=ORIENTED_EDGE('',*,*,#8848,.T.);
#13964=ORIENTED_EDGE('',*,*,#8844,.T.);
#13965=ORIENTED_EDGE('',*,*,#8843,.T.);
#13966=ORIENTED_EDGE('',*,*,#8839,.T.);
#13967=ORIENTED_EDGE('',*,*,#8838,.T.);
#13968=ORIENTED_EDGE('',*,*,#8834,.T.);
#13969=ORIENTED_EDGE('',*,*,#8833,.T.);
#13970=ORIENTED_EDGE('',*,*,#8829,.T.);
#13971=ORIENTED_EDGE('',*,*,#8828,.T.);
#13972=ORIENTED_EDGE('',*,*,#8824,.T.);
#13973=ORIENTED_EDGE('',*,*,#8823,.T.);
#13974=ORIENTED_EDGE('',*,*,#8819,.T.);
#13975=ORIENTED_EDGE('',*,*,#8818,.T.);
#13976=ORIENTED_EDGE('',*,*,#8814,.T.);
#13977=ORIENTED_EDGE('',*,*,#8813,.T.);
#13978=ORIENTED_EDGE('',*,*,#8809,.T.);
#13979=ORIENTED_EDGE('',*,*,#8808,.T.);
#13980=ORIENTED_EDGE('',*,*,#8804,.T.);
#13981=ORIENTED_EDGE('',*,*,#8803,.T.);
#13982=ORIENTED_EDGE('',*,*,#8799,.T.);
#13983=ORIENTED_EDGE('',*,*,#8798,.T.);
#13984=ORIENTED_EDGE('',*,*,#8794,.T.);
#13985=ORIENTED_EDGE('',*,*,#8793,.T.);
#13986=ORIENTED_EDGE('',*,*,#8789,.T.);
#13987=ORIENTED_EDGE('',*,*,#8788,.T.);
#13988=ORIENTED_EDGE('',*,*,#8929,.F.);
#13989=ORIENTED_EDGE('',*,*,#8923,.T.);
#13990=ORIENTED_EDGE('',*,*,#8922,.T.);
#13991=ORIENTED_EDGE('',*,*,#8930,.F.);
#13992=ORIENTED_EDGE('',*,*,#8931,.F.);
#13993=ORIENTED_EDGE('',*,*,#8932,.F.);
#13994=ORIENTED_EDGE('',*,*,#8873,.F.);
#13995=ORIENTED_EDGE('',*,*,#8933,.F.);
#13996=ORIENTED_EDGE('',*,*,#8931,.T.);
#13997=ORIENTED_EDGE('',*,*,#8934,.F.);
#13998=ORIENTED_EDGE('',*,*,#8935,.T.);
#13999=ORIENTED_EDGE('',*,*,#8871,.T.);
#14000=ORIENTED_EDGE('',*,*,#8896,.T.);
#14001=ORIENTED_EDGE('',*,*,#8926,.T.);
#14002=ORIENTED_EDGE('',*,*,#8900,.T.);
#14003=ORIENTED_EDGE('',*,*,#8877,.T.);
#14004=ORIENTED_EDGE('',*,*,#8867,.T.);
#14005=ORIENTED_EDGE('',*,*,#8928,.T.);
#14006=ORIENTED_EDGE('',*,*,#8936,.T.);
#14007=ORIENTED_EDGE('',*,*,#8937,.T.);
#14008=ORIENTED_EDGE('',*,*,#8936,.F.);
#14009=ORIENTED_EDGE('',*,*,#8927,.T.);
#14010=ORIENTED_EDGE('',*,*,#8897,.T.);
#14011=ORIENTED_EDGE('',*,*,#8869,.T.);
#14012=ORIENTED_EDGE('',*,*,#8935,.F.);
#14013=ORIENTED_EDGE('',*,*,#8929,.T.);
#14014=ORIENTED_EDGE('',*,*,#8787,.T.);
#14015=ORIENTED_EDGE('',*,*,#8874,.T.);
#14016=ORIENTED_EDGE('',*,*,#8932,.T.);
#14017=ORIENTED_EDGE('',*,*,#8933,.T.);
#14018=ORIENTED_EDGE('',*,*,#8930,.T.);
#14019=ORIENTED_EDGE('',*,*,#8872,.T.);
#14020=ORIENTED_EDGE('',*,*,#8899,.T.);
#14021=ORIENTED_EDGE('',*,*,#8925,.T.);
#14022=ORIENTED_EDGE('',*,*,#8921,.T.);
#14023=ORIENTED_EDGE('',*,*,#8924,.T.);
#14024=ORIENTED_EDGE('',*,*,#8937,.F.);
#14025=ORIENTED_EDGE('',*,*,#8934,.T.);
#14439=CYLINDRICAL_SURFACE('',#15609,4.91825);
#14440=CYLINDRICAL_SURFACE('',#15610,4.91825);
#14441=CYLINDRICAL_SURFACE('',#15611,4.91825);
#14442=CYLINDRICAL_SURFACE('',#15612,4.91825);
#14443=CYLINDRICAL_SURFACE('',#15613,4.91825);
#14444=CYLINDRICAL_SURFACE('',#15614,4.91825);
#14445=CYLINDRICAL_SURFACE('',#15615,4.91825);
#14446=CYLINDRICAL_SURFACE('',#15616,4.91825);
#14447=CYLINDRICAL_SURFACE('',#15617,4.91825);
#14448=CYLINDRICAL_SURFACE('',#15618,4.91825);
#14449=CYLINDRICAL_SURFACE('',#15619,4.91825);
#14450=CYLINDRICAL_SURFACE('',#15620,4.91825);
#14451=CYLINDRICAL_SURFACE('',#15621,4.91825);
#14452=CYLINDRICAL_SURFACE('',#15622,4.91825);
#14453=CYLINDRICAL_SURFACE('',#15623,4.91825);
#14454=CYLINDRICAL_SURFACE('',#15624,4.91825);
#14455=CYLINDRICAL_SURFACE('',#15625,4.91825);
#14456=CYLINDRICAL_SURFACE('',#15626,5.91675);
#14457=CYLINDRICAL_SURFACE('',#15627,5.91675);
#14458=CYLINDRICAL_SURFACE('',#15628,4.91825);
#14459=CYLINDRICAL_SURFACE('',#15629,4.91825);
#14460=CYLINDRICAL_SURFACE('',#15630,5.91675);
#14461=CYLINDRICAL_SURFACE('',#15631,15.2420394990918);
#14895=ADVANCED_FACE('',(#2537),#14439,.F.);
#14896=ADVANCED_FACE('',(#2538),#14440,.F.);
#14897=ADVANCED_FACE('',(#2539),#14441,.F.);
#14898=ADVANCED_FACE('',(#2540),#14442,.F.);
#14899=ADVANCED_FACE('',(#2541),#14443,.F.);
#14900=ADVANCED_FACE('',(#2542),#14444,.F.);
#14901=ADVANCED_FACE('',(#2543),#14445,.F.);
#14902=ADVANCED_FACE('',(#2544),#14446,.F.);
#14903=ADVANCED_FACE('',(#2545),#14447,.F.);
#14904=ADVANCED_FACE('',(#2546),#14448,.F.);
#14905=ADVANCED_FACE('',(#2547),#14449,.F.);
#14906=ADVANCED_FACE('',(#2548),#14450,.F.);
#14907=ADVANCED_FACE('',(#2549),#14451,.F.);
#14908=ADVANCED_FACE('',(#2550),#14452,.F.);
#14909=ADVANCED_FACE('',(#2551),#14453,.F.);
#14910=ADVANCED_FACE('',(#2552),#14454,.F.);
#14911=ADVANCED_FACE('',(#2553),#14455,.F.);
#14912=ADVANCED_FACE('',(#2554),#53,.T.);
#14913=ADVANCED_FACE('',(#2555),#54,.T.);
#14914=ADVANCED_FACE('',(#2556),#14456,.F.);
#14915=ADVANCED_FACE('',(#2557),#14457,.F.);
#14916=ADVANCED_FACE('',(#2558),#14458,.F.);
#14917=ADVANCED_FACE('',(#2559),#14459,.F.);
#14918=ADVANCED_FACE('',(#2560),#55,.T.);
#14919=ADVANCED_FACE('',(#2561),#14460,.F.);
#14920=ADVANCED_FACE('',(#2562),#56,.T.);
#14921=ADVANCED_FACE('',(#2563,#2017),#14461,.T.);
#14922=ADVANCED_FACE('',(#2564),#2100,.F.);
#14923=ADVANCED_FACE('',(#2565),#2101,.T.);
#14945=CLOSED_SHELL('',(#14895,#14896,#14897,#14898,#14899,#14900,#14901,
#14902,#14903,#14904,#14905,#14906,#14907,#14908,#14909,#14910,#14911,#14912,
#14913,#14914,#14915,#14916,#14917,#14918,#14919,#14920,#14921,#14922,#14923));
#15608=AXIS2_PLACEMENT_3D('',#240805,#17285,#17286);
#15609=AXIS2_PLACEMENT_3D('',#240806,#17287,#17288);
#15610=AXIS2_PLACEMENT_3D('',#241157,#17290,#17291);
#15611=AXIS2_PLACEMENT_3D('',#241617,#17293,#17294);
#15612=AXIS2_PLACEMENT_3D('',#241870,#17296,#17297);
#15613=AXIS2_PLACEMENT_3D('',#242129,#17299,#17300);
#15614=AXIS2_PLACEMENT_3D('',#242592,#17302,#17303);
#15615=AXIS2_PLACEMENT_3D('',#243058,#17305,#17306);
#15616=AXIS2_PLACEMENT_3D('',#243521,#17308,#17309);
#15617=AXIS2_PLACEMENT_3D('',#243987,#17311,#17312);
#15618=AXIS2_PLACEMENT_3D('',#244450,#17314,#17315);
#15619=AXIS2_PLACEMENT_3D('',#244919,#17317,#17318);
#15620=AXIS2_PLACEMENT_3D('',#245388,#17320,#17321);
#15621=AXIS2_PLACEMENT_3D('',#245848,#17323,#17324);
#15622=AXIS2_PLACEMENT_3D('',#246314,#17326,#17327);
#15623=AXIS2_PLACEMENT_3D('',#246777,#17329,#17330);
#15624=AXIS2_PLACEMENT_3D('',#247240,#17332,#17333);
#15625=AXIS2_PLACEMENT_3D('',#247703,#17335,#17336);
#15626=AXIS2_PLACEMENT_3D('',#263671,#17338,#17339);
#15627=AXIS2_PLACEMENT_3D('',#263690,#17340,#17341);
#15628=AXIS2_PLACEMENT_3D('',#265076,#17342,#17343);
#15629=AXIS2_PLACEMENT_3D('',#265311,#17344,#17345);
#15630=AXIS2_PLACEMENT_3D('',#272334,#17346,#17347);
#15631=AXIS2_PLACEMENT_3D('',#279156,#17348,#17349);
#15632=AXIS2_PLACEMENT_3D('',#279158,#17350,#17351);
#15633=AXIS2_PLACEMENT_3D('',#279162,#17354,#17355);
#15634=AXIS2_PLACEMENT_3D('',#279163,#17356,#17357);
#15635=AXIS2_PLACEMENT_3D('',#279164,#17358,#17359);
#17285=DIRECTION('axis',(0.,0.,1.));
#17286=DIRECTION('refdir',(1.,0.,0.));
#17287=DIRECTION('center_axis',(-1.,0.,0.));
#17288=DIRECTION('ref_axis',(0.,0.968648305440766,0.248436028721142));
#17289=DIRECTION('',(-1.,0.,0.));
#17290=DIRECTION('center_axis',(-1.,0.,0.));
#17291=DIRECTION('ref_axis',(0.,0.968648305440766,0.248436028721142));
#17292=DIRECTION('',(-1.,0.,0.));
#17293=DIRECTION('center_axis',(-1.,0.,0.));
#17294=DIRECTION('ref_axis',(0.,0.968648305440766,0.248436028721142));
#17295=DIRECTION('',(-1.,0.,0.));
#17296=DIRECTION('center_axis',(-1.,0.,0.));
#17297=DIRECTION('ref_axis',(0.,0.968648305440766,0.248436028721142));
#17298=DIRECTION('',(-1.,0.,0.));
#17299=DIRECTION('center_axis',(-1.,0.,0.));
#17300=DIRECTION('ref_axis',(0.,0.968648305440766,0.248436028721142));
#17301=DIRECTION('',(-1.,0.,0.));
#17302=DIRECTION('center_axis',(-1.,0.,0.));
#17303=DIRECTION('ref_axis',(0.,0.968648305440766,0.248436028721142));
#17304=DIRECTION('',(-1.,0.,0.));
#17305=DIRECTION('center_axis',(-1.,0.,0.));
#17306=DIRECTION('ref_axis',(0.,0.968648305440766,0.248436028721142));
#17307=DIRECTION('',(-1.,0.,0.));
#17308=DIRECTION('center_axis',(-1.,0.,0.));
#17309=DIRECTION('ref_axis',(0.,0.968648305440766,0.248436028721142));
#17310=DIRECTION('',(-1.,0.,0.));
#17311=DIRECTION('center_axis',(-1.,0.,0.));
#17312=DIRECTION('ref_axis',(0.,0.968648305440766,0.248436028721142));
#17313=DIRECTION('',(-1.,0.,0.));
#17314=DIRECTION('center_axis',(-1.,0.,0.));
#17315=DIRECTION('ref_axis',(0.,0.968648305440766,0.248436028721142));
#17316=DIRECTION('',(-1.,0.,0.));
#17317=DIRECTION('center_axis',(-1.,0.,0.));
#17318=DIRECTION('ref_axis',(0.,0.968648305440766,0.248436028721142));
#17319=DIRECTION('',(-1.,0.,0.));
#17320=DIRECTION('center_axis',(-1.,0.,0.));
#17321=DIRECTION('ref_axis',(0.,0.968648305440766,0.248436028721142));
#17322=DIRECTION('',(-1.,0.,0.));
#17323=DIRECTION('center_axis',(-1.,0.,0.));
#17324=DIRECTION('ref_axis',(0.,0.968648305440766,0.248436028721142));
#17325=DIRECTION('',(-1.,0.,0.));
#17326=DIRECTION('center_axis',(-1.,0.,0.));
#17327=DIRECTION('ref_axis',(0.,0.968648305440766,0.248436028721142));
#17328=DIRECTION('',(-1.,0.,0.));
#17329=DIRECTION('center_axis',(-1.,0.,0.));
#17330=DIRECTION('ref_axis',(0.,0.968648305440766,0.248436028721142));
#17331=DIRECTION('',(-1.,0.,0.));
#17332=DIRECTION('center_axis',(-1.,0.,0.));
#17333=DIRECTION('ref_axis',(0.,0.968648305440766,0.248436028721142));
#17334=DIRECTION('',(-1.,0.,0.));
#17335=DIRECTION('center_axis',(-1.,0.,0.));
#17336=DIRECTION('ref_axis',(0.,0.968648305440766,0.248436028721142));
#17337=DIRECTION('',(-1.,0.,0.));
#17338=DIRECTION('center_axis',(-1.,0.,0.));
#17339=DIRECTION('ref_axis',(0.,1.,0.));
#17340=DIRECTION('center_axis',(-1.,0.,0.));
#17341=DIRECTION('ref_axis',(0.,1.,0.));
#17342=DIRECTION('center_axis',(-1.,0.,0.));
#17343=DIRECTION('ref_axis',(0.,0.968648305440766,0.248436028721142));
#17344=DIRECTION('center_axis',(-1.,0.,0.));
#17345=DIRECTION('ref_axis',(0.,-0.960836623023769,-0.277115470257942));
#17346=DIRECTION('center_axis',(-1.,0.,0.));
#17347=DIRECTION('ref_axis',(0.,1.,0.));
#17348=DIRECTION('center_axis',(0.,1.,0.));
#17349=DIRECTION('ref_axis',(-1.,0.,0.));
#17350=DIRECTION('center_axis',(0.,1.,0.));
#17351=DIRECTION('ref_axis',(-1.,0.,0.));
#17352=DIRECTION('',(0.,-1.,0.));
#17353=DIRECTION('',(0.,-1.,0.));
#17354=DIRECTION('center_axis',(0.,1.,0.));
#17355=DIRECTION('ref_axis',(-1.,0.,0.));
#17356=DIRECTION('center_axis',(0.,1.,0.));
#17357=DIRECTION('ref_axis',(-1.,0.,0.));
#17358=DIRECTION('center_axis',(0.,1.,0.));
#17359=DIRECTION('ref_axis',(-1.,0.,0.));
#240805=CARTESIAN_POINT('',(0.,0.,0.));
#240806=CARTESIAN_POINT('Origin',(213.235140564004,0.,130.804360617566));
#240807=CARTESIAN_POINT('',(-205.820054717884,-4.76405452823395,129.582490119308));
#240808=CARTESIAN_POINT('',(-206.164998470905,-4.76405452823394,129.582490119308));
#240809=CARTESIAN_POINT('',(213.235140564004,-4.76405452823405,129.582490119308));
#240810=CARTESIAN_POINT('',(-206.235140563976,-4.91824935292959,130.806883494435));
#240811=CARTESIAN_POINT('Ctrl Pts',(-206.164998470905,-4.76405452823394,
129.582490119308));
#240812=CARTESIAN_POINT('Ctrl Pts',(-206.172665944474,-4.79776118631657,
129.713911867602));
#240813=CARTESIAN_POINT('Ctrl Pts',(-206.180333418043,-4.82600172992664,
129.846636618208));
#240814=CARTESIAN_POINT('Ctrl Pts',(-206.188000891612,-4.84869920343357,
129.980164586805));
#240815=CARTESIAN_POINT('Ctrl Pts',(-206.195857503673,-4.87195657008729,
130.116986375504));
#240816=CARTESIAN_POINT('Ctrl Pts',(-206.203714115733,-4.88939378574457,
130.254651075192));
#240817=CARTESIAN_POINT('Ctrl Pts',(-206.211570727794,-4.90098467145666,
130.392617599839));
#240818=CARTESIAN_POINT('Ctrl Pts',(-206.219427339854,-4.91257555716875,
130.530584124486));
#240819=CARTESIAN_POINT('Ctrl Pts',(-206.227283951915,-4.91832015787954,
130.668852025862));
#240820=CARTESIAN_POINT('Ctrl Pts',(-206.235140563975,-4.91824935292959,
130.806883494435));
#240821=CARTESIAN_POINT('',(-207.389991015301,2.65316544558642,126.664162929598));
#240822=CARTESIAN_POINT('Ctrl Pts',(-206.235140564013,-4.91824935292925,
130.806883495092));
#240823=CARTESIAN_POINT('Ctrl Pts',(-206.243296577379,-4.91817584971133,
130.950175093808));
#240824=CARTESIAN_POINT('Ctrl Pts',(-206.251452590746,-4.9118408081057,
131.09330184757));
#240825=CARTESIAN_POINT('Ctrl Pts',(-206.259608604113,-4.89928367079141,
131.235872582194));
#240826=CARTESIAN_POINT('Ctrl Pts',(-206.267382938232,-4.88731417335877,
131.371771394107));
#240827=CARTESIAN_POINT('Ctrl Pts',(-206.275157272351,-4.86966698677397,
131.507387058606));
#240828=CARTESIAN_POINT('Ctrl Pts',(-206.28293160647,-4.846359096209,131.64220700748));
#240829=CARTESIAN_POINT('Ctrl Pts',(-206.290696359417,-4.82307993053606,
131.776860802817));
#240830=CARTESIAN_POINT('Ctrl Pts',(-206.298461112364,-4.79415400762733,
131.910720452176));
#240831=CARTESIAN_POINT('Ctrl Pts',(-206.306225865311,-4.75965019918353,
132.043276693784));
#240832=CARTESIAN_POINT('Ctrl Pts',(-206.313982906196,-4.72518066040869,
132.175701278665));
#240833=CARTESIAN_POINT('Ctrl Pts',(-206.321739947081,-4.68514435886508,
132.306824656126));
#240834=CARTESIAN_POINT('Ctrl Pts',(-206.329496987965,-4.63966146046592,
132.436146324933));
#240835=CARTESIAN_POINT('Ctrl Pts',(-206.337248179205,-4.59421286107431,
132.565370471264));
#240836=CARTESIAN_POINT('Ctrl Pts',(-206.344999370445,-4.5433259693909,
132.69279524599));
#240837=CARTESIAN_POINT('Ctrl Pts',(-206.352750561685,-4.48717107061851,
132.817934267946));
#240838=CARTESIAN_POINT('Ctrl Pts',(-206.360498458462,-4.43104003917615,
132.943020102479));
#240839=CARTESIAN_POINT('Ctrl Pts',(-206.368246355239,-4.36964561366111,
133.065821760543));
#240840=CARTESIAN_POINT('Ctrl Pts',(-206.375994252016,-4.30320651608381,
133.185872058318));
#240841=CARTESIAN_POINT('Ctrl Pts',(-206.3837405281,-4.23678131613346,133.305897244159));
#240842=CARTESIAN_POINT('Ctrl Pts',(-206.391486804184,-4.16531373223735,
133.423171872606));
#240843=CARTESIAN_POINT('Ctrl Pts',(-206.399233080268,-4.08906864095504,
133.537252988674));
#240844=CARTESIAN_POINT('Ctrl Pts',(-206.406979413534,-4.01282298684869,
133.651334946862));
#240845=CARTESIAN_POINT('Ctrl Pts',(-206.414725746799,-3.93179997222957,
133.762223020581));
#240846=CARTESIAN_POINT('Ctrl Pts',(-206.422472080064,-3.84630781202687,
133.869503237028));
#240847=CARTESIAN_POINT('Ctrl Pts',(-206.430220148067,-3.76079650644777,
133.976807478135));
#240848=CARTESIAN_POINT('Ctrl Pts',(-206.43796821607,-3.67081430735097,
134.080501948538));
#240849=CARTESIAN_POINT('Ctrl Pts',(-206.445716284073,-3.5767094513966,
134.180206076527));
#240850=CARTESIAN_POINT('Ctrl Pts',(-206.453472586815,-3.48250457968159,
134.280016171251));
#240851=CARTESIAN_POINT('Ctrl Pts',(-206.461228889557,-3.38416856715666,
134.375827166964));
#240852=CARTESIAN_POINT('Ctrl Pts',(-206.468985192298,-3.28208662334993,
134.467295296116));
#240853=CARTESIAN_POINT('Ctrl Pts',(-206.476745634812,-3.17995019533615,
134.558812244563));
#240854=CARTESIAN_POINT('Ctrl Pts',(-206.484506077326,-3.07406415392714,
134.645981459434));
#240855=CARTESIAN_POINT('Ctrl Pts',(-206.49226651984,-2.96484568166884,
134.728500414565));
#240856=CARTESIAN_POINT('Ctrl Pts',(-206.500039420106,-2.8554518822229,
134.811151836448));
#240857=CARTESIAN_POINT('Ctrl Pts',(-206.507812320371,-2.74271528361125,
134.889137858572));
#240858=CARTESIAN_POINT('Ctrl Pts',(-206.515585220636,-2.62708159836639,
134.962199640186));
#240859=CARTESIAN_POINT('Ctrl Pts',(-206.523075556399,-2.51565148882853,
135.032605442017));
#240860=CARTESIAN_POINT('Ctrl Pts',(-206.530565892162,-2.40153153536177,
135.098438650812));
#240861=CARTESIAN_POINT('Ctrl Pts',(-206.538056227925,-2.2851392588354,
135.159509481868));
#240862=CARTESIAN_POINT('Ctrl Pts',(-206.545830562044,-2.16433393378268,
135.222895832038));
#240863=CARTESIAN_POINT('Ctrl Pts',(-206.553604896163,-2.04069789899693,
135.281352333429));
#240864=CARTESIAN_POINT('Ctrl Pts',(-206.561379230282,-1.91467157352999,
135.334616220511));
#240865=CARTESIAN_POINT('Ctrl Pts',(-206.56914398323,-1.78880056424624,
135.387814464613));
#240866=CARTESIAN_POINT('Ctrl Pts',(-206.576908736177,-1.66054548224971,
135.435832676627));
#240867=CARTESIAN_POINT('Ctrl Pts',(-206.584673489124,-1.53037201072842,
135.478453531841));
#240868=CARTESIAN_POINT('Ctrl Pts',(-206.592430530009,-1.40032782933418,
135.521032055421));
#240869=CARTESIAN_POINT('Ctrl Pts',(-206.600187570894,-1.26836941934266,
135.55822376943));
#240870=CARTESIAN_POINT('Ctrl Pts',(-206.607944611779,-1.13498281922694,
135.589859239712));
#240871=CARTESIAN_POINT('Ctrl Pts',(-206.615695803019,-1.00169680698415,
135.62147085344));
#240872=CARTESIAN_POINT('Ctrl Pts',(-206.623446994259,-0.866985127212026,
135.647534473537));
#240873=CARTESIAN_POINT('Ctrl Pts',(-206.631198185499,-0.731349029471388,
135.667930464869));
#240874=CARTESIAN_POINT('Ctrl Pts',(-206.638946082276,-0.595770580690315,
135.688317787359));
#240875=CARTESIAN_POINT('Ctrl Pts',(-206.646693979053,-0.459268881202547,
135.703042214174));
#240876=CARTESIAN_POINT('Ctrl Pts',(-206.65444187583,-0.322355210575576,
135.712035238068));
#240877=CARTESIAN_POINT('Ctrl Pts',(-206.662188151914,-0.185470179336983,
135.721026380815));
#240878=CARTESIAN_POINT('Ctrl Pts',(-206.669934427998,-0.0481737382443191,
135.724288479683));
#240879=CARTESIAN_POINT('Ctrl Pts',(-206.677680704082,0.0890182698783709,
135.721804954834));
#240880=CARTESIAN_POINT('Ctrl Pts',(-206.685427037348,0.226211290721486,
135.719321411652));
#240881=CARTESIAN_POINT('Ctrl Pts',(-206.693173370613,0.36329948615519,
135.711092167198));
#240882=CARTESIAN_POINT('Ctrl Pts',(-206.700919703878,0.499767971438338,
135.697152769009));
#240883=CARTESIAN_POINT('Ctrl Pts',(-206.708667771881,0.636267017892372,
135.683210249189));
#240884=CARTESIAN_POINT('Ctrl Pts',(-206.716415839884,0.772145689173082,
135.66355507079));
#240885=CARTESIAN_POINT('Ctrl Pts',(-206.724163907887,0.906895569102237,
135.638274506874));
#240886=CARTESIAN_POINT('Ctrl Pts',(-206.731920210629,1.04178866280751,
135.612967074473));
#240887=CARTESIAN_POINT('Ctrl Pts',(-206.739676513371,1.17555018377165,
135.582022385611));
#240888=CARTESIAN_POINT('Ctrl Pts',(-206.747432816113,1.30768269545861,
135.545578713214));
#240889=CARTESIAN_POINT('Ctrl Pts',(-206.755193258627,1.4398857302455,135.509115589732));
#240890=CARTESIAN_POINT('Ctrl Pts',(-206.762953701141,1.57045765127054,
135.467147754108));
#240891=CARTESIAN_POINT('Ctrl Pts',(-206.770714143655,1.69891843734635,
135.419862671053));
#240892=CARTESIAN_POINT('Ctrl Pts',(-206.77848704392,1.82758544008018,135.372501681785));
#240893=CARTESIAN_POINT('Ctrl Pts',(-206.786259944186,1.9541341744678,135.319806538378));
#240894=CARTESIAN_POINT('Ctrl Pts',(-206.794032844451,2.07810595194281,
135.262012321659));
#240895=CARTESIAN_POINT('Ctrl Pts',(-206.801523180213,2.19757104304053,
135.206319070292));
#240896=CARTESIAN_POINT('Ctrl Pts',(-206.809013515975,2.31464300846158,
135.145891178822));
#240897=CARTESIAN_POINT('Ctrl Pts',(-206.816503851737,2.42893649673259,
135.080977336111));
#240898=CARTESIAN_POINT('Ctrl Pts',(-206.824278185856,2.5475634573503,135.013602265324));
#240899=CARTESIAN_POINT('Ctrl Pts',(-206.832052519975,2.66357286432491,
134.941180934586));
#240900=CARTESIAN_POINT('Ctrl Pts',(-206.839826854094,2.77650558831772,
134.86394184973));
#240901=CARTESIAN_POINT('Ctrl Pts',(-206.847591607042,2.88929913282099,
134.786797955144));
#240902=CARTESIAN_POINT('Ctrl Pts',(-206.855356359989,2.99902321915925,
134.704848338791));
#240903=CARTESIAN_POINT('Ctrl Pts',(-206.863121112936,3.1052432927571,134.618367323812));
#240904=CARTESIAN_POINT('Ctrl Pts',(-206.870878153821,3.21135786708041,
134.531972202995));
#240905=CARTESIAN_POINT('Ctrl Pts',(-206.878635194706,3.31397505326374,
134.441054885293));
#240906=CARTESIAN_POINT('Ctrl Pts',(-206.886392235591,3.41268958588663,
134.345932705337));
#240907=CARTESIAN_POINT('Ctrl Pts',(-206.894143426831,3.51132967711271,
134.250882257758));
#240908=CARTESIAN_POINT('Ctrl Pts',(-206.901894618071,3.6060726922938,134.151633529634));
#240909=CARTESIAN_POINT('Ctrl Pts',(-206.909645809311,3.69654704137007,
134.048543570705));
#240910=CARTESIAN_POINT('Ctrl Pts',(-206.917393706088,3.78698293643439,
133.945497427759));
#240911=CARTESIAN_POINT('Ctrl Pts',(-206.925141602865,3.87315351654314,
133.838613594408));
#240912=CARTESIAN_POINT('Ctrl Pts',(-206.932889499642,3.95472478551692,
133.728285194794));
#240913=CARTESIAN_POINT('Ctrl Pts',(-206.940635775726,4.0362789915397,133.617979873503));
#240914=CARTESIAN_POINT('Ctrl Pts',(-206.948382051811,4.11323556776735,
133.504231733294));
#240915=CARTESIAN_POINT('Ctrl Pts',(-206.956128327895,4.18530173946635,
133.387465805536));
#240916=CARTESIAN_POINT('Ctrl Pts',(-206.96387466116,4.25736844314155,133.270699015839));
#240917=CARTESIAN_POINT('Ctrl Pts',(-206.971620994426,4.32454446491532,
133.150914726844));
#240918=CARTESIAN_POINT('Ctrl Pts',(-206.979367327691,4.38658140415818,
133.028565339977));
#240919=CARTESIAN_POINT('Ctrl Pts',(-206.987115395694,4.44863223614336,
132.906188553813));
#240920=CARTESIAN_POINT('Ctrl Pts',(-206.994863463697,4.50554151874139,
132.781245875352));
#240921=CARTESIAN_POINT('Ctrl Pts',(-207.0026115317,4.55710786588625,132.654212222743));
#240922=CARTESIAN_POINT('Ctrl Pts',(-207.010367834442,4.60872901835857,
132.527043557257));
#240923=CARTESIAN_POINT('Ctrl Pts',(-207.018124137184,4.65499574460735,
132.397779841151));
#240924=CARTESIAN_POINT('Ctrl Pts',(-207.025880439925,4.69575550096411,
132.266914321765));
#240925=CARTESIAN_POINT('Ctrl Pts',(-207.03364088244,4.73653701203008,132.13597895551));
#240926=CARTESIAN_POINT('Ctrl Pts',(-207.041401324954,4.77180559603988,
132.003440460087));
#240927=CARTESIAN_POINT('Ctrl Pts',(-207.049161767468,4.80145950918554,
131.86980402017));
#240928=CARTESIAN_POINT('Ctrl Pts',(-207.056934667734,4.83116102542514,
131.735953055175));
#240929=CARTESIAN_POINT('Ctrl Pts',(-207.064707567999,4.85522979093357,
131.601001008726));
#240930=CARTESIAN_POINT('Ctrl Pts',(-207.072480468265,4.87361565349489,
131.465460855434));
#240931=CARTESIAN_POINT('Ctrl Pts',(-207.079970804027,4.89133314364086,
131.33484792812));
#240932=CARTESIAN_POINT('Ctrl Pts',(-207.087461139788,4.90377370409151,
131.203689216588));
#240933=CARTESIAN_POINT('Ctrl Pts',(-207.09495147555,4.91093827194779,131.072443350353));
#240934=CARTESIAN_POINT('Ctrl Pts',(-207.102725809669,4.91837448657198,
130.936221257207));
#240935=CARTESIAN_POINT('Ctrl Pts',(-207.110500143789,4.92015028810036,
130.79947375931));
#240936=CARTESIAN_POINT('Ctrl Pts',(-207.118274477908,4.91620975433994,
130.66271064816));
#240937=CARTESIAN_POINT('Ctrl Pts',(-207.126039230855,4.91227407693521,
130.526116085322));
#240938=CARTESIAN_POINT('Ctrl Pts',(-207.133803983802,4.90263609258996,
130.389506334569));
#240939=CARTESIAN_POINT('Ctrl Pts',(-207.141568736749,4.88729170976703,
130.253395277329));
#240940=CARTESIAN_POINT('Ctrl Pts',(-207.149325777634,4.87196256720145,
130.11741940751));
#240941=CARTESIAN_POINT('Ctrl Pts',(-207.157082818519,4.85093834860235,
129.981941631508));
#240942=CARTESIAN_POINT('Ctrl Pts',(-207.164839859404,4.824266980725,129.847474437717));
#240943=CARTESIAN_POINT('Ctrl Pts',(-207.172591050644,4.79761572593367,
129.713108646683));
#240944=CARTESIAN_POINT('Ctrl Pts',(-207.180342241884,4.76532587402565,
129.579752302914));
#240945=CARTESIAN_POINT('Ctrl Pts',(-207.188093433124,4.72749696755391,
129.447911029756));
#240946=CARTESIAN_POINT('Ctrl Pts',(-207.195841329901,4.68968413937648,
129.316125792657));
#240947=CARTESIAN_POINT('Ctrl Pts',(-207.203589226679,4.64633704665318,
129.185854720425));
#240948=CARTESIAN_POINT('Ctrl Pts',(-207.211337123456,4.59760590276493,
129.057591306706));
#240949=CARTESIAN_POINT('Ctrl Pts',(-207.21908339954,4.54888495238146,128.929354722929));
#240950=CARTESIAN_POINT('Ctrl Pts',(-207.226829675624,4.49478232972868,
128.80312532759));
#240951=CARTESIAN_POINT('Ctrl Pts',(-207.234575951708,4.43549737384086,
128.6793791802));
#240952=CARTESIAN_POINT('Ctrl Pts',(-207.242322284973,4.37621198032504,
128.555632119344));
#240953=CARTESIAN_POINT('Ctrl Pts',(-207.250068618239,4.31174434616012,
128.434368695606));
#240954=CARTESIAN_POINT('Ctrl Pts',(-207.257814951504,4.24234082287173,
128.316042429493));
#240955=CARTESIAN_POINT('Ctrl Pts',(-207.265563019507,4.17292175714561,
128.197689665032));
#240956=CARTESIAN_POINT('Ctrl Pts',(-207.27331108751,4.09856480052667,128.082275704225));
#240957=CARTESIAN_POINT('Ctrl Pts',(-207.281059155513,4.01956066101754,
127.970226683734));
#240958=CARTESIAN_POINT('Ctrl Pts',(-207.288815458255,3.94047255496867,
127.858058576209));
#240959=CARTESIAN_POINT('Ctrl Pts',(-207.296571760996,3.85672762533503,
127.749262873077));
#240960=CARTESIAN_POINT('Ctrl Pts',(-207.304328063738,3.76865840149488,
127.644234525882));
#240961=CARTESIAN_POINT('Ctrl Pts',(-207.312088506252,3.68054217245802,
127.539150121895));
#240962=CARTESIAN_POINT('Ctrl Pts',(-207.319848948767,3.58809731371382,
127.437837369101));
#240963=CARTESIAN_POINT('Ctrl Pts',(-207.327609391281,3.4916938564228,127.340654932101));
#240964=CARTESIAN_POINT('Ctrl Pts',(-207.335382291546,3.3951356437441,127.243316489227));
#240965=CARTESIAN_POINT('Ctrl Pts',(-207.343155191812,3.29460642069608,
127.15012187765));
#240966=CARTESIAN_POINT('Ctrl Pts',(-207.350928092077,3.19051065884962,
127.061390567156));
#240967=CARTESIAN_POINT('Ctrl Pts',(-207.358418427839,3.09019904014599,
126.975884863298));
#240968=CARTESIAN_POINT('Ctrl Pts',(-207.365908763601,2.98657592832593,
126.894523780142));
#240969=CARTESIAN_POINT('Ctrl Pts',(-207.373399099363,2.88002768791472,
126.817554429733));
#240970=CARTESIAN_POINT('Ctrl Pts',(-207.378631136696,2.80560320424821,
126.763790950015));
#240971=CARTESIAN_POINT('Ctrl Pts',(-207.383863174029,2.72959351183089,
126.712054947007));
#240972=CARTESIAN_POINT('Ctrl Pts',(-207.389095211362,2.65211837414998,
126.662446664815));
#240973=CARTESIAN_POINT('',(-207.161386959855,0.717556610101921,125.938940090646));
#240974=CARTESIAN_POINT('Ctrl Pts',(-207.16240288731,0.705992749060373,
125.937045412982));
#240975=CARTESIAN_POINT('Ctrl Pts',(-207.181988187458,1.10669090187245,
125.995165748024));
#240976=CARTESIAN_POINT('Ctrl Pts',(-207.218876175974,1.50830544278856,
126.105044865929));
#240977=CARTESIAN_POINT('Ctrl Pts',(-207.303250137215,2.1584231714227,126.375368867204));
#240978=CARTESIAN_POINT('Ctrl Pts',(-207.34444557399,2.41814945805675,126.511911515592));
#240979=CARTESIAN_POINT('Ctrl Pts',(-207.388495272009,2.66099574923083,
126.668144389529));
#240980=CARTESIAN_POINT('',(-205.889859436046,-4.91824930584068,130.806973680448));
#240981=CARTESIAN_POINT('Ctrl Pts',(-205.889859436046,-4.91824930584068,
130.806973680447));
#240982=CARTESIAN_POINT('Ctrl Pts',(-205.898419073697,-4.91816863288146,
130.958814544507));
#240983=CARTESIAN_POINT('Ctrl Pts',(-205.906978711349,-4.91105222461682,
131.11040905316));
#240984=CARTESIAN_POINT('Ctrl Pts',(-205.915538349,-4.89699280558849,131.261136847809));
#240985=CARTESIAN_POINT('Ctrl Pts',(-205.924144711242,-4.88285664025042,
131.412687421976));
#240986=CARTESIAN_POINT('Ctrl Pts',(-205.932751073485,-4.86170154469193,
131.563361562213));
#240987=CARTESIAN_POINT('Ctrl Pts',(-205.941357435727,-4.8336719627189,
131.712544750507));
#240988=CARTESIAN_POINT('Ctrl Pts',(-205.949987994199,-4.80556357739427,
131.862147357658));
#240989=CARTESIAN_POINT('Ctrl Pts',(-205.95861855267,-4.77054211518795,
132.010250401408));
#240990=CARTESIAN_POINT('Ctrl Pts',(-205.967249111142,-4.72880199806623,
132.15625363315));
#240991=CARTESIAN_POINT('Ctrl Pts',(-205.975911032462,-4.68691020026427,
132.302787430473));
#240992=CARTESIAN_POINT('Ctrl Pts',(-205.984572953782,-4.63825094856085,
132.447205915682));
#240993=CARTESIAN_POINT('Ctrl Pts',(-205.993234875102,-4.58306805029199,
132.588925076725));
#240994=CARTESIAN_POINT('Ctrl Pts',(-205.995739908888,-4.5671091169981,
132.629910358551));
#240995=CARTESIAN_POINT('Ctrl Pts',(-205.998244942673,-4.55060485959071,
132.67067003316));
#240996=CARTESIAN_POINT('Ctrl Pts',(-206.000749976459,-4.53356188569129,
132.711190366418));
#240997=CARTESIAN_POINT('Ctrl Pts',(-206.008524310578,-4.48066927631869,
132.836944602228));
#240998=CARTESIAN_POINT('Ctrl Pts',(-206.016298644698,-4.42245657148283,
132.960695612929));
#240999=CARTESIAN_POINT('Ctrl Pts',(-206.024072978817,-4.35909645044119,
133.081960494246));
#241000=CARTESIAN_POINT('Ctrl Pts',(-206.031837731764,-4.29581441508608,
133.203075927434));
#241001=CARTESIAN_POINT('Ctrl Pts',(-206.039602484712,-4.22739776497256,
133.321710984359));
#241002=CARTESIAN_POINT('Ctrl Pts',(-206.047367237659,-4.15406757846652,
133.437401752078));
#241003=CARTESIAN_POINT('Ctrl Pts',(-206.055124278544,-4.0808102245355,
133.552977614096));
#241004=CARTESIAN_POINT('Ctrl Pts',(-206.06288131943,-4.00264925397073,
133.665614678334));
#241005=CARTESIAN_POINT('Ctrl Pts',(-206.070638360315,-3.91985191488636,
133.774873035965));
#241006=CARTESIAN_POINT('Ctrl Pts',(-206.078389551555,-3.83711701391935,
133.884049001019));
#241007=CARTESIAN_POINT('Ctrl Pts',(-206.086140742796,-3.7497529388275,
133.989851020585));
#241008=CARTESIAN_POINT('Ctrl Pts',(-206.093891934036,-3.65807035220528,
134.091867934792));
#241009=CARTESIAN_POINT('Ctrl Pts',(-206.101639830814,-3.5664267331282,
134.193841489089));
#241010=CARTESIAN_POINT('Ctrl Pts',(-206.109387727591,-3.47046851394157,
134.292032847568));
#241011=CARTESIAN_POINT('Ctrl Pts',(-206.117135624368,-3.37054661931243,
134.386063920401));
#241012=CARTESIAN_POINT('Ctrl Pts',(-206.124881900453,-3.2706456261893,
134.480075323962));
#241013=CARTESIAN_POINT('Ctrl Pts',(-206.132628176537,-3.16678289131879,
134.569927905073));
#241014=CARTESIAN_POINT('Ctrl Pts',(-206.140374452621,-3.0593458918801,
134.655280738308));
#241015=CARTESIAN_POINT('Ctrl Pts',(-206.148120785887,-2.95190809936603,
134.740634201599));
#241016=CARTESIAN_POINT('Ctrl Pts',(-206.155867119153,-2.84089629575584,
134.821487607538));
#241017=CARTESIAN_POINT('Ctrl Pts',(-206.163613452418,-2.72673037768329,
134.897540861572));
#241018=CARTESIAN_POINT('Ctrl Pts',(-206.171361520422,-2.61253889294479,
134.973611147205));
#241019=CARTESIAN_POINT('Ctrl Pts',(-206.179109588425,-2.49519221352086,
135.044878925172));
#241020=CARTESIAN_POINT('Ctrl Pts',(-206.186857656428,-2.37513814799737,
135.11108812699));
#241021=CARTESIAN_POINT('Ctrl Pts',(-206.19461395917,-2.25495648758455,
135.177367696735));
#241022=CARTESIAN_POINT('Ctrl Pts',(-206.202370261912,-2.13206203597101,
135.238577761457));
#241023=CARTESIAN_POINT('Ctrl Pts',(-206.210126564654,-2.00692657135467,
135.294508588367));
#241024=CARTESIAN_POINT('Ctrl Pts',(-206.217887007169,-1.88172431817278,
135.350469267244));
#241025=CARTESIAN_POINT('Ctrl Pts',(-206.225647449683,-1.75427903178613,
135.401144949441));
#241026=CARTESIAN_POINT('Ctrl Pts',(-206.233407892198,-1.6250803440804,
135.446374936564));
#241027=CARTESIAN_POINT('Ctrl Pts',(-206.241180792463,-1.49567425517145,
135.491677530877));
#241028=CARTESIAN_POINT('Ctrl Pts',(-206.248953692729,-1.36450951455032,
135.531516847299));
#241029=CARTESIAN_POINT('Ctrl Pts',(-206.256726592995,-1.23208958293334,
135.565782497858));
#241030=CARTESIAN_POINT('Ctrl Pts',(-206.264216928754,-1.10448344942972,
135.598802505697));
#241031=CARTESIAN_POINT('Ctrl Pts',(-206.271707264513,-0.975712100315515,
135.626646980716));
#241032=CARTESIAN_POINT('Ctrl Pts',(-206.279197600272,-0.846231065683617,
135.649262685304));
#241033=CARTESIAN_POINT('Ctrl Pts',(-206.286971934391,-0.711840718217051,
135.672735871215));
#241034=CARTESIAN_POINT('Ctrl Pts',(-206.29474626851,-0.576260099220195,
135.690650318037));
#241035=CARTESIAN_POINT('Ctrl Pts',(-206.302520602629,-0.439988827093508,
135.702890284163));
#241036=CARTESIAN_POINT('Ctrl Pts',(-206.310285355577,-0.303885497130804,
135.715115165626));
#241037=CARTESIAN_POINT('Ctrl Pts',(-206.318050108524,-0.16709359326881,
135.721679446316));
#241038=CARTESIAN_POINT('Ctrl Pts',(-206.325814861471,-0.030122916862644,
135.722518369446));
#241039=CARTESIAN_POINT('Ctrl Pts',(-206.333571902356,0.106711718336767,
135.723356459347));
#241040=CARTESIAN_POINT('Ctrl Pts',(-206.341328943241,0.243724384301109,
135.718480505712));
#241041=CARTESIAN_POINT('Ctrl Pts',(-206.349085984126,0.380400519141976,
135.707877570482));
#241042=CARTESIAN_POINT('Ctrl Pts',(-206.356837175366,0.516973585446189,
135.697282631009));
#241043=CARTESIAN_POINT('Ctrl Pts',(-206.364588366606,0.653210237545264,
135.68096933629));
#241044=CARTESIAN_POINT('Ctrl Pts',(-206.372339557846,0.78859663427342,
135.658976813612));
#241045=CARTESIAN_POINT('Ctrl Pts',(-206.380087454624,0.9239254881716,135.636993638342));
#241046=CARTESIAN_POINT('Ctrl Pts',(-206.387835351401,1.0584044203597,135.60933609858));
#241047=CARTESIAN_POINT('Ctrl Pts',(-206.395583248178,1.19152564980452,
135.576095070399));
#241048=CARTESIAN_POINT('Ctrl Pts',(-206.403329524262,1.3246190331579,135.542860995525));
#241049=CARTESIAN_POINT('Ctrl Pts',(-206.411075800346,1.45635489958587,
135.504045849998));
#241050=CARTESIAN_POINT('Ctrl Pts',(-206.41882207643,1.58623697799247,135.459791350823));
#241051=CARTESIAN_POINT('Ctrl Pts',(-206.426568409696,1.71612001515889,
135.41553652497));
#241052=CARTESIAN_POINT('Ctrl Pts',(-206.434314742961,1.84414886692504,
135.365842391443));
#241053=CARTESIAN_POINT('Ctrl Pts',(-206.442061076226,1.96984409085683,
135.310900012736));
#241054=CARTESIAN_POINT('Ctrl Pts',(-206.449809144229,2.09556746336268,
135.255945330063));
#241055=CARTESIAN_POINT('Ctrl Pts',(-206.457557212232,2.21895580995249,
135.195740220041));
#241056=CARTESIAN_POINT('Ctrl Pts',(-206.465305280235,2.33955164148073,
135.130523025445));
#241057=CARTESIAN_POINT('Ctrl Pts',(-206.473061582977,2.46027564369365,
135.065236517239));
#241058=CARTESIAN_POINT('Ctrl Pts',(-206.480817885719,2.57820085766173,
134.99492746967));
#241059=CARTESIAN_POINT('Ctrl Pts',(-206.488574188461,2.69289582161183,
134.919879437405));
#241060=CARTESIAN_POINT('Ctrl Pts',(-206.496334630975,2.80765200171758,
134.844791349744));
#241061=CARTESIAN_POINT('Ctrl Pts',(-206.504095073489,2.91917417867433,
134.764959464925));
#241062=CARTESIAN_POINT('Ctrl Pts',(-206.511855516003,3.02706249437732,
134.68070886271));
#241063=CARTESIAN_POINT('Ctrl Pts',(-206.519628416269,3.13512400198284,
134.59632301395));
#241064=CARTESIAN_POINT('Ctrl Pts',(-206.527401316534,3.23953969337777,
134.507504526547));
#241065=CARTESIAN_POINT('Ctrl Pts',(-206.5351742168,3.33994456322253,134.414617308869));
#241066=CARTESIAN_POINT('Ctrl Pts',(-206.542664552561,3.43669946314165,
134.325106775525));
#241067=CARTESIAN_POINT('Ctrl Pts',(-206.550154888323,3.52972986821838,
134.231818411375));
#241068=CARTESIAN_POINT('Ctrl Pts',(-206.557645224085,3.61874476299928,
134.13510669056));
#241069=CARTESIAN_POINT('Ctrl Pts',(-206.565419558204,3.71113468457249,
134.034728115454));
#241070=CARTESIAN_POINT('Ctrl Pts',(-206.573193892323,3.79949125235512,
133.930343496942));
#241071=CARTESIAN_POINT('Ctrl Pts',(-206.580968226442,3.88344703370601,
133.82231061697));
#241072=CARTESIAN_POINT('Ctrl Pts',(-206.588732979389,3.9672993470595,133.714410877866));
#241073=CARTESIAN_POINT('Ctrl Pts',(-206.596497732336,4.04676142767885,
133.602872129055));
#241074=CARTESIAN_POINT('Ctrl Pts',(-206.604262485283,4.12150323375985,
133.488088278229));
#241075=CARTESIAN_POINT('Ctrl Pts',(-206.612019526168,4.19617080522537,
133.373418432341));
#241076=CARTESIAN_POINT('Ctrl Pts',(-206.619776567053,4.2661272200117,133.255510224025));
#241077=CARTESIAN_POINT('Ctrl Pts',(-206.627533607938,4.33108345969385,
133.134789575433));
#241078=CARTESIAN_POINT('Ctrl Pts',(-206.635284799178,4.39599071537045,
133.014159963221));
#241079=CARTESIAN_POINT('Ctrl Pts',(-206.643035990418,4.45590511673205,
132.890722475119));
#241080=CARTESIAN_POINT('Ctrl Pts',(-206.650787181658,4.51058183897033,
132.764930569506));
#241081=CARTESIAN_POINT('Ctrl Pts',(-206.658535078435,4.56523532214318,
132.639192128808));
#241082=CARTESIAN_POINT('Ctrl Pts',(-206.666282975212,4.61465539831717,
132.511101618704));
#241083=CARTESIAN_POINT('Ctrl Pts',(-206.674030871989,4.65864405605593,
132.381135370495));
#241084=CARTESIAN_POINT('Ctrl Pts',(-206.681777148073,4.70262351231578,
132.251196308424));
#241085=CARTESIAN_POINT('Ctrl Pts',(-206.689523424157,4.74117368471374,
132.119382658775));
#241086=CARTESIAN_POINT('Ctrl Pts',(-206.697269700241,4.77414555713005,
131.986188549981));
#241087=CARTESIAN_POINT('Ctrl Pts',(-206.705016033506,4.80711767293719,
131.852993457978));
#241088=CARTESIAN_POINT('Ctrl Pts',(-206.712762366772,4.83451131264874,
131.718418266004));
#241089=CARTESIAN_POINT('Ctrl Pts',(-206.720508700037,4.8562280722051,131.582969616504));
#241090=CARTESIAN_POINT('Ctrl Pts',(-206.72825676804,4.87794969507915,131.447490634218));
#241091=CARTESIAN_POINT('Ctrl Pts',(-206.736004836043,4.89399184618037,
131.311138191135));
#241092=CARTESIAN_POINT('Ctrl Pts',(-206.743752904046,4.90430776597871,
131.174426015923));
#241093=CARTESIAN_POINT('Ctrl Pts',(-206.751509206787,4.91463464965938,
131.037568541384));
#241094=CARTESIAN_POINT('Ctrl Pts',(-206.759265509529,4.91922311531838,
130.900350961453));
#241095=CARTESIAN_POINT('Ctrl Pts',(-206.767021812271,4.91807850989876,
130.763289545363));
#241096=CARTESIAN_POINT('Ctrl Pts',(-206.774782254785,4.91693329356877,
130.626154975468));
#241097=CARTESIAN_POINT('Ctrl Pts',(-206.782542697299,4.91004892864024,
130.489177125775));
#241098=CARTESIAN_POINT('Ctrl Pts',(-206.790303139813,4.89748278085339,
130.352868121787));
#241099=CARTESIAN_POINT('Ctrl Pts',(-206.798076040079,4.88489646077053,
130.216340302485));
#241100=CARTESIAN_POINT('Ctrl Pts',(-206.805848940344,4.86661018354394,
130.080483862156));
#241101=CARTESIAN_POINT('Ctrl Pts',(-206.813621840609,4.84273282128629,
129.945802591492));
#241102=CARTESIAN_POINT('Ctrl Pts',(-206.821112176372,4.81972346128801,
129.816017324245));
#241103=CARTESIAN_POINT('Ctrl Pts',(-206.828602512135,4.79152252480077,
129.687323570165));
#241104=CARTESIAN_POINT('Ctrl Pts',(-206.836092847897,4.75827093999596,
129.560157770724));
#241105=CARTESIAN_POINT('Ctrl Pts',(-206.843867182016,4.72375861124946,
129.428170441356));
#241106=CARTESIAN_POINT('Ctrl Pts',(-206.851641516135,4.68369575848463,
129.29741112245));
#241107=CARTESIAN_POINT('Ctrl Pts',(-206.859415850255,4.63818478746673,
129.168382335371));
#241108=CARTESIAN_POINT('Ctrl Pts',(-206.867180603202,4.59272990465331,
129.039512564742));
#241109=CARTESIAN_POINT('Ctrl Pts',(-206.874945356149,4.54184039188006,
128.912369447615));
#241110=CARTESIAN_POINT('Ctrl Pts',(-206.882710109096,4.4856692591883,128.787443574236));
#241111=CARTESIAN_POINT('Ctrl Pts',(-206.890467149981,4.42955391645741,
128.662641778997));
#241112=CARTESIAN_POINT('Ctrl Pts',(-206.898224190866,4.36816755243845,
128.540053199304));
#241113=CARTESIAN_POINT('Ctrl Pts',(-206.905981231751,4.30171228598306,
128.420151215873));
#241114=CARTESIAN_POINT('Ctrl Pts',(-206.913732422991,4.23530713396096,
128.300339651459));
#241115=CARTESIAN_POINT('Ctrl Pts',(-206.921483614231,4.16384087671486,
128.183210991282));
#241116=CARTESIAN_POINT('Ctrl Pts',(-206.929234805471,4.08756268783238,
128.069216318714));
#241117=CARTESIAN_POINT('Ctrl Pts',(-206.936982702249,4.01131691921485,
127.955270096924));
#241118=CARTESIAN_POINT('Ctrl Pts',(-206.944730599026,3.93026350367536,
127.844455537692));
#241119=CARTESIAN_POINT('Ctrl Pts',(-206.952478495803,3.844696162211,127.737196702354));
#241120=CARTESIAN_POINT('Ctrl Pts',(-206.960224771887,3.75914671958986,
127.629960303251));
#241121=CARTESIAN_POINT('Ctrl Pts',(-206.967971047971,3.66908547280403,
127.526278454052));
#241122=CARTESIAN_POINT('Ctrl Pts',(-206.975717324055,3.5748475992442,127.426543614726));
#241123=CARTESIAN_POINT('Ctrl Pts',(-206.983463657321,3.48060903004192,
127.326808039179));
#241124=CARTESIAN_POINT('Ctrl Pts',(-206.991209990586,3.38219404105675,
127.231019815818));
#241125=CARTESIAN_POINT('Ctrl Pts',(-206.998956323851,3.27997569512705,
127.13953558738));
#241126=CARTESIAN_POINT('Ctrl Pts',(-207.006704391854,3.17773445810738,
127.048030871684));
#241127=CARTESIAN_POINT('Ctrl Pts',(-207.014452459857,3.07168846055954,
126.960832329545));
#241128=CARTESIAN_POINT('Ctrl Pts',(-207.022200527861,2.96224464229277,
126.878256983974));
#241129=CARTESIAN_POINT('Ctrl Pts',(-207.029956830602,2.85268450583369,
126.795593876342));
#241130=CARTESIAN_POINT('Ctrl Pts',(-207.037713133344,2.73971964740063,
126.717564016553));
#241131=CARTESIAN_POINT('Ctrl Pts',(-207.045469436086,2.62378730907338,
126.644441962202));
#241132=CARTESIAN_POINT('Ctrl Pts',(-207.0532298786,2.50779309416619,126.571280880408));
#241133=CARTESIAN_POINT('Ctrl Pts',(-207.060990321115,2.38882858239987,
126.50303301797));
#241134=CARTESIAN_POINT('Ctrl Pts',(-207.068750763629,2.26735564704684,
126.439926927807));
#241135=CARTESIAN_POINT('Ctrl Pts',(-207.076523663894,2.14568771255446,
126.376719534146));
#241136=CARTESIAN_POINT('Ctrl Pts',(-207.08429656416,2.02150366214178,126.318670572596));
#241137=CARTESIAN_POINT('Ctrl Pts',(-207.092069464425,1.89528619722091,
126.265960757139));
#241138=CARTESIAN_POINT('Ctrl Pts',(-207.099559800187,1.77365705507833,
126.215167076244));
#241139=CARTESIAN_POINT('Ctrl Pts',(-207.107050135949,1.65014005997225,
126.16933120521));
#241140=CARTESIAN_POINT('Ctrl Pts',(-207.114540471711,1.52517857759403,
126.12857048445));
#241141=CARTESIAN_POINT('Ctrl Pts',(-207.122366202396,1.39462169226328,
126.08598462003));
#241142=CARTESIAN_POINT('Ctrl Pts',(-207.130191933081,1.26207165493998,
126.048803145944));
#241143=CARTESIAN_POINT('Ctrl Pts',(-207.138017663766,1.12801622149789,
126.017215072825));
#241144=CARTESIAN_POINT('Ctrl Pts',(-207.145843394452,0.993960788056163,
125.985626999705));
#241145=CARTESIAN_POINT('Ctrl Pts',(-207.153669125137,0.858400328457906,
125.959632493955));
#241146=CARTESIAN_POINT('Ctrl Pts',(-207.161494855822,0.721842234581774,
125.939370704845));
#241147=CARTESIAN_POINT('Ctrl Pts',(-205.820054717884,-4.76405452823395,
129.582490119308));
#241148=CARTESIAN_POINT('Ctrl Pts',(-205.827905852165,-4.79858606955834,
129.717128074842));
#241149=CARTESIAN_POINT('Ctrl Pts',(-205.835756986446,-4.82742791349959,
129.853316954026));
#241150=CARTESIAN_POINT('Ctrl Pts',(-205.843608120727,-4.85045202410955,
129.99054354702));
#241151=CARTESIAN_POINT('Ctrl Pts',(-205.851456131429,-4.87346697456125,
130.12771554432));
#241152=CARTESIAN_POINT('Ctrl Pts',(-205.859304142131,-4.8906687356244,
130.265924063211));
#241153=CARTESIAN_POINT('Ctrl Pts',(-205.867152152832,-4.9019802890764,
130.404645333887));
#241154=CARTESIAN_POINT('Ctrl Pts',(-205.87472124722,-4.91288983278145,
130.538436485711));
#241155=CARTESIAN_POINT('Ctrl Pts',(-205.882290341607,-4.91832064309359,
130.672704230441));
#241156=CARTESIAN_POINT('Ctrl Pts',(-205.889859435995,-4.91824930584116,
130.806973679544));
#241157=CARTESIAN_POINT('Origin',(213.235140564004,0.,130.804360617566));
#241158=CARTESIAN_POINT('',(-204.070038127516,-4.76405452823409,129.582490119308));
#241159=CARTESIAN_POINT('',(-204.415385129731,-4.7580624943176,129.583982083009));
#241160=CARTESIAN_POINT('',(213.235140564004,-4.76405452823405,129.582490119308));
#241161=CARTESIAN_POINT('',(-204.485140564013,-4.91500524972814,130.807513005812));
#241162=CARTESIAN_POINT('Ctrl Pts',(-204.415385129731,-4.7580624943176,
129.583982083009));
#241163=CARTESIAN_POINT('Ctrl Pts',(-204.438636941158,-4.85784969763347,
129.983485013898));
#241164=CARTESIAN_POINT('Ctrl Pts',(-204.461888752586,-4.90979750657223,
130.395767923279));
#241165=CARTESIAN_POINT('Ctrl Pts',(-204.485140564013,-4.91220180825584,
130.807511207739));
#241166=CARTESIAN_POINT('Ctrl Pts',(-204.485140564013,-4.91824898839283,
130.807515086282));
#241167=CARTESIAN_POINT('Ctrl Pts',(-204.49387773296,-4.91814963363141,
130.962422774028));
#241168=CARTESIAN_POINT('Ctrl Pts',(-204.502614901907,-4.91072767197462,
131.117052050995));
#241169=CARTESIAN_POINT('Ctrl Pts',(-204.511352070854,-4.8960860736549,
131.27075553806));
#241170=CARTESIAN_POINT('Ctrl Pts',(-204.520123591854,-4.88138690875277,
131.425063343332));
#241171=CARTESIAN_POINT('Ctrl Pts',(-204.528895112854,-4.85941133515114,
131.578437879815));
#241172=CARTESIAN_POINT('Ctrl Pts',(-204.537666633853,-4.83031338638245,
131.73024163143));
#241173=CARTESIAN_POINT('Ctrl Pts',(-204.546486847053,-4.8010539099665,
131.882888071409));
#241174=CARTESIAN_POINT('Ctrl Pts',(-204.555307060253,-4.76459286084652,
132.033946055602));
#241175=CARTESIAN_POINT('Ctrl Pts',(-204.564127273453,-4.72113560423765,
132.182787862255));
#241176=CARTESIAN_POINT('Ctrl Pts',(-204.572392469381,-4.68041292189577,
132.322263707821));
#241177=CARTESIAN_POINT('Ctrl Pts',(-204.580657665308,-4.63354733828304,
132.459793589481));
#241178=CARTESIAN_POINT('Ctrl Pts',(-204.588922861235,-4.58074515708572,
132.594879220747));
#241179=CARTESIAN_POINT('Ctrl Pts',(-204.596697195354,-4.53107884518496,
132.721942250031));
#241180=CARTESIAN_POINT('Ctrl Pts',(-204.604471529473,-4.47604305081149,
132.847138467984));
#241181=CARTESIAN_POINT('Ctrl Pts',(-204.612245863592,-4.41579807394511,
132.969980721057));
#241182=CARTESIAN_POINT('Ctrl Pts',(-204.620010616539,-4.35562734362847,
133.092671582031));
#241183=CARTESIAN_POINT('Ctrl Pts',(-204.627775369486,-4.29026037490912,
133.213013902697));
#241184=CARTESIAN_POINT('Ctrl Pts',(-204.635540122433,-4.21990633574634,
133.330538279574));
#241185=CARTESIAN_POINT('Ctrl Pts',(-204.643297163318,-4.14962217320707,
133.447945929583));
#241186=CARTESIAN_POINT('Ctrl Pts',(-204.651054204203,-4.07436099688629,
133.562540872303));
#241187=CARTESIAN_POINT('Ctrl Pts',(-204.658811245088,-3.99437874200781,
133.673876522365));
#241188=CARTESIAN_POINT('Ctrl Pts',(-204.666562436328,-3.91445680236981,
133.785128213348));
#241189=CARTESIAN_POINT('Ctrl Pts',(-204.674313627568,-3.82982109772313,
133.89312518765));
#241190=CARTESIAN_POINT('Ctrl Pts',(-204.682064818808,-3.74077169726714,
133.997448491619));
#241191=CARTESIAN_POINT('Ctrl Pts',(-204.689812715585,-3.65176014518169,
134.101727455401));
#241192=CARTESIAN_POINT('Ctrl Pts',(-204.697560612362,-3.55833888168141,
134.202335557629));
#241193=CARTESIAN_POINT('Ctrl Pts',(-204.705308509139,-3.46084906882826,
134.298885876495));
#241194=CARTESIAN_POINT('Ctrl Pts',(-204.713054785223,-3.36337964874233,
134.395415999115));
#241195=CARTESIAN_POINT('Ctrl Pts',(-204.720801061307,-3.26184364970766,
134.487889751746));
#241196=CARTESIAN_POINT('Ctrl Pts',(-204.728547337392,-3.15661972277871,
134.575956432107));
#241197=CARTESIAN_POINT('Ctrl Pts',(-204.736293670657,-3.05139501911078,
134.664023762557));
#241198=CARTESIAN_POINT('Ctrl Pts',(-204.744040003922,-2.94248263304068,
134.747683704894));
#241199=CARTESIAN_POINT('Ctrl Pts',(-204.751786337187,-2.83029466646686,
134.826625547114));
#241200=CARTESIAN_POINT('Ctrl Pts',(-204.75953440519,-2.71808157617563,
134.905585067812));
#241201=CARTESIAN_POINT('Ctrl Pts',(-204.767282473193,-2.60259176539364,
134.979824160965));
#241202=CARTESIAN_POINT('Ctrl Pts',(-204.775030541196,-2.48426636236587,
135.04907541403));
#241203=CARTESIAN_POINT('Ctrl Pts',(-204.782786843938,-2.36581520169152,
135.11840026815));
#241204=CARTESIAN_POINT('Ctrl Pts',(-204.79054314668,-2.24452276654071,
135.182726494795));
#241205=CARTESIAN_POINT('Ctrl Pts',(-204.798299449421,-2.12085532938707,
135.241832390356));
#241206=CARTESIAN_POINT('Ctrl Pts',(-204.806059891935,-1.99712188719867,
135.300969832514));
#241207=CARTESIAN_POINT('Ctrl Pts',(-204.81382033445,-1.87101127650509,
135.354881238147));
#241208=CARTESIAN_POINT('Ctrl Pts',(-204.821580776964,-1.74300886894293,
135.403393466469));
#241209=CARTESIAN_POINT('Ctrl Pts',(-204.829353677229,-1.61480098055263,
135.451983570926));
#241210=CARTESIAN_POINT('Ctrl Pts',(-204.837126577494,-1.48469559792147,
135.495157054964));
#241211=CARTESIAN_POINT('Ctrl Pts',(-204.84489947776,-1.35319320086527,
135.532790718946));
#241212=CARTESIAN_POINT('Ctrl Pts',(-204.852389813522,-1.22647124717054,
135.569056304449));
#241213=CARTESIAN_POINT('Ctrl Pts',(-204.859880149284,-1.09845238493452,
135.600177777234));
#241214=CARTESIAN_POINT('Ctrl Pts',(-204.867370485047,-0.969590637356454,
135.626090292532));
#241215=CARTESIAN_POINT('Ctrl Pts',(-204.875144819166,-0.835843057454864,
135.652985288723));
#241216=CARTESIAN_POINT('Ctrl Pts',(-204.882919153285,-0.700763742363002,
135.674353730114));
#241217=CARTESIAN_POINT('Ctrl Pts',(-204.890693487405,-0.564849194214768,
135.690067163225));
#241218=CARTESIAN_POINT('Ctrl Pts',(-204.898458240352,-0.42910214860009,
135.705761230934));
#241219=CARTESIAN_POINT('Ctrl Pts',(-204.906222993299,-0.292522302678767,
135.715814112706));
#241220=CARTESIAN_POINT('Ctrl Pts',(-204.913987746246,-0.155617639284803,
135.720148063423));
#241221=CARTESIAN_POINT('Ctrl Pts',(-204.921744787131,-0.0188489515325352,
135.724477709599));
#241222=CARTESIAN_POINT('Ctrl Pts',(-204.929501828017,0.118243523436565,
135.723099716129));
#241223=CARTESIAN_POINT('Ctrl Pts',(-204.937258868902,0.255145721463766,
135.715988018267));
#241224=CARTESIAN_POINT('Ctrl Pts',(-204.945010060142,0.391944680478308,
135.708881683392));
#241225=CARTESIAN_POINT('Ctrl Pts',(-204.952761251382,0.528553259298798,
135.696050270647));
#241226=CARTESIAN_POINT('Ctrl Pts',(-204.960512442623,0.664456785619391,
135.677519782065));
#241227=CARTESIAN_POINT('Ctrl Pts',(-204.9682603394,0.80030254931577,135.658997169436));
#241228=CARTESIAN_POINT('Ctrl Pts',(-204.976008236177,0.935443469955528,
135.634780351368));
#241229=CARTESIAN_POINT('Ctrl Pts',(-204.983756132954,1.06936961283493,
135.604947216477));
#241230=CARTESIAN_POINT('Ctrl Pts',(-204.991502409038,1.20326774125236,
135.575120322035));
#241231=CARTESIAN_POINT('Ctrl Pts',(-204.999248685123,1.33595121596879,
135.53967953249));
#241232=CARTESIAN_POINT('Ctrl Pts',(-205.006994961207,1.46692031107978,
135.49875385455));
#241233=CARTESIAN_POINT('Ctrl Pts',(-205.014741294472,1.59789037297505,
135.457827874506));
#241234=CARTESIAN_POINT('Ctrl Pts',(-205.022487627738,1.72714565684219,
135.411417041884));
#241235=CARTESIAN_POINT('Ctrl Pts',(-205.030233961003,1.85420200073023,
135.359700122256));
#241236=CARTESIAN_POINT('Ctrl Pts',(-205.037982029006,1.98128679800571,
135.307971620982));
#241237=CARTESIAN_POINT('Ctrl Pts',(-205.04573009701,2.10617131336159,135.250934815567));
#241238=CARTESIAN_POINT('Ctrl Pts',(-205.053478165013,2.22839212445938,
135.188816296684));
#241239=CARTESIAN_POINT('Ctrl Pts',(-205.061234467755,2.35074283328949,
135.1266317575));
#241240=CARTESIAN_POINT('Ctrl Pts',(-205.068990770497,2.47042383351275,
135.059354893381));
#241241=CARTESIAN_POINT('Ctrl Pts',(-205.076747073239,2.58699656794278,
134.987258156348));
#241242=CARTESIAN_POINT('Ctrl Pts',(-205.084507515753,2.70363152075111,
134.915122939117));
#241243=CARTESIAN_POINT('Ctrl Pts',(-205.092267958267,2.81715457866475,
134.838162942302));
#241244=CARTESIAN_POINT('Ctrl Pts',(-205.100028400782,2.9271577182112,134.756692935985));
#241245=CARTESIAN_POINT('Ctrl Pts',(-205.107801301047,3.03733744456286,
134.67509214678));
#241246=CARTESIAN_POINT('Ctrl Pts',(-205.115574201313,3.1439856567345,134.588967126286));
#241247=CARTESIAN_POINT('Ctrl Pts',(-205.123347101578,3.24672818181712,
134.498672349932));
#241248=CARTESIAN_POINT('Ctrl Pts',(-205.130837437339,3.3457357573013,134.411660016153));
#241249=CARTESIAN_POINT('Ctrl Pts',(-205.1383277731,3.4411164558133,134.320776037914));
#241250=CARTESIAN_POINT('Ctrl Pts',(-205.145818108861,3.53257031098373,
134.226367347609));
#241251=CARTESIAN_POINT('Ctrl Pts',(-205.15359244298,3.62749166688566,134.128379123099));
#241252=CARTESIAN_POINT('Ctrl Pts',(-205.161366777099,3.71848321111434,
134.026283234194));
#241253=CARTESIAN_POINT('Ctrl Pts',(-205.169141111218,3.80516850058741,
133.920427969957));
#241254=CARTESIAN_POINT('Ctrl Pts',(-205.176905864165,3.89174695818848,
133.814703162873));
#241255=CARTESIAN_POINT('Ctrl Pts',(-205.184670617112,3.97402947520282,
133.705228498512));
#241256=CARTESIAN_POINT('Ctrl Pts',(-205.192435370059,4.05167606532983,
133.592389334085));
#241257=CARTESIAN_POINT('Ctrl Pts',(-205.200192410944,4.1292455357689,133.479662243106));
#241258=CARTESIAN_POINT('Ctrl Pts',(-205.207949451829,4.2021880222257,133.363577622127));
#241259=CARTESIAN_POINT('Ctrl Pts',(-205.215706492714,4.27020373145505,
133.24455387925));
#241260=CARTESIAN_POINT('Ctrl Pts',(-205.223457683954,4.33816814950907,
133.125619893103));
#241261=CARTESIAN_POINT('Ctrl Pts',(-205.231208875195,4.40121299226405,
133.003751534774));
#241262=CARTESIAN_POINT('Ctrl Pts',(-205.238960066435,4.45908194301358,
132.879395867385));
#241263=CARTESIAN_POINT('Ctrl Pts',(-205.246707963212,4.51692629791526,
132.755093054471));
#241264=CARTESIAN_POINT('Ctrl Pts',(-205.254455859989,4.56959897162442,
132.628305388855));
#241265=CARTESIAN_POINT('Ctrl Pts',(-205.262203756766,4.61688986187661,
132.499503993744));
#241266=CARTESIAN_POINT('Ctrl Pts',(-205.26995003285,4.66417085989403,132.370729541109));
#241267=CARTESIAN_POINT('Ctrl Pts',(-205.277696308934,4.70607217897284,
132.239942563603));
#241268=CARTESIAN_POINT('Ctrl Pts',(-205.285442585018,4.74243224205182,
132.107633226059));
#241269=CARTESIAN_POINT('Ctrl Pts',(-205.293188918284,4.77879257353258,
131.975322911837));
#241270=CARTESIAN_POINT('Ctrl Pts',(-205.300935251549,4.80961146379121,
131.841490592143));
#241271=CARTESIAN_POINT('Ctrl Pts',(-205.308681584814,4.83477761200457,
131.706640233295));
#241272=CARTESIAN_POINT('Ctrl Pts',(-205.316429652817,4.8599493960023,131.571759675644));
#241273=CARTESIAN_POINT('Ctrl Pts',(-205.32417772082,4.8794658472645,131.435861009436));
#241274=CARTESIAN_POINT('Ctrl Pts',(-205.331925788823,4.89326711184883,
131.299456602804));
#241275=CARTESIAN_POINT('Ctrl Pts',(-205.339682091565,4.90708304458142,
131.162907223945));
#241276=CARTESIAN_POINT('Ctrl Pts',(-205.347438394307,4.91517161741112,
131.025851420532));
#241277=CARTESIAN_POINT('Ctrl Pts',(-205.355194697049,4.91752500106838,
130.888805430121));
#241278=CARTESIAN_POINT('Ctrl Pts',(-205.362955139563,4.91987964079736,
130.751686294138));
#241279=CARTESIAN_POINT('Ctrl Pts',(-205.370715582077,4.91649300161557,
130.614577372247));
#241280=CARTESIAN_POINT('Ctrl Pts',(-205.378476024592,4.9074093618528,130.477992087068));
#241281=CARTESIAN_POINT('Ctrl Pts',(-205.386248924857,4.89831114022507,
130.341187543064));
#241282=CARTESIAN_POINT('Ctrl Pts',(-205.394021825122,4.88349768500393,
130.204908704434));
#241283=CARTESIAN_POINT('Ctrl Pts',(-205.401794725388,4.86306497681123,
130.069661976073));
#241284=CARTESIAN_POINT('Ctrl Pts',(-205.40928506115,4.84337504902889,129.939331806958));
#241285=CARTESIAN_POINT('Ctrl Pts',(-205.416775396912,4.81846738151463,
129.809960313757));
#241286=CARTESIAN_POINT('Ctrl Pts',(-205.424265732673,4.78847171916799,
129.681987392107));
#241287=CARTESIAN_POINT('Ctrl Pts',(-205.432040066792,4.75733876216599,
129.549162338233));
#241288=CARTESIAN_POINT('Ctrl Pts',(-205.439814400911,4.72062575157316,
129.417423253277));
#241289=CARTESIAN_POINT('Ctrl Pts',(-205.44758873503,4.67842223616104,129.287275108211));
#241290=CARTESIAN_POINT('Ctrl Pts',(-205.455353487977,4.63627073280972,
129.157287359103));
#241291=CARTESIAN_POINT('Ctrl Pts',(-205.463118240924,4.58864230750925,
129.028887017024));
#241292=CARTESIAN_POINT('Ctrl Pts',(-205.470882993871,4.53567740129338,
128.902568417062));
#241293=CARTESIAN_POINT('Ctrl Pts',(-205.478640034756,4.48276510056905,
128.776375278515));
#241294=CARTESIAN_POINT('Ctrl Pts',(-205.486397075641,4.4245270169024,128.652260125658));
#241295=CARTESIAN_POINT('Ctrl Pts',(-205.494154116526,4.36115312330836,
128.530701342838));
#241296=CARTESIAN_POINT('Ctrl Pts',(-205.501905307766,4.29782702046055,
128.409234228441));
#241297=CARTESIAN_POINT('Ctrl Pts',(-205.509656499006,4.22937299657398,
128.290319992233));
#241298=CARTESIAN_POINT('Ctrl Pts',(-205.517407690246,4.15602863307309,
128.174415929255));
#241299=CARTESIAN_POINT('Ctrl Pts',(-205.525155587023,4.08271544288332,
128.058561128595));
#241300=CARTESIAN_POINT('Ctrl Pts',(-205.5329034838,4.00451625573041,127.94571428621));
#241301=CARTESIAN_POINT('Ctrl Pts',(-205.540651380577,3.92171387550616,
127.836306820688));
#241302=CARTESIAN_POINT('Ctrl Pts',(-205.548397656661,3.83892881575483,
127.726922240849));
#241303=CARTESIAN_POINT('Ctrl Pts',(-205.556143932745,3.75154271395995,
127.62097591841));
#241304=CARTESIAN_POINT('Ctrl Pts',(-205.563890208829,3.65988062332928,
127.518868738794));
#241305=CARTESIAN_POINT('Ctrl Pts',(-205.571636542094,3.56821785606976,
127.416760805445));
#241306=CARTESIAN_POINT('Ctrl Pts',(-205.579382875359,3.47227929816279,
127.318492362404));
#241307=CARTESIAN_POINT('Ctrl Pts',(-205.587129208625,3.37242878993213,
127.224429456309));
#241308=CARTESIAN_POINT('Ctrl Pts',(-205.594877276628,3.27255592087287,
127.130345485479));
#241309=CARTESIAN_POINT('Ctrl Pts',(-205.60262534463,3.16876964276772,127.040469193703));
#241310=CARTESIAN_POINT('Ctrl Pts',(-205.610373412633,3.06146867291942,
126.955127885289));
#241311=CARTESIAN_POINT('Ctrl Pts',(-205.618129715375,2.95405366232302,
126.869695875116));
#241312=CARTESIAN_POINT('Ctrl Pts',(-205.625886018117,2.84311680448129,
126.788808720195));
#241313=CARTESIAN_POINT('Ctrl Pts',(-205.633642320859,2.72908819275771,
126.712752046521));
#241314=CARTESIAN_POINT('Ctrl Pts',(-205.641402763373,2.61499872053071,
126.63665477911));
#241315=CARTESIAN_POINT('Ctrl Pts',(-205.649163205887,2.4978145402187,126.565393333214));
#241316=CARTESIAN_POINT('Ctrl Pts',(-205.656923648401,2.37799154233177,
126.499207973687));
#241317=CARTESIAN_POINT('Ctrl Pts',(-205.664696548666,2.25797619393123,
126.432916367546));
#241318=CARTESIAN_POINT('Ctrl Pts',(-205.672469448932,2.13531391299143,
126.371717305886));
#241319=CARTESIAN_POINT('Ctrl Pts',(-205.680242349197,2.01048263216247,
126.315803761708));
#241320=CARTESIAN_POINT('Ctrl Pts',(-205.68773268496,1.89018928280237,126.261922815689));
#241321=CARTESIAN_POINT('Ctrl Pts',(-205.695223020723,1.76788217886368,
126.212949889631));
#241322=CARTESIAN_POINT('Ctrl Pts',(-205.702713356486,1.64400154729095,
126.169013599812));
#241323=CARTESIAN_POINT('Ctrl Pts',(-205.710487690606,1.5154239439371,126.123411452216));
#241324=CARTESIAN_POINT('Ctrl Pts',(-205.718262024725,1.38474384172379,
126.083090954468));
#241325=CARTESIAN_POINT('Ctrl Pts',(-205.726036358844,1.25243449033019,
126.048249715796));
#241326=CARTESIAN_POINT('Ctrl Pts',(-205.733801111791,1.12028819838735,
126.013451415837));
#241327=CARTESIAN_POINT('Ctrl Pts',(-205.741565864738,0.986517026841535,
125.984119037703));
#241328=CARTESIAN_POINT('Ctrl Pts',(-205.749330617686,0.85161278561181,
125.960401624564));
#241329=CARTESIAN_POINT('Ctrl Pts',(-205.757087658571,0.716842533176288,
125.936707767895));
#241330=CARTESIAN_POINT('Ctrl Pts',(-205.764844699456,0.5809418331833,125.918617845271));
#241331=CARTESIAN_POINT('Ctrl Pts',(-205.772601740341,0.444415848987914,
125.906230605442));
#241332=CARTESIAN_POINT('Ctrl Pts',(-205.780352931581,0.307992820099411,
125.893852706927));
#241333=CARTESIAN_POINT('Ctrl Pts',(-205.788104122822,0.170945833354071,
125.88716896663));
#241334=CARTESIAN_POINT('Ctrl Pts',(-205.795855314062,0.0337880425846281,
125.886226679711));
#241335=CARTESIAN_POINT('Ctrl Pts',(-205.803603210839,-0.103311452464748,
125.885284793289));
#241336=CARTESIAN_POINT('Ctrl Pts',(-205.811351107616,-0.240521267733049,
125.890079509413));
#241337=CARTESIAN_POINT('Ctrl Pts',(-205.819099004394,-0.377325576133052,
125.900606089442));
#241338=CARTESIAN_POINT('Ctrl Pts',(-205.826845280478,-0.514101268020897,
125.911130467538));
#241339=CARTESIAN_POINT('Ctrl Pts',(-205.834591556562,-0.650471232192675,
125.927384294722));
#241340=CARTESIAN_POINT('Ctrl Pts',(-205.842337832646,-0.785922493189801,
125.949310782889));
#241341=CARTESIAN_POINT('Ctrl Pts',(-205.850084165912,-0.921374754057551,
125.971237432912));
#241342=CARTESIAN_POINT('Ctrl Pts',(-205.857830499177,-1.05590791227709,
125.998836764999));
#241343=CARTESIAN_POINT('Ctrl Pts',(-205.865576832443,-1.18901733786065,
126.032000527132));
#241344=CARTESIAN_POINT('Ctrl Pts',(-205.873324900446,-1.32215657237697,
126.065171716059));
#241345=CARTESIAN_POINT('Ctrl Pts',(-205.881072968449,-1.45387106051707,
126.103909720158));
#241346=CARTESIAN_POINT('Ctrl Pts',(-205.888821036452,-1.58366991545586,
126.148056003241));
#241347=CARTESIAN_POINT('Ctrl Pts',(-205.896577339194,-1.71360672216248,
126.19224920552));
#241348=CARTESIAN_POINT('Ctrl Pts',(-205.904333641936,-1.8416234578902,
126.241862042909));
#241349=CARTESIAN_POINT('Ctrl Pts',(-205.912089944678,-1.96724734143226,
126.296687053506));
#241350=CARTESIAN_POINT('Ctrl Pts',(-205.919850387192,-2.09293827422343,
126.351541325862));
#241351=CARTESIAN_POINT('Ctrl Pts',(-205.927610829707,-2.21623345872856,
126.411613143427));
#241352=CARTESIAN_POINT('Ctrl Pts',(-205.935371272221,-2.33668433336452,
126.476648821627));
#241353=CARTESIAN_POINT('Ctrl Pts',(-205.943144172487,-2.45732856643756,
126.541788900871));
#241354=CARTESIAN_POINT('Ctrl Pts',(-205.950917072752,-2.57511902930189,
126.61190856411));
#241355=CARTESIAN_POINT('Ctrl Pts',(-205.958689973018,-2.68963503403625,
126.68671001969));
#241356=CARTESIAN_POINT('Ctrl Pts',(-205.966180308779,-2.79998809352685,
126.758792253932));
#241357=CARTESIAN_POINT('Ctrl Pts',(-205.973670644539,-2.90730038036246,
126.835221621603));
#241358=CARTESIAN_POINT('Ctrl Pts',(-205.9811609803,-3.0112257326097,126.915697267549));
#241359=CARTESIAN_POINT('Ctrl Pts',(-205.988843416406,-3.11781639876974,
126.998236826237));
#241360=CARTESIAN_POINT('Ctrl Pts',(-205.996525852513,-3.22119867281582,
127.085307874707));
#241361=CARTESIAN_POINT('Ctrl Pts',(-206.004208288619,-3.32095599792357,
127.1766293262));
#241362=CARTESIAN_POINT('Ctrl Pts',(-206.01188194727,-3.42059934675241,
127.267846439699));
#241363=CARTESIAN_POINT('Ctrl Pts',(-206.019555605921,-3.5166256876976,
127.363304034671));
#241364=CARTESIAN_POINT('Ctrl Pts',(-206.027229264572,-3.60864870074115,
127.462678762999));
#241365=CARTESIAN_POINT('Ctrl Pts',(-206.034895912193,-3.70058763704767,
127.561962697703));
#241366=CARTESIAN_POINT('Ctrl Pts',(-206.042562559813,-3.78853024788272,
127.665156357538));
#241367=CARTESIAN_POINT('Ctrl Pts',(-206.050229207433,-3.87212489877666,
127.771897620137));
#241368=CARTESIAN_POINT('Ctrl Pts',(-206.057890604246,-3.95566229656263,
127.878565776755));
#241369=CARTESIAN_POINT('Ctrl Pts',(-206.065552001059,-4.03485741114901,
127.988776389217));
#241370=CARTESIAN_POINT('Ctrl Pts',(-206.073213397872,-4.10939732791692,
128.102132525082));
#241371=CARTESIAN_POINT('Ctrl Pts',(-206.080872341447,-4.18391337642932,
128.215452363439));
#241372=CARTESIAN_POINT('Ctrl Pts',(-206.088531285021,-4.25377696648902,
128.331915391257));
#241373=CARTESIAN_POINT('Ctrl Pts',(-206.096190228596,-4.31871736387104,
128.451094080707));
#241374=CARTESIAN_POINT('Ctrl Pts',(-206.103847441602,-4.38364308771443,
128.570245841263));
#241375=CARTESIAN_POINT('Ctrl Pts',(-206.111504654608,-4.44364764309317,
128.692111689209));
#241376=CARTESIAN_POINT('Ctrl Pts',(-206.119161867614,-4.49850566380742,
128.816238424341));
#241377=CARTESIAN_POINT('Ctrl Pts',(-206.1268221242,-4.55338548942266,128.940414497221));
#241378=CARTESIAN_POINT('Ctrl Pts',(-206.134482380787,-4.60311452764392,
129.066852887145));
#241379=CARTESIAN_POINT('Ctrl Pts',(-206.142142637373,-4.64751508729958,
129.195079232654));
#241380=CARTESIAN_POINT('Ctrl Pts',(-206.14976124855,-4.69167426085744,
129.322608468546));
#241381=CARTESIAN_POINT('Ctrl Pts',(-206.157379859728,-4.73056267205465,
129.451905880375));
#241382=CARTESIAN_POINT('Ctrl Pts',(-206.164998470905,-4.76405452823394,
129.582490119308));
#241383=CARTESIAN_POINT('',(-204.139859435948,-4.91824831916273,130.80029447038));
#241384=CARTESIAN_POINT('Ctrl Pts',(-204.139859435995,-4.91824831916343,
130.800294471219));
#241385=CARTESIAN_POINT('Ctrl Pts',(-204.147784635894,-4.91836431326766,
130.94059630973));
#241386=CARTESIAN_POINT('Ctrl Pts',(-204.155709835794,-4.91247201397862,
131.080987232013));
#241387=CARTESIAN_POINT('Ctrl Pts',(-204.163635035693,-4.900578301156,131.220912387145));
#241388=CARTESIAN_POINT('Ctrl Pts',(-204.171354581511,-4.88899322289429,
131.357206570228));
#241389=CARTESIAN_POINT('Ctrl Pts',(-204.179074127329,-4.87171440627009,
131.493058448163));
#241390=CARTESIAN_POINT('Ctrl Pts',(-204.186793673146,-4.84880093828704,
131.627957924122));
#241391=CARTESIAN_POINT('Ctrl Pts',(-204.194513059106,-4.8258879448005,
131.762854606557));
#241392=CARTESIAN_POINT('Ctrl Pts',(-204.202232445066,-4.79734059760185,
131.896798538118));
#241393=CARTESIAN_POINT('Ctrl Pts',(-204.209951831025,-4.76326941003805,
132.029288203138));
#241394=CARTESIAN_POINT('Ctrl Pts',(-204.217672755543,-4.72919143171145,
132.161804274807));
#241395=CARTESIAN_POINT('Ctrl Pts',(-204.225393680062,-4.68958752045796,
132.29286512203));
#241396=CARTESIAN_POINT('Ctrl Pts',(-204.23311460458,-4.6446184041067,132.421983238183));
#241397=CARTESIAN_POINT('Ctrl Pts',(-204.24119374033,-4.59756295178294,
132.55709177159));
#241398=CARTESIAN_POINT('Ctrl Pts',(-204.24927287608,-4.54463267751754,
132.69007253139));
#241399=CARTESIAN_POINT('Ctrl Pts',(-204.25735201183,-4.48606813212016,
132.820390323814));
#241400=CARTESIAN_POINT('Ctrl Pts',(-204.265085528802,-4.43000892977471,
132.945133228333));
#241401=CARTESIAN_POINT('Ctrl Pts',(-204.272819045774,-4.36878776769414,
133.067435961724));
#241402=CARTESIAN_POINT('Ctrl Pts',(-204.280552562746,-4.30266231755848,
133.186855117783));
#241403=CARTESIAN_POINT('Ctrl Pts',(-204.288291669847,-4.23648906901836,
133.306360595297));
#241404=CARTESIAN_POINT('Ctrl Pts',(-204.296030776948,-4.16540467691822,
133.422978009958));
#241405=CARTESIAN_POINT('Ctrl Pts',(-204.303769884048,-4.08970977527734,
133.53629345285));
#241406=CARTESIAN_POINT('Ctrl Pts',(-204.311519964139,-4.01390754867324,
133.649769561459));
#241407=CARTESIAN_POINT('Ctrl Pts',(-204.319270044229,-3.93348199885383,
133.759934040129));
#241408=CARTESIAN_POINT('Ctrl Pts',(-204.32702012432,-3.84877374515481,
133.866406293435));
#241409=CARTESIAN_POINT('Ctrl Pts',(-204.328034827407,-3.83768305634567,
133.880346500872));
#241410=CARTESIAN_POINT('Ctrl Pts',(-204.329049530494,-3.82651900354742,
133.894223468265));
#241411=CARTESIAN_POINT('Ctrl Pts',(-204.330064233581,-3.81528239632779,
133.908036389739));
#241412=CARTESIAN_POINT('Ctrl Pts',(-204.3378385677,-3.72919106576708,134.013866625264));
#241413=CARTESIAN_POINT('Ctrl Pts',(-204.345612901819,-3.63855667661419,
134.116279706243));
#241414=CARTESIAN_POINT('Ctrl Pts',(-204.353387235938,-3.54368061892281,
134.21486068846));
#241415=CARTESIAN_POINT('Ctrl Pts',(-204.361151988886,-3.44892148749296,
134.313320178428));
#241416=CARTESIAN_POINT('Ctrl Pts',(-204.368916741833,-3.3499313571539,
134.407956687445));
#241417=CARTESIAN_POINT('Ctrl Pts',(-204.37668149478,-3.24705273251776,
134.498387094833));
#241418=CARTESIAN_POINT('Ctrl Pts',(-204.384438535665,-3.14427628838194,
134.588727685466));
#241419=CARTESIAN_POINT('Ctrl Pts',(-204.39219557655,-3.03761932746507,
134.674870231555));
#241420=CARTESIAN_POINT('Ctrl Pts',(-204.399952617435,-2.92746192108998,
134.756467620554));
#241421=CARTESIAN_POINT('Ctrl Pts',(-204.407703808675,-2.81738758527178,
134.838003476328));
#241422=CARTESIAN_POINT('Ctrl Pts',(-204.415454999916,-2.70381837107695,
134.915000765548));
#241423=CARTESIAN_POINT('Ctrl Pts',(-204.423206191156,-2.58716793923965,
134.987152163492));
#241424=CARTESIAN_POINT('Ctrl Pts',(-204.430954087933,-2.47056708694779,
135.059272895167));
#241425=CARTESIAN_POINT('Ctrl Pts',(-204.43870198471,-2.35088795351289,
135.126551626789));
#241426=CARTESIAN_POINT('Ctrl Pts',(-204.446449881487,-2.22857354968108,
135.188724082901));
#241427=CARTESIAN_POINT('Ctrl Pts',(-204.454196157571,-2.1062847313861,
135.250883533874));
#241428=CARTESIAN_POINT('Ctrl Pts',(-204.461942433656,-1.98136208744859,
135.307938656849));
#241429=CARTESIAN_POINT('Ctrl Pts',(-204.46968870974,-1.85427326821161,
135.359671112943));
#241430=CARTESIAN_POINT('Ctrl Pts',(-204.477435043005,-1.72718351083332,
135.411403950916));
#241431=CARTESIAN_POINT('Ctrl Pts',(-204.485181376271,-1.59792790836239,
135.457813896205));
#241432=CARTESIAN_POINT('Ctrl Pts',(-204.492927709536,-1.46699375409005,
135.498730904192));
#241433=CARTESIAN_POINT('Ctrl Pts',(-204.500675777539,-1.33603027802187,
135.53965707526));
#241434=CARTESIAN_POINT('Ctrl Pts',(-204.508423845542,-1.20338787525171,
135.575087744666));
#241435=CARTESIAN_POINT('Ctrl Pts',(-204.516171913545,-1.06956825840305,
135.604902962251));
#241436=CARTESIAN_POINT('Ctrl Pts',(-204.523928216287,-0.935606416472946,
135.634749867804));
#241437=CARTESIAN_POINT('Ctrl Pts',(-204.531684519029,-0.800465243359993,
135.658969314318));
#241438=CARTESIAN_POINT('Ctrl Pts',(-204.539440821771,-0.664656438594865,
135.677492555153));
#241439=CARTESIAN_POINT('Ctrl Pts',(-204.547201264285,-0.528775148581879,
135.696025682401));
#241440=CARTESIAN_POINT('Ctrl Pts',(-204.5549617068,-0.392225905948943,
135.708856509484));
#241441=CARTESIAN_POINT('Ctrl Pts',(-204.562722149314,-0.255523769358385,
135.715968365116));
#241442=CARTESIAN_POINT('Ctrl Pts',(-204.570495049579,-0.118602186361955,
135.72309163733));
#241443=CARTESIAN_POINT('Ctrl Pts',(-204.578267949845,0.0184723898871198,
135.724477588372));
#241444=CARTESIAN_POINT('Ctrl Pts',(-204.58604085011,0.155185762840657,
135.720161716218));
#241445=CARTESIAN_POINT('Ctrl Pts',(-204.593531185872,0.286929260314916,
135.716002736889));
#241446=CARTESIAN_POINT('Ctrl Pts',(-204.601021521633,0.418337052633677,
135.70654931052));
#241447=CARTESIAN_POINT('Ctrl Pts',(-204.608511857394,0.548956999130425,
135.691878318363));
#241448=CARTESIAN_POINT('Ctrl Pts',(-204.616286191514,0.684529440611316,
135.676651071078));
#241449=CARTESIAN_POINT('Ctrl Pts',(-204.624060525633,0.819682567332442,
135.655754564432));
#241450=CARTESIAN_POINT('Ctrl Pts',(-204.631834859752,0.953904366288411,
135.62921807893));
#241451=CARTESIAN_POINT('Ctrl Pts',(-204.639599612699,1.08796074887291,
135.602714297274));
#241452=CARTESIAN_POINT('Ctrl Pts',(-204.647364365646,1.22108770756962,
135.570584441822));
#241453=CARTESIAN_POINT('Ctrl Pts',(-204.655129118593,1.35277777999265,
135.532909585321));
#241454=CARTESIAN_POINT('Ctrl Pts',(-204.662886159478,1.48433705597924,
135.495272148018));
#241455=CARTESIAN_POINT('Ctrl Pts',(-204.670643200363,1.6144619123036,135.452100776427));
#241456=CARTESIAN_POINT('Ctrl Pts',(-204.678400241248,1.74265487551586,
135.403527612506));
#241457=CARTESIAN_POINT('Ctrl Pts',(-204.686151432488,1.8707511674172,135.354991077985));
#241458=CARTESIAN_POINT('Ctrl Pts',(-204.693902623728,1.99691810186812,
135.301060997223));
#241459=CARTESIAN_POINT('Ctrl Pts',(-204.701653814969,2.12067352414457,
135.241919278191));
#241460=CARTESIAN_POINT('Ctrl Pts',(-204.709401711746,2.24437634706579,
135.182802695968));
#241461=CARTESIAN_POINT('Ctrl Pts',(-204.717149608523,2.36566934435866,
135.118479049337));
#241462=CARTESIAN_POINT('Ctrl Pts',(-204.7248975053,2.48409071546674,135.049178208445));
#241463=CARTESIAN_POINT('Ctrl Pts',(-204.732643781384,2.60248731537686,
134.979891863794));
#241464=CARTESIAN_POINT('Ctrl Pts',(-204.740390057468,2.71801314667377,
134.905630593073));
#241465=CARTESIAN_POINT('Ctrl Pts',(-204.748136333552,2.83023173824012,
134.826669826262));
#241466=CARTESIAN_POINT('Ctrl Pts',(-204.755882666818,2.94245115817848,
134.74770847658));
#241467=CARTESIAN_POINT('Ctrl Pts',(-204.763629000083,3.05136296992693,
134.664047786568));
#241468=CARTESIAN_POINT('Ctrl Pts',(-204.771375333349,3.15656071620505,
134.576005816602));
#241469=CARTESIAN_POINT('Ctrl Pts',(-204.779123401352,3.26178202078891,
134.487944130248));
#241470=CARTESIAN_POINT('Ctrl Pts',(-204.786871469354,3.36328730507665,
134.395499462426));
#241471=CARTESIAN_POINT('Ctrl Pts',(-204.794619537357,3.46070446367402,
134.299029082186));
#241472=CARTESIAN_POINT('Ctrl Pts',(-204.802375840099,3.55822515838696,
134.202456172077));
#241473=CARTESIAN_POINT('Ctrl Pts',(-204.810132142841,3.65164876974275,
134.101849278174));
#241474=CARTESIAN_POINT('Ctrl Pts',(-204.817888445583,3.74064087315327,
133.997601748548));
#241475=CARTESIAN_POINT('Ctrl Pts',(-204.825648888097,3.82968047432912,
133.893298578876));
#241476=CARTESIAN_POINT('Ctrl Pts',(-204.833409330612,3.91428361358645,
133.785351209223));
#241477=CARTESIAN_POINT('Ctrl Pts',(-204.841169773126,3.99415786311061,
133.67418396179));
#241478=CARTESIAN_POINT('Ctrl Pts',(-204.848942673391,4.07416033387079,
133.562838258822));
#241479=CARTESIAN_POINT('Ctrl Pts',(-204.856715573657,4.14941853042956,
133.448262676063));
#241480=CARTESIAN_POINT('Ctrl Pts',(-204.864488473922,4.21968438244643,
133.330909009154));
#241481=CARTESIAN_POINT('Ctrl Pts',(-204.871978809684,4.28739589375082,
133.217821443638));
#241482=CARTESIAN_POINT('Ctrl Pts',(-204.879469145446,4.35047157997676,
133.102154538428));
#241483=CARTESIAN_POINT('Ctrl Pts',(-204.886959481207,4.40873173042483,
132.984330248466));
#241484=CARTESIAN_POINT('Ctrl Pts',(-204.894733815326,4.4692008321869,132.862038614734));
#241485=CARTESIAN_POINT('Ctrl Pts',(-204.902508149446,4.52467357561692,
132.737035389221));
#241486=CARTESIAN_POINT('Ctrl Pts',(-204.910282483565,4.57489783969652,
132.609767169797));
#241487=CARTESIAN_POINT('Ctrl Pts',(-204.918047236512,4.62506020685945,
132.48265579708));
#241488=CARTESIAN_POINT('Ctrl Pts',(-204.925811989459,4.66998682248568,
132.35328534469));
#241489=CARTESIAN_POINT('Ctrl Pts',(-204.933576742406,4.70947159955726,
132.222126576906));
#241490=CARTESIAN_POINT('Ctrl Pts',(-204.941333783291,4.74891715979151,
132.091098077859));
#241491=CARTESIAN_POINT('Ctrl Pts',(-204.949090824176,4.78293152551465,
131.958285170043));
#241492=CARTESIAN_POINT('Ctrl Pts',(-204.956847865061,4.81135697494726,
131.824177817914));
#241493=CARTESIAN_POINT('Ctrl Pts',(-204.964599056301,4.8397609885273,131.690171597184));
#241494=CARTESIAN_POINT('Ctrl Pts',(-204.972350247541,4.86258439407255,
131.55487325603));
#241495=CARTESIAN_POINT('Ctrl Pts',(-204.980101438781,4.87971961950594,
131.418786770581));
#241496=CARTESIAN_POINT('Ctrl Pts',(-204.987849335558,4.89684756201144,
131.282758125518));
#241497=CARTESIAN_POINT('Ctrl Pts',(-204.995597232335,4.90829208414323,
131.145942389504));
#241498=CARTESIAN_POINT('Ctrl Pts',(-205.003345129112,4.91399696768572,
131.008852338855));
#241499=CARTESIAN_POINT('Ctrl Pts',(-205.011091405196,4.91970065788955,
130.871790964489));
#241500=CARTESIAN_POINT('Ctrl Pts',(-205.01883768128,4.91966708133521,130.734455780001));
#241501=CARTESIAN_POINT('Ctrl Pts',(-205.026583957365,4.91389204176511,
130.597362877536));
#241502=CARTESIAN_POINT('Ctrl Pts',(-205.03433029063,4.90811695956499,130.460268963083));
#241503=CARTESIAN_POINT('Ctrl Pts',(-205.042076623895,4.89660034623337,
130.323417724839));
#241504=CARTESIAN_POINT('Ctrl Pts',(-205.04982295716,4.87939009488483,130.18732304623));
#241505=CARTESIAN_POINT('Ctrl Pts',(-205.057571025163,4.86217598941975,
130.051197890161));
#241506=CARTESIAN_POINT('Ctrl Pts',(-205.065319093166,4.83926575777492,
129.915830018667));
#241507=CARTESIAN_POINT('Ctrl Pts',(-205.073067161169,4.81075884846427,
129.781725607202));
#241508=CARTESIAN_POINT('Ctrl Pts',(-205.080823463911,4.78222164167122,
129.647478667972));
#241509=CARTESIAN_POINT('Ctrl Pts',(-205.088579766653,4.74807595643261,
129.514498254231));
#241510=CARTESIAN_POINT('Ctrl Pts',(-205.096336069395,4.70847196296183,
129.383278341094));
#241511=CARTESIAN_POINT('Ctrl Pts',(-205.104096511909,4.66884683164728,
129.251988391939));
#241512=CARTESIAN_POINT('Ctrl Pts',(-205.111856954423,4.62375771564571,
129.122461184739));
#241513=CARTESIAN_POINT('Ctrl Pts',(-205.119617396937,4.5734035448659,128.99517210381));
#241514=CARTESIAN_POINT('Ctrl Pts',(-205.127390297203,4.52296854110091,
128.867678687148));
#241515=CARTESIAN_POINT('Ctrl Pts',(-205.135163197468,4.46725175190091,
128.742430933815));
#241516=CARTESIAN_POINT('Ctrl Pts',(-205.142936097734,4.40649919765708,
128.619881758994));
#241517=CARTESIAN_POINT('Ctrl Pts',(-205.150426433496,4.34795515178448,
128.501787555357));
#241518=CARTESIAN_POINT('Ctrl Pts',(-205.157916769258,4.28473525768429,
128.386199406543));
#241519=CARTESIAN_POINT('Ctrl Pts',(-205.16540710502,4.21709737997774,128.273496585208));
#241520=CARTESIAN_POINT('Ctrl Pts',(-205.17318143914,4.14689499158213,128.15652060215));
#241521=CARTESIAN_POINT('Ctrl Pts',(-205.180955773259,4.0717106105036,128.042282515269));
#241522=CARTESIAN_POINT('Ctrl Pts',(-205.188730107378,3.9917836946099,127.931235838176));
#241523=CARTESIAN_POINT('Ctrl Pts',(-205.196494860325,3.91195528149677,
127.820326016188));
#241524=CARTESIAN_POINT('Ctrl Pts',(-205.204259613272,3.82739618907955,
127.712600092508));
#241525=CARTESIAN_POINT('Ctrl Pts',(-205.212024366219,3.73839108960982,
127.608485913572));
#241526=CARTESIAN_POINT('Ctrl Pts',(-205.219781407104,3.64947439125963,
127.504475142307));
#241527=CARTESIAN_POINT('Ctrl Pts',(-205.227538447989,3.55612072597651,
127.404069272277));
#241528=CARTESIAN_POINT('Ctrl Pts',(-205.235295488874,3.45865706226162,
127.307665837039));
#241529=CARTESIAN_POINT('Ctrl Pts',(-205.243046680114,3.36126689665303,
127.21133510038));
#241530=CARTESIAN_POINT('Ctrl Pts',(-205.250797871354,3.2597731785813,127.119001064663));
#241531=CARTESIAN_POINT('Ctrl Pts',(-205.258549062594,3.15454177209991,
127.031026644728));
#241532=CARTESIAN_POINT('Ctrl Pts',(-205.266296959371,3.04935509177414,
126.943089616268));
#241533=CARTESIAN_POINT('Ctrl Pts',(-205.274044856149,2.94043418200212,
126.859508768447));
#241534=CARTESIAN_POINT('Ctrl Pts',(-205.281792752926,2.82818006870287,
126.780608567366));
#241535=CARTESIAN_POINT('Ctrl Pts',(-205.28953902901,2.71594943654389,126.701724870505));
#241536=CARTESIAN_POINT('Ctrl Pts',(-205.297285305094,2.60038730735141,
126.627520097597));
#241537=CARTESIAN_POINT('Ctrl Pts',(-205.305031581178,2.48192561588327,
126.558276739482));
#241538=CARTESIAN_POINT('Ctrl Pts',(-205.312777914443,2.36346304995832,
126.489032870229));
#241539=CARTESIAN_POINT('Ctrl Pts',(-205.320524247709,2.24210121658067,
126.424750686145));
#241540=CARTESIAN_POINT('Ctrl Pts',(-205.328270580974,2.11829834782731,
126.365667659938));
#241541=CARTESIAN_POINT('Ctrl Pts',(-205.336018648977,1.99446775428004,
126.306571402498));
#241542=CARTESIAN_POINT('Ctrl Pts',(-205.34376671698,1.86819539035735,126.252676788146));
#241543=CARTESIAN_POINT('Ctrl Pts',(-205.351514784983,1.73996087015536,
126.204173748228));
#241544=CARTESIAN_POINT('Ctrl Pts',(-205.359271087725,1.61159006077877,
126.155619158702));
#241545=CARTESIAN_POINT('Ctrl Pts',(-205.367027390467,1.48125329557024,
126.112467728895));
#241546=CARTESIAN_POINT('Ctrl Pts',(-205.374783693208,1.34944734045477,
126.07486012197));
#241547=CARTESIAN_POINT('Ctrl Pts',(-205.382544135723,1.21757103653245,
126.037232442734));
#241548=CARTESIAN_POINT('Ctrl Pts',(-205.390304578237,1.0842243601514,126.005154573647));
#241549=CARTESIAN_POINT('Ctrl Pts',(-205.398065020751,0.94991479207595,
125.978716106177));
#241550=CARTESIAN_POINT('Ctrl Pts',(-205.405837921016,0.815389618358384,
125.952235197333));
#241551=CARTESIAN_POINT('Ctrl Pts',(-205.413610821282,0.679898850757354,
125.931411840046));
#241552=CARTESIAN_POINT('Ctrl Pts',(-205.421383721547,0.543956519674996,
125.916283862113));
#241553=CARTESIAN_POINT('Ctrl Pts',(-205.428874057309,0.412956034745918,
125.901705824283));
#241554=CARTESIAN_POINT('Ctrl Pts',(-205.436364393071,0.281536554534047,
125.892416293839));
#241555=CARTESIAN_POINT('Ctrl Pts',(-205.443854728833,0.150156553991709,
125.888403328106));
#241556=CARTESIAN_POINT('Ctrl Pts',(-205.451629062952,0.0137952407976317,
125.884238209558));
#241557=CARTESIAN_POINT('Ctrl Pts',(-205.459403397071,-0.122955491538462,
125.885744482312));
#241558=CARTESIAN_POINT('Ctrl Pts',(-205.46717773119,-0.259584656345014,
125.892965818867));
#241559=CARTESIAN_POINT('Ctrl Pts',(-205.474942484137,-0.396045437916839,
125.900178255769));
#241560=CARTESIAN_POINT('Ctrl Pts',(-205.482707237084,-0.532384563386209,
125.913091721957));
#241561=CARTESIAN_POINT('Ctrl Pts',(-205.490471990031,-0.668088201124236,
125.931697976051));
#241562=CARTESIAN_POINT('Ctrl Pts',(-205.498229030916,-0.803657056095805,
125.950285750151));
#241563=CARTESIAN_POINT('Ctrl Pts',(-205.505986071801,-0.938591294568638,
125.974555007365));
#241564=CARTESIAN_POINT('Ctrl Pts',(-205.513743112686,-1.07237972584027,
126.004445536431));
#241565=CARTESIAN_POINT('Ctrl Pts',(-205.521494303926,-1.20606726621606,
126.034313524817));
#241566=CARTESIAN_POINT('Ctrl Pts',(-205.529245495166,-1.33861033923932,
126.069794262592));
#241567=CARTESIAN_POINT('Ctrl Pts',(-205.536996686406,-1.4695058559177,
126.110776102302));
#241568=CARTESIAN_POINT('Ctrl Pts',(-205.544744583183,-1.60034573850956,
126.151740523638));
#241569=CARTESIAN_POINT('Ctrl Pts',(-205.55249247996,-1.72953908518632,
126.198201280005));
#241570=CARTESIAN_POINT('Ctrl Pts',(-205.560240376737,-1.85659614912279,
126.249996358796));
#241571=CARTESIAN_POINT('Ctrl Pts',(-205.567986652821,-1.98362663546017,
126.301780603172));
#241572=CARTESIAN_POINT('Ctrl Pts',(-205.575732928906,-2.10852136608529,
126.358896803041));
#241573=CARTESIAN_POINT('Ctrl Pts',(-205.58347920499,-2.23080920216611,
126.421134252657));
#241574=CARTESIAN_POINT('Ctrl Pts',(-205.591225538255,-2.35309794094813,
126.483372161696));
#241575=CARTESIAN_POINT('Ctrl Pts',(-205.59897187152,-2.47277939835213,
126.550731218584));
#241576=CARTESIAN_POINT('Ctrl Pts',(-205.606718204785,-2.58940609623158,
126.622954259497));
#241577=CARTESIAN_POINT('Ctrl Pts',(-205.614466272788,-2.70605891185186,
126.69519347426));
#241578=CARTESIAN_POINT('Ctrl Pts',(-205.622214340791,-2.81965527435539,
126.77229863474));
#241579=CARTESIAN_POINT('Ctrl Pts',(-205.629962408794,-2.92977614598774,
126.853968890547));
#241580=CARTESIAN_POINT('Ctrl Pts',(-205.637718711536,-3.04001405539247,
126.935725946473));
#241581=CARTESIAN_POINT('Ctrl Pts',(-205.645475014278,-3.14676878064829,
127.022057556528));
#241582=CARTESIAN_POINT('Ctrl Pts',(-205.65323131702,-3.24965346373534,
127.112621809344));
#241583=CARTESIAN_POINT('Ctrl Pts',(-205.660991759534,-3.35259305947554,
127.203234399029));
#241584=CARTESIAN_POINT('Ctrl Pts',(-205.668752202048,-3.45165821498836,
127.298083862653));
#241585=CARTESIAN_POINT('Ctrl Pts',(-205.676512644562,-3.54649924868453,
127.396791668655));
#241586=CARTESIAN_POINT('Ctrl Pts',(-205.684285544827,-3.64149252962784,
127.495657929191));
#241587=CARTESIAN_POINT('Ctrl Pts',(-205.692058445093,-3.73224787929608,
127.598394616017));
#241588=CARTESIAN_POINT('Ctrl Pts',(-205.699831345358,-3.81845562610398,
127.704589707648));
#241589=CARTESIAN_POINT('Ctrl Pts',(-205.707321681121,-3.90152950417868,
127.806924340218));
#241590=CARTESIAN_POINT('Ctrl Pts',(-205.714812016883,-3.98038048839516,
127.912470052807));
#241591=CARTESIAN_POINT('Ctrl Pts',(-205.722302352646,-4.05477080955335,
128.020834662146));
#241592=CARTESIAN_POINT('Ctrl Pts',(-205.730448383082,-4.13567316687673,
128.138685374571));
#241593=CARTESIAN_POINT('Ctrl Pts',(-205.738594413519,-4.21155944536966,
128.260249366182));
#241594=CARTESIAN_POINT('Ctrl Pts',(-205.746740443956,-4.28207823747369,
128.385065465946));
#241595=CARTESIAN_POINT('Ctrl Pts',(-205.754614573043,-4.35024322610434,
128.505715405734));
#241596=CARTESIAN_POINT('Ctrl Pts',(-205.76248870213,-4.41339304358188,
128.629403491818));
#241597=CARTESIAN_POINT('Ctrl Pts',(-205.770362831217,-4.47125192901984,
128.755680737805));
#241598=CARTESIAN_POINT('Ctrl Pts',(-205.778228904709,-4.52905162216871,
128.881828796388));
#241599=CARTESIAN_POINT('Ctrl Pts',(-205.786094978202,-4.58157099847426,
129.010560404246));
#241600=CARTESIAN_POINT('Ctrl Pts',(-205.793961051694,-4.62857939142672,
129.141400642173));
#241601=CARTESIAN_POINT('Ctrl Pts',(-205.801819026306,-4.67553938470417,
129.272106167454));
#241602=CARTESIAN_POINT('Ctrl Pts',(-205.809677000917,-4.7169995704176,
129.404915645517));
#241603=CARTESIAN_POINT('Ctrl Pts',(-205.817534975528,-4.75277695961418,
129.539333252383));
#241604=CARTESIAN_POINT('Ctrl Pts',(-205.818374889647,-4.75660109188932,
129.553700726375));
#241605=CARTESIAN_POINT('Ctrl Pts',(-205.819214803765,-4.76036034493871,
129.568086554707));
#241606=CARTESIAN_POINT('Ctrl Pts',(-205.820054717884,-4.76405452823395,
129.582490119308));
#241607=CARTESIAN_POINT('Ctrl Pts',(-204.070038127516,-4.76405452823409,
129.582490119308));
#241608=CARTESIAN_POINT('Ctrl Pts',(-204.079301788646,-4.80448438634937,
129.740125522491));
#241609=CARTESIAN_POINT('Ctrl Pts',(-204.088565449776,-4.837125792116,129.899922785572));
#241610=CARTESIAN_POINT('Ctrl Pts',(-204.097829110906,-4.86177557562907,
130.061177386649));
#241611=CARTESIAN_POINT('Ctrl Pts',(-204.106997320508,-4.88617137106238,
130.220770441836));
#241612=CARTESIAN_POINT('Ctrl Pts',(-204.11616553011,-4.9027393278596,130.381790901728));
#241613=CARTESIAN_POINT('Ctrl Pts',(-204.125333739712,-4.91132906577983,
130.543535254293));
#241614=CARTESIAN_POINT('Ctrl Pts',(-204.130175638457,-4.91586546307692,
130.628955397563));
#241615=CARTESIAN_POINT('Ctrl Pts',(-204.135017537202,-4.91817745258136,
130.71457709991));
#241616=CARTESIAN_POINT('Ctrl Pts',(-204.139859435948,-4.91824831916273,
130.80029447038));
#241617=CARTESIAN_POINT('Origin',(213.235140564004,0.,130.804360617566));
#241618=CARTESIAN_POINT('',(-202.319765235154,-4.76405452823411,129.582490119309));
#241619=CARTESIAN_POINT('',(-202.665364488388,-4.77027151308326,129.580941132323));
#241620=CARTESIAN_POINT('',(213.235140564004,-4.76405452823405,129.582490119308));
#241621=CARTESIAN_POINT('',(-202.735140564013,-4.91326211273809,130.800663901985));
#241622=CARTESIAN_POINT('Ctrl Pts',(-202.665364488388,-4.77027151308407,
129.580941132326));
#241623=CARTESIAN_POINT('Ctrl Pts',(-202.688623180263,-4.86916182929373,
129.978023072962));
#241624=CARTESIAN_POINT('Ctrl Pts',(-202.711881872138,-4.91612258108715,
130.389021896046));
#241625=CARTESIAN_POINT('Ctrl Pts',(-202.735140564013,-4.91326211273809,
130.800663901985));
#241626=CARTESIAN_POINT('Ctrl Pts',(-202.735140564013,-4.91326211273809,
130.800663901985));
#241627=CARTESIAN_POINT('Ctrl Pts',(-202.796172748794,-4.90575607440281,
131.880836901629));
#241628=CARTESIAN_POINT('Ctrl Pts',(-202.950020808181,-4.02207680521533,
134.614867738963));
#241629=CARTESIAN_POINT('Ctrl Pts',(-203.19668474217,0.501577616433585,
136.600057273287));
#241630=CARTESIAN_POINT('Ctrl Pts',(-203.475132365984,5.14719869251641,
133.515084773622));
#241631=CARTESIAN_POINT('Ctrl Pts',(-203.753579989796,5.06279562480976,
127.939089200777));
#241632=CARTESIAN_POINT('Ctrl Pts',(-204.032027613609,0.325930709221482,
124.996138083671));
#241633=CARTESIAN_POINT('Ctrl Pts',(-204.25262932692,-3.66416944143293,
126.893211472255));
#241634=CARTESIAN_POINT('Ctrl Pts',(-204.380415165628,-4.60798580335201,
128.983142737816));
#241635=CARTESIAN_POINT('Ctrl Pts',(-204.415385129731,-4.7580624943176,
129.583982083009));
#241636=CARTESIAN_POINT('',(-202.389859436034,-4.91824990320504,130.803384849354));
#241637=CARTESIAN_POINT('Ctrl Pts',(-202.389859436034,-4.91824990320504,
130.803384849353));
#241638=CARTESIAN_POINT('Ctrl Pts',(-202.397592511015,-4.91827683063906,
130.939109551199));
#241639=CARTESIAN_POINT('Ctrl Pts',(-202.405325585996,-4.91268128621269,
131.075059385912));
#241640=CARTESIAN_POINT('Ctrl Pts',(-202.413058660977,-4.90143341606133,
131.210726869139));
#241641=CARTESIAN_POINT('Ctrl Pts',(-202.42078228894,-4.89019928673439,
131.346228615827));
#241642=CARTESIAN_POINT('Ctrl Pts',(-202.428505916903,-4.87332660037077,
131.481448306892));
#241643=CARTESIAN_POINT('Ctrl Pts',(-202.436229544867,-4.8508374788153,
131.615876986237));
#241644=CARTESIAN_POINT('Ctrl Pts',(-202.443945635588,-4.82837030367676,
131.750174480918));
#241645=CARTESIAN_POINT('Ctrl Pts',(-202.451661726309,-4.80029766335863,
131.883682112162));
#241646=CARTESIAN_POINT('Ctrl Pts',(-202.45937781703,-4.76669356115084,
132.015894998664));
#241647=CARTESIAN_POINT('Ctrl Pts',(-202.467088273264,-4.73311399751808,
132.148011339935));
#241648=CARTESIAN_POINT('Ctrl Pts',(-202.474798729498,-4.69401110747945,
132.278834436168));
#241649=CARTESIAN_POINT('Ctrl Pts',(-202.482509185732,-4.64951007925511,
132.407868985304));
#241650=CARTESIAN_POINT('Ctrl Pts',(-202.490216665053,-4.6050262323335,
132.536853715778));
#241651=CARTESIAN_POINT('Ctrl Pts',(-202.497924144375,-4.55514851955673,
132.664050898828));
#241652=CARTESIAN_POINT('Ctrl Pts',(-202.505631623696,-4.50005207787166,
132.788980066968));
#241653=CARTESIAN_POINT('Ctrl Pts',(-202.513337751278,-4.44496529901407,
132.913887324999));
#241654=CARTESIAN_POINT('Ctrl Pts',(-202.521043878859,-4.38466177095691,
133.036526997411));
#241655=CARTESIAN_POINT('Ctrl Pts',(-202.528750006441,-4.31936471923195,
133.156438738028));
#241656=CARTESIAN_POINT('Ctrl Pts',(-202.536456496514,-4.25406459597308,
133.27635611922));
#241657=CARTESIAN_POINT('Ctrl Pts',(-202.544162986588,-4.18377067092648,
133.39354496595));
#241658=CARTESIAN_POINT('Ctrl Pts',(-202.551869476661,-4.10875183304938,
133.507570087236));
#241659=CARTESIAN_POINT('Ctrl Pts',(-202.559578043381,-4.03371278004685,
133.621625934566));
#241660=CARTESIAN_POINT('Ctrl Pts',(-202.567286610102,-3.95394649875435,
133.732516030231));
#241661=CARTESIAN_POINT('Ctrl Pts',(-202.574995176822,-3.86976457714697,
133.839835074708));
#241662=CARTESIAN_POINT('Ctrl Pts',(-202.582712029366,-3.78549216965473,
133.947269474815));
#241663=CARTESIAN_POINT('Ctrl Pts',(-202.590428881909,-3.69679488857133,
134.051124847371));
#241664=CARTESIAN_POINT('Ctrl Pts',(-202.598145734452,-3.60402417816858,
134.151029526448));
#241665=CARTESIAN_POINT('Ctrl Pts',(-202.605867103336,-3.51119917307237,
134.250992675422));
#241666=CARTESIAN_POINT('Ctrl Pts',(-202.61358847222,-3.41429627095629,
134.347000247896));
#241667=CARTESIAN_POINT('Ctrl Pts',(-202.621309841104,-3.31370214936235,
134.438719037949));
#241668=CARTESIAN_POINT('Ctrl Pts',(-202.629042866836,-3.21295616217193,
134.530576294631));
#241669=CARTESIAN_POINT('Ctrl Pts',(-202.636775892567,-3.10850812896895,
134.618131584567));
#241670=CARTESIAN_POINT('Ctrl Pts',(-202.644508918298,-3.00077647222385,
134.701093046954));
#241671=CARTESIAN_POINT('Ctrl Pts',(-202.649465442433,-2.93172529156538,
134.754267639271));
#241672=CARTESIAN_POINT('Ctrl Pts',(-202.654421966569,-2.86132571321719,
134.80555585624));
#241673=CARTESIAN_POINT('Ctrl Pts',(-202.659378490704,-2.7896934030652,
134.8548906791));
#241674=CARTESIAN_POINT('Ctrl Pts',(-202.667152824823,-2.67733774865093,
134.932272607676));
#241675=CARTESIAN_POINT('Ctrl Pts',(-202.674927158942,-2.56158200219939,
135.005098693772));
#241676=CARTESIAN_POINT('Ctrl Pts',(-202.682701493061,-2.4428319884996,
135.07305537574));
#241677=CARTESIAN_POINT('Ctrl Pts',(-202.690466246008,-2.32422832357901,
135.140928307171));
#241678=CARTESIAN_POINT('Ctrl Pts',(-202.698230998955,-2.20263806981494,
135.203943582563));
#241679=CARTESIAN_POINT('Ctrl Pts',(-202.705995751903,-2.078497570351,135.261829732719));
#241680=CARTESIAN_POINT('Ctrl Pts',(-202.713752792788,-1.95448036898086,
135.319658389536));
#241681=CARTESIAN_POINT('Ctrl Pts',(-202.721509833673,-1.82791831461926,
135.372367894886));
#241682=CARTESIAN_POINT('Ctrl Pts',(-202.729266874558,-1.69927368819759,
135.419731891375));
#241683=CARTESIAN_POINT('Ctrl Pts',(-202.737018065798,-1.57072607368995,
135.467060170305));
#241684=CARTESIAN_POINT('Ctrl Pts',(-202.744769257038,-1.44009937847901,
135.50905082948));
#241685=CARTESIAN_POINT('Ctrl Pts',(-202.752520448278,-1.30787694231266,
135.545525133407));
#241686=CARTESIAN_POINT('Ctrl Pts',(-202.760268345055,-1.17571070420829,
135.581983934782));
#241687=CARTESIAN_POINT('Ctrl Pts',(-202.768016241832,-1.04195045020032,
135.612930940387));
#241688=CARTESIAN_POINT('Ctrl Pts',(-202.77576413861,-0.907095593932953,
135.638236975725));
#241689=CARTESIAN_POINT('Ctrl Pts',(-202.783510414694,-0.772268946394382,
135.663537717586));
#241690=CARTESIAN_POINT('Ctrl Pts',(-202.791256690778,-0.636348536039387,
135.683199764143));
#241691=CARTESIAN_POINT('Ctrl Pts',(-202.799002966862,-0.49984451854849,
135.697144949598));
#241692=CARTESIAN_POINT('Ctrl Pts',(-202.806749300127,-0.363339493416131,
135.711090237993));
#241693=CARTESIAN_POINT('Ctrl Pts',(-202.814495633393,-0.226251241492333,
135.719318541345));
#241694=CARTESIAN_POINT('Ctrl Pts',(-202.822241966658,-0.0890952027191759,
135.721803561551));
#241695=CARTESIAN_POINT('Ctrl Pts',(-202.829990034661,0.0480915511977042,
135.724289138261));
#241696=CARTESIAN_POINT('Ctrl Pts',(-202.837738102664,0.18534573134494,
135.721028865417));
#241697=CARTESIAN_POINT('Ctrl Pts',(-202.845486170667,0.322152132501905,
135.712048572808));
#241698=CARTESIAN_POINT('Ctrl Pts',(-202.853242473409,0.459103933130223,
135.703058735837));
#241699=CARTESIAN_POINT('Ctrl Pts',(-202.860998776151,0.595606613349426,
135.688336760683));
#241700=CARTESIAN_POINT('Ctrl Pts',(-202.868755078893,0.731149768151804,
135.667960424194));
#241701=CARTESIAN_POINT('Ctrl Pts',(-202.876515521407,0.866765266417027,
135.647573212241));
#241702=CARTESIAN_POINT('Ctrl Pts',(-202.884275963921,1.00141983514607,
135.62152569974));
#241703=CARTESIAN_POINT('Ctrl Pts',(-202.892036406435,1.1346144753236,135.589946585333));
#241704=CARTESIAN_POINT('Ctrl Pts',(-202.899809306701,1.268022931362,135.558316777328));
#241705=CARTESIAN_POINT('Ctrl Pts',(-202.907582206966,1.39996639904794,
135.521137728808));
#241706=CARTESIAN_POINT('Ctrl Pts',(-202.915355107232,1.52996136298433,
135.478587964441));
#241707=CARTESIAN_POINT('Ctrl Pts',(-202.922845442994,1.65523068254303,
135.437584991186));
#241708=CARTESIAN_POINT('Ctrl Pts',(-202.930335778755,1.77869041621811,
135.391595108432));
#241709=CARTESIAN_POINT('Ctrl Pts',(-202.937826114517,1.89992823133841,
135.340819123743));
#241710=CARTESIAN_POINT('Ctrl Pts',(-202.945600448637,2.02576281507001,
135.28811795216));
#241711=CARTESIAN_POINT('Ctrl Pts',(-202.953374782756,2.14960227229255,
135.230093642708));
#241712=CARTESIAN_POINT('Ctrl Pts',(-202.961149116875,2.27096343650089,
135.166918139545));
#241713=CARTESIAN_POINT('Ctrl Pts',(-202.968913869822,2.39217503392037,
135.103820494544));
#241714=CARTESIAN_POINT('Ctrl Pts',(-202.976678622769,2.51091407195934,
135.03558446602));
#241715=CARTESIAN_POINT('Ctrl Pts',(-202.984443375716,2.62671630176767,
134.962430426086));
#241716=CARTESIAN_POINT('Ctrl Pts',(-202.992200416601,2.74240351516851,
134.889349043777));
#241717=CARTESIAN_POINT('Ctrl Pts',(-202.999957457486,2.85515939666273,
134.811359578162));
#241718=CARTESIAN_POINT('Ctrl Pts',(-203.007714498371,2.96454363122682,
134.728728607581));
#241719=CARTESIAN_POINT('Ctrl Pts',(-203.015465689611,3.07384537828889,
134.646159949657));
#241720=CARTESIAN_POINT('Ctrl Pts',(-203.023216880851,3.1797802285859,134.558956988398));
#241721=CARTESIAN_POINT('Ctrl Pts',(-203.030968072092,3.28193654994615,
134.467429760324));
#241722=CARTESIAN_POINT('Ctrl Pts',(-203.038715968869,3.38404945214513,
134.375941433763));
#241723=CARTESIAN_POINT('Ctrl Pts',(-203.046463865646,3.48238672899254,
134.280132756231));
#241724=CARTESIAN_POINT('Ctrl Pts',(-203.054211762423,3.57656975705238,
134.1803540766));
#241725=CARTESIAN_POINT('Ctrl Pts',(-203.061958038507,3.67073308405285,
134.080596268517));
#241726=CARTESIAN_POINT('Ctrl Pts',(-203.069704314591,3.76074362251624,
133.976870394256));
#241727=CARTESIAN_POINT('Ctrl Pts',(-203.077450590675,3.84625985773754,
133.869563411715));
#241728=CARTESIAN_POINT('Ctrl Pts',(-203.085196923941,3.93177672422038,
133.762255637058));
#241729=CARTESIAN_POINT('Ctrl Pts',(-203.092943257206,4.01279897759957,
133.651367007122));
#241730=CARTESIAN_POINT('Ctrl Pts',(-203.100689590471,4.08902588465788,
133.537316961363));
#241731=CARTESIAN_POINT('Ctrl Pts',(-203.108437658474,4.1652698622036,133.423241374886));
#241732=CARTESIAN_POINT('Ctrl Pts',(-203.116185726477,4.23671613931385,
133.306003288778));
#241733=CARTESIAN_POINT('Ctrl Pts',(-203.12393379448,4.30310796631424,133.186050121415));
#241734=CARTESIAN_POINT('Ctrl Pts',(-203.131690097222,4.36957035533834,
133.065969466397));
#241735=CARTESIAN_POINT('Ctrl Pts',(-203.139446399964,4.43096737361537,
132.943168308397));
#241736=CARTESIAN_POINT('Ctrl Pts',(-203.147202702706,4.48708857063544,
132.818118105888));
#241737=CARTESIAN_POINT('Ctrl Pts',(-203.15496314522,4.54323972122798,132.693001160321));
#241738=CARTESIAN_POINT('Ctrl Pts',(-203.162723587734,4.59410929477576,
132.565633141281));
#241739=CARTESIAN_POINT('Ctrl Pts',(-203.170484030249,4.63953584793378,
132.436503435532));
#241740=CARTESIAN_POINT('Ctrl Pts',(-203.178256930514,4.68503532382784,
132.307166439315));
#241741=CARTESIAN_POINT('Ctrl Pts',(-203.18602983078,4.72507420452498,132.176062479243));
#241742=CARTESIAN_POINT('Ctrl Pts',(-203.193802731045,4.75954133600245,
132.043694847459));
#241743=CARTESIAN_POINT('Ctrl Pts',(-203.201293066807,4.79275550043213,
131.916139112508));
#241744=CARTESIAN_POINT('Ctrl Pts',(-203.208783402569,4.82079591129226,
131.787410287015));
#241745=CARTESIAN_POINT('Ctrl Pts',(-203.21627373833,4.84360863779292,131.657963819527));
#241746=CARTESIAN_POINT('Ctrl Pts',(-203.224048072449,4.86728631575333,
131.523609349876));
#241747=CARTESIAN_POINT('Ctrl Pts',(-203.231822406569,4.8854070724529,131.388056150618));
#241748=CARTESIAN_POINT('Ctrl Pts',(-203.239596740688,4.89785440608457,
131.251803663437));
#241749=CARTESIAN_POINT('Ctrl Pts',(-203.247361493635,4.91028639949003,
131.115719095268));
#241750=CARTESIAN_POINT('Ctrl Pts',(-203.255126246582,4.91705884657044,
130.978937339527));
#241751=CARTESIAN_POINT('Ctrl Pts',(-203.262890999529,4.91810621478259,
130.841968098429));
#241752=CARTESIAN_POINT('Ctrl Pts',(-203.270648040414,4.91915254273387,
130.705134897112));
#241753=CARTESIAN_POINT('Ctrl Pts',(-203.278405081299,4.91448510469911,
130.568114969434));
#241754=CARTESIAN_POINT('Ctrl Pts',(-203.286162122184,4.90409017955869,
130.431422857));
#241755=CARTESIAN_POINT('Ctrl Pts',(-203.293913313424,4.89370309331222,
130.294833825151));
#241756=CARTESIAN_POINT('Ctrl Pts',(-203.301664504664,4.8775971464774,130.158572504755));
#241757=CARTESIAN_POINT('Ctrl Pts',(-203.309415695904,4.85581068431517,
130.023152795927));
#241758=CARTESIAN_POINT('Ctrl Pts',(-203.317163592681,4.8340334819805,129.887790644087));
#241759=CARTESIAN_POINT('Ctrl Pts',(-203.324911489458,4.8065806282877,129.753269777556));
#241760=CARTESIAN_POINT('Ctrl Pts',(-203.332659386236,4.77354222644985,
129.620098115078));
#241761=CARTESIAN_POINT('Ctrl Pts',(-203.34040566232,4.74051073553344,129.48695430924));
#241762=CARTESIAN_POINT('Ctrl Pts',(-203.348151938404,4.70189611451706,
129.355159525316));
#241763=CARTESIAN_POINT('Ctrl Pts',(-203.355898214488,4.65783932500118,
129.225210249497));
#241764=CARTESIAN_POINT('Ctrl Pts',(-203.363644547753,4.61378221026816,
129.095260014422));
#241765=CARTESIAN_POINT('Ctrl Pts',(-203.371390881019,4.56428297240465,
128.967155684899));
#241766=CARTESIAN_POINT('Ctrl Pts',(-203.379137214284,4.50953194405326,
128.841376993573));
#241767=CARTESIAN_POINT('Ctrl Pts',(-203.386885282287,4.45476865458861,
128.715570134981));
#241768=CARTESIAN_POINT('Ctrl Pts',(-203.39463335029,4.39475139034221,128.592090309345));
#241769=CARTESIAN_POINT('Ctrl Pts',(-203.402381418293,4.32971779759376,
128.471395367996));
#241770=CARTESIAN_POINT('Ctrl Pts',(-203.410137721035,4.26461508636893,
128.350572150628));
#241771=CARTESIAN_POINT('Ctrl Pts',(-203.417894023777,4.19448558231854,
128.232540074813));
#241772=CARTESIAN_POINT('Ctrl Pts',(-203.425650326518,4.11961218316801,
128.117731033348));
#241773=CARTESIAN_POINT('Ctrl Pts',(-203.433410769033,4.04469882182997,
128.002860714841));
#241774=CARTESIAN_POINT('Ctrl Pts',(-203.441171211547,3.96503674722332,
127.891217176486));
#241775=CARTESIAN_POINT('Ctrl Pts',(-203.448931654061,3.88095043022052,
127.783200770641));
#241776=CARTESIAN_POINT('Ctrl Pts',(-203.456704554326,3.79672913039707,
127.675010967273));
#241777=CARTESIAN_POINT('Ctrl Pts',(-203.464477454592,3.70806964875335,
127.570460230171));
#241778=CARTESIAN_POINT('Ctrl Pts',(-203.472250354857,3.61533533775766,
127.469914118061));
#241779=CARTESIAN_POINT('Ctrl Pts',(-203.479740690619,3.52597215254956,
127.373023110385));
#241780=CARTESIAN_POINT('Ctrl Pts',(-203.487231026381,3.4328254728641,127.279850844024));
#241781=CARTESIAN_POINT('Ctrl Pts',(-203.494721362143,3.3362493295539,127.190688873543));
#241782=CARTESIAN_POINT('Ctrl Pts',(-203.502495696262,3.23601147241738,
127.098146299852));
#241783=CARTESIAN_POINT('Ctrl Pts',(-203.510270030382,3.13176143843621,
127.009630978764));
#241784=CARTESIAN_POINT('Ctrl Pts',(-203.518044364501,3.0238564499707,126.92551088698));
#241785=CARTESIAN_POINT('Ctrl Pts',(-203.525809117448,2.91608444475944,
126.84149446569));
#241786=CARTESIAN_POINT('Ctrl Pts',(-203.533573870395,2.80466675286709,
126.761862734097));
#241787=CARTESIAN_POINT('Ctrl Pts',(-203.541338623342,2.68999677926315,
126.686946333084));
#241788=CARTESIAN_POINT('Ctrl Pts',(-203.549095664227,2.57544069749386,
126.612104340097));
#241789=CARTESIAN_POINT('Ctrl Pts',(-203.556852705112,2.45763908746732,
126.541968570097));
#241790=CARTESIAN_POINT('Ctrl Pts',(-203.564609745997,2.33701743100642,
126.476828689357));
#241791=CARTESIAN_POINT('Ctrl Pts',(-203.572360937237,2.2164867362748,126.411737931106));
#241792=CARTESIAN_POINT('Ctrl Pts',(-203.580112128477,2.09314057063032,
126.35163574828));
#241793=CARTESIAN_POINT('Ctrl Pts',(-203.587863319717,1.96743201934503,
126.29676765549));
#241794=CARTESIAN_POINT('Ctrl Pts',(-203.595611216494,1.84177689754726,
126.241922883103));
#241795=CARTESIAN_POINT('Ctrl Pts',(-203.603359113271,1.71376174471187,
126.192307932205));
#241796=CARTESIAN_POINT('Ctrl Pts',(-203.611107010048,1.58386259025,126.148121538899));
#241797=CARTESIAN_POINT('Ctrl Pts',(-203.618853286132,1.45399060789093,
126.103944388434));
#241798=CARTESIAN_POINT('Ctrl Pts',(-203.626599562217,1.32223577767975,
126.06519366274));
#241799=CARTESIAN_POINT('Ctrl Pts',(-203.634345838301,1.18909200069798,
126.032019129745));
#241800=CARTESIAN_POINT('Ctrl Pts',(-203.642092171566,1.05594724087891,
125.998844351863));
#241801=CARTESIAN_POINT('Ctrl Pts',(-203.649838504831,0.921413893196879,
125.97124594334));
#241802=CARTESIAN_POINT('Ctrl Pts',(-203.657584838097,0.785998449754042,
125.949323079144));
#241803=CARTESIAN_POINT('Ctrl Pts',(-203.6653329061,0.650552680961736,125.927395305475));
#241804=CARTESIAN_POINT('Ctrl Pts',(-203.673080974103,0.514224809194846,
125.911145667744));
#241805=CARTESIAN_POINT('Ctrl Pts',(-203.680829042106,0.377528491365758,
125.900621707234));
#241806=CARTESIAN_POINT('Ctrl Pts',(-203.688585344847,0.240686891063561,
125.890086561733));
#241807=CARTESIAN_POINT('Ctrl Pts',(-203.696341647589,0.103476452891485,
125.88528927959));
#241808=CARTESIAN_POINT('Ctrl Pts',(-203.704097950331,-0.0335865463790532,
125.886225299541));
#241809=CARTESIAN_POINT('Ctrl Pts',(-203.711858392845,-0.17072270029919,
125.887161819075));
#241810=CARTESIAN_POINT('Ctrl Pts',(-203.719618835359,-0.307710868205461,
125.893837719063));
#241811=CARTESIAN_POINT('Ctrl Pts',(-203.727379277873,-0.44403883788848,
125.906196413199));
#241812=CARTESIAN_POINT('Ctrl Pts',(-203.735152178139,-0.580585653331063,
125.918574946608));
#241813=CARTESIAN_POINT('Ctrl Pts',(-203.742925078404,-0.716469764941721,
125.936654452284));
#241814=CARTESIAN_POINT('Ctrl Pts',(-203.75069797867,-0.851187216928724,
125.960326824926));
#241815=CARTESIAN_POINT('Ctrl Pts',(-203.758188314432,-0.981007350205763,
125.983138647196));
#241816=CARTESIAN_POINT('Ctrl Pts',(-203.765678650194,-1.10974387227684,
126.011143701039));
#241817=CARTESIAN_POINT('Ctrl Pts',(-203.773168985956,-1.23696012770498,
126.044201722637));
#241818=CARTESIAN_POINT('Ctrl Pts',(-203.780943320075,-1.36899982612075,
126.078513149172));
#241819=CARTESIAN_POINT('Ctrl Pts',(-203.788717654194,-1.4998199624505,
126.118376962119));
#241820=CARTESIAN_POINT('Ctrl Pts',(-203.796491988313,-1.62891786006441,
126.163691520586));
#241821=CARTESIAN_POINT('Ctrl Pts',(-203.80425674126,-1.75785665605768,
126.20895023291));
#241822=CARTESIAN_POINT('Ctrl Pts',(-203.812021494207,-1.88507707112989,
126.259646196572));
#241823=CARTESIAN_POINT('Ctrl Pts',(-203.819786247154,-2.01008828274693,
126.315627148305));
#241824=CARTESIAN_POINT('Ctrl Pts',(-203.827543288039,-2.13497533146623,
126.371552498967));
#241825=CARTESIAN_POINT('Ctrl Pts',(-203.835300328924,-2.25765718879851,
126.432752232951));
#241826=CARTESIAN_POINT('Ctrl Pts',(-203.843057369809,-2.37766016698767,
126.499024952043));
#241827=CARTESIAN_POINT('Ctrl Pts',(-203.850808561049,-2.49757264999765,
126.565247694363));
#241828=CARTESIAN_POINT('Ctrl Pts',(-203.858559752289,-2.61480993401946,
126.63653561897));
#241829=CARTESIAN_POINT('Ctrl Pts',(-203.866310943529,-2.72892055700057,
126.712640239036));
#241830=CARTESIAN_POINT('Ctrl Pts',(-203.874058840306,-2.84298267992244,
126.788712512608));
#241831=CARTESIAN_POINT('Ctrl Pts',(-203.881806737083,-2.95392046033182,
126.869597193392));
#241832=CARTESIAN_POINT('Ctrl Pts',(-203.88955463386,-3.06130939039301,
126.955001206081));
#241833=CARTESIAN_POINT('Ctrl Pts',(-203.897300909944,-3.16867585700537,
127.040387354091));
#241834=CARTESIAN_POINT('Ctrl Pts',(-203.905047186028,-3.27249464402813,
127.130290710461));
#241835=CARTESIAN_POINT('Ctrl Pts',(-203.912793462112,-3.3723727818643,
127.224376695446));
#241836=CARTESIAN_POINT('Ctrl Pts',(-203.920539795377,-3.47225165697833,
127.318463374952));
#241837=CARTESIAN_POINT('Ctrl Pts',(-203.928286128643,-3.56818954027803,
127.416732476603));
#241838=CARTESIAN_POINT('Ctrl Pts',(-203.936032461908,-3.65982922170008,
127.518811480741));
#241839=CARTESIAN_POINT('Ctrl Pts',(-203.943780529911,-3.75148942519278,
127.620913344764));
#241840=CARTESIAN_POINT('Ctrl Pts',(-203.951528597914,-3.83884925031249,
127.726826518173));
#241841=CARTESIAN_POINT('Ctrl Pts',(-203.959276665916,-3.92159105512307,
127.836144544084));
#241842=CARTESIAN_POINT('Ctrl Pts',(-203.967032968658,-4.00442079890878,
127.945578754494));
#241843=CARTESIAN_POINT('Ctrl Pts',(-203.9747892714,-4.08262248162509,128.05842473395));
#241844=CARTESIAN_POINT('Ctrl Pts',(-203.982545574142,-4.15592088058601,
128.174245658708));
#241845=CARTESIAN_POINT('Ctrl Pts',(-203.990306016656,-4.22925840110944,
128.290128400581));
#241846=CARTESIAN_POINT('Ctrl Pts',(-203.99806645917,-4.29768722825386,
128.408988912957));
#241847=CARTESIAN_POINT('Ctrl Pts',(-204.005826901684,-4.36097810647042,
128.530365670917));
#241848=CARTESIAN_POINT('Ctrl Pts',(-204.013599801949,-4.42437058482357,
128.651937273624));
#241849=CARTESIAN_POINT('Ctrl Pts',(-204.021372702215,-4.48260846613932,
128.776032839594));
#241850=CARTESIAN_POINT('Ctrl Pts',(-204.02914560248,-4.53551030205551,
128.902169942989));
#241851=CARTESIAN_POINT('Ctrl Pts',(-204.036635938243,-4.58648902298876,
129.023721644965));
#241852=CARTESIAN_POINT('Ctrl Pts',(-204.044126274005,-4.63251281279301,
129.147168742662));
#241853=CARTESIAN_POINT('Ctrl Pts',(-204.051616609768,-4.67346365646167,
129.272068049473));
#241854=CARTESIAN_POINT('Ctrl Pts',(-204.057757115684,-4.70703476806217,
129.374459311585));
#241855=CARTESIAN_POINT('Ctrl Pts',(-204.0638976216,-4.73725521212647,129.477999992541));
#241856=CARTESIAN_POINT('Ctrl Pts',(-204.070038127516,-4.76405452823409,
129.582490119308));
#241857=CARTESIAN_POINT('Ctrl Pts',(-202.319765235154,-4.76405452823412,
129.582490119309));
#241858=CARTESIAN_POINT('Ctrl Pts',(-202.327527427096,-4.79811327357253,
129.715284650469));
#241859=CARTESIAN_POINT('Ctrl Pts',(-202.335289619037,-4.82658544150759,
129.849387011775));
#241860=CARTESIAN_POINT('Ctrl Pts',(-202.343051810979,-4.84939821559733,
129.984287444574));
#241861=CARTESIAN_POINT('Ctrl Pts',(-202.350825702342,-4.87224537382299,
130.11939120358));
#241862=CARTESIAN_POINT('Ctrl Pts',(-202.358599593705,-4.88941605217232,
130.255295049384));
#241863=CARTESIAN_POINT('Ctrl Pts',(-202.366373485068,-4.90088936486764,
130.391484733277));
#241864=CARTESIAN_POINT('Ctrl Pts',(-202.371225945676,-4.90805100313769,
130.476494292247));
#241865=CARTESIAN_POINT('Ctrl Pts',(-202.376078406283,-4.91299384376543,
130.561615199731));
#241866=CARTESIAN_POINT('Ctrl Pts',(-202.380930866891,-4.91572308414765,
130.646722987294));
#241867=CARTESIAN_POINT('Ctrl Pts',(-202.383907056592,-4.91739702604547,
130.698922673462));
#241868=CARTESIAN_POINT('Ctrl Pts',(-202.386883246294,-4.9182395397714,
130.751149164821));
#241869=CARTESIAN_POINT('Ctrl Pts',(-202.389859435995,-4.9182499032049,
130.803384848665));
#241870=CARTESIAN_POINT('Origin',(213.235140564004,0.,130.804360617566));
#241871=CARTESIAN_POINT('',(-200.569853205643,-4.76405452823395,129.582490119308));
#241872=CARTESIAN_POINT('',(-200.91504706349,-4.76405452823395,129.582490119308));
#241873=CARTESIAN_POINT('',(213.235140564004,-4.76405452823405,129.582490119308));
#241874=CARTESIAN_POINT('',(-200.985142080239,-4.92392244591489,130.802667972596));
#241875=CARTESIAN_POINT('Ctrl Pts',(-200.91504706349,-4.76405452823395,
129.582490119308));
#241876=CARTESIAN_POINT('Ctrl Pts',(-200.922810977094,-4.79810171876979,
129.715239598469));
#241877=CARTESIAN_POINT('Ctrl Pts',(-200.930574890699,-4.82656335624725,
129.849285219688));
#241878=CARTESIAN_POINT('Ctrl Pts',(-200.938338804304,-4.84936942606639,
129.984117219523));
#241879=CARTESIAN_POINT('Ctrl Pts',(-200.946113769782,-4.87220796015882,
130.119141151722));
#241880=CARTESIAN_POINT('Ctrl Pts',(-200.953888735261,-4.88937480602331,
130.254953310856));
#241881=CARTESIAN_POINT('Ctrl Pts',(-200.96166370074,-4.90085188096385,
130.39104003575));
#241882=CARTESIAN_POINT('Ctrl Pts',(-200.964143717715,-4.90451277704879,
130.434448252648));
#241883=CARTESIAN_POINT('Ctrl Pts',(-200.966623734691,-4.90759516567256,
130.477884416332));
#241884=CARTESIAN_POINT('Ctrl Pts',(-200.969103751666,-4.91009957319356,
130.521331919685));
#241885=CARTESIAN_POINT('Ctrl Pts',(-200.974449355782,-4.91549775041753,
130.614981743472));
#241886=CARTESIAN_POINT('Ctrl Pts',(-200.979794959898,-4.91821692815383,
130.708787473997));
#241887=CARTESIAN_POINT('Ctrl Pts',(-200.985140564013,-4.91824970017718,
130.802643292019));
#241888=CARTESIAN_POINT('Ctrl Pts',(-200.985142543985,-4.92565748492521,
130.802675521279));
#241889=CARTESIAN_POINT('Ctrl Pts',(-201.072612154484,-4.9187069394712,
132.340745200837));
#241890=CARTESIAN_POINT('Ctrl Pts',(-201.252897639586,-3.31467917127183,
135.523358464972));
#241891=CARTESIAN_POINT('Ctrl Pts',(-201.525998999293,2.10959714028603,
136.225733113176));
#241892=CARTESIAN_POINT('Ctrl Pts',(-201.804446623106,5.70144300590434,
131.959881054809));
#241893=CARTESIAN_POINT('Ctrl Pts',(-202.082894246919,4.05394128007133,
126.632162164928));
#241894=CARTESIAN_POINT('Ctrl Pts',(-202.361341870732,-1.31893443610527,
125.138489829794));
#241895=CARTESIAN_POINT('Ctrl Pts',(-202.555498617888,-4.22021631041374,
127.727491303473));
#241896=CARTESIAN_POINT('Ctrl Pts',(-202.65683949044,-4.73402528963851,
129.435398865923));
#241897=CARTESIAN_POINT('Ctrl Pts',(-202.665364488388,-4.77027151308407,
129.580941132326));
#241898=CARTESIAN_POINT('',(-200.639859436051,-4.91824790596759,130.808899113513));
#241899=CARTESIAN_POINT('Ctrl Pts',(-200.639859436051,-4.91824790596758,
130.808899113514));
#241900=CARTESIAN_POINT('Ctrl Pts',(-200.649775499558,-4.91808625878195,
130.984071889128));
#241901=CARTESIAN_POINT('Ctrl Pts',(-200.659691563065,-4.9085624689396,
131.15882584626));
#241902=CARTESIAN_POINT('Ctrl Pts',(-200.669607626572,-4.8898314044626,
131.332311276654));
#241903=CARTESIAN_POINT('Ctrl Pts',(-200.679740109887,-4.87069153125199,
131.50958305668));
#241904=CARTESIAN_POINT('Ctrl Pts',(-200.689872593201,-4.84193809215862,
131.685530583323));
#241905=CARTESIAN_POINT('Ctrl Pts',(-200.700005076516,-4.80378435667934,
131.859272422895));
#241906=CARTESIAN_POINT('Ctrl Pts',(-200.703418425682,-4.7909314343376,
131.917801170958));
#241907=CARTESIAN_POINT('Ctrl Pts',(-200.706831774848,-4.77701213815199,
131.976079801564));
#241908=CARTESIAN_POINT('Ctrl Pts',(-200.710245124013,-4.76203582549044,
132.034075161371));
#241909=CARTESIAN_POINT('Ctrl Pts',(-200.718019458133,-4.72792538063196,
132.166166923039));
#241910=CARTESIAN_POINT('Ctrl Pts',(-200.725793792252,-4.68826069982342,
132.297047573819));
#241911=CARTESIAN_POINT('Ctrl Pts',(-200.733568126371,-4.64314265885356,
132.426214282985));
#241912=CARTESIAN_POINT('Ctrl Pts',(-200.741332879318,-4.59808022183689,
132.555221805726));
#241913=CARTESIAN_POINT('Ctrl Pts',(-200.749097632265,-4.5475779246939,
132.682519224107));
#241914=CARTESIAN_POINT('Ctrl Pts',(-200.756862385212,-4.49178728356926,
132.807615484443));
#241915=CARTESIAN_POINT('Ctrl Pts',(-200.764619426097,-4.43605205449589,
132.932587497409));
#241916=CARTESIAN_POINT('Ctrl Pts',(-200.772376466982,-4.37503909228266,
133.055362348256));
#241917=CARTESIAN_POINT('Ctrl Pts',(-200.780133507867,-4.30894907403695,
133.175466043281));
#241918=CARTESIAN_POINT('Ctrl Pts',(-200.787884699107,-4.2429088947882,
133.295479167176));
#241919=CARTESIAN_POINT('Ctrl Pts',(-200.795635890348,-4.17179946792055,
133.412824803525));
#241920=CARTESIAN_POINT('Ctrl Pts',(-200.803387081588,-4.09586859292485,
133.527051112645));
#241921=CARTESIAN_POINT('Ctrl Pts',(-200.811134978365,-4.01996999057645,
133.641228872536));
#241922=CARTESIAN_POINT('Ctrl Pts',(-200.818882875142,-3.93925423187122,
133.752289617197));
#241923=CARTESIAN_POINT('Ctrl Pts',(-200.826630771919,-3.85401374574893,
133.859808393274));
#241924=CARTESIAN_POINT('Ctrl Pts',(-200.834377048003,-3.76879109009876,
133.96730467874));
#241925=CARTESIAN_POINT('Ctrl Pts',(-200.842123324087,-3.67904583235511,
134.071260163147));
#241926=CARTESIAN_POINT('Ctrl Pts',(-200.849869600171,-3.58511195384299,
134.17128136818));
#241927=CARTESIAN_POINT('Ctrl Pts',(-200.857615933436,-3.49117738193219,
134.271303311546));
#241928=CARTESIAN_POINT('Ctrl Pts',(-200.865362266702,-3.39305439520117,
134.367390632596));
#241929=CARTESIAN_POINT('Ctrl Pts',(-200.873108599967,-3.29111496926247,
134.459185554768));
#241930=CARTESIAN_POINT('Ctrl Pts',(-200.88085666797,-3.18915271469628,
134.551001033777));
#241931=CARTESIAN_POINT('Ctrl Pts',(-200.888604735973,-3.08337261071428,
134.638521939557));
#241932=CARTESIAN_POINT('Ctrl Pts',(-200.896352803976,-2.9741806303318,
134.721430011981));
#241933=CARTESIAN_POINT('Ctrl Pts',(-200.904109106718,-2.86487259941302,
134.80442620009));
#241934=CARTESIAN_POINT('Ctrl Pts',(-200.91186540946,-2.75214576027803,
134.882799524622));
#241935=CARTESIAN_POINT('Ctrl Pts',(-200.919621712202,-2.63643651732246,
134.956274098436));
#241936=CARTESIAN_POINT('Ctrl Pts',(-200.927382154716,-2.52066551685999,
135.029787887842));
#241937=CARTESIAN_POINT('Ctrl Pts',(-200.93514259723,-2.40190927914698,
135.098397521213));
#241938=CARTESIAN_POINT('Ctrl Pts',(-200.942903039744,-2.28062897968,135.161873040904));
#241939=CARTESIAN_POINT('Ctrl Pts',(-200.95067594001,-2.15915399030956,
135.225450457134));
#241940=CARTESIAN_POINT('Ctrl Pts',(-200.958448840275,-2.03514719618037,
135.283877123337));
#241941=CARTESIAN_POINT('Ctrl Pts',(-200.966221740541,-1.90909074643751,
135.336970857192));
#241942=CARTESIAN_POINT('Ctrl Pts',(-200.973712076303,-1.78761676615949,
135.388134500087));
#241943=CARTESIAN_POINT('Ctrl Pts',(-200.981202412065,-1.66423985179437,
135.434346102061));
#241944=CARTESIAN_POINT('Ctrl Pts',(-200.988692747827,-1.5394030098361,
135.47548697379));
#241945=CARTESIAN_POINT('Ctrl Pts',(-200.996467081946,-1.40983294107218,
135.518187714174));
#241946=CARTESIAN_POINT('Ctrl Pts',(-201.004241416065,-1.27827961399708,
135.555560883532));
#241947=CARTESIAN_POINT('Ctrl Pts',(-201.012015750184,-1.14522060017088,
135.587419559231));
#241948=CARTESIAN_POINT('Ctrl Pts',(-201.019780503131,-1.01232556968741,
135.61923897196));
#241949=CARTESIAN_POINT('Ctrl Pts',(-201.027545256078,-0.877928921160667,
135.645557323121));
#241950=CARTESIAN_POINT('Ctrl Pts',(-201.035310009025,-0.742525690139992,
135.666236661027));
#241951=CARTESIAN_POINT('Ctrl Pts',(-201.04306704991,-0.607256943517217,
135.686895459924));
#241952=CARTESIAN_POINT('Ctrl Pts',(-201.050824090795,-0.470983987934914,
135.701926332662));
#241953=CARTESIAN_POINT('Ctrl Pts',(-201.05858113168,-0.33421407859659,
135.711241909402));
#241954=CARTESIAN_POINT('Ctrl Pts',(-201.066332322921,-0.197547308510626,
135.720550461193));
#241955=CARTESIAN_POINT('Ctrl Pts',(-201.074083514161,-0.0603847190823009,
135.724152269219));
#241956=CARTESIAN_POINT('Ctrl Pts',(-201.081834705401,0.076759602487468,
135.722011583823));
#241957=CARTESIAN_POINT('Ctrl Pts',(-201.089582602178,0.213845634062312,
135.719871808275));
#241958=CARTESIAN_POINT('Ctrl Pts',(-201.097330498955,0.350913023122092,
135.711994399786));
#241959=CARTESIAN_POINT('Ctrl Pts',(-201.105078395732,0.487446179389158,
135.698395689437));
#241960=CARTESIAN_POINT('Ctrl Pts',(-201.112824671816,0.623950775863247,
135.684799823644));
#241961=CARTESIAN_POINT('Ctrl Pts',(-201.1205709479,0.759920973027649,135.665485075162));
#241962=CARTESIAN_POINT('Ctrl Pts',(-201.128317223985,0.894845201367628,
135.640519747298));
#241963=CARTESIAN_POINT('Ctrl Pts',(-201.13606355725,1.02977042568743,135.615554235145));
#241964=CARTESIAN_POINT('Ctrl Pts',(-201.143809890515,1.16364928133632,
135.584938131512));
#241965=CARTESIAN_POINT('Ctrl Pts',(-201.151556223781,1.29597969885603,
135.548791003045));
#241966=CARTESIAN_POINT('Ctrl Pts',(-201.159304291784,1.42833975085505,
135.512635779679));
#241967=CARTESIAN_POINT('Ctrl Pts',(-201.167052359787,1.55915029763305,
135.470947169741));
#241968=CARTESIAN_POINT('Ctrl Pts',(-201.17480042779,1.68792413960081,135.423894702455));
#241969=CARTESIAN_POINT('Ctrl Pts',(-201.182556730532,1.81683484394041,
135.376792227247));
#241970=CARTESIAN_POINT('Ctrl Pts',(-201.190313033273,1.94370415157494,
135.324314641176));
#241971=CARTESIAN_POINT('Ctrl Pts',(-201.198069336015,2.06806406360551,
135.266679979885));
#241972=CARTESIAN_POINT('Ctrl Pts',(-201.205829778529,2.19249035026554,
135.209014557239));
#241973=CARTESIAN_POINT('Ctrl Pts',(-201.213590221043,2.31440422521268,
135.14618675382));
#241974=CARTESIAN_POINT('Ctrl Pts',(-201.221350663558,2.4333629419461,135.07846027191));
#241975=CARTESIAN_POINT('Ctrl Pts',(-201.229123563823,2.55251262177229,
135.010625069439));
#241976=CARTESIAN_POINT('Ctrl Pts',(-201.236896464089,2.66869733203954,
134.937875681717));
#241977=CARTESIAN_POINT('Ctrl Pts',(-201.244669364354,2.7815031842106,134.860519280479));
#241978=CARTESIAN_POINT('Ctrl Pts',(-201.252159700116,2.89020825951414,
134.785974979276));
#241979=CARTESIAN_POINT('Ctrl Pts',(-201.259650035878,2.99577562489767,
134.707152986653));
#241980=CARTESIAN_POINT('Ctrl Pts',(-201.26714037164,3.09786596784007,134.624361862042));
#241981=CARTESIAN_POINT('Ctrl Pts',(-201.274914705759,3.20382709716525,
134.538431686777));
#241982=CARTESIAN_POINT('Ctrl Pts',(-201.282689039878,3.30637798966232,
134.447953257853));
#241983=CARTESIAN_POINT('Ctrl Pts',(-201.290463373997,3.40510324293289,
134.353227333501));
#241984=CARTESIAN_POINT('Ctrl Pts',(-201.298228126944,3.50370682615185,
134.258618150384));
#241985=CARTESIAN_POINT('Ctrl Pts',(-201.305992879892,3.59849387170741,
134.159772155332));
#241986=CARTESIAN_POINT('Ctrl Pts',(-201.313757632839,3.68908073813156,
134.057031269514));
#241987=CARTESIAN_POINT('Ctrl Pts',(-201.321514673724,3.77957763240292,
133.954392427393));
#241988=CARTESIAN_POINT('Ctrl Pts',(-201.329271714609,3.86588239247803,
133.847866684276));
#241989=CARTESIAN_POINT('Ctrl Pts',(-201.337028755494,3.94764732780846,
133.737833582798));
#241990=CARTESIAN_POINT('Ctrl Pts',(-201.344779946734,4.02935060356523,
133.627883458138));
#241991=CARTESIAN_POINT('Ctrl Pts',(-201.352531137974,4.10652063663432,
133.514431552222));
#241992=CARTESIAN_POINT('Ctrl Pts',(-201.360282329214,4.1788494731278,133.397891057611));
#241993=CARTESIAN_POINT('Ctrl Pts',(-201.368030225991,4.25114756793644,
133.281400095818));
#241994=CARTESIAN_POINT('Ctrl Pts',(-201.375778122768,4.31860835291871,
133.161823487747));
#241995=CARTESIAN_POINT('Ctrl Pts',(-201.383526019545,4.38096687873627,
133.039603841449));
#241996=CARTESIAN_POINT('Ctrl Pts',(-201.39127229563,4.44331236049435,132.917409760867));
#241997=CARTESIAN_POINT('Ctrl Pts',(-201.399018571714,4.50055752839833,
132.792574089773));
#241998=CARTESIAN_POINT('Ctrl Pts',(-201.406764847798,4.55248333213625,
132.665564145695));
#241999=CARTESIAN_POINT('Ctrl Pts',(-201.414511181063,4.60440951917872,
132.538553264059));
#242000=CARTESIAN_POINT('Ctrl Pts',(-201.422257514328,4.65101611574979,
132.409368439302));
#242001=CARTESIAN_POINT('Ctrl Pts',(-201.430003847594,4.69213233585013,
132.278496705371));
#242002=CARTESIAN_POINT('Ctrl Pts',(-201.437751915597,4.73325776364294,
132.147595663623));
#242003=CARTESIAN_POINT('Ctrl Pts',(-201.4454999836,4.76889025117849,132.015007333899));
#242004=CARTESIAN_POINT('Ctrl Pts',(-201.453248051603,4.79890908491508,
131.881233245698));
#242005=CARTESIAN_POINT('Ctrl Pts',(-201.461004354345,4.82895982302535,
131.747316980804));
#242006=CARTESIAN_POINT('Ctrl Pts',(-201.468760657086,4.85338490335348,
131.612212822058));
#242007=CARTESIAN_POINT('Ctrl Pts',(-201.476516959828,4.87211480062235,
131.476432363778));
#242008=CARTESIAN_POINT('Ctrl Pts',(-201.484277402342,4.89085469460135,
131.340579435379));
#242009=CARTESIAN_POINT('Ctrl Pts',(-201.492037844857,4.90389331153006,
131.204049877203));
#242010=CARTESIAN_POINT('Ctrl Pts',(-201.499798287371,4.91121319630827,
131.067358721946));
#242011=CARTESIAN_POINT('Ctrl Pts',(-201.507571187636,4.91854483161535,
130.930448137912));
#242012=CARTESIAN_POINT('Ctrl Pts',(-201.515344087902,4.92013938522368,
130.793375829575));
#242013=CARTESIAN_POINT('Ctrl Pts',(-201.523116988167,4.91603157254995,
130.656656046912));
#242014=CARTESIAN_POINT('Ctrl Pts',(-201.530607323929,4.9120730892139,130.524906372726));
#242015=CARTESIAN_POINT('Ctrl Pts',(-201.538097659691,4.90281965408166,
130.39348434606));
#242016=CARTESIAN_POINT('Ctrl Pts',(-201.545587995453,4.88834746023548,
130.262842224056));
#242017=CARTESIAN_POINT('Ctrl Pts',(-201.553362329572,4.87332654876078,
130.127246766288));
#242018=CARTESIAN_POINT('Ctrl Pts',(-201.561136663691,4.8526357463644,129.992061995147));
#242019=CARTESIAN_POINT('Ctrl Pts',(-201.56891099781,4.82630355432022,129.857799967604));
#242020=CARTESIAN_POINT('Ctrl Pts',(-201.576675750757,4.80000381434937,
129.723703406011));
#242021=CARTESIAN_POINT('Ctrl Pts',(-201.584440503704,4.76807659267288,
129.590527705303));
#242022=CARTESIAN_POINT('Ctrl Pts',(-201.592205256651,4.73060218967124,
129.458780450657));
#242023=CARTESIAN_POINT('Ctrl Pts',(-201.599962297536,4.69316500677496,
129.327164049242));
#242024=CARTESIAN_POINT('Ctrl Pts',(-201.607719338421,4.65019171305585,
129.196973644122));
#242025=CARTESIAN_POINT('Ctrl Pts',(-201.615476379306,4.60181369324896,
129.068706909269));
#242026=CARTESIAN_POINT('Ctrl Pts',(-201.623227570546,4.5534721556832,128.940536901358));
#242027=CARTESIAN_POINT('Ctrl Pts',(-201.630978761786,4.49973414196849,
128.814288040604));
#242028=CARTESIAN_POINT('Ctrl Pts',(-201.638729953027,4.44078082610854,
128.690442758006));
#242029=CARTESIAN_POINT('Ctrl Pts',(-201.646477849804,4.38185256698038,
128.566650112956));
#242030=CARTESIAN_POINT('Ctrl Pts',(-201.654225746581,4.31771358212929,
128.445259366479));
#242031=CARTESIAN_POINT('Ctrl Pts',(-201.661973643358,4.24859303865466,
128.326732668419));
#242032=CARTESIAN_POINT('Ctrl Pts',(-201.669719919442,4.17948695370766,
128.208230763589));
#242033=CARTESIAN_POINT('Ctrl Pts',(-201.677466195526,4.10540157962988,
128.092592053057));
#242034=CARTESIAN_POINT('Ctrl Pts',(-201.68521247161,4.0266116818476,127.980253426592));
#242035=CARTESIAN_POINT('Ctrl Pts',(-201.692958804875,3.9478212024563,127.86791397087));
#242036=CARTESIAN_POINT('Ctrl Pts',(-201.700705138141,3.86432635455989,
127.758874967912));
#242037=CARTESIAN_POINT('Ctrl Pts',(-201.708451471406,3.77644457960803,
127.65354335856));
#242038=CARTESIAN_POINT('Ctrl Pts',(-201.716199539409,3.68854312414213,
127.548188160925));
#242039=CARTESIAN_POINT('Ctrl Pts',(-201.723947607412,3.59625303713412,
127.446542309132));
#242040=CARTESIAN_POINT('Ctrl Pts',(-201.731695675415,3.49993102093752,
127.348978451846));
#242041=CARTESIAN_POINT('Ctrl Pts',(-201.739451978156,3.40350663255572,
127.251310902531));
#242042=CARTESIAN_POINT('Ctrl Pts',(-201.747208280898,3.30304202998784,
127.157734292792));
#242043=CARTESIAN_POINT('Ctrl Pts',(-201.75496458364,3.19893005191173,127.068583645439));
#242044=CARTESIAN_POINT('Ctrl Pts',(-201.762725026154,3.09476250613789,
126.979385415701));
#242045=CARTESIAN_POINT('Ctrl Pts',(-201.770485468669,2.98694401306269,
126.894618096892));
#242046=CARTESIAN_POINT('Ctrl Pts',(-201.778245911183,2.87589844937092,
126.814574762234));
#242047=CARTESIAN_POINT('Ctrl Pts',(-201.786018811448,2.76467462548215,
126.73440293491));
#242048=CARTESIAN_POINT('Ctrl Pts',(-201.793791711714,2.65021370556392,
126.658970460966));
#242049=CARTESIAN_POINT('Ctrl Pts',(-201.801564611979,2.5329671072149,126.588526098011));
#242050=CARTESIAN_POINT('Ctrl Pts',(-201.809054947741,2.41998271804094,
126.520642565088));
#242051=CARTESIAN_POINT('Ctrl Pts',(-201.816545283503,2.3044119372224,126.45739092656));
#242052=CARTESIAN_POINT('Ctrl Pts',(-201.824035619265,2.18667644572457,
126.398951535061));
#242053=CARTESIAN_POINT('Ctrl Pts',(-201.831809953384,2.06447697728321,
126.338296396273));
#242054=CARTESIAN_POINT('Ctrl Pts',(-201.839584287503,1.93955831659402,
126.282633483449));
#242055=CARTESIAN_POINT('Ctrl Pts',(-201.847358621622,1.81236667732486,
126.232215596963));
#242056=CARTESIAN_POINT('Ctrl Pts',(-201.85512337457,1.68533179038399,126.181859846017));
#242057=CARTESIAN_POINT('Ctrl Pts',(-201.862888127517,1.55602985846499,
126.136736402609));
#242058=CARTESIAN_POINT('Ctrl Pts',(-201.870652880464,1.42493133167005,
126.097052069943));
#242059=CARTESIAN_POINT('Ctrl Pts',(-201.878409921349,1.29396301378008,
126.057407152316));
#242060=CARTESIAN_POINT('Ctrl Pts',(-201.886166962234,1.16120202383286,
126.023190707344));
#242061=CARTESIAN_POINT('Ctrl Pts',(-201.893924003119,1.02713808569387,
125.994561202266));
#242062=CARTESIAN_POINT('Ctrl Pts',(-201.901675194359,0.893175246212959,
125.965953286921));
#242063=CARTESIAN_POINT('Ctrl Pts',(-201.909426385599,0.757911795070179,
125.942924006762));
#242064=CARTESIAN_POINT('Ctrl Pts',(-201.917177576839,0.621851544102284,
125.925581700706));
#242065=CARTESIAN_POINT('Ctrl Pts',(-201.924925473616,0.485849122370762,
125.908246765593));
#242066=CARTESIAN_POINT('Ctrl Pts',(-201.932673370393,0.349050961400987,
125.896594046454));
#242067=CARTESIAN_POINT('Ctrl Pts',(-201.940421267171,0.211969751361186,
125.890680541797));
#242068=CARTESIAN_POINT('Ctrl Pts',(-201.948167543255,0.0749172157553973,
125.884768274118));
#242069=CARTESIAN_POINT('Ctrl Pts',(-201.955913819339,-0.0624178607984672,
125.884592849862));
#242070=CARTESIAN_POINT('Ctrl Pts',(-201.963660095423,-0.199519393139578,
125.890159250684));
#242071=CARTESIAN_POINT('Ctrl Pts',(-201.971406428688,-0.336621937532869,
125.895725692597));
#242072=CARTESIAN_POINT('Ctrl Pts',(-201.979152761954,-0.473490543629981,
125.907034028304));
#242073=CARTESIAN_POINT('Ctrl Pts',(-201.986899095219,-0.609611255716637,
125.92403714679));
#242074=CARTESIAN_POINT('Ctrl Pts',(-201.994647163222,-0.745762451093156,
125.941044073007));
#242075=CARTESIAN_POINT('Ctrl Pts',(-202.002395231225,-0.881165031306035,
125.963748271266));
#242076=CARTESIAN_POINT('Ctrl Pts',(-202.010143299228,-1.01531267014358,
125.99205106348));
#242077=CARTESIAN_POINT('Ctrl Pts',(-202.01789960197,-1.14960288268788,
126.020383936239));
#242078=CARTESIAN_POINT('Ctrl Pts',(-202.025655904712,-1.28263510636064,
126.054327208385));
#242079=CARTESIAN_POINT('Ctrl Pts',(-202.033412207453,-1.41391513808278,
126.093731461625));
#242080=CARTESIAN_POINT('Ctrl Pts',(-202.041172649968,-1.54526523791097,
126.133156746102));
#242081=CARTESIAN_POINT('Ctrl Pts',(-202.048933092482,-1.67486091308033,
126.178048691531));
#242082=CARTESIAN_POINT('Ctrl Pts',(-202.056693534996,-1.80222647708686,
126.228209091689));
#242083=CARTESIAN_POINT('Ctrl Pts',(-202.064466435261,-1.92979649960372,
126.278450013774));
#242084=CARTESIAN_POINT('Ctrl Pts',(-202.072239335527,-2.0551288993706,
126.333976132696));
#242085=CARTESIAN_POINT('Ctrl Pts',(-202.080012235792,-2.17777038732706,
126.394542117607));
#242086=CARTESIAN_POINT('Ctrl Pts',(-202.087502571554,-2.29595354828237,
126.452906376411));
#242087=CARTESIAN_POINT('Ctrl Pts',(-202.094992907316,-2.41163777316133,
126.515950291816));
#242088=CARTESIAN_POINT('Ctrl Pts',(-202.102483243079,-2.52444339732246,
126.583416576689));
#242089=CARTESIAN_POINT('Ctrl Pts',(-202.110258818857,-2.64154478059957,
126.653452050026));
#242090=CARTESIAN_POINT('Ctrl Pts',(-202.118034394636,-2.7559149798318,
126.728475270979));
#242091=CARTESIAN_POINT('Ctrl Pts',(-202.125809970415,-2.86709990176267,
126.808247353929));
#242092=CARTESIAN_POINT('Ctrl Pts',(-202.133891439779,-2.98265887332797,
126.891157695595));
#242093=CARTESIAN_POINT('Ctrl Pts',(-202.141972909144,-3.09477643568045,
126.979198038385));
#242094=CARTESIAN_POINT('Ctrl Pts',(-202.150054378508,-3.20297036422735,
127.072047138183));
#242095=CARTESIAN_POINT('Ctrl Pts',(-202.157810400925,-3.30680724058814,
127.161157133776));
#242096=CARTESIAN_POINT('Ctrl Pts',(-202.165566423341,-3.40702999075184,
127.254695853762));
#242097=CARTESIAN_POINT('Ctrl Pts',(-202.173322445758,-3.50324203012239,
127.352335365503));
#242098=CARTESIAN_POINT('Ctrl Pts',(-202.181073173471,-3.59938838965428,
127.44990822293));
#242099=CARTESIAN_POINT('Ctrl Pts',(-202.188823901183,-3.69152921254174,
127.551576025106));
#242100=CARTESIAN_POINT('Ctrl Pts',(-202.196574628896,-3.77930256283194,
127.65697198553));
#242101=CARTESIAN_POINT('Ctrl Pts',(-202.20432174412,-3.86703500338546,
127.762318822604));
#242102=CARTESIAN_POINT('Ctrl Pts',(-202.212068859344,-3.95040377296826,
127.871390059986));
#242103=CARTESIAN_POINT('Ctrl Pts',(-202.219815974568,-4.02908552554411,
127.983783922925));
#242104=CARTESIAN_POINT('Ctrl Pts',(-202.227561156713,-4.10774764526049,
128.096149741079));
#242105=CARTESIAN_POINT('Ctrl Pts',(-202.235306338858,-4.18172485302055,
128.211836213856));
#242106=CARTESIAN_POINT('Ctrl Pts',(-202.243051521003,-4.25073589056795,
128.330410850263));
#242107=CARTESIAN_POINT('Ctrl Pts',(-202.250798386813,-4.31976192988371,
128.449011262681));
#242108=CARTESIAN_POINT('Ctrl Pts',(-202.258545252622,-4.38381944209067,
128.570500757135));
#242109=CARTESIAN_POINT('Ctrl Pts',(-202.266292118432,-4.44267209747922,
128.694420405906));
#242110=CARTESIAN_POINT('Ctrl Pts',(-202.274040018994,-4.50153261384766,
128.818356606689));
#242111=CARTESIAN_POINT('Ctrl Pts',(-202.281787919557,-4.55518672851136,
128.944723251757));
#242112=CARTESIAN_POINT('Ctrl Pts',(-202.289535820119,-4.60344577788972,
129.07304030274));
#242113=CARTESIAN_POINT('Ctrl Pts',(-202.297288826251,-4.6517366281298,
129.201441909736));
#242114=CARTESIAN_POINT('Ctrl Pts',(-202.305041832382,-4.6946251865411,
129.331796119675));
#242115=CARTESIAN_POINT('Ctrl Pts',(-202.312794838514,-4.73197225875476,
129.463606499588));
#242116=CARTESIAN_POINT('Ctrl Pts',(-202.315118304061,-4.74316464453239,
129.503108193671));
#242117=CARTESIAN_POINT('Ctrl Pts',(-202.317441769608,-4.75385968611253,
129.542740584605));
#242118=CARTESIAN_POINT('Ctrl Pts',(-202.319765235154,-4.76405452823412,
129.582490119309));
#242119=CARTESIAN_POINT('Ctrl Pts',(-200.569853205643,-4.76405452823395,
129.582490119308));
#242120=CARTESIAN_POINT('Ctrl Pts',(-200.577513488277,-4.79778564433713,
129.714007229053));
#242121=CARTESIAN_POINT('Ctrl Pts',(-200.58517377091,-4.82606367990543,
129.846911054034));
#242122=CARTESIAN_POINT('Ctrl Pts',(-200.592834053543,-4.84879096813837,
129.980704615463));
#242123=CARTESIAN_POINT('Ctrl Pts',(-200.600671617285,-4.87204423159276,
130.117594547097));
#242124=CARTESIAN_POINT('Ctrl Pts',(-200.608509181027,-4.88948659380923,
130.255415469519));
#242125=CARTESIAN_POINT('Ctrl Pts',(-200.616346744769,-4.90106945198536,
130.393627992473));
#242126=CARTESIAN_POINT('Ctrl Pts',(-200.624184308511,-4.9126523101615,
130.531840515427));
#242127=CARTESIAN_POINT('Ctrl Pts',(-200.632021872253,-4.91837567036258,
130.670444191001));
#242128=CARTESIAN_POINT('Ctrl Pts',(-200.639859435995,-4.91824790596849,
130.808899112527));
#242129=CARTESIAN_POINT('Origin',(213.235140564004,0.,130.804360617566));
#242130=CARTESIAN_POINT('',(-198.820145221536,-4.76405452823399,129.582490119308));
#242131=CARTESIAN_POINT('',(-199.165100499421,-4.76405452823391,129.582490119308));
#242132=CARTESIAN_POINT('',(213.235140564004,-4.76405452823405,129.582490119308));
#242133=CARTESIAN_POINT('',(-199.235140563976,-4.91824791219353,130.808892361601));
#242134=CARTESIAN_POINT('Ctrl Pts',(-199.165100499421,-4.76405452823391,
129.582490119308));
#242135=CARTESIAN_POINT('Ctrl Pts',(-199.172747479307,-4.79772404353953,
129.713767048478));
#242136=CARTESIAN_POINT('Ctrl Pts',(-199.180394459193,-4.8259562660387,
129.846409655637));
#242137=CARTESIAN_POINT('Ctrl Pts',(-199.188041439078,-4.84865793162383,
129.979921823839));
#242138=CARTESIAN_POINT('Ctrl Pts',(-199.195891293228,-4.87196187206307,
130.116976067901));
#242139=CARTESIAN_POINT('Ctrl Pts',(-199.203741147378,-4.8894376250516,
130.254946212889));
#242140=CARTESIAN_POINT('Ctrl Pts',(-199.211591001527,-4.90104104578751,
130.393289176079));
#242141=CARTESIAN_POINT('Ctrl Pts',(-199.219440855677,-4.91264446652345,
130.53163213927));
#242142=CARTESIAN_POINT('Ctrl Pts',(-199.227290709826,-4.91837556944563,
130.67034746391));
#242143=CARTESIAN_POINT('Ctrl Pts',(-199.235140563976,-4.91824791219353,
130.808892361601));
#242144=CARTESIAN_POINT('Ctrl Pts',(-199.235140564013,-4.91824791219293,
130.80889236225));
#242145=CARTESIAN_POINT('Ctrl Pts',(-199.245686804809,-4.91807640527225,
130.995026757141));
#242146=CARTESIAN_POINT('Ctrl Pts',(-199.256233045605,-4.90733475277425,
131.180693350563));
#242147=CARTESIAN_POINT('Ctrl Pts',(-199.266779286401,-4.88620319730163,
131.364897304304));
#242148=CARTESIAN_POINT('Ctrl Pts',(-199.277325527197,-4.86507164182904,
131.549101258045));
#242149=CARTESIAN_POINT('Ctrl Pts',(-199.287871767993,-4.83355032983892,
131.731843197017));
#242150=CARTESIAN_POINT('Ctrl Pts',(-199.298418008789,-4.79186565731639,
131.912154183503));
#242151=CARTESIAN_POINT('Ctrl Pts',(-199.306192342908,-4.76113711829408,
132.045073380155));
#242152=CARTESIAN_POINT('Ctrl Pts',(-199.313966677027,-4.72482524621133,
132.176923596683));
#242153=CARTESIAN_POINT('Ctrl Pts',(-199.321741011146,-4.68301805246697,
132.307199591897));
#242154=CARTESIAN_POINT('Ctrl Pts',(-199.329505764093,-4.64126238235248,
132.43731503359));
#242155=CARTESIAN_POINT('Ctrl Pts',(-199.337270517041,-4.59402498413645,
132.565859745473));
#242156=CARTESIAN_POINT('Ctrl Pts',(-199.345035269988,-4.54144479361619,
132.692338967293));
#242157=CARTESIAN_POINT('Ctrl Pts',(-199.352792310873,-4.48891682648241,
132.818692568166));
#242158=CARTESIAN_POINT('Ctrl Pts',(-199.360549351758,-4.43105677640118,
132.942984402826));
#242159=CARTESIAN_POINT('Ctrl Pts',(-199.368306392643,-4.36805315947013,
133.064735510928));
#242160=CARTESIAN_POINT('Ctrl Pts',(-199.376057583883,-4.3050970540568,
133.186394805573));
#242161=CARTESIAN_POINT('Ctrl Pts',(-199.383808775123,-4.2370052812737,
133.305516841482));
#242162=CARTESIAN_POINT('Ctrl Pts',(-199.391559966363,-4.16401402959605,
133.421643602615));
#242163=CARTESIAN_POINT('Ctrl Pts',(-199.39930786314,-4.09105380114736,
133.537721006777));
#242164=CARTESIAN_POINT('Ctrl Pts',(-199.407055759917,-4.01319844317672,
133.650805337891));
#242165=CARTESIAN_POINT('Ctrl Pts',(-199.414803656695,-3.93072944517622,
133.76046431861));
#242166=CARTESIAN_POINT('Ctrl Pts',(-199.422549932779,-3.84827769791228,
133.870100361034));
#242167=CARTESIAN_POINT('Ctrl Pts',(-199.430296208863,-3.76121446504357,
133.976312165972));
#242168=CARTESIAN_POINT('Ctrl Pts',(-199.438042484947,-3.66986357811492,
134.078697860509));
#242169=CARTESIAN_POINT('Ctrl Pts',(-199.445788818212,-3.57851201685465,
134.181084310835));
#242170=CARTESIAN_POINT('Ctrl Pts',(-199.453535151478,-3.48287299866424,
134.279644302673));
#242171=CARTESIAN_POINT('Ctrl Pts',(-199.461281484743,-3.38330924806213,
134.374010683676));
#242172=CARTESIAN_POINT('Ctrl Pts',(-199.469029552746,-3.28372320084826,
134.468398197375));
#242173=CARTESIAN_POINT('Ctrl Pts',(-199.476777620749,-3.18021095598737,
134.558589962581));
#242174=CARTESIAN_POINT('Ctrl Pts',(-199.484525688752,-3.07317023273365,
134.644257462943));
#242175=CARTESIAN_POINT('Ctrl Pts',(-199.492281991494,-2.9660157453259,
134.730016011745));
#242176=CARTESIAN_POINT('Ctrl Pts',(-199.500038294236,-2.85532559400969,
134.811240445636));
#242177=CARTESIAN_POINT('Ctrl Pts',(-199.507794596978,-2.74152900080911,
134.887643830891));
#242178=CARTESIAN_POINT('Ctrl Pts',(-199.515555039492,-2.62767167094008,
134.964087994933));
#242179=CARTESIAN_POINT('Ctrl Pts',(-199.523315482006,-2.51070492874323,
135.035705779087));
#242180=CARTESIAN_POINT('Ctrl Pts',(-199.53107592452,-2.39108393133343,
135.102255532035));
#242181=CARTESIAN_POINT('Ctrl Pts',(-199.538848824786,-2.27127090767914,
135.168912116555));
#242182=CARTESIAN_POINT('Ctrl Pts',(-199.546621725051,-2.14879546379233,
135.230484236534));
#242183=CARTESIAN_POINT('Ctrl Pts',(-199.554394625317,-2.02413494276591,
135.286777465202));
#242184=CARTESIAN_POINT('Ctrl Pts',(-199.561884961079,-1.90400614567938,
135.341024293215));
#242185=CARTESIAN_POINT('Ctrl Pts',(-199.569375296841,-1.781848665018,135.390369253178));
#242186=CARTESIAN_POINT('Ctrl Pts',(-199.576865632603,-1.65810233422333,
135.43468238951));
#242187=CARTESIAN_POINT('Ctrl Pts',(-199.584639966722,-1.52966412368488,
135.480675671875));
#242188=CARTESIAN_POINT('Ctrl Pts',(-199.592414300841,-1.39910734850033,
135.52139372814));
#242189=CARTESIAN_POINT('Ctrl Pts',(-199.60018863496,-1.26690465470224,
135.556637509582));
#242190=CARTESIAN_POINT('Ctrl Pts',(-199.607953387907,-1.13486488890897,
135.591837856214));
#242191=CARTESIAN_POINT('Ctrl Pts',(-199.615718140854,-1.00118361465327,
135.621577251914));
#242192=CARTESIAN_POINT('Ctrl Pts',(-199.623482893801,-0.866352185939986,
135.645705157301));
#242193=CARTESIAN_POINT('Ctrl Pts',(-199.631239934686,-0.731654673702493,
135.669809098511));
#242194=CARTESIAN_POINT('Ctrl Pts',(-199.638996975571,-0.595809662696144,
135.688312572326));
#242195=CARTESIAN_POINT('Ctrl Pts',(-199.646754016456,-0.459322013378897,
135.701115292912));
#242196=CARTESIAN_POINT('Ctrl Pts',(-199.654505207696,-0.322937290459533,
135.713908358867));
#242197=CARTESIAN_POINT('Ctrl Pts',(-199.662256398937,-0.185911281514558,
135.721009192091));
#242198=CARTESIAN_POINT('Ctrl Pts',(-199.670007590177,-0.0487569940496048,
135.722368935781));
#242199=CARTESIAN_POINT('Ctrl Pts',(-199.677755486954,0.0883389991842788,
135.723728101544));
#242200=CARTESIAN_POINT('Ctrl Pts',(-199.685503383731,0.225562772370937,
135.719351027109));
#242201=CARTESIAN_POINT('Ctrl Pts',(-199.693251280508,0.362398486389647,
135.709240881096));
#242202=CARTESIAN_POINT('Ctrl Pts',(-199.700997556592,0.499205577326821,
135.699132849906));
#242203=CARTESIAN_POINT('Ctrl Pts',(-199.708743832676,0.635624380899426,
135.683294161272));
#242204=CARTESIAN_POINT('Ctrl Pts',(-199.71649010876,0.771141751181498,
135.661780041713));
#242205=CARTESIAN_POINT('Ctrl Pts',(-199.724236442026,0.906660121822196,
135.640265763343));
#242206=CARTESIAN_POINT('Ctrl Pts',(-199.731982775291,1.04127665976482,
135.613076031752));
#242207=CARTESIAN_POINT('Ctrl Pts',(-199.739729108556,1.17448640787711,
135.580317562536));
#242208=CARTESIAN_POINT('Ctrl Pts',(-199.747477176559,1.3077259873887,135.547551757289));
#242209=CARTESIAN_POINT('Ctrl Pts',(-199.755225244562,1.43955777059391,
135.509214826219));
#242210=CARTESIAN_POINT('Ctrl Pts',(-199.762973312565,1.56949039041183,
135.465463810685));
#242211=CARTESIAN_POINT('Ctrl Pts',(-199.770729615307,1.69956110416447,
135.421666296052));
#242212=CARTESIAN_POINT('Ctrl Pts',(-199.778485918049,1.82772825133692,
135.372443327376));
#242213=CARTESIAN_POINT('Ctrl Pts',(-199.786242220791,1.95351842146964,
135.318000926616));
#242214=CARTESIAN_POINT('Ctrl Pts',(-199.794002663305,2.07937572960363,
135.263529468307));
#242215=CARTESIAN_POINT('Ctrl Pts',(-199.801763105819,2.20285318096146,
135.203833197122));
#242216=CARTESIAN_POINT('Ctrl Pts',(-199.809523548333,2.32350144390913,
135.139164431195));
#242217=CARTESIAN_POINT('Ctrl Pts',(-199.817296448599,2.44434338215913,
135.074391853224));
#242218=CARTESIAN_POINT('Ctrl Pts',(-199.825069348864,2.56234671955976,
135.004631028427));
#242219=CARTESIAN_POINT('Ctrl Pts',(-199.83284224913,2.67708986376302,134.930178466652));
#242220=CARTESIAN_POINT('Ctrl Pts',(-199.840332584892,2.78766180565022,
134.858432443034));
#242221=CARTESIAN_POINT('Ctrl Pts',(-199.847822920653,2.89520622014493,
134.782330051055));
#242222=CARTESIAN_POINT('Ctrl Pts',(-199.855313256415,2.99937603121739,
134.702171090878));
#242223=CARTESIAN_POINT('Ctrl Pts',(-199.863087590534,3.1074954723416,134.618972879359));
#242224=CARTESIAN_POINT('Ctrl Pts',(-199.870861924653,3.21232185228549,
134.531140870842));
#242225=CARTESIAN_POINT('Ctrl Pts',(-199.878636258772,3.31343222899665,
134.438965125122));
#242226=CARTESIAN_POINT('Ctrl Pts',(-199.886401011719,3.414417996205,134.346902977771));
#242227=CARTESIAN_POINT('Ctrl Pts',(-199.894165764666,3.51169658615192,
134.25050800549));
#242228=CARTESIAN_POINT('Ctrl Pts',(-199.901930517614,3.60487575695146,
134.150112228108));
#242229=CARTESIAN_POINT('Ctrl Pts',(-199.909687558499,3.69796238088497,
134.049816165227));
#242230=CARTESIAN_POINT('Ctrl Pts',(-199.917444599384,3.78695742409865,
133.945527489707));
#242231=CARTESIAN_POINT('Ctrl Pts',(-199.925201640269,3.87150362387128,
133.837616748006));
#242232=CARTESIAN_POINT('Ctrl Pts',(-199.932952831509,3.95598606669709,
133.729787382635));
#242233=CARTESIAN_POINT('Ctrl Pts',(-199.940704022749,4.03602610367543,
133.618341694337));
#242234=CARTESIAN_POINT('Ctrl Pts',(-199.948455213989,4.11130533710608,
133.50368488256));
#242235=CARTESIAN_POINT('Ctrl Pts',(-199.956203110766,4.18655257485428,
133.389076802986));
#242236=CARTESIAN_POINT('Ctrl Pts',(-199.963951007543,4.25704281945193,
133.271260640578));
#242237=CARTESIAN_POINT('Ctrl Pts',(-199.97169890432,4.32249991310147,133.150672098111));
#242238=CARTESIAN_POINT('Ctrl Pts',(-199.979445180404,4.38794331453812,
133.030108780168));
#242239=CARTESIAN_POINT('Ctrl Pts',(-199.987191456488,4.44835547276005,
132.906774579053));
#242240=CARTESIAN_POINT('Ctrl Pts',(-199.994937732572,4.50350548349756,
132.781131070251));
#242241=CARTESIAN_POINT('Ctrl Pts',(-200.002684065838,4.55865590134,132.655486633977));
#242242=CARTESIAN_POINT('Ctrl Pts',(-200.010430399103,4.60854393704874,
132.527533213996));
#242243=CARTESIAN_POINT('Ctrl Pts',(-200.018176732369,4.65298643181374,
132.397753327433));
#242244=CARTESIAN_POINT('Ctrl Pts',(-200.025924800372,4.69743887916725,
132.267944377564));
#242245=CARTESIAN_POINT('Ctrl Pts',(-200.033672868375,4.73644323229192,
132.136308517008));
#242246=CARTESIAN_POINT('Ctrl Pts',(-200.041420936378,4.76986601862287,
132.003344031499));
#242247=CARTESIAN_POINT('Ctrl Pts',(-200.04917723912,4.80332432708882,131.870238229753));
#242248=CARTESIAN_POINT('Ctrl Pts',(-200.056933541861,4.83118912317878,
131.735801362048));
#242249=CARTESIAN_POINT('Ctrl Pts',(-200.064689844603,4.85337784908269,
131.600543081913));
#242250=CARTESIAN_POINT('Ctrl Pts',(-200.072450287117,4.87557841777776,
131.465212610361));
#242251=CARTESIAN_POINT('Ctrl Pts',(-200.080210729631,4.89209683270756,
131.329060240733));
#242252=CARTESIAN_POINT('Ctrl Pts',(-200.087971172146,4.90290250153954,
131.192600392573));
#242253=CARTESIAN_POINT('Ctrl Pts',(-200.095744072411,4.9137255165904,131.05592148695));
#242254=CARTESIAN_POINT('Ctrl Pts',(-200.103516972676,4.91881744521724,
130.918934507362));
#242255=CARTESIAN_POINT('Ctrl Pts',(-200.111289872942,4.91819986858887,
130.782154422205));
#242256=CARTESIAN_POINT('Ctrl Pts',(-200.118780208704,4.91760474242652,
130.650346637671));
#242257=CARTESIAN_POINT('Ctrl Pts',(-200.126270544466,4.91170802767491,
130.518731274167));
#242258=CARTESIAN_POINT('Ctrl Pts',(-200.133760880228,4.90057435163176,
130.387762385898));
#242259=CARTESIAN_POINT('Ctrl Pts',(-200.141535214347,4.88901853887747,
130.251827772423));
#242260=CARTESIAN_POINT('Ctrl Pts',(-200.149309548466,4.87178420146617,
130.116159024119));
#242261=CARTESIAN_POINT('Ctrl Pts',(-200.157083882586,4.8488867644099,129.981268758518));
#242262=CARTESIAN_POINT('Ctrl Pts',(-200.164848635533,4.8260175463984,129.846544733114));
#242263=CARTESIAN_POINT('Ctrl Pts',(-200.17261338848,4.79749918019917,129.712597663223));
#242264=CARTESIAN_POINT('Ctrl Pts',(-200.180378141427,4.76339898717628,
129.57993701788));
#242265=CARTESIAN_POINT('Ctrl Pts',(-200.188135182312,4.72933266294583,
129.44740813296));
#242266=CARTESIAN_POINT('Ctrl Pts',(-200.195892223197,4.68969564130355,
129.316163506122));
#242267=CARTESIAN_POINT('Ctrl Pts',(-200.203649264082,4.64460656425249,
129.186704002025));
#242268=CARTESIAN_POINT('Ctrl Pts',(-200.211400455322,4.59955148922512,
129.057342124347));
#242269=CARTESIAN_POINT('Ctrl Pts',(-200.219151646562,4.5490526704274,128.929763057648));
#242270=CARTESIAN_POINT('Ctrl Pts',(-200.226902837802,4.49327891189645,
128.80445369913));
#242271=CARTESIAN_POINT('Ctrl Pts',(-200.23465073458,4.43752885870062,128.679197600433));
#242272=CARTESIAN_POINT('Ctrl Pts',(-200.242398631357,4.37650848356419,
128.556209647663));
#242273=CARTESIAN_POINT('Ctrl Pts',(-200.250146528134,4.31043508553766,
128.435957688192));
#242274=CARTESIAN_POINT('Ctrl Pts',(-200.257892804218,4.2443755086418,128.315730882839));
#242275=CARTESIAN_POINT('Ctrl Pts',(-200.265639080302,4.17326519940549,
128.198239274858));
#242276=CARTESIAN_POINT('Ctrl Pts',(-200.273385356386,4.09736768495884,
128.083926623374));
#242277=CARTESIAN_POINT('Ctrl Pts',(-200.281131689651,4.02146961025387,
127.96961312806));
#242278=CARTESIAN_POINT('Ctrl Pts',(-200.288878022917,3.94078447607879,
127.85847896178));
#242279=CARTESIAN_POINT('Ctrl Pts',(-200.296624356182,3.85561923594436,
127.75093903352));
#242280=CARTESIAN_POINT('Ctrl Pts',(-200.304372424185,3.770434923645,127.643375022439));
#242281=CARTESIAN_POINT('Ctrl Pts',(-200.312120492188,3.68076875163644,
127.53940715748));
#242282=CARTESIAN_POINT('Ctrl Pts',(-200.319868560191,3.58696779663645,
127.439417068501));
#242283=CARTESIAN_POINT('Ctrl Pts',(-200.327624862933,3.49306714886511,
127.339320708866));
#242284=CARTESIAN_POINT('Ctrl Pts',(-200.335381165675,3.39502320753719,
127.243210855946));
#242285=CARTESIAN_POINT('Ctrl Pts',(-200.343137468417,3.29322013408638,
127.151432448145));
#242286=CARTESIAN_POINT('Ctrl Pts',(-200.350897910931,3.19136272527004,
127.059605055445));
#242287=CARTESIAN_POINT('Ctrl Pts',(-200.358658353445,3.08574248742091,
126.972113963648));
#242288=CARTESIAN_POINT('Ctrl Pts',(-200.366418795959,2.97677568036702,
126.88926296728));
#242289=CARTESIAN_POINT('Ctrl Pts',(-200.374191696225,2.86763395012082,
126.806278971137));
#242290=CARTESIAN_POINT('Ctrl Pts',(-200.38196459649,2.75513523632046,126.727950178812));
#242291=CARTESIAN_POINT('Ctrl Pts',(-200.389737496756,2.63972446161173,
126.654536786454));
#242292=CARTESIAN_POINT('Ctrl Pts',(-200.397227832518,2.52850915926618,
126.583792155825));
#242293=CARTESIAN_POINT('Ctrl Pts',(-200.40471816828,2.41459010805134,126.517611910091));
#242294=CARTESIAN_POINT('Ctrl Pts',(-200.412208504042,2.29838424926308,
126.456187103866));
#242295=CARTESIAN_POINT('Ctrl Pts',(-200.419982838161,2.17777241001932,
126.392433357444));
#242296=CARTESIAN_POINT('Ctrl Pts',(-200.42775717228,2.05431486939034,126.333600821259));
#242297=CARTESIAN_POINT('Ctrl Pts',(-200.435531506399,1.92845124462011,
126.279953600108));
#242298=CARTESIAN_POINT('Ctrl Pts',(-200.443296259346,1.8027427355183,126.226372494363));
#242299=CARTESIAN_POINT('Ctrl Pts',(-200.451061012293,1.67463439851077,
126.177964140413));
#242300=CARTESIAN_POINT('Ctrl Pts',(-200.45882576524,1.54459125316685,126.134947279347));
#242301=CARTESIAN_POINT('Ctrl Pts',(-200.466582806125,1.41467726850817,
126.091973143233));
#242302=CARTESIAN_POINT('Ctrl Pts',(-200.47433984701,1.28283266852345,126.054379965485));
#242303=CARTESIAN_POINT('Ctrl Pts',(-200.482096887895,1.14954297373518,
126.022338658809));
#242304=CARTESIAN_POINT('Ctrl Pts',(-200.489848079135,1.01635379374277,
125.990321514731));
#242305=CARTESIAN_POINT('Ctrl Pts',(-200.497599270375,0.881722066640452,
125.963847999343));
#242306=CARTESIAN_POINT('Ctrl Pts',(-200.505350461615,0.746148675539075,
125.94303927286));
#242307=CARTESIAN_POINT('Ctrl Pts',(-200.513098358392,0.61063290674527,
125.922239390641));
#242308=CARTESIAN_POINT('Ctrl Pts',(-200.520846255169,0.474176655614721,
125.90709956781));
#242309=CARTESIAN_POINT('Ctrl Pts',(-200.528594151946,0.337290990834222,
125.897689867454));
#242310=CARTESIAN_POINT('Ctrl Pts',(-200.53634042803,0.200433959583882,
125.888282135405));
#242311=CARTESIAN_POINT('Ctrl Pts',(-200.544086704114,0.0631480831462334,
125.884602168507));
#242312=CARTESIAN_POINT('Ctrl Pts',(-200.551832980198,-0.0740508485073515,
125.886668116572));
#242313=CARTESIAN_POINT('Ctrl Pts',(-200.559579313464,-0.211250792932096,
125.888734079886));
#242314=CARTESIAN_POINT('Ctrl Pts',(-200.567325646729,-0.348363400371211,
125.896546036912));
#242315=CARTESIAN_POINT('Ctrl Pts',(-200.575071979994,-0.484873680273991,
125.910070007408));
#242316=CARTESIAN_POINT('Ctrl Pts',(-200.582820047997,-0.621414530707646,
125.923597006504));
#242317=CARTESIAN_POINT('Ctrl Pts',(-200.590568116,-0.757352396209157,125.942838525925));
#242318=CARTESIAN_POINT('Ctrl Pts',(-200.598316184003,-0.892178597326069,
125.967708840461));
#242319=CARTESIAN_POINT('Ctrl Pts',(-200.606072486745,-1.0271480933338,
125.992605587463));
#242320=CARTESIAN_POINT('Ctrl Pts',(-200.613828789487,-1.16100317971131,
126.023143008933));
#242321=CARTESIAN_POINT('Ctrl Pts',(-200.621585092229,-1.29324600137144,
126.059184346611));
#242322=CARTESIAN_POINT('Ctrl Pts',(-200.629345534743,-1.42555940500761,
126.095244920636));
#242323=CARTESIAN_POINT('Ctrl Pts',(-200.637105977257,-1.55625845688736,
126.136815145853));
#242324=CARTESIAN_POINT('Ctrl Pts',(-200.644866419771,-1.68486256746866,
126.183709019442));
#242325=CARTESIAN_POINT('Ctrl Pts',(-200.652639320036,-1.8136731247852,
126.23067817124));
#242326=CARTESIAN_POINT('Ctrl Pts',(-200.660412220302,-1.94038165889755,
126.28298789975));
#242327=CARTESIAN_POINT('Ctrl Pts',(-200.668185120567,-2.06452876785875,
126.340404521323));
#242328=CARTESIAN_POINT('Ctrl Pts',(-200.675675456329,-2.18416281670689,
126.395733904081));
#242329=CARTESIAN_POINT('Ctrl Pts',(-200.683165792092,-2.30141816157879,
126.455805188864));
#242330=CARTESIAN_POINT('Ctrl Pts',(-200.690656127854,-2.41590869586259,
126.520370860837));
#242331=CARTESIAN_POINT('Ctrl Pts',(-200.698431549059,-2.53475678976688,
126.587393930419));
#242332=CARTESIAN_POINT('Ctrl Pts',(-200.706206970264,-2.65100197297227,
126.659472618184));
#242333=CARTESIAN_POINT('Ctrl Pts',(-200.713982391469,-2.7641842313008,
126.736379718161));
#242334=CARTESIAN_POINT('Ctrl Pts',(-200.721747993784,-2.87722356178429,
126.813189698976));
#242335=CARTESIAN_POINT('Ctrl Pts',(-200.729513596099,-2.98720734372281,
126.894815740927));
#242336=CARTESIAN_POINT('Ctrl Pts',(-200.737279198413,-3.09370005168907,
126.980984746339));
#242337=CARTESIAN_POINT('Ctrl Pts',(-200.745035419852,-3.20006411607945,
127.067049659281));
#242338=CARTESIAN_POINT('Ctrl Pts',(-200.752791641291,-3.30294520389971,
127.15764636104));
#242339=CARTESIAN_POINT('Ctrl Pts',(-200.76054786273,-3.40193722042223,
127.252458843754));
#242340=CARTESIAN_POINT('Ctrl Pts',(-200.768298765275,-3.50086135232833,
127.347206308003));
#242341=CARTESIAN_POINT('Ctrl Pts',(-200.776049667819,-3.5959014377128,
127.446163532372));
#242342=CARTESIAN_POINT('Ctrl Pts',(-200.783800570363,-3.68668484751337,
127.548974634673));
#242343=CARTESIAN_POINT('Ctrl Pts',(-200.791547836284,-3.77742566291104,
127.651737499334));
#242344=CARTESIAN_POINT('Ctrl Pts',(-200.799295102205,-3.86391351900049,
127.758350351215));
#242345=CARTESIAN_POINT('Ctrl Pts',(-200.807042368126,-3.94581330905367,
127.868421178035));
#242346=CARTESIAN_POINT('Ctrl Pts',(-200.814787676884,-4.0276924090674,
127.97846419807));
#242347=CARTESIAN_POINT('Ctrl Pts',(-200.822532985642,-4.10498551777313,
128.091963140353));
#242348=CARTESIAN_POINT('Ctrl Pts',(-200.8302782944,-4.17739867669816,128.208494026537));
#242349=CARTESIAN_POINT('Ctrl Pts',(-200.838025646966,-4.24983094378865,
128.325055662539));
#242350=CARTESIAN_POINT('Ctrl Pts',(-200.845772999533,-4.31738047721026,
128.444650511683));
#242351=CARTESIAN_POINT('Ctrl Pts',(-200.8535203521,-4.37979740039574,128.566826753244));
#242352=CARTESIAN_POINT('Ctrl Pts',(-200.861268696023,-4.4422223104952,
128.689018628564));
#242353=CARTESIAN_POINT('Ctrl Pts',(-200.869017039946,-4.49951313147677,
128.813792202435));
#242354=CARTESIAN_POINT('Ctrl Pts',(-200.87676538387,-4.55146701346846,
128.940673120208));
#242355=CARTESIAN_POINT('Ctrl Pts',(-200.884519834436,-4.60346184147747,
129.067654035672));
#242356=CARTESIAN_POINT('Ctrl Pts',(-200.892274285003,-4.65011118842505,
129.19674524743));
#242357=CARTESIAN_POINT('Ctrl Pts',(-200.90002873557,-4.69126111778874,
129.327454328317));
#242358=CARTESIAN_POINT('Ctrl Pts',(-200.905034844876,-4.71782664201108,
129.411837346905));
#242359=CARTESIAN_POINT('Ctrl Pts',(-200.910040954183,-4.74210117247926,
129.496894318409));
#242360=CARTESIAN_POINT('Ctrl Pts',(-200.91504706349,-4.76405452823395,
129.582490119308));
#242361=CARTESIAN_POINT('',(-198.889859435951,-4.91824989448309,130.8033418354));
#242362=CARTESIAN_POINT('Ctrl Pts',(-198.889859435995,-4.91824989448325,
130.803341836187));
#242363=CARTESIAN_POINT('Ctrl Pts',(-198.897858632837,-4.91827931260921,
130.945360229872));
#242364=CARTESIAN_POINT('Ctrl Pts',(-198.905857829679,-4.91215304597155,
131.087301810736));
#242365=CARTESIAN_POINT('Ctrl Pts',(-198.913857026521,-4.89991714960293,
131.228618781338));
#242366=CARTESIAN_POINT('Ctrl Pts',(-198.921862893465,-4.88767105037535,
131.370053588597));
#242367=CARTESIAN_POINT('Ctrl Pts',(-198.929868760409,-4.86930519372858,
131.510862395327));
#242368=CARTESIAN_POINT('Ctrl Pts',(-198.937874627353,-4.84491724488214,
131.650504785391));
#242369=CARTESIAN_POINT('Ctrl Pts',(-198.945888336214,-4.82050540752001,
131.790283958152));
#242370=CARTESIAN_POINT('Ctrl Pts',(-198.953902045075,-4.79005977639878,
131.928894088689));
#242371=CARTESIAN_POINT('Ctrl Pts',(-198.961915753937,-4.75372862315488,
132.065807104698));
#242372=CARTESIAN_POINT('Ctrl Pts',(-198.969944216913,-4.71733058028216,
132.202972192552));
#242373=CARTESIAN_POINT('Ctrl Pts',(-198.977972679889,-4.67502545496002,
132.338433581101));
#242374=CARTESIAN_POINT('Ctrl Pts',(-198.986001142865,-4.62701107698537,
132.471679290152));
#242375=CARTESIAN_POINT('Ctrl Pts',(-198.994038134277,-4.57894569453759,
132.605066542788));
#242376=CARTESIAN_POINT('Ctrl Pts',(-199.002075125689,-4.52515909597119,
132.736233095487));
#242377=CARTESIAN_POINT('Ctrl Pts',(-199.0101121171,-4.46589624387441,132.864689183948));
#242378=CARTESIAN_POINT('Ctrl Pts',(-199.018163714144,-4.40652569334159,
132.993378715777));
#242379=CARTESIAN_POINT('Ctrl Pts',(-199.026215311188,-4.34165916726409,
133.119347629071));
#242380=CARTESIAN_POINT('Ctrl Pts',(-199.034266908231,-4.27158681882194,
133.242131958723));
#242381=CARTESIAN_POINT('Ctrl Pts',(-199.036031065866,-4.25623350843576,
133.269034809357));
#242382=CARTESIAN_POINT('Ctrl Pts',(-199.037795223501,-4.2406304385508,
133.295784893293));
#242383=CARTESIAN_POINT('Ctrl Pts',(-199.039559381137,-4.2247809262074,
133.322377533326));
#242384=CARTESIAN_POINT('Ctrl Pts',(-199.047333715256,-4.15493489763892,
133.439566646481));
#242385=CARTESIAN_POINT('Ctrl Pts',(-199.055108049375,-4.08009856624961,
133.554033039613));
#242386=CARTESIAN_POINT('Ctrl Pts',(-199.062882383494,-4.00051000845862,
133.665322472384));
#242387=CARTESIAN_POINT('Ctrl Pts',(-199.070647136441,-3.92101953645207,
133.776474750875));
#242388=CARTESIAN_POINT('Ctrl Pts',(-199.078411889388,-3.83678871636238,
133.884457544366));
#242389=CARTESIAN_POINT('Ctrl Pts',(-199.086176642335,-3.74810091690515,
133.988842141958));
#242390=CARTESIAN_POINT('Ctrl Pts',(-199.09393368322,-3.65950120342062,
134.093123063297));
#242391=CARTESIAN_POINT('Ctrl Pts',(-199.101690724105,-3.56645357147556,
134.193812604699));
#242392=CARTESIAN_POINT('Ctrl Pts',(-199.10944776499,-3.46928377810122,
134.290512239269));
#242393=CARTESIAN_POINT('Ctrl Pts',(-199.11719895623,-3.37218726122407,
134.387138951893));
#242394=CARTESIAN_POINT('Ctrl Pts',(-199.12495014747,-3.27097504630834,
134.47978147189));
#242395=CARTESIAN_POINT('Ctrl Pts',(-199.132701338711,-3.16601189112494,
134.568075772537));
#242396=CARTESIAN_POINT('Ctrl Pts',(-199.140449235488,-3.06109334808233,
134.65633254575));
#242397=CARTESIAN_POINT('Ctrl Pts',(-199.148197132265,-2.95242733417478,
134.740244524213));
#242398=CARTESIAN_POINT('Ctrl Pts',(-199.155945029042,-2.84041388590054,
134.819486022741));
#242399=CARTESIAN_POINT('Ctrl Pts',(-199.163691305126,-2.72842386842495,
134.898710945656));
#242400=CARTESIAN_POINT('Ctrl Pts',(-199.17143758121,-2.61308812831208,
134.973267106223));
#242401=CARTESIAN_POINT('Ctrl Pts',(-199.179183857294,-2.49483773851418,
135.042870700247));
#242402=CARTESIAN_POINT('Ctrl Pts',(-199.186930190559,-2.3765864758186,
135.112474808069));
#242403=CARTESIAN_POINT('Ctrl Pts',(-199.194676523825,-2.25542085743659,
135.177126078077));
#242404=CARTESIAN_POINT('Ctrl Pts',(-199.20242285709,-2.13179839053741,
135.236585643961));
#242405=CARTESIAN_POINT('Ctrl Pts',(-199.210170925093,-2.0081482392444,
135.296058525402));
#242406=CARTESIAN_POINT('Ctrl Pts',(-199.217918993096,-1.88204049687381,
135.350337219758));
#242407=CARTESIAN_POINT('Ctrl Pts',(-199.225667061099,-1.75395419721453,
135.399230336783));
#242408=CARTESIAN_POINT('Ctrl Pts',(-199.233423363841,-1.6257317659112,
135.448175417994));
#242409=CARTESIAN_POINT('Ctrl Pts',(-199.241179666583,-1.49552694252251,
135.491723348206));
#242410=CARTESIAN_POINT('Ctrl Pts',(-199.248935969325,-1.3638360625422,
135.529731952923));
#242411=CARTESIAN_POINT('Ctrl Pts',(-199.256696411839,-1.23207489517375,
135.567760843976));
#242412=CARTESIAN_POINT('Ctrl Pts',(-199.264456854353,-1.0988264704442,
135.600244425895));
#242413=CARTESIAN_POINT('Ctrl Pts',(-199.272217296867,-0.96459799408161,
135.627091563028));
#242414=CARTESIAN_POINT('Ctrl Pts',(-199.279990197133,-0.830154042252889,
135.653981797568));
#242415=CARTESIAN_POINT('Ctrl Pts',(-199.287763097398,-0.694727281372439,
135.675217445693));
#242416=CARTESIAN_POINT('Ctrl Pts',(-199.295535997664,-0.558831624326638,
135.690759115248));
#242417=CARTESIAN_POINT('Ctrl Pts',(-199.303026333426,-0.427876116714585,
135.705735805968));
#242418=CARTESIAN_POINT('Ctrl Pts',(-199.310516669188,-0.296485519363162,
135.715425289075));
#242419=CARTESIAN_POINT('Ctrl Pts',(-199.31800700495,-0.16511834145049,
135.719838111749));
#242420=CARTESIAN_POINT('Ctrl Pts',(-199.325781339069,-0.0287703370596385,
135.724418247935));
#242421=CARTESIAN_POINT('Ctrl Pts',(-199.333555673188,0.10798434643372,
135.723328204347));
#242422=CARTESIAN_POINT('Ctrl Pts',(-199.341330007307,0.244634857648935,
135.716522753421));
#242423=CARTESIAN_POINT('Ctrl Pts',(-199.349094760254,0.381116959321885,
135.709725689604));
#242424=CARTESIAN_POINT('Ctrl Pts',(-199.356859513201,0.517494757427955,
135.69722725263));
#242425=CARTESIAN_POINT('Ctrl Pts',(-199.364624266149,0.653254397634356,
135.679034119912));
#242426=CARTESIAN_POINT('Ctrl Pts',(-199.372381307034,0.788879199452228,
135.660859056869));
#242427=CARTESIAN_POINT('Ctrl Pts',(-199.380138347918,0.923886680191096,
135.637000605475));
#242428=CARTESIAN_POINT('Ctrl Pts',(-199.387895388803,1.05776546825392,
135.607517420823));
#242429=CARTESIAN_POINT('Ctrl Pts',(-199.395646580044,1.19154329728142,
135.578056469669));
#242430=CARTESIAN_POINT('Ctrl Pts',(-199.403397771284,1.32419374753591,
135.542979311759));
#242431=CARTESIAN_POINT('Ctrl Pts',(-199.411148962524,1.45521339253885,
135.5023960628));
#242432=CARTESIAN_POINT('Ctrl Pts',(-199.418896859301,1.58617735069778,
135.461830062804));
#242433=CARTESIAN_POINT('Ctrl Pts',(-199.426644756078,1.71551150952141,
135.415762741745));
#242434=CARTESIAN_POINT('Ctrl Pts',(-199.434392652855,1.84272563134234,
135.364354620862));
#242435=CARTESIAN_POINT('Ctrl Pts',(-199.442138928939,1.96991314271106,
135.312957253449));
#242436=CARTESIAN_POINT('Ctrl Pts',(-199.449885205023,2.09498113689857,
135.256221454736));
#242437=CARTESIAN_POINT('Ctrl Pts',(-199.457631481108,2.21745783593928,
135.194356495506));
#242438=CARTESIAN_POINT('Ctrl Pts',(-199.465377814373,2.33993543907532,
135.132491079603));
#242439=CARTESIAN_POINT('Ctrl Pts',(-199.473124147638,2.45982135992249,
135.065496603904));
#242440=CARTESIAN_POINT('Ctrl Pts',(-199.480870480904,2.57666733968873,
134.993628869073));
#242441=CARTESIAN_POINT('Ctrl Pts',(-199.488618548907,2.69353948630213,
134.92174503996));
#242442=CARTESIAN_POINT('Ctrl Pts',(-199.49636661691,2.80737000422098,134.844985984877));
#242443=CARTESIAN_POINT('Ctrl Pts',(-199.504114684913,2.91773894194668,
134.763651277413));
#242444=CARTESIAN_POINT('Ctrl Pts',(-199.511870987655,3.02822518109265,
134.682230126454));
#242445=CARTESIAN_POINT('Ctrl Pts',(-199.519627290396,3.13524217559271,
134.596223840941));
#242446=CARTESIAN_POINT('Ctrl Pts',(-199.527383593138,3.23840202855827,
134.505973153196));
#242447=CARTESIAN_POINT('Ctrl Pts',(-199.535144035652,3.34161694104344,
134.41567429594));
#242448=CARTESIAN_POINT('Ctrl Pts',(-199.542904478166,3.44097032683412,
134.321126791907));
#242449=CARTESIAN_POINT('Ctrl Pts',(-199.550664920681,3.5361113538409,134.222708106593));
#242450=CARTESIAN_POINT('Ctrl Pts',(-199.558437820946,3.63140510967045,
134.124131430869));
#242451=CARTESIAN_POINT('Ctrl Pts',(-199.566210721212,3.72247273410093,
134.021671447976));
#242452=CARTESIAN_POINT('Ctrl Pts',(-199.573983621477,3.80900330292975,
133.915739234959));
#242453=CARTESIAN_POINT('Ctrl Pts',(-199.581473957239,3.89238826762382,
133.813657924713));
#242454=CARTESIAN_POINT('Ctrl Pts',(-199.588964293001,3.97156013144357,
133.708352696285));
#242455=CARTESIAN_POINT('Ctrl Pts',(-199.596454628763,4.04627993261936,
133.600215007441));
#242456=CARTESIAN_POINT('Ctrl Pts',(-199.604228962882,4.12383275776765,
133.487977245255));
#242457=CARTESIAN_POINT('Ctrl Pts',(-199.612003297001,4.1968349200723,133.372332461753));
#242458=CARTESIAN_POINT('Ctrl Pts',(-199.61977763112,4.26497224065351,133.253686004066));
#242459=CARTESIAN_POINT('Ctrl Pts',(-199.627542384067,4.33302558807671,
133.135185767535));
#242460=CARTESIAN_POINT('Ctrl Pts',(-199.635307137014,4.39622583016546,
133.013691553092));
#242461=CARTESIAN_POINT('Ctrl Pts',(-199.643071889961,4.45430083399845,
132.889639290248));
#242462=CARTESIAN_POINT('Ctrl Pts',(-199.650828930846,4.51231815691907,
132.765710237859));
#242463=CARTESIAN_POINT('Ctrl Pts',(-199.658585971731,4.56522020713492,
132.639228544949));
#242464=CARTESIAN_POINT('Ctrl Pts',(-199.666343012616,4.61277992399897,
132.510656147435));
#242465=CARTESIAN_POINT('Ctrl Pts',(-199.674094203857,4.66030377571063,
132.382180707367));
#242466=CARTESIAN_POINT('Ctrl Pts',(-199.681845395097,4.70249317785453,
132.251618066054));
#242467=CARTESIAN_POINT('Ctrl Pts',(-199.689596586337,4.73916865958453,
132.11945129068));
#242468=CARTESIAN_POINT('Ctrl Pts',(-199.697344483114,4.77582855325628,
131.987340689712));
#242469=CARTESIAN_POINT('Ctrl Pts',(-199.705092379891,4.80697908336153,
131.853627686671));
#242470=CARTESIAN_POINT('Ctrl Pts',(-199.712840276668,4.83249031553063,
131.718811498042));
#242471=CARTESIAN_POINT('Ctrl Pts',(-199.720586552752,4.85799621129998,
131.584023510052));
#242472=CARTESIAN_POINT('Ctrl Pts',(-199.728332828836,4.87786508281496,
131.448133179379));
#242473=CARTESIAN_POINT('Ctrl Pts',(-199.73607910492,4.89201798799939,131.311650542156));
#242474=CARTESIAN_POINT('Ctrl Pts',(-199.743825438185,4.9061709976573,131.17516689745));
#242475=CARTESIAN_POINT('Ctrl Pts',(-199.751571771451,4.91460791646383,
131.038091326349));
#242476=CARTESIAN_POINT('Ctrl Pts',(-199.759318104716,4.91730166193535,
130.900939228179));
#242477=CARTESIAN_POINT('Ctrl Pts',(-199.767066172719,4.91999601065249,
130.763756415746));
#242478=CARTESIAN_POINT('Ctrl Pts',(-199.774814240722,4.91694461908141,
130.626497432957));
#242479=CARTESIAN_POINT('Ctrl Pts',(-199.782562308725,4.90817253292527,
130.489677523743));
#242480=CARTESIAN_POINT('Ctrl Pts',(-199.790318611467,4.89939112369156,
130.352712200701));
#242481=CARTESIAN_POINT('Ctrl Pts',(-199.798074914209,4.88487689942825,
130.21618727421));
#242482=CARTESIAN_POINT('Ctrl Pts',(-199.805831216951,4.8647068601427,130.080613267049));
#242483=CARTESIAN_POINT('Ctrl Pts',(-199.813591659465,4.84452605549987,
129.944966899958));
#242484=CARTESIAN_POINT('Ctrl Pts',(-199.821352101979,4.81868349449313,
129.810272847277));
#242485=CARTESIAN_POINT('Ctrl Pts',(-199.829112544493,4.78730711622281,
129.6770303033));
#242486=CARTESIAN_POINT('Ctrl Pts',(-199.836885444758,4.75588036980463,
129.543573866563));
#242487=CARTESIAN_POINT('Ctrl Pts',(-199.844658345024,4.71890215983434,
129.411573971483));
#242488=CARTESIAN_POINT('Ctrl Pts',(-199.852431245289,4.67655027494581,
129.281514404581));
#242489=CARTESIAN_POINT('Ctrl Pts',(-199.859921581051,4.63573798775117,
129.156182830536));
#242490=CARTESIAN_POINT('Ctrl Pts',(-199.867411916813,4.58993604295062,
129.032653251052));
#242491=CARTESIAN_POINT('Ctrl Pts',(-199.874902252575,4.53934462037534,
128.911338303918));
#242492=CARTESIAN_POINT('Ctrl Pts',(-199.882676586694,4.48683500863597,
128.78542366369));
#242493=CARTESIAN_POINT('Ctrl Pts',(-199.890450920813,4.42899922894786,
128.66149604675));
#242494=CARTESIAN_POINT('Ctrl Pts',(-199.898225254932,4.36600848997413,
128.540038880715));
#242495=CARTESIAN_POINT('Ctrl Pts',(-199.905990007879,4.30309538145654,
128.418731399783));
#242496=CARTESIAN_POINT('Ctrl Pts',(-199.913754760827,4.23504013255191,
128.299888655622));
#242497=CARTESIAN_POINT('Ctrl Pts',(-199.921519513774,4.16206240861067,
128.183975231916));
#242498=CARTESIAN_POINT('Ctrl Pts',(-199.929276554659,4.08915716717364,
128.068176935055));
#242499=CARTESIAN_POINT('Ctrl Pts',(-199.937033595544,4.01133938712683,
127.95530249744));
#242500=CARTESIAN_POINT('Ctrl Pts',(-199.944790636429,3.9288749764153,127.84579263927));
#242501=CARTESIAN_POINT('Ctrl Pts',(-199.952541827669,3.84647275275725,
127.736365363336));
#242502=CARTESIAN_POINT('Ctrl Pts',(-199.960293018909,3.75943110728714,
127.630297927647));
#242503=CARTESIAN_POINT('Ctrl Pts',(-199.968044210149,3.6680594497312,127.528002435722));
#242504=CARTESIAN_POINT('Ctrl Pts',(-199.975792106926,3.57672662756702,
127.425750422109));
#242505=CARTESIAN_POINT('Ctrl Pts',(-199.983540003703,3.48106771357534,
127.327267454637));
#242506=CARTESIAN_POINT('Ctrl Pts',(-199.99128790048,3.38143248002231,127.232932689475));
#242507=CARTESIAN_POINT('Ctrl Pts',(-199.999034176564,3.2818180880128,127.138617657112));
#242508=CARTESIAN_POINT('Ctrl Pts',(-200.006780452648,3.17822931458165,
127.048449369756));
#242509=CARTESIAN_POINT('Ctrl Pts',(-200.014526728732,3.07105259745354,
126.962769930601));
#242510=CARTESIAN_POINT('Ctrl Pts',(-200.022273061998,2.9638750891711,126.87708985898));
#242511=CARTESIAN_POINT('Ctrl Pts',(-200.030019395263,2.85310988972064,
126.795898945805));
#242512=CARTESIAN_POINT('Ctrl Pts',(-200.037765728529,2.73917598040633,
126.719498562262));
#242513=CARTESIAN_POINT('Ctrl Pts',(-200.045513796531,2.62521655638345,
126.643081069382));
#242514=CARTESIAN_POINT('Ctrl Pts',(-200.053261864534,2.50808733510855,
126.571456458597));
#242515=CARTESIAN_POINT('Ctrl Pts',(-200.061009932537,2.38823534370891,
126.504882160176));
#242516=CARTESIAN_POINT('Ctrl Pts',(-200.068766235279,2.26825597218606,
126.438237105799));
#242517=CARTESIAN_POINT('Ctrl Pts',(-200.076522538021,2.14554839219856,
126.37665327616));
#242518=CARTESIAN_POINT('Ctrl Pts',(-200.084278840763,2.02058374140458,
126.320341839007));
#242519=CARTESIAN_POINT('Ctrl Pts',(-200.092039283277,1.89555239321386,
126.264000346744));
#242520=CARTESIAN_POINT('Ctrl Pts',(-200.099799725791,1.76826193649607,
126.212936999659));
#242521=CARTESIAN_POINT('Ctrl Pts',(-200.107560168305,1.63920151175827,
126.167313985673));
#242522=CARTESIAN_POINT('Ctrl Pts',(-200.115333068571,1.50993390776888,
126.121617733575));
#242523=CARTESIAN_POINT('Ctrl Pts',(-200.123105968836,1.37889103187466,
126.081379381333));
#242524=CARTESIAN_POINT('Ctrl Pts',(-200.130878869102,1.24657600647687,
126.046710848765));
#242525=CARTESIAN_POINT('Ctrl Pts',(-200.138369204864,1.11907096553192,
126.01330260468));
#242526=CARTESIAN_POINT('Ctrl Pts',(-200.145859540626,0.99038496183093,
125.985066322929));
#242527=CARTESIAN_POINT('Ctrl Pts',(-200.153349876388,0.860973361320397,
125.962056627357));
#242528=CARTESIAN_POINT('Ctrl Pts',(-200.161124210507,0.726655080644413,
125.938174512183));
#242529=CARTESIAN_POINT('Ctrl Pts',(-200.168898544626,0.591129615061729,
125.919847487573));
#242530=CARTESIAN_POINT('Ctrl Pts',(-200.176672878745,0.454896228380958,
125.907192815264));
#242531=CARTESIAN_POINT('Ctrl Pts',(-200.184437631692,0.318830737174114,
125.894553738707));
#242532=CARTESIAN_POINT('Ctrl Pts',(-200.19220238464,0.182059446335804,
125.887573140922));
#242533=CARTESIAN_POINT('Ctrl Pts',(-200.199967137587,0.0450919577624086,
125.886317330054));
#242534=CARTESIAN_POINT('Ctrl Pts',(-200.207724178472,-0.0917394927708051,
125.885062766475));
#242535=CARTESIAN_POINT('Ctrl Pts',(-200.215481219357,-0.228766364827308,
125.8895216781));
#242536=CARTESIAN_POINT('Ctrl Pts',(-200.223238260242,-0.365474138281122,
125.899708569077));
#242537=CARTESIAN_POINT('Ctrl Pts',(-200.230989451482,-0.502078819338985,
125.90988777804));
#242538=CARTESIAN_POINT('Ctrl Pts',(-200.238740642722,-0.638364492456307,
125.925786339691));
#242539=CARTESIAN_POINT('Ctrl Pts',(-200.246491833962,-0.773817199757398,
125.947366690881));
#242540=CARTESIAN_POINT('Ctrl Pts',(-200.254239730739,-0.909212336044752,
125.968937869845));
#242541=CARTESIAN_POINT('Ctrl Pts',(-200.261987627516,-1.04377482537243,
125.996185973889));
#242542=CARTESIAN_POINT('Ctrl Pts',(-200.269735524293,-1.17699661246376,
126.029021672868));
#242543=CARTESIAN_POINT('Ctrl Pts',(-200.277481800377,-1.31019053242917,
126.061850503327));
#242544=CARTESIAN_POINT('Ctrl Pts',(-200.285228076462,-1.44204392861639,
126.100264510403));
#242545=CARTESIAN_POINT('Ctrl Pts',(-200.292974352546,-1.57206010089031,
126.144123488225));
#242546=CARTESIAN_POINT('Ctrl Pts',(-200.300720685811,-1.70207723291426,
126.187982789804));
#242547=CARTESIAN_POINT('Ctrl Pts',(-200.308467019076,-1.83025674350794,
126.237287017366));
#242548=CARTESIAN_POINT('Ctrl Pts',(-200.316213352342,-1.9561186109295,
126.29184656856));
#242549=CARTESIAN_POINT('Ctrl Pts',(-200.323961420345,-2.08200866424412,
126.346418337987));
#242550=CARTESIAN_POINT('Ctrl Pts',(-200.331709488348,-2.20557968295316,
126.40624761746));
#242551=CARTESIAN_POINT('Ctrl Pts',(-200.339457556351,-2.32637345459673,
126.471097457747));
#242552=CARTESIAN_POINT('Ctrl Pts',(-200.347213859093,-2.44729560729777,
126.536016221215));
#242553=CARTESIAN_POINT('Ctrl Pts',(-200.354970161835,-2.56543427159992,
126.605966019329));
#242554=CARTESIAN_POINT('Ctrl Pts',(-200.362726464576,-2.68035712468567,
126.68066461196));
#242555=CARTESIAN_POINT('Ctrl Pts',(-200.370486907091,-2.79534131555868,
126.75540307348));
#242556=CARTESIAN_POINT('Ctrl Pts',(-200.378247349605,-2.90710595674912,
126.834895153379));
#242557=CARTESIAN_POINT('Ctrl Pts',(-200.386007792119,-3.01525020257337,
126.918816990429));
#242558=CARTESIAN_POINT('Ctrl Pts',(-200.393780692384,-3.12356805114131,
127.002873546263));
#242559=CARTESIAN_POINT('Ctrl Pts',(-200.40155359265,-3.22825359181314,
127.091373816816));
#242560=CARTESIAN_POINT('Ctrl Pts',(-200.409326492915,-3.32894071332805,
127.183955006361));
#242561=CARTESIAN_POINT('Ctrl Pts',(-200.416816828677,-3.42596760435925,
127.273170636466));
#242562=CARTESIAN_POINT('Ctrl Pts',(-200.424307164439,-3.51928151621706,
127.366175415959));
#242563=CARTESIAN_POINT('Ctrl Pts',(-200.431797500201,-3.60859035589865,
127.462615758093));
#242564=CARTESIAN_POINT('Ctrl Pts',(-200.439483530572,-3.70023250333136,
127.561575727608));
#242565=CARTESIAN_POINT('Ctrl Pts',(-200.447169560944,-3.78796263802236,
127.664483128439));
#242566=CARTESIAN_POINT('Ctrl Pts',(-200.454855591315,-3.87141551944836,
127.770992038202));
#242567=CARTESIAN_POINT('Ctrl Pts',(-200.462532485089,-3.95476919812291,
127.877374337873));
#242568=CARTESIAN_POINT('Ctrl Pts',(-200.470209378863,-4.03385548881044,
127.987349321958));
#242569=CARTESIAN_POINT('Ctrl Pts',(-200.477886272637,-4.10834596593192,
128.100534349717));
#242570=CARTESIAN_POINT('Ctrl Pts',(-200.48555463187,-4.18275363065011,
128.213593547645));
#242571=CARTESIAN_POINT('Ctrl Pts',(-200.493222991104,-4.25257543216279,
128.329855354119));
#242572=CARTESIAN_POINT('Ctrl Pts',(-200.500891350337,-4.3175236951057,
128.44890477958));
#242573=CARTESIAN_POINT('Ctrl Pts',(-200.508554665913,-4.38242924007743,
128.567875903488));
#242574=CARTESIAN_POINT('Ctrl Pts',(-200.516217981489,-4.44246742915597,
128.689630650553));
#242575=CARTESIAN_POINT('Ctrl Pts',(-200.523881297066,-4.49739444895502,
128.813725986849));
#242576=CARTESIAN_POINT('Ctrl Pts',(-200.531543281829,-4.55231193011296,
128.937799772716));
#242577=CARTESIAN_POINT('Ctrl Pts',(-200.539205266592,-4.60211982992361,
129.064212980692));
#242578=CARTESIAN_POINT('Ctrl Pts',(-200.546867251355,-4.64662086241272,
129.192499077765));
#242579=CARTESIAN_POINT('Ctrl Pts',(-200.554529236118,-4.69112189490171,
129.320785174837));
#242580=CARTESIAN_POINT('Ctrl Pts',(-200.56219122088,-4.73031591701161,
129.450943786207));
#242581=CARTESIAN_POINT('Ctrl Pts',(-200.569853205643,-4.76405452823395,
129.582490119308));
#242582=CARTESIAN_POINT('Ctrl Pts',(-198.820145221536,-4.76405452823399,
129.582490119308));
#242583=CARTESIAN_POINT('Ctrl Pts',(-198.828426476198,-4.80034991023985,
129.72400526289));
#242584=CARTESIAN_POINT('Ctrl Pts',(-198.836707730859,-4.83037656394087,
129.867298369273));
#242585=CARTESIAN_POINT('Ctrl Pts',(-198.844988985521,-4.85397223469977,
130.011809920598));
#242586=CARTESIAN_POINT('Ctrl Pts',(-198.853248087719,-4.87750478673457,
130.155934901657));
#242587=CARTESIAN_POINT('Ctrl Pts',(-198.861507189918,-4.89464061291577,
130.301271527841));
#242588=CARTESIAN_POINT('Ctrl Pts',(-198.869766292116,-4.90526800462946,
130.44724877898));
#242589=CARTESIAN_POINT('Ctrl Pts',(-198.876464006728,-4.91388628238558,
130.5656289545));
#242590=CARTESIAN_POINT('Ctrl Pts',(-198.883161721339,-4.91822526271462,
130.684430063471));
#242591=CARTESIAN_POINT('Ctrl Pts',(-198.889859435951,-4.91824989448309,
130.803341835399));
#242592=CARTESIAN_POINT('Origin',(213.235140564004,0.,130.804360617566));
#242593=CARTESIAN_POINT('',(-197.069830899744,-4.76405452823391,129.582490119308));
#242594=CARTESIAN_POINT('',(-197.415422870675,-4.76405452823413,129.582490119309));
#242595=CARTESIAN_POINT('',(213.235140564004,-4.76405452823405,129.582490119308));
#242596=CARTESIAN_POINT('',(-197.485140563979,-4.91824998893204,130.804030662974));
#242597=CARTESIAN_POINT('Ctrl Pts',(-197.415422870675,-4.76405452823413,
129.582490119309));
#242598=CARTESIAN_POINT('Ctrl Pts',(-197.423600431488,-4.79992281658223,
129.722340031201));
#242599=CARTESIAN_POINT('Ctrl Pts',(-197.431777992302,-4.82966733555782,
129.863920110019));
#242600=CARTESIAN_POINT('Ctrl Pts',(-197.439955553115,-4.85313234200592,
130.006683030144));
#242601=CARTESIAN_POINT('Ctrl Pts',(-197.448116021641,-4.87654830318953,
130.149147555073));
#242602=CARTESIAN_POINT('Ctrl Pts',(-197.456276490167,-4.89371087298272,
130.292789672346));
#242603=CARTESIAN_POINT('Ctrl Pts',(-197.464436958693,-4.90451488430555,
130.437050377952));
#242604=CARTESIAN_POINT('Ctrl Pts',(-197.471338160455,-4.91365169572061,
130.559049774504));
#242605=CARTESIAN_POINT('Ctrl Pts',(-197.478239362217,-4.91824176802981,
130.681491218841));
#242606=CARTESIAN_POINT('Ctrl Pts',(-197.485140563979,-4.91824998893204,
130.804030662974));
#242607=CARTESIAN_POINT('Ctrl Pts',(-197.485140564012,-4.91824998893207,
130.804030663556));
#242608=CARTESIAN_POINT('Ctrl Pts',(-197.493215691151,-4.91825960822969,
130.947414616808));
#242609=CARTESIAN_POINT('Ctrl Pts',(-197.501290818289,-4.91199470079414,
131.0906909398));
#242610=CARTESIAN_POINT('Ctrl Pts',(-197.509365945428,-4.8995093582954,
131.233302467326));
#242611=CARTESIAN_POINT('Ctrl Pts',(-197.517450328902,-4.88700970413012,
131.37607746723));
#242612=CARTESIAN_POINT('Ctrl Pts',(-197.525534712377,-4.86827541990526,
131.518185812766));
#242613=CARTESIAN_POINT('Ctrl Pts',(-197.533619095851,-4.84341207736157,
131.659078413899));
#242614=CARTESIAN_POINT('Ctrl Pts',(-197.541721259799,-4.81849405136742,
131.800280888636));
#242615=CARTESIAN_POINT('Ctrl Pts',(-197.549823423746,-4.78742007700962,
131.940261937201));
#242616=CARTESIAN_POINT('Ctrl Pts',(-197.557925587693,-4.75034662328381,
132.078483853818));
#242617=CARTESIAN_POINT('Ctrl Pts',(-197.566036944332,-4.71323110612685,
132.216862596612));
#242618=CARTESIAN_POINT('Ctrl Pts',(-197.57414830097,-4.67010262962301,
132.353477900727));
#242619=CARTESIAN_POINT('Ctrl Pts',(-197.582259657609,-4.62116662589813,
132.487810075728));
#242620=CARTESIAN_POINT('Ctrl Pts',(-197.590389437885,-4.57211947193716,
132.622447364588));
#242621=CARTESIAN_POINT('Ctrl Pts',(-197.598519218162,-4.51723854412096,
132.754790839472));
#242622=CARTESIAN_POINT('Ctrl Pts',(-197.606648998438,-4.45677700646237,
132.884341813916));
#242623=CARTESIAN_POINT('Ctrl Pts',(-197.613676754263,-4.40451127368774,
132.996331632124));
#242624=CARTESIAN_POINT('Ctrl Pts',(-197.620704510087,-4.34807614872925,
133.106234993745));
#242625=CARTESIAN_POINT('Ctrl Pts',(-197.627732265912,-4.28766139771813,
133.213747012692));
#242626=CARTESIAN_POINT('Ctrl Pts',(-197.635506600031,-4.22082861755148,
133.332680336215));
#242627=CARTESIAN_POINT('Ctrl Pts',(-197.64328093415,-4.14893767964865,
133.449019171949));
#242628=CARTESIAN_POINT('Ctrl Pts',(-197.651055268269,-4.0722149913182,
133.562303352103));
#242629=CARTESIAN_POINT('Ctrl Pts',(-197.658820021216,-3.99558685684443,
133.675447919629));
#242630=CARTESIAN_POINT('Ctrl Pts',(-197.666584774163,-3.91413903715416,
133.785545001383));
#242631=CARTESIAN_POINT('Ctrl Pts',(-197.67434952711,-3.82814386857856,
133.892158794903));
#242632=CARTESIAN_POINT('Ctrl Pts',(-197.682106567995,-3.74223411161671,
133.9986666981));
#242633=CARTESIAN_POINT('Ctrl Pts',(-197.68986360888,-3.65178623765968,
134.101697895584));
#242634=CARTESIAN_POINT('Ctrl Pts',(-197.697620649765,-3.55711572780408,
134.200845677375));
#242635=CARTESIAN_POINT('Ctrl Pts',(-197.705371841005,-3.46251660971625,
134.299918691053));
#242636=CARTESIAN_POINT('Ctrl Pts',(-197.713123032246,-3.36370146283428,
134.395113836446));
#242637=CARTESIAN_POINT('Ctrl Pts',(-197.720874223486,-3.26102563669002,
134.486057897266));
#242638=CARTESIAN_POINT('Ctrl Pts',(-197.728622120263,-3.15839345051069,
134.576963304434));
#242639=CARTESIAN_POINT('Ctrl Pts',(-197.73637001704,-3.05190414073299,
134.663620961979));
#242640=CARTESIAN_POINT('Ctrl Pts',(-197.744117913817,-2.94194930255022,
134.745695082405));
#242641=CARTESIAN_POINT('Ctrl Pts',(-197.751864189901,-2.83201746454923,
134.827752034693));
#242642=CARTESIAN_POINT('Ctrl Pts',(-197.759610465985,-2.71862185314553,
134.905227123207));
#242643=CARTESIAN_POINT('Ctrl Pts',(-197.767356742069,-2.6021861586238,
134.977825635793));
#242644=CARTESIAN_POINT('Ctrl Pts',(-197.775103075335,-2.48574960460007,
135.050424684285));
#242645=CARTESIAN_POINT('Ctrl Pts',(-197.7828494086,-2.3662732544387,135.118146878164));
#242646=CARTESIAN_POINT('Ctrl Pts',(-197.790595741865,-2.24420837078515,
135.180741753961));
#242647=CARTESIAN_POINT('Ctrl Pts',(-197.798343809868,-2.12211615154708,
135.243350647447));
#242648=CARTESIAN_POINT('Ctrl Pts',(-197.806091877871,-1.9974345931365,
135.300829759648));
#242649=CARTESIAN_POINT('Ctrl Pts',(-197.813839945874,-1.87063768933132,
135.352975538369));
#242650=CARTESIAN_POINT('Ctrl Pts',(-197.821596248616,-1.74370602426839,
135.405176738244));
#242651=CARTESIAN_POINT('Ctrl Pts',(-197.829352551358,-1.61465488491918,
135.452033132601));
#242652=CARTESIAN_POINT('Ctrl Pts',(-197.8371088541,-1.48397681704943,135.493389927451));
#242653=CARTESIAN_POINT('Ctrl Pts',(-197.844869296614,-1.35322900236022,
135.534768795668));
#242654=CARTESIAN_POINT('Ctrl Pts',(-197.852629739128,-1.22085290607787,
135.57064211333));
#242655=CARTESIAN_POINT('Ctrl Pts',(-197.860390181642,-1.08735324310278,
135.600905831281));
#242656=CARTESIAN_POINT('Ctrl Pts',(-197.868163081908,-0.953639274617129,
135.631218131239));
#242657=CARTESIAN_POINT('Ctrl Pts',(-197.875935982173,-0.818798519968866,
135.65590276613));
#242658=CARTESIAN_POINT('Ctrl Pts',(-197.883708882439,-0.683343719454388,
135.674907242287));
#242659=CARTESIAN_POINT('Ctrl Pts',(-197.891199218201,-0.55281304212647,
135.693220857867));
#242660=CARTESIAN_POINT('Ctrl Pts',(-197.898689553963,-0.421712494577103,
135.706260090511));
#242661=CARTESIAN_POINT('Ctrl Pts',(-197.906179889725,-0.290500705819022,
135.714023783448));
#242662=CARTESIAN_POINT('Ctrl Pts',(-197.913954223844,-0.154313982210954,
135.722081839163));
#242663=CARTESIAN_POINT('Ctrl Pts',(-197.921728557963,-0.0175760168504587,
135.724481939496));
#242664=CARTESIAN_POINT('Ctrl Pts',(-197.929502892082,0.119203659386324,
135.721165835397));
#242665=CARTESIAN_POINT('Ctrl Pts',(-197.937267645029,0.255814766896124,
135.7178538181));
#242666=CARTESIAN_POINT('Ctrl Pts',(-197.945032397976,0.392467095903496,
135.708839622631));
#242667=CARTESIAN_POINT('Ctrl Pts',(-197.952797150924,0.528646789015383,
135.694116811382));
#242668=CARTESIAN_POINT('Ctrl Pts',(-197.960554191809,0.664691226536644,
135.679408623037));
#242669=CARTESIAN_POINT('Ctrl Pts',(-197.968311232694,0.800263576161697,
135.659003143977));
#242670=CARTESIAN_POINT('Ctrl Pts',(-197.976068273579,0.93485113602674,
135.632945960704));
#242671=CARTESIAN_POINT('Ctrl Pts',(-197.983819464819,1.0693372023654,135.606908427356));
#242672=CARTESIAN_POINT('Ctrl Pts',(-197.991570656059,1.20283957483479,
135.575227747049));
#242673=CARTESIAN_POINT('Ctrl Pts',(-197.999321847299,1.33485218089917,
135.538001152889));
#242674=CARTESIAN_POINT('Ctrl Pts',(-198.007069744076,1.46680867808496,
135.500790381023));
#242675=CARTESIAN_POINT('Ctrl Pts',(-198.014817640853,1.59727629273097,
135.458038489407));
#242676=CARTESIAN_POINT('Ctrl Pts',(-198.02256553763,1.72576085053872,135.409893436822));
#242677=CARTESIAN_POINT('Ctrl Pts',(-198.030311813714,1.85421853214679,
135.361758455145));
#242678=CARTESIAN_POINT('Ctrl Pts',(-198.038058089798,1.98069361612735,
135.308232693516));
#242679=CARTESIAN_POINT('Ctrl Pts',(-198.045804365883,2.1047091378518,135.249513315454));
#242680=CARTESIAN_POINT('Ctrl Pts',(-198.053550699148,2.22872557503048,
135.19079350394));
#242681=CARTESIAN_POINT('Ctrl Pts',(-198.061297032413,2.35028206036682,
135.126880166801));
#242682=CARTESIAN_POINT('Ctrl Pts',(-198.069043365679,2.46892395336895,
135.058017582459));
#242683=CARTESIAN_POINT('Ctrl Pts',(-198.076791433682,2.58759241540058,
134.989139576819));
#242684=CARTESIAN_POINT('Ctrl Pts',(-198.084539501685,2.70334464822494,
134.915310314712));
#242685=CARTESIAN_POINT('Ctrl Pts',(-198.092287569688,2.8157531924012,134.836818555596));
#242686=CARTESIAN_POINT('Ctrl Pts',(-198.10004387243,2.92828120571605,134.758243374504));
#242687=CARTESIAN_POINT('Ctrl Pts',(-198.107800175171,3.03745811039781,
134.674996021732));
#242688=CARTESIAN_POINT('Ctrl Pts',(-198.115556477913,3.14288744086359,
134.587407220049));
#242689=CARTESIAN_POINT('Ctrl Pts',(-198.123316920427,3.24837304213745,
134.499771669587));
#242690=CARTESIAN_POINT('Ctrl Pts',(-198.131077362942,3.35010679377825,
134.407790315149));
#242691=CARTESIAN_POINT('Ctrl Pts',(-198.138837805456,3.44772834555247,
134.311831546565));
#242692=CARTESIAN_POINT('Ctrl Pts',(-198.146610705722,3.54550660810803,
134.215718736448));
#242693=CARTESIAN_POINT('Ctrl Pts',(-198.154383605987,3.6391592121027,134.115616038787));
#242694=CARTESIAN_POINT('Ctrl Pts',(-198.162156506252,3.7283648444739,134.011926462407));
#242695=CARTESIAN_POINT('Ctrl Pts',(-198.169646842014,3.81432762741104,
133.912006263309));
#242696=CARTESIAN_POINT('Ctrl Pts',(-198.177137177776,3.89616095138074,
133.808755683444));
#242697=CARTESIAN_POINT('Ctrl Pts',(-198.184627513538,3.97361594297526,
133.702559955126));
#242698=CARTESIAN_POINT('Ctrl Pts',(-198.192401847657,4.05400766411971,
133.592337783489));
#242699=CARTESIAN_POINT('Ctrl Pts',(-198.200176181776,4.12993714679204,
133.478593573467));
#242700=CARTESIAN_POINT('Ctrl Pts',(-198.207950515895,4.20107997053173,
133.361724522781));
#242701=CARTESIAN_POINT('Ctrl Pts',(-198.215715268842,4.27213511709918,
133.244999502756));
#242702=CARTESIAN_POINT('Ctrl Pts',(-198.22348002179,4.33841514090281,133.125157635332));
#242703=CARTESIAN_POINT('Ctrl Pts',(-198.231244774737,4.39963687332856,
133.002627763603));
#242704=CARTESIAN_POINT('Ctrl Pts',(-198.239001815622,4.46079779946676,
132.88021959027));
#242705=CARTESIAN_POINT('Ctrl Pts',(-198.246758856507,4.5169102585312,132.755129073059));
#242706=CARTESIAN_POINT('Ctrl Pts',(-198.254515897392,4.56773547585683,
132.627812203186));
#242707=CARTESIAN_POINT('Ctrl Pts',(-198.262267088632,4.61852236549037,
132.500591343955));
#242708=CARTESIAN_POINT('Ctrl Pts',(-198.270018279872,4.66402980520103,
132.371147835464));
#242709=CARTESIAN_POINT('Ctrl Pts',(-198.277769471112,4.70406605538651,
132.239960007737));
#242710=CARTESIAN_POINT('Ctrl Pts',(-198.285517367889,4.74408528909782,
132.108827938336));
#242711=CARTESIAN_POINT('Ctrl Pts',(-198.293265264666,4.77863784444936,
131.975953397409));
#242712=CARTESIAN_POINT('Ctrl Pts',(-198.301013161443,4.80758109007599,
131.841832123124));
#242713=CARTESIAN_POINT('Ctrl Pts',(-198.308759437527,4.83651828139958,
131.707738904118));
#242714=CARTESIAN_POINT('Ctrl Pts',(-198.316505713611,4.8598484144299,131.572399852405));
#242715=CARTESIAN_POINT('Ctrl Pts',(-198.324251989695,4.87747955738707,
131.436322823533));
#242716=CARTESIAN_POINT('Ctrl Pts',(-198.331998322961,4.89511083049331,
131.300244790173));
#242717=CARTESIAN_POINT('Ctrl Pts',(-198.339744656226,4.90704297934507,
131.163429156507));
#242718=CARTESIAN_POINT('Ctrl Pts',(-198.347490989491,4.91323577800568,
131.026390462913));
#242719=CARTESIAN_POINT('Ctrl Pts',(-198.355239057494,4.91942996350062,
130.889321080454));
#242720=CARTESIAN_POINT('Ctrl Pts',(-198.362987125497,4.91988222358433,
130.752028929157));
#242721=CARTESIAN_POINT('Ctrl Pts',(-198.3707351935,4.91460444749664,130.615029724296));
#242722=CARTESIAN_POINT('Ctrl Pts',(-198.378491496242,4.9093210621257,130.47788491505));
#242723=CARTESIAN_POINT('Ctrl Pts',(-198.386247798984,4.8982954903254,130.341034065488));
#242724=CARTESIAN_POINT('Ctrl Pts',(-198.394004101726,4.88159167919793,
130.204989497069));
#242725=CARTESIAN_POINT('Ctrl Pts',(-198.40176454424,4.86487895274352,130.068872317568));
#242726=CARTESIAN_POINT('Ctrl Pts',(-198.409524986754,4.84248201195462,
129.93356266222));
#242727=CARTESIAN_POINT('Ctrl Pts',(-198.417285429268,4.8145160155251,129.799562827584));
#242728=CARTESIAN_POINT('Ctrl Pts',(-198.425058329534,4.78650512559541,
129.665347884518));
#242729=CARTESIAN_POINT('Ctrl Pts',(-198.432831229799,4.7529074110492,129.532447343168));
#242730=CARTESIAN_POINT('Ctrl Pts',(-198.440604130065,4.71388825706518,
129.401349369428));
#242731=CARTESIAN_POINT('Ctrl Pts',(-198.448094465827,4.67628754761169,
129.275017137248));
#242732=CARTESIAN_POINT('Ctrl Pts',(-198.455584801589,4.6336528210575,129.150358983697));
#242733=CARTESIAN_POINT('Ctrl Pts',(-198.463075137351,4.58617366210336,
129.027792520495));
#242734=CARTESIAN_POINT('Ctrl Pts',(-198.47084947147,4.53689431640671,128.900578912589));
#242735=CARTESIAN_POINT('Ctrl Pts',(-198.478623805589,4.48223983117683,
128.775215764509));
#242736=CARTESIAN_POINT('Ctrl Pts',(-198.486398139708,4.42236902292319,
128.652190715446));
#242737=CARTESIAN_POINT('Ctrl Pts',(-198.494162892655,4.36257200009024,
128.529317283763));
#242738=CARTESIAN_POINT('Ctrl Pts',(-198.501927645602,4.29757161477436,
128.408776565947));
#242739=CARTESIAN_POINT('Ctrl Pts',(-198.509692398549,4.22757560526325,
128.29103859994));
#242740=CARTESIAN_POINT('Ctrl Pts',(-198.517449439434,4.15764911677518,
128.173417572941));
#242741=CARTESIAN_POINT('Ctrl Pts',(-198.525206480319,4.08273707664526,
128.058594091884));
#242742=CARTESIAN_POINT('Ctrl Pts',(-198.532963521204,4.0030940596596,127.947015519049));
#242743=CARTESIAN_POINT('Ctrl Pts',(-198.540714712445,3.92351110209268,
127.835521088484));
#242744=CARTESIAN_POINT('Ctrl Pts',(-198.548465903685,3.8392044951129,127.727267012445));
#242745=CARTESIAN_POINT('Ctrl Pts',(-198.556217094925,3.7504730313789,127.622673155951));
#242746=CARTESIAN_POINT('Ctrl Pts',(-198.563964991702,3.66177928088409,
127.518123754636));
#242747=CARTESIAN_POINT('Ctrl Pts',(-198.571712888479,3.56866466656006,
127.417231776227));
#242748=CARTESIAN_POINT('Ctrl Pts',(-198.579460785256,3.47146917123165,
127.320385179121));
#242749=CARTESIAN_POINT('Ctrl Pts',(-198.58720706134,3.37429400710557,127.223558840235));
#242750=CARTESIAN_POINT('Ctrl Pts',(-198.594953337424,3.27303993667195,
127.130776475282));
#242751=CARTESIAN_POINT('Ctrl Pts',(-198.602699613508,3.16808454181421,
127.042389937401));
#242752=CARTESIAN_POINT('Ctrl Pts',(-198.610445946774,3.06312837219946,
126.954002747071));
#242753=CARTESIAN_POINT('Ctrl Pts',(-198.618192280039,2.95447112269024,
126.870011700402));
#242754=CARTESIAN_POINT('Ctrl Pts',(-198.625938613304,2.84252394757572,
126.790728762256));
#242755=CARTESIAN_POINT('Ctrl Pts',(-198.633686681307,2.73055170266768,
126.711428069246));
#242756=CARTESIAN_POINT('Ctrl Pts',(-198.64143474931,2.61528838508869,126.636837808705));
#242757=CARTESIAN_POINT('Ctrl Pts',(-198.649182817313,2.49717430712868,
126.567226734584));
#242758=CARTESIAN_POINT('Ctrl Pts',(-198.656939120055,2.37893469612088,
126.497541676984));
#242759=CARTESIAN_POINT('Ctrl Pts',(-198.664695422797,2.2578386096946,126.432846575844));
#242760=CARTESIAN_POINT('Ctrl Pts',(-198.672451725539,2.13435164337421,
126.373364552918));
#242761=CARTESIAN_POINT('Ctrl Pts',(-198.680212168053,2.01079876834144,
126.313850782646));
#242762=CARTESIAN_POINT('Ctrl Pts',(-198.687972610567,1.88485282955681,
126.259555789408));
#242763=CARTESIAN_POINT('Ctrl Pts',(-198.695733053081,1.75699866942774,
126.210654190493));
#242764=CARTESIAN_POINT('Ctrl Pts',(-198.703505953346,1.62893926645082,
126.161674090391));
#242765=CARTESIAN_POINT('Ctrl Pts',(-198.711278853612,1.49896589169275,
126.1181048103));
#242766=CARTESIAN_POINT('Ctrl Pts',(-198.719051753877,1.36757864767384,
126.080071072573));
#242767=CARTESIAN_POINT('Ctrl Pts',(-198.726542089639,1.24096766091596,
126.043419957014));
#242768=CARTESIAN_POINT('Ctrl Pts',(-198.734032425402,1.11304411471436,
126.011908983002));
#242769=CARTESIAN_POINT('Ctrl Pts',(-198.741522761164,0.984261832800122,
125.985604376896));
#242770=CARTESIAN_POINT('Ctrl Pts',(-198.749297095283,0.850596731528147,
125.958302423656));
#242771=CARTESIAN_POINT('Ctrl Pts',(-198.757071429402,0.715583080302673,
125.936522946273));
#242772=CARTESIAN_POINT('Ctrl Pts',(-198.764845763521,0.579716987989611,
125.920395908814));
#242773=CARTESIAN_POINT('Ctrl Pts',(-198.772610516468,0.444018338491886,
125.904288746487));
#242774=CARTESIAN_POINT('Ctrl Pts',(-198.780375269415,0.307469722715481,
125.89382020921));
#242775=CARTESIAN_POINT('Ctrl Pts',(-198.788140022362,0.170578884512039,
125.889069587865));
#242776=CARTESIAN_POINT('Ctrl Pts',(-198.795897063247,0.0338240082189226,
125.884323684905));
#242777=CARTESIAN_POINT('Ctrl Pts',(-198.803654104132,-0.103272025883022,
125.885284409655));
#242778=CARTESIAN_POINT('Ctrl Pts',(-198.811411145017,-0.240195235348314,
125.891979391377));
#242779=CARTESIAN_POINT('Ctrl Pts',(-198.819162336258,-0.377015189955682,
125.898669324361));
#242780=CARTESIAN_POINT('Ctrl Pts',(-198.826913527498,-0.513662190418549,
125.911084888148));
#242781=CARTESIAN_POINT('Ctrl Pts',(-198.834664718738,-0.649621487673782,
125.929201647312));
#242782=CARTESIAN_POINT('Ctrl Pts',(-198.842412615515,-0.785522998601034,
125.947310706369));
#242783=CARTESIAN_POINT('Ctrl Pts',(-198.850160512292,-0.920737000939123,
125.971116089789));
#242784=CARTESIAN_POINT('Ctrl Pts',(-198.857908409069,-1.05475332528018,
126.000541461383));
#242785=CARTESIAN_POINT('Ctrl Pts',(-198.865654685153,-1.18874161629487,
126.029960677823));
#242786=CARTESIAN_POINT('Ctrl Pts',(-198.873400961237,-1.32153234600044,
126.064997460351));
#242787=CARTESIAN_POINT('Ctrl Pts',(-198.881147237321,-1.45262539815508,
126.105524323851));
#242788=CARTESIAN_POINT('Ctrl Pts',(-198.888893570586,-1.58371941800903,
126.14605148651));
#242789=CARTESIAN_POINT('Ctrl Pts',(-198.896639903852,-1.71311536178222,
126.192068695536));
#242790=CARTESIAN_POINT('Ctrl Pts',(-198.904386237117,-1.84032852566538,
126.243398659807));
#242791=CARTESIAN_POINT('Ctrl Pts',(-198.91213430512,-1.96757017805508,
126.294740119068));
#242792=CARTESIAN_POINT('Ctrl Pts',(-198.919882373123,-2.09262771536865,
126.351396554784));
#242793=CARTESIAN_POINT('Ctrl Pts',(-198.927630441126,-2.2150370277501,
126.413142787829));
#242794=CARTESIAN_POINT('Ctrl Pts',(-198.935386743868,-2.33757643820495,
126.474954645506));
#242795=CARTESIAN_POINT('Ctrl Pts',(-198.94314304661,-2.4574616517044,126.541866930204));
#242796=CARTESIAN_POINT('Ctrl Pts',(-198.950899349351,-2.57425328384323,
126.613608525981));
#242797=CARTESIAN_POINT('Ctrl Pts',(-198.958659791866,-2.69110725119298,
126.685388412409));
#242798=CARTESIAN_POINT('Ctrl Pts',(-198.96642023438,-2.80486402303167,
126.762002527609));
#242799=CARTESIAN_POINT('Ctrl Pts',(-198.974180676894,-2.91511461972486,
126.843137344842));
#242800=CARTESIAN_POINT('Ctrl Pts',(-198.981953577159,-3.02554220046346,
126.924402406887));
#242801=CARTESIAN_POINT('Ctrl Pts',(-198.989726477425,-3.13245205358369,
127.010202427981));
#242802=CARTESIAN_POINT('Ctrl Pts',(-198.99749937769,-3.23546892900845,
127.100184073188));
#242803=CARTESIAN_POINT('Ctrl Pts',(-199.004989713452,-3.33474088152516,
127.186894658939));
#242804=CARTESIAN_POINT('Ctrl Pts',(-199.012480049214,-3.43039775782205,
127.277487910186));
#242805=CARTESIAN_POINT('Ctrl Pts',(-199.019970384976,-3.52213853697615,
127.371617809133));
#242806=CARTESIAN_POINT('Ctrl Pts',(-199.027641276347,-3.6160907406696,
127.468016722693));
#242807=CARTESIAN_POINT('Ctrl Pts',(-199.035312167719,-3.70625045185473,
127.568448295507));
#242808=CARTESIAN_POINT('Ctrl Pts',(-199.04298305909,-3.79224452810265,
127.672577658679));
#242809=CARTESIAN_POINT('Ctrl Pts',(-199.0506449325,-3.87813750901698,127.776584606526));
#242810=CARTESIAN_POINT('Ctrl Pts',(-199.058306805909,-3.9598743377894,
127.884280395336));
#242811=CARTESIAN_POINT('Ctrl Pts',(-199.065968679319,-4.03711767976908,
127.995292462075));
#242812=CARTESIAN_POINT('Ctrl Pts',(-199.073623311162,-4.11428801574521,
128.106199606536));
#242813=CARTESIAN_POINT('Ctrl Pts',(-199.081277943005,-4.1869730825278,
128.220416467907));
#242814=CARTESIAN_POINT('Ctrl Pts',(-199.088932574849,-4.25487528640376,
128.337536878494));
#242815=CARTESIAN_POINT('Ctrl Pts',(-199.096581319393,-4.32272526561704,
128.454567209913));
#242816=CARTESIAN_POINT('Ctrl Pts',(-199.104230063938,-4.38579950174855,
128.574496299718));
#242817=CARTESIAN_POINT('Ctrl Pts',(-199.111878808483,-4.44384363448245,
128.696888953517));
#242818=CARTESIAN_POINT('Ctrl Pts',(-199.119524183703,-4.50186219837772,
128.819227692512));
#242819=CARTESIAN_POINT('Ctrl Pts',(-199.127169558923,-4.55485489515574,
128.944027473816));
#242820=CARTESIAN_POINT('Ctrl Pts',(-199.134814934143,-4.60261344758878,
129.070828813827));
#242821=CARTESIAN_POINT('Ctrl Pts',(-199.142459303634,-4.65036571750983,
129.197613473455));
#242822=CARTESIAN_POINT('Ctrl Pts',(-199.150103673125,-4.69288506876711,
129.32639879276));
#242823=CARTESIAN_POINT('Ctrl Pts',(-199.157748042617,-4.73001164933185,
129.456706040278));
#242824=CARTESIAN_POINT('Ctrl Pts',(-199.160198861551,-4.74191459655825,
129.498483124697));
#242825=CARTESIAN_POINT('Ctrl Pts',(-199.162649680486,-4.75326361641396,
129.540416517897));
#242826=CARTESIAN_POINT('Ctrl Pts',(-199.165100499421,-4.76405452823391,
129.582490119308));
#242827=CARTESIAN_POINT('',(-197.13985943604,-4.91824821858491,130.800174582878));
#242828=CARTESIAN_POINT('Ctrl Pts',(-197.13985943604,-4.91824821858491,
130.800174582878));
#242829=CARTESIAN_POINT('Ctrl Pts',(-197.147506112978,-4.91836287925791,
130.93489149106));
#242830=CARTESIAN_POINT('Ctrl Pts',(-197.155152789915,-4.91293828803124,
131.069802457209));
#242831=CARTESIAN_POINT('Ctrl Pts',(-197.162799466852,-4.9019533167259,
131.204406543854));
#242832=CARTESIAN_POINT('Ctrl Pts',(-197.170439161222,-4.89097837635308,
131.338887716705));
#242833=CARTESIAN_POINT('Ctrl Pts',(-197.178078855592,-4.87445318757935,
131.473062167562));
#242834=CARTESIAN_POINT('Ctrl Pts',(-197.185718549962,-4.85240867394315,
131.606428646814));
#242835=CARTESIAN_POINT('Ctrl Pts',(-197.193353528545,-4.83037776781788,
131.73971280237));
#242836=CARTESIAN_POINT('Ctrl Pts',(-197.200988507129,-4.80283437820965,
131.872189581299));
#242837=CARTESIAN_POINT('Ctrl Pts',(-197.208623485712,-4.76986124614636,
132.003363017485));
#242838=CARTESIAN_POINT('Ctrl Pts',(-197.216256000669,-4.73689875372977,
132.134494127118));
#242839=CARTESIAN_POINT('Ctrl Pts',(-197.223888515626,-4.69851009985092,
132.264322339006));
#242840=CARTESIAN_POINT('Ctrl Pts',(-197.231521030583,-4.6548290030468,
132.392362511423));
#242841=CARTESIAN_POINT('Ctrl Pts',(-197.239152849597,-4.61115188914653,
132.520391008958));
#242842=CARTESIAN_POINT('Ctrl Pts',(-197.24678466861,-4.56218342217936,
132.646631409198));
#242843=CARTESIAN_POINT('Ctrl Pts',(-197.254416487624,-4.50810682560393,
132.770614902099));
#242844=CARTESIAN_POINT('Ctrl Pts',(-197.262049377602,-4.45402264051946,
132.894615793466));
#242845=CARTESIAN_POINT('Ctrl Pts',(-197.26968226758,-4.39482906232151,
133.016358777953));
#242846=CARTESIAN_POINT('Ctrl Pts',(-197.277315157558,-4.33075673716147,
133.135396684647));
#242847=CARTESIAN_POINT('Ctrl Pts',(-197.284955576458,-4.26662121241328,
133.254552007817));
#242848=CARTESIAN_POINT('Ctrl Pts',(-197.292595995358,-4.19759752046628,
133.37099656774));
#242849=CARTESIAN_POINT('Ctrl Pts',(-197.300236414258,-4.1239615861599,
133.484309105574));
#242850=CARTESIAN_POINT('Ctrl Pts',(-197.307880546064,-4.05028986803414,
133.597676708309));
#242851=CARTESIAN_POINT('Ctrl Pts',(-197.315524677871,-3.97200167824627,
133.707908929455));
#242852=CARTESIAN_POINT('Ctrl Pts',(-197.323168809677,-3.88941447193958,
133.814616109707));
#242853=CARTESIAN_POINT('Ctrl Pts',(-197.330825110679,-3.8066957896451,
133.921493164115));
#242854=CARTESIAN_POINT('Ctrl Pts',(-197.33848141168,-3.71966467800465,
134.024833657621));
#242855=CARTESIAN_POINT('Ctrl Pts',(-197.346137712681,-3.62867730838004,
134.124282913968));
#242856=CARTESIAN_POINT('Ctrl Pts',(-197.35371635454,-3.53861283886426,
134.222723439874));
#242857=CARTESIAN_POINT('Ctrl Pts',(-197.3612949964,-3.44467233174058,134.317351104802));
#242858=CARTESIAN_POINT('Ctrl Pts',(-197.368873638259,-3.34723265001436,
134.407861227969));
#242859=CARTESIAN_POINT('Ctrl Pts',(-197.376647972378,-3.24727692493325,
134.500708462567));
#242860=CARTESIAN_POINT('Ctrl Pts',(-197.384422306497,-3.14329678401998,
134.589540674901));
#242861=CARTESIAN_POINT('Ctrl Pts',(-197.392196640617,-3.03564832798573,
134.673988802715));
#242862=CARTESIAN_POINT('Ctrl Pts',(-197.399961393564,-2.92813253905301,
134.758332855758));
#242863=CARTESIAN_POINT('Ctrl Pts',(-197.407726146511,-2.81695773483861,
134.83830333563));
#242864=CARTESIAN_POINT('Ctrl Pts',(-197.415490899458,-2.70251631213269,
134.91356840559));
#242865=CARTESIAN_POINT('Ctrl Pts',(-197.423247940343,-2.58818855426113,
134.988758721222));
#242866=CARTESIAN_POINT('Ctrl Pts',(-197.431004981228,-2.47060095904148,
135.059252713936));
#242867=CARTESIAN_POINT('Ctrl Pts',(-197.438762022113,-2.35017812468133,
135.124759423784));
#242868=CARTESIAN_POINT('Ctrl Pts',(-197.446513213353,-2.22984610211716,
135.190216734512));
#242869=CARTESIAN_POINT('Ctrl Pts',(-197.454264404593,-2.1066834381736,
135.250694062248));
#242870=CARTESIAN_POINT('Ctrl Pts',(-197.462015595833,-1.98114246876202,
135.305944514481));
#242871=CARTESIAN_POINT('Ctrl Pts',(-197.46976349261,-1.85565485761151,
135.361171483799));
#242872=CARTESIAN_POINT('Ctrl Pts',(-197.477511389387,-1.72779130857727,
135.411175838973));
#242873=CARTESIAN_POINT('Ctrl Pts',(-197.485259286164,-1.59802724398115,
135.455757395954));
#242874=CARTESIAN_POINT('Ctrl Pts',(-197.493005562248,-1.46829032322996,
135.500329627433));
#242875=CARTESIAN_POINT('Ctrl Pts',(-197.500751838333,-1.33665404717749,
135.539481190017));
#242876=CARTESIAN_POINT('Ctrl Pts',(-197.508498114417,-1.20361185877549,
135.573060813208));
#242877=CARTESIAN_POINT('Ctrl Pts',(-197.516244447682,-1.0705686882861,
135.606640684276));
#242878=CARTESIAN_POINT('Ctrl Pts',(-197.523990780947,-0.936119963815441,
135.634648438198));
#242879=CARTESIAN_POINT('Ctrl Pts',(-197.531737114213,-0.800771873265166,
135.656983358877));
#242880=CARTESIAN_POINT('Ctrl Pts',(-197.539485182216,-0.665393472448266,
135.679323281307));
#242881=CARTESIAN_POINT('Ctrl Pts',(-197.547233250219,-0.52911569045003,
135.695987778918));
#242882=CARTESIAN_POINT('Ctrl Pts',(-197.554981318222,-0.392452037104296,
135.706927747252));
#242883=CARTESIAN_POINT('Ctrl Pts',(-197.562737620963,-0.255643136002026,
135.717879342714));
#242884=CARTESIAN_POINT('Ctrl Pts',(-197.570493923705,-0.118447934655994,
135.723094224012));
#242885=CARTESIAN_POINT('Ctrl Pts',(-197.578250226447,0.0186172786708312,
135.722575381018));
#242886=CARTESIAN_POINT('Ctrl Pts',(-197.586010668961,0.155755647829336,
135.722056261102));
#242887=CARTESIAN_POINT('Ctrl Pts',(-197.593771111476,0.292763500359275,
135.715797336897));
#242888=CARTESIAN_POINT('Ctrl Pts',(-197.60153155399,0.429128454194537,
135.703853635451));
#242889=CARTESIAN_POINT('Ctrl Pts',(-197.609304454255,0.565712313159607,
135.691890760914));
#242890=CARTESIAN_POINT('Ctrl Pts',(-197.617077354521,0.701650823160877,
135.674224923474));
#242891=CARTESIAN_POINT('Ctrl Pts',(-197.624850254786,0.836439701705548,
135.650962694064));
#242892=CARTESIAN_POINT('Ctrl Pts',(-197.632340590548,0.966328665002057,
135.628546105287));
#242893=CARTESIAN_POINT('Ctrl Pts',(-197.63983092631,1.09514982852237,135.600933010851));
#242894=CARTESIAN_POINT('Ctrl Pts',(-197.647321262072,1.2224661119373,135.568262344897));
#242895=CARTESIAN_POINT('Ctrl Pts',(-197.655095596191,1.35460963093539,
135.534352960713));
#242896=CARTESIAN_POINT('Ctrl Pts',(-197.66286993031,1.48555049305068,135.494887503906));
#242897=CARTESIAN_POINT('Ctrl Pts',(-197.670644264429,1.61478571462178,
135.449966084925));
#242898=CARTESIAN_POINT('Ctrl Pts',(-197.678409017376,1.74386166533168,
135.405100027578));
#242899=CARTESIAN_POINT('Ctrl Pts',(-197.686173770323,1.87123579220267,
135.354791513917));
#242900=CARTESIAN_POINT('Ctrl Pts',(-197.693938523271,1.99641681153709,
135.29919131261));
#242901=CARTESIAN_POINT('Ctrl Pts',(-197.701695564156,2.1214734993187,135.243646334207));
#242902=CARTESIAN_POINT('Ctrl Pts',(-197.70945260504,2.24434105933608,135.182820285069));
#242903=CARTESIAN_POINT('Ctrl Pts',(-197.717209645925,2.36454519304033,
135.116913120733));
#242904=CARTESIAN_POINT('Ctrl Pts',(-197.724960837166,2.4846586798728,135.051055657502));
#242905=CARTESIAN_POINT('Ctrl Pts',(-197.732712028406,2.60211239678094,
134.98012489306));
#242906=CARTESIAN_POINT('Ctrl Pts',(-197.740463219646,2.7164541274949,134.904367938988));
#242907=CARTESIAN_POINT('Ctrl Pts',(-197.748211116423,2.83074725992267,
134.828643183643));
#242908=CARTESIAN_POINT('Ctrl Pts',(-197.7559590132,2.94193071162179,134.748096533953));
#242909=CARTESIAN_POINT('Ctrl Pts',(-197.763706909977,3.04957908470244,
134.663019771812));
#242910=CARTESIAN_POINT('Ctrl Pts',(-197.771453186061,3.15720494006407,
134.577960805895));
#242911=CARTESIAN_POINT('Ctrl Pts',(-197.779199462145,3.26129688109708,
134.488373854626));
#242912=CARTESIAN_POINT('Ctrl Pts',(-197.786945738229,3.361460921679,134.394592300135));
#242913=CARTESIAN_POINT('Ctrl Pts',(-197.794692071495,3.46162570164924,
134.30081005337));
#242914=CARTESIAN_POINT('Ctrl Pts',(-197.80243840476,3.55786223791384,134.20283340881));
#242915=CARTESIAN_POINT('Ctrl Pts',(-197.810184738026,3.64981218824234,
134.101033797161));
#242916=CARTESIAN_POINT('Ctrl Pts',(-197.817932806029,3.74178273012479,
133.999211388194));
#242917=CARTESIAN_POINT('Ctrl Pts',(-197.825680874032,3.82946451386792,
133.893564598623));
#242918=CARTESIAN_POINT('Ctrl Pts',(-197.833428942035,3.91253866189194,
133.784498916656));
#242919=CARTESIAN_POINT('Ctrl Pts',(-197.841185244776,3.99570110210896,
133.675317318384));
#242920=CARTESIAN_POINT('Ctrl Pts',(-197.848941547518,4.07424588694472,
133.562709880643));
#242921=CARTESIAN_POINT('Ctrl Pts',(-197.85669785026,4.14789646544683,133.44711258747));
#242922=CARTESIAN_POINT('Ctrl Pts',(-197.864458292774,4.22158635348026,
133.331453596542));
#242923=CARTESIAN_POINT('Ctrl Pts',(-197.872218735289,4.29037663418042,
133.212801908529));
#242924=CARTESIAN_POINT('Ctrl Pts',(-197.879979177803,4.35403664833725,
133.091618348439));
#242925=CARTESIAN_POINT('Ctrl Pts',(-197.887752078068,4.41779885520026,
132.970240253739));
#242926=CARTESIAN_POINT('Ctrl Pts',(-197.895524978334,4.4764141709775,132.846322518647));
#242927=CARTESIAN_POINT('Ctrl Pts',(-197.903297878599,4.52969967980894,
132.720347014501));
#242928=CARTESIAN_POINT('Ctrl Pts',(-197.910788214361,4.58104812617597,
132.598951037243));
#242929=CARTESIAN_POINT('Ctrl Pts',(-197.918278550123,4.62744743329827,
132.475644591939));
#242930=CARTESIAN_POINT('Ctrl Pts',(-197.925768885885,4.66877823780837,
132.350870503945));
#242931=CARTESIAN_POINT('Ctrl Pts',(-197.933543220004,4.71167611233399,
132.221365568478));
#242932=CARTESIAN_POINT('Ctrl Pts',(-197.941317554123,4.74924944018407,
132.089869269341));
#242933=CARTESIAN_POINT('Ctrl Pts',(-197.949091888242,4.78131057215974,
131.956858893076));
#242934=CARTESIAN_POINT('Ctrl Pts',(-197.956856641189,4.81333219165545,
131.824012440213));
#242935=CARTESIAN_POINT('Ctrl Pts',(-197.964621394136,4.83985504116094,
131.689655999366));
#242936=CARTESIAN_POINT('Ctrl Pts',(-197.972386147084,4.86074041578861,
131.554284395572));
#242937=CARTESIAN_POINT('Ctrl Pts',(-197.980143187969,4.88160504676788,
131.419047244763));
#242938=CARTESIAN_POINT('Ctrl Pts',(-197.987900228854,4.89684328634105,
131.282797321412));
#242939=CARTESIAN_POINT('Ctrl Pts',(-197.995657269739,4.90636699281359,
131.146041747173));
#242940=CARTESIAN_POINT('Ctrl Pts',(-198.003408460979,4.91588351738501,
131.009389301376));
#242941=CARTESIAN_POINT('Ctrl Pts',(-198.011159652219,4.91969405935185,
130.872232352118));
#242942=CARTESIAN_POINT('Ctrl Pts',(-198.018910843459,4.91776208674575,
130.7350849316));
#242943=CARTESIAN_POINT('Ctrl Pts',(-198.026658740236,4.91583093527955,
130.597995802394));
#242944=CARTESIAN_POINT('Ctrl Pts',(-198.034406637013,4.90816212914558,
130.460916583982));
#242945=CARTESIAN_POINT('Ctrl Pts',(-198.04215453379,4.89477121476498,130.324362890896));
#242946=CARTESIAN_POINT('Ctrl Pts',(-198.049900809875,4.881383101475,130.187837761899));
#242947=CARTESIAN_POINT('Ctrl Pts',(-198.057647085959,4.86227529885319,
130.051838328427));
#242948=CARTESIAN_POINT('Ctrl Pts',(-198.065393362043,4.83751533160561,
129.916876263349));
#242949=CARTESIAN_POINT('Ctrl Pts',(-198.073139695308,4.81275518158554,
129.78191320201));
#242950=CARTESIAN_POINT('Ctrl Pts',(-198.080886028573,4.78234285423304,
129.647987908893));
#242951=CARTESIAN_POINT('Ctrl Pts',(-198.088632361839,4.74639715199262,
129.515602634834));
#242952=CARTESIAN_POINT('Ctrl Pts',(-198.096380429842,4.71044339996136,
129.38318771401));
#242953=CARTESIAN_POINT('Ctrl Pts',(-198.104128497845,4.66895390968266,
129.25231387574));
#242954=CARTESIAN_POINT('Ctrl Pts',(-198.111876565848,4.62209746874859,
129.123468577045));
#242955=CARTESIAN_POINT('Ctrl Pts',(-198.11963286859,4.57519122823157,128.994486340033));
#242956=CARTESIAN_POINT('Ctrl Pts',(-198.127389171331,4.52290677641864,
128.867537317358));
#242957=CARTESIAN_POINT('Ctrl Pts',(-198.135145474073,4.46546143648297,
128.743089839191));
#242958=CARTESIAN_POINT('Ctrl Pts',(-198.142905916588,4.40798543623973,
128.618575939658));
#242959=CARTESIAN_POINT('Ctrl Pts',(-198.150666359102,4.34534323773866,
128.496566592663));
#242960=CARTESIAN_POINT('Ctrl Pts',(-198.158426801616,4.27779786917148,
128.377504945506));
#242961=CARTESIAN_POINT('Ctrl Pts',(-198.166199701881,4.21014407078227,
128.258252170022));
#242962=CARTESIAN_POINT('Ctrl Pts',(-198.173972602147,4.13757158065354,
128.141956882111));
#242963=CARTESIAN_POINT('Ctrl Pts',(-198.181745502412,4.06038694029745,
128.029033437293));
#242964=CARTESIAN_POINT('Ctrl Pts',(-198.189235838174,3.98600815603532,
127.920215044132));
#242965=CARTESIAN_POINT('Ctrl Pts',(-198.196726173936,3.90734691024696,
127.81452784734));
#242966=CARTESIAN_POINT('Ctrl Pts',(-198.204216509698,3.8247112456301,127.712311628619));
#242967=CARTESIAN_POINT('Ctrl Pts',(-198.211990843817,3.73894242467187,
127.606219850896));
#242968=CARTESIAN_POINT('Ctrl Pts',(-198.219765177936,3.64862016552164,
127.503531384384));
#242969=CARTESIAN_POINT('Ctrl Pts',(-198.227539512055,3.55404459388961,
127.404662088704));
#242970=CARTESIAN_POINT('Ctrl Pts',(-198.235304265002,3.45958557819766,
127.305914640596));
#242971=CARTESIAN_POINT('Ctrl Pts',(-198.24306901795,3.36088394735533,127.210977278024));
#242972=CARTESIAN_POINT('Ctrl Pts',(-198.250833770897,3.25828103830071,
127.12023416236));
#242973=CARTESIAN_POINT('Ctrl Pts',(-198.258590811782,3.15578003590126,
127.029581174037));
#242974=CARTESIAN_POINT('Ctrl Pts',(-198.266347852667,3.04938575729155,
126.943114399854));
#242975=CARTESIAN_POINT('Ctrl Pts',(-198.274104893552,2.93947721554274,
126.861182107556));
#242976=CARTESIAN_POINT('Ctrl Pts',(-198.281856084792,2.82965155668068,
126.779311601038));
#242977=CARTESIAN_POINT('Ctrl Pts',(-198.289607276032,2.71631722179468,
126.701969002842));
#242978=CARTESIAN_POINT('Ctrl Pts',(-198.297358467272,2.59988693431213,
126.629462895311));
#242979=CARTESIAN_POINT('Ctrl Pts',(-198.305106364049,2.48350613280748,
126.556987604809));
#242980=CARTESIAN_POINT('Ctrl Pts',(-198.312854260826,2.36403232703562,
126.489344922703));
#242981=CARTESIAN_POINT('Ctrl Pts',(-198.320602157603,2.24190772132709,
126.4268004716));
#242982=CARTESIAN_POINT('Ctrl Pts',(-198.328348433687,2.11980866145337,
126.364269103447));
#242983=CARTESIAN_POINT('Ctrl Pts',(-198.336094709771,1.99506025231821,
126.306834023191));
#242984=CARTESIAN_POINT('Ctrl Pts',(-198.343840985855,1.8681294775501,126.254714992069));
#242985=CARTESIAN_POINT('Ctrl Pts',(-198.351587319121,1.74119776580766,
126.202595576215));
#242986=CARTESIAN_POINT('Ctrl Pts',(-198.359333652386,1.61208401795031,
126.155792436301));
#242987=CARTESIAN_POINT('Ctrl Pts',(-198.367079985652,1.48127500745482,
126.114477099312));
#242988=CARTESIAN_POINT('Ctrl Pts',(-198.374828053655,1.35043670318858,
126.07315251004));
#242989=CARTESIAN_POINT('Ctrl Pts',(-198.382576121657,1.21790275358034,
126.037318286899));
#242990=CARTESIAN_POINT('Ctrl Pts',(-198.39032418966,1.08417450384265,126.007095906534));
#242991=CARTESIAN_POINT('Ctrl Pts',(-198.398080492402,0.950304126129575,
125.976841405463));
#242992=CARTESIAN_POINT('Ctrl Pts',(-198.405836795144,0.81523729464666,
125.952210747888));
#242993=CARTESIAN_POINT('Ctrl Pts',(-198.413593097886,0.679485497313303,
125.933274237564));
#242994=CARTESIAN_POINT('Ctrl Pts',(-198.4213535404,0.543661245157932,125.914327620255));
#242995=CARTESIAN_POINT('Ctrl Pts',(-198.429113982914,0.407151687636302,
125.901081243678));
#242996=CARTESIAN_POINT('Ctrl Pts',(-198.436874425429,0.270471830283358,
125.893553346707));
#242997=CARTESIAN_POINT('Ctrl Pts',(-198.444647325694,0.133572562289896,
125.886013365287));
#242998=CARTESIAN_POINT('Ctrl Pts',(-198.45242022596,-0.00349716067967948,
125.884210212806));
#242999=CARTESIAN_POINT('Ctrl Pts',(-198.460193126225,-0.140223036415281,
125.888109956487));
#243000=CARTESIAN_POINT('Ctrl Pts',(-198.467683461987,-0.271978582175825,
125.891867934663));
#243001=CARTESIAN_POINT('Ctrl Pts',(-198.475173797749,-0.403414538811383,
125.900921357127));
#243002=CARTESIAN_POINT('Ctrl Pts',(-198.482664133511,-0.534078533749533,
125.915194719144));
#243003=CARTESIAN_POINT('Ctrl Pts',(-198.49043846763,-0.669696693770792,
125.930009260021));
#243004=CARTESIAN_POINT('Ctrl Pts',(-198.498212801749,-0.804912796249909,
125.950494310249));
#243005=CARTESIAN_POINT('Ctrl Pts',(-198.505987135868,-0.939214741433294,
125.97662214785));
#243006=CARTESIAN_POINT('Ctrl Pts',(-198.513751888815,-1.07335117147142,
126.002717785227));
#243007=CARTESIAN_POINT('Ctrl Pts',(-198.521516641762,-1.20657530576016,
126.034442299186));
#243008=CARTESIAN_POINT('Ctrl Pts',(-198.529281394709,-1.33837943750662,
126.071716161899));
#243009=CARTESIAN_POINT('Ctrl Pts',(-198.537038435594,-1.47005265953166,
126.108953003685));
#243010=CARTESIAN_POINT('Ctrl Pts',(-198.544795476479,-1.60030831193102,
126.151728120008));
#243011=CARTESIAN_POINT('Ctrl Pts',(-198.552552517364,-1.72864852136443,
126.199910883658));
#243012=CARTESIAN_POINT('Ctrl Pts',(-198.560303708605,-1.85689194844843,
126.248057312312));
#243013=CARTESIAN_POINT('Ctrl Pts',(-198.568054899845,-1.9832224431181,
126.301603134525));
#243014=CARTESIAN_POINT('Ctrl Pts',(-198.575806091085,-2.10715729921745,
126.36036791068));
#243015=CARTESIAN_POINT('Ctrl Pts',(-198.583553987862,-2.23103947969604,
126.419107710238));
#243016=CARTESIAN_POINT('Ctrl Pts',(-198.591301884639,-2.3525276942214,
126.483061884765));
#243017=CARTESIAN_POINT('Ctrl Pts',(-198.599049781416,-2.47115944473042,
126.552001970742));
#243018=CARTESIAN_POINT('Ctrl Pts',(-198.6067960575,-2.58976638003497,126.620927635939));
#243019=CARTESIAN_POINT('Ctrl Pts',(-198.614542333584,-2.70551770198718,
126.694836941795));
#243020=CARTESIAN_POINT('Ctrl Pts',(-198.622288609669,-2.81797610317734,
126.773455788074));
#243021=CARTESIAN_POINT('Ctrl Pts',(-198.630034942934,-2.93043533450971,
126.852075214699));
#243022=CARTESIAN_POINT('Ctrl Pts',(-198.637781276199,-3.03960127614829,
126.93540402711));
#243023=CARTESIAN_POINT('Ctrl Pts',(-198.645527609465,-3.14506650462893,
127.023125403517));
#243024=CARTESIAN_POINT('Ctrl Pts',(-198.653275677468,-3.25055535131611,
127.110866424519));
#243025=CARTESIAN_POINT('Ctrl Pts',(-198.661023745471,-3.35234153520745,
127.203001716974));
#243026=CARTESIAN_POINT('Ctrl Pts',(-198.668771813474,-3.4500518652282,
127.299175146049));
#243027=CARTESIAN_POINT('Ctrl Pts',(-198.676528116215,-3.54786604295059,
127.395450789389));
#243028=CARTESIAN_POINT('Ctrl Pts',(-198.684284418957,-3.64159543435231,
127.49577286795));
#243029=CARTESIAN_POINT('Ctrl Pts',(-198.692040721699,-3.73090441917804,
127.599749053358));
#243030=CARTESIAN_POINT('Ctrl Pts',(-198.699801164213,-3.82026107089802,
127.703780733986));
#243031=CARTESIAN_POINT('Ctrl Pts',(-198.707561606727,-3.90519237294011,
127.81147010078));
#243032=CARTESIAN_POINT('Ctrl Pts',(-198.715322049242,-3.98540460735336,
127.922393723553));
#243033=CARTESIAN_POINT('Ctrl Pts',(-198.723094949507,-4.06574560556619,
128.033495410773));
#243034=CARTESIAN_POINT('Ctrl Pts',(-198.730867849773,-4.14135218219585,
128.147841402763));
#243035=CARTESIAN_POINT('Ctrl Pts',(-198.738640750038,-4.21197489294038,
128.264980661014));
#243036=CARTESIAN_POINT('Ctrl Pts',(-198.7461310858,-4.28003029026089,128.37786161217));
#243037=CARTESIAN_POINT('Ctrl Pts',(-198.753621421562,-4.34345773459829,
128.493336000931));
#243038=CARTESIAN_POINT('Ctrl Pts',(-198.761111757324,-4.40207623179987,
128.610982421285));
#243039=CARTESIAN_POINT('Ctrl Pts',(-198.769439516326,-4.46724830596083,
128.741781769581));
#243040=CARTESIAN_POINT('Ctrl Pts',(-198.777767275329,-4.52666005472299,
128.87563467257));
#243041=CARTESIAN_POINT('Ctrl Pts',(-198.786095034331,-4.58003551060785,
129.012027561443));
#243042=CARTESIAN_POINT('Ctrl Pts',(-198.794402369264,-4.63328006164643,
129.148085942819));
#243043=CARTESIAN_POINT('Ctrl Pts',(-198.802709704197,-4.6805177289175,
129.2866716051));
#243044=CARTESIAN_POINT('Ctrl Pts',(-198.811017039129,-4.72151946632294,
129.427248787817));
#243045=CARTESIAN_POINT('Ctrl Pts',(-198.814059766598,-4.73653717220337,
129.478737990889));
#243046=CARTESIAN_POINT('Ctrl Pts',(-198.817102494067,-4.75071875239664,
129.530494131717));
#243047=CARTESIAN_POINT('Ctrl Pts',(-198.820145221536,-4.76405452823399,
129.582490119308));
#243048=CARTESIAN_POINT('Ctrl Pts',(-197.069830899744,-4.76405452823391,
129.582490119308));
#243049=CARTESIAN_POINT('Ctrl Pts',(-197.076695937978,-4.79406056862158,
129.699483215374));
#243050=CARTESIAN_POINT('Ctrl Pts',(-197.083560976212,-4.81971881788819,
129.817443076));
#243051=CARTESIAN_POINT('Ctrl Pts',(-197.090426014446,-4.84098812800867,
129.936019090873));
#243052=CARTESIAN_POINT('Ctrl Pts',(-197.102330337474,-4.87787018599897,
130.14163588954));
#243053=CARTESIAN_POINT('Ctrl Pts',(-197.114234660503,-4.90165998726396,
130.349666738386));
#243054=CARTESIAN_POINT('Ctrl Pts',(-197.126138983531,-4.91211451822462,
130.558771484364));
#243055=CARTESIAN_POINT('Ctrl Pts',(-197.130712467685,-4.91613101135752,
130.639106774339));
#243056=CARTESIAN_POINT('Ctrl Pts',(-197.13528595184,-4.91817963992249,
130.719600281634));
#243057=CARTESIAN_POINT('Ctrl Pts',(-197.139859435995,-4.91824821858423,
130.80017458208));
#243058=CARTESIAN_POINT('Origin',(213.235140564004,0.,130.804360617566));
#243059=CARTESIAN_POINT('',(-195.319719904489,-4.76405452823413,129.582490119309));
#243060=CARTESIAN_POINT('',(-195.665141276266,-4.76405452823396,129.582490119308));
#243061=CARTESIAN_POINT('',(213.235140564004,-4.76405452823405,129.582490119308));
#243062=CARTESIAN_POINT('',(-195.735140564062,-4.91824801533315,130.799942227414));
#243063=CARTESIAN_POINT('Ctrl Pts',(-195.665141276266,-4.76405452823396,
129.582490119308));
#243064=CARTESIAN_POINT('Ctrl Pts',(-195.669627150585,-4.78364500634694,
129.658873096143));
#243065=CARTESIAN_POINT('Ctrl Pts',(-195.674113024903,-4.80138190659694,
129.735664461695));
#243066=CARTESIAN_POINT('Ctrl Pts',(-195.678598899222,-4.81725278166829,
129.812766597813));
#243067=CARTESIAN_POINT('Ctrl Pts',(-195.689674595893,-4.85643823041579,
130.00313302623));
#243068=CARTESIAN_POINT('Ctrl Pts',(-195.700750292564,-4.88435001913631,
130.195892860283));
#243069=CARTESIAN_POINT('Ctrl Pts',(-195.711825989234,-4.90075931060626,
130.38994386838));
#243070=CARTESIAN_POINT('Ctrl Pts',(-195.71959751416,-4.91227327866349,
130.526104354821));
#243071=CARTESIAN_POINT('Ctrl Pts',(-195.727369039086,-4.91812490136763,
130.662900256424));
#243072=CARTESIAN_POINT('Ctrl Pts',(-195.735140564012,-4.91824801533235,
130.799942226527));
#243073=CARTESIAN_POINT('Ctrl Pts',(-195.735140564062,-4.91824801533315,
130.799942227414));
#243074=CARTESIAN_POINT('Ctrl Pts',(-195.742788954033,-4.91836917860973,
130.934812853151));
#243075=CARTESIAN_POINT('Ctrl Pts',(-195.750437344004,-4.91293844047973,
131.069862221547));
#243076=CARTESIAN_POINT('Ctrl Pts',(-195.758085733975,-4.90193846711678,
131.204588461551));
#243077=CARTESIAN_POINT('Ctrl Pts',(-195.765727802631,-4.89094758511626,
131.339203351733));
#243078=CARTESIAN_POINT('Ctrl Pts',(-195.773369871288,-4.87439665663672,
131.473495244947));
#243079=CARTESIAN_POINT('Ctrl Pts',(-195.781011939945,-4.85232041130353,
131.606962441977));
#243080=CARTESIAN_POINT('Ctrl Pts',(-195.788650174382,-4.83025524218319,
131.740362675125));
#243081=CARTESIAN_POINT('Ctrl Pts',(-195.796288408819,-4.80267033378295,
131.872938638019));
#243082=CARTESIAN_POINT('Ctrl Pts',(-195.803926643255,-4.7696521975637,
132.00419434637));
#243083=CARTESIAN_POINT('Ctrl Pts',(-195.811563004816,-4.73664215730885,
132.13541787115));
#243084=CARTESIAN_POINT('Ctrl Pts',(-195.819199366377,-4.69820163590381,
132.265321394214));
#243085=CARTESIAN_POINT('Ctrl Pts',(-195.826835727938,-4.65446802695667,
132.393420228952));
#243086=CARTESIAN_POINT('Ctrl Pts',(-195.834471981253,-4.6107350379391,
132.521517247872));
#243087=CARTESIAN_POINT('Ctrl Pts',(-195.842108234567,-4.56170924103285,
132.647809247807));
#243088=CARTESIAN_POINT('Ctrl Pts',(-195.849744487881,-4.50757738476626,
132.771828325775));
#243089=CARTESIAN_POINT('Ctrl Pts',(-195.857382397285,-4.4534337888199,
132.895874299998));
#243090=CARTESIAN_POINT('Ctrl Pts',(-195.865020306688,-4.39418209327545,
133.01764600283));
#243091=CARTESIAN_POINT('Ctrl Pts',(-195.872658216092,-4.33005626833118,
133.136697594846));
#243092=CARTESIAN_POINT('Ctrl Pts',(-195.880303983217,-4.26586447207508,
133.255871664657));
#243093=CARTESIAN_POINT('Ctrl Pts',(-195.887949750342,-4.19678872589688,
133.37231968092));
#243094=CARTESIAN_POINT('Ctrl Pts',(-195.895595517468,-4.12310800759558,
133.485622152777));
#243095=CARTESIAN_POINT('Ctrl Pts',(-195.903245518399,-4.04938648895914,
133.59898736532));
#243096=CARTESIAN_POINT('Ctrl Pts',(-195.91089551933,-3.9710551549251,133.709203237835));
#243097=CARTESIAN_POINT('Ctrl Pts',(-195.918545520261,-3.88843420921999,
133.815882236792));
#243098=CARTESIAN_POINT('Ctrl Pts',(-195.926207035089,-3.8056889120232,
133.922721796641));
#243099=CARTESIAN_POINT('Ctrl Pts',(-195.933868549917,-3.71864137075232,
134.026013545911));
#243100=CARTESIAN_POINT('Ctrl Pts',(-195.941530064745,-3.62765000128713,
134.125405412606));
#243101=CARTESIAN_POINT('Ctrl Pts',(-195.946702217508,-3.56622334173219,
134.192503098836));
#243102=CARTESIAN_POINT('Ctrl Pts',(-195.951874370271,-3.50300009789946,
134.257824245905));
#243103=CARTESIAN_POINT('Ctrl Pts',(-195.957046523035,-3.43809892864949,
134.321271025768));
#243104=CARTESIAN_POINT('Ctrl Pts',(-195.964820857154,-3.34054508645473,
134.416638755225));
#243105=CARTESIAN_POINT('Ctrl Pts',(-195.972595191273,-3.23886568121659,
134.508095467405));
#243106=CARTESIAN_POINT('Ctrl Pts',(-195.980369525392,-3.13340727972664,
134.595263133044));
#243107=CARTESIAN_POINT('Ctrl Pts',(-195.988134278339,-3.02807884629143,
134.682323372325));
#243108=CARTESIAN_POINT('Ctrl Pts',(-195.995899031286,-2.91898098165016,
134.765104835671));
#243109=CARTESIAN_POINT('Ctrl Pts',(-196.003663784233,-2.80649748679672,
134.843265780986));
#243110=CARTESIAN_POINT('Ctrl Pts',(-196.011420825118,-2.69412571213581,
134.921349095749));
#243111=CARTESIAN_POINT('Ctrl Pts',(-196.019177866003,-2.5783753180853,
134.994820803471));
#243112=CARTESIAN_POINT('Ctrl Pts',(-196.026934906888,-2.45966333968881,
135.063379203801));
#243113=CARTESIAN_POINT('Ctrl Pts',(-196.034686098128,-2.34104088291883,
135.131885903706));
#243114=CARTESIAN_POINT('Ctrl Pts',(-196.042437289368,-2.21946162434935,
135.195486476388));
#243115=CARTESIAN_POINT('Ctrl Pts',(-196.050188480608,-2.09537145223453,
135.253922566754));
#243116=CARTESIAN_POINT('Ctrl Pts',(-196.057936377386,-1.9713340217529,
135.312333820223));
#243117=CARTESIAN_POINT('Ctrl Pts',(-196.065684274163,-1.84478815328316,
135.365584790931));
#243118=CARTESIAN_POINT('Ctrl Pts',(-196.07343217094,-1.71620400590661,
135.413463227902));
#243119=CARTESIAN_POINT('Ctrl Pts',(-196.081178447024,-1.58764675556175,
135.461331649737));
#243120=CARTESIAN_POINT('Ctrl Pts',(-196.088924723108,-1.45705244052956,
135.503829636831));
#243121=CARTESIAN_POINT('Ctrl Pts',(-196.096670999192,-1.32491048285849,
135.540793375973));
#243122=CARTESIAN_POINT('Ctrl Pts',(-196.104417332458,-1.19276754974533,
135.577757387973));
#243123=CARTESIAN_POINT('Ctrl Pts',(-196.112163665723,-1.05907732770887,
135.60918696518));
#243124=CARTESIAN_POINT('Ctrl Pts',(-196.119909998988,-0.92434326967486,
135.634968507087));
#243125=CARTESIAN_POINT('Ctrl Pts',(-196.127658066991,-0.789579038882551,
135.660755822592));
#243126=CARTESIAN_POINT('Ctrl Pts',(-196.135406134994,-0.653770890862492,
135.680892512449));
#243127=CARTESIAN_POINT('Ctrl Pts',(-196.143154202997,-0.517430915145343,
135.695316384137));
#243128=CARTESIAN_POINT('Ctrl Pts',(-196.150910505739,-0.380946035680092,
135.709755585687));
#243129=CARTESIAN_POINT('Ctrl Pts',(-196.158666808481,-0.243928588819814,
135.718469799092));
#243130=CARTESIAN_POINT('Ctrl Pts',(-196.166423111223,-0.106894770994205,
135.721448838295));
#243131=CARTESIAN_POINT('Ctrl Pts',(-196.174183553737,0.0302121859059867,
135.724429467501));
#243132=CARTESIAN_POINT('Ctrl Pts',(-196.181943996251,0.167335140487332,
135.721668830999));
#243133=CARTESIAN_POINT('Ctrl Pts',(-196.189704438765,0.303960473328762,
135.713208862639));
#243134=CARTESIAN_POINT('Ctrl Pts',(-196.197477339031,0.440805129283496,
135.704735313586));
#243135=CARTESIAN_POINT('Ctrl Pts',(-196.205250239296,0.577150178099871,
135.690544190408));
#243136=CARTESIAN_POINT('Ctrl Pts',(-196.213023139562,0.712488781964307,
135.670729160748));
#243137=CARTESIAN_POINT('Ctrl Pts',(-196.220513475324,0.842907486683093,
135.651634457327));
#243138=CARTESIAN_POINT('Ctrl Pts',(-196.228003811086,0.972391346940213,
135.627317691741));
#243139=CARTESIAN_POINT('Ctrl Pts',(-196.235494146848,1.10049987933717,
135.597906599204));
#243140=CARTESIAN_POINT('Ctrl Pts',(-196.243268480967,1.23346568567565,
135.567380376155));
#243141=CARTESIAN_POINT('Ctrl Pts',(-196.251042815086,1.3653710100103,135.531269199705));
#243142=CARTESIAN_POINT('Ctrl Pts',(-196.258817149205,1.49571047779856,
135.48966031226));
#243143=CARTESIAN_POINT('Ctrl Pts',(-196.266581902152,1.62588931384153,
135.448102704051));
#243144=CARTESIAN_POINT('Ctrl Pts',(-196.274346655099,1.75450576414976,
135.401060983704));
#243145=CARTESIAN_POINT('Ctrl Pts',(-196.282111408047,1.88106485760708,
135.348673333915));
#243146=CARTESIAN_POINT('Ctrl Pts',(-196.289868448932,2.00749825078861,
135.296337716279));
#243147=CARTESIAN_POINT('Ctrl Pts',(-196.297625489817,2.1318779946668,135.238666884213));
#243148=CARTESIAN_POINT('Ctrl Pts',(-196.305382530702,2.25372484256268,
135.1758486247));
#243149=CARTESIAN_POINT('Ctrl Pts',(-196.313133721942,2.37547980480323,
135.113077736925));
#243150=CARTESIAN_POINT('Ctrl Pts',(-196.320884913182,2.49470532685751,
135.045167326451));
#243151=CARTESIAN_POINT('Ctrl Pts',(-196.328636104422,2.61094303377791,
134.972352884457));
#243152=CARTESIAN_POINT('Ctrl Pts',(-196.336384001199,2.72713133657197,
134.899569390544));
#243153=CARTESIAN_POINT('Ctrl Pts',(-196.344131897976,2.8403340193372,134.82188621783));
#243154=CARTESIAN_POINT('Ctrl Pts',(-196.351879794753,2.95011837684841,
134.739584197629));
#243155=CARTESIAN_POINT('Ctrl Pts',(-196.359626070838,3.05987976983901,
134.657299393235));
#243156=CARTESIAN_POINT('Ctrl Pts',(-196.367372346922,3.16622394720568,
134.57039789747));
#243157=CARTESIAN_POINT('Ctrl Pts',(-196.375118623006,3.26874854368119,
134.479202929922));
#243158=CARTESIAN_POINT('Ctrl Pts',(-196.382864956271,3.37127389696957,
134.388007289193));
#243159=CARTESIAN_POINT('Ctrl Pts',(-196.390611289537,3.46997932098188,
134.292518373281));
#243160=CARTESIAN_POINT('Ctrl Pts',(-196.398357622802,3.56449711178872,
134.19309834754));
#243161=CARTESIAN_POINT('Ctrl Pts',(-196.406105690805,3.6590360691996,134.093656057373));
#243162=CARTESIAN_POINT('Ctrl Pts',(-196.413853758808,3.74938525798013,
133.990281188891));
#243163=CARTESIAN_POINT('Ctrl Pts',(-196.421601826811,3.83521555689988,
133.883370960941));
#243164=CARTESIAN_POINT('Ctrl Pts',(-196.429358129553,3.92113707728282,
133.776347107529));
#243165=CARTESIAN_POINT('Ctrl Pts',(-196.437114432295,4.00252986868535,
133.665780694151));
#243166=CARTESIAN_POINT('Ctrl Pts',(-196.444870735037,4.07910634450957,
133.552100505671));
#243167=CARTESIAN_POINT('Ctrl Pts',(-196.452631177551,4.1557236915046,133.438359642651));
#243168=CARTESIAN_POINT('Ctrl Pts',(-196.460391620065,4.22751939619557,
133.321502025975));
#243169=CARTESIAN_POINT('Ctrl Pts',(-196.468152062579,4.29425111487522,
133.20198244448));
#243170=CARTESIAN_POINT('Ctrl Pts',(-196.475924962845,4.36108995723385,
133.082270999541));
#243171=CARTESIAN_POINT('Ctrl Pts',(-196.48369786311,4.42284839268908,132.959889399764));
#243172=CARTESIAN_POINT('Ctrl Pts',(-196.491470763375,4.47933126826296,
132.835314691803));
#243173=CARTESIAN_POINT('Ctrl Pts',(-196.498961099137,4.53376084903658,
132.715268588265));
#243174=CARTESIAN_POINT('Ctrl Pts',(-196.506451434899,4.58329165474819,
132.593186343692));
#243175=CARTESIAN_POINT('Ctrl Pts',(-196.513941770661,4.62779306061534,
132.469507593247));
#243176=CARTESIAN_POINT('Ctrl Pts',(-196.52171610478,4.67398175081282,132.341139525385));
#243177=CARTESIAN_POINT('Ctrl Pts',(-196.529490438899,4.71489844511337,
132.210644867334));
#243178=CARTESIAN_POINT('Ctrl Pts',(-196.537264773018,4.75034337573913,
132.078495961661));
#243179=CARTESIAN_POINT('Ctrl Pts',(-196.545029525966,4.7857446236558,131.946509917703));
#243180=CARTESIAN_POINT('Ctrl Pts',(-196.552794278913,4.81568742506033,
131.812874056546));
#243181=CARTESIAN_POINT('Ctrl Pts',(-196.56055903186,4.84002049298939,131.67807950253));
#243182=CARTESIAN_POINT('Ctrl Pts',(-196.568316072745,4.86432939297227,
131.543418828366));
#243183=CARTESIAN_POINT('Ctrl Pts',(-196.57607311363,4.88303957834233,131.407602133804));
#243184=CARTESIAN_POINT('Ctrl Pts',(-196.583830154515,4.89604999507073,
131.271134126099));
#243185=CARTESIAN_POINT('Ctrl Pts',(-196.591581345755,4.90905060054271,
131.134769029979));
#243186=CARTESIAN_POINT('Ctrl Pts',(-196.599332536995,4.91635995580379,
130.997753985968));
#243187=CARTESIAN_POINT('Ctrl Pts',(-196.607083728235,4.91792842339693,
130.860601926624));
#243188=CARTESIAN_POINT('Ctrl Pts',(-196.614831625012,4.91949622434951,
130.723508160564));
#243189=CARTESIAN_POINT('Ctrl Pts',(-196.622579521789,4.91532798620717,
130.586277885118));
#243190=CARTESIAN_POINT('Ctrl Pts',(-196.630327418567,4.90542609256398,
130.449426943632));
#243191=CARTESIAN_POINT('Ctrl Pts',(-196.638073694651,4.89552627018349,
130.312604628412));
#243192=CARTESIAN_POINT('Ctrl Pts',(-196.645819970735,4.87989520608599,
130.176161879023));
#243193=CARTESIAN_POINT('Ctrl Pts',(-196.653566246819,4.85858734580939,
130.04061192484));
#243194=CARTESIAN_POINT('Ctrl Pts',(-196.661312580084,4.83727932824304,
129.905060970058));
#243195=CARTESIAN_POINT('Ctrl Pts',(-196.669058913349,4.81029449159206,
129.770403209857));
#243196=CARTESIAN_POINT('Ctrl Pts',(-196.676805246615,4.77773878287119,
129.637143763186));
#243197=CARTESIAN_POINT('Ctrl Pts',(-196.684553314618,4.74517578352494,
129.503854473986));
#243198=CARTESIAN_POINT('Ctrl Pts',(-196.692301382621,4.70703952237994,
129.371964501156));
#243199=CARTESIAN_POINT('Ctrl Pts',(-196.700049450624,4.6634862928383,129.2419654502));
#243200=CARTESIAN_POINT('Ctrl Pts',(-196.707805753366,4.61988677440618,
129.111828234706));
#243201=CARTESIAN_POINT('Ctrl Pts',(-196.715562056108,4.57085891131053,
128.98358632697));
#243202=CARTESIAN_POINT('Ctrl Pts',(-196.723318358849,4.51660800481933,
128.857713450434));
#243203=CARTESIAN_POINT('Ctrl Pts',(-196.731078801364,4.46232814298588,
128.731773391754));
#243204=CARTESIAN_POINT('Ctrl Pts',(-196.738839243878,4.40281985259029,
128.608205235819));
#243205=CARTESIAN_POINT('Ctrl Pts',(-196.746599686392,4.33833476766696,
128.487458697727));
#243206=CARTESIAN_POINT('Ctrl Pts',(-196.754372586657,4.27374616556059,
128.366518326573));
#243207=CARTESIAN_POINT('Ctrl Pts',(-196.762145486923,4.20416500253837,
128.248408961719));
#243208=CARTESIAN_POINT('Ctrl Pts',(-196.769918387188,4.12988714651096,
128.133552646262));
#243209=CARTESIAN_POINT('Ctrl Pts',(-196.77740872295,4.05830947764578,128.022871647178));
#243210=CARTESIAN_POINT('Ctrl Pts',(-196.784899058712,3.98237083808165,
127.915211542331));
#243211=CARTESIAN_POINT('Ctrl Pts',(-196.792389394474,3.90237049944579,
127.810919863592));
#243212=CARTESIAN_POINT('Ctrl Pts',(-196.800163728593,3.81933692365392,
127.702673934153));
#243213=CARTESIAN_POINT('Ctrl Pts',(-196.807938062712,3.73166454474996,
127.597714010231));
#243214=CARTESIAN_POINT('Ctrl Pts',(-196.815712396831,3.63964277854941,
127.49646347481));
#243215=CARTESIAN_POINT('Ctrl Pts',(-196.823477149778,3.54773442095174,
127.395337721625));
#243216=CARTESIAN_POINT('Ctrl Pts',(-196.831241902725,3.4514876017493,127.297912547587));
#243217=CARTESIAN_POINT('Ctrl Pts',(-196.839006655673,3.35123374346011,
127.204580699405));
#243218=CARTESIAN_POINT('Ctrl Pts',(-196.846763696558,3.25107945871658,
127.111341549731));
#243219=CARTESIAN_POINT('Ctrl Pts',(-196.854520737442,3.14692633926754,
127.022187899961));
#243220=CARTESIAN_POINT('Ctrl Pts',(-196.862277778327,3.03914438745001,
126.937477576313));
#243221=CARTESIAN_POINT('Ctrl Pts',(-196.870028969567,2.93144371484062,
126.852831133378));
#243222=CARTESIAN_POINT('Ctrl Pts',(-196.877780160808,2.82011996290654,
126.772621587719));
#243223=CARTESIAN_POINT('Ctrl Pts',(-196.885531352048,2.70557784607938,
126.697167953312));
#243224=CARTESIAN_POINT('Ctrl Pts',(-196.893279248825,2.59108441270722,
126.621746388711));
#243225=CARTESIAN_POINT('Ctrl Pts',(-196.901027145602,2.47337566088124,
126.551076929597));
#243226=CARTESIAN_POINT('Ctrl Pts',(-196.908775042379,2.35288687260822,
126.485436396512));
#243227=CARTESIAN_POINT('Ctrl Pts',(-196.916521318463,2.23242328799227,
126.419809594011));
#243228=CARTESIAN_POINT('Ctrl Pts',(-196.924267594547,2.10918116671744,
126.359209812087));
#243229=CARTESIAN_POINT('Ctrl Pts',(-196.932013870631,1.98362173233724,
126.30386865718));
#243230=CARTESIAN_POINT('Ctrl Pts',(-196.939760203896,1.85806137110565,
126.248527093757));
#243231=CARTESIAN_POINT('Ctrl Pts',(-196.947506537162,1.73018402039162,
126.198444392494));
#243232=CARTESIAN_POINT('Ctrl Pts',(-196.955252870427,1.60047191802326,
126.153804446298));
#243233=CARTESIAN_POINT('Ctrl Pts',(-196.96300093843,1.47073076752877,126.109154503295));
#243234=CARTESIAN_POINT('Ctrl Pts',(-196.970749006433,1.33915441739122,
126.069949867965));
#243235=CARTESIAN_POINT('Ctrl Pts',(-196.978497074436,1.2062409496441,126.036324771025));
#243236=CARTESIAN_POINT('Ctrl Pts',(-196.986253377178,1.07318621988194,
126.002663936931));
#243237=CARTESIAN_POINT('Ctrl Pts',(-196.99400967992,0.938791913329507,
125.974594583081));
#243238=CARTESIAN_POINT('Ctrl Pts',(-197.001765982662,0.803567557284923,
125.952200042793));
#243239=CARTESIAN_POINT('Ctrl Pts',(-197.009526425176,0.668271027929991,
125.929793549866));
#243240=CARTESIAN_POINT('Ctrl Pts',(-197.01728686769,0.532143954180493,
125.913067953334));
#243241=CARTESIAN_POINT('Ctrl Pts',(-197.025047310204,0.395700708427855,
125.902054628355));
#243242=CARTESIAN_POINT('Ctrl Pts',(-197.032820210469,0.259038431864272,
125.89102362381));
#243243=CARTESIAN_POINT('Ctrl Pts',(-197.040593110735,0.122059359953858,
125.885723230215));
#243244=CARTESIAN_POINT('Ctrl Pts',(-197.048366011,-0.0147215066600589,
125.886132650123));
#243245=CARTESIAN_POINT('Ctrl Pts',(-197.055856346762,-0.146530044246793,
125.886527186585));
#243246=CARTESIAN_POINT('Ctrl Pts',(-197.063346682525,-0.27815422914227,
125.89222359833));
#243247=CARTESIAN_POINT('Ctrl Pts',(-197.070837018287,-0.409139909314695,
125.903157949128));
#243248=CARTESIAN_POINT('Ctrl Pts',(-197.078611352406,-0.545091951359064,
125.914506879159));
#243249=CARTESIAN_POINT('Ctrl Pts',(-197.086385686525,-0.680786770288788,
125.931534731873));
#243250=CARTESIAN_POINT('Ctrl Pts',(-197.094160020644,-0.815711725690703,
125.954226862393));
#243251=CARTESIAN_POINT('Ctrl Pts',(-197.101924773591,-0.950470398142942,
125.976891026889));
#243252=CARTESIAN_POINT('Ctrl Pts',(-197.109689526538,-1.08446071302349,
126.005205515426));
#243253=CARTESIAN_POINT('Ctrl Pts',(-197.117454279485,-1.21717309943613,
126.039103782042));
#243254=CARTESIAN_POINT('Ctrl Pts',(-197.12521132037,-1.3497536740364,126.072968380422));
#243255=CARTESIAN_POINT('Ctrl Pts',(-197.132968361255,-1.48105846969448,
126.112405624185));
#243256=CARTESIAN_POINT('Ctrl Pts',(-197.14072540214,-1.61058644177957,
126.157297633696));
#243257=CARTESIAN_POINT('Ctrl Pts',(-197.148476593381,-1.74001673581351,
126.202155789794));
#243258=CARTESIAN_POINT('Ctrl Pts',(-197.156227784621,-1.86767250538385,
126.252460396493));
#243259=CARTESIAN_POINT('Ctrl Pts',(-197.163978975861,-1.99306659696161,
126.308043390926));
#243260=CARTESIAN_POINT('Ctrl Pts',(-197.171726872638,-2.11840739270528,
126.363602761105));
#243261=CARTESIAN_POINT('Ctrl Pts',(-197.179474769415,-2.24148806567971,
126.424435898852));
#243262=CARTESIAN_POINT('Ctrl Pts',(-197.187222666192,-2.3618404383649,
126.490326217355));
#243263=CARTESIAN_POINT('Ctrl Pts',(-197.194968942276,-2.48216763592822,
126.556202753023));
#243264=CARTESIAN_POINT('Ctrl Pts',(-197.20271521836,-2.59976732564188,
126.627134177688));
#243265=CARTESIAN_POINT('Ctrl Pts',(-197.210461494444,-2.71419534785042,
126.702857639851));
#243266=CARTESIAN_POINT('Ctrl Pts',(-197.21820782771,-2.82862421474047,
126.778581660986));
#243267=CARTESIAN_POINT('Ctrl Pts',(-197.225954160975,-2.93988104136766,
126.859097574447));
#243268=CARTESIAN_POINT('Ctrl Pts',(-197.23370049424,-3.0475504520959,126.944099058496));
#243269=CARTESIAN_POINT('Ctrl Pts',(-197.241448562243,-3.15524397464228,
127.029119578039));
#243270=CARTESIAN_POINT('Ctrl Pts',(-197.249196630246,-3.25934817585858,
127.118627424824));
#243271=CARTESIAN_POINT('Ctrl Pts',(-197.256944698249,-3.35948089813607,
127.21227610331));
#243272=CARTESIAN_POINT('Ctrl Pts',(-197.264701000991,-3.45972004266226,
127.306024312726));
#243273=CARTESIAN_POINT('Ctrl Pts',(-197.272457303733,-3.55597899047717,
127.403921877684));
#243274=CARTESIAN_POINT('Ctrl Pts',(-197.280213606475,-3.64791221894775,
127.505585162135));
#243275=CARTESIAN_POINT('Ctrl Pts',(-197.287974048989,-3.73989451495042,
127.607302707342));
#243276=CARTESIAN_POINT('Ctrl Pts',(-197.295734491503,-3.82754624145586,
127.712789676336));
#243277=CARTESIAN_POINT('Ctrl Pts',(-197.303494934017,-3.91056297081482,
127.821630272095));
#243278=CARTESIAN_POINT('Ctrl Pts',(-197.311267834283,-3.99371296599786,
127.930645588441));
#243279=CARTESIAN_POINT('Ctrl Pts',(-197.319040734548,-4.07221287151127,
128.043024968882));
#243280=CARTESIAN_POINT('Ctrl Pts',(-197.326813634813,-4.14580181441111,
128.158323887261));
#243281=CARTESIAN_POINT('Ctrl Pts',(-197.334303970575,-4.21671561387579,
128.269431399534));
#243282=CARTESIAN_POINT('Ctrl Pts',(-197.341794306337,-4.2830691483762,
128.383249603762));
#243283=CARTESIAN_POINT('Ctrl Pts',(-197.349284642099,-4.3446707290067,
128.499361849885));
#243284=CARTESIAN_POINT('Ctrl Pts',(-197.357505688457,-4.41228177691909,
128.626801284969));
#243285=CARTESIAN_POINT('Ctrl Pts',(-197.365726734815,-4.47436294437082,
128.757370335874));
#243286=CARTESIAN_POINT('Ctrl Pts',(-197.373947781172,-4.5306305492326,
128.890576437242));
#243287=CARTESIAN_POINT('Ctrl Pts',(-197.382149938232,-4.58676886939006,
129.023476474196));
#243288=CARTESIAN_POINT('Ctrl Pts',(-197.390352095292,-4.63712013449305,
129.159001183372));
#243289=CARTESIAN_POINT('Ctrl Pts',(-197.398554252352,-4.68144684635498,
129.296634353534));
#243290=CARTESIAN_POINT('Ctrl Pts',(-197.404177125126,-4.71183439678685,
129.390986826878));
#243291=CARTESIAN_POINT('Ctrl Pts',(-197.409799997901,-4.73939157229638,
129.48632962842));
#243292=CARTESIAN_POINT('Ctrl Pts',(-197.415422870675,-4.76405452823413,
129.582490119309));
#243293=CARTESIAN_POINT('',(-195.389859435957,-4.9182490946383,130.807344841003));
#243294=CARTESIAN_POINT('Ctrl Pts',(-195.389859435995,-4.9182490946379,
130.807344841668));
#243295=CARTESIAN_POINT('Ctrl Pts',(-195.39981971452,-4.91814286233046,
130.982424504574));
#243296=CARTESIAN_POINT('Ctrl Pts',(-195.409779993045,-4.90868858456078,
131.157218844946));
#243297=CARTESIAN_POINT('Ctrl Pts',(-195.41974027157,-4.88997301345931,
131.330998054651));
#243298=CARTESIAN_POINT('Ctrl Pts',(-195.427514605689,-4.87536487749105,
131.466638602838));
#243299=CARTESIAN_POINT('Ctrl Pts',(-195.435288939808,-4.85508562687483,
131.601885723498));
#243300=CARTESIAN_POINT('Ctrl Pts',(-195.443063273927,-4.82916220422726,
131.736227275282));
#243301=CARTESIAN_POINT('Ctrl Pts',(-195.450828026874,-4.80327072988126,
131.87040326311));
#243302=CARTESIAN_POINT('Ctrl Pts',(-195.458592779821,-4.77174899711198,
132.003675522438));
#243303=CARTESIAN_POINT('Ctrl Pts',(-195.466357532768,-4.73467576101327,
132.135536226031));
#243304=CARTESIAN_POINT('Ctrl Pts',(-195.474114573653,-4.69763934657529,
132.267265963715));
#243305=CARTESIAN_POINT('Ctrl Pts',(-195.481871614538,-4.65506250671518,
132.397586561726));
#243306=CARTESIAN_POINT('Ctrl Pts',(-195.489628655423,-4.60707511081103,
132.525999948508));
#243307=CARTESIAN_POINT('Ctrl Pts',(-195.497379846663,-4.55912390257549,
132.654316497755));
#243308=CARTESIAN_POINT('Ctrl Pts',(-195.505131037903,-4.50577039587603,
132.780728333762));
#243309=CARTESIAN_POINT('Ctrl Pts',(-195.512882229143,-4.44719429552313,
132.904752476331));
#243310=CARTESIAN_POINT('Ctrl Pts',(-195.52063012592,-4.38864309157538,
133.028723905332));
#243311=CARTESIAN_POINT('Ctrl Pts',(-195.528378022698,-4.32487387548738,
133.150309306542));
#243312=CARTESIAN_POINT('Ctrl Pts',(-195.536125919475,-4.2561144066719,
133.269045834753));
#243313=CARTESIAN_POINT('Ctrl Pts',(-195.543872195559,-4.18736932085501,
133.387757525841));
#243314=CARTESIAN_POINT('Ctrl Pts',(-195.551618471643,-4.11363625439252,
133.503621191137));
#243315=CARTESIAN_POINT('Ctrl Pts',(-195.559364747727,-4.03518864169585,
133.616199106603));
#243316=CARTESIAN_POINT('Ctrl Pts',(-195.567111080992,-3.95674044991661,
133.728777853093));
#243317=CARTESIAN_POINT('Ctrl Pts',(-195.574857414257,-3.87357786597965,
133.838070480587));
#243318=CARTESIAN_POINT('Ctrl Pts',(-195.582603747523,-3.78601709127631,
133.943669083943));
#243319=CARTESIAN_POINT('Ctrl Pts',(-195.590351815526,-3.69843670794469,
134.049291335373));
#243320=CARTESIAN_POINT('Ctrl Pts',(-195.598099883529,-3.60645642342602,
134.151217615629));
#243321=CARTESIAN_POINT('Ctrl Pts',(-195.605847951532,-3.51043180420721,
134.24907419209));
#243322=CARTESIAN_POINT('Ctrl Pts',(-195.613604254274,-3.41430512888052,
134.347034771685));
#243323=CARTESIAN_POINT('Ctrl Pts',(-195.621360557015,-3.3141258066689,
134.440916727675));
#243324=CARTESIAN_POINT('Ctrl Pts',(-195.629116859757,-3.21028565473641,
134.530383843137));
#243325=CARTESIAN_POINT('Ctrl Pts',(-195.636877302271,-3.10639008018798,
134.619898709892));
#243326=CARTESIAN_POINT('Ctrl Pts',(-195.644637744786,-2.99883008908042,
134.704993798469));
#243327=CARTESIAN_POINT('Ctrl Pts',(-195.6523981873,-2.88802866412109,134.78537474687));
#243328=CARTESIAN_POINT('Ctrl Pts',(-195.660171087565,-2.77704937087823,
134.865884729904));
#243329=CARTESIAN_POINT('Ctrl Pts',(-195.667943987831,-2.66281857163852,
134.941665234117));
#243330=CARTESIAN_POINT('Ctrl Pts',(-195.675716888096,-2.54578692477708,
135.012466129092));
#243331=CARTESIAN_POINT('Ctrl Pts',(-195.683207223858,-2.43300967306273,
135.080693233198));
#243332=CARTESIAN_POINT('Ctrl Pts',(-195.69069755962,-2.31763194379055,
135.144296336452));
#243333=CARTESIAN_POINT('Ctrl Pts',(-195.698187895382,-2.20007486704126,
135.2030938036));
#243334=CARTESIAN_POINT('Ctrl Pts',(-195.705962229501,-2.07806057799752,
135.264120594585));
#243335=CARTESIAN_POINT('Ctrl Pts',(-195.71373656362,-1.95331191468248,
135.320163459015));
#243336=CARTESIAN_POINT('Ctrl Pts',(-195.721510897739,-1.82627431925977,
135.370968239566));
#243337=CARTESIAN_POINT('Ctrl Pts',(-195.729275650686,-1.69939328631975,
135.421710407767));
#243338=CARTESIAN_POINT('Ctrl Pts',(-195.737040403634,-1.57022929355805,
135.467227192768));
#243339=CARTESIAN_POINT('Ctrl Pts',(-195.744805156581,-1.43925215945998,
135.507310360439));
#243340=CARTESIAN_POINT('Ctrl Pts',(-195.752562197466,-1.30840511369795,
135.547353716943));
#243341=CARTESIAN_POINT('Ctrl Pts',(-195.760319238351,-1.17574888177873,
135.581974082212));
#243342=CARTESIAN_POINT('Ctrl Pts',(-195.768076279236,-1.04177270297969,
135.611011499191));
#243343=CARTESIAN_POINT('Ctrl Pts',(-195.775827470476,-0.907897556659447,
135.640027018828));
#243344=CARTESIAN_POINT('Ctrl Pts',(-195.783578661716,-0.772704825255148,
135.663467887734));
#243345=CARTESIAN_POINT('Ctrl Pts',(-195.791329852956,-0.63669798852352,
135.681224234063));
#243346=CARTESIAN_POINT('Ctrl Pts',(-195.799077749733,-0.500748958325419,
135.698973033471));
#243347=CARTESIAN_POINT('Ctrl Pts',(-195.80682564651,-0.363986897864043,
135.711042065181));
#243348=CARTESIAN_POINT('Ctrl Pts',(-195.814573543287,-0.226924321449017,
135.717372770496));
#243349=CARTESIAN_POINT('Ctrl Pts',(-195.822319819371,-0.0898904155702491,
135.723702151564));
#243350=CARTESIAN_POINT('Ctrl Pts',(-195.830066095455,0.0474434909258787,
135.724295575739));
#243351=CARTESIAN_POINT('Ctrl Pts',(-195.837812371539,0.184561330431458,
135.719146490604));
#243352=CARTESIAN_POINT('Ctrl Pts',(-195.845558704805,0.321680182109967,
135.713997367458));
#243353=CARTESIAN_POINT('Ctrl Pts',(-195.85330503807,0.458582572925475,
135.703105665086));
#243354=CARTESIAN_POINT('Ctrl Pts',(-195.861051371335,0.594754406154578,
135.686516929982));
#243355=CARTESIAN_POINT('Ctrl Pts',(-195.868799439338,0.730956734121398,
135.669924479945));
#243356=CARTESIAN_POINT('Ctrl Pts',(-195.876547507341,0.866427790928436,
135.647632505728));
#243357=CARTESIAN_POINT('Ctrl Pts',(-195.884295575344,1.00066095236712,
135.619738143878));
#243358=CARTESIAN_POINT('Ctrl Pts',(-195.892051878086,1.13503677840698,
135.591814135568));
#243359=CARTESIAN_POINT('Ctrl Pts',(-195.899808180828,1.26817169752809,
135.558275924972));
#243360=CARTESIAN_POINT('Ctrl Pts',(-195.90756448357,1.39957105416255,135.519271425508));
#243361=CARTESIAN_POINT('Ctrl Pts',(-195.915324926084,1.53104054259037,
135.480246108168));
#243362=CARTESIAN_POINT('Ctrl Pts',(-195.923085368598,1.66077225312122,
135.435748815331));
#243363=CARTESIAN_POINT('Ctrl Pts',(-195.930845811113,1.78828989818289,
135.385976304478));
#243364=CARTESIAN_POINT('Ctrl Pts',(-195.938618711378,1.91601224588891,
135.336123894371));
#243365=CARTESIAN_POINT('Ctrl Pts',(-195.946391611643,2.04151306753059,
135.280979501355));
#243366=CARTESIAN_POINT('Ctrl Pts',(-195.954164511909,2.16433832944441,
135.220787075484));
#243367=CARTESIAN_POINT('Ctrl Pts',(-195.961654847671,2.28269858371017,
135.162782795908));
#243368=CARTESIAN_POINT('Ctrl Pts',(-195.969145183433,2.39857415673948,
135.100091275505));
#243369=CARTESIAN_POINT('Ctrl Pts',(-195.976635519195,2.5115846025559,135.032968644648));
#243370=CARTESIAN_POINT('Ctrl Pts',(-195.984409853314,2.6288798737734,134.963301038841));
#243371=CARTESIAN_POINT('Ctrl Pts',(-195.992184187433,2.74346002251183,
134.888638992476));
#243372=CARTESIAN_POINT('Ctrl Pts',(-195.999958521552,2.85487044664782,
134.809219890419));
#243373=CARTESIAN_POINT('Ctrl Pts',(-196.007723274499,2.9661435673931,134.729898665308));
#243374=CARTESIAN_POINT('Ctrl Pts',(-196.015488027446,3.07425442081109,
134.645832274185));
#243375=CARTESIAN_POINT('Ctrl Pts',(-196.023252780394,3.17877386526114,
134.557303433015));
#243376=CARTESIAN_POINT('Ctrl Pts',(-196.031009821279,3.2831894995255,134.468862519938));
#243377=CARTESIAN_POINT('Ctrl Pts',(-196.038766862164,3.38402052698728,
134.375968228082));
#243378=CARTESIAN_POINT('Ctrl Pts',(-196.046523903049,3.48086792546511,
134.278945707612));
#243379=CARTESIAN_POINT('Ctrl Pts',(-196.054275094289,3.57764229056651,
134.181996352578));
#243380=CARTESIAN_POINT('Ctrl Pts',(-196.062026285529,3.67043873104742,
134.080925241009));
#243381=CARTESIAN_POINT('Ctrl Pts',(-196.069777476769,3.75889266550496,
133.976096576266));
#243382=CARTESIAN_POINT('Ctrl Pts',(-196.077525373546,3.84730900468066,
133.871312466503));
#243383=CARTESIAN_POINT('Ctrl Pts',(-196.085273270323,3.93138625714945,
133.762774278175));
#243384=CARTESIAN_POINT('Ctrl Pts',(-196.0930211671,4.01079812931765,133.650881551682));
#243385=CARTESIAN_POINT('Ctrl Pts',(-196.100767443184,4.09019339023412,
133.539012230735));
#243386=CARTESIAN_POINT('Ctrl Pts',(-196.108513719268,4.16492498582819,
133.423790085964));
#243387=CARTESIAN_POINT('Ctrl Pts',(-196.116259995352,4.23470845621583,
133.30564575792));
#243388=CARTESIAN_POINT('Ctrl Pts',(-196.124006328618,4.30449244172929,
133.187500557761));
#243389=CARTESIAN_POINT('Ctrl Pts',(-196.131752661883,4.36932803031741,
133.066433467914));
#243390=CARTESIAN_POINT('Ctrl Pts',(-196.139498995149,4.42897565969853,
132.942901631505));
#243391=CARTESIAN_POINT('Ctrl Pts',(-196.147247063151,4.48863664675259,
132.819342130998));
#243392=CARTESIAN_POINT('Ctrl Pts',(-196.154995131154,4.54310719277129,
132.69331713759));
#243393=CARTESIAN_POINT('Ctrl Pts',(-196.162743199157,4.59219517872211,
132.565305393254));
#243394=CARTESIAN_POINT('Ctrl Pts',(-196.170499501899,4.64133533596847,
132.437157596512));
#243395=CARTESIAN_POINT('Ctrl Pts',(-196.178255804641,4.68508136532905,
132.307019196435));
#243396=CARTESIAN_POINT('Ctrl Pts',(-196.186012107383,4.72329033713375,
132.175386311577));
#243397=CARTESIAN_POINT('Ctrl Pts',(-196.193772549897,4.76151970221726,
132.043683170285));
#243398=CARTESIAN_POINT('Ctrl Pts',(-196.201532992411,4.79420602793986,
131.910484334337));
#243399=CARTESIAN_POINT('Ctrl Pts',(-196.209293434926,4.8212574068754,131.776296870182));
#243400=CARTESIAN_POINT('Ctrl Pts',(-196.217066335191,4.84835221108591,
131.641893996397));
#243401=CARTESIAN_POINT('Ctrl Pts',(-196.224839235456,4.86979393109643,
131.50649970938));
#243402=CARTESIAN_POINT('Ctrl Pts',(-196.232612135722,4.88554239271103,
131.370627861474));
#243403=CARTESIAN_POINT('Ctrl Pts',(-196.240102471484,4.900718358078,131.23969529748));
#243404=CARTESIAN_POINT('Ctrl Pts',(-196.247592807246,4.91060778408717,
131.108319598021));
#243405=CARTESIAN_POINT('Ctrl Pts',(-196.255083143008,4.91522052013289,
130.976959287794));
#243406=CARTESIAN_POINT('Ctrl Pts',(-196.262857477127,4.92000814946778,
130.84061841148));
#243407=CARTESIAN_POINT('Ctrl Pts',(-196.270631811246,4.91912622449037,
130.703862227485));
#243408=CARTESIAN_POINT('Ctrl Pts',(-196.278406145365,4.91252874026042,
130.567201517771));
#243409=CARTESIAN_POINT('Ctrl Pts',(-196.286170898312,4.90593938684015,
130.430709230169));
#243410=CARTESIAN_POINT('Ctrl Pts',(-196.293935651259,4.89364850813207,
130.294312569492));
#243411=CARTESIAN_POINT('Ctrl Pts',(-196.301700404207,4.87566199954319,
130.158525399642));
#243412=CARTESIAN_POINT('Ctrl Pts',(-196.309457445092,4.85769335540821,
130.022873095524));
#243413=CARTESIAN_POINT('Ctrl Pts',(-196.317214485976,4.8340403900447,129.88782946262));
#243414=CARTESIAN_POINT('Ctrl Pts',(-196.324971526861,4.8047609802586,129.753905961198));
#243415=CARTESIAN_POINT('Ctrl Pts',(-196.332722718102,4.77550365030315,
129.620083452531));
#243416=CARTESIAN_POINT('Ctrl Pts',(-196.340473909342,4.74062840441648,
129.48737977442));
#243417=CARTESIAN_POINT('Ctrl Pts',(-196.348225100582,4.70024459204801,
129.35629852034));
#243418=CARTESIAN_POINT('Ctrl Pts',(-196.355972997359,4.65987794387701,
129.225272979288));
#243419=CARTESIAN_POINT('Ctrl Pts',(-196.363720894136,4.61400750073638,
129.095868863611));
#243420=CARTESIAN_POINT('Ctrl Pts',(-196.371468790913,4.56279303762065,
128.968576654693));
#243421=CARTESIAN_POINT('Ctrl Pts',(-196.379215066997,4.51158928746668,
128.841311072562));
#243422=CARTESIAN_POINT('Ctrl Pts',(-196.386961343081,4.45504388664914,
128.716156880974));
#243423=CARTESIAN_POINT('Ctrl Pts',(-196.394707619166,4.39336538774464,
128.593586175822));
#243424=CARTESIAN_POINT('Ctrl Pts',(-196.402453952431,4.33168643354339,
128.471014565882));
#243425=CARTESIAN_POINT('Ctrl Pts',(-196.410200285696,4.26487448138624,
128.351026829673));
#243426=CARTESIAN_POINT('Ctrl Pts',(-196.417946618962,4.19318464946682,
128.234071614754));
#243427=CARTESIAN_POINT('Ctrl Pts',(-196.425694686965,4.1214787631067,128.117090208526));
#243428=CARTESIAN_POINT('Ctrl Pts',(-196.433442754968,4.04489302757999,
128.003143008206));
#243429=CARTESIAN_POINT('Ctrl Pts',(-196.441190822971,3.96372637703559,
127.892650420707));
#243430=CARTESIAN_POINT('Ctrl Pts',(-196.448947125713,3.88247346160899,
127.782040400371));
#243431=CARTESIAN_POINT('Ctrl Pts',(-196.456703428454,3.79663013733879,
127.674892642869));
#243432=CARTESIAN_POINT('Ctrl Pts',(-196.464459731196,3.70653654583702,
127.571595563178));
#243433=CARTESIAN_POINT('Ctrl Pts',(-196.47222017371,3.6163948686728,127.468243350725));
#243434=CARTESIAN_POINT('Ctrl Pts',(-196.479980616225,3.52199867306387,
127.368746194777));
#243435=CARTESIAN_POINT('Ctrl Pts',(-196.487741058739,3.42372489016486,
127.273455501457));
#243436=CARTESIAN_POINT('Ctrl Pts',(-196.495513959004,3.32529334946519,
127.178011839056));
#243437=CARTESIAN_POINT('Ctrl Pts',(-196.50328685927,3.22297207464116,127.086788393428));
#243438=CARTESIAN_POINT('Ctrl Pts',(-196.511059759535,3.11717166908787,
127.000096714005));
#243439=CARTESIAN_POINT('Ctrl Pts',(-196.518550095297,3.01521737477187,
126.916556495492));
#243440=CARTESIAN_POINT('Ctrl Pts',(-196.526040431059,2.91003275438475,
126.837224466721));
#243441=CARTESIAN_POINT('Ctrl Pts',(-196.533530766821,2.80200890157942,
126.762340184915));
#243442=CARTESIAN_POINT('Ctrl Pts',(-196.54130510094,2.68988929156167,126.684616642804));
#243443=CARTESIAN_POINT('Ctrl Pts',(-196.549079435059,2.57435573883828,
126.61143857336));
#243444=CARTESIAN_POINT('Ctrl Pts',(-196.556853769178,2.45581311194474,
126.543120771969));
#243445=CARTESIAN_POINT('Ctrl Pts',(-196.564618522125,2.33741657824439,
126.474887166163));
#243446=CARTESIAN_POINT('Ctrl Pts',(-196.572383275073,2.2160186845002,126.411502103747));
#243447=CARTESIAN_POINT('Ctrl Pts',(-196.58014802802,2.09205494557583,126.353238380737));
#243448=CARTESIAN_POINT('Ctrl Pts',(-196.587905068905,1.96821432918454,
126.295032526079));
#243449=CARTESIAN_POINT('Ctrl Pts',(-196.59566210979,1.84181329065324,126.241938053517));
#243450=CARTESIAN_POINT('Ctrl Pts',(-196.603419150675,1.71331341981801,
126.194182726424));
#243451=CARTESIAN_POINT('Ctrl Pts',(-196.611170341915,1.58491045173478,
126.146463411995));
#243452=CARTESIAN_POINT('Ctrl Pts',(-196.618921533155,1.45441216669993,
126.104075364592));
#243453=CARTESIAN_POINT('Ctrl Pts',(-196.626672724395,1.32230135821319,
126.067198789998));
#243454=CARTESIAN_POINT('Ctrl Pts',(-196.634420621172,1.19024670034405,
126.030337888932));
#243455=CARTESIAN_POINT('Ctrl Pts',(-196.642168517949,1.05658125794433,
125.99898390647));
#243456=CARTESIAN_POINT('Ctrl Pts',(-196.649916414726,0.921804049182246,
125.973267536553));
#243457=CARTESIAN_POINT('Ctrl Pts',(-196.65766269081,0.78705503290714,125.947556545946));
#243458=CARTESIAN_POINT('Ctrl Pts',(-196.665408966895,0.651195096632955,
125.927480895489));
#243459=CARTESIAN_POINT('Ctrl Pts',(-196.673155242979,0.514734155767422,
125.913120303353));
#243460=CARTESIAN_POINT('Ctrl Pts',(-196.680901576244,0.378272207578036,
125.89875960521));
#243461=CARTESIAN_POINT('Ctrl Pts',(-196.688647909509,0.241209634762758,
125.890114090488));
#243462=CARTESIAN_POINT('Ctrl Pts',(-196.696394242775,0.104061794833803,
125.88721162599));
#243463=CARTESIAN_POINT('Ctrl Pts',(-196.704142310778,-0.0331167584028003,
125.884308511505));
#243464=CARTESIAN_POINT('Ctrl Pts',(-196.711890378781,-0.170380225947006,
125.887151014736));
#243465=CARTESIAN_POINT('Ctrl Pts',(-196.719638446784,-0.307213326347598,
125.895714874124));
#243466=CARTESIAN_POINT('Ctrl Pts',(-196.727394749525,-0.444191854595816,
125.904287835283));
#243467=CARTESIAN_POINT('Ctrl Pts',(-196.735151052267,-0.580738711172077,
125.918594275041));
#243468=CARTESIAN_POINT('Ctrl Pts',(-196.742907355009,-0.716343256706872,
125.93855797041));
#243469=CARTESIAN_POINT('Ctrl Pts',(-196.750667797523,-0.852020178470593,
125.958532321004));
#243470=CARTESIAN_POINT('Ctrl Pts',(-196.758428240037,-0.986753403156911,
125.984169870666));
#243471=CARTESIAN_POINT('Ctrl Pts',(-196.766188682552,-1.12004354234743,
126.015343440133));
#243472=CARTESIAN_POINT('Ctrl Pts',(-196.773961582817,-1.25354765070231,
126.046567052181));
#243473=CARTESIAN_POINT('Ctrl Pts',(-196.781734483082,-1.38560366746973,
126.083344337961));
#243474=CARTESIAN_POINT('Ctrl Pts',(-196.789507383348,-1.51572753612455,
126.125498245286));
#243475=CARTESIAN_POINT('Ctrl Pts',(-196.79699771911,-1.64112107439117,
126.166119751901));
#243476=CARTESIAN_POINT('Ctrl Pts',(-196.804488054872,-1.76472021359313,
126.211733652672));
#243477=CARTESIAN_POINT('Ctrl Pts',(-196.811978390634,-1.88611201178001,
126.262140395965));
#243478=CARTESIAN_POINT('Ctrl Pts',(-196.819753120516,-2.01211283081602,
126.31446098957));
#243479=CARTESIAN_POINT('Ctrl Pts',(-196.827527850399,-2.13613453277524,
126.372111311885));
#243480=CARTESIAN_POINT('Ctrl Pts',(-196.835302580282,-2.25769335655606,
126.434920862831));
#243481=CARTESIAN_POINT('Ctrl Pts',(-196.84306763844,-2.37910096178886,
126.49765227902));
#243482=CARTESIAN_POINT('Ctrl Pts',(-196.850832696599,-2.49805144108238,
126.565529975486));
#243483=CARTESIAN_POINT('Ctrl Pts',(-196.858597754758,-2.61407982358089,
126.638334964927));
#243484=CARTESIAN_POINT('Ctrl Pts',(-196.866355010688,-2.72999162227744,
126.711066800866));
#243485=CARTESIAN_POINT('Ctrl Pts',(-196.874112266618,-2.84298683835341,
126.788715870278));
#243486=CARTESIAN_POINT('Ctrl Pts',(-196.881869522548,-2.95262431338359,
126.871016909407));
#243487=CARTESIAN_POINT('Ctrl Pts',(-196.889701246598,-3.06331428645066,
126.954108022204));
#243488=CARTESIAN_POINT('Ctrl Pts',(-196.897532970648,-3.17058134690447,
127.041940717171));
#243489=CARTESIAN_POINT('Ctrl Pts',(-196.905364694697,-3.27400009449339,
127.134196255612));
#243490=CARTESIAN_POINT('Ctrl Pts',(-196.913112250324,-3.37630738911646,
127.225460313357));
#243491=CARTESIAN_POINT('Ctrl Pts',(-196.92085980595,-3.47484838652523,
127.321052344723));
#243492=CARTESIAN_POINT('Ctrl Pts',(-196.928607361577,-3.56924381249012,
127.420622792394));
#243493=CARTESIAN_POINT('Ctrl Pts',(-196.936353185915,-3.66361814461469,
127.520170989801));
#243494=CARTESIAN_POINT('Ctrl Pts',(-196.944099010253,-3.75384847999537,
127.623695550915));
#243495=CARTESIAN_POINT('Ctrl Pts',(-196.951844834592,-3.83959259305698,
127.730810263034));
#243496=CARTESIAN_POINT('Ctrl Pts',(-196.959590605432,-3.92533611390858,
127.837924235343));
#243497=CARTESIAN_POINT('Ctrl Pts',(-196.967336376272,-4.00659323053975,
127.948628003653));
#243498=CARTESIAN_POINT('Ctrl Pts',(-196.975082147112,-4.08306244107213,
128.062502823149));
#243499=CARTESIAN_POINT('Ctrl Pts',(-196.982977876498,-4.16101209969199,
128.178582265363));
#243500=CARTESIAN_POINT('Ctrl Pts',(-196.990873605884,-4.23398630132602,
128.297956468713));
#243501=CARTESIAN_POINT('Ctrl Pts',(-196.99876933527,-4.30171285759348,
128.420152247202));
#243502=CARTESIAN_POINT('Ctrl Pts',(-197.006523360613,-4.36822393061056,
128.540154987535));
#243503=CARTESIAN_POINT('Ctrl Pts',(-197.014277385956,-4.42967400356862,
128.662878498698));
#243504=CARTESIAN_POINT('Ctrl Pts',(-197.0220314113,-4.48585278789196,128.787851795899));
#243505=CARTESIAN_POINT('Ctrl Pts',(-197.029997992707,-4.54357156476701,
128.916250904981));
#243506=CARTESIAN_POINT('Ctrl Pts',(-197.037964574115,-4.59572572575124,
129.047024507953));
#243507=CARTESIAN_POINT('Ctrl Pts',(-197.045931155522,-4.64214130697621,
129.179643057938));
#243508=CARTESIAN_POINT('Ctrl Pts',(-197.053897736929,-4.68855688820118,
129.312261607922));
#243509=CARTESIAN_POINT('Ctrl Pts',(-197.061864318336,-4.72923380978975,
129.446724666572));
#243510=CARTESIAN_POINT('Ctrl Pts',(-197.069830899744,-4.76405452823391,
129.582490119308));
#243511=CARTESIAN_POINT('Ctrl Pts',(-195.319719904489,-4.76405452823413,
129.582490119309));
#243512=CARTESIAN_POINT('Ctrl Pts',(-195.327375268945,-4.79771771013328,
129.713742354623));
#243513=CARTESIAN_POINT('Ctrl Pts',(-195.335030633401,-4.82593039702568,
129.846300244023));
#243514=CARTESIAN_POINT('Ctrl Pts',(-195.342685997857,-4.84861431659377,
129.979665357836));
#243515=CARTESIAN_POINT('Ctrl Pts',(-195.35054823754,-4.87191123650242,
130.116634472268));
#243516=CARTESIAN_POINT('Ctrl Pts',(-195.358410477224,-4.88937627244404,
130.25445460389));
#243517=CARTESIAN_POINT('Ctrl Pts',(-195.366272716907,-4.90098169012487,
130.392582114532));
#243518=CARTESIAN_POINT('Ctrl Pts',(-195.37413495659,-4.91258710780571,
130.530709625174));
#243519=CARTESIAN_POINT('Ctrl Pts',(-195.381997196274,-4.91833295009223,
130.669144059767));
#243520=CARTESIAN_POINT('Ctrl Pts',(-195.389859435957,-4.9182490946383,
130.807344841003));
#243521=CARTESIAN_POINT('Origin',(213.235140564004,0.,130.804360617566));
#243522=CARTESIAN_POINT('',(-193.570047426085,-4.7640545282341,129.582490119308));
#243523=CARTESIAN_POINT('',(-193.914998640423,-4.76405452823412,129.582490119309));
#243524=CARTESIAN_POINT('',(213.235140564004,-4.76405452823405,129.582490119308));
#243525=CARTESIAN_POINT('',(-193.985140563976,-4.91824942956879,130.80672938227));
#243526=CARTESIAN_POINT('Ctrl Pts',(-193.914998640423,-4.76405452823412,
129.582490119309));
#243527=CARTESIAN_POINT('Ctrl Pts',(-193.92267052425,-4.79777746561117,
129.713975340325));
#243528=CARTESIAN_POINT('Ctrl Pts',(-193.930342408077,-4.82602859703584,
129.84676320345));
#243529=CARTESIAN_POINT('Ctrl Pts',(-193.938014291904,-4.84873130167584,
129.980353441233));
#243530=CARTESIAN_POINT('Ctrl Pts',(-193.945868670583,-4.87197404665051,
130.117121455314));
#243531=CARTESIAN_POINT('Ctrl Pts',(-193.953723049261,-4.88940102937192,
130.254730049252));
#243532=CARTESIAN_POINT('Ctrl Pts',(-193.96157742794,-4.90098647655538,
130.392639086527));
#243533=CARTESIAN_POINT('Ctrl Pts',(-193.969431806619,-4.91257192373883,
130.530548123802));
#243534=CARTESIAN_POINT('Ctrl Pts',(-193.977286185297,-4.91831588080072,
130.668757158678));
#243535=CARTESIAN_POINT('Ctrl Pts',(-193.985140563975,-4.91824942956879,
130.806729382271));
#243536=CARTESIAN_POINT('Ctrl Pts',(-193.985140564012,-4.91824942956849,
130.806729382913));
#243537=CARTESIAN_POINT('Ctrl Pts',(-193.992731428123,-4.91818520775937,
130.940072635538));
#243538=CARTESIAN_POINT('Ctrl Pts',(-194.000322292233,-4.91269870967798,
131.073280898492));
#243539=CARTESIAN_POINT('Ctrl Pts',(-194.007913156344,-4.90181963422078,
131.206041256965));
#243540=CARTESIAN_POINT('Ctrl Pts',(-194.015687490463,-4.89067761319646,
131.342010412719));
#243541=CARTESIAN_POINT('Ctrl Pts',(-194.023461824582,-4.87385628461547,
131.47773098801));
#243542=CARTESIAN_POINT('Ctrl Pts',(-194.031236158701,-4.85136951318697,
131.612690320732));
#243543=CARTESIAN_POINT('Ctrl Pts',(-194.039000911648,-4.82891045469462,
131.747483328137));
#243544=CARTESIAN_POINT('Ctrl Pts',(-194.046765664595,-4.80079990939565,
131.881516577692));
#243545=CARTESIAN_POINT('Ctrl Pts',(-194.054530417543,-4.76710364769382,
132.014280397818));
#243546=CARTESIAN_POINT('Ctrl Pts',(-194.062287458428,-4.73344085359424,
132.146912355046));
#243547=CARTESIAN_POINT('Ctrl Pts',(-194.070044499313,-4.69420347904607,
132.278277015427));
#243548=CARTESIAN_POINT('Ctrl Pts',(-194.077801540198,-4.64950864104312,
132.407873155517));
#243549=CARTESIAN_POINT('Ctrl Pts',(-194.085552731438,-4.604847507765,132.53737156615));
#243550=CARTESIAN_POINT('Ctrl Pts',(-194.093303922678,-4.55473722966819,
132.665103742946));
#243551=CARTESIAN_POINT('Ctrl Pts',(-194.101055113918,-4.49934512806033,
132.790582277175));
#243552=CARTESIAN_POINT('Ctrl Pts',(-194.108803010695,-4.44397656957337,
132.91600747968));
#243553=CARTESIAN_POINT('Ctrl Pts',(-194.116550907472,-4.38333081010158,
133.039180587809));
#243554=CARTESIAN_POINT('Ctrl Pts',(-194.124298804249,-4.3176237237225,
133.159633094977));
#243555=CARTESIAN_POINT('Ctrl Pts',(-194.132045080334,-4.25193038184923,
133.280060406077));
#243556=CARTESIAN_POINT('Ctrl Pts',(-194.139791356418,-4.18117800603018,
133.397767905166));
#243557=CARTESIAN_POINT('Ctrl Pts',(-194.147537632502,-4.10562877152469,
133.512311033089));
#243558=CARTESIAN_POINT('Ctrl Pts',(-194.155283965767,-4.03007897933201,
133.626855006542));
#243559=CARTESIAN_POINT('Ctrl Pts',(-194.163030299033,-3.94973247305859,
133.73823423585));
#243560=CARTESIAN_POINT('Ctrl Pts',(-194.170776632298,-3.86489494195318,
133.846032879688));
#243561=CARTESIAN_POINT('Ctrl Pts',(-194.178524700301,-3.78003841207102,
133.953855664285));
#243562=CARTESIAN_POINT('Ctrl Pts',(-194.186272768304,-3.69068909780753,
134.058095960657));
#243563=CARTESIAN_POINT('Ctrl Pts',(-194.194020836307,-3.59719291272284,
134.158371084329));
#243564=CARTESIAN_POINT('Ctrl Pts',(-194.201777139049,-3.50359735877989,
134.258752781596));
#243565=CARTESIAN_POINT('Ctrl Pts',(-194.209533441791,-3.40584639691667,
134.355160601374));
#243566=CARTESIAN_POINT('Ctrl Pts',(-194.217289744533,-3.30432313691359,
134.447248437601));
#243567=CARTESIAN_POINT('Ctrl Pts',(-194.225050187047,-3.20274569088985,
134.539385423878));
#243568=CARTESIAN_POINT('Ctrl Pts',(-194.232810629561,-3.09739223505416,
134.627197582094));
#243569=CARTESIAN_POINT('Ctrl Pts',(-194.240571072075,-2.9886781026604,
134.71037985218));
#243570=CARTESIAN_POINT('Ctrl Pts',(-194.248343972341,-2.87978945269014,
134.793695653831));
#243571=CARTESIAN_POINT('Ctrl Pts',(-194.256116872606,-2.76752966587593,
134.87236649073));
#243572=CARTESIAN_POINT('Ctrl Pts',(-194.263889772872,-2.65234287085514,
134.946130813741));
#243573=CARTESIAN_POINT('Ctrl Pts',(-194.271380108634,-2.54134340597169,
135.01721361781));
#243574=CARTESIAN_POINT('Ctrl Pts',(-194.278870444396,-2.427626312325,135.083740287406));
#243575=CARTESIAN_POINT('Ctrl Pts',(-194.286360780158,-2.31160794777514,
135.145518499777));
#243576=CARTESIAN_POINT('Ctrl Pts',(-194.294135114277,-2.19119071166986,
135.209639051847));
#243577=CARTESIAN_POINT('Ctrl Pts',(-194.301909448396,-2.06791280888925,
135.268847077811));
#243578=CARTESIAN_POINT('Ctrl Pts',(-194.309683782515,-1.94221305079689,
135.32287713605));
#243579=CARTESIAN_POINT('Ctrl Pts',(-194.317448535462,-1.81666820642226,
135.376840607072));
#243580=CARTESIAN_POINT('Ctrl Pts',(-194.325213288409,-1.68870780118061,
135.425638654508));
#243581=CARTESIAN_POINT('Ctrl Pts',(-194.332978041356,-1.55879618671472,
135.469051122925));
#243582=CARTESIAN_POINT('Ctrl Pts',(-194.340735082241,-1.42901360229611,
135.512420473466));
#243583=CARTESIAN_POINT('Ctrl Pts',(-194.348492123126,-1.29728403370762,
135.550414766694));
#243584=CARTESIAN_POINT('Ctrl Pts',(-194.356249164011,-1.1640924790234,
135.582861612939));
#243585=CARTESIAN_POINT('Ctrl Pts',(-194.364000355251,-1.03100136512646,
135.615283990765));
#243586=CARTESIAN_POINT('Ctrl Pts',(-194.371751546491,-0.896450837902563,
135.642167156194));
#243587=CARTESIAN_POINT('Ctrl Pts',(-194.379502737732,-0.760941409372517,
135.66338842506));
#243588=CARTESIAN_POINT('Ctrl Pts',(-194.387250634509,-0.625489575964244,
135.684600674321));
#243589=CARTESIAN_POINT('Ctrl Pts',(-194.394998531286,-0.489080037301672,
135.700155752914));
#243590=CARTESIAN_POINT('Ctrl Pts',(-194.402746428063,-0.352223646456436,
135.709982042562));
#243591=CARTESIAN_POINT('Ctrl Pts',(-194.410492704147,-0.215395883017882,
135.719806276762));
#243592=CARTESIAN_POINT('Ctrl Pts',(-194.418238980231,-0.0781218430315514,
135.723904077597));
#243593=CARTESIAN_POINT('Ctrl Pts',(-194.425985256315,0.0590827411620631,
135.722255725455));
#243594=CARTESIAN_POINT('Ctrl Pts',(-194.433731589581,0.196288338168563,
135.720607361145));
#243595=CARTESIAN_POINT('Ctrl Pts',(-194.441477922846,0.333424087422282,
135.713212763916));
#243596=CARTESIAN_POINT('Ctrl Pts',(-194.449224256111,0.469974897333745,
135.700104346396));
#243597=CARTESIAN_POINT('Ctrl Pts',(-194.456972324114,0.606556286852497,
135.686992993336));
#243598=CARTESIAN_POINT('Ctrl Pts',(-194.464720392117,0.742552087266234,
135.668165311142));
#243599=CARTESIAN_POINT('Ctrl Pts',(-194.47246846012,0.877453360560609,
135.643705476381));
#243600=CARTESIAN_POINT('Ctrl Pts',(-194.480224762862,1.0124980085334,135.619219645417));
#243601=CARTESIAN_POINT('Ctrl Pts',(-194.487981065604,1.1464454203106,135.589089774232));
#243602=CARTESIAN_POINT('Ctrl Pts',(-194.495737368346,1.27879732686596,
135.553451105154));
#243603=CARTESIAN_POINT('Ctrl Pts',(-194.50349781086,1.41121987361924,135.517793414645));
#243604=CARTESIAN_POINT('Ctrl Pts',(-194.511258253374,1.54204484557664,
135.476621184933));
#243605=CARTESIAN_POINT('Ctrl Pts',(-194.519018695888,1.67079108929357,
135.430118955227));
#243606=CARTESIAN_POINT('Ctrl Pts',(-194.526791596154,1.79974400791011,
135.383542076013));
#243607=CARTESIAN_POINT('Ctrl Pts',(-194.534564496419,1.92661116793729,
135.33161824699));
#243608=CARTESIAN_POINT('Ctrl Pts',(-194.542337396684,2.05093245830343,
135.274579752461));
#243609=CARTESIAN_POINT('Ctrl Pts',(-194.549827732446,2.17073435661631,
135.21961475088));
#243610=CARTESIAN_POINT('Ctrl Pts',(-194.557318068208,2.28817199468981,
135.159900629281));
#243611=CARTESIAN_POINT('Ctrl Pts',(-194.56480840397,2.40285851435058,135.095683726179));
#243612=CARTESIAN_POINT('Ctrl Pts',(-194.572582738089,2.52189340826435,
135.029032019675));
#243613=CARTESIAN_POINT('Ctrl Pts',(-194.580357072209,2.63834151504885,
134.957318212925));
#243614=CARTESIAN_POINT('Ctrl Pts',(-194.588131406328,2.75174232289214,
134.880768012676));
#243615=CARTESIAN_POINT('Ctrl Pts',(-194.595896159275,2.86500337437468,
134.804312153707));
#243616=CARTESIAN_POINT('Ctrl Pts',(-194.603660912222,2.97522427835457,
134.723031977348));
#243617=CARTESIAN_POINT('Ctrl Pts',(-194.611425665169,3.08196881842492,
134.637199156398));
#243618=CARTESIAN_POINT('Ctrl Pts',(-194.619182706054,3.18860733831322,
134.551451585816));
#243619=CARTESIAN_POINT('Ctrl Pts',(-194.626939746939,3.29177606275606,
134.461160612539));
#243620=CARTESIAN_POINT('Ctrl Pts',(-194.634696787824,3.39106780213559,
134.366641098356));
#243621=CARTESIAN_POINT('Ctrl Pts',(-194.642447979064,3.49028466484221,
134.272192862074));
#243622=CARTESIAN_POINT('Ctrl Pts',(-194.650199170304,3.58563007983292,
134.173522700424));
#243623=CARTESIAN_POINT('Ctrl Pts',(-194.657950361544,3.6767302904695,134.070985394556));
#243624=CARTESIAN_POINT('Ctrl Pts',(-194.665698258321,3.76779178108626,
133.968491669778));
#243625=CARTESIAN_POINT('Ctrl Pts',(-194.673446155098,3.85461139688462,
133.862134361516));
#243626=CARTESIAN_POINT('Ctrl Pts',(-194.681194051876,3.93685275481512,
133.752304553499));
#243627=CARTESIAN_POINT('Ctrl Pts',(-194.68894032796,4.01907690962669,133.64249771951));
#243628=CARTESIAN_POINT('Ctrl Pts',(-194.696686604044,4.09672447724247,
133.529220143312));
#243629=CARTESIAN_POINT('Ctrl Pts',(-194.704432880128,4.1695001010668,133.412895066199));
#243630=CARTESIAN_POINT('Ctrl Pts',(-194.712179213393,4.24227626210415,
133.2965691304));
#243631=CARTESIAN_POINT('Ctrl Pts',(-194.719925546659,4.31018020022778,
133.177195980241));
#243632=CARTESIAN_POINT('Ctrl Pts',(-194.727671879924,4.3729607655146,133.055226496682));
#243633=CARTESIAN_POINT('Ctrl Pts',(-194.735419947927,4.43575539007363,
132.933229698903));
#243634=CARTESIAN_POINT('Ctrl Pts',(-194.74316801593,4.49342417982122,132.808635758297));
#243635=CARTESIAN_POINT('Ctrl Pts',(-194.750916083933,4.54576286146099,
132.681918358319));
#243636=CARTESIAN_POINT('Ctrl Pts',(-194.758672386675,4.59815716927451,
132.555066281581));
#243637=CARTESIAN_POINT('Ctrl Pts',(-194.766428689417,4.64520990323737,
132.426086599126));
#243638=CARTESIAN_POINT('Ctrl Pts',(-194.774184992159,4.68676551997081,
132.295471620581));
#243639=CARTESIAN_POINT('Ctrl Pts',(-194.781945434673,4.72834331618813,
132.164786928889));
#243640=CARTESIAN_POINT('Ctrl Pts',(-194.789705877187,4.76441804619331,
132.032465578979));
#243641=CARTESIAN_POINT('Ctrl Pts',(-194.797466319701,4.79488489286097,
131.899012126821));
#243642=CARTESIAN_POINT('Ctrl Pts',(-194.805239219967,4.82540064761563,
131.765344443334));
#243643=CARTESIAN_POINT('Ctrl Pts',(-194.813012120232,4.85029045859629,
131.630541410641));
#243644=CARTESIAN_POINT('Ctrl Pts',(-194.820785020498,4.86950105189414,
131.495115688559));
#243645=CARTESIAN_POINT('Ctrl Pts',(-194.82827535626,4.88801329173705,131.36461303259));
#243646=CARTESIAN_POINT('Ctrl Pts',(-194.835765692022,4.90125202199734,
131.233532480348));
#243647=CARTESIAN_POINT('Ctrl Pts',(-194.843256027784,4.90921538795057,
131.102332658552));
#243648=CARTESIAN_POINT('Ctrl Pts',(-194.851030361903,4.91748068734433,
130.966158355635));
#243649=CARTESIAN_POINT('Ctrl Pts',(-194.858804696022,4.92008887680447,
130.82942420116));
#243650=CARTESIAN_POINT('Ctrl Pts',(-194.866579030141,4.91698093192857,
130.692639636767));
#243651=CARTESIAN_POINT('Ctrl Pts',(-194.874343783088,4.91387681731697,
130.556023647124));
#243652=CARTESIAN_POINT('Ctrl Pts',(-194.882108536035,4.90507059386854,
130.419357758287));
#243653=CARTESIAN_POINT('Ctrl Pts',(-194.889873288982,4.89055504197982,
130.283155817256));
#243654=CARTESIAN_POINT('Ctrl Pts',(-194.897630329867,4.87605390714187,
130.147089153914));
#243655=CARTESIAN_POINT('Ctrl Pts',(-194.905387370752,4.85585476974856,
130.011485907615));
#243656=CARTESIAN_POINT('Ctrl Pts',(-194.913144411637,4.83000243600482,
129.876858849003));
#243657=CARTESIAN_POINT('Ctrl Pts',(-194.920895602877,4.80416959770702,
129.742333313703));
#243658=CARTESIAN_POINT('Ctrl Pts',(-194.928646794117,4.77269212197063,
129.608782883225));
#243659=CARTESIAN_POINT('Ctrl Pts',(-194.936397985358,4.73566647163151,
129.476713777489));
#243660=CARTESIAN_POINT('Ctrl Pts',(-194.944145882135,4.69865655818142,
129.344700804647));
#243661=CARTESIAN_POINT('Ctrl Pts',(-194.951893778912,4.6561032655712,129.214168279979));
#243662=CARTESIAN_POINT('Ctrl Pts',(-194.959641675689,4.6081538003628,129.08561060238));
#243663=CARTESIAN_POINT('Ctrl Pts',(-194.967387951773,4.56021436514899,
128.957079816276));
#243664=CARTESIAN_POINT('Ctrl Pts',(-194.975134227857,4.50688113905005,
128.830523421655));
#243665=CARTESIAN_POINT('Ctrl Pts',(-194.982880503941,4.44835055949762,
128.706418682641));
#243666=CARTESIAN_POINT('Ctrl Pts',(-194.990626837206,4.38981954788566,
128.582313027514));
#243667=CARTESIAN_POINT('Ctrl Pts',(-194.998373170472,4.32609127303541,
128.460659417719));
#243668=CARTESIAN_POINT('Ctrl Pts',(-195.006119503737,4.25740932120014,
128.341912864971));
#243669=CARTESIAN_POINT('Ctrl Pts',(-195.01386757174,4.18871198851806,128.223139719757));
#243670=CARTESIAN_POINT('Ctrl Pts',(-195.021615639743,4.11505896709885,
128.107275265403));
#243671=CARTESIAN_POINT('Ctrl Pts',(-195.029363707746,4.03673836554418,
127.994747400299));
#243672=CARTESIAN_POINT('Ctrl Pts',(-195.037120010488,3.95833452392204,
127.88209993924));
#243673=CARTESIAN_POINT('Ctrl Pts',(-195.04487631323,3.87525341621253,127.772796472684));
#243674=CARTESIAN_POINT('Ctrl Pts',(-195.052632615971,3.78782516145076,
127.667233969058));
#243675=CARTESIAN_POINT('Ctrl Pts',(-195.060393058486,3.70035024359701,
127.561615123545));
#243676=CARTESIAN_POINT('Ctrl Pts',(-195.068153501,3.60852381712407,127.459741509747));
#243677=CARTESIAN_POINT('Ctrl Pts',(-195.075913943514,3.51271372304341,
127.361974038107));
#243678=CARTESIAN_POINT('Ctrl Pts',(-195.083686843779,3.41674982609412,
127.264049621441));
#243679=CARTESIAN_POINT('Ctrl Pts',(-195.091459744045,3.31678976767184,
127.170244786629));
#243680=CARTESIAN_POINT('Ctrl Pts',(-195.09923264431,3.21323606715028,127.080881459673));
#243681=CARTESIAN_POINT('Ctrl Pts',(-195.106722980072,3.11344680447899,
126.994766714744));
#243682=CARTESIAN_POINT('Ctrl Pts',(-195.114213315834,3.01032088056308,
126.912776355728));
#243683=CARTESIAN_POINT('Ctrl Pts',(-195.121703651596,2.90424314852822,
126.835159842003));
#243684=CARTESIAN_POINT('Ctrl Pts',(-195.129477985715,2.79414344704178,
126.75460047457));
#243685=CARTESIAN_POINT('Ctrl Pts',(-195.137252319834,2.68051492048119,
126.678497980498));
#243686=CARTESIAN_POINT('Ctrl Pts',(-195.145026653953,2.56375427239589,
126.60717738434));
#243687=CARTESIAN_POINT('Ctrl Pts',(-195.1527914069,2.44713752137415,126.535944684443));
#243688=CARTESIAN_POINT('Ctrl Pts',(-195.160556159847,2.32739665963895,
126.469482358469));
#243689=CARTESIAN_POINT('Ctrl Pts',(-195.168320912794,2.20496009885318,
126.408074227331));
#243690=CARTESIAN_POINT('Ctrl Pts',(-195.176077953679,2.0826451437853,126.346727087614));
#243691=CARTESIAN_POINT('Ctrl Pts',(-195.183834994564,1.95764016503764,
126.290424327054));
#243692=CARTESIAN_POINT('Ctrl Pts',(-195.191592035449,1.83040078992447,
126.23940541398));
#243693=CARTESIAN_POINT('Ctrl Pts',(-195.19934322669,1.70325736701403,126.188424974666));
#243694=CARTESIAN_POINT('Ctrl Pts',(-195.20709441793,1.57388326299252,126.142720596667));
#243695=CARTESIAN_POINT('Ctrl Pts',(-195.21484560917,1.44275651553619,126.102484747301));
#243696=CARTESIAN_POINT('Ctrl Pts',(-195.222593505947,1.31168550044528,
126.062265999245));
#243697=CARTESIAN_POINT('Ctrl Pts',(-195.230341402724,1.17886369649157,
126.027511271472));
#243698=CARTESIAN_POINT('Ctrl Pts',(-195.238089299501,1.04478662420943,
125.998363949613));
#243699=CARTESIAN_POINT('Ctrl Pts',(-195.245835575585,0.910737597960802,
125.969222724746));
#243700=CARTESIAN_POINT('Ctrl Pts',(-195.253581851669,0.775434207459803,
125.945686655733));
#243701=CARTESIAN_POINT('Ctrl Pts',(-195.261328127753,0.63938416776216,
125.927848447119));
#243702=CARTESIAN_POINT('Ctrl Pts',(-195.269074461019,0.503333123773844,
125.910010106827));
#243703=CARTESIAN_POINT('Ctrl Pts',(-195.276820794284,0.366535807238244,
125.897869761689));
#243704=CARTESIAN_POINT('Ctrl Pts',(-195.284567127549,0.229506696718071,
125.891468420635));
#243705=CARTESIAN_POINT('Ctrl Pts',(-195.292315195552,0.0924468994788774,
125.885065646046));
#243706=CARTESIAN_POINT('Ctrl Pts',(-195.300063263555,-0.0448444045725537,
125.884404451203));
#243707=CARTESIAN_POINT('Ctrl Pts',(-195.307811331558,-0.181851482666569,
125.889473731711));
#243708=CARTESIAN_POINT('Ctrl Pts',(-195.3155676343,-0.319004173513774,
125.89454839991));
#243709=CARTESIAN_POINT('Ctrl Pts',(-195.323323937042,-0.455871643647917,
125.905365695246));
#243710=CARTESIAN_POINT('Ctrl Pts',(-195.331080239784,-0.591941474886092,
125.921862450356));
#243711=CARTESIAN_POINT('Ctrl Pts',(-195.338840682298,-0.728083930690183,
125.938368010281));
#243712=CARTESIAN_POINT('Ctrl Pts',(-195.346601124812,-0.863427513682498,
125.960559006873));
#243713=CARTESIAN_POINT('Ctrl Pts',(-195.354361567326,-0.997469752634241,
125.98832104598));
#243714=CARTESIAN_POINT('Ctrl Pts',(-195.362134467592,-1.13172716808766,
126.016127651178));
#243715=CARTESIAN_POINT('Ctrl Pts',(-195.369907367857,-1.26467868554271,
126.049523074818));
#243716=CARTESIAN_POINT('Ctrl Pts',(-195.377680268122,-1.39583588798348,
126.088342674818));
#243717=CARTESIAN_POINT('Ctrl Pts',(-195.385170603885,-1.52222519575403,
126.12575108458));
#243718=CARTESIAN_POINT('Ctrl Pts',(-195.392660939647,-1.64694808775228,
126.168196053275));
#243719=CARTESIAN_POINT('Ctrl Pts',(-195.400151275409,-1.76958666422382,
126.215488631958));
#243720=CARTESIAN_POINT('Ctrl Pts',(-195.407925865569,-1.89687931172836,
126.264575939728));
#243721=CARTESIAN_POINT('Ctrl Pts',(-195.415700455729,-2.02232956017334,
126.319041551411));
#243722=CARTESIAN_POINT('Ctrl Pts',(-195.423475045889,-2.1454494812566,
126.378727376336));
#243723=CARTESIAN_POINT('Ctrl Pts',(-195.431239995709,-2.26841673604816,
126.438339192008));
#243724=CARTESIAN_POINT('Ctrl Pts',(-195.43900494553,-2.38905906452119,
126.503158172355));
#243725=CARTESIAN_POINT('Ctrl Pts',(-195.44676989535,-2.50690607821073,
126.57297727668));
#243726=CARTESIAN_POINT('Ctrl Pts',(-195.454527074191,-2.62463515337862,
126.642726507686));
#243727=CARTESIAN_POINT('Ctrl Pts',(-195.462284253032,-2.73957414685786,
126.717465706102));
#243728=CARTESIAN_POINT('Ctrl Pts',(-195.470041431874,-2.85127528719056,
126.796940961583));
#243729=CARTESIAN_POINT('Ctrl Pts',(-195.478170592057,-2.96833285167254,
126.880227307771));
#243730=CARTESIAN_POINT('Ctrl Pts',(-195.48629975224,-3.08183394409786,
126.968714999343));
#243731=CARTESIAN_POINT('Ctrl Pts',(-195.494428912423,-3.19129454302132,
127.0620588924));
#243732=CARTESIAN_POINT('Ctrl Pts',(-195.50217647144,-3.29561681384803,
127.151021011987));
#243733=CARTESIAN_POINT('Ctrl Pts',(-195.509924030457,-3.39626895266872,
127.244393515566));
#243734=CARTESIAN_POINT('Ctrl Pts',(-195.517671589474,-3.49286418306127,
127.341835114239));
#243735=CARTESIAN_POINT('Ctrl Pts',(-195.525417525999,-3.58943918449754,
127.43925630671));
#243736=CARTESIAN_POINT('Ctrl Pts',(-195.533163462523,-3.68195869289281,
127.540744621327));
#243737=CARTESIAN_POINT('Ctrl Pts',(-195.540909399048,-3.77007218189079,
127.645921318508));
#243738=CARTESIAN_POINT('Ctrl Pts',(-195.548655390858,-3.85818629978034,
127.751098766365));
#243739=CARTESIAN_POINT('Ctrl Pts',(-195.556401382667,-3.94189408507239,
127.859964349216));
#243740=CARTESIAN_POINT('Ctrl Pts',(-195.564147374477,-4.02088502556128,
127.972105919677));
#243741=CARTESIAN_POINT('Ctrl Pts',(-195.571895099012,-4.09989363577994,
128.084272575435));
#243742=CARTESIAN_POINT('Ctrl Pts',(-195.579642823547,-4.17418307720177,
128.199716357132));
#243743=CARTESIAN_POINT('Ctrl Pts',(-195.587390548081,-4.24348615363837,
128.317996137772));
#243744=CARTESIAN_POINT('Ctrl Pts',(-195.595145422041,-4.31285318138828,
128.436385064323));
#243745=CARTESIAN_POINT('Ctrl Pts',(-195.602900296001,-4.37722445952681,
128.557614877344));
#243746=CARTESIAN_POINT('Ctrl Pts',(-195.610655169961,-4.43637859937377,
128.681219551711));
#243747=CARTESIAN_POINT('Ctrl Pts',(-195.61841422265,-4.49556461454609,
128.804890830702));
#243748=CARTESIAN_POINT('Ctrl Pts',(-195.626173275339,-4.54952773652002,
128.930939161969));
#243749=CARTESIAN_POINT('Ctrl Pts',(-195.633932328028,-4.59809510986851,
129.05887947384));
#243750=CARTESIAN_POINT('Ctrl Pts',(-195.64170116025,-4.64672369767602,
129.186981042053));
#243751=CARTESIAN_POINT('Ctrl Pts',(-195.649469992472,-4.68994283555458,
129.316978981968));
#243752=CARTESIAN_POINT('Ctrl Pts',(-195.657238824693,-4.72762969271982,
129.448373688789));
#243753=CARTESIAN_POINT('Ctrl Pts',(-195.659872975218,-4.74040804237829,
129.492925228326));
#243754=CARTESIAN_POINT('Ctrl Pts',(-195.662507125742,-4.7525508024199,
129.537637266952));
#243755=CARTESIAN_POINT('Ctrl Pts',(-195.665141276266,-4.76405452823396,
129.582490119308));
#243756=CARTESIAN_POINT('',(-193.639859436047,-4.91824923219391,130.807108803159));
#243757=CARTESIAN_POINT('Ctrl Pts',(-193.639859436047,-4.91824923219391,
130.80710880316));
#243758=CARTESIAN_POINT('Ctrl Pts',(-193.648453682647,-4.91816405453979,
130.959545717499));
#243759=CARTESIAN_POINT('Ctrl Pts',(-193.657047929247,-4.91098784782448,
131.11172896582));
#243760=CARTESIAN_POINT('Ctrl Pts',(-193.665642175847,-4.89681553245056,
131.263033380711));
#243761=CARTESIAN_POINT('Ctrl Pts',(-193.674285738832,-4.88256189204551,
131.415206026086));
#243762=CARTESIAN_POINT('Ctrl Pts',(-193.682929301818,-4.86123170846623,
131.566489499949));
#243763=CARTESIAN_POINT('Ctrl Pts',(-193.691572864804,-4.83297164334981,
131.716264207359));
#243764=CARTESIAN_POINT('Ctrl Pts',(-193.700242045639,-4.8046278208643,
131.866482818043));
#243765=CARTESIAN_POINT('Ctrl Pts',(-193.708911226474,-4.76931309557723,
132.015183498403));
#243766=CARTESIAN_POINT('Ctrl Pts',(-193.717580407309,-4.7272241103825,
132.161760806426));
#243767=CARTESIAN_POINT('Ctrl Pts',(-193.726281692355,-4.6849792588291,
132.308880927995));
#243768=CARTESIAN_POINT('Ctrl Pts',(-193.734982977401,-4.63590999828547,
132.453861718932));
#243769=CARTESIAN_POINT('Ctrl Pts',(-193.743684262447,-4.5802623667498,
132.596113869059));
#243770=CARTESIAN_POINT('Ctrl Pts',(-193.745474351195,-4.56881414978355,
132.625378968644));
#243771=CARTESIAN_POINT('Ctrl Pts',(-193.747264439944,-4.55708766805062,
132.654528665305));
#243772=CARTESIAN_POINT('Ctrl Pts',(-193.749054528692,-4.5450853031912,
132.683557959309));
#243773=CARTESIAN_POINT('Ctrl Pts',(-193.756828862811,-4.49295917552469,
132.809631837505));
#243774=CARTESIAN_POINT('Ctrl Pts',(-193.76460319693,-4.4355008567645,132.933734912639));
#243775=CARTESIAN_POINT('Ctrl Pts',(-193.772377531049,-4.37288008339332,
133.055383238235));
#243776=CARTESIAN_POINT('Ctrl Pts',(-193.780142283997,-4.31033648452892,
133.17688164314));
#243777=CARTESIAN_POINT('Ctrl Pts',(-193.787907036944,-4.24264326728463,
133.295930973597));
#243778=CARTESIAN_POINT('Ctrl Pts',(-193.795671789891,-4.17001868196047,
133.412065979489));
#243779=CARTESIAN_POINT('Ctrl Pts',(-193.803428830776,-4.09746622839829,
133.528085638456));
#243780=CARTESIAN_POINT('Ctrl Pts',(-193.811185871661,-4.01999235975909,
133.641196403798));
#243781=CARTESIAN_POINT('Ctrl Pts',(-193.818942912546,-3.93786164135559,
133.750956748026));
#243782=CARTESIAN_POINT('Ctrl Pts',(-193.826694103786,-3.8557928583656,
133.860634321124));
#243783=CARTESIAN_POINT('Ctrl Pts',(-193.834445295026,-3.76907444885508,
133.966966190343));
#243784=CARTESIAN_POINT('Ctrl Pts',(-193.842196486266,-3.67801456681571,
134.069539312338));
#243785=CARTESIAN_POINT('Ctrl Pts',(-193.849944383043,-3.58699338765545,
134.172068838019));
#243786=CARTESIAN_POINT('Ctrl Pts',(-193.85769227982,-3.4916346650259,134.270842502153));
#243787=CARTESIAN_POINT('Ctrl Pts',(-193.865440176597,-3.39228701555218,
134.365480085741));
#243788=CARTESIAN_POINT('Ctrl Pts',(-193.873186452681,-3.29296014746504,
134.460097873187));
#243789=CARTESIAN_POINT('Ctrl Pts',(-193.880932728766,-3.18964629509992,
134.550581031482));
#243790=CARTESIAN_POINT('Ctrl Pts',(-193.88867900485,-3.0827308531471,134.636586282836));
#243791=CARTESIAN_POINT('Ctrl Pts',(-193.896425338115,-2.97581462196864,
134.722592169061));
#243792=CARTESIAN_POINT('Ctrl Pts',(-193.90417167138,-2.86529705278595,
134.804119837331));
#243793=CARTESIAN_POINT('Ctrl Pts',(-193.911918004646,-2.75159620769232,
134.880866642621));
#243794=CARTESIAN_POINT('Ctrl Pts',(-193.919666072649,-2.63786990008324,
134.957630634827));
#243795=CARTESIAN_POINT('Ctrl Pts',(-193.927414140652,-2.52095922202,135.029611414911));
#243796=CARTESIAN_POINT('Ctrl Pts',(-193.935162208655,-2.40131041503007,
135.096550193198));
#243797=CARTESIAN_POINT('Ctrl Pts',(-193.942918511396,-2.28153444386374,
135.163560114816));
#243798=CARTESIAN_POINT('Ctrl Pts',(-193.950674814138,-2.15901487224249,
135.225517138867));
#243799=CARTESIAN_POINT('Ctrl Pts',(-193.95843111688,-2.03422219292027,
135.2822086646));
#243800=CARTESIAN_POINT('Ctrl Pts',(-193.966191559394,-1.90936290798765,
135.338930448309));
#243801=CARTESIAN_POINT('Ctrl Pts',(-193.973952001908,-1.78222846013368,
135.390380987236));
#243802=CARTESIAN_POINT('Ctrl Pts',(-193.981712444423,-1.65330749395548,
135.436396605437));
#243803=CARTESIAN_POINT('Ctrl Pts',(-193.989485344688,-1.52417957239731,
135.482486091993));
#243804=CARTESIAN_POINT('Ctrl Pts',(-193.997258244953,-1.39325977518751,
135.523123107292));
#243805=CARTESIAN_POINT('Ctrl Pts',(-194.005031145219,-1.26105088175151,
135.5581942007));
#243806=CARTESIAN_POINT('Ctrl Pts',(-194.012521480981,-1.133648114606,135.591990371525));
#243807=CARTESIAN_POINT('Ctrl Pts',(-194.020011816743,-1.00504864850035,
135.620618198415));
#243808=CARTESIAN_POINT('Ctrl Pts',(-194.027502152505,-0.875707681015639,
135.644021671804));
#243809=CARTESIAN_POINT('Ctrl Pts',(-194.035276486624,-0.741462711436587,
135.668312495));
#243810=CARTESIAN_POINT('Ctrl Pts',(-194.043050820743,-0.605993654757619,
135.687051927619));
#243811=CARTESIAN_POINT('Ctrl Pts',(-194.050825154862,-0.469799415570403,
135.70012118888));
#243812=CARTESIAN_POINT('Ctrl Pts',(-194.058589907809,-0.333773023610957,
135.713174343443));
#243813=CARTESIAN_POINT('Ctrl Pts',(-194.066354660756,-0.197023612826312,
135.720571193658));
#243814=CARTESIAN_POINT('Ctrl Pts',(-194.074119413703,-0.0600605809332014,
135.722243880629));
#243815=CARTESIAN_POINT('Ctrl Pts',(-194.081876454588,0.0767664173457922,
135.723914906265));
#243816=CARTESIAN_POINT('Ctrl Pts',(-194.089633495473,0.213806226096077,
135.719873077956));
#243817=CARTESIAN_POINT('Ctrl Pts',(-194.097390536358,0.35054437172053,
135.710102325601));
#243818=CARTESIAN_POINT('Ctrl Pts',(-194.105141727599,0.487179402045514,
135.700338941446));
#243819=CARTESIAN_POINT('Ctrl Pts',(-194.112892918839,0.6235128336498,135.684855260145));
#243820=CARTESIAN_POINT('Ctrl Pts',(-194.120644110079,0.759030596709005,
135.663687280362));
#243821=CARTESIAN_POINT('Ctrl Pts',(-194.128392006856,0.894490761104039,
135.642528297535));
#243822=CARTESIAN_POINT('Ctrl Pts',(-194.136139903633,1.02913556100334,
135.615689881632));
#243823=CARTESIAN_POINT('Ctrl Pts',(-194.14388780041,1.16245667159326,135.583259816039));
#243824=CARTESIAN_POINT('Ctrl Pts',(-194.151634076494,1.29574989428092,
135.550836534117));
#243825=CARTESIAN_POINT('Ctrl Pts',(-194.159380352578,1.42771959875601,
135.512824021355));
#243826=CARTESIAN_POINT('Ctrl Pts',(-194.167126628662,1.55786866044568,
135.469360971189));
#243827=CARTESIAN_POINT('Ctrl Pts',(-194.174872961928,1.68801868286598,
135.425897600189));
#243828=CARTESIAN_POINT('Ctrl Pts',(-194.182619295193,1.81634766484947,
135.376983735339));
#243829=CARTESIAN_POINT('Ctrl Pts',(-194.190365628458,1.9423750097934,135.322807517091));
#243830=CARTESIAN_POINT('Ctrl Pts',(-194.198113696461,2.06843057768725,
135.268619166455));
#243831=CARTESIAN_POINT('Ctrl Pts',(-194.205861764464,2.19218312376924,
135.209166271782));
#243832=CARTESIAN_POINT('Ctrl Pts',(-194.213609832467,2.31317371650994,
135.144684386566));
#243833=CARTESIAN_POINT('Ctrl Pts',(-194.221366135209,2.43429289949258,
135.080133969235));
#243834=CARTESIAN_POINT('Ctrl Pts',(-194.229122437951,2.55264391970813,
135.010544068579));
#243835=CARTESIAN_POINT('Ctrl Pts',(-194.236878740693,2.66779359729971,
134.93619560758));
#243836=CARTESIAN_POINT('Ctrl Pts',(-194.244639183207,2.78300473374162,
134.861807464569));
#243837=CARTESIAN_POINT('Ctrl Pts',(-194.252399625721,2.8950108037929,134.782655925994));
#243838=CARTESIAN_POINT('Ctrl Pts',(-194.260160068235,3.00340997790441,
134.699063631548));
#243839=CARTESIAN_POINT('Ctrl Pts',(-194.2679329685,3.11198316399314,134.615337147331));
#243840=CARTESIAN_POINT('Ctrl Pts',(-194.275705868766,3.2169375841494,134.527155913481));
#243841=CARTESIAN_POINT('Ctrl Pts',(-194.283478769031,3.3179060245828,134.434881609729));
#243842=CARTESIAN_POINT('Ctrl Pts',(-194.290969104794,3.41520400788394,
134.345961709343));
#243843=CARTESIAN_POINT('Ctrl Pts',(-194.298459440556,3.50880056207708,
134.253241376088));
#243844=CARTESIAN_POINT('Ctrl Pts',(-194.305949776318,3.59840251931591,
134.157073306044));
#243845=CARTESIAN_POINT('Ctrl Pts',(-194.313724110437,3.69140176199619,
134.057258994396));
#243846=CARTESIAN_POINT('Ctrl Pts',(-194.321498444556,3.78039211153777,
133.953414161395));
#243847=CARTESIAN_POINT('Ctrl Pts',(-194.329272778675,3.8650039641869,133.845894345691));
#243848=CARTESIAN_POINT('Ctrl Pts',(-194.337037531622,3.94951154028939,
133.73850703855));
#243849=CARTESIAN_POINT('Ctrl Pts',(-194.344802284569,4.02965111668345,
133.627454064531));
#243850=CARTESIAN_POINT('Ctrl Pts',(-194.352567037516,4.10509025985185,
133.513127314971));
#243851=CARTESIAN_POINT('Ctrl Pts',(-194.360324078401,4.18045447579975,
133.39891411635));
#243852=CARTESIAN_POINT('Ctrl Pts',(-194.368081119286,4.25112733518645,
133.281433937151));
#243853=CARTESIAN_POINT('Ctrl Pts',(-194.375838160171,4.31681723223276,
133.1611109323));
#243854=CARTESIAN_POINT('Ctrl Pts',(-194.383589351411,4.38245759201679,
133.040878663962));
#243855=CARTESIAN_POINT('Ctrl Pts',(-194.391340542651,4.44312228232928,
132.917808178837));
#243856=CARTESIAN_POINT('Ctrl Pts',(-194.399091733892,4.49856372256806,
132.792351436583));
#243857=CARTESIAN_POINT('Ctrl Pts',(-194.406839630669,4.55398159871571,
132.666948016791));
#243858=CARTESIAN_POINT('Ctrl Pts',(-194.414587527446,4.60418048254142,
132.539160713937));
#243859=CARTESIAN_POINT('Ctrl Pts',(-194.422335424223,4.64895946671369,
132.409464645146));
#243860=CARTESIAN_POINT('Ctrl Pts',(-194.430081700307,4.69372908408779,
132.279795705977));
#243861=CARTESIAN_POINT('Ctrl Pts',(-194.437827976391,4.73308092933866,
132.14821916437));
#243862=CARTESIAN_POINT('Ctrl Pts',(-194.445574252475,4.76686298120744,
132.015228232499));
#243863=CARTESIAN_POINT('Ctrl Pts',(-194.45332058574,4.80064528244769,131.882236318919));
#243864=CARTESIAN_POINT('Ctrl Pts',(-194.461066919006,4.82885761200875,
131.747830373172));
#243865=CARTESIAN_POINT('Ctrl Pts',(-194.468813252271,4.85139848357786,
131.612516429299));
#243866=CARTESIAN_POINT('Ctrl Pts',(-194.476561320274,4.87394440301884,
131.477172182808));
#243867=CARTESIAN_POINT('Ctrl Pts',(-194.484309388277,4.89081627291814,
131.340919919146));
#243868=CARTESIAN_POINT('Ctrl Pts',(-194.49205745628,4.90196420739985,131.204273072824));
#243869=CARTESIAN_POINT('Ctrl Pts',(-194.499813759022,4.913123990039,131.067480996608));
#243870=CARTESIAN_POINT('Ctrl Pts',(-194.507570061764,4.91854765303973,
130.930293890293));
#243871=CARTESIAN_POINT('Ctrl Pts',(-194.515326364506,4.91823740056867,
130.793228046095));
#243872=CARTESIAN_POINT('Ctrl Pts',(-194.52308680702,4.91792698250651,130.656089045728));
#243873=CARTESIAN_POINT('Ctrl Pts',(-194.530847249534,4.91187656817852,
130.519071826834));
#243874=CARTESIAN_POINT('Ctrl Pts',(-194.538607692048,4.90014040480876,
130.382688854626));
#243875=CARTESIAN_POINT('Ctrl Pts',(-194.546380592313,4.88838540150768,
130.246086948365));
#243876=CARTESIAN_POINT('Ctrl Pts',(-194.554153492579,4.8709264597954,130.110121711381));
#243877=CARTESIAN_POINT('Ctrl Pts',(-194.561926392844,4.84786938305054,
129.975297587766));
#243878=CARTESIAN_POINT('Ctrl Pts',(-194.569416728606,4.8256504891227,129.845374660647));
#243879=CARTESIAN_POINT('Ctrl Pts',(-194.576907064368,4.79823347054425,
129.71651162387));
#243880=CARTESIAN_POINT('Ctrl Pts',(-194.58439740013,4.76575659613236,129.589145768693));
#243881=CARTESIAN_POINT('Ctrl Pts',(-194.592171734249,4.73204835115597,
129.456950798405));
#243882=CARTESIAN_POINT('Ctrl Pts',(-194.599946068368,4.69278220975143,
129.325950028211));
#243883=CARTESIAN_POINT('Ctrl Pts',(-194.607720402487,4.64805751679649,
129.196646593539));
#243884=CARTESIAN_POINT('Ctrl Pts',(-194.615485155434,4.60338794302845,
129.067502513795));
#243885=CARTESIAN_POINT('Ctrl Pts',(-194.623249908382,4.55327332936175,
128.940051973427));
#243886=CARTESIAN_POINT('Ctrl Pts',(-194.631014661329,4.49786369664073,
128.814786485009));
#243887=CARTESIAN_POINT('Ctrl Pts',(-194.638771702214,4.44250909754792,
128.689645412039));
#243888=CARTESIAN_POINT('Ctrl Pts',(-194.646528743099,4.38187010235564,
128.566685427407));
#243889=CARTESIAN_POINT('Ctrl Pts',(-194.654285783984,4.31614594456795,
128.446381133412));
#243890=CARTESIAN_POINT('Ctrl Pts',(-194.662036975224,4.250471349879,128.326167561822));
#243891=CARTESIAN_POINT('Ctrl Pts',(-194.669788166464,4.17971941213704,
128.208606036374));
#243892=CARTESIAN_POINT('Ctrl Pts',(-194.677539357704,4.10413655444054,
128.094149148879));
#243893=CARTESIAN_POINT('Ctrl Pts',(-194.685287254481,4.0285858214747,127.979740908613));
#243894=CARTESIAN_POINT('Ctrl Pts',(-194.693035151258,3.94820846734261,
127.868435007373));
#243895=CARTESIAN_POINT('Ctrl Pts',(-194.700783048035,3.86329562621768,
127.760657286598));
#243896=CARTESIAN_POINT('Ctrl Pts',(-194.708529324119,3.77840054702884,
127.652902110599));
#243897=CARTESIAN_POINT('Ctrl Pts',(-194.716275600204,3.68897210971447,
127.548673954013));
#243898=CARTESIAN_POINT('Ctrl Pts',(-194.724021876288,3.59534309643996,
127.448367309858));
#243899=CARTESIAN_POINT('Ctrl Pts',(-194.731768209553,3.50171339201721,
127.348059925262));
#243900=CARTESIAN_POINT('Ctrl Pts',(-194.739514542818,3.40388331653783,
127.251674396663));
#243901=CARTESIAN_POINT('Ctrl Pts',(-194.747260876084,3.3022237549426,127.159569631132));
#243902=CARTESIAN_POINT('Ctrl Pts',(-194.755008944087,3.20054142739355,
127.067444239377));
#243903=CARTESIAN_POINT('Ctrl Pts',(-194.76275701209,3.09502819690908,126.979601780738));
#243904=CARTESIAN_POINT('Ctrl Pts',(-194.770505080093,2.98608906594972,
126.896361749511));
#243905=CARTESIAN_POINT('Ctrl Pts',(-194.778261382835,2.87703415318544,
126.813033249789));
#243906=CARTESIAN_POINT('Ctrl Pts',(-194.786017685576,2.76454637763411,
126.734317186555));
#243907=CARTESIAN_POINT('Ctrl Pts',(-194.793773988318,2.6490613019644,126.660490773937));
#243908=CARTESIAN_POINT('Ctrl Pts',(-194.801534430832,2.53351458843263,
126.58662495794));
#243909=CARTESIAN_POINT('Ctrl Pts',(-194.809294873347,2.41496772491371,
126.517654189227));
#243910=CARTESIAN_POINT('Ctrl Pts',(-194.817055315861,2.29388118485612,
126.453809828038));
#243911=CARTESIAN_POINT('Ctrl Pts',(-194.824828216126,2.17260026593488,
126.389862978213));
#243912=CARTESIAN_POINT('Ctrl Pts',(-194.832601116392,2.04877187687075,
126.331059148613));
#243913=CARTESIAN_POINT('Ctrl Pts',(-194.840374016657,1.92287761007517,
126.277581988213));
#243914=CARTESIAN_POINT('Ctrl Pts',(-194.847864352419,1.80155991698648,
126.226048857294));
#243915=CARTESIAN_POINT('Ctrl Pts',(-194.855354688181,1.67832422631585,
126.179461952482));
#243916=CARTESIAN_POINT('Ctrl Pts',(-194.862845023943,1.55361318125574,
126.13794131091));
#243917=CARTESIAN_POINT('Ctrl Pts',(-194.870619358062,1.42417367901689,
126.094846401594));
#243918=CARTESIAN_POINT('Ctrl Pts',(-194.878393692181,1.29273471235955,
126.05707300227));
#243919=CARTESIAN_POINT('Ctrl Pts',(-194.886168026301,1.15977328170358,
126.024809488271));
#243920=CARTESIAN_POINT('Ctrl Pts',(-194.893932779248,1.02697571412778,
125.992585736169));
#243921=CARTESIAN_POINT('Ctrl Pts',(-194.901697532195,0.892659792124973,
125.965858449745));
#243922=CARTESIAN_POINT('Ctrl Pts',(-194.909462285142,0.757320129074038,
125.944767086765));
#243923=CARTESIAN_POINT('Ctrl Pts',(-194.917219326027,0.6221148872844,125.923696672025));
#243924=CARTESIAN_POINT('Ctrl Pts',(-194.924976366912,0.485888311715355,
125.908251100908));
#243925=CARTESIAN_POINT('Ctrl Pts',(-194.932733407797,0.349147389297095,
125.89851928676));
#243926=CARTESIAN_POINT('Ctrl Pts',(-194.940484599037,0.212509584271935,
125.888794811448));
#243927=CARTESIAN_POINT('Ctrl Pts',(-194.948235790277,0.0753585928360218,
125.884775544365));
#243928=CARTESIAN_POINT('Ctrl Pts',(-194.955986981517,-0.0617916090006001,
125.886498799707));
#243929=CARTESIAN_POINT('Ctrl Pts',(-194.963734878294,-0.198883518342653,
125.888221322619));
#243930=CARTESIAN_POINT('Ctrl Pts',(-194.971482775071,-0.335974248637008,
125.895681508637));
#243931=CARTESIAN_POINT('Ctrl Pts',(-194.979230671849,-0.472548162288011,
125.908864596036));
#243932=CARTESIAN_POINT('Ctrl Pts',(-194.986976947933,-0.60909350762047,
125.922044925817));
#243933=CARTESIAN_POINT('Ctrl Pts',(-194.994723224017,-0.745121862430249,
125.940945738326));
#243934=CARTESIAN_POINT('Ctrl Pts',(-195.002469500101,-0.880121451680396,
125.965500287613));
#243935=CARTESIAN_POINT('Ctrl Pts',(-195.010215833366,-1.01512203746703,
125.990055018157));
#243936=CARTESIAN_POINT('Ctrl Pts',(-195.017962166632,-1.14909345788622,
126.020263498794));
#243937=CARTESIAN_POINT('Ctrl Pts',(-195.025708499897,-1.28153328188549,
126.056007691559));
#243938=CARTESIAN_POINT('Ctrl Pts',(-195.0334565679,-1.41400276486489,126.091759888988));
#243939=CARTESIAN_POINT('Ctrl Pts',(-195.041204635903,-1.54493959152582,
126.133050163519));
#243940=CARTESIAN_POINT('Ctrl Pts',(-195.048952703906,-1.67385604854705,
126.179710469583));
#243941=CARTESIAN_POINT('Ctrl Pts',(-195.056709006648,-1.80290951951275,
126.226420366775));
#243942=CARTESIAN_POINT('Ctrl Pts',(-195.06446530939,-1.92993796321751,
126.278511563241));
#243943=CARTESIAN_POINT('Ctrl Pts',(-195.072221612131,-2.0544727193047,
126.335767448779));
#243944=CARTESIAN_POINT('Ctrl Pts',(-195.079982054646,-2.17907394334121,
126.393053893507));
#243945=CARTESIAN_POINT('Ctrl Pts',(-195.08774249716,-2.30117847981346,
126.455510342012));
#243946=CARTESIAN_POINT('Ctrl Pts',(-195.095502939674,-2.42034278165234,
126.522874440804));
#243947=CARTESIAN_POINT('Ctrl Pts',(-195.10327583994,-2.53969837660744,
126.590346678427));
#243948=CARTESIAN_POINT('Ctrl Pts',(-195.111048740205,-2.65610397282664,
126.662742102887));
#243949=CARTESIAN_POINT('Ctrl Pts',(-195.11882164047,-2.76914474876468,
126.739754803605));
#243950=CARTESIAN_POINT('Ctrl Pts',(-195.126311976232,-2.87807620776515,
126.813967898668));
#243951=CARTESIAN_POINT('Ctrl Pts',(-195.133802311994,-2.98388299120046,
126.892468215446));
#243952=CARTESIAN_POINT('Ctrl Pts',(-195.141292647756,-3.08622484897237,
126.974948228689));
#243953=CARTESIAN_POINT('Ctrl Pts',(-195.148964038384,-3.19104049321887,
127.059421931958));
#243954=CARTESIAN_POINT('Ctrl Pts',(-195.156635429012,-3.29257225117811,
127.148353103153));
#243955=CARTESIAN_POINT('Ctrl Pts',(-195.164306819639,-3.39040972582631,
127.241453805211));
#243956=CARTESIAN_POINT('Ctrl Pts',(-195.171969427545,-3.48813518957756,
127.334447919347));
#243957=CARTESIAN_POINT('Ctrl Pts',(-195.17963203545,-3.58217448966821,
127.431601801204));
#243958=CARTESIAN_POINT('Ctrl Pts',(-195.187294643356,-3.67214823682183,
127.532585810324));
#243959=CARTESIAN_POINT('Ctrl Pts',(-195.194950242633,-3.76203968920446,
127.633477454101));
#243960=CARTESIAN_POINT('Ctrl Pts',(-195.20260584191,-3.84787271682651,
127.738191961579));
#243961=CARTESIAN_POINT('Ctrl Pts',(-195.210261441187,-3.92930333398827,
127.846361568883));
#243962=CARTESIAN_POINT('Ctrl Pts',(-195.217911799506,-4.01067820443681,
127.954457124187));
#243963=CARTESIAN_POINT('Ctrl Pts',(-195.225562157824,-4.0876564179061,
128.066002754977));
#243964=CARTESIAN_POINT('Ctrl Pts',(-195.233212516142,-4.15993336229173,
128.180596625933));
#243965=CARTESIAN_POINT('Ctrl Pts',(-195.24086026656,-4.23218566846759,
128.295151433424));
#243966=CARTESIAN_POINT('Ctrl Pts',(-195.248508016977,-4.29973967457936,
128.412752077692));
#243967=CARTESIAN_POINT('Ctrl Pts',(-195.256155767394,-4.36233354812221,
128.532966975454));
#243968=CARTESIAN_POINT('Ctrl Pts',(-195.263801822143,-4.42491354327928,
128.65315521903));
#243969=CARTESIAN_POINT('Ctrl Pts',(-195.271447876892,-4.48253541118757,
128.775956204889));
#243970=CARTESIAN_POINT('Ctrl Pts',(-195.279093931642,-4.53498317575593,
128.900913571255));
#243971=CARTESIAN_POINT('Ctrl Pts',(-195.286742468474,-4.58744796606283,
129.025911501627));
#243972=CARTESIAN_POINT('Ctrl Pts',(-195.294391005307,-4.63473514030973,
129.153066840563));
#243973=CARTESIAN_POINT('Ctrl Pts',(-195.30203954214,-4.67667684027603,
129.281903132404));
#243974=CARTESIAN_POINT('Ctrl Pts',(-195.307932996256,-4.70899432657831,
129.38117581568));
#243975=CARTESIAN_POINT('Ctrl Pts',(-195.313826450373,-4.73813905169708,
129.481446069613));
#243976=CARTESIAN_POINT('Ctrl Pts',(-195.319719904489,-4.76405452823413,
129.582490119309));
#243977=CARTESIAN_POINT('Ctrl Pts',(-193.570047426085,-4.76405452823409,
129.582490119308));
#243978=CARTESIAN_POINT('Ctrl Pts',(-193.577886143416,-4.79853512568151,
129.71692944544));
#243979=CARTESIAN_POINT('Ctrl Pts',(-193.585724860747,-4.82734183515294,
129.852911410386));
#243980=CARTESIAN_POINT('Ctrl Pts',(-193.593563578078,-4.85034802871446,
129.989923963893));
#243981=CARTESIAN_POINT('Ctrl Pts',(-193.601399678027,-4.87334654040656,
130.126890768305));
#243982=CARTESIAN_POINT('Ctrl Pts',(-193.609235777976,-4.8905483261116,
130.264887104432));
#243983=CARTESIAN_POINT('Ctrl Pts',(-193.617071877925,-4.90187780366035,
130.40339046845));
#243984=CARTESIAN_POINT('Ctrl Pts',(-193.624667730615,-4.91285993036604,
130.537647453052));
#243985=CARTESIAN_POINT('Ctrl Pts',(-193.632263583305,-4.91832451473222,
130.672380489236));
#243986=CARTESIAN_POINT('Ctrl Pts',(-193.639859435995,-4.91824923219442,
130.807108802231));
#243987=CARTESIAN_POINT('Origin',(213.235140564004,0.,130.804360617566));
#243988=CARTESIAN_POINT('',(-191.820046567589,-4.76405452823394,129.582490119308));
#243989=CARTESIAN_POINT('',(-192.165295998532,-4.76405452823416,129.582490119309));
#243990=CARTESIAN_POINT('',(213.235140564004,-4.76405452823405,129.582490119308));
#243991=CARTESIAN_POINT('',(-192.235140564068,-4.9182489107902,130.807633843951));
#243992=CARTESIAN_POINT('Ctrl Pts',(-192.165295998532,-4.76405452823416,
129.582490119309));
#243993=CARTESIAN_POINT('Ctrl Pts',(-192.173087299489,-4.79834001608084,
129.716168716068));
#243994=CARTESIAN_POINT('Ctrl Pts',(-192.180878600447,-4.82701148740486,
129.851356535398));
#243995=CARTESIAN_POINT('Ctrl Pts',(-192.188669901404,-4.84994811259561,
129.987545848092));
#243996=CARTESIAN_POINT('Ctrl Pts',(-192.196460544,-4.87288279965338,130.12372365286));
#243997=CARTESIAN_POINT('Ctrl Pts',(-192.204251186596,-4.89008353206788,
130.260902405253));
#243998=CARTESIAN_POINT('Ctrl Pts',(-192.212041829192,-4.90148064217082,
130.398564391703));
#243999=CARTESIAN_POINT('Ctrl Pts',(-192.219741407466,-4.9127445321833,
130.534617256005));
#244000=CARTESIAN_POINT('Ctrl Pts',(-192.227440985739,-4.91833974990952,
130.671141747254));
#244001=CARTESIAN_POINT('Ctrl Pts',(-192.235140564013,-4.91824891079085,
130.807633842979));
#244002=CARTESIAN_POINT('Ctrl Pts',(-192.235140564068,-4.9182489107902,
130.80763384395));
#244003=CARTESIAN_POINT('Ctrl Pts',(-192.243918515748,-4.9181453490622,
130.963242499187));
#244004=CARTESIAN_POINT('Ctrl Pts',(-192.252696467428,-4.91065281771742,
131.118565439462));
#244005=CARTESIAN_POINT('Ctrl Pts',(-192.261474419109,-4.89587660554873,
131.272949270588));
#244006=CARTESIAN_POINT('Ctrl Pts',(-192.270289110367,-4.88103854845119,
131.42797926576));
#244007=CARTESIAN_POINT('Ctrl Pts',(-192.279103801625,-4.85885582307568,
131.582062100835));
#244008=CARTESIAN_POINT('Ctrl Pts',(-192.287918492883,-4.8294847853578,
131.734554022454));
#244009=CARTESIAN_POINT('Ctrl Pts',(-192.296783739358,-4.79994529486645,
131.887920536499));
#244010=CARTESIAN_POINT('Ctrl Pts',(-192.305648985834,-4.76313489578936,
132.039677664175));
#244011=CARTESIAN_POINT('Ctrl Pts',(-192.314514232309,-4.71926132012198,
132.189191168536));
#244012=CARTESIAN_POINT('Ctrl Pts',(-192.322085292695,-4.68179259416399,
132.316878060629));
#244013=CARTESIAN_POINT('Ctrl Pts',(-192.329656353081,-4.63917323850466,
132.442928873986));
#244014=CARTESIAN_POINT('Ctrl Pts',(-192.337227413468,-4.59155968143751,
132.566961750635));
#244015=CARTESIAN_POINT('Ctrl Pts',(-192.345001747587,-4.54266775846242,
132.694324758674));
#244016=CARTESIAN_POINT('Ctrl Pts',(-192.352776081706,-4.48839508868817,
132.819853675534));
#244017=CARTESIAN_POINT('Ctrl Pts',(-192.360550415825,-4.42889900368266,
132.943060380899));
#244018=CARTESIAN_POINT('Ctrl Pts',(-192.368315168772,-4.3694762422846,
133.06611524501));
#244019=CARTESIAN_POINT('Ctrl Pts',(-192.376079921719,-4.30484304252658,
133.186853243304));
#244020=CARTESIAN_POINT('Ctrl Pts',(-192.383844674666,-4.23520571110023,
133.304803707733));
#244021=CARTESIAN_POINT('Ctrl Pts',(-192.391601715551,-4.16563754445317,
133.422637022098));
#244022=CARTESIAN_POINT('Ctrl Pts',(-192.399358756436,-4.09107533448945,
133.537687977781));
#244023=CARTESIAN_POINT('Ctrl Pts',(-192.407115797321,-4.01177229319911,
133.64950843974));
#244024=CARTESIAN_POINT('Ctrl Pts',(-192.414866988561,-3.9325290549492,
133.761244577018));
#244025=CARTESIAN_POINT('Ctrl Pts',(-192.422618179801,-3.84855232664149,
133.869754751943));
#244026=CARTESIAN_POINT('Ctrl Pts',(-192.430369371041,-3.76013962162594,
133.974618192019));
#244027=CARTESIAN_POINT('Ctrl Pts',(-192.438117267819,-3.67176449436839,
134.079437062336));
#244028=CARTESIAN_POINT('Ctrl Pts',(-192.445865164596,-3.57895739182149,
134.180611982277));
#244029=CARTESIAN_POINT('Ctrl Pts',(-192.453613061373,-3.4820571144234,
134.27775396045));
#244030=CARTESIAN_POINT('Ctrl Pts',(-192.461359337457,-3.38517710647442,
134.374875618616));
#244031=CARTESIAN_POINT('Ctrl Pts',(-192.469105613541,-3.28420590264548,
134.467965736369));
#244032=CARTESIAN_POINT('Ctrl Pts',(-192.476851889625,-3.17952001215119,
134.556671312968));
#244033=CARTESIAN_POINT('Ctrl Pts',(-192.48459822289,-3.07483334888957,
134.645377544372));
#244034=CARTESIAN_POINT('Ctrl Pts',(-192.492344556156,-2.96643224252753,
134.729698917291));
#244035=CARTESIAN_POINT('Ctrl Pts',(-192.500090889421,-2.85472689593607,
134.809322216897));
#244036=CARTESIAN_POINT('Ctrl Pts',(-192.507838957424,-2.7429965337069,
134.888963347589));
#244037=CARTESIAN_POINT('Ctrl Pts',(-192.515587025427,-2.62796077711468,
134.963904084522));
#244038=CARTESIAN_POINT('Ctrl Pts',(-192.52333509343,-2.51005911841526,
135.033874334834));
#244039=CARTESIAN_POINT('Ctrl Pts',(-192.531091396171,-2.39203215242945,
135.103918950361));
#244040=CARTESIAN_POINT('Ctrl Pts',(-192.538847698913,-2.27113353654513,
135.16898232667));
#244041=CARTESIAN_POINT('Ctrl Pts',(-192.546604001655,-2.14782818502421,
135.228839925927));
#244042=CARTESIAN_POINT('Ctrl Pts',(-192.554364444169,-2.02445702172452,
135.288729472987));
#244043=CARTESIAN_POINT('Ctrl Pts',(-192.562124886684,-1.89867692159537,
135.343407550848));
#244044=CARTESIAN_POINT('Ctrl Pts',(-192.569885329198,-1.77097219332344,
135.392698067337));
#244045=CARTESIAN_POINT('Ctrl Pts',(-192.577658229463,-1.64306246208459,
135.442067709339));
#244046=CARTESIAN_POINT('Ctrl Pts',(-192.585431129729,-1.51322229925508,
135.486032381865));
#244047=CARTESIAN_POINT('Ctrl Pts',(-192.593204029994,-1.38195142542684,
135.524465840997));
#244048=CARTESIAN_POINT('Ctrl Pts',(-192.600694365756,-1.25545257851221,
135.561502147082));
#244049=CARTESIAN_POINT('Ctrl Pts',(-192.608184701518,-1.12762553341084,
135.593402330408));
#244050=CARTESIAN_POINT('Ctrl Pts',(-192.61567503728,-0.998923910181445,
135.620098783639));
#244051=CARTESIAN_POINT('Ctrl Pts',(-192.623449371399,-0.865342525790616,
135.647807441008));
#244052=CARTESIAN_POINT('Ctrl Pts',(-192.631223705518,-0.730395789175812,
135.669997752622));
#244053=CARTESIAN_POINT('Ctrl Pts',(-192.638998039637,-0.594579411339083,
135.68653824503));
#244054=CARTESIAN_POINT('Ctrl Pts',(-192.646762792585,-0.45893041504978,
135.70305835276));
#244055=CARTESIAN_POINT('Ctrl Pts',(-192.654527545532,-0.32241429438374,
135.713942448564));
#244056=CARTESIAN_POINT('Ctrl Pts',(-192.662292298479,-0.185538549506594,
135.719109696527));
#244057=CARTESIAN_POINT('Ctrl Pts',(-192.670049339364,-0.0487987515492415,
135.724271812306));
#244058=CARTESIAN_POINT('Ctrl Pts',(-192.677806380249,0.0882995716484737,
135.723728365175));
#244059=CARTESIAN_POINT('Ctrl Pts',(-192.685563421134,0.225242524115774,
135.717450161614));
#244060=CARTESIAN_POINT('Ctrl Pts',(-192.693314612374,0.362082206837544,
135.711176692494));
#244061=CARTESIAN_POINT('Ctrl Pts',(-192.701065803614,0.498766363066561,
135.69917709268));
#244062=CARTESIAN_POINT('Ctrl Pts',(-192.708816994854,0.63478017175093,
135.681474230765));
#244063=CARTESIAN_POINT('Ctrl Pts',(-192.716564891631,0.770736170938507,
135.663778893039));
#244064=CARTESIAN_POINT('Ctrl Pts',(-192.724312788408,0.906022002373333,
135.640385164795));
#244065=CARTESIAN_POINT('Ctrl Pts',(-192.732060685185,1.04012726666948,
135.611367829089));
#244066=CARTESIAN_POINT('Ctrl Pts',(-192.73980696127,1.17420447903531,135.582356563184));
#244067=CARTESIAN_POINT('Ctrl Pts',(-192.747553237354,1.30710123357782,
135.547724112247));
#244068=CARTESIAN_POINT('Ctrl Pts',(-192.755299513438,1.4383170283509,135.507596438621));
#244069=CARTESIAN_POINT('Ctrl Pts',(-192.763045846703,1.56953379172899,
135.467468468782));
#244070=CARTESIAN_POINT('Ctrl Pts',(-192.770792179969,1.69906919670432,
135.421845309648));
#244071=CARTESIAN_POINT('Ctrl Pts',(-192.778538513234,1.82643800209956,
135.370902776244));
#244072=CARTESIAN_POINT('Ctrl Pts',(-192.786286581237,1.95383533085548,
135.319948834614));
#244073=CARTESIAN_POINT('Ctrl Pts',(-192.79403464924,2.07906473161203,135.263673293452));
#244074=CARTESIAN_POINT('Ctrl Pts',(-192.801782717243,2.20166141129512,
135.202299918251));
#244075=CARTESIAN_POINT('Ctrl Pts',(-192.809539019985,2.32438838818846,
135.140861314697));
#244076=CARTESIAN_POINT('Ctrl Pts',(-192.817295322727,2.44447670436585,
135.074314229283));
#244077=CARTESIAN_POINT('Ctrl Pts',(-192.825051625468,2.56148615227356,
135.002928439361));
#244078=CARTESIAN_POINT('Ctrl Pts',(-192.832812067983,2.67855805164703,
134.931504548693));
#244079=CARTESIAN_POINT('Ctrl Pts',(-192.840572510497,2.79254748358488,
134.855237024847));
#244080=CARTESIAN_POINT('Ctrl Pts',(-192.848332953011,2.90304451607954,
134.774438148315));
#244081=CARTESIAN_POINT('Ctrl Pts',(-192.856105853276,3.01371892821992,
134.693509566255));
#244082=CARTESIAN_POINT('Ctrl Pts',(-192.863878753542,3.12088943189119,
134.608035339398));
#244083=CARTESIAN_POINT('Ctrl Pts',(-192.871651653807,3.22417970332439,
134.518367658912));
#244084=CARTESIAN_POINT('Ctrl Pts',(-192.879141989569,3.32371511321709,
134.431959624473));
#244085=CARTESIAN_POINT('Ctrl Pts',(-192.886632325331,3.41964728113286,
134.341657939474));
#244086=CARTESIAN_POINT('Ctrl Pts',(-192.894122661093,3.51167413438388,
134.247807703902));
#244087=CARTESIAN_POINT('Ctrl Pts',(-192.901896995212,3.60719021374836,
134.150399108123));
#244088=CARTESIAN_POINT('Ctrl Pts',(-192.909671329331,3.69880155876895,
134.048859002174));
#244089=CARTESIAN_POINT('Ctrl Pts',(-192.91744566345,3.78612961320351,133.943533377151));
#244090=CARTESIAN_POINT('Ctrl Pts',(-192.925210416397,3.87335004361548,
133.838337556548));
#244091=CARTESIAN_POINT('Ctrl Pts',(-192.932975169344,3.95629743948013,
133.729365797536));
#244092=CARTESIAN_POINT('Ctrl Pts',(-192.940739922292,4.0346294750173,133.61700138059));
#244093=CARTESIAN_POINT('Ctrl Pts',(-192.948496963177,4.11288371007249,
133.504748565566));
#244094=CARTESIAN_POINT('Ctrl Pts',(-192.956254004062,4.18653148511081,
133.389110116985));
#244095=CARTESIAN_POINT('Ctrl Pts',(-192.964011044947,4.25527046547266,
133.27050261027));
#244096=CARTESIAN_POINT('Ctrl Pts',(-192.971762236187,4.32395760923461,
133.151984546398));
#244097=CARTESIAN_POINT('Ctrl Pts',(-192.979513427427,4.38774313120223,
133.03050221786));
#244098=CARTESIAN_POINT('Ctrl Pts',(-192.987264618667,4.44636799801797,
132.906501119222));
#244099=CARTESIAN_POINT('Ctrl Pts',(-192.995012515444,4.50496794770152,
132.782552724358));
#244100=CARTESIAN_POINT('Ctrl Pts',(-193.002760412221,4.55841143801551,
132.656088041339));
#244101=CARTESIAN_POINT('Ctrl Pts',(-193.010508308998,4.60648550272751,
132.527576905692));
#244102=CARTESIAN_POINT('Ctrl Pts',(-193.018254585082,4.65454951138154,
132.399092651803));
#244103=CARTESIAN_POINT('Ctrl Pts',(-193.026000861166,4.69724619158006,
132.268563162699));
#244104=CARTESIAN_POINT('Ctrl Pts',(-193.03374713725,4.73441098548304,132.136477610565));
#244105=CARTESIAN_POINT('Ctrl Pts',(-193.041493470516,4.77157605372813,
132.004391083406));
#244106=CARTESIAN_POINT('Ctrl Pts',(-193.049239803781,4.80320904830049,
131.870748846647));
#244107=CARTESIAN_POINT('Ctrl Pts',(-193.056986137046,4.82919560265308,
131.736054179751));
#244108=CARTESIAN_POINT('Ctrl Pts',(-193.064734205049,4.8551879765143,131.601329348918));
#244109=CARTESIAN_POINT('Ctrl Pts',(-193.072482273053,4.87553131993598,
131.465552002776));
#244110=CARTESIAN_POINT('Ctrl Pts',(-193.080230341056,4.89016266115448,
131.329234135616));
#244111=CARTESIAN_POINT('Ctrl Pts',(-193.087986643797,4.90480955273655,
131.192771388205));
#244112=CARTESIAN_POINT('Ctrl Pts',(-193.095742946539,4.91373227328045,
131.055767361558));
#244113=CARTESIAN_POINT('Ctrl Pts',(-193.103499249281,4.91691985117717,
130.918738236006));
#244114=CARTESIAN_POINT('Ctrl Pts',(-193.111259691795,4.92010913038018,
130.781635973883));
#244115=CARTESIAN_POINT('Ctrl Pts',(-193.119020134309,4.91755717486896,
130.644508976869));
#244116=CARTESIAN_POINT('Ctrl Pts',(-193.126780576824,4.90930513680369,
130.507870927605));
#244117=CARTESIAN_POINT('Ctrl Pts',(-193.134553477089,4.90103985183434,
130.371013534815));
#244118=CARTESIAN_POINT('Ctrl Pts',(-193.142326377354,4.88705623904379,
130.23464704741));
#244119=CARTESIAN_POINT('Ctrl Pts',(-193.15009927762,4.86744719464528,130.099278445164));
#244120=CARTESIAN_POINT('Ctrl Pts',(-193.157589613382,4.84855098840286,
129.968830832581));
#244121=CARTESIAN_POINT('Ctrl Pts',(-193.165079949144,4.82443130336841,
129.839310116289));
#244122=CARTESIAN_POINT('Ctrl Pts',(-193.172570284906,4.79521520426802,
129.711156973565));
#244123=CARTESIAN_POINT('Ctrl Pts',(-193.180344619025,4.76489136789024,
129.578144865484));
#244124=CARTESIAN_POINT('Ctrl Pts',(-193.188118953144,4.7289809707059,129.44618473883));
#244125=CARTESIAN_POINT('Ctrl Pts',(-193.195893287263,4.68757048592578,
129.31578210033));
#244126=CARTESIAN_POINT('Ctrl Pts',(-193.20365804021,4.64621103586719,129.185540171426));
#244127=CARTESIAN_POINT('Ctrl Pts',(-193.211422793157,4.59936510233688,
129.056852280564));
#244128=CARTESIAN_POINT('Ctrl Pts',(-193.219187546105,4.54717011460856,
128.930213608575));
#244129=CARTESIAN_POINT('Ctrl Pts',(-193.22694458699,4.49502696767788,128.8037007159));
#244130=CARTESIAN_POINT('Ctrl Pts',(-193.234701627874,4.43754548719051,
128.679233350863));
#244131=CARTESIAN_POINT('Ctrl Pts',(-193.242458668759,4.37491273058033,
128.557291045366));
#244132=CARTESIAN_POINT('Ctrl Pts',(-193.25020986,4.31232720581922,128.435440697511));
#244133=CARTESIAN_POINT('Ctrl Pts',(-193.25796105124,4.24459831493363,128.316111965434));
#244134=CARTESIAN_POINT('Ctrl Pts',(-193.26571224248,4.17196085126148,128.19976358193));
#244135=CARTESIAN_POINT('Ctrl Pts',(-193.273460139257,4.09935426044897,
128.083464649593));
#244136=CARTESIAN_POINT('Ctrl Pts',(-193.281208036034,4.02184345290365,
127.97014387735));
#244137=CARTESIAN_POINT('Ctrl Pts',(-193.288955932811,3.93970860111024,
127.860234397303));
#244138=CARTESIAN_POINT('Ctrl Pts',(-193.296702208895,3.8575909301572,127.75034790795));
#244139=CARTESIAN_POINT('Ctrl Pts',(-193.304448484979,3.77085137275848,
127.643871604446));
#244140=CARTESIAN_POINT('Ctrl Pts',(-193.312194761063,3.67981253579604,
127.541208343476));
#244141=CARTESIAN_POINT('Ctrl Pts',(-193.319941094329,3.58877302680572,
127.43854432467));
#244142=CARTESIAN_POINT('Ctrl Pts',(-193.327687427594,3.49343443432112,
127.339693697082));
#244143=CARTESIAN_POINT('Ctrl Pts',(-193.335433760859,3.39415836369511,
127.24502471537));
#244144=CARTESIAN_POINT('Ctrl Pts',(-193.343181828862,3.29486006088155,
127.150334533197));
#244145=CARTESIAN_POINT('Ctrl Pts',(-193.350929896865,3.19162280819176,
127.059828130087));
#244146=CARTESIAN_POINT('Ctrl Pts',(-193.358677964868,3.08484332314698,
126.97383523139));
#244147=CARTESIAN_POINT('Ctrl Pts',(-193.36643426761,2.97795035159466,126.887750938417));
#244148=CARTESIAN_POINT('Ctrl Pts',(-193.374190570352,2.86750793222474,
126.806189978007));
#244149=CARTESIAN_POINT('Ctrl Pts',(-193.381946873094,2.7539444117456,126.729440588962));
#244150=CARTESIAN_POINT('Ctrl Pts',(-193.389707315608,2.64032027899594,
126.652650236458));
#244151=CARTESIAN_POINT('Ctrl Pts',(-193.397467758122,2.52357205848088,
126.580676777505));
#244152=CARTESIAN_POINT('Ctrl Pts',(-193.405228200636,2.40415416970356,
126.513763247642));
#244153=CARTESIAN_POINT('Ctrl Pts',(-193.413001100902,2.28454458072975,
126.446742302241));
#244154=CARTESIAN_POINT('Ctrl Pts',(-193.420774001167,2.16225710849449,
126.384797694339));
#244155=CARTESIAN_POINT('Ctrl Pts',(-193.428546901433,2.03776850211148,
126.328125302672));
#244156=CARTESIAN_POINT('Ctrl Pts',(-193.436037237195,1.91780537013702,
126.273513095191));
#244157=CARTESIAN_POINT('Ctrl Pts',(-193.443527572957,1.79579864438425,
126.223796558439));
#244158=CARTESIAN_POINT('Ctrl Pts',(-193.451017908719,1.67218776071735,
126.179106986098));
#244159=CARTESIAN_POINT('Ctrl Pts',(-193.458792242838,1.54389013282677,
126.132722995039));
#244160=CARTESIAN_POINT('Ctrl Pts',(-193.466566576957,1.41345789412949,
126.091607757464));
#244161=CARTESIAN_POINT('Ctrl Pts',(-193.474340911076,1.28136308263296,
126.055961759744));
#244162=CARTESIAN_POINT('Ctrl Pts',(-193.482105664023,1.1494310661863,126.020359692531));
#244163=CARTESIAN_POINT('Ctrl Pts',(-193.48987041697,1.01584092762441,125.990213554768));
#244164=CARTESIAN_POINT('Ctrl Pts',(-193.497635169917,0.88108356048614,
125.965675380651));
#244165=CARTESIAN_POINT('Ctrl Pts',(-193.505392210802,0.746460036264656,
125.941161578194));
#244166=CARTESIAN_POINT('Ctrl Pts',(-193.513149251688,0.610671972693172,
125.922244724601));
#244167=CARTESIAN_POINT('Ctrl Pts',(-193.520906292573,0.47422392265558,
125.909026641862));
#244168=CARTESIAN_POINT('Ctrl Pts',(-193.528657483813,0.337878769153747,
125.895818526982));
#244169=CARTESIAN_POINT('Ctrl Pts',(-193.536408675053,0.200875007398296,
125.888300666612));
#244170=CARTESIAN_POINT('Ctrl Pts',(-193.544159866293,0.0637254938153366,
125.886523478748));
#244171=CARTESIAN_POINT('Ctrl Pts',(-193.55190776307,-0.0733657275659535,
125.884747046236));
#244172=CARTESIAN_POINT('Ctrl Pts',(-193.559655659847,-0.210602187450144,
125.888706438433));
#244173=CARTESIAN_POINT('Ctrl Pts',(-193.567403556624,-0.347468039461664,
125.898400056773));
#244174=CARTESIAN_POINT('Ctrl Pts',(-193.575149832708,-0.48430526208743,
125.908091647417));
#244175=CARTESIAN_POINT('Ctrl Pts',(-193.582896108792,-0.620771641297166,
125.923515050776));
#244176=CARTESIAN_POINT('Ctrl Pts',(-193.590642384876,-0.756353865451232,
125.944616602423));
#244177=CARTESIAN_POINT('Ctrl Pts',(-193.598388718142,-0.891937090442292,
125.965718309837));
#244178=CARTESIAN_POINT('Ctrl Pts',(-193.606135051407,-1.02663576103986,
125.992498189051));
#244179=CARTESIAN_POINT('Ctrl Pts',(-193.613881384672,-1.15994459764504,
126.02485106188));
#244180=CARTESIAN_POINT('Ctrl Pts',(-193.621629452675,-1.29328328784007,
126.05721117991));
#244181=CARTESIAN_POINT('Ctrl Pts',(-193.629377520678,-1.42523114484017,
126.095146682807));
#244182=CARTESIAN_POINT('Ctrl Pts',(-193.637125588681,-1.55529632586053,
126.138502025488));
#244183=CARTESIAN_POINT('Ctrl Pts',(-193.644881891423,-1.68549974170325,
126.181903446744));
#244184=CARTESIAN_POINT('Ctrl Pts',(-193.652638194165,-1.81381611299879,
126.230736090713));
#244185=CARTESIAN_POINT('Ctrl Pts',(-193.660394496907,-1.93977140442049,
126.284795377292));
#244186=CARTESIAN_POINT('Ctrl Pts',(-193.668154939421,-2.06579392197332,
126.33888351694));
#244187=CARTESIAN_POINT('Ctrl Pts',(-193.675915381935,-2.1894524963065,
126.398203688727));
#244188=CARTESIAN_POINT('Ctrl Pts',(-193.683675824449,-2.31029702989768,
126.462504943301));
#244189=CARTESIAN_POINT('Ctrl Pts',(-193.691448724715,-2.43133555386226,
126.526909419958));
#244190=CARTESIAN_POINT('Ctrl Pts',(-193.69922162498,-2.54955067263316,
126.596310760058));
#244191=CARTESIAN_POINT('Ctrl Pts',(-193.706994525246,-2.6645198933412,
126.670413738313));
#244192=CARTESIAN_POINT('Ctrl Pts',(-193.714484861008,-2.77530969328494,
126.741822886652));
#244193=CARTESIAN_POINT('Ctrl Pts',(-193.72197519677,-2.88308523914618,
126.817597597928));
#244194=CARTESIAN_POINT('Ctrl Pts',(-193.729465532532,-2.98749854401419,
126.897439129743));
#244195=CARTESIAN_POINT('Ctrl Pts',(-193.737196078694,-3.0952603185036,
126.97984112973));
#244196=CARTESIAN_POINT('Ctrl Pts',(-193.744926624856,-3.19980039402153,
127.066850545295));
#244197=CARTESIAN_POINT('Ctrl Pts',(-193.752657171018,-3.30069311752396,
127.158183440517));
#244198=CARTESIAN_POINT('Ctrl Pts',(-193.760334883215,-3.40089629561768,
127.248892126417));
#244199=CARTESIAN_POINT('Ctrl Pts',(-193.768012595413,-3.49750149279864,
127.343865140785));
#244200=CARTESIAN_POINT('Ctrl Pts',(-193.77569030761,-3.5901203904032,127.44278083346));
#244201=CARTESIAN_POINT('Ctrl Pts',(-193.783361016429,-3.68265480383977,
127.54160629822));
#244202=CARTESIAN_POINT('Ctrl Pts',(-193.791031725249,-3.77120987628044,
127.644366999939));
#244203=CARTESIAN_POINT('Ctrl Pts',(-193.798702434068,-3.855431774176,127.750702336557));
#244204=CARTESIAN_POINT('Ctrl Pts',(-193.80636789687,-3.93959607249805,
127.856964950164));
#244205=CARTESIAN_POINT('Ctrl Pts',(-193.814033359672,-4.01943284300044,
127.966797023577));
#244206=CARTESIAN_POINT('Ctrl Pts',(-193.821698822474,-4.09462678788818,
128.079802941464));
#244207=CARTESIAN_POINT('Ctrl Pts',(-193.829473807303,-4.17089508320833,
128.194423456868));
#244208=CARTESIAN_POINT('Ctrl Pts',(-193.837248792132,-4.24238657353508,
128.312308902551));
#244209=CARTESIAN_POINT('Ctrl Pts',(-193.845023776961,-4.30881615492087,
128.433013657378));
#244210=CARTESIAN_POINT('Ctrl Pts',(-193.852685093457,-4.37427455244702,
128.551953738889));
#244211=CARTESIAN_POINT('Ctrl Pts',(-193.860346409954,-4.43481787122632,
128.673630879259));
#244212=CARTESIAN_POINT('Ctrl Pts',(-193.86800772645,-4.49021873156322,
128.79759236856));
#244213=CARTESIAN_POINT('Ctrl Pts',(-193.875839545445,-4.54685253732966,
128.924312619201));
#244214=CARTESIAN_POINT('Ctrl Pts',(-193.883671364441,-4.5981120887347,
129.053419710477));
#244215=CARTESIAN_POINT('Ctrl Pts',(-193.891503183436,-4.64380612801652,
129.184407621984));
#244216=CARTESIAN_POINT('Ctrl Pts',(-193.899335002432,-4.68950016729845,
129.315395533491));
#244217=CARTESIAN_POINT('Ctrl Pts',(-193.907166821427,-4.72962857139135,
129.448263836065));
#244218=CARTESIAN_POINT('Ctrl Pts',(-193.914998640423,-4.76405452823412,
129.582490119309));
#244219=CARTESIAN_POINT('',(-191.889859435946,-4.91824838362704,130.800373206121));
#244220=CARTESIAN_POINT('Ctrl Pts',(-191.889859435995,-4.91824838362774,
130.800373206994));
#244221=CARTESIAN_POINT('Ctrl Pts',(-191.897713992238,-4.91836113829842,
130.939449799867));
#244222=CARTESIAN_POINT('Ctrl Pts',(-191.90556854848,-4.91257017733928,
131.078607516704));
#244223=CARTESIAN_POINT('Ctrl Pts',(-191.913423104722,-4.90088344947465,
131.217306712311));
#244224=CARTESIAN_POINT('Ctrl Pts',(-191.921150059273,-4.88938657908931,
131.353752661333));
#244225=CARTESIAN_POINT('Ctrl Pts',(-191.928877013823,-4.87218410818176,
131.489754471933));
#244226=CARTESIAN_POINT('Ctrl Pts',(-191.936603968374,-4.84933606598093,
131.624801219728));
#244227=CARTESIAN_POINT('Ctrl Pts',(-191.944330975815,-4.82648786738739,
131.759848891906));
#244228=CARTESIAN_POINT('Ctrl Pts',(-191.952057983256,-4.7979940857108,
131.893941100987));
#244229=CARTESIAN_POINT('Ctrl Pts',(-191.959784990697,-4.76396615906066,
132.02657561413));
#244230=CARTESIAN_POINT('Ctrl Pts',(-191.967513741978,-4.72993055294498,
132.159240060396));
#244231=CARTESIAN_POINT('Ctrl Pts',(-191.97524249326,-4.69035841421798,
132.290445775788));
#244232=CARTESIAN_POINT('Ctrl Pts',(-191.982971244541,-4.64541136803275,
132.419704631778));
#244233=CARTESIAN_POINT('Ctrl Pts',(-191.990921039647,-4.59917882738299,
132.552660316771));
#244234=CARTESIAN_POINT('Ctrl Pts',(-191.998870834754,-4.54725946423311,
132.6835556899));
#244235=CARTESIAN_POINT('Ctrl Pts',(-192.00682062986,-4.48988223286208,
132.811881625558));
#244236=CARTESIAN_POINT('Ctrl Pts',(-192.01456223062,-4.43400763331795,
132.936846879103));
#244237=CARTESIAN_POINT('Ctrl Pts',(-192.022303831381,-4.37295770825076,
133.059375276236));
#244238=CARTESIAN_POINT('Ctrl Pts',(-192.030045432141,-4.30699015546567,
133.179022459434));
#244239=CARTESIAN_POINT('Ctrl Pts',(-192.03809932442,-4.23836151127706,
133.30349613804));
#244240=CARTESIAN_POINT('Ctrl Pts',(-192.046153216699,-4.16441045295695,
133.424850879837));
#244241=CARTESIAN_POINT('Ctrl Pts',(-192.054207108978,-4.08547567197879,
133.542621305698));
#244242=CARTESIAN_POINT('Ctrl Pts',(-192.062261001257,-4.00654089100041,
133.660391731559));
#244243=CARTESIAN_POINT('Ctrl Pts',(-192.070314893536,-3.9226227251379,
133.77457750615));
#244244=CARTESIAN_POINT('Ctrl Pts',(-192.078368785815,-3.83410466332919,
133.88475417897));
#244245=CARTESIAN_POINT('Ctrl Pts',(-192.086143119934,-3.74865914652369,
133.99110651607));
#244246=CARTESIAN_POINT('Ctrl Pts',(-192.093917454053,-3.65864985410877,
134.094069416823));
#244247=CARTESIAN_POINT('Ctrl Pts',(-192.101691788172,-3.56437564467085,
134.193226110054));
#244248=CARTESIAN_POINT('Ctrl Pts',(-192.109456541119,-3.47021761977078,
134.292260601523));
#244249=CARTESIAN_POINT('Ctrl Pts',(-192.117221294066,-3.37180540278206,
134.387497938163));
#244250=CARTESIAN_POINT('Ctrl Pts',(-192.124986047013,-3.26947915980666,
134.478552921473));
#244251=CARTESIAN_POINT('Ctrl Pts',(-192.132743087898,-3.16725454869806,
134.56951746769));
#244252=CARTESIAN_POINT('Ctrl Pts',(-192.140500128783,-3.06112393801676,
134.656307668951));
#244253=CARTESIAN_POINT('Ctrl Pts',(-192.148257169668,-2.95146527907113,
134.738574105538));
#244254=CARTESIAN_POINT('Ctrl Pts',(-192.156008360908,-2.84188931457368,
134.820778504364));
#244255=CARTESIAN_POINT('Ctrl Pts',(-192.163759552148,-2.72879090890884,
134.898465695044));
#244256=CARTESIAN_POINT('Ctrl Pts',(-192.171510743389,-2.6125818443738,
134.971325840477));
#244257=CARTESIAN_POINT('Ctrl Pts',(-192.179258640166,-2.49642217179069,
135.044155018405));
#244258=CARTESIAN_POINT('Ctrl Pts',(-192.187006536943,-2.37715480046932,
135.112161024362));
#244259=CARTESIAN_POINT('Ctrl Pts',(-192.19475443372,-2.25522112422815,
135.175076891054));
#244260=CARTESIAN_POINT('Ctrl Pts',(-192.202500709804,-2.13331295388346,
135.237979597104));
#244261=CARTESIAN_POINT('Ctrl Pts',(-192.210246985888,-2.00873993520163,
135.29579410257));
#244262=CARTESIAN_POINT('Ctrl Pts',(-192.217993261972,-1.88196838077047,
135.348299225897));
#244263=CARTESIAN_POINT('Ctrl Pts',(-192.225739595237,-1.75519589054102,
135.400804736805));
#244264=CARTESIAN_POINT('Ctrl Pts',(-192.233485928503,-1.62622519338845,
135.448000637764));
#244265=CARTESIAN_POINT('Ctrl Pts',(-192.241232261768,-1.49554253846573,
135.489713921015));
#244266=CARTESIAN_POINT('Ctrl Pts',(-192.248980329771,-1.36483061806836,
135.531436545666));
#244267=CARTESIAN_POINT('Ctrl Pts',(-192.256728397774,-1.2324063493972,
135.567673990578));
#244268=CARTESIAN_POINT('Ctrl Pts',(-192.264476465777,-1.09877070560949,
135.598303253747));
#244269=CARTESIAN_POINT('Ctrl Pts',(-192.272232768519,-0.964993032269096,
135.628965070061));
#244270=CARTESIAN_POINT('Ctrl Pts',(-192.279989071261,-0.830001793655666,
135.654006710523));
#244271=CARTESIAN_POINT('Ctrl Pts',(-192.287745374002,-0.694308261338982,
135.673356314908));
#244272=CARTESIAN_POINT('Ctrl Pts',(-192.295505816517,-0.558542305298078,
135.69271624676));
#244273=CARTESIAN_POINT('Ctrl Pts',(-192.303266259031,-0.422073697493207,
135.706378050116));
#244274=CARTESIAN_POINT('Ctrl Pts',(-192.311026701545,-0.28541738556099,
135.714321918688));
#244275=CARTESIAN_POINT('Ctrl Pts',(-192.31879960181,-0.148541700785455,
135.722278539464));
#244276=CARTESIAN_POINT('Ctrl Pts',(-192.326572502076,-0.0114781008894383,
135.72449887668));
#244277=CARTESIAN_POINT('Ctrl Pts',(-192.334345402341,0.125259011019499,
135.721015297596));
#244278=CARTESIAN_POINT('Ctrl Pts',(-192.341835738103,0.257025384489433,
135.717658355386));
#244279=CARTESIAN_POINT('Ctrl Pts',(-192.349326073865,0.388488287825575,
135.709005020696));
#244280=CARTESIAN_POINT('Ctrl Pts',(-192.356816409627,0.519195120740406,
135.695129421047));
#244281=CARTESIAN_POINT('Ctrl Pts',(-192.364590743746,0.654857742953279,
135.680727723819));
#244282=CARTESIAN_POINT('Ctrl Pts',(-192.372365077865,0.790135568566218,
135.66065431978));
#244283=CARTESIAN_POINT('Ctrl Pts',(-192.380139411984,0.924516415821493,
135.634935372124));
#244284=CARTESIAN_POINT('Ctrl Pts',(-192.387904164931,1.05873165069249,
135.609248120773));
#244285=CARTESIAN_POINT('Ctrl Pts',(-192.395668917878,1.19205172640386,
135.577929242197));
#244286=CARTESIAN_POINT('Ctrl Pts',(-192.403433670826,1.32396869645902,
135.541056718573));
#244287=CARTESIAN_POINT('Ctrl Pts',(-192.411190711711,1.45575464472018,
135.504220817259));
#244288=CARTESIAN_POINT('Ctrl Pts',(-192.418947752595,1.58613988652435,
135.461842352468));
#244289=CARTESIAN_POINT('Ctrl Pts',(-192.42670479348,1.71462615325309,135.414050435448));
#244290=CARTESIAN_POINT('Ctrl Pts',(-192.43445598472,1.84301552748845,135.366294558683));
#244291=CARTESIAN_POINT('Ctrl Pts',(-192.442207175961,1.96950841206677,
135.313133491062));
#244292=CARTESIAN_POINT('Ctrl Pts',(-192.449958367201,2.0936215538718,135.254746202171));
#244293=CARTESIAN_POINT('Ctrl Pts',(-192.457706263978,2.21768194428091,
135.196383729436));
#244294=CARTESIAN_POINT('Ctrl Pts',(-192.465454160755,2.33936425058921,
135.132799619475));
#244295=CARTESIAN_POINT('Ctrl Pts',(-192.473202057532,2.45820528151151,
135.064220927065));
#244296=CARTESIAN_POINT('Ctrl Pts',(-192.480948333616,2.57702145345207,
134.99565657984));
#244297=CARTESIAN_POINT('Ctrl Pts',(-192.4886946097,2.6929971937552,134.922099923534));
#244298=CARTESIAN_POINT('Ctrl Pts',(-192.496440885784,2.80569436276991,
134.843823726102));
#244299=CARTESIAN_POINT('Ctrl Pts',(-192.50418721905,2.91839236368936,134.765546950852));
#244300=CARTESIAN_POINT('Ctrl Pts',(-192.511933552315,3.0278114239197,134.682550787991));
#244301=CARTESIAN_POINT('Ctrl Pts',(-192.51967988558,3.13354315758743,134.59515081778));
#244302=CARTESIAN_POINT('Ctrl Pts',(-192.527427953583,3.23929856914339,
134.507731274952));
#244303=CARTESIAN_POINT('Ctrl Pts',(-192.535176021586,3.34136470970479,
134.415906211393));
#244304=CARTESIAN_POINT('Ctrl Pts',(-192.542924089589,3.43936730597353,
134.320030624421));
#244305=CARTESIAN_POINT('Ctrl Pts',(-192.550680392331,3.53747406056822,
134.224053139734));
#244306=CARTESIAN_POINT('Ctrl Pts',(-192.558436695073,3.63150836371962,
134.124016805884));
#244307=CARTESIAN_POINT('Ctrl Pts',(-192.566192997815,3.72113340261438,
134.020312927916));
#244308=CARTESIAN_POINT('Ctrl Pts',(-192.573953440329,3.81080627709143,
133.916553700066));
#244309=CARTESIAN_POINT('Ctrl Pts',(-192.581713882843,3.896064955127,133.80912333375));
#244310=CARTESIAN_POINT('Ctrl Pts',(-192.589474325357,3.97661443135476,
133.698444363217));
#244311=CARTESIAN_POINT('Ctrl Pts',(-192.597247225623,4.05729321275217,
133.587587720975));
#244312=CARTESIAN_POINT('Ctrl Pts',(-192.605020125888,4.13324746904369,
133.47347237904));
#244313=CARTESIAN_POINT('Ctrl Pts',(-192.612793026153,4.20422638427667,
133.356548614609));
#244314=CARTESIAN_POINT('Ctrl Pts',(-192.620283361916,4.27262503715757,
133.243875323526));
#244315=CARTESIAN_POINT('Ctrl Pts',(-192.627773697678,4.3364036520234,133.128594520953));
#244316=CARTESIAN_POINT('Ctrl Pts',(-192.63526403344,4.39537995294483,133.011127060068));
#244317=CARTESIAN_POINT('Ctrl Pts',(-192.643038367559,4.45659235823986,
132.889205784701));
#244318=CARTESIAN_POINT('Ctrl Pts',(-192.650812701678,4.51282500400254,
132.764542553542));
#244319=CARTESIAN_POINT('Ctrl Pts',(-192.658587035797,4.56382305531772,
132.637582421454));
#244320=CARTESIAN_POINT('Ctrl Pts',(-192.666351788744,4.6147582560922,132.510778756383));
#244321=CARTESIAN_POINT('Ctrl Pts',(-192.674116541692,4.66047155399552,
132.381684181989));
#244322=CARTESIAN_POINT('Ctrl Pts',(-192.681881294639,4.70075400015228,
132.250768199319));
#244323=CARTESIAN_POINT('Ctrl Pts',(-192.689638335524,4.74099643721574,
132.119982244248));
#244324=CARTESIAN_POINT('Ctrl Pts',(-192.697395376409,4.77581864259817,
131.987378852245));
#244325=CARTESIAN_POINT('Ctrl Pts',(-192.705152417294,4.80505991488965,
131.853447018593));
#244326=CARTESIAN_POINT('Ctrl Pts',(-192.712903608534,4.83427913611028,
131.71961618398));
#244327=CARTESIAN_POINT('Ctrl Pts',(-192.720654799774,4.85792571819555,
131.584459282138));
#244328=CARTESIAN_POINT('Ctrl Pts',(-192.728405991014,4.87588902321573,
131.448479625036));
#244329=CARTESIAN_POINT('Ctrl Pts',(-192.736153887791,4.89384469335207,
131.312557762916));
#244330=CARTESIAN_POINT('Ctrl Pts',(-192.743901784568,4.90612183966131,
131.175814227835));
#244331=CARTESIAN_POINT('Ctrl Pts',(-192.751649681345,4.91266112355447,
131.038761444392));
#244332=CARTESIAN_POINT('Ctrl Pts',(-192.759395957429,4.9191990395704,130.901737329437));
#244333=CARTESIAN_POINT('Ctrl Pts',(-192.767142233513,4.92000146188634,
130.764404485061));
#244334=CARTESIAN_POINT('Ctrl Pts',(-192.774888509598,4.91506105272305,
130.627278968305));
#244335=CARTESIAN_POINT('Ctrl Pts',(-192.782634842863,4.91012060709078,
130.490152439319));
#244336=CARTESIAN_POINT('Ctrl Pts',(-192.790381176128,4.89943725946526,
130.353233631717));
#244337=CARTESIAN_POINT('Ctrl Pts',(-192.798127509394,4.88305577391945,
130.217036710942));
#244338=CARTESIAN_POINT('Ctrl Pts',(-192.805875577397,4.86667061985355,
130.080809289811));
#244339=CARTESIAN_POINT('Ctrl Pts',(-192.8136236454,4.84458483533778,129.945304465287));
#244340=CARTESIAN_POINT('Ctrl Pts',(-192.821371713403,4.81689478580987,
129.811029008818));
#244341=CARTESIAN_POINT('Ctrl Pts',(-192.829128016144,4.78917530696777,
129.676610842796));
#244342=CARTESIAN_POINT('Ctrl Pts',(-192.836884318886,4.75583974389208,
129.543425038395));
#244343=CARTESIAN_POINT('Ctrl Pts',(-192.844640621628,4.71703525704713,
129.41196647571));
#244344=CARTESIAN_POINT('Ctrl Pts',(-192.852401064142,4.67821005907918,
129.280437749632));
#244345=CARTESIAN_POINT('Ctrl Pts',(-192.860161506656,4.63391024734856,
129.150638472024));
#244346=CARTESIAN_POINT('Ctrl Pts',(-192.867921949171,4.58433185427907,
129.023045229337));
#244347=CARTESIAN_POINT('Ctrl Pts',(-192.875694849436,4.53467387357166,
128.895247162649));
#244348=CARTESIAN_POINT('Ctrl Pts',(-192.883467749701,4.47972053529839,
128.769662565957));
#244349=CARTESIAN_POINT('Ctrl Pts',(-192.891240649967,4.41971509826897,
128.646745843647));
#244350=CARTESIAN_POINT('Ctrl Pts',(-192.898730985729,4.36189101002015,
128.528297453802));
#244351=CARTESIAN_POINT('Ctrl Pts',(-192.906221321491,4.29937590510965,
128.412326609133));
#244352=CARTESIAN_POINT('Ctrl Pts',(-192.913711657253,4.23242533464076,
128.299214144964));
#244353=CARTESIAN_POINT('Ctrl Pts',(-192.921485991372,4.16293631294325,
128.181812987336));
#244354=CARTESIAN_POINT('Ctrl Pts',(-192.929260325491,4.08844872451645,
128.067119348354));
#244355=CARTESIAN_POINT('Ctrl Pts',(-192.93703465961,4.00919926212544,127.955588190875));
#244356=CARTESIAN_POINT('Ctrl Pts',(-192.944799412557,3.93004746761452,
127.844194485581));
#244357=CARTESIAN_POINT('Ctrl Pts',(-192.952564165504,3.84614570015536,
127.735955822617));
#244358=CARTESIAN_POINT('Ctrl Pts',(-192.960328918452,3.75777602230254,
127.631301773374));
#244359=CARTESIAN_POINT('Ctrl Pts',(-192.968085959337,3.66949411445908,
127.526751668006));
#244360=CARTESIAN_POINT('Ctrl Pts',(-192.975843000222,3.57675337783237,
127.425779388006));
#244361=CARTESIAN_POINT('Ctrl Pts',(-192.983600041107,3.47987835496601,
127.328784449916));
#244362=CARTESIAN_POINT('Ctrl Pts',(-192.991351232347,3.38307638630784,
127.231862656463));
#244363=CARTESIAN_POINT('Ctrl Pts',(-192.999102423587,3.28214661216284,
127.138912510412));
#244364=CARTESIAN_POINT('Ctrl Pts',(-193.006853614827,3.17745268064025,
127.050299146999));
#244365=CARTESIAN_POINT('Ctrl Pts',(-193.014601511604,3.07280324683178,
126.961723446631));
#244366=CARTESIAN_POINT('Ctrl Pts',(-193.022349408381,2.96439313545571,
126.877481114876));
#244367=CARTESIAN_POINT('Ctrl Pts',(-193.030097305158,2.85262138988372,
126.797899052983));
#244368=CARTESIAN_POINT('Ctrl Pts',(-193.037843581242,2.74087302455107,
126.718333637942));
#244369=CARTESIAN_POINT('Ctrl Pts',(-193.045589857326,2.62576474197169,
126.643426780396));
#244370=CARTESIAN_POINT('Ctrl Pts',(-193.053336133411,2.50772674929877,
126.573463595261));
#244371=CARTESIAN_POINT('Ctrl Pts',(-193.061082466676,2.38968788529636,
126.503499893673));
#244372=CARTESIAN_POINT('Ctrl Pts',(-193.068828799941,2.26871960437203,
126.438480136662));
#244373=CARTESIAN_POINT('Ctrl Pts',(-193.076575133207,2.145278684549,126.378644581926));
#244374=CARTESIAN_POINT('Ctrl Pts',(-193.08432320121,2.02181012098801,126.318795627432));
#244375=CARTESIAN_POINT('Ctrl Pts',(-193.092071269213,1.89586816841405,
126.264133355903));
#244376=CARTESIAN_POINT('Ctrl Pts',(-193.099819337216,1.7679312758711,126.214850614712));
#244377=CARTESIAN_POINT('Ctrl Pts',(-193.107575639958,1.63985841047612,
126.165515495237));
#244378=CARTESIAN_POINT('Ctrl Pts',(-193.115331942699,1.50978673510698,
126.121571468042));
#244379=CARTESIAN_POINT('Ctrl Pts',(-193.123088245441,1.37821215022817,
126.08316221764));
#244380=CARTESIAN_POINT('Ctrl Pts',(-193.130848687956,1.24656734003178,
126.044732467064));
#244381=CARTESIAN_POINT('Ctrl Pts',(-193.13860913047,1.11341840134966,126.011843473238));
#244382=CARTESIAN_POINT('Ctrl Pts',(-193.146369572984,0.979272260174981,
125.98458791515));
#244383=CARTESIAN_POINT('Ctrl Pts',(-193.154142473249,0.844910775705553,
125.957288604021));
#244384=CARTESIAN_POINT('Ctrl Pts',(-193.161915373515,0.70954927612074,
125.935640861783));
#244385=CARTESIAN_POINT('Ctrl Pts',(-193.16968827378,0.573701552030352,
125.919685644582));
#244386=CARTESIAN_POINT('Ctrl Pts',(-193.177178609542,0.442792234891523,
125.904310439715));
#244387=CARTESIAN_POINT('Ctrl Pts',(-193.184668945304,0.311431737587399,
125.894221093707));
#244388=CARTESIAN_POINT('Ctrl Pts',(-193.192159281066,0.180078599274265,
125.889408454972));
#244389=CARTESIAN_POINT('Ctrl Pts',(-193.199933615185,0.0437451667967284,
125.884413343577));
#244390=CARTESIAN_POINT('Ctrl Pts',(-193.207707949304,-0.0930122009763956,
125.885087147901));
#244391=CARTESIAN_POINT('Ctrl Pts',(-193.215482283423,-0.229682792687816,
125.891476650155));
#244392=CARTESIAN_POINT('Ctrl Pts',(-193.22324703637,-0.366184950108441,
125.897858277918));
#244393=CARTESIAN_POINT('Ctrl Pts',(-193.231011789318,-0.502600157464022,
125.909941569895));
#244394=CARTESIAN_POINT('Ctrl Pts',(-193.238776542265,-0.638414542478167,
125.927721412698));
#244395=CARTESIAN_POINT('Ctrl Pts',(-193.24653358315,-0.774094034730837,
125.945483596311));
#244396=CARTESIAN_POINT('Ctrl Pts',(-193.254290624035,-0.909173507043042,
125.968931020864));
#244397=CARTESIAN_POINT('Ctrl Pts',(-193.26204766492,-1.04314141166046,
125.998006587974));
#244398=CARTESIAN_POINT('Ctrl Pts',(-193.26979885616,-1.17700829003943,
126.027060228972));
#244399=CARTESIAN_POINT('Ctrl Pts',(-193.2775500474,-1.30976488866881,126.061733482066));
#244400=CARTESIAN_POINT('Ctrl Pts',(-193.28530123864,-1.44090744824757,
126.101917764316));
#244401=CARTESIAN_POINT('Ctrl Pts',(-193.293049135417,-1.57199426873999,
126.142084967174));
#244402=CARTESIAN_POINT('Ctrl Pts',(-193.300797032194,-1.70146804157518,
126.187758426161));
#244403=CARTESIAN_POINT('Ctrl Pts',(-193.308544928971,-1.82883804278507,
126.238779112898));
#244404=CARTESIAN_POINT('Ctrl Pts',(-193.316291205055,-1.95618140093683,
126.289789127208));
#244405=CARTESIAN_POINT('Ctrl Pts',(-193.324037481139,-2.08142150007336,
126.346143999172));
#244406=CARTESIAN_POINT('Ctrl Pts',(-193.331783757224,-2.20408592746605,
126.407635894906));
#244407=CARTESIAN_POINT('Ctrl Pts',(-193.339530090489,-2.32675126033885,
126.469128244559));
#244408=CARTESIAN_POINT('Ctrl Pts',(-193.347276423754,-2.44684053402099,
126.53575751844));
#244409=CARTESIAN_POINT('Ctrl Pts',(-193.35502275702,-2.5639047132275,126.607269281415));
#244410=CARTESIAN_POINT('Ctrl Pts',(-193.362770825023,-2.68099510814607,
126.678797058955));
#244411=CARTESIAN_POINT('Ctrl Pts',(-193.370518893026,-2.79505872696956,
126.755209297555));
#244412=CARTESIAN_POINT('Ctrl Pts',(-193.378266961029,-2.90567470834559,
126.836207703201));
#244413=CARTESIAN_POINT('Ctrl Pts',(-193.38602326377,-3.01640825370252,
126.917292194916));
#244414=CARTESIAN_POINT('Ctrl Pts',(-193.393779566512,-3.12368652605522,
127.002972359134));
#244415=CARTESIAN_POINT('Ctrl Pts',(-193.401535869254,-3.22712059323985,
127.092908645738));
#244416=CARTESIAN_POINT('Ctrl Pts',(-193.409296311768,-3.33060986630048,
127.182892934046));
#244417=CARTESIAN_POINT('Ctrl Pts',(-193.417056754283,-3.4302505619723,
127.277137602611));
#244418=CARTESIAN_POINT('Ctrl Pts',(-193.424817196797,-3.52569070091577,
127.375266255497));
#244419=CARTESIAN_POINT('Ctrl Pts',(-193.432590097062,-3.62128404884331,
127.473552433207));
#244420=CARTESIAN_POINT('Ctrl Pts',(-193.440362997328,-3.71266310439815,
127.57573476299));
#244421=CARTESIAN_POINT('Ctrl Pts',(-193.448135897593,-3.79951569364077,
127.68140311605));
#244422=CARTESIAN_POINT('Ctrl Pts',(-193.455626233355,-3.88321097249688,
127.783230158314));
#244423=CARTESIAN_POINT('Ctrl Pts',(-193.463116569117,-3.9627029824913,
127.888293927058));
#244424=CARTESIAN_POINT('Ctrl Pts',(-193.470606904879,-4.03775157149843,
127.996203693646));
#244425=CARTESIAN_POINT('Ctrl Pts',(-193.47889361498,-4.12077934492612,
128.115586453127));
#244426=CARTESIAN_POINT('Ctrl Pts',(-193.48718032508,-4.19864109136327,
128.238845638589));
#244427=CARTESIAN_POINT('Ctrl Pts',(-193.495467035181,-4.27096326554449,
128.365496979133));
#244428=CARTESIAN_POINT('Ctrl Pts',(-193.503328207986,-4.33957156751243,
128.485644548189));
#244429=CARTESIAN_POINT('Ctrl Pts',(-193.511189380792,-4.40319473039249,
128.608844226595));
#244430=CARTESIAN_POINT('Ctrl Pts',(-193.519050553597,-4.46155570869261,
128.734649594082));
#244431=CARTESIAN_POINT('Ctrl Pts',(-193.526903815789,-4.51985795897289,
128.86032836499));
#244432=CARTESIAN_POINT('Ctrl Pts',(-193.534757077982,-4.57290840298805,
128.988607267093));
#244433=CARTESIAN_POINT('Ctrl Pts',(-193.542610340174,-4.62047497514472,
129.119013749244));
#244434=CARTESIAN_POINT('Ctrl Pts',(-193.550455704939,-4.66799371322391,
129.249289091533));
#244435=CARTESIAN_POINT('Ctrl Pts',(-193.558301069704,-4.71003943508657,
129.381687398499));
#244436=CARTESIAN_POINT('Ctrl Pts',(-193.566146434469,-4.74642766497959,
129.515715017094));
#244437=CARTESIAN_POINT('Ctrl Pts',(-193.567446765008,-4.75245883472166,
129.537929434235));
#244438=CARTESIAN_POINT('Ctrl Pts',(-193.568747095547,-4.75833469270917,
129.560188567407));
#244439=CARTESIAN_POINT('Ctrl Pts',(-193.570047426085,-4.76405452823409,
129.582490119308));
#244440=CARTESIAN_POINT('Ctrl Pts',(-191.820046567589,-4.76405452823394,
129.582490119308));
#244441=CARTESIAN_POINT('Ctrl Pts',(-191.82924828616,-4.80421977364591,
129.739093801576));
#244442=CARTESIAN_POINT('Ctrl Pts',(-191.83845000473,-4.83669951198726,
129.897836547039));
#244443=CARTESIAN_POINT('Ctrl Pts',(-191.847651723301,-4.86129257036642,
130.058024495031));
#244444=CARTESIAN_POINT('Ctrl Pts',(-191.856764218548,-4.88564716520422,
130.216659200447));
#244445=CARTESIAN_POINT('Ctrl Pts',(-191.865876713795,-4.90226722063982,
130.376711144536));
#244446=CARTESIAN_POINT('Ctrl Pts',(-191.874989209043,-4.91100407682167,
130.537486077864));
#244447=CARTESIAN_POINT('Ctrl Pts',(-191.879945951344,-4.91575649023196,
130.624939611869));
#244448=CARTESIAN_POINT('Ctrl Pts',(-191.884902693645,-4.9181772279881,
130.712606716241));
#244449=CARTESIAN_POINT('Ctrl Pts',(-191.889859435946,-4.91824838362704,
130.800373206121));
#244450=CARTESIAN_POINT('Origin',(213.235140564004,0.,130.804360617566));
#244451=CARTESIAN_POINT('',(-190.06976504276,-4.76405452823418,129.582490119309));
#244452=CARTESIAN_POINT('',(-190.415359814329,-4.76405452823405,129.582490119308));
#244453=CARTESIAN_POINT('',(213.235140564004,-4.76405452823405,129.582490119308));
#244454=CARTESIAN_POINT('',(-190.485140563957,-4.91824868249715,130.800760671037));
#244455=CARTESIAN_POINT('Ctrl Pts',(-190.415359814329,-4.76405452823405,
129.582490119308));
#244456=CARTESIAN_POINT('Ctrl Pts',(-190.424329050674,-4.80323055054687,
129.735236835727));
#244457=CARTESIAN_POINT('Ctrl Pts',(-190.433298287018,-4.83509936457335,
129.890036533855));
#244458=CARTESIAN_POINT('Ctrl Pts',(-190.442267523362,-4.85946771299443,
130.04623357751));
#244459=CARTESIAN_POINT('Ctrl Pts',(-190.451168803988,-4.88365143381179,
130.201247189058));
#244460=CARTESIAN_POINT('Ctrl Pts',(-190.460070084614,-4.9004478339706,
130.357636916376));
#244461=CARTESIAN_POINT('Ctrl Pts',(-190.46897136524,-4.90971529438901,
130.51474226431));
#244462=CARTESIAN_POINT('Ctrl Pts',(-190.474361098146,-4.9153267494672,
130.609869684625));
#244463=CARTESIAN_POINT('Ctrl Pts',(-190.479750831051,-4.9181787794553,
130.705259101589));
#244464=CARTESIAN_POINT('Ctrl Pts',(-190.485140563957,-4.91824868249715,
130.800760671037));
#244465=CARTESIAN_POINT('Ctrl Pts',(-190.485140564012,-4.91824868249786,
130.800760672006));
#244466=CARTESIAN_POINT('Ctrl Pts',(-190.492903044254,-4.9183493592558,
130.938305344235));
#244467=CARTESIAN_POINT('Ctrl Pts',(-190.500665524497,-4.91267582439302,
131.075902460375));
#244468=CARTESIAN_POINT('Ctrl Pts',(-190.508428004739,-4.90124163143306,
131.213033509752));
#244469=CARTESIAN_POINT('Ctrl Pts',(-190.516189892968,-4.88980831051287,
131.350154100696));
#244470=CARTESIAN_POINT('Ctrl Pts',(-190.523951781197,-4.87261523719499,
131.486808308646));
#244471=CARTESIAN_POINT('Ctrl Pts',(-190.531713669427,-4.8497279622425,
131.622481485619));
#244472=CARTESIAN_POINT('Ctrl Pts',(-190.539476617656,-4.8268375616964,
131.758173190757));
#244473=CARTESIAN_POINT('Ctrl Pts',(-190.547239565885,-4.7982514760145,
131.892883215297));
#244474=CARTESIAN_POINT('Ctrl Pts',(-190.555002514114,-4.76408655954542,
132.026106219424));
#244475=CARTESIAN_POINT('Ctrl Pts',(-190.562768174686,-4.72990970599202,
132.159375771132));
#244476=CARTESIAN_POINT('Ctrl Pts',(-190.570533835258,-4.69015023823709,
132.291156892345));
#244477=CARTESIAN_POINT('Ctrl Pts',(-190.57829949583,-4.64497503635937,
132.420958889895));
#244478=CARTESIAN_POINT('Ctrl Pts',(-190.586074494797,-4.59974551020291,
132.550916977504));
#244479=CARTESIAN_POINT('Ctrl Pts',(-190.593849493765,-4.54908737022984,
132.678890820855));
#244480=CARTESIAN_POINT('Ctrl Pts',(-190.601624492733,-4.49321610342936,
132.804408644585));
#244481=CARTESIAN_POINT('Ctrl Pts',(-190.609404441072,-4.4373092703673,
132.930006369846));
#244482=CARTESIAN_POINT('Ctrl Pts',(-190.617184389411,-4.37618287100597,
133.053144613246));
#244483=CARTESIAN_POINT('Ctrl Pts',(-190.62496433775,-4.31009818111834,
133.173376601391));
#244484=CARTESIAN_POINT('Ctrl Pts',(-190.632757105409,-4.24390460094357,
133.293806700412));
#244485=CARTESIAN_POINT('Ctrl Pts',(-190.640549873068,-4.17273660894555,
133.411320645231));
#244486=CARTESIAN_POINT('Ctrl Pts',(-190.648342640727,-4.09689905135302,
133.52550030996));
#244487=CARTESIAN_POINT('Ctrl Pts',(-190.654408984015,-4.0378626885938,
133.614384397484));
#244488=CARTESIAN_POINT('Ctrl Pts',(-190.660475327302,-3.97599746982579,
133.701248499452));
#244489=CARTESIAN_POINT('Ctrl Pts',(-190.66654167059,-3.91146342789147,
133.78591003268));
#244490=CARTESIAN_POINT('Ctrl Pts',(-190.674316004709,-3.82875970007991,
133.894408186373));
#244491=CARTESIAN_POINT('Ctrl Pts',(-190.682090338828,-3.74140718917245,
133.999634468692));
#244492=CARTESIAN_POINT('Ctrl Pts',(-190.689864672947,-3.64969402101185,
134.101164617729));
#244493=CARTESIAN_POINT('Ctrl Pts',(-190.697629425894,-3.55809388113412,
134.202569639932));
#244494=CARTESIAN_POINT('Ctrl Pts',(-190.705394178841,-3.46214403645708,
134.300287304914));
#244495=CARTESIAN_POINT('Ctrl Pts',(-190.713158931788,-3.36217471257771,
134.393923859049));
#244496=CARTESIAN_POINT('Ctrl Pts',(-190.720915972673,-3.26230467964042,
134.487467412037));
#244497=CARTESIAN_POINT('Ctrl Pts',(-190.728673013558,-3.15842339566355,
134.576937655122));
#244498=CARTESIAN_POINT('Ctrl Pts',(-190.736430054443,-3.05089977217039,
134.661975637584));
#244499=CARTESIAN_POINT('Ctrl Pts',(-190.744181245683,-2.94345723307797,
134.746949492243));
#244500=CARTESIAN_POINT('Ctrl Pts',(-190.751932436923,-2.83237812705361,
134.827497497584));
#244501=CARTESIAN_POINT('Ctrl Pts',(-190.759683628163,-2.7180661956855,
134.903299409299));
#244502=CARTESIAN_POINT('Ctrl Pts',(-190.76743152494,-2.60380284993743,
134.979069103179));
#244503=CARTESIAN_POINT('Ctrl Pts',(-190.775179421717,-2.48630973685419,
135.050096499908));
#244504=CARTESIAN_POINT('Ctrl Pts',(-190.782927318495,-2.36602129387989,
135.116103455376));
#244505=CARTESIAN_POINT('Ctrl Pts',(-190.790673594579,-2.24575801265473,
135.182096603612));
#244506=CARTESIAN_POINT('Ctrl Pts',(-190.798419870663,-2.12270090711924,
135.243071211466));
#244507=CARTESIAN_POINT('Ctrl Pts',(-190.806166146747,-1.99731049376025,
135.298794269765));
#244508=CARTESIAN_POINT('Ctrl Pts',(-190.813912480012,-1.87191915479789,
135.354517739398));
#244509=CARTESIAN_POINT('Ctrl Pts',(-190.821658813278,-1.74419483091776,
135.404989423349));
#244510=CARTESIAN_POINT('Ctrl Pts',(-190.829405146543,-1.61461919800756,
135.450023961796));
#244511=CARTESIAN_POINT('Ctrl Pts',(-190.837153214546,-1.4850145475326,
135.495068585417));
#244512=CARTESIAN_POINT('Ctrl Pts',(-190.844901282549,-1.35355813227166,
135.534673512303));
#244513=CARTESIAN_POINT('Ctrl Pts',(-190.852649350552,-1.22074762339899,
135.56870299637));
#244514=CARTESIAN_POINT('Ctrl Pts',(-190.860405653294,-1.0877959619372,
135.602768647377));
#244515=CARTESIAN_POINT('Ctrl Pts',(-190.868161956036,-0.953487711347482,
135.631246921252));
#244516=CARTESIAN_POINT('Ctrl Pts',(-190.875918258778,-0.818332142929902,
135.654052934234));
#244517=CARTESIAN_POINT('Ctrl Pts',(-190.883678701292,-0.683104437916002,
135.676871119472));
#244518=CARTESIAN_POINT('Ctrl Pts',(-190.891439143806,-0.54702890166007,
135.694010962518));
#244519=CARTESIAN_POINT('Ctrl Pts',(-190.89919958632,-0.410619808675805,
135.705439522789));
#244520=CARTESIAN_POINT('Ctrl Pts',(-190.906972486586,-0.273991739705651,
135.7168864292));
#244521=CARTESIAN_POINT('Ctrl Pts',(-190.914745386851,-0.137029434847546,
135.722603715419));
#244522=CARTESIAN_POINT('Ctrl Pts',(-190.922518287116,-0.00024795565964834,
135.722610611316));
#244523=CARTESIAN_POINT('Ctrl Pts',(-190.930008622879,0.131561172230973,
135.722617256529));
#244524=CARTESIAN_POINT('Ctrl Pts',(-190.937498958641,0.263202085368852,
135.717321489911));
#244525=CARTESIAN_POINT('Ctrl Pts',(-190.944989294403,0.394220439225914,
135.706785865114));
#244526=CARTESIAN_POINT('Ctrl Pts',(-190.952763628522,0.530206393788766,
135.695850778901));
#244527=CARTESIAN_POINT('Ctrl Pts',(-190.960537962641,0.665952411115588,
135.67923601341));
#244528=CARTESIAN_POINT('Ctrl Pts',(-190.96831229676,0.800945808593782,
135.656954653151));
#244529=CARTESIAN_POINT('Ctrl Pts',(-190.976077049707,0.935772838774291,
135.634700752677));
#244530=CARTESIAN_POINT('Ctrl Pts',(-190.983841802654,1.06984871258484,
135.606794215719));
#244531=CARTESIAN_POINT('Ctrl Pts',(-190.991606555601,1.20266365894648,
135.57330003697));
#244532=CARTESIAN_POINT('Ctrl Pts',(-190.999363596486,1.33534669163104,
135.539839125113));
#244533=CARTESIAN_POINT('Ctrl Pts',(-191.007120637371,1.46677091249836,
135.500801710651));
#244534=CARTESIAN_POINT('Ctrl Pts',(-191.014877678256,1.59643492045341,
135.456304147668));
#244535=CARTESIAN_POINT('Ctrl Pts',(-191.022628869497,1.7260011477716,135.411840140643));
#244536=CARTESIAN_POINT('Ctrl Pts',(-191.030380060737,1.85380943596783,
135.361924307202));
#244537=CARTESIAN_POINT('Ctrl Pts',(-191.038131251977,1.97937212224398,
135.306723226706));
#244538=CARTESIAN_POINT('Ctrl Pts',(-191.045879148754,2.10488144102913,
135.251545608142));
#244539=CARTESIAN_POINT('Ctrl Pts',(-191.053627045531,2.22814669904816,
135.191087367399));
#244540=CARTESIAN_POINT('Ctrl Pts',(-191.061374942308,2.34869906173386,
135.125563665319));
#244541=CARTESIAN_POINT('Ctrl Pts',(-191.069121218392,2.46922620746376,
135.060053669385));
#244542=CARTESIAN_POINT('Ctrl Pts',(-191.076867494477,2.58704124332095,
134.989480506272));
#244543=CARTESIAN_POINT('Ctrl Pts',(-191.084613770561,2.70169921167772,
134.914105674394));
#244544=CARTESIAN_POINT('Ctrl Pts',(-191.092360103826,2.81635802641402,
134.838730286115));
#244545=CARTESIAN_POINT('Ctrl Pts',(-191.100106437091,2.927859400452,134.758553373108));
#244546=CARTESIAN_POINT('Ctrl Pts',(-191.107852770357,3.03578702774157,
134.673879991428));
#244547=CARTESIAN_POINT('Ctrl Pts',(-191.11560083836,3.14373882467452,134.589187647732));
#244548=CARTESIAN_POINT('Ctrl Pts',(-191.123348906363,3.24811497478342,
134.49999707292));
#244549=CARTESIAN_POINT('Ctrl Pts',(-191.131096974365,3.34853226761644,
134.406653597771));
#244550=CARTESIAN_POINT('Ctrl Pts',(-191.138853277107,3.44905628514341,
134.313210916065));
#244551=CARTESIAN_POINT('Ctrl Pts',(-191.146609579849,3.54561275360605,
134.215606783686));
#244552=CARTESIAN_POINT('Ctrl Pts',(-191.154365882591,3.63785498431555,
134.114223783256));
#244553=CARTESIAN_POINT('Ctrl Pts',(-191.162126325105,3.73014644748118,
134.012786671666));
#244554=CARTESIAN_POINT('Ctrl Pts',(-191.16988676762,3.81811883403782,133.907566972984));
#244555=CARTESIAN_POINT('Ctrl Pts',(-191.177647210134,3.9014664522032,133.798979555734));
#244556=CARTESIAN_POINT('Ctrl Pts',(-191.185420110399,3.98494786736428,
133.690217824322));
#244557=CARTESIAN_POINT('Ctrl Pts',(-191.193193010664,4.06378945344856,
133.578077891125));
#244558=CARTESIAN_POINT('Ctrl Pts',(-191.20096591093,4.1377289857357,133.463003486231));
#244559=CARTESIAN_POINT('Ctrl Pts',(-191.208456246692,4.20898062978117,
133.352112325811));
#244560=CARTESIAN_POINT('Ctrl Pts',(-191.215946582454,4.27568028039896,
133.238496606114));
#244561=CARTESIAN_POINT('Ctrl Pts',(-191.223436918216,4.33763498143187,
133.122572391835));
#244562=CARTESIAN_POINT('Ctrl Pts',(-191.231211252335,4.40193871378563,
133.002252875736));
#244563=CARTESIAN_POINT('Ctrl Pts',(-191.238985586454,4.46133427916974,
132.879065220246));
#244564=CARTESIAN_POINT('Ctrl Pts',(-191.246759920573,4.51555556847681,
132.753447832264));
#244565=CARTESIAN_POINT('Ctrl Pts',(-191.25452467352,4.56971003489071,132.627985256485));
#244566=CARTESIAN_POINT('Ctrl Pts',(-191.262289426467,4.61870275977333,
132.500099261741));
#244567=CARTESIAN_POINT('Ctrl Pts',(-191.270054179414,4.66231288128167,
132.370253864098));
#244568=CARTESIAN_POINT('Ctrl Pts',(-191.277811220299,4.70587968860265,
132.240537430734));
#244569=CARTESIAN_POINT('Ctrl Pts',(-191.285568261184,4.74407440781323,
132.108865835533));
#244570=CARTESIAN_POINT('Ctrl Pts',(-191.293325302069,4.77672391135812,
131.975723813658));
#244571=CARTESIAN_POINT('Ctrl Pts',(-191.301076493309,4.80934879365846,
131.842682195218));
#244572=CARTESIAN_POINT('Ctrl Pts',(-191.30882768455,4.83643669095588,131.708172735403));
#244573=CARTESIAN_POINT('Ctrl Pts',(-191.31657887579,4.85786415753015,131.572695758949));
#244574=CARTESIAN_POINT('Ctrl Pts',(-191.324326772567,4.87928251685945,
131.437276363824));
#244575=CARTESIAN_POINT('Ctrl Pts',(-191.332074669344,4.89504516953697,
131.300890655304));
#244576=CARTESIAN_POINT('Ctrl Pts',(-191.339822566121,4.9050797199358,131.164049376877));
#244577=CARTESIAN_POINT('Ctrl Pts',(-191.347568842205,4.91511217132304,
131.027236722695));
#244578=CARTESIAN_POINT('Ctrl Pts',(-191.355315118289,4.91941887513359,
130.889969077825));
#244579=CARTESIAN_POINT('Ctrl Pts',(-191.363061394373,4.91797932692134,
130.752762144001));
#244580=CARTESIAN_POINT('Ctrl Pts',(-191.370807727638,4.91653976808269,
130.615554197346));
#244581=CARTESIAN_POINT('Ctrl Pts',(-191.378554060904,4.90935387668189,
130.478407353576));
#244582=CARTESIAN_POINT('Ctrl Pts',(-191.386300394169,4.89645328142879,
130.341836753008));
#244583=CARTESIAN_POINT('Ctrl Pts',(-191.394048462172,4.88354979717682,
130.205235568402));
#244584=CARTESIAN_POINT('Ctrl Pts',(-191.401796530175,4.86492909924203,
130.069211272942));
#244585=CARTESIAN_POINT('Ctrl Pts',(-191.409544598178,4.84067458957936,
129.934272932157));
#244586=CARTESIAN_POINT('Ctrl Pts',(-191.41730090092,4.81639430193517,129.799191177297));
#244587=CARTESIAN_POINT('Ctrl Pts',(-191.425057203662,4.78646831079896,
129.665198068094));
#244588=CARTESIAN_POINT('Ctrl Pts',(-191.432813506404,4.75103110006152,
129.532792078812));
#244589=CARTESIAN_POINT('Ctrl Pts',(-191.440573948918,4.71557497541762,
129.400315420467));
#244590=CARTESIAN_POINT('Ctrl Pts',(-191.448334391432,4.67460188671874,
129.269427942878));
#244591=CARTESIAN_POINT('Ctrl Pts',(-191.456094833946,4.6282956407281,129.14061107977));
#244592=CARTESIAN_POINT('Ctrl Pts',(-191.463867734212,4.58191505984064,
129.011587428397));
#244593=CARTESIAN_POINT('Ctrl Pts',(-191.471640634477,4.53018436116495,
128.884641396051));
#244594=CARTESIAN_POINT('Ctrl Pts',(-191.479413534742,4.47333512852615,
128.760233446768));
#244595=CARTESIAN_POINT('Ctrl Pts',(-191.486903870504,4.41855250868881,
128.640348039807));
#244596=CARTESIAN_POINT('Ctrl Pts',(-191.494394206266,4.35901717633166,
128.522819662996));
#244597=CARTESIAN_POINT('Ctrl Pts',(-191.501884542028,4.29497488095036,
128.408035548944));
#244598=CARTESIAN_POINT('Ctrl Pts',(-191.509658876147,4.22850440247415,
128.28889936032));
#244599=CARTESIAN_POINT('Ctrl Pts',(-191.517433210267,4.15696789296251,
128.172342252175));
#244600=CARTESIAN_POINT('Ctrl Pts',(-191.525207544386,4.08059035808282,
128.058825079275));
#244601=CARTESIAN_POINT('Ctrl Pts',(-191.532972297333,4.0043069516886,127.945447806144));
#244602=CARTESIAN_POINT('Ctrl Pts',(-191.54073705028,3.92319460690395,127.835103335206));
#244603=CARTESIAN_POINT('Ctrl Pts',(-191.548501803227,3.83752433236579,
127.728228295802));
#244604=CARTESIAN_POINT('Ctrl Pts',(-191.556258844112,3.75193914675227,
127.621459406194));
#244605=CARTESIAN_POINT('Ctrl Pts',(-191.564015884997,3.6618052832676,127.518153393728));
#244606=CARTESIAN_POINT('Ctrl Pts',(-191.571772925882,3.5674369836618,127.418717926717));
#244607=CARTESIAN_POINT('Ctrl Pts',(-191.579524117122,3.47313984792494,
127.319357444764));
#244608=CARTESIAN_POINT('Ctrl Pts',(-191.587275308362,3.37461490002521,
127.223861980993));
#244609=CARTESIAN_POINT('Ctrl Pts',(-191.595026499602,3.27221635190649,
127.132605831525));
#244610=CARTESIAN_POINT('Ctrl Pts',(-191.602774396379,3.16986132590188,
127.041388468354));
#244611=CARTESIAN_POINT('Ctrl Pts',(-191.610522293156,3.06363626547616,
126.954407095373));
#244612=CARTESIAN_POINT('Ctrl Pts',(-191.618270189933,2.95393174198714,
126.871998690406));
#244613=CARTESIAN_POINT('Ctrl Pts',(-191.626016466018,2.84425016631949,
126.789607523499));
#244614=CARTESIAN_POINT('Ctrl Pts',(-191.633762742102,2.73109088767587,
126.711787656611));
#244615=CARTESIAN_POINT('Ctrl Pts',(-191.641509018186,2.61487669737603,
126.638835090094));
#244616=CARTESIAN_POINT('Ctrl Pts',(-191.649255351451,2.49866164920991,
126.565881985059));
#244617=CARTESIAN_POINT('Ctrl Pts',(-191.657001684716,2.37939197551846,
126.497796459953));
#244618=CARTESIAN_POINT('Ctrl Pts',(-191.664748017982,2.25751817453226,
126.434830350574));
#244619=CARTESIAN_POINT('Ctrl Pts',(-191.672496085985,2.1356170807535,126.371850140372));
#244620=CARTESIAN_POINT('Ctrl Pts',(-191.680244153988,2.01111104650626,
126.313991806636));
#244621=CARTESIAN_POINT('Ctrl Pts',(-191.687992221991,1.88447344383008,
126.261460343292));
#244622=CARTESIAN_POINT('Ctrl Pts',(-191.695748524732,1.75770124920225,
126.208873048883));
#244623=CARTESIAN_POINT('Ctrl Pts',(-191.703504827474,1.62879332235594,
126.161624084286));
#244624=CARTESIAN_POINT('Ctrl Pts',(-191.711261130216,1.49824173563579,
126.119869741911));
#244625=CARTESIAN_POINT('Ctrl Pts',(-191.71902157273,1.36762046960263,126.078093113985));
#244626=CARTESIAN_POINT('Ctrl Pts',(-191.726782015244,1.23535417251634,
126.041817055184));
#244627=CARTESIAN_POINT('Ctrl Pts',(-191.734542457759,1.10194724024969,
126.01114715036));
#244628=CARTESIAN_POINT('Ctrl Pts',(-191.742315358024,0.968326151332061,
125.980428011482));
#244629=CARTESIAN_POINT('Ctrl Pts',(-191.750088258289,0.833561152794384,
125.955333082055));
#244630=CARTESIAN_POINT('Ctrl Pts',(-191.757861158555,0.698164822785404,
125.935916416106));
#244631=CARTESIAN_POINT('Ctrl Pts',(-191.765351494317,0.567690490411714,
125.917205594873));
#244632=CARTESIAN_POINT('Ctrl Pts',(-191.772841830079,0.436630237048816,
125.903767397656));
#244633=CARTESIAN_POINT('Ctrl Pts',(-191.780332165842,0.305442686064309,
125.895604377129));
#244634=CARTESIAN_POINT('Ctrl Pts',(-191.788106499961,0.169281119213901,
125.887131853198));
#244635=CARTESIAN_POINT('Ctrl Pts',(-191.79588083408,0.0325510922944527,
125.884315580651));
#244636=CARTESIAN_POINT('Ctrl Pts',(-191.803655168199,-0.104238043468105,
125.887215359106));
#244637=CARTESIAN_POINT('Ctrl Pts',(-191.811419921146,-0.240858598845289,
125.890111563843));
#244638=CARTESIAN_POINT('Ctrl Pts',(-191.819184674093,-0.377537730998018,
125.898709794876));
#244639=CARTESIAN_POINT('Ctrl Pts',(-191.82694942704,-0.513761604507242,
125.913018053787));
#244640=CARTESIAN_POINT('Ctrl Pts',(-191.834706467925,-0.649850178545986,
125.927312101534));
#244641=CARTESIAN_POINT('Ctrl Pts',(-191.84246350881,-0.785484007468369,
125.94730485048));
#244642=CARTESIAN_POINT('Ctrl Pts',(-191.850220549695,-0.920150253035749,
125.972952274822));
#244643=CARTESIAN_POINT('Ctrl Pts',(-191.857971740935,-1.05471494573815,
125.998580358241));
#244644=CARTESIAN_POINT('Ctrl Pts',(-191.865722932175,-1.18831312492588,
126.029854556506));
#244645=CARTESIAN_POINT('Ctrl Pts',(-191.873474123415,-1.32043842446319,
126.066679177273));
#244646=CARTESIAN_POINT('Ctrl Pts',(-191.881222020193,-1.4525075672249,
126.103488146594));
#244647=CARTESIAN_POINT('Ctrl Pts',(-191.88896991697,-1.58310469960573,
126.145842741646));
#244648=CARTESIAN_POINT('Ctrl Pts',(-191.896717813747,-1.71173519926051,
126.193596508428));
#244649=CARTESIAN_POINT('Ctrl Pts',(-191.904464089831,-1.84033879218771,
126.241340286152));
#244650=CARTESIAN_POINT('Ctrl Pts',(-191.912210365915,-1.96697620435051,
126.294480853203));
#244651=CARTESIAN_POINT('Ctrl Pts',(-191.919956641999,-2.09116987323163,
126.352822498692));
#244652=CARTESIAN_POINT('Ctrl Pts',(-191.927702975264,-2.21536445888204,
126.411164574845));
#244653=CARTESIAN_POINT('Ctrl Pts',(-191.93544930853,-2.33711491138994,
126.474707639814));
#244654=CARTESIAN_POINT('Ctrl Pts',(-191.943195641795,-2.45596584886988,
126.543208800078));
#244655=CARTESIAN_POINT('Ctrl Pts',(-191.950943709798,-2.57484340219369,
126.611725300701));
#244656=CARTESIAN_POINT('Ctrl Pts',(-191.958691777801,-2.69081980973953,
126.685201910856));
#244657=CARTESIAN_POINT('Ctrl Pts',(-191.966439845804,-2.80346673516209,
126.763351173462));
#244658=CARTESIAN_POINT('Ctrl Pts',(-191.974196148546,-2.91623338307735,
126.841583494034));
#244659=CARTESIAN_POINT('Ctrl Pts',(-191.981952451288,-3.02566315836508,
126.924498164268));
#244660=CARTESIAN_POINT('Ctrl Pts',(-191.98970875403,-3.13135859067244,
127.011765669628));
#244661=CARTESIAN_POINT('Ctrl Pts',(-191.997469196544,-3.23711043581445,
127.099079752284));
#244662=CARTESIAN_POINT('Ctrl Pts',(-192.005229639058,-3.33912367583414,
127.190751038126));
#244663=CARTESIAN_POINT('Ctrl Pts',(-192.012990081572,-3.43703684091518,
127.286412235811));
#244664=CARTESIAN_POINT('Ctrl Pts',(-192.020762981838,-3.53510718490086,
127.382226997343));
#244665=CARTESIAN_POINT('Ctrl Pts',(-192.028535882103,-3.62906403328069,
127.482044185023));
#244666=CARTESIAN_POINT('Ctrl Pts',(-192.036308782368,-3.71858484786014,
127.58546176986));
#244667=CARTESIAN_POINT('Ctrl Pts',(-192.04379911813,-3.80485135533908,
127.685119864993));
#244668=CARTESIAN_POINT('Ctrl Pts',(-192.051289453892,-3.88699855951138,
127.78812089412));
#244669=CARTESIAN_POINT('Ctrl Pts',(-192.058779789654,-3.9647764156074,
127.894080384196));
#244670=CARTESIAN_POINT('Ctrl Pts',(-192.066605571333,-4.04603746191827,
128.004785145967));
#244671=CARTESIAN_POINT('Ctrl Pts',(-192.074431353011,-4.12278666815336,
128.119070688909));
#244672=CARTESIAN_POINT('Ctrl Pts',(-192.08225713469,-4.19469433982913,
128.236536157463));
#244673=CARTESIAN_POINT('Ctrl Pts',(-192.090069792819,-4.26648142497111,
128.353804640724));
#244674=CARTESIAN_POINT('Ctrl Pts',(-192.097882450948,-4.33344294894402,
128.474242102797));
#244675=CARTESIAN_POINT('Ctrl Pts',(-192.105695109077,-4.3952906467389,
128.597416306264));
#244676=CARTESIAN_POINT('Ctrl Pts',(-192.113500201717,-4.4570784535094,
128.720471232385));
#244677=CARTESIAN_POINT('Ctrl Pts',(-192.121305294356,-4.51376211373051,
128.846257287088));
#244678=CARTESIAN_POINT('Ctrl Pts',(-192.129110386996,-4.5650974649776,
128.974314662472));
#244679=CARTESIAN_POINT('Ctrl Pts',(-192.136908171869,-4.61638475186583,
129.102252140057));
#244680=CARTESIAN_POINT('Ctrl Pts',(-192.144705956742,-4.66233355954381,
129.232456348203));
#244681=CARTESIAN_POINT('Ctrl Pts',(-192.152503741615,-4.70274661817135,
129.364444888164));
#244682=CARTESIAN_POINT('Ctrl Pts',(-192.156767827254,-4.72484580989491,
129.436620569713));
#244683=CARTESIAN_POINT('Ctrl Pts',(-192.161031912893,-4.7452904916293,
129.50932942537));
#244684=CARTESIAN_POINT('Ctrl Pts',(-192.165295998532,-4.76405452823416,
129.582490119309));
#244685=CARTESIAN_POINT('',(-190.13985943604,-4.91824986400714,130.803204030469));
#244686=CARTESIAN_POINT('Ctrl Pts',(-190.13985943604,-4.91824986400714,
130.803204030469));
#244687=CARTESIAN_POINT('Ctrl Pts',(-190.147585601233,-4.91828175505972,
130.938816960416));
#244688=CARTESIAN_POINT('Ctrl Pts',(-190.155311766426,-4.91270043226599,
131.074655996844));
#244689=CARTESIAN_POINT('Ctrl Pts',(-190.163037931618,-4.90147587807679,
131.210214383264));
#244690=CARTESIAN_POINT('Ctrl Pts',(-190.170754697744,-4.89026497882958,
131.345607859624));
#244691=CARTESIAN_POINT('Ctrl Pts',(-190.178471463869,-4.87342453696202,
131.48072097409));
#244692=CARTESIAN_POINT('Ctrl Pts',(-190.186188229995,-4.85097651155595,
131.615045480403));
#244693=CARTESIAN_POINT('Ctrl Pts',(-190.193897512807,-4.82855025506256,
131.749239725884));
#244694=CARTESIAN_POINT('Ctrl Pts',(-190.201606795619,-4.80052729930736,
131.882646496431));
#244695=CARTESIAN_POINT('Ctrl Pts',(-190.209316078432,-4.76698148662643,
132.014761612551));
#244696=CARTESIAN_POINT('Ctrl Pts',(-190.217019786611,-4.73345993114099,
132.14678119537));
#244697=CARTESIAN_POINT('Ctrl Pts',(-190.224723494791,-4.69442356335619,
132.277510599873));
#244698=CARTESIAN_POINT('Ctrl Pts',(-190.232427202971,-4.6499974110266,
132.406455227739));
#244699=CARTESIAN_POINT('Ctrl Pts',(-190.240128016859,-4.60558794964859,
132.535351410974));
#244700=CARTESIAN_POINT('Ctrl Pts',(-190.247828830748,-4.55579285811654,
132.662463776619));
#244701=CARTESIAN_POINT('Ctrl Pts',(-190.255529644636,-4.50078711110052,
132.787312569342));
#244702=CARTESIAN_POINT('Ctrl Pts',(-190.263229171694,-4.44579055572119,
132.912140499431));
#244703=CARTESIAN_POINT('Ctrl Pts',(-190.270928698752,-4.38558523610426,
133.034705246309));
#244704=CARTESIAN_POINT('Ctrl Pts',(-190.27862822581,-4.32039420672799,
133.1545471976));
#244705=CARTESIAN_POINT('Ctrl Pts',(-190.286328185659,-4.25519951295482,
133.274395885223));
#244706=CARTESIAN_POINT('Ctrl Pts',(-190.294028145508,-4.18501874133744,
133.391521124698));
#244707=CARTESIAN_POINT('Ctrl Pts',(-190.301728105358,-4.1101205931154,
133.505488488021));
#244708=CARTESIAN_POINT('Ctrl Pts',(-190.309430217604,-4.03520150834462,
133.619487709051));
#244709=CARTESIAN_POINT('Ctrl Pts',(-190.317132329851,-3.95556264143853,
133.73032696698));
#244710=CARTESIAN_POINT('Ctrl Pts',(-190.324834442098,-3.87151536636673,
133.837601760384));
#244711=CARTESIAN_POINT('Ctrl Pts',(-190.332544856977,-3.78737749100206,
133.944992192609));
#244712=CARTESIAN_POINT('Ctrl Pts',(-190.340255271856,-3.69882196354237,
134.048810176041));
#244713=CARTESIAN_POINT('Ctrl Pts',(-190.347965686736,-3.60619996799212,
134.148684892117));
#244714=CARTESIAN_POINT('Ctrl Pts',(-190.3556806963,-3.51352277841163,134.248619124166));
#244715=CARTESIAN_POINT('Ctrl Pts',(-190.363395705863,-3.41677457553636,
134.344605130585));
#244716=CARTESIAN_POINT('Ctrl Pts',(-190.371110715427,-3.31634172458628,
134.43631059358));
#244717=CARTESIAN_POINT('Ctrl Pts',(-190.378837231148,-3.21575908819369,
134.528152826001));
#244718=CARTESIAN_POINT('Ctrl Pts',(-190.386563746869,-3.11148113317161,
134.615701512883));
#244719=CARTESIAN_POINT('Ctrl Pts',(-190.394290262589,-3.00392586603647,
134.698665748633));
#244720=CARTESIAN_POINT('Ctrl Pts',(-190.398754522705,-2.94178211240861,
134.746601188372));
#244721=CARTESIAN_POINT('Ctrl Pts',(-190.403218782821,-2.87854480706385,
134.793006993218));
#244722=CARTESIAN_POINT('Ctrl Pts',(-190.407683042937,-2.81429844266184,
134.837833976612));
#244723=CARTESIAN_POINT('Ctrl Pts',(-190.415457377056,-2.70241591570069,
134.915898412238));
#244724=CARTESIAN_POINT('Ctrl Pts',(-190.423231711176,-2.58710562699183,
134.989427787118));
#244725=CARTESIAN_POINT('Ctrl Pts',(-190.431006045295,-2.46877148506654,
135.058106075045));
#244726=CARTESIAN_POINT('Ctrl Pts',(-190.438770798242,-2.35058317939566,
135.126699723119));
#244727=CARTESIAN_POINT('Ctrl Pts',(-190.446535551189,-2.2293787702848,
135.19045398537));
#244728=CARTESIAN_POINT('Ctrl Pts',(-190.454300304136,-2.1055929402831,
135.249094741485));
#244729=CARTESIAN_POINT('Ctrl Pts',(-190.462057345021,-1.98193005611249,
135.307677254775));
#244730=CARTESIAN_POINT('Ctrl Pts',(-190.469814385906,-1.85569120437271,
135.361156202688));
#244731=CARTESIAN_POINT('Ctrl Pts',(-190.477571426791,-1.72733727952841,
135.409302417986));
#244732=CARTESIAN_POINT('Ctrl Pts',(-190.485322618031,-1.59908014737782,
135.457412325848));
#244733=CARTESIAN_POINT('Ctrl Pts',(-190.493073809271,-1.46871148143803,
135.500197368803));
#244734=CARTESIAN_POINT('Ctrl Pts',(-190.500825000511,-1.3367135244881,
135.537475872443));
#244735=CARTESIAN_POINT('Ctrl Pts',(-190.508572897288,-1.2047716701905,
135.574738531725));
#244736=CARTESIAN_POINT('Ctrl Pts',(-190.516320794066,-1.07120227765744,
135.606499200586));
#244737=CARTESIAN_POINT('Ctrl Pts',(-190.524068690843,-0.9365039649583,
135.632625666848));
#244738=CARTESIAN_POINT('Ctrl Pts',(-190.531814966927,-0.80183382824242,
135.658746668017));
#244739=CARTESIAN_POINT('Ctrl Pts',(-190.539561243011,-0.666035624636225,
135.679235736398));
#244740=CARTESIAN_POINT('Ctrl Pts',(-190.547307519095,-0.529619024550856,
135.69401160218));
#244741=CARTESIAN_POINT('Ctrl Pts',(-190.55505385236,-0.39320141746932,
135.708787577034));
#244742=CARTESIAN_POINT('Ctrl Pts',(-190.562800185626,-0.25616579349155,
135.717850223034));
#244743=CARTESIAN_POINT('Ctrl Pts',(-190.570546518891,-0.119027422925699,
135.721170104936));
#244744=CARTESIAN_POINT('Ctrl Pts',(-190.578294586894,0.0181416588272017,
135.724490730303));
#244745=CARTESIAN_POINT('Ctrl Pts',(-190.586042654897,0.155413142178313,
135.722066023016));
#244746=CARTESIAN_POINT('Ctrl Pts',(-190.5937907229,0.292271674219316,135.713918676185));
#244747=CARTESIAN_POINT('Ctrl Pts',(-190.601547025642,0.429275661136996,
135.705762670257));
#244748=CARTESIAN_POINT('Ctrl Pts',(-190.609303328384,0.565865429118824,
135.691871898426));
#244749=CARTESIAN_POINT('Ctrl Pts',(-190.617059631125,0.70153010916397,
135.672321029118));
#244750=CARTESIAN_POINT('Ctrl Pts',(-190.62482007364,0.837267197534009,
135.652759724922));
#244751=CARTESIAN_POINT('Ctrl Pts',(-190.632580516154,0.972077830027677,
135.627532375601));
#244752=CARTESIAN_POINT('Ctrl Pts',(-190.640340958668,1.1054622334498,135.596764639862));
#244753=CARTESIAN_POINT('Ctrl Pts',(-190.648113858933,1.23906075735725,
135.565947513022));
#244754=CARTESIAN_POINT('Ctrl Pts',(-190.655886759199,1.37122809985715,
135.529572330681));
#244755=CARTESIAN_POINT('Ctrl Pts',(-190.663659659464,1.50147966778053,
135.487814670905));
#244756=CARTESIAN_POINT('Ctrl Pts',(-190.671149995226,1.62699626312459,
135.447575007244));
#244757=CARTESIAN_POINT('Ctrl Pts',(-190.678640330988,1.75073366284605,
135.402337511017));
#244758=CARTESIAN_POINT('Ctrl Pts',(-190.68613066675,1.8722783195407,135.352300476082));
#244759=CARTESIAN_POINT('Ctrl Pts',(-190.693905000869,1.99843137883754,
135.300366271758));
#244760=CARTESIAN_POINT('Ctrl Pts',(-190.701679334988,2.12262175204157,
135.243096883288));
#244761=CARTESIAN_POINT('Ctrl Pts',(-190.709453669107,2.24436523492668,
135.180661310475));
#244762=CARTESIAN_POINT('Ctrl Pts',(-190.717218422054,2.36595867984999,
135.118302683924));
#244763=CARTESIAN_POINT('Ctrl Pts',(-190.724983175001,2.48511089000259,
135.050790717883));
#244764=CARTESIAN_POINT('Ctrl Pts',(-190.732747927949,2.6013562836682,134.978342954366));
#244765=CARTESIAN_POINT('Ctrl Pts',(-190.740504968834,2.71748622077004,
134.90596714699));
#244766=CARTESIAN_POINT('Ctrl Pts',(-190.748262009719,2.83071475717223,
134.828665503394));
#244767=CARTESIAN_POINT('Ctrl Pts',(-190.756019050603,2.94059996327127,
134.746701916656));
#244768=CARTESIAN_POINT('Ctrl Pts',(-190.763770241844,3.05040230408146,
134.664800139296));
#244769=CARTESIAN_POINT('Ctrl Pts',(-190.771521433084,3.15686602082719,
134.578243649209));
#244770=CARTESIAN_POINT('Ctrl Pts',(-190.779272624324,3.25957760168308,
134.487339971446));
#244771=CARTESIAN_POINT('Ctrl Pts',(-190.787020521101,3.36224552737705,
134.396474930171));
#244772=CARTESIAN_POINT('Ctrl Pts',(-190.794768417878,3.46116419687574,
134.301266634669));
#244773=CARTESIAN_POINT('Ctrl Pts',(-190.802516314655,3.55595286108516,
134.20206312253));
#244774=CARTESIAN_POINT('Ctrl Pts',(-190.810262590739,3.65072169754968,
134.102880361628));
#244775=CARTESIAN_POINT('Ctrl Pts',(-190.818008866823,3.74136197716383,
133.999704328862));
#244776=CARTESIAN_POINT('Ctrl Pts',(-190.825755142907,3.82752983602749,
133.892919896068));
#244777=CARTESIAN_POINT('Ctrl Pts',(-190.833501476173,3.91369833096282,
133.786134675015));
#244778=CARTESIAN_POINT('Ctrl Pts',(-190.841247809438,3.99539409375177,
133.675741305042));
#244779=CARTESIAN_POINT('Ctrl Pts',(-190.848994142703,4.07231384350195,
133.562157387185));
#244780=CARTESIAN_POINT('Ctrl Pts',(-190.856742210706,4.14925081889687,
133.448548032997));
#244781=CARTESIAN_POINT('Ctrl Pts',(-190.864490278709,4.2214094337795,133.331747032808));
#244782=CARTESIAN_POINT('Ctrl Pts',(-190.872238346712,4.28853021966979,
133.212200233794));
#244783=CARTESIAN_POINT('Ctrl Pts',(-190.879994649454,4.3557223423298,133.092526379021));
#244784=CARTESIAN_POINT('Ctrl Pts',(-190.887750952196,4.41786574856622,
132.970101237319));
#244785=CARTESIAN_POINT('Ctrl Pts',(-190.895507254938,4.47474712186675,
132.845394977356));
#244786=CARTESIAN_POINT('Ctrl Pts',(-190.903267697452,4.53165885446903,
132.720622157908));
#244787=CARTESIAN_POINT('Ctrl Pts',(-190.911028139966,4.5833028108051,132.593566156235));
#244788=CARTESIAN_POINT('Ctrl Pts',(-190.91878858248,4.62951457148501,132.464715367283));
#244789=CARTESIAN_POINT('Ctrl Pts',(-190.926561482746,4.67580051538552,
132.335657735606));
#244790=CARTESIAN_POINT('Ctrl Pts',(-190.934334383011,4.71663672127184,
132.204799932619));
#244791=CARTESIAN_POINT('Ctrl Pts',(-190.942107283277,4.75190897349856,
132.072644564513));
#244792=CARTESIAN_POINT('Ctrl Pts',(-190.949597619039,4.78589899051188,
131.945293376915));
#244793=CARTESIAN_POINT('Ctrl Pts',(-190.957087954801,4.81472249074796,
131.816737626403));
#244794=CARTESIAN_POINT('Ctrl Pts',(-190.964578290563,4.83832277197152,
131.687432424795));
#244795=CARTESIAN_POINT('Ctrl Pts',(-190.972352624682,4.86281786503052,
131.553224577167));
#244796=CARTESIAN_POINT('Ctrl Pts',(-190.980126958801,4.88176343679289,
131.417784195585));
#244797=CARTESIAN_POINT('Ctrl Pts',(-190.98790129292,4.89503994736683,131.281610003299));
#244798=CARTESIAN_POINT('Ctrl Pts',(-190.995666045867,4.90830009582805,
131.145603633535));
#244799=CARTESIAN_POINT('Ctrl Pts',(-191.003430798814,4.91590504680117,
131.008865637851));
#244800=CARTESIAN_POINT('Ctrl Pts',(-191.011195551762,4.91778616625509,
130.871905310104));
#244801=CARTESIAN_POINT('Ctrl Pts',(-191.018952592647,4.91966541735466,
130.735081013285));
#244802=CARTESIAN_POINT('Ctrl Pts',(-191.026709633532,4.9158321449874,130.59803521225));
#244803=CARTESIAN_POINT('Ctrl Pts',(-191.034466674417,4.90626949612716,
130.461282355544));
#244804=CARTESIAN_POINT('Ctrl Pts',(-191.042217865657,4.89671405853478,
130.324632625231));
#244805=CARTESIAN_POINT('Ctrl Pts',(-191.049969056897,4.88143787143859,
130.18827578797));
#244806=CARTESIAN_POINT('Ctrl Pts',(-191.057720248137,4.86047615113323,
130.052725967776));
#244807=CARTESIAN_POINT('Ctrl Pts',(-191.065468144914,4.83952334011826,
129.917233759872));
#244808=CARTESIAN_POINT('Ctrl Pts',(-191.073216041691,4.81288986175936,
129.782548272388));
#244809=CARTESIAN_POINT('Ctrl Pts',(-191.080963938468,4.78066272575466,
129.649177963143));
#244810=CARTESIAN_POINT('Ctrl Pts',(-191.088710214552,4.74844233097209,
129.515835552091));
#244811=CARTESIAN_POINT('Ctrl Pts',(-191.096456490636,4.71063069765271,
129.383808151861));
#244812=CARTESIAN_POINT('Ctrl Pts',(-191.104202766721,4.66736576253298,
129.253593097518));
#244813=CARTESIAN_POINT('Ctrl Pts',(-191.111949099986,4.62410050804126,
129.123377081957));
#244814=CARTESIAN_POINT('Ctrl Pts',(-191.119695433251,4.57538199469793,
128.994973810001));
#244815=CARTESIAN_POINT('Ctrl Pts',(-191.127441766517,4.52139763135042,
128.868864164012));
#244816=CARTESIAN_POINT('Ctrl Pts',(-191.13518983452,4.46740117857896,128.742726276643));
#244817=CARTESIAN_POINT('Ctrl Pts',(-191.142937902523,4.40813668305963,
128.618883396679));
#244818=CARTESIAN_POINT('Ctrl Pts',(-191.150685970526,4.34383899959804,
128.49779481359));
#244819=CARTESIAN_POINT('Ctrl Pts',(-191.158442273267,4.2794729797934,128.376577536114));
#244820=CARTESIAN_POINT('Ctrl Pts',(-191.166198576009,4.21006326982718,
128.258120748965));
#244821=CARTESIAN_POINT('Ctrl Pts',(-191.173954878751,4.13589013312932,
128.142858059013));
#244822=CARTESIAN_POINT('Ctrl Pts',(-191.181715321265,4.0616774079951,128.027533849893));
#244823=CARTESIAN_POINT('Ctrl Pts',(-191.18947576378,3.98269641524828,127.915407454376));
#244824=CARTESIAN_POINT('Ctrl Pts',(-191.197236206294,3.89926918269119,
127.806881192547));
#244825=CARTESIAN_POINT('Ctrl Pts',(-191.205009106559,3.81570802533407,
127.698180714727));
#244826=CARTESIAN_POINT('Ctrl Pts',(-191.212782006825,3.72768661635664,
127.59309221928));
#244827=CARTESIAN_POINT('Ctrl Pts',(-191.22055490709,3.63556607623541,127.491983469984));
#244828=CARTESIAN_POINT('Ctrl Pts',(-191.228045242852,3.54679434978573,
127.394550278402));
#244829=CARTESIAN_POINT('Ctrl Pts',(-191.235535578614,3.4542165619243,127.300812728031));
#244830=CARTESIAN_POINT('Ctrl Pts',(-191.243025914376,3.35818496216893,
127.21106452312));
#244831=CARTESIAN_POINT('Ctrl Pts',(-191.250800248495,3.25851229511997,
127.11791348774));
#244832=CARTESIAN_POINT('Ctrl Pts',(-191.258574582614,3.15480301053301,
127.02876520709));
#244833=CARTESIAN_POINT('Ctrl Pts',(-191.266348916733,3.04741208417123,
126.943989825563));
#244834=CARTESIAN_POINT('Ctrl Pts',(-191.27411366968,2.94015350752896,126.859318922119));
#244835=CARTESIAN_POINT('Ctrl Pts',(-191.281878422628,2.82922262090105,
126.779010434803));
#244836=CARTESIAN_POINT('Ctrl Pts',(-191.289643175575,2.71501080926322,
126.703397393141));
#244837=CARTESIAN_POINT('Ctrl Pts',(-191.29740021646,2.60091243440618,126.627859451418));
#244838=CARTESIAN_POINT('Ctrl Pts',(-191.305157257345,2.48353994330888,
126.557007889035));
#244839=CARTESIAN_POINT('Ctrl Pts',(-191.31291429823,2.3633170466302,126.491134956926));
#244840=CARTESIAN_POINT('Ctrl Pts',(-191.32066548947,2.24318481097262,126.425311700106));
#244841=CARTESIAN_POINT('Ctrl Pts',(-191.32841668071,2.12020678969177,126.364459787714));
#244842=CARTESIAN_POINT('Ctrl Pts',(-191.33616787195,1.99483456514794,126.30882748787));
#244843=CARTESIAN_POINT('Ctrl Pts',(-191.343915768727,1.86951562714447,
126.253218833238));
#244844=CARTESIAN_POINT('Ctrl Pts',(-191.351663665504,1.74180486642149,
126.20282553702));
#244845=CARTESIAN_POINT('Ctrl Pts',(-191.359411562281,1.61217709380733,
126.157849229363));
#244846=CARTESIAN_POINT('Ctrl Pts',(-191.367157838366,1.48257643652876,
126.112882329779));
#244847=CARTESIAN_POINT('Ctrl Pts',(-191.37490411445,1.35105993409509,126.073330292999));
#244848=CARTESIAN_POINT('Ctrl Pts',(-191.382650390534,1.21812056675712,
126.03934589069));
#244849=CARTESIAN_POINT('Ctrl Pts',(-191.390396723799,1.08518021809113,
126.005361237516));
#244850=CARTESIAN_POINT('Ctrl Pts',(-191.398143057064,0.950817362346455,
125.976944397655));
#244851=CARTESIAN_POINT('Ctrl Pts',(-191.40588939033,0.815537878534929,
125.9541976274));
#244852=CARTESIAN_POINT('Ctrl Pts',(-191.413637458333,0.68022809982115,
125.931445763164));
#244853=CARTESIAN_POINT('Ctrl Pts',(-191.421385526336,0.544001670051006,
125.914366560051));
#244854=CARTESIAN_POINT('Ctrl Pts',(-191.429133594339,0.407371947222745,
125.90301068524));
#244855=CARTESIAN_POINT('Ctrl Pts',(-191.436889897081,0.270597012698589,
125.89164274127));
#244856=CARTESIAN_POINT('Ctrl Pts',(-191.444646199823,0.133418319135421,
125.886010309127));
#244857=CARTESIAN_POINT('Ctrl Pts',(-191.452402502564,-0.00364783849507481,
125.886111970357));
#244858=CARTESIAN_POINT('Ctrl Pts',(-191.460162945079,-0.14078715246088,
125.886213685846));
#244859=CARTESIAN_POINT('Ctrl Pts',(-191.467923387593,-0.277813420392517,
125.892055576286));
#244860=CARTESIAN_POINT('Ctrl Pts',(-191.475683830107,-0.414214095113777,
125.903584174398));
#244861=CARTESIAN_POINT('Ctrl Pts',(-191.483456730372,-0.550833732307181,
125.91513127924));
#244862=CARTESIAN_POINT('Ctrl Pts',(-191.491229630638,-0.686825381383332,
125.93238328479));
#244863=CARTESIAN_POINT('Ctrl Pts',(-191.499002530903,-0.821684437819978,
125.95523515547));
#244864=CARTESIAN_POINT('Ctrl Pts',(-191.506492866665,-0.951641027862406,
125.977256303091));
#244865=CARTESIAN_POINT('Ctrl Pts',(-191.513983202427,-1.08054563945036,
126.004477182315));
#244866=CARTESIAN_POINT('Ctrl Pts',(-191.521473538189,-1.20796077141146,
126.036760189968));
#244867=CARTESIAN_POINT('Ctrl Pts',(-191.529247872308,-1.3402068868303,
126.07026721767));
#244868=CARTESIAN_POINT('Ctrl Pts',(-191.537022206427,-1.47126726171084,
126.109333952733));
#244869=CARTESIAN_POINT('Ctrl Pts',(-191.544796540546,-1.6006386100197,
126.153861816081));
#244870=CARTESIAN_POINT('Ctrl Pts',(-191.552561293493,-1.72985051970473,
126.198334802817));
#244871=CARTESIAN_POINT('Ctrl Pts',(-191.560326046441,-1.85737717839847,
126.248255400426));
#244872=CARTESIAN_POINT('Ctrl Pts',(-191.568090799388,-1.98272684579087,
126.303474336234));
#244873=CARTESIAN_POINT('Ctrl Pts',(-191.575847840273,-2.10795201412615,
126.358638427817));
#244874=CARTESIAN_POINT('Ctrl Pts',(-191.583604881158,-2.2310041385998,
126.419090228625));
#244875=CARTESIAN_POINT('Ctrl Pts',(-191.591361922043,-2.35140831426397,
126.484631227649));
#244876=CARTESIAN_POINT('Ctrl Pts',(-191.599113113283,-2.47172169220282,
126.550122801696));
#244877=CARTESIAN_POINT('Ctrl Pts',(-191.606864304523,-2.58939075392098,
126.62069574888));
#244878=CARTESIAN_POINT('Ctrl Pts',(-191.614615495763,-2.70396253312058,
126.696104335154));
#244879=CARTESIAN_POINT('Ctrl Pts',(-191.62236339254,-2.81848561625756,
126.771480870767));
#244880=CARTESIAN_POINT('Ctrl Pts',(-191.630111289317,-2.92991370925743,
126.851688743189));
#244881=CARTESIAN_POINT('Ctrl Pts',(-191.637859186094,-3.03782052811709,
126.936437466642));
#244882=CARTESIAN_POINT('Ctrl Pts',(-191.645605462178,-3.14570477519644,
127.02116846249));
#244883=CARTESIAN_POINT('Ctrl Pts',(-191.653351738262,-3.25006890594588,
127.110438178736));
#244884=CARTESIAN_POINT('Ctrl Pts',(-191.661098014347,-3.35051792136731,
127.203914433953));
#244885=CARTESIAN_POINT('Ctrl Pts',(-191.668844347612,-3.45096767828041,
127.29739137919));
#244886=CARTESIAN_POINT('Ctrl Pts',(-191.676590680877,-3.54750197598732,
127.395074659016));
#244887=CARTESIAN_POINT('Ctrl Pts',(-191.684337014142,-3.63976134341008,
127.496593935117));
#244888=CARTESIAN_POINT('Ctrl Pts',(-191.692085082145,-3.73204137167862,
127.598135945756));
#244889=CARTESIAN_POINT('Ctrl Pts',(-191.699833150149,-3.82004430177213,
127.70351537279));
#244890=CARTESIAN_POINT('Ctrl Pts',(-191.707581218151,-3.90345002342118,
127.812327700442));
#244891=CARTESIAN_POINT('Ctrl Pts',(-191.715337520893,-3.98694438966386,
127.921255675131));
#244892=CARTESIAN_POINT('Ctrl Pts',(-191.723093823635,-4.06583154899084,
128.033623527975));
#244893=CARTESIAN_POINT('Ctrl Pts',(-191.730850126377,-4.13983362474526,
128.148996118683));
#244894=CARTESIAN_POINT('Ctrl Pts',(-191.738610568891,-4.21387519763547,
128.264430287216));
#244895=CARTESIAN_POINT('Ctrl Pts',(-191.746371011405,-4.28302629462755,
128.38287205169));
#244896=CARTESIAN_POINT('Ctrl Pts',(-191.754131453919,-4.34705485498703,
128.503861291282));
#244897=CARTESIAN_POINT('Ctrl Pts',(-191.761904354185,-4.41118619967579,
128.625044753542));
#244898=CARTESIAN_POINT('Ctrl Pts',(-191.76967725445,-4.47017840691058,
128.748783509796));
#244899=CARTESIAN_POINT('Ctrl Pts',(-191.777450154716,-4.52384709502806,
128.874596247674));
#244900=CARTESIAN_POINT('Ctrl Pts',(-191.784940490478,-4.57556479114977,
128.995835375627));
#244901=CARTESIAN_POINT('Ctrl Pts',(-191.79243082624,-4.62233918575824,
129.119000026256));
#244902=CARTESIAN_POINT('Ctrl Pts',(-191.799921162002,-4.6640495682308,
129.243647739556));
#244903=CARTESIAN_POINT('Ctrl Pts',(-191.806629630531,-4.70140607627558,
129.355284292103));
#244904=CARTESIAN_POINT('Ctrl Pts',(-191.81333809906,-4.73477224984779,
129.468318960301));
#244905=CARTESIAN_POINT('Ctrl Pts',(-191.820046567589,-4.76405452823394,
129.582490119308));
#244906=CARTESIAN_POINT('Ctrl Pts',(-190.06976504276,-4.76405452823418,
129.582490119309));
#244907=CARTESIAN_POINT('Ctrl Pts',(-190.077527632497,-4.79811061399697,
129.715274280825));
#244908=CARTESIAN_POINT('Ctrl Pts',(-190.085290222234,-4.82658033576797,
129.849363494492));
#244909=CARTESIAN_POINT('Ctrl Pts',(-190.093052811971,-4.84939154448578,
129.984247996782));
#244910=CARTESIAN_POINT('Ctrl Pts',(-190.100826943755,-4.87223667075837,
130.119333056286));
#244911=CARTESIAN_POINT('Ctrl Pts',(-190.10860107554,-4.88940643253583,
130.255215378942));
#244912=CARTESIAN_POINT('Ctrl Pts',(-190.116375207325,-4.90088061235472,
130.391380852994));
#244913=CARTESIAN_POINT('Ctrl Pts',(-190.120661944591,-4.90720759465933,
130.466463914131));
#244914=CARTESIAN_POINT('Ctrl Pts',(-190.124948681858,-4.91180373898945,
130.541633066273));
#244915=CARTESIAN_POINT('Ctrl Pts',(-190.129235419125,-4.91467242218679,
130.616802506313));
#244916=CARTESIAN_POINT('Ctrl Pts',(-190.132776758081,-4.91704228507516,
130.678901125798));
#244917=CARTESIAN_POINT('Ctrl Pts',(-190.136318097038,-4.91823524652186,
130.741044945587));
#244918=CARTESIAN_POINT('Ctrl Pts',(-190.139859435995,-4.91824986400696,
130.803204029673));
#244919=CARTESIAN_POINT('Origin',(213.235140564004,0.,130.804360617566));
#244920=CARTESIAN_POINT('',(-188.319844903182,-4.76405452823404,129.582490119308));
#244921=CARTESIAN_POINT('',(-188.665047832579,-4.76405452823406,129.582490119308));
#244922=CARTESIAN_POINT('',(213.235140564004,-4.76405452823405,129.582490119308));
#244923=CARTESIAN_POINT('',(-188.735140564044,-4.9182496381179,130.802473913264));
#244924=CARTESIAN_POINT('Ctrl Pts',(-188.665047832579,-4.76405452823406,
129.582490119308));
#244925=CARTESIAN_POINT('Ctrl Pts',(-188.672812177752,-4.7980988056188,
129.715228240137));
#244926=CARTESIAN_POINT('Ctrl Pts',(-188.680576522925,-4.82655782458609,
129.849259699109));
#244927=CARTESIAN_POINT('Ctrl Pts',(-188.688340868098,-4.84936224031761,
129.984074737716));
#244928=CARTESIAN_POINT('Ctrl Pts',(-188.696116115444,-4.87219867648161,
130.119079074566));
#244929=CARTESIAN_POINT('Ctrl Pts',(-188.703891362791,-4.88936461210996,
130.254868801069));
#244930=CARTESIAN_POINT('Ctrl Pts',(-188.711666610137,-4.90084263355078,
130.390930401361));
#244931=CARTESIAN_POINT('Ctrl Pts',(-188.713580508058,-4.90366797921412,
130.424422328024));
#244932=CARTESIAN_POINT('Ctrl Pts',(-188.715494405978,-4.90614893497245,
130.457930736052));
#244933=CARTESIAN_POINT('Ctrl Pts',(-188.717408303899,-4.90828572440508,
130.491447993817));
#244934=CARTESIAN_POINT('Ctrl Pts',(-188.72331905727,-4.91488484090139,
130.594960434142));
#244935=CARTESIAN_POINT('Ctrl Pts',(-188.729229810641,-4.9182098228819,
130.6986838224));
#244936=CARTESIAN_POINT('Ctrl Pts',(-188.735140564012,-4.91824963811768,
130.802473912695));
#244937=CARTESIAN_POINT('Ctrl Pts',(-188.735140564045,-4.9182496381179,
130.802473913264));
#244938=CARTESIAN_POINT('Ctrl Pts',(-188.742840932869,-4.91830150830916,
130.937688821655));
#244939=CARTESIAN_POINT('Ctrl Pts',(-188.750541301692,-4.91277307334292,
131.073131498441));
#244940=CARTESIAN_POINT('Ctrl Pts',(-188.758241670516,-4.90163420131192,
131.208297764941));
#244941=CARTESIAN_POINT('Ctrl Pts',(-188.76593290635,-4.89050854049381,
131.343303718052));
#244942=CARTESIAN_POINT('Ctrl Pts',(-188.773624142184,-4.87378571052704,
131.478033519156));
#244943=CARTESIAN_POINT('Ctrl Pts',(-188.781315378017,-4.85148756347388,
131.611981496418));
#244944=CARTESIAN_POINT('Ctrl Pts',(-188.788999416841,-4.82921028172503,
131.745804132983));
#244945=CARTESIAN_POINT('Ctrl Pts',(-188.796683455665,-4.80136812688925,
131.87884601002));
#244946=CARTESIAN_POINT('Ctrl Pts',(-188.804367494489,-4.76803483755962,
132.010605555511));
#244947=CARTESIAN_POINT('Ctrl Pts',(-188.812346179207,-4.73342337706943,
132.147417445207));
#244948=CARTESIAN_POINT('Ctrl Pts',(-188.820324863925,-4.69289129475855,
132.282846262811));
#244949=CARTESIAN_POINT('Ctrl Pts',(-188.828303548642,-4.64657983212241,
132.416340433263));
#244950=CARTESIAN_POINT('Ctrl Pts',(-188.835979763627,-4.6020240242359,
132.544773876606));
#244951=CARTESIAN_POINT('Ctrl Pts',(-188.843655978612,-4.55211916674477,
132.671416266738));
#244952=CARTESIAN_POINT('Ctrl Pts',(-188.851332193597,-4.49704201443896,
132.795791305004));
#244953=CARTESIAN_POINT('Ctrl Pts',(-188.859007503027,-4.44197135952829,
132.920151670875));
#244954=CARTESIAN_POINT('Ctrl Pts',(-188.866682812457,-4.3817297846288,
133.042244852048));
#244955=CARTESIAN_POINT('Ctrl Pts',(-188.874358121887,-4.31654198168248,
133.161615033804));
#244956=CARTESIAN_POINT('Ctrl Pts',(-188.882034263867,-4.25134710773214,
133.280998163795));
#244957=CARTESIAN_POINT('Ctrl Pts',(-188.889710405848,-4.18120513001891,
133.397657356846));
#244958=CARTESIAN_POINT('Ctrl Pts',(-188.897386547828,-4.10638618677583,
133.511162336857));
#244959=CARTESIAN_POINT('Ctrl Pts',(-188.905065260793,-4.03154218428859,
133.624705333297));
#244960=CARTESIAN_POINT('Ctrl Pts',(-188.912743973757,-3.95201832019808,
133.735091682711));
#244961=CARTESIAN_POINT('Ctrl Pts',(-188.920422686722,-3.86812714267184,
133.841921394016));
#244962=CARTESIAN_POINT('Ctrl Pts',(-188.928109823954,-3.78414392866631,
133.94886830752));
#244963=CARTESIAN_POINT('Ctrl Pts',(-188.935796961185,-3.69578408429893,
134.052250480927));
#244964=CARTESIAN_POINT('Ctrl Pts',(-188.943484098417,-3.60339959857195,
134.151702009703));
#244965=CARTESIAN_POINT('Ctrl Pts',(-188.951176241949,-3.5109549468263,
134.251218306957));
#244966=CARTESIAN_POINT('Ctrl Pts',(-188.958868385481,-3.41448071785227,
134.346798583313));
#244967=CARTESIAN_POINT('Ctrl Pts',(-188.966560529013,-3.31436367286446,
134.438115769815));
#244968=CARTESIAN_POINT('Ctrl Pts',(-188.974263479165,-3.21410597437231,
134.529561246983));
#244969=CARTESIAN_POINT('Ctrl Pts',(-188.981966429318,-3.11019555105514,
134.616731427316));
#244970=CARTESIAN_POINT('Ctrl Pts',(-188.98966937947,-3.00305014572403,
134.699341090529));
#244971=CARTESIAN_POINT('Ctrl Pts',(-188.991731562218,-2.97436588814104,
134.721456801895));
#244972=CARTESIAN_POINT('Ctrl Pts',(-188.993793744965,-2.94544992466852,
134.743245908247));
#244973=CARTESIAN_POINT('Ctrl Pts',(-188.995855927712,-2.91631057808861,
134.764703490933));
#244974=CARTESIAN_POINT('Ctrl Pts',(-189.003630261831,-2.80645658157905,
134.84559759084));
#244975=CARTESIAN_POINT('Ctrl Pts',(-189.01140459595,-2.69306021115118,
134.92204557856));
#244976=CARTESIAN_POINT('Ctrl Pts',(-189.01917893007,-2.57651717925398,
134.993721223614));
#244977=CARTESIAN_POINT('Ctrl Pts',(-189.026943683017,-2.46011777622816,
135.065308534842));
#244978=CARTESIAN_POINT('Ctrl Pts',(-189.034708435964,-2.34057975758224,
135.132135002961));
#244979=CARTESIAN_POINT('Ctrl Pts',(-189.042473188911,-2.21833066914151,
135.193915504436));
#244980=CARTESIAN_POINT('Ctrl Pts',(-189.050230229796,-2.09620300021883,
135.255634644646));
#244981=CARTESIAN_POINT('Ctrl Pts',(-189.057987270681,-1.97136996672141,
135.312317616571));
#244982=CARTESIAN_POINT('Ctrl Pts',(-189.065744311566,-1.84428646499388,
135.363723566218));
#244983=CARTESIAN_POINT('Ctrl Pts',(-189.073495502806,-1.71729879792339,
135.415090750238));
#244984=CARTESIAN_POINT('Ctrl Pts',(-189.081246694046,-1.58806440155843,
135.461188686808));
#244985=CARTESIAN_POINT('Ctrl Pts',(-189.088997885286,-1.4570607255567,
135.501823454517));
#244986=CARTESIAN_POINT('Ctrl Pts',(-189.096745782063,-1.32611272961209,
135.542440951367));
#244987=CARTESIAN_POINT('Ctrl Pts',(-189.10449367884,-1.19339732231602,
135.57759978204));
#244988=CARTESIAN_POINT('Ctrl Pts',(-189.112241575618,-1.05940958549109,
135.607155053378));
#244989=CARTESIAN_POINT('Ctrl Pts',(-189.119987851702,-0.925449876012263,
135.636704142391));
#244990=CARTESIAN_POINT('Ctrl Pts',(-189.127734127786,-0.790218747924846,
135.660651919364));
#244991=CARTESIAN_POINT('Ctrl Pts',(-189.13548040387,-0.65422363177214,
135.678904134874));
#244992=CARTESIAN_POINT('Ctrl Pts',(-189.143226737135,-0.518227511734195,
135.697156485118));
#244993=CARTESIAN_POINT('Ctrl Pts',(-189.150973070401,-0.381467779868424,
135.709713137999));
#244994=CARTESIAN_POINT('Ctrl Pts',(-189.158719403666,-0.244458787537432,
135.716531518878));
#244995=CARTESIAN_POINT('Ctrl Pts',(-189.166467471669,-0.107419112992374,
135.723351426686));
#244996=CARTESIAN_POINT('Ctrl Pts',(-189.174215539672,0.0298695426863131,
135.72443048597));
#244997=CARTESIAN_POINT('Ctrl Pts',(-189.181963607675,0.166891415319874,
135.71977823136));
#244998=CARTESIAN_POINT('Ctrl Pts',(-189.189719910417,0.304058916429691,
135.715121032278));
#244999=CARTESIAN_POINT('Ctrl Pts',(-189.197476213158,0.440958676729197,
135.704720364546));
#245000=CARTESIAN_POINT('Ctrl Pts',(-189.2052325159,0.577078088149238,135.688637835607));
#245001=CARTESIAN_POINT('Ctrl Pts',(-189.212992958415,0.713270150598,135.672546722939));
#245002=CARTESIAN_POINT('Ctrl Pts',(-189.220753400929,0.848680648448811,
135.650767768445));
#245003=CARTESIAN_POINT('Ctrl Pts',(-189.228513843443,0.982806764623835,
135.623413836395));
#245004=CARTESIAN_POINT('Ctrl Pts',(-189.236286743708,1.1171481919477,135.596015993386));
#245005=CARTESIAN_POINT('Ctrl Pts',(-189.244059643974,1.25020073776289,
135.563025383117));
#245006=CARTESIAN_POINT('Ctrl Pts',(-189.251832544239,1.38147548620193,
135.524605160333));
#245007=CARTESIAN_POINT('Ctrl Pts',(-189.259322880001,1.50797806687371,
135.487581609423));
#245008=CARTESIAN_POINT('Ctrl Pts',(-189.266813215763,1.63282956904491,
135.445516450911));
#245009=CARTESIAN_POINT('Ctrl Pts',(-189.274303551525,1.75561151980122,
135.398597360926));
#245010=CARTESIAN_POINT('Ctrl Pts',(-189.282077885644,1.88304878554009,
135.349899319384));
#245011=CARTESIAN_POINT('Ctrl Pts',(-189.289852219764,2.0086601508045,135.295817746099));
#245012=CARTESIAN_POINT('Ctrl Pts',(-189.297626553883,2.1319572564113,135.23650922962));
#245013=CARTESIAN_POINT('Ctrl Pts',(-189.30539130683,2.25510240935448,135.177273805588));
#245014=CARTESIAN_POINT('Ctrl Pts',(-189.313156059777,2.37593862856379,
135.112824423354));
#245015=CARTESIAN_POINT('Ctrl Pts',(-189.320920812724,2.49399493257179,
135.043366673094));
#245016=CARTESIAN_POINT('Ctrl Pts',(-189.328677853609,2.61193398139434,
134.973977909251));
#245017=CARTESIAN_POINT('Ctrl Pts',(-189.336434894494,2.72709827484188,
134.899590873599));
#245018=CARTESIAN_POINT('Ctrl Pts',(-189.344191935379,2.8390392930429,134.820458095847));
#245019=CARTESIAN_POINT('Ctrl Pts',(-189.351943126619,2.95089589565147,
134.741384992739));
#245020=CARTESIAN_POINT('Ctrl Pts',(-189.359694317859,3.0595337432095,134.657573495689));
#245021=CARTESIAN_POINT('Ctrl Pts',(-189.3674455091,3.16453161094203,134.569320477358));
#245022=CARTESIAN_POINT('Ctrl Pts',(-189.375193405877,3.26948485177972,
134.481104968915));
#245023=CARTESIAN_POINT('Ctrl Pts',(-189.382941302654,3.37080089117263,
134.388451944842));
#245024=CARTESIAN_POINT('Ctrl Pts',(-189.390689199431,3.46809022258434,
134.291699613207));
#245025=CARTESIAN_POINT('Ctrl Pts',(-189.398435475515,3.5653592031655,134.194967520073));
#245026=CARTESIAN_POINT('Ctrl Pts',(-189.406181751599,3.65860287410479,
134.094138100479));
#245027=CARTESIAN_POINT('Ctrl Pts',(-189.413928027683,3.74746766208944,
133.989587325996));
#245028=CARTESIAN_POINT('Ctrl Pts',(-189.421674360949,3.83633310605366,
133.885035779743));
#245029=CARTESIAN_POINT('Ctrl Pts',(-189.429420694214,3.92081934936079,
133.776763121682));
#245030=CARTESIAN_POINT('Ctrl Pts',(-189.437167027479,4.00061255328625,
133.665179077551));
#245031=CARTESIAN_POINT('Ctrl Pts',(-189.444915095482,4.08042362634638,
133.553570044946));
#245032=CARTESIAN_POINT('Ctrl Pts',(-189.452663163485,4.15553934133821,
133.438648468607));
#245033=CARTESIAN_POINT('Ctrl Pts',(-189.460411231488,4.22568893687965,
133.320853429245));
#245034=CARTESIAN_POINT('Ctrl Pts',(-189.46816753423,4.29591308824612,133.202933195913));
#245035=CARTESIAN_POINT('Ctrl Pts',(-189.475923836972,4.36116037632517,
133.08213373541));
#245036=CARTESIAN_POINT('Ctrl Pts',(-189.483680139714,4.42120555602244,
132.958919619751));
#245037=CARTESIAN_POINT('Ctrl Pts',(-189.491440582228,4.4812827836402,132.835639741008));
#245038=CARTESIAN_POINT('Ctrl Pts',(-189.499201024743,4.53615221408563,
132.709942997256));
#245039=CARTESIAN_POINT('Ctrl Pts',(-189.506961467257,4.58563701835403,
132.582313428639));
#245040=CARTESIAN_POINT('Ctrl Pts',(-189.514734367522,4.63520126002316,
132.454478977708));
#245041=CARTESIAN_POINT('Ctrl Pts',(-189.522507267788,4.67936347626291,
132.324705871978));
#245042=CARTESIAN_POINT('Ctrl Pts',(-189.530280168053,4.7179966628129,132.193493639341));
#245043=CARTESIAN_POINT('Ctrl Pts',(-189.537770503815,4.7552254357191,132.06705130187));
#245044=CARTESIAN_POINT('Ctrl Pts',(-189.545260839577,4.78732011310547,
131.939272951445));
#245045=CARTESIAN_POINT('Ctrl Pts',(-189.552751175338,4.81421239738261,
131.810612104714));
#245046=CARTESIAN_POINT('Ctrl Pts',(-189.560525509457,4.84212431079291,
131.677073042868));
#245047=CARTESIAN_POINT('Ctrl Pts',(-189.568299843577,4.86451996267185,
131.542160232397));
#245048=CARTESIAN_POINT('Ctrl Pts',(-189.576074177696,4.88126712533379,
131.406369183648));
#245049=CARTESIAN_POINT('Ctrl Pts',(-189.583838930643,4.89799364861444,
131.27074548523));
#245050=CARTESIAN_POINT('Ctrl Pts',(-189.59160368359,4.90908548611105,131.134246086389));
#245051=CARTESIAN_POINT('Ctrl Pts',(-189.599368436537,4.91446102967388,
130.997378363685));
#245052=CARTESIAN_POINT('Ctrl Pts',(-189.607125477422,4.91983123417105,
130.860646579932));
#245053=CARTESIAN_POINT('Ctrl Pts',(-189.614882518307,4.91949642797885,
130.723547588459));
#245054=CARTESIAN_POINT('Ctrl Pts',(-189.622639559192,4.91342663554939,
130.586595240213));
#245055=CARTESIAN_POINT('Ctrl Pts',(-189.630390750432,4.90736142039758,
130.449746168797));
#245056=CARTESIAN_POINT('Ctrl Pts',(-189.638141941672,4.8955698444968,130.313043909499));
#245057=CARTESIAN_POINT('Ctrl Pts',(-189.645893132912,4.87807399294504,
130.177003317574));
#245058=CARTESIAN_POINT('Ctrl Pts',(-189.653641029689,4.86058557759692,
130.04102054653));
#245059=CARTESIAN_POINT('Ctrl Pts',(-189.661388926466,4.83739775844842,
129.905699270483));
#245060=CARTESIAN_POINT('Ctrl Pts',(-189.669136823243,4.80858454172782,
129.771550002034));
#245061=CARTESIAN_POINT('Ctrl Pts',(-189.676883099327,4.77977735211094,
129.637428794719));
#245062=CARTESIAN_POINT('Ctrl Pts',(-189.684629375411,4.74534718751536,
129.504479489374));
#245063=CARTESIAN_POINT('Ctrl Pts',(-189.692375651495,4.70541924846024,
129.373202779059));
#245064=CARTESIAN_POINT('Ctrl Pts',(-189.700121984761,4.66549101466631,
129.241925099689));
#245065=CARTESIAN_POINT('Ctrl Pts',(-189.707868318026,4.62006503919849,
129.112320414033));
#245066=CARTESIAN_POINT('Ctrl Pts',(-189.715614651291,4.56931639842622,
128.984874230265));
#245067=CARTESIAN_POINT('Ctrl Pts',(-189.723362719294,4.51855639284751,
128.857399505808));
#245068=CARTESIAN_POINT('Ctrl Pts',(-189.731110787297,4.46247149468235,
128.732084608271));
#245069=CARTESIAN_POINT('Ctrl Pts',(-189.7388588553,4.40128476182806,128.609394670723));
#245070=CARTESIAN_POINT('Ctrl Pts',(-189.746615158042,4.34003299898604,
128.48657433685));
#245071=CARTESIAN_POINT('Ctrl Pts',(-189.754371460784,4.2736687446074,128.366384886397));
#245072=CARTESIAN_POINT('Ctrl Pts',(-189.762127763526,4.20246110581043,
128.249266936964));
#245073=CARTESIAN_POINT('Ctrl Pts',(-189.76988820604,4.13121546135242,128.132086478155));
#245074=CARTESIAN_POINT('Ctrl Pts',(-189.777648648554,4.0551214983341,128.017981112027));
#245075=CARTESIAN_POINT('Ctrl Pts',(-189.785409091068,3.97449087304063,
127.907361245351));
#245076=CARTESIAN_POINT('Ctrl Pts',(-189.793181991334,3.89373081230961,
127.796563801844));
#245077=CARTESIAN_POINT('Ctrl Pts',(-189.800954891599,3.80841977969454,
127.689263345051));
#245078=CARTESIAN_POINT('Ctrl Pts',(-189.808727791865,3.71890939325291,
127.585836734281));
#245079=CARTESIAN_POINT('Ctrl Pts',(-189.816218127627,3.63265293481907,
127.486169941325));
#245080=CARTESIAN_POINT('Ctrl Pts',(-189.823708463389,3.54249734681371,
127.390100460701));
#245081=CARTESIAN_POINT('Ctrl Pts',(-189.831198799151,3.44878726912054,
127.29793088993));
#245082=CARTESIAN_POINT('Ctrl Pts',(-189.83897313327,3.3515241453514,127.20226668187));
#245083=CARTESIAN_POINT('Ctrl Pts',(-189.846747467389,3.25012357385693,
127.110500916178));
#245084=CARTESIAN_POINT('Ctrl Pts',(-189.854521801508,3.14493096923238,
127.023012675196));
#245085=CARTESIAN_POINT('Ctrl Pts',(-189.862286554456,3.03986800509226,
126.935632255653));
#245086=CARTESIAN_POINT('Ctrl Pts',(-189.870051307403,2.93102260408373,
126.852519119373));
#245087=CARTESIAN_POINT('Ctrl Pts',(-189.87781606035,2.81877752527758,126.774016175029));
#245088=CARTESIAN_POINT('Ctrl Pts',(-189.885573101235,2.70664392986547,
126.695591200915));
#245089=CARTESIAN_POINT('Ctrl Pts',(-189.89333014212,2.59111769456779,126.621767529126));
#245090=CARTESIAN_POINT('Ctrl Pts',(-189.901087183005,2.47261493422438,
126.552848127928));
#245091=CARTESIAN_POINT('Ctrl Pts',(-189.908838374245,2.35420153773453,
126.483980699386));
#245092=CARTESIAN_POINT('Ctrl Pts',(-189.916589565485,2.23281642057723,
126.420010375857));
#245093=CARTESIAN_POINT('Ctrl Pts',(-189.924340756725,2.10890468259733,
126.361196868364));
#245094=CARTESIAN_POINT('Ctrl Pts',(-189.932088653502,1.98504561041135,
126.302408358181));
#245095=CARTESIAN_POINT('Ctrl Pts',(-189.93983655028,1.8586624057305,126.248772472034));
#245096=CARTESIAN_POINT('Ctrl Pts',(-189.947584447057,1.73022457943941,
126.200502890919));
#245097=CARTESIAN_POINT('Ctrl Pts',(-189.955330723141,1.60181361957279,
126.15224340676));
#245098=CARTESIAN_POINT('Ctrl Pts',(-189.963076999225,1.47134925869841,
126.109348132341));
#245099=CARTESIAN_POINT('Ctrl Pts',(-189.970823275309,1.33932041800663,
126.071982369749));
#245100=CARTESIAN_POINT('Ctrl Pts',(-189.978569608574,1.20729060270813,
126.034616331331));
#245101=CARTESIAN_POINT('Ctrl Pts',(-189.98631594184,1.07369666073754,126.002779992655));
#245102=CARTESIAN_POINT('Ctrl Pts',(-189.994062275105,0.939041696927769,
125.976588486041));
#245103=CARTESIAN_POINT('Ctrl Pts',(-190.001810343108,0.804356578073038,
125.95039111402));
#245104=CARTESIAN_POINT('Ctrl Pts',(-190.009558411111,0.668610348265179,
125.929841164149));
#245105=CARTESIAN_POINT('Ctrl Pts',(-190.017306479114,0.532314905370259,
125.915002387285));
#245106=CARTESIAN_POINT('Ctrl Pts',(-190.025062781856,0.395874606056136,
125.900147839592));
#245107=CARTESIAN_POINT('Ctrl Pts',(-190.032819084598,0.258884316919199,
125.891016632574));
#245108=CARTESIAN_POINT('Ctrl Pts',(-190.040575387339,0.12186020099531,
125.887620523366));
#245109=CARTESIAN_POINT('Ctrl Pts',(-190.048335829854,-0.0152370488249634,
125.884222601552));
#245110=CARTESIAN_POINT('Ctrl Pts',(-190.056096272368,-0.152367770690179,
125.886565870162));
#245111=CARTESIAN_POINT('Ctrl Pts',(-190.063856714882,-0.28901821992613,
125.894609958821));
#245112=CARTESIAN_POINT('Ctrl Pts',(-190.071629615147,-0.42588803259445,
125.902666960564));
#245113=CARTESIAN_POINT('Ctrl Pts',(-190.079402515413,-0.562275642767436,
125.916443030582));
#245114=CARTESIAN_POINT('Ctrl Pts',(-190.087175415678,-0.697673929887046,
125.935846044305));
#245115=CARTESIAN_POINT('Ctrl Pts',(-190.09466575144,-0.82815014822142,
125.954543709606));
#245116=CARTESIAN_POINT('Ctrl Pts',(-190.102156087202,-0.957707420585213,
125.978466258228));
#245117=CARTESIAN_POINT('Ctrl Pts',(-190.109646422964,-1.0859048768382,
126.007487296229));
#245118=CARTESIAN_POINT('Ctrl Pts',(-190.117420757083,-1.21896297860964,
126.037608675706));
#245119=CARTESIAN_POINT('Ctrl Pts',(-190.125195091202,-1.35097760196638,
126.073318210457));
#245120=CARTESIAN_POINT('Ctrl Pts',(-190.132969425321,-1.48144310917082,
126.114530196667));
#245121=CARTESIAN_POINT('Ctrl Pts',(-190.140734178268,-1.61174782929803,
126.155691392787));
#245122=CARTESIAN_POINT('Ctrl Pts',(-190.148498931215,-1.74050686267825,
126.202341431007));
#245123=CARTESIAN_POINT('Ctrl Pts',(-190.156263684163,-1.86722481990743,
126.254343635793));
#245124=CARTESIAN_POINT('Ctrl Pts',(-190.164020725047,-1.9938169190744,
126.306294191256));
#245125=CARTESIAN_POINT('Ctrl Pts',(-190.171777765932,-2.11837161700793,
126.363586187039));
#245126=CARTESIAN_POINT('Ctrl Pts',(-190.179534806817,-2.24040909768993,
126.42603329569));
#245127=CARTESIAN_POINT('Ctrl Pts',(-190.187285998058,-2.36235454895925,
126.488433312491));
#245128=CARTESIAN_POINT('Ctrl Pts',(-190.195037189298,-2.48178621469771,
126.55598052693));
#245129=CARTESIAN_POINT('Ctrl Pts',(-190.202788380538,-2.59824500532673,
126.628440844056));
#245130=CARTESIAN_POINT('Ctrl Pts',(-190.210536277315,-2.71465429786326,
126.700870363613));
#245131=CARTESIAN_POINT('Ctrl Pts',(-190.218284174092,-2.82809289713704,
126.778208626477));
#245132=CARTESIAN_POINT('Ctrl Pts',(-190.226032070869,-2.93812724517321,
126.860176119641));
#245133=CARTESIAN_POINT('Ctrl Pts',(-190.233778346953,-3.04813857639583,
126.942126466972));
#245134=CARTESIAN_POINT('Ctrl Pts',(-190.241524623037,-3.15474675944337,
127.028703885119));
#245135=CARTESIAN_POINT('Ctrl Pts',(-190.249270899121,-3.25754844714305,
127.119586380653));
#245136=CARTESIAN_POINT('Ctrl Pts',(-190.257017232387,-3.36035089370159,
127.210469547061));
#245137=CARTESIAN_POINT('Ctrl Pts',(-190.264763565652,-3.45934649593055,
127.305657595318));
#245138=CARTESIAN_POINT('Ctrl Pts',(-190.272509898917,-3.55416644929697,
127.404789480909));
#245139=CARTESIAN_POINT('Ctrl Pts',(-190.28025796692,-3.64900763693438,
127.503943566399));
#245140=CARTESIAN_POINT('Ctrl Pts',(-190.288006034923,-3.73967104476384,
127.607042964203));
#245141=CARTESIAN_POINT('Ctrl Pts',(-190.295754102926,-3.82582634408186,
127.713691459046));
#245142=CARTESIAN_POINT('Ctrl Pts',(-190.303510405668,-3.91207321027691,
127.820453301177));
#245143=CARTESIAN_POINT('Ctrl Pts',(-190.31126670841,-3.99380215080234,
127.930771470759));
#245144=CARTESIAN_POINT('Ctrl Pts',(-190.319023011152,-4.07072427531871,
128.044218060228));
#245145=CARTESIAN_POINT('Ctrl Pts',(-190.326783453666,-4.14768745548943,
128.157725199558));
#245146=CARTESIAN_POINT('Ctrl Pts',(-190.33454389618,-4.21983850201565,
128.274363753527));
#245147=CARTESIAN_POINT('Ctrl Pts',(-190.342304338694,-4.28693368809188,
128.393679673019));
#245148=CARTESIAN_POINT('Ctrl Pts',(-190.35007723896,-4.35413658131705,
128.513187129016));
#245149=CARTESIAN_POINT('Ctrl Pts',(-190.357850139225,-4.41626721820383,
128.635380190496));
#245150=CARTESIAN_POINT('Ctrl Pts',(-190.36562303949,-4.47312899471228,
128.759782406989));
#245151=CARTESIAN_POINT('Ctrl Pts',(-190.373113375253,-4.52792370242032,
128.879662289568));
#245152=CARTESIAN_POINT('Ctrl Pts',(-190.380603711015,-4.57782585506955,
129.001593213935));
#245153=CARTESIAN_POINT('Ctrl Pts',(-190.388094046777,-4.62270349038433,
129.125135944543));
#245154=CARTESIAN_POINT('Ctrl Pts',(-190.397182635961,-4.67715690927988,
129.275039655247));
#245155=CARTESIAN_POINT('Ctrl Pts',(-190.406271225145,-4.72435719403422,
129.427710815754));
#245156=CARTESIAN_POINT('Ctrl Pts',(-190.415359814329,-4.76405452823405,
129.582490119308));
#245157=CARTESIAN_POINT('',(-188.389859436034,-4.91824789781227,130.808907942626));
#245158=CARTESIAN_POINT('Ctrl Pts',(-188.389859436034,-4.91824789781227,
130.808907942627));
#245159=CARTESIAN_POINT('Ctrl Pts',(-188.399867117337,-4.9180844751749,
130.985660875825));
#245160=CARTESIAN_POINT('Ctrl Pts',(-188.409874798639,-4.90838934841572,
131.161987856138));
#245161=CARTESIAN_POINT('Ctrl Pts',(-188.419882479942,-4.88932061848566,
131.33702087716));
#245162=CARTESIAN_POINT('Ctrl Pts',(-188.430125673914,-4.86980314050388,
131.516172983589));
#245163=CARTESIAN_POINT('Ctrl Pts',(-188.440368867886,-4.84046566695456,
131.693969810191));
#245164=CARTESIAN_POINT('Ctrl Pts',(-188.450612061858,-4.80152560262522,
131.86950612398));
#245165=CARTESIAN_POINT('Ctrl Pts',(-188.453257933321,-4.79146717697613,
131.914848087107));
#245166=CARTESIAN_POINT('Ctrl Pts',(-188.455903804784,-4.78076829602226,
131.960039341272));
#245167=CARTESIAN_POINT('Ctrl Pts',(-188.458549676247,-4.76943321745608,
132.005064513923));
#245168=CARTESIAN_POINT('Ctrl Pts',(-188.466324010366,-4.73612748463049,
132.137361468194));
#245169=CARTESIAN_POINT('Ctrl Pts',(-188.474098344485,-4.69726024638632,
132.268481144229));
#245170=CARTESIAN_POINT('Ctrl Pts',(-188.481872678604,-4.65292931576995,
132.397920106556));
#245171=CARTESIAN_POINT('Ctrl Pts',(-188.489637431551,-4.60865301906372,
132.527199546929));
#245172=CARTESIAN_POINT('Ctrl Pts',(-188.497402184498,-4.55892655312866,
132.654802028599));
#245173=CARTESIAN_POINT('Ctrl Pts',(-188.505166937445,-4.503898442119,132.780235584657));
#245174=CARTESIAN_POINT('Ctrl Pts',(-188.51292397833,-4.44892498580481,
132.90554455834));
#245175=CARTESIAN_POINT('Ctrl Pts',(-188.520681019215,-4.38866051938554,
133.028688537671));
#245176=CARTESIAN_POINT('Ctrl Pts',(-188.5284380601,-4.32330283091627,133.149192316152));
#245177=CARTESIAN_POINT('Ctrl Pts',(-188.53618925134,-4.25799442918837,
133.269605221796));
#245178=CARTESIAN_POINT('Ctrl Pts',(-188.54394044258,-4.18760063600923,
133.387381547266));
#245179=CARTESIAN_POINT('Ctrl Pts',(-188.551691633821,-4.11236649580212,
133.502067952824));
#245180=CARTESIAN_POINT('Ctrl Pts',(-188.559439530598,-4.03716433211143,
133.6167056136));
#245181=CARTESIAN_POINT('Ctrl Pts',(-188.567187427375,-3.95712612715828,
133.728255640296));
#245182=CARTESIAN_POINT('Ctrl Pts',(-188.574935324152,-3.87254171765271,
133.836291307331));
#245183=CARTESIAN_POINT('Ctrl Pts',(-188.582681600236,-3.78797500138217,
133.944304375634));
#245184=CARTESIAN_POINT('Ctrl Pts',(-188.59042787632,-3.69886421295048,
134.048804238843));
#245185=CARTESIAN_POINT('Ctrl Pts',(-188.598174152404,-3.60554093228053,
134.149395392893));
#245186=CARTESIAN_POINT('Ctrl Pts',(-188.605920485669,-3.51221696271946,
134.249987289485));
#245187=CARTESIAN_POINT('Ctrl Pts',(-188.613666818935,-3.41468070477701,
134.34667013273));
#245188=CARTESIAN_POINT('Ctrl Pts',(-188.6214131522,-3.31330194928639,134.439083888374));
#245189=CARTESIAN_POINT('Ctrl Pts',(-188.629161220203,-3.21190049072653,
134.531518339438));
#245190=CARTESIAN_POINT('Ctrl Pts',(-188.636909288206,-3.10665511120062,
134.619681537175));
#245191=CARTESIAN_POINT('Ctrl Pts',(-188.644657356209,-2.99796983886249,
134.703252756081));
#245192=CARTESIAN_POINT('Ctrl Pts',(-188.652413658951,-2.88916905452341,
134.786912795473));
#245193=CARTESIAN_POINT('Ctrl Pts',(-188.660169961693,-2.77692138462799,
134.865970868193));
#245194=CARTESIAN_POINT('Ctrl Pts',(-188.667926264434,-2.661661546083,134.940148435697));
#245195=CARTESIAN_POINT('Ctrl Pts',(-188.675686706949,-2.54634018989178,
135.014365594003));
#245196=CARTESIAN_POINT('Ctrl Pts',(-188.683447149463,-2.4280037987698,
135.083696859122));
#245197=CARTESIAN_POINT('Ctrl Pts',(-188.691207591977,-2.30711213985166,
135.147909470365));
#245198=CARTESIAN_POINT('Ctrl Pts',(-188.698980492242,-2.18602641491037,
135.212225161391));
#245199=CARTESIAN_POINT('Ctrl Pts',(-188.706753392507,-2.06237757804144,
135.271405609637));
#245200=CARTESIAN_POINT('Ctrl Pts',(-188.714526292773,-1.93664666046133,
135.325265701177));
#245201=CARTESIAN_POINT('Ctrl Pts',(-188.722016628535,-1.81548637842552,
135.377167842728));
#245202=CARTESIAN_POINT('Ctrl Pts',(-188.729506964298,-1.69239305308073,
135.424129618806));
#245203=CARTESIAN_POINT('Ctrl Pts',(-188.73699730006,-1.56780896021745,
135.466029645582));
#245204=CARTESIAN_POINT('Ctrl Pts',(-188.744771634179,-1.43850122361313,
135.509518324605));
#245205=CARTESIAN_POINT('Ctrl Pts',(-188.752545968298,-1.30717783500581,
135.547691603967));
#245206=CARTESIAN_POINT('Ctrl Pts',(-188.760320302418,-1.17431521925618,
135.580359657382));
#245207=CARTESIAN_POINT('Ctrl Pts',(-188.768085055365,-1.04161634480655,
135.612987450341));
#245208=CARTESIAN_POINT('Ctrl Pts',(-188.775849808312,-0.907382393612003,
135.64012342443));
#245209=CARTESIAN_POINT('Ctrl Pts',(-188.783614561259,-0.772107552298939,
135.661626617095));
#245210=CARTESIAN_POINT('Ctrl Pts',(-188.791371602144,-0.636967067865308,
135.683108452486));
#245211=CARTESIAN_POINT('Ctrl Pts',(-188.799128643029,-0.500788134293892,
135.698968578897));
#245212=CARTESIAN_POINT('Ctrl Pts',(-188.806885683914,-0.36407746554492,
135.709116540299));
#245213=CARTESIAN_POINT('Ctrl Pts',(-188.814636875154,-0.227469891374892,
135.719256849044));
#245214=CARTESIAN_POINT('Ctrl Pts',(-188.822388066394,-0.0903317684798211,
135.72369353795));
#245215=CARTESIAN_POINT('Ctrl Pts',(-188.830139257634,0.0468230430825336,
135.722387728628));
#245216=CARTESIAN_POINT('Ctrl Pts',(-188.837887154411,0.183919560191437,
135.721082474309));
#245217=CARTESIAN_POINT('Ctrl Pts',(-188.845635051188,0.321032361730929,
135.714039579871));
#245218=CARTESIAN_POINT('Ctrl Pts',(-188.853382947965,0.457645767564134,
135.70127223755));
#245219=CARTESIAN_POINT('Ctrl Pts',(-188.861129224049,0.594230596817883,
135.688507565881));
#245220=CARTESIAN_POINT('Ctrl Pts',(-188.868875500133,0.730315849125278,
135.670020864439));
#245221=CARTESIAN_POINT('Ctrl Pts',(-188.876621776217,0.865389548668166,
135.645877321199));
#245222=CARTESIAN_POINT('Ctrl Pts',(-188.884368109483,1.0004642452946,135.621733599736));
#245223=CARTESIAN_POINT('Ctrl Pts',(-188.892114442748,1.1345269893911,135.591933021942));
#245224=CARTESIAN_POINT('Ctrl Pts',(-188.899860776013,1.26707499296545,
135.556592096009));
#245225=CARTESIAN_POINT('Ctrl Pts',(-188.907608844016,1.39965267974599,
135.52124325572));
#245226=CARTESIAN_POINT('Ctrl Pts',(-188.915356912019,1.53071457330889,
135.480351699103));
#245227=CARTESIAN_POINT('Ctrl Pts',(-188.923104980022,1.65977245111908,
135.434083986516));
#245228=CARTESIAN_POINT('Ctrl Pts',(-188.930861282764,1.7889674931778,135.387767100054));
#245229=CARTESIAN_POINT('Ctrl Pts',(-188.938617585506,1.91615389617927,
135.336062775758));
#245230=CARTESIAN_POINT('Ctrl Pts',(-188.946373888248,2.04086234265069,
135.279186196385));
#245231=CARTESIAN_POINT('Ctrl Pts',(-188.954134330762,2.16563734977488,
135.222279260269));
#245232=CARTESIAN_POINT('Ctrl Pts',(-188.961894773276,2.2879314166124,135.160194745264));
#245233=CARTESIAN_POINT('Ctrl Pts',(-188.96965521579,2.40730019963481,135.093193653642));
#245234=CARTESIAN_POINT('Ctrl Pts',(-188.977428116055,2.5268606040248,135.02608500592));
#245235=CARTESIAN_POINT('Ctrl Pts',(-188.985201016321,2.64348600783031,
134.954044215384));
#245236=CARTESIAN_POINT('Ctrl Pts',(-188.992973916586,2.75676066034094,
134.877375928622));
#245237=CARTESIAN_POINT('Ctrl Pts',(-189.000464252348,2.86591749391118,
134.803494727199));
#245238=CARTESIAN_POINT('Ctrl Pts',(-189.00795458811,2.97196271521771,134.725316813482));
#245239=CARTESIAN_POINT('Ctrl Pts',(-189.015444923872,3.07455513973725,
134.643148675693));
#245240=CARTESIAN_POINT('Ctrl Pts',(-189.023219257991,3.18103738721459,
134.557865107985));
#245241=CARTESIAN_POINT('Ctrl Pts',(-189.03099359211,3.2841371475586,134.468012611807));
#245242=CARTESIAN_POINT('Ctrl Pts',(-189.038767926229,3.38343719526661,
134.373889411145));
#245243=CARTESIAN_POINT('Ctrl Pts',(-189.046532679176,3.48261486454052,
134.279882208915));
#245244=CARTESIAN_POINT('Ctrl Pts',(-189.054297432124,3.57800185753944,
134.1816150409));
#245245=CARTESIAN_POINT('Ctrl Pts',(-189.062062185071,3.66921245853213,
134.079427486601));
#245246=CARTESIAN_POINT('Ctrl Pts',(-189.069819225956,3.76033246787007,
133.977341426422));
#245247=CARTESIAN_POINT('Ctrl Pts',(-189.077576266841,3.84728408135189,
133.87134301855));
#245248=CARTESIAN_POINT('Ctrl Pts',(-189.085333307726,3.92971730448732,
133.7618096821));
#245249=CARTESIAN_POINT('Ctrl Pts',(-189.093084498966,4.01208836408783,
133.652358945591));
#245250=CARTESIAN_POINT('Ctrl Pts',(-189.100835690206,4.0899475813276,133.539378897572));
#245251=CARTESIAN_POINT('Ctrl Pts',(-189.108586881446,4.16298449280398,
133.423280848343));
#245252=CARTESIAN_POINT('Ctrl Pts',(-189.116334778223,4.23599036164477,
133.307232143882));
#245253=CARTESIAN_POINT('Ctrl Pts',(-189.124082675,4.30417779348807,133.188068404235));
#245254=CARTESIAN_POINT('Ctrl Pts',(-189.131830571777,4.36727914962361,
133.06623061643));
#245255=CARTESIAN_POINT('Ctrl Pts',(-189.139576847861,4.43036730631575,
132.944418314464));
#245256=CARTESIAN_POINT('Ctrl Pts',(-189.147323123945,4.48837132376201,
132.819933423872));
#245257=CARTESIAN_POINT('Ctrl Pts',(-189.15506940003,4.54106931101448,132.6932419201));
#245258=CARTESIAN_POINT('Ctrl Pts',(-189.162815733295,4.59376768727144,
132.56654948112));
#245259=CARTESIAN_POINT('Ctrl Pts',(-189.17056206656,4.64115980502555,132.437650757441));
#245260=CARTESIAN_POINT('Ctrl Pts',(-189.178308399826,4.68307191672785,
132.307031734363));
#245261=CARTESIAN_POINT('Ctrl Pts',(-189.186056467829,4.72499341435691,
132.17638346006));
#245262=CARTESIAN_POINT('Ctrl Pts',(-189.193804535832,4.76143234450105,
132.044014491957));
#245263=CARTESIAN_POINT('Ctrl Pts',(-189.201552603835,4.7922649429027,131.910425615442));
#245264=CARTESIAN_POINT('Ctrl Pts',(-189.209308906576,4.82313031055689,
131.776694759079));
#245265=CARTESIAN_POINT('Ctrl Pts',(-189.217065209318,4.84837735570641,
131.641741785897));
#245266=CARTESIAN_POINT('Ctrl Pts',(-189.22482151206,4.86793344014249,131.506077857516));
#245267=CARTESIAN_POINT('Ctrl Pts',(-189.232581954574,4.8874999622497,131.37034152121));
#245268=CARTESIAN_POINT('Ctrl Pts',(-189.240342397089,4.90136943177558,
131.233893862373));
#245269=CARTESIAN_POINT('Ctrl Pts',(-189.248102839603,4.90952125879313,
131.097249797903));
#245270=CARTESIAN_POINT('Ctrl Pts',(-189.255875739868,4.91768617184709,
130.960386380249));
#245271=CARTESIAN_POINT('Ctrl Pts',(-189.263648640134,4.92011509395886,
130.823326318046));
#245272=CARTESIAN_POINT('Ctrl Pts',(-189.271421540399,4.91683960951637,
130.686584063062));
#245273=CARTESIAN_POINT('Ctrl Pts',(-189.278911876161,4.91368319718378,
130.554812733478));
#245274=CARTESIAN_POINT('Ctrl Pts',(-189.286402211923,4.90522993667453,
130.423336813468));
#245275=CARTESIAN_POINT('Ctrl Pts',(-189.293892547685,4.8915532666416,130.292609015607));
#245276=CARTESIAN_POINT('Ctrl Pts',(-189.301666881805,4.87735804150758,
130.156924633557));
#245277=CARTESIAN_POINT('Ctrl Pts',(-189.309441215924,4.85749053053571,
130.021616416288));
#245278=CARTESIAN_POINT('Ctrl Pts',(-189.317215550043,4.83197611743572,
129.887196584783));
#245279=CARTESIAN_POINT('Ctrl Pts',(-189.32498030299,4.80649314856966,129.752942413707));
#245280=CARTESIAN_POINT('Ctrl Pts',(-189.332745055937,4.77537719672058,
129.619574830376));
#245281=CARTESIAN_POINT('Ctrl Pts',(-189.340509808884,4.73870547096616,
129.487601899374));
#245282=CARTESIAN_POINT('Ctrl Pts',(-189.348266849769,4.70207016808673,
129.355760045747));
#245283=CARTESIAN_POINT('Ctrl Pts',(-189.356023890654,4.6598901765116,129.225310462118));
#245284=CARTESIAN_POINT('Ctrl Pts',(-189.363780931539,4.61229384905882,
129.096751613012));
#245285=CARTESIAN_POINT('Ctrl Pts',(-189.371532122779,4.56473341436676,
128.968289711134));
#245286=CARTESIAN_POINT('Ctrl Pts',(-189.379283314019,4.5117649089419,128.841716070937));
#245287=CARTESIAN_POINT('Ctrl Pts',(-189.387034505259,4.45356656673678,
128.717514217338));
#245288=CARTESIAN_POINT('Ctrl Pts',(-189.394782402037,4.39539296037968,
128.59336515284));
#245289=CARTESIAN_POINT('Ctrl Pts',(-189.402530298814,4.33199410380397,
128.471586223247));
#245290=CARTESIAN_POINT('Ctrl Pts',(-189.410278195591,4.26359634662585,
128.352640964845));
#245291=CARTESIAN_POINT('Ctrl Pts',(-189.418024471675,4.19521289678404,
128.233720587227));
#245292=CARTESIAN_POINT('Ctrl Pts',(-189.425770747759,4.12183282098978,
128.117633040512));
#245293=CARTESIAN_POINT('Ctrl Pts',(-189.433517023843,4.04372822010655,
128.004816878952));
#245294=CARTESIAN_POINT('Ctrl Pts',(-189.441263357108,3.9656230426728,127.891999884608));
#245295=CARTESIAN_POINT('Ctrl Pts',(-189.449009690374,3.88279349310222,
127.782454645051));
#245296=CARTESIAN_POINT('Ctrl Pts',(-189.456756023639,3.7955545297986,127.676590025942));
#245297=CARTESIAN_POINT('Ctrl Pts',(-189.464504091642,3.70829602993413,
127.570701699186));
#245298=CARTESIAN_POINT('Ctrl Pts',(-189.472252159645,3.61662639999776,
127.4684959347));
#245299=CARTESIAN_POINT('Ctrl Pts',(-189.480000227648,3.5209000673159,127.370347545594));
#245300=CARTESIAN_POINT('Ctrl Pts',(-189.48775653039,3.42507199554838,127.272094843212));
#245301=CARTESIAN_POINT('Ctrl Pts',(-189.495512833132,3.32517888174022,
127.17790841068));
#245302=CARTESIAN_POINT('Ctrl Pts',(-189.503269135873,3.22161151791196,
127.08812565592));
#245303=CARTESIAN_POINT('Ctrl Pts',(-189.511029578388,3.11798887706327,
126.998294981402));
#245304=CARTESIAN_POINT('Ctrl Pts',(-189.518790020902,3.01068838434436,
126.912872911365));
#245305=CARTESIAN_POINT('Ctrl Pts',(-189.526550463416,2.90013212456667,
126.832155093861));
#245306=CARTESIAN_POINT('Ctrl Pts',(-189.534323363681,2.78939839006606,
126.751307700949));
#245307=CARTESIAN_POINT('Ctrl Pts',(-189.542096263947,2.67539876972268,
126.675179868487));
#245308=CARTESIAN_POINT('Ctrl Pts',(-189.549869164212,2.55858315851329,
126.604023097381));
#245309=CARTESIAN_POINT('Ctrl Pts',(-189.557359499974,2.44601408901245,
126.535453054138));
#245310=CARTESIAN_POINT('Ctrl Pts',(-189.564849835736,2.33083048013107,
126.471499075371));
#245311=CARTESIAN_POINT('Ctrl Pts',(-189.572340171498,2.21345290716398,
126.412344077266));
#245312=CARTESIAN_POINT('Ctrl Pts',(-189.580114505617,2.0916249278412,126.350946199428));
#245313=CARTESIAN_POINT('Ctrl Pts',(-189.587888839736,1.96704741755451,
126.294523902565));
#245314=CARTESIAN_POINT('Ctrl Pts',(-189.595663173855,1.84016504283681,
126.243332698596));
#245315=CARTESIAN_POINT('Ctrl Pts',(-189.603427926802,1.7134390393065,126.192204583211));
#245316=CARTESIAN_POINT('Ctrl Pts',(-189.61119267975,1.58441418226004,126.146294878277));
#245317=CARTESIAN_POINT('Ctrl Pts',(-189.618957432697,1.45355965421348,
126.105813246927));
#245318=CARTESIAN_POINT('Ctrl Pts',(-189.626714473582,1.3228350927289,126.065371822503));
#245319=CARTESIAN_POINT('Ctrl Pts',(-189.634471514467,1.19028484774728,
126.030347857655));
#245320=CARTESIAN_POINT('Ctrl Pts',(-189.642228555352,1.0563976694256,126.000902797773));
#245321=CARTESIAN_POINT('Ctrl Pts',(-189.649979746592,0.922611456466401,
125.971479942639));
#245322=CARTESIAN_POINT('Ctrl Pts',(-189.657730937832,0.787490697206884,
125.94762770214));
#245323=CARTESIAN_POINT('Ctrl Pts',(-189.665482129072,0.651538534659585,
125.92945748003));
#245324=CARTESIAN_POINT('Ctrl Pts',(-189.673230025849,0.515644155408197,
125.91129498075));
#245325=CARTESIAN_POINT('Ctrl Pts',(-189.680977922626,0.378919462400322,
125.898809748275));
#245326=CARTESIAN_POINT('Ctrl Pts',(-189.688725819403,0.241876789339127,
125.892061900949));
#245327=CARTESIAN_POINT('Ctrl Pts',(-189.696472095488,0.104862782650838,
125.885315465126));
#245328=CARTESIAN_POINT('Ctrl Pts',(-189.704218371572,-0.0324686815449168,
125.884304046529));
#245329=CARTESIAN_POINT('Ctrl Pts',(-189.711964647656,-0.169601557973934,
125.889035768278));
#245330=CARTESIAN_POINT('Ctrl Pts',(-189.719710980921,-0.30673544668688,
125.893767524955));
#245331=CARTESIAN_POINT('Ctrl Pts',(-189.727457314187,-0.443670353975256,
125.904242493092));
#245332=CARTESIAN_POINT('Ctrl Pts',(-189.735203647452,-0.57989204686906,
125.92041669114));
#245333=CARTESIAN_POINT('Ctrl Pts',(-189.742951715455,-0.716144245666308,
125.936594511287));
#245334=CARTESIAN_POINT('Ctrl Pts',(-189.750699783458,-0.851682524082018,
125.958474054952));
#245335=CARTESIAN_POINT('Ctrl Pts',(-189.758447851461,-0.985999964604032,
125.985959728028));
#245336=CARTESIAN_POINT('Ctrl Pts',(-189.766204154203,-1.12046015930041,
126.013474613205));
#245337=CARTESIAN_POINT('Ctrl Pts',(-189.773960456944,-1.25369654052637,
126.046607451556));
#245338=CARTESIAN_POINT('Ctrl Pts',(-189.781716759686,-1.38521400480768,
126.085211835912));
#245339=CARTESIAN_POINT('Ctrl Pts',(-189.7894772022,-1.51680166391959,126.12383682459));
#245340=CARTESIAN_POINT('Ctrl Pts',(-189.797237644715,-1.64666820799493,
126.167939052618));
#245341=CARTESIAN_POINT('Ctrl Pts',(-189.804998087229,-1.77433675280554,
126.217323213081));
#245342=CARTESIAN_POINT('Ctrl Pts',(-189.812770987494,-1.90221024249816,
126.266786649383));
#245343=CARTESIAN_POINT('Ctrl Pts',(-189.82054388776,-2.02787832339203,
126.321548805643));
#245344=CARTESIAN_POINT('Ctrl Pts',(-189.828316788025,-2.1508862214266,
126.38136711486));
#245345=CARTESIAN_POINT('Ctrl Pts',(-189.835807123787,-2.26942247252908,
126.439010877864));
#245346=CARTESIAN_POINT('Ctrl Pts',(-189.843297459549,-2.38548832025277,
126.501349422499));
#245347=CARTESIAN_POINT('Ctrl Pts',(-189.850787795311,-2.49870254081068,
126.568127777524));
#245348=CARTESIAN_POINT('Ctrl Pts',(-189.858563333984,-2.61622751943143,
126.637448793101));
#245349=CARTESIAN_POINT('Ctrl Pts',(-189.866338872658,-2.73105175223908,
126.711774041575));
#245350=CARTESIAN_POINT('Ctrl Pts',(-189.874114411331,-2.84271970669593,
126.790867409441));
#245351=CARTESIAN_POINT('Ctrl Pts',(-189.882266520974,-2.95979576362285,
126.873791285713));
#245352=CARTESIAN_POINT('Ctrl Pts',(-189.890418630616,-3.07340178179484,
126.961956537243));
#245353=CARTESIAN_POINT('Ctrl Pts',(-189.898570740259,-3.18304092391845,
127.055036206534));
#245354=CARTESIAN_POINT('Ctrl Pts',(-189.906326693971,-3.28735209593799,
127.14359262176));
#245355=CARTESIAN_POINT('Ctrl Pts',(-189.914082647682,-3.38807246231964,
127.236596825632));
#245356=CARTESIAN_POINT('Ctrl Pts',(-189.921838601394,-3.48480374559348,
127.333722935929));
#245357=CARTESIAN_POINT('Ctrl Pts',(-189.929589286311,-3.58146931712576,
127.43078306627));
#245358=CARTESIAN_POINT('Ctrl Pts',(-189.937339971229,-3.67415092233515,
127.531959256202));
#245359=CARTESIAN_POINT('Ctrl Pts',(-189.945090656146,-3.7624847314623,
127.636886591151));
#245360=CARTESIAN_POINT('Ctrl Pts',(-189.952837754435,-3.8507776641283,
127.741765370987));
#245361=CARTESIAN_POINT('Ctrl Pts',(-189.960584852723,-3.93472655359425,
127.850391542837));
#245362=CARTESIAN_POINT('Ctrl Pts',(-189.968331951012,-4.01400597908118,
127.962365004902));
#245363=CARTESIAN_POINT('Ctrl Pts',(-189.976077142051,-4.09326588685833,
128.07431090035));
#245364=CARTESIAN_POINT('Ctrl Pts',(-189.983822333091,-4.1678583942436,
128.189602126264));
#245365=CARTESIAN_POINT('Ctrl Pts',(-189.99156752413,-4.23750000942929,
128.307807647452));
#245366=CARTESIAN_POINT('Ctrl Pts',(-189.999314507378,-4.30715773942337,
128.426040520954));
#245367=CARTESIAN_POINT('Ctrl Pts',(-190.007061490626,-4.37186208637682,
128.54718870223));
#245368=CARTESIAN_POINT('Ctrl Pts',(-190.014808473873,-4.43137434301563,
128.67079447269));
#245369=CARTESIAN_POINT('Ctrl Pts',(-190.022556509817,-4.49089468645619,
128.794417039275));
#245370=CARTESIAN_POINT('Ctrl Pts',(-190.030304545761,-4.54522137225773,
128.920497504471));
#245371=CARTESIAN_POINT('Ctrl Pts',(-190.038052581704,-4.59416325289056,
129.04855679359));
#245372=CARTESIAN_POINT('Ctrl Pts',(-190.045805933935,-4.64313871481742,
129.176703950126));
#245373=CARTESIAN_POINT('Ctrl Pts',(-190.053559286166,-4.68672186348919,
129.30683227332));
#245374=CARTESIAN_POINT('Ctrl Pts',(-190.061312638396,-4.72477092847605,
129.438446002399));
#245375=CARTESIAN_POINT('Ctrl Pts',(-190.064130106518,-4.73859746756062,
129.486272732696));
#245376=CARTESIAN_POINT('Ctrl Pts',(-190.066947574639,-4.75169371319282,
129.534295489064));
#245377=CARTESIAN_POINT('Ctrl Pts',(-190.06976504276,-4.76405452823418,
129.582490119309));
#245378=CARTESIAN_POINT('Ctrl Pts',(-188.319844903182,-4.76405452823404,
129.582490119308));
#245379=CARTESIAN_POINT('Ctrl Pts',(-188.327501512409,-4.79776899317125,
129.71394230641));
#245380=CARTESIAN_POINT('Ctrl Pts',(-188.335158121637,-4.82603476089132,
129.846775959306));
#245381=CARTESIAN_POINT('Ctrl Pts',(-188.342814730864,-4.84875524607537,
129.980494350411));
#245382=CARTESIAN_POINT('Ctrl Pts',(-188.350655515053,-4.87202225836387,
130.117429254037));
#245383=CARTESIAN_POINT('Ctrl Pts',(-188.358496299241,-4.88947373540814,
130.255291565461));
#245384=CARTESIAN_POINT('Ctrl Pts',(-188.36633708343,-4.90106215269356,
130.393540902929));
#245385=CARTESIAN_POINT('Ctrl Pts',(-188.374177867618,-4.91265056997894,
130.531790240396));
#245386=CARTESIAN_POINT('Ctrl Pts',(-188.382018651807,-4.91837593560674,
130.670426153596));
#245387=CARTESIAN_POINT('Ctrl Pts',(-188.389859435995,-4.91824789781291,
130.808907941932));
#245388=CARTESIAN_POINT('Origin',(213.235140564004,0.,130.804360617566));
#245389=CARTESIAN_POINT('',(-186.570144995258,-4.76405452823391,129.582490119308));
#245390=CARTESIAN_POINT('',(-186.915092859931,-4.76405452823404,129.582490119308));
#245391=CARTESIAN_POINT('',(213.235140564004,-4.76405452823405,129.582490119308));
#245392=CARTESIAN_POINT('',(-186.985140563973,-4.91824792938353,130.808873666935));
#245393=CARTESIAN_POINT('Ctrl Pts',(-186.915092859931,-4.76405452823404,
129.582490119308));
#245394=CARTESIAN_POINT('Ctrl Pts',(-186.922737472684,-4.79771251131355,
129.713722084504));
#245395=CARTESIAN_POINT('Ctrl Pts',(-186.930382085436,-4.82593597496495,
129.846315094707));
#245396=CARTESIAN_POINT('Ctrl Pts',(-186.938026698189,-4.84863265225042,
129.979773165545));
#245397=CARTESIAN_POINT('Ctrl Pts',(-186.945879009153,-4.87194598068921,
130.116857188863));
#245398=CARTESIAN_POINT('Ctrl Pts',(-186.953731320117,-4.88942783458341,
130.2548535049));
#245399=CARTESIAN_POINT('Ctrl Pts',(-186.961583631081,-4.90103510324496,
130.393218331659));
#245400=CARTESIAN_POINT('Ctrl Pts',(-186.969435942045,-4.91264237190651,
130.531583158419));
#245401=CARTESIAN_POINT('Ctrl Pts',(-186.977288253009,-4.91837507169744,
130.670316037513));
#245402=CARTESIAN_POINT('Ctrl Pts',(-186.985140563973,-4.91824792938353,
130.808873666936));
#245403=CARTESIAN_POINT('Ctrl Pts',(-186.985140564012,-4.9182479293829,
130.808873667626));
#245404=CARTESIAN_POINT('Ctrl Pts',(-186.995772027482,-4.91807578782115,
130.996470718023));
#245405=CARTESIAN_POINT('Ctrl Pts',(-187.006403490951,-4.90716688700063,
131.183595083917));
#245406=CARTESIAN_POINT('Ctrl Pts',(-187.017034954421,-4.88570371797789,
131.369234269489));
#245407=CARTESIAN_POINT('Ctrl Pts',(-187.026930823288,-4.86572559297847,
131.542029016165));
#245408=CARTESIAN_POINT('Ctrl Pts',(-187.036826692156,-4.83660372490796,
131.71353778882));
#245409=CARTESIAN_POINT('Ctrl Pts',(-187.046722561023,-4.79852032900577,
131.882964212321));
#245410=CARTESIAN_POINT('Ctrl Pts',(-187.054496895142,-4.76860147618899,
132.016067999625));
#245411=CARTESIAN_POINT('Ctrl Pts',(-187.062271229261,-4.73309288657269,
132.148136813944));
#245412=CARTESIAN_POINT('Ctrl Pts',(-187.07004556338,-4.69207949437852,
132.278664887699));
#245413=CARTESIAN_POINT('Ctrl Pts',(-187.077810316327,-4.65111664752476,
132.409032097269));
#245414=CARTESIAN_POINT('Ctrl Pts',(-187.085575069274,-4.60466261265512,
132.537861974965));
#245415=CARTESIAN_POINT('Ctrl Pts',(-187.093339822221,-4.55285331124662,
132.66465892396));
#245416=CARTESIAN_POINT('Ctrl Pts',(-187.101096863106,-4.50109546756681,
132.791329936437));
#245417=CARTESIAN_POINT('Ctrl Pts',(-187.108853903991,-4.44399308917469,
132.915971678803));
#245418=CARTESIAN_POINT('Ctrl Pts',(-187.116610944876,-4.38173177310754,
133.038104052036));
#245419=CARTESIAN_POINT('Ctrl Pts',(-187.124362136116,-4.31951740878307,
133.160144324298));
#245420=CARTESIAN_POINT('Ctrl Pts',(-187.132113327356,-4.25215202722686,
133.279678647097));
#245421=CARTESIAN_POINT('Ctrl Pts',(-187.139864518596,-4.17986902446443,
133.396247575136));
#245422=CARTESIAN_POINT('Ctrl Pts',(-187.147612415373,-4.1076167439063,
133.512766958271));
#245423=CARTESIAN_POINT('Ctrl Pts',(-187.15536031215,-4.03045120483651,
133.626323121855));
#245424=CARTESIAN_POINT('Ctrl Pts',(-187.163108208927,-3.9486512601369,
133.736482083044));
#245425=CARTESIAN_POINT('Ctrl Pts',(-187.170854485011,-3.86686842622231,
133.846618001354));
#245426=CARTESIAN_POINT('Ctrl Pts',(-187.178600761095,-3.78045334783767,
133.953357817043));
#245427=CARTESIAN_POINT('Ctrl Pts',(-187.186347037179,-3.68972740421345,
134.056297693387));
#245428=CARTESIAN_POINT('Ctrl Pts',(-187.194093370445,-3.59900079087104,
134.159238329609));
#245429=CARTESIAN_POINT('Ctrl Pts',(-187.20183970371,-3.50396350729632,
134.258378677208));
#245430=CARTESIAN_POINT('Ctrl Pts',(-187.209586036975,-3.40497603632671,
134.353349382629));
#245431=CARTESIAN_POINT('Ctrl Pts',(-187.217334104978,-3.30596639779917,
134.44834135608));
#245432=CARTESIAN_POINT('Ctrl Pts',(-187.225082172981,-3.20300509365603,
134.539161558656));
#245433=CARTESIAN_POINT('Ctrl Pts',(-187.232830240984,-3.09648783601041,
134.625479059062));
#245434=CARTESIAN_POINT('Ctrl Pts',(-187.240586543725,-2.98985737055593,
134.711888298734));
#245435=CARTESIAN_POINT('Ctrl Pts',(-187.248342846467,-2.8796637062563,
134.793785030094));
#245436=CARTESIAN_POINT('Ctrl Pts',(-187.256099149209,-2.76633431053606,
134.870879711933));
#245437=CARTESIAN_POINT('Ctrl Pts',(-187.263859591723,-2.65294442750473,
134.948015541525));
#245438=CARTESIAN_POINT('Ctrl Pts',(-187.271620034237,-2.53641581021152,
135.020344008526));
#245439=CARTESIAN_POINT('Ctrl Pts',(-187.279380476751,-2.41720213633815,
135.087620695425));
#245440=CARTESIAN_POINT('Ctrl Pts',(-187.287153377017,-2.2977970900922,
135.155005380835));
#245441=CARTESIAN_POINT('Ctrl Pts',(-187.294926277282,-2.1756987223634,
135.217321902815));
#245442=CARTESIAN_POINT('Ctrl Pts',(-187.302699177547,-2.05138318386969,
135.274372932475));
#245443=CARTESIAN_POINT('Ctrl Pts',(-187.31018951331,-1.93158682832274,
135.329350013508));
#245444=CARTESIAN_POINT('Ctrl Pts',(-187.317679849073,-1.80973198772532,
135.379437666485));
#245445=CARTESIAN_POINT('Ctrl Pts',(-187.325170184835,-1.68625769629345,
135.424503260839));
#245446=CARTESIAN_POINT('Ctrl Pts',(-187.332944518954,-1.5581018395823,
135.471277530897));
#245447=CARTESIAN_POINT('Ctrl Pts',(-187.340718853073,-1.42779534567859,
135.512789568897));
#245448=CARTESIAN_POINT('Ctrl Pts',(-187.348493187192,-1.29580964019177,
135.548837452675));
#245449=CARTESIAN_POINT('Ctrl Pts',(-187.356257940139,-1.16398659529106,
135.584840910658));
#245450=CARTESIAN_POINT('Ctrl Pts',(-187.364022693087,-1.03048882998293,
135.615393511214));
#245451=CARTESIAN_POINT('Ctrl Pts',(-187.371787446034,-0.895806772792648,
135.640341726743));
#245452=CARTESIAN_POINT('Ctrl Pts',(-187.379544486919,-0.761258483720252,
135.665265163353));
#245453=CARTESIAN_POINT('Ctrl Pts',(-187.387301527804,-0.625528625504841,
135.68459522148));
#245454=CARTESIAN_POINT('Ctrl Pts',(-187.395058568689,-0.48912143878214,
135.698228543923));
#245455=CARTESIAN_POINT('Ctrl Pts',(-187.402809759929,-0.352817117779854,
135.711851585371));
#245456=CARTESIAN_POINT('Ctrl Pts',(-187.410560951169,-0.215836872397206,
135.719786403242));
#245457=CARTESIAN_POINT('Ctrl Pts',(-187.418312142409,-0.0786934032297544,
135.721981018816));
#245458=CARTESIAN_POINT('Ctrl Pts',(-187.426060039186,0.0583917763046921,
135.72417470162));
#245459=CARTESIAN_POINT('Ctrl Pts',(-187.433807935963,0.195639651546684,
135.720633028339));
#245460=CARTESIAN_POINT('Ctrl Pts',(-187.44155583274,0.33253437364453,135.711356027473));
#245461=CARTESIAN_POINT('Ctrl Pts',(-187.449302108824,0.469400460317623,
135.702080967155));
#245462=CARTESIAN_POINT('Ctrl Pts',(-187.457048384909,0.605913150958659,
135.687072991952));
#245463=CARTESIAN_POINT('Ctrl Pts',(-187.464794660993,0.741558972969566,
135.666384203698));
#245464=CARTESIAN_POINT('Ctrl Pts',(-187.472540994258,0.877205796287302,
135.645695262725));
#245465=CARTESIAN_POINT('Ctrl Pts',(-187.480287327523,1.01198535171049,
135.619325483972));
#245466=CARTESIAN_POINT('Ctrl Pts',(-187.488033660789,1.14539204185446,
135.587378507242));
#245467=CARTESIAN_POINT('Ctrl Pts',(-187.495781728792,1.27882860750151,
135.555424376208));
#245468=CARTESIAN_POINT('Ctrl Pts',(-187.503529796795,1.41089131594959,
135.517890652914));
#245469=CARTESIAN_POINT('Ctrl Pts',(-187.511277864798,1.54108785326631,
135.474931384722));
#245470=CARTESIAN_POINT('Ctrl Pts',(-187.51903416754,1.67142276501208,135.431926458909));
#245471=CARTESIAN_POINT('Ctrl Pts',(-187.526790470281,1.79988717172503,
135.383484592025));
#245472=CARTESIAN_POINT('Ctrl Pts',(-187.534546773023,1.92600641760273,
135.329808920425));
#245473=CARTESIAN_POINT('Ctrl Pts',(-187.542307215538,2.05219297711968,
135.276104600504));
#245474=CARTESIAN_POINT('Ctrl Pts',(-187.550067658052,2.17603152887269,
135.217161077647));
#245475=CARTESIAN_POINT('Ctrl Pts',(-187.557828100566,2.29707121362073,
135.153227930103));
#245476=CARTESIAN_POINT('Ctrl Pts',(-187.565601000831,2.41830520201613,
135.089192151395));
#245477=CARTESIAN_POINT('Ctrl Pts',(-187.573373901097,2.53673100702913,
135.020150938914));
#245478=CARTESIAN_POINT('Ctrl Pts',(-187.581146801362,2.65192523918329,
134.94639823066));
#245479=CARTESIAN_POINT('Ctrl Pts',(-187.588637137124,2.7629318708422,134.875326619122));
#245480=CARTESIAN_POINT('Ctrl Pts',(-187.596127472886,2.87093754965219,
134.799880290516));
#245481=CARTESIAN_POINT('Ctrl Pts',(-187.603617808648,2.9755933810453,134.720356926704));
#245482=CARTESIAN_POINT('Ctrl Pts',(-187.611392142768,3.08421727009468,
134.637818410382));
#245483=CARTESIAN_POINT('Ctrl Pts',(-187.619166476887,3.18957636621408,
134.550626137116));
#245484=CARTESIAN_POINT('Ctrl Pts',(-187.626940811006,3.29124596951094,
134.45906758676));
#245485=CARTESIAN_POINT('Ctrl Pts',(-187.634705563953,3.3927902741082,134.367621874136));
#245486=CARTESIAN_POINT('Ctrl Pts',(-187.6424703169,3.49065384526458,134.271820850219));
#245487=CARTESIAN_POINT('Ctrl Pts',(-187.650235069847,3.58444242726253,
134.171994140998));
#245488=CARTESIAN_POINT('Ctrl Pts',(-187.657992110732,3.67813785711891,
134.072266581071));
#245489=CARTESIAN_POINT('Ctrl Pts',(-187.665749151617,3.76776608622933,
133.968521575866));
#245490=CARTESIAN_POINT('Ctrl Pts',(-187.673506192502,3.85296760287033,
133.861127490216));
#245491=CARTESIAN_POINT('Ctrl Pts',(-187.681257383742,3.93810486838475,
133.753814391282));
#245492=CARTESIAN_POINT('Ctrl Pts',(-187.689008574982,4.01882182394327,
133.642857994237));
#245493=CARTESIAN_POINT('Ctrl Pts',(-187.696759766223,4.0947976111808,133.528661552846));
#245494=CARTESIAN_POINT('Ctrl Pts',(-187.704507663,4.17074110668214,133.414513647989));
#245495=CARTESIAN_POINT('Ctrl Pts',(-187.712255559777,4.24194722567974,
133.297128762567));
#245496=CARTESIAN_POINT('Ctrl Pts',(-187.720003456554,4.30813716324615,
133.176940910234));
#245497=CARTESIAN_POINT('Ctrl Pts',(-187.727749732638,4.37431325530452,
133.056778198609));
#245498=CARTESIAN_POINT('Ctrl Pts',(-187.735496008722,4.43547506451776,
132.933814028545));
#245499=CARTESIAN_POINT('Ctrl Pts',(-187.743242284806,4.4913888811533,132.808508561395));
#245500=CARTESIAN_POINT('Ctrl Pts',(-187.750988618071,4.54730311053187,
132.683202169268));
#245501=CARTESIAN_POINT('Ctrl Pts',(-187.758734951337,4.59796911071568,
132.555554802601));
#245502=CARTESIAN_POINT('Ctrl Pts',(-187.766481284602,4.64320078906951,
132.426047854639));
#245503=CARTESIAN_POINT('Ctrl Pts',(-187.774229352605,4.68844259674417,
132.296511904493));
#245504=CARTESIAN_POINT('Ctrl Pts',(-187.781977420608,4.72824753205442,
132.165115913412));
#245505=CARTESIAN_POINT('Ctrl Pts',(-187.789725488611,4.76247909170162,
132.032357345414));
#245506=CARTESIAN_POINT('Ctrl Pts',(-187.797481791353,4.79674703305773,
131.899457680029));
#245507=CARTESIAN_POINT('Ctrl Pts',(-187.805238094095,4.82542966824893,
131.765192924051));
#245508=CARTESIAN_POINT('Ctrl Pts',(-187.812994396837,4.8484413385891,131.630072219011));
#245509=CARTESIAN_POINT('Ctrl Pts',(-187.820754839351,4.87146529095061,
131.494879395982));
#245510=CARTESIAN_POINT('Ctrl Pts',(-187.828515281865,4.88881219795085,
131.358830101222));
#245511=CARTESIAN_POINT('Ctrl Pts',(-187.836275724379,4.90044833640633,
131.22243855852));
#245512=CARTESIAN_POINT('Ctrl Pts',(-187.844048624645,4.91210315422426,
131.085828068006));
#245513=CARTESIAN_POINT('Ctrl Pts',(-187.85182152491,4.9180288671356,130.948874622484));
#245514=CARTESIAN_POINT('Ctrl Pts',(-187.859594425176,4.91824392115051,
130.812093312181));
#245515=CARTESIAN_POINT('Ctrl Pts',(-187.867084760937,4.9184511574103,130.68028434704));
#245516=CARTESIAN_POINT('Ctrl Pts',(-187.874575096699,4.91335573198571,
130.548635527089));
#245517=CARTESIAN_POINT('Ctrl Pts',(-187.882065432461,4.90301950702024,
130.417601291526));
#245518=CARTESIAN_POINT('Ctrl Pts',(-187.88983976658,4.89229138094348,130.281598853093));
#245519=CARTESIAN_POINT('Ctrl Pts',(-187.897614100699,4.87588321702286,
130.145827708113));
#245520=CARTESIAN_POINT('Ctrl Pts',(-187.905388434818,4.85380731953623,
130.010800558518));
#245521=CARTESIAN_POINT('Ctrl Pts',(-187.913153187766,4.83175862862026,
129.875939817817));
#245522=CARTESIAN_POINT('Ctrl Pts',(-187.920917940713,4.80405616463346,
129.741821630265));
#245523=CARTESIAN_POINT('Ctrl Pts',(-187.92868269366,4.77076414640998,129.608955865263));
#245524=CARTESIAN_POINT('Ctrl Pts',(-187.936439734545,4.73750519428833,
129.476222064411));
#245525=CARTESIAN_POINT('Ctrl Pts',(-187.94419677543,4.69866783032351,129.344738587432));
#245526=CARTESIAN_POINT('Ctrl Pts',(-187.951953816315,4.65436764541508,
129.21500701191));
#245527=CARTESIAN_POINT('Ctrl Pts',(-187.959705007555,4.61010086762063,
129.085373267977));
#245528=CARTESIAN_POINT('Ctrl Pts',(-187.967456198795,4.56037959443934,
128.95748916438));
#245529=CARTESIAN_POINT('Ctrl Pts',(-187.975207390035,4.50536966289933,
128.831842616856));
#245530=CARTESIAN_POINT('Ctrl Pts',(-187.982955286812,4.45038311204773,
128.706249472466));
#245531=CARTESIAN_POINT('Ctrl Pts',(-187.990703183589,4.39011253005438,
128.582892350036));
#245532=CARTESIAN_POINT('Ctrl Pts',(-187.998451080366,4.32477236402399,
128.462240411028));
#245533=CARTESIAN_POINT('Ctrl Pts',(-188.006197356451,4.25944586574759,
128.341613709804));
#245534=CARTESIAN_POINT('Ctrl Pts',(-188.013943632535,4.18905207878634,
128.223691410034));
#245535=CARTESIAN_POINT('Ctrl Pts',(-188.021689908619,4.11385182410005,
128.108918866786));
#245536=CARTESIAN_POINT('Ctrl Pts',(-188.029436241884,4.03865101430267,
127.994145476313));
#245537=CARTESIAN_POINT('Ctrl Pts',(-188.03718257515,3.95864388025005,127.882522215779));
#245538=CARTESIAN_POINT('Ctrl Pts',(-188.044928908415,3.87413484409709,
127.774465854995));
#245539=CARTESIAN_POINT('Ctrl Pts',(-188.052676976418,3.78960688273153,
127.666385295739));
#245540=CARTESIAN_POINT('Ctrl Pts',(-188.060425044421,3.70057525393309,
127.561873533624));
#245541=CARTESIAN_POINT('Ctrl Pts',(-188.068173112424,3.60738470489975,
127.461314304193));
#245542=CARTESIAN_POINT('Ctrl Pts',(-188.075929415166,3.51409511184179,
127.360648199217));
#245543=CARTESIAN_POINT('Ctrl Pts',(-188.083685717908,3.416638034995,127.26394330569));
#245544=CARTESIAN_POINT('Ctrl Pts',(-188.091442020649,3.31539552893747,
127.171546894128));
#245545=CARTESIAN_POINT('Ctrl Pts',(-188.099202463164,3.21409898670611,
127.079101167818));
#245546=CARTESIAN_POINT('Ctrl Pts',(-188.106962905678,3.10901328886408,
126.990968756662));
#245547=CARTESIAN_POINT('Ctrl Pts',(-188.114723348192,3.00055283824357,
126.907455983448));
#245548=CARTESIAN_POINT('Ctrl Pts',(-188.122496248457,2.89191827727905,
126.823809148117));
#245549=CARTESIAN_POINT('Ctrl Pts',(-188.130269148723,2.77989845741056,
126.744796995441));
#245550=CARTESIAN_POINT('Ctrl Pts',(-188.138042048988,2.66493670915268,
126.670682425119));
#245551=CARTESIAN_POINT('Ctrl Pts',(-188.14553238475,2.55415411001514,126.599262106112));
#245552=CARTESIAN_POINT('Ctrl Pts',(-188.153022720512,2.44064002739613,
126.532389628946));
#245553=CARTESIAN_POINT('Ctrl Pts',(-188.160513056274,2.32481023186287,
126.470258582735));
#245554=CARTESIAN_POINT('Ctrl Pts',(-188.168287390393,2.2045887144261,126.405771819022));
#245555=CARTESIAN_POINT('Ctrl Pts',(-188.176061724512,2.0814915915248,126.346188851776));
#245556=CARTESIAN_POINT('Ctrl Pts',(-188.183836058631,1.95595686457699,
126.291776456975));
#245557=CARTESIAN_POINT('Ctrl Pts',(-188.191600811579,1.83057684796112,
126.237431120589));
#245558=CARTESIAN_POINT('Ctrl Pts',(-188.199365564526,1.70276555989438,
126.188243831725));
#245559=CARTESIAN_POINT('Ctrl Pts',(-188.207130317473,1.5729866797913,126.144436158125));
#245560=CARTESIAN_POINT('Ctrl Pts',(-188.214887358358,1.4433366979015,126.100671994924));
#245561=CARTESIAN_POINT('Ctrl Pts',(-188.222644399243,1.3117233810346,126.062276938189));
#245562=CARTESIAN_POINT('Ctrl Pts',(-188.230401440128,1.17863120032339,
126.029424852959));
#245563=CARTESIAN_POINT('Ctrl Pts',(-188.238152631368,1.04563938546079,
125.996597541742));
#245564=CARTESIAN_POINT('Ctrl Pts',(-188.245903822608,0.911171304574001,
125.969304975312));
#245565=CARTESIAN_POINT('Ctrl Pts',(-188.253655013848,0.775727093957084,
125.947671360654));
#245566=CARTESIAN_POINT('Ctrl Pts',(-188.261402910625,0.640340450742956,
125.92604694086));
#245567=CARTESIAN_POINT('Ctrl Pts',(-188.269150807402,0.503978888229026,
125.910076750604));
#245568=CARTESIAN_POINT('Ctrl Pts',(-188.276898704179,0.36715303913928,
125.899833962694));
#245569=CARTESIAN_POINT('Ctrl Pts',(-188.284644980264,0.230355811067541,
125.889593317354));
#245570=CARTESIAN_POINT('Ctrl Pts',(-188.292391256348,0.0930948792217825,
125.885077720542));
#245571=CARTESIAN_POINT('Ctrl Pts',(-188.300137532432,-0.0441140864660505,
125.886308461491));
#245572=CARTESIAN_POINT('Ctrl Pts',(-188.307883865697,-0.181324064999486,
125.887539211525));
#245573=CARTESIAN_POINT('Ctrl Pts',(-188.315630198963,-0.318481685660068,
125.894516380455));
#245574=CARTESIAN_POINT('Ctrl Pts',(-188.323376532228,-0.455071760591299,
125.907209123563));
#245575=CARTESIAN_POINT('Ctrl Pts',(-188.331124600231,-0.591692423922576,
125.919904709124));
#245576=CARTESIAN_POINT('Ctrl Pts',(-188.338872668234,-0.727744899400813,
125.938318379674));
#245577=CARTESIAN_POINT('Ctrl Pts',(-188.346620736237,-0.862719995164512,
125.962367508066));
#245578=CARTESIAN_POINT('Ctrl Pts',(-188.354377038979,-0.997838544066398,
125.986442196158));
#245579=CARTESIAN_POINT('Ctrl Pts',(-188.362133341721,-1.13187704037199,
126.016164237938));
#245580=CARTESIAN_POINT('Ctrl Pts',(-188.369889644462,-1.26433680573185,
126.051399908264));
#245581=CARTESIAN_POINT('Ctrl Pts',(-188.377650086977,-1.39686726885678,
126.086654384927));
#245582=CARTESIAN_POINT('Ctrl Pts',(-188.385410529491,-1.52781694894612,
126.12742823772));
#245583=CARTESIAN_POINT('Ctrl Pts',(-188.393170972005,-1.65670413311006,
126.173538392751));
#245584=CARTESIAN_POINT('Ctrl Pts',(-188.40094387227,-1.78579821842409,
126.219722567897));
#245585=CARTESIAN_POINT('Ctrl Pts',(-188.408716772536,-1.91282282908581,
126.271260016418));
#245586=CARTESIAN_POINT('Ctrl Pts',(-188.416489672801,-2.03731714916122,
126.327919855506));
#245587=CARTESIAN_POINT('Ctrl Pts',(-188.423980008563,-2.15728578711929,
126.382519966725));
#245588=CARTESIAN_POINT('Ctrl Pts',(-188.431470344325,-2.27490463047672,
126.441876371959));
#245589=CARTESIAN_POINT('Ctrl Pts',(-188.438960680087,-2.38978607308234,
126.505743911299));
#245590=CARTESIAN_POINT('Ctrl Pts',(-188.446736064809,-2.50903939390405,
126.572041965939));
#245591=CARTESIAN_POINT('Ctrl Pts',(-188.454511449531,-2.62572065138844,
126.643411342122));
#245592=CARTESIAN_POINT('Ctrl Pts',(-188.462286834253,-2.73936846326012,
126.719627641594));
#245593=CARTESIAN_POINT('Ctrl Pts',(-188.470052407546,-2.85287286776605,
126.795747766942));
#245594=CARTESIAN_POINT('Ctrl Pts',(-188.477817980839,-2.96335112181759,
126.876702429187));
#245595=CARTESIAN_POINT('Ctrl Pts',(-188.485583554132,-3.07036605036914,
126.96222119021));
#245596=CARTESIAN_POINT('Ctrl Pts',(-188.493339764738,-3.177251954663,127.047636844174));
#245597=CARTESIAN_POINT('Ctrl Pts',(-188.501095975344,-3.28068254643464,
127.137605394597));
#245598=CARTESIAN_POINT('Ctrl Pts',(-188.508852185949,-3.38024981628517,
127.23181331319));
#245599=CARTESIAN_POINT('Ctrl Pts',(-188.516603088238,-3.47974894273336,
127.325956756297));
#245600=CARTESIAN_POINT('Ctrl Pts',(-188.524353990527,-3.57538972474253,
127.424333527832));
#245601=CARTESIAN_POINT('Ctrl Pts',(-188.532104892816,-3.66679737349336,
127.526590020919));
#245602=CARTESIAN_POINT('Ctrl Pts',(-188.539852169042,-3.75816225948245,
127.628798675886));
#245603=CARTESIAN_POINT('Ctrl Pts',(-188.547599445267,-3.84529769319432,
127.734883149714));
#245604=CARTESIAN_POINT('Ctrl Pts',(-188.555346721492,-3.92786618611514,
127.844453476037));
#245605=CARTESIAN_POINT('Ctrl Pts',(-188.563092051104,-4.01041393253067,
127.953996271261));
#245606=CARTESIAN_POINT('Ctrl Pts',(-188.570837380716,-4.08839678790403,
128.067022863189));
#245607=CARTESIAN_POINT('Ctrl Pts',(-188.578582710328,-4.1615182156311,
128.183111067548));
#245608=CARTESIAN_POINT('Ctrl Pts',(-188.586330187877,-4.23465992141677,
128.299231465526));
#245609=CARTESIAN_POINT('Ctrl Pts',(-188.594077665427,-4.302937292578,128.41841484449));
#245610=CARTESIAN_POINT('Ctrl Pts',(-188.601825142976,-4.36609769469263,
128.540210891311));
#245611=CARTESIAN_POINT('Ctrl Pts',(-188.609573616128,-4.42926621333887,
128.662022589734));
#245612=CARTESIAN_POINT('Ctrl Pts',(-188.617322089279,-4.48731628029937,
128.78644727399));
#245613=CARTESIAN_POINT('Ctrl Pts',(-188.625070562431,-4.54004215253343,
128.913011808985));
#245614=CARTESIAN_POINT('Ctrl Pts',(-188.632825393423,-4.59281128782829,
129.03968019374));
#245615=CARTESIAN_POINT('Ctrl Pts',(-188.640580224415,-4.64024735853174,
129.168491572479));
#245616=CARTESIAN_POINT('Ctrl Pts',(-188.648335055407,-4.68219341291706,
129.298954391149));
#245617=CARTESIAN_POINT('Ctrl Pts',(-188.653905981131,-4.7123266748338,
129.392676443031));
#245618=CARTESIAN_POINT('Ctrl Pts',(-188.659476906855,-4.73962772385923,
129.487250379779));
#245619=CARTESIAN_POINT('Ctrl Pts',(-188.665047832579,-4.76405452823406,
129.582490119308));
#245620=CARTESIAN_POINT('',(-186.639859435958,-4.91824992550734,130.803504611091));
#245621=CARTESIAN_POINT('Ctrl Pts',(-186.639859435995,-4.91824992550745,
130.803504611754));
#245622=CARTESIAN_POINT('Ctrl Pts',(-186.647875869329,-4.91827469762084,
130.945834772432));
#245623=CARTESIAN_POINT('Ctrl Pts',(-186.655892302664,-4.91211675181942,
131.08808080582));
#245624=CARTESIAN_POINT('Ctrl Pts',(-186.663908735998,-4.89982403781472,
131.229692794756));
#245625=CARTESIAN_POINT('Ctrl Pts',(-186.671932409808,-4.88752022097909,
131.371432688235));
#245626=CARTESIAN_POINT('Ctrl Pts',(-186.679956083619,-4.86907061660121,
131.512537046391));
#245627=CARTESIAN_POINT('Ctrl Pts',(-186.68797975743,-4.84457475465937,
131.652463505792));
#245628=CARTESIAN_POINT('Ctrl Pts',(-186.696303438758,-4.81916298525302,
131.797621856561));
#245629=CARTESIAN_POINT('Ctrl Pts',(-186.704627120086,-4.78724414801483,
131.941512102986));
#245630=CARTESIAN_POINT('Ctrl Pts',(-186.712950801415,-4.74898628261018,
132.083544869377));
#245631=CARTESIAN_POINT('Ctrl Pts',(-186.720998349268,-4.71199760050266,
132.220865778145));
#245632=CARTESIAN_POINT('Ctrl Pts',(-186.729045897121,-4.6690839408078,
132.356450179057));
#245633=CARTESIAN_POINT('Ctrl Pts',(-186.737093444975,-4.62044665828881,
132.489785116144));
#245634=CARTESIAN_POINT('Ctrl Pts',(-186.745555193041,-4.56930605760306,
132.629982685208));
#245635=CARTESIAN_POINT('Ctrl Pts',(-186.754016941106,-4.51183726098221,
132.767692681952));
#245636=CARTESIAN_POINT('Ctrl Pts',(-186.762478689172,-4.44832931978521,
132.902347587316));
#245637=CARTESIAN_POINT('Ctrl Pts',(-186.770940437238,-4.38482137858837,
133.037002492679));
#245638=CARTESIAN_POINT('Ctrl Pts',(-186.779402185303,-4.31527456651344,
133.168601951196));
#245639=CARTESIAN_POINT('Ctrl Pts',(-186.787863933369,-4.2400305344674,
133.29661343967));
#245640=CARTESIAN_POINT('Ctrl Pts',(-186.795638267488,-4.17089916337693,
133.414225554185));
#245641=CARTESIAN_POINT('Ctrl Pts',(-186.803412601607,-4.09676100795466,
133.529145376511));
#245642=CARTESIAN_POINT('Ctrl Pts',(-186.811186935727,-4.0178513751189,
133.64091722549));
#245643=CARTESIAN_POINT('Ctrl Pts',(-186.818951688674,-3.93903899135325,
133.752551325653));
#245644=CARTESIAN_POINT('Ctrl Pts',(-186.826716441621,-3.85546705377721,
133.861044855384));
#245645=CARTESIAN_POINT('Ctrl Pts',(-186.834481194568,-3.76741631617132,
133.965967386781));
#245646=CARTESIAN_POINT('Ctrl Pts',(-186.842238235453,-3.67945303179932,
134.070785707641));
#245647=CARTESIAN_POINT('Ctrl Pts',(-186.849995276338,-3.5870200496273,
134.172039790846));
#245648=CARTESIAN_POINT('Ctrl Pts',(-186.857752317224,-3.49044069470467,
134.269329133909));
#245649=CARTESIAN_POINT('Ctrl Pts',(-186.865503508464,-3.39393417102474,
134.366545110322));
#245650=CARTESIAN_POINT('Ctrl Pts',(-186.873254699704,-3.29328777264913,
134.459802021349));
#245651=CARTESIAN_POINT('Ctrl Pts',(-186.881005890944,-3.18886403465664,
134.548733626626));
#245652=CARTESIAN_POINT('Ctrl Pts',(-186.888753787722,-3.08448467953826,
134.637627433597));
#245653=CARTESIAN_POINT('Ctrl Pts',(-186.896501684499,-2.97633147498796,
134.722199338236));
#245654=CARTESIAN_POINT('Ctrl Pts',(-186.904249581276,-2.86480246755412,
134.802121226256));
#245655=CARTESIAN_POINT('Ctrl Pts',(-186.91199585736,-2.75329678958435,
134.882026396341));
#245656=CARTESIAN_POINT('Ctrl Pts',(-186.919742133444,-2.63841703088417,
134.957283256941));
#245657=CARTESIAN_POINT('Ctrl Pts',(-186.927488409529,-2.52059252882238,
135.027605385058));
#245658=CARTESIAN_POINT('Ctrl Pts',(-186.935234742794,-2.40276715700672,
135.097928032277));
#245659=CARTESIAN_POINT('Ctrl Pts',(-186.94298107606,-2.2819973341713,135.163315673957));
#245660=CARTESIAN_POINT('Ctrl Pts',(-186.950727409325,-2.15873910496181,
135.223526663237));
#245661=CARTESIAN_POINT('Ctrl Pts',(-186.958475477328,-2.03545327292633,
135.28375113635));
#245662=CARTESIAN_POINT('Ctrl Pts',(-186.966223545331,-1.90967827685561,
135.338796478669));
#245663=CARTESIAN_POINT('Ctrl Pts',(-186.973971613335,-1.78189197661644,
135.388468387478));
#245664=CARTESIAN_POINT('Ctrl Pts',(-186.981727916077,-1.65396986357687,
135.438193088183));
#245665=CARTESIAN_POINT('Ctrl Pts',(-186.989484218819,-1.52403254119107,
135.482532805269));
#245666=CARTESIAN_POINT('Ctrl Pts',(-186.997240521561,-1.3925754703003,
135.521342345538));
#245667=CARTESIAN_POINT('Ctrl Pts',(-187.005000964075,-1.2610482368127,
135.560172599627));
#245668=CARTESIAN_POINT('Ctrl Pts',(-187.012761406589,-1.12800001764879,
135.59346670068));
#245669=CARTESIAN_POINT('Ctrl Pts',(-187.020521849103,-0.993937454370752,
135.621130427231));
#245670=CARTESIAN_POINT('Ctrl Pts',(-187.028294749369,-0.85965968196463,
135.648838562051));
#245671=CARTESIAN_POINT('Ctrl Pts',(-187.036067649635,-0.724364697643503,
135.670898197859));
#245672=CARTESIAN_POINT('Ctrl Pts',(-187.0438405499,-0.588566164980932,
135.687266814898));
#245673=CARTESIAN_POINT('Ctrl Pts',(-187.051330885661,-0.457704251061874,
135.703040391474));
#245674=CARTESIAN_POINT('Ctrl Pts',(-187.058821221422,-0.326375070731452,
135.713529506913));
#245675=CARTESIAN_POINT('Ctrl Pts',(-187.066311557182,-0.19503718887608,
135.718741917125));
#245676=CARTESIAN_POINT('Ctrl Pts',(-187.074085891301,-0.0587195912883398,
135.724151957455));
#245677=CARTESIAN_POINT('Ctrl Pts',(-187.08186022542,0.0780391938607504,
135.723894398637));
#245678=CARTESIAN_POINT('Ctrl Pts',(-187.089634559539,0.214728599968461,
135.717920904248));
#245679=CARTESIAN_POINT('Ctrl Pts',(-187.097399312486,0.351249548599797,
135.711954771656));
#245680=CARTESIAN_POINT('Ctrl Pts',(-187.105164065433,0.48770090147341,
135.700286736615));
#245681=CARTESIAN_POINT('Ctrl Pts',(-187.11292881838,0.62356877312973,135.682920348437));
#245682=CARTESIAN_POINT('Ctrl Pts',(-187.120685859265,0.759301698900149,
135.665571208801));
#245683=CARTESIAN_POINT('Ctrl Pts',(-187.12844290015,0.894451911427142,
135.642535028303));
#245684=CARTESIAN_POINT('Ctrl Pts',(-187.136199941035,1.028507691538,135.613867348089));
#245685=CARTESIAN_POINT('Ctrl Pts',(-187.143951132275,1.16246237914208,
135.585221286396));
#245686=CARTESIAN_POINT('Ctrl Pts',(-187.151702323515,1.2953238963055,135.550952259327));
#245687=CARTESIAN_POINT('Ctrl Pts',(-187.159453514755,1.42658815557148,
135.511167316049));
#245688=CARTESIAN_POINT('Ctrl Pts',(-187.167201411532,1.55779662402658,
135.471399282433));
#245689=CARTESIAN_POINT('Ctrl Pts',(-187.174949308309,1.68740881144558,
135.42612010863));
#245690=CARTESIAN_POINT('Ctrl Pts',(-187.182697205086,1.81493351210572,
135.375487328688));
#245691=CARTESIAN_POINT('Ctrl Pts',(-187.19044348117,1.94243153734725,135.324865140033));
#245692=CARTESIAN_POINT('Ctrl Pts',(-187.198189757255,2.0678425812239,135.268891716883));
#245693=CARTESIAN_POINT('Ctrl Pts',(-187.205936033339,2.19069360062039,
135.207773454299));
#245694=CARTESIAN_POINT('Ctrl Pts',(-187.213682366604,2.31354552687536,
135.146654740553));
#245695=CARTESIAN_POINT('Ctrl Pts',(-187.221428699869,2.43383704090215,
135.080391285736));
#245696=CARTESIAN_POINT('Ctrl Pts',(-187.229175033134,2.55111833508265,
135.009236157092));
#245697=CARTESIAN_POINT('Ctrl Pts',(-187.236923101137,2.66842589359566,
134.938065093751));
#245698=CARTESIAN_POINT('Ctrl Pts',(-187.24467116914,2.78272155665276,134.862000379508));
#245699=CARTESIAN_POINT('Ctrl Pts',(-187.252419237143,2.89358355694662,
134.78133902604));
#245700=CARTESIAN_POINT('Ctrl Pts',(-187.260175539885,3.00456338269382,
134.700591944726));
#245701=CARTESIAN_POINT('Ctrl Pts',(-187.267931842627,3.11210193908768,
134.615238695533));
#245702=CARTESIAN_POINT('Ctrl Pts',(-187.275688145368,3.21580926229213,
134.52561764323));
#245703=CARTESIAN_POINT('Ctrl Pts',(-187.283448587883,3.31957193721782,
134.435948757473));
#245704=CARTESIAN_POINT('Ctrl Pts',(-187.291209030397,3.41949901971309,
134.342007797447));
#245705=CARTESIAN_POINT('Ctrl Pts',(-187.298969472911,3.51523738644899,
134.244170086041));
#245706=CARTESIAN_POINT('Ctrl Pts',(-187.306742373176,3.61112944091017,
134.146175316856));
#245707=CARTESIAN_POINT('Ctrl Pts',(-187.314515273441,3.70281908106574,
134.044271586789));
#245708=CARTESIAN_POINT('Ctrl Pts',(-187.322288173707,3.7899928861312,133.938868072586));
#245709=CARTESIAN_POINT('Ctrl Pts',(-187.329778509469,3.87399770381394,
133.837296241609));
#245710=CARTESIAN_POINT('Ctrl Pts',(-187.337268845232,3.95380912358556,
133.732474905839));
#245711=CARTESIAN_POINT('Ctrl Pts',(-187.344759180995,4.02918580518921,
133.624794061163));
#245712=CARTESIAN_POINT('Ctrl Pts',(-187.352533515114,4.10742041657999,
133.513030464541));
#245713=CARTESIAN_POINT('Ctrl Pts',(-187.360307849233,4.181125188946,133.39783220855));
#245714=CARTESIAN_POINT('Ctrl Pts',(-187.368082183353,4.24998348176541,
133.279602720315));
#245715=CARTESIAN_POINT('Ctrl Pts',(-187.3758469363,4.31875691289296,133.161518939358));
#245716=CARTESIAN_POINT('Ctrl Pts',(-187.383611689247,4.38269555379604,
133.040411693732));
#245717=CARTESIAN_POINT('Ctrl Pts',(-187.391376442194,4.44152462296868,
132.916715248319));
#245718=CARTESIAN_POINT('Ctrl Pts',(-187.399133483079,4.50029526228031,
132.793141659959));
#245719=CARTESIAN_POINT('Ctrl Pts',(-187.406890523964,4.55396626230861,
132.666984340256));
#245720=CARTESIAN_POINT('Ctrl Pts',(-187.414647564849,4.60230775467839,
132.538703834385));
#245721=CARTESIAN_POINT('Ctrl Pts',(-187.42239875609,4.6506127923528,132.410520065842));
#245722=CARTESIAN_POINT('Ctrl Pts',(-187.43014994733,4.69359618468073,132.280216662417));
#245723=CARTESIAN_POINT('Ctrl Pts',(-187.43790113857,4.73107552357416,132.148275589853));
#245724=CARTESIAN_POINT('Ctrl Pts',(-187.445649035347,4.76853893274882,
132.016390595764));
#245725=CARTESIAN_POINT('Ctrl Pts',(-187.453396932125,4.80050283470879,
131.882869692232));
#245726=CARTESIAN_POINT('Ctrl Pts',(-187.461144828902,4.82683425861936,
131.748211295543));
#245727=CARTESIAN_POINT('Ctrl Pts',(-187.468891104986,4.85316017456368,
131.613581066489));
#245728=CARTESIAN_POINT('Ctrl Pts',(-187.47663738107,4.87385588096731,131.477814201007));
#245729=CARTESIAN_POINT('Ctrl Pts',(-187.484383657154,4.88883933248194,
131.34142024524));
#245730=CARTESIAN_POINT('Ctrl Pts',(-187.49212999042,4.90382289460099,131.205025282644));
#245731=CARTESIAN_POINT('Ctrl Pts',(-187.499876323685,4.91309407499838,
131.068003609154));
#245732=CARTESIAN_POINT('Ctrl Pts',(-187.507622656951,4.91662265431028,
130.930870449686));
#245733=CARTESIAN_POINT('Ctrl Pts',(-187.515370724954,4.92015202382305,
130.793706580197));
#245734=CARTESIAN_POINT('Ctrl Pts',(-187.523118792957,4.91793622317329,
130.65643156581));
#245735=CARTESIAN_POINT('Ctrl Pts',(-187.53086686096,4.90999716116407,130.519560793372));
#245736=CARTESIAN_POINT('Ctrl Pts',(-187.538623163702,4.90204966142525,
130.382544553048));
#245737=CARTESIAN_POINT('Ctrl Pts',(-187.546379466444,4.88836677205368,
130.245933803843));
#245738=CARTESIAN_POINT('Ctrl Pts',(-187.554135769186,4.86902238393298,
130.110239527799));
#245739=CARTESIAN_POINT('Ctrl Pts',(-187.5618962117,4.8496676711299,129.974472827634));
#245740=CARTESIAN_POINT('Ctrl Pts',(-187.569656654214,4.82464550985388,
129.839623959516));
#245741=CARTESIAN_POINT('Ctrl Pts',(-187.577417096728,4.79408079809747,
129.706192887293));
#245742=CARTESIAN_POINT('Ctrl Pts',(-187.585189996994,4.76346702115233,
129.572547619668));
#245743=CARTESIAN_POINT('Ctrl Pts',(-187.59296289726,4.72729301712821,129.440325073378));
#245744=CARTESIAN_POINT('Ctrl Pts',(-187.600735797525,4.6857336264191,129.310010108232));
#245745=CARTESIAN_POINT('Ctrl Pts',(-187.608226133286,4.64568502424898,
129.184432420329));
#245746=CARTESIAN_POINT('Ctrl Pts',(-187.615716469048,4.60063588766843,
129.060626320137));
#245747=CARTESIAN_POINT('Ctrl Pts',(-187.623206804809,4.55078388095632,
128.939005656351));
#245748=CARTESIAN_POINT('Ctrl Pts',(-187.630981138928,4.49904172025193,
128.812773708119));
#245749=CARTESIAN_POINT('Ctrl Pts',(-187.638755473047,4.4419613947056,128.688496324464));
#245750=CARTESIAN_POINT('Ctrl Pts',(-187.646529807166,4.37971116704724,
128.566657966242));
#245751=CARTESIAN_POINT('Ctrl Pts',(-187.654294560113,4.31753765723083,
128.444969762907));
#245752=CARTESIAN_POINT('Ctrl Pts',(-187.66205931306,4.25020709874698,128.325714949011));
#245753=CARTESIAN_POINT('Ctrl Pts',(-187.669824066007,4.17793632482349,
128.209359436792));
#245754=CARTESIAN_POINT('Ctrl Pts',(-187.677581106892,4.1057373312515,128.093119490508));
#245755=CARTESIAN_POINT('Ctrl Pts',(-187.685338147778,4.02860809172652,
127.979773445279));
#245756=CARTESIAN_POINT('Ctrl Pts',(-187.693095188663,3.94681182647804,
127.869763631799));
#245757=CARTESIAN_POINT('Ctrl Pts',(-187.700846379903,3.86507724442891,
127.759836777574));
#245758=CARTESIAN_POINT('Ctrl Pts',(-187.708597571143,3.77868287422416,
127.653241459867));
#245759=CARTESIAN_POINT('Ctrl Pts',(-187.716348762383,3.68793561126631,
127.550391658025));
#245760=CARTESIAN_POINT('Ctrl Pts',(-187.72409665916,3.59722691831658,127.447585570094));
#245761=CARTESIAN_POINT('Ctrl Pts',(-187.731844555937,3.50216927043818,
127.348522124323));
#245762=CARTESIAN_POINT('Ctrl Pts',(-187.739592452715,3.40311012538557,
127.253582599019));
#245763=CARTESIAN_POINT('Ctrl Pts',(-187.747338728799,3.30407170137063,
127.158662933017));
#245764=CARTESIAN_POINT('Ctrl Pts',(-187.755085004883,3.20103372715624,
127.067865742005));
#245765=CARTESIAN_POINT('Ctrl Pts',(-187.762831280967,3.09438055082806,
126.981535475193));
#245766=CARTESIAN_POINT('Ctrl Pts',(-187.770577614232,2.9877265872108,126.895204571112));
#245767=CARTESIAN_POINT('Ctrl Pts',(-187.778323947498,2.87745767211547,
126.813340903009));
#245768=CARTESIAN_POINT('Ctrl Pts',(-187.786070280763,2.76399094455158,
126.736248386944));
#245769=CARTESIAN_POINT('Ctrl Pts',(-187.793818348766,2.6504988069003,126.659138606544));
#245770=CARTESIAN_POINT('Ctrl Pts',(-187.801566416769,2.53380775509228,
126.586802323981));
#245771=CARTESIAN_POINT('Ctrl Pts',(-187.809314484772,2.41436324092127,
126.519499685938));
#245772=CARTESIAN_POINT('Ctrl Pts',(-187.817070787514,2.29479177969936,
126.452125517851));
#245773=CARTESIAN_POINT('Ctrl Pts',(-187.824827090256,2.17246135144864,
126.389795873351));
#245774=CARTESIAN_POINT('Ctrl Pts',(-187.832583392998,2.0478417996602,126.33272478422));
#245775=CARTESIAN_POINT('Ctrl Pts',(-187.840343835512,1.92315573466474,
126.27562323453));
#245776=CARTESIAN_POINT('Ctrl Pts',(-187.848104278026,1.79617847343045,
126.223785980392));
#245777=CARTESIAN_POINT('Ctrl Pts',(-187.855864720541,1.66739816011783,
126.177378184259));
#245778=CARTESIAN_POINT('Ctrl Pts',(-187.863637620806,1.53841111721335,
126.130895890211));
#245779=CARTESIAN_POINT('Ctrl Pts',(-187.871410521072,1.40761561151015,
126.089860588313));
#245780=CARTESIAN_POINT('Ctrl Pts',(-187.879183421337,1.27551407480012,
126.054387258958));
#245781=CARTESIAN_POINT('Ctrl Pts',(-187.886673757098,1.14821476170498,
126.02020347448));
#245782=CARTESIAN_POINT('Ctrl Pts',(-187.89416409286,1.01970302453186,125.991184367656));
#245783=CARTESIAN_POINT('Ctrl Pts',(-187.901654428621,0.890433888279403,
125.967387333259));
#245784=CARTESIAN_POINT('Ctrl Pts',(-187.90942876274,0.756263473425365,
125.942688027067));
#245785=CARTESIAN_POINT('Ctrl Pts',(-187.917203096859,0.620852080617946,
125.923536360038));
#245786=CARTESIAN_POINT('Ctrl Pts',(-187.924977430978,0.484698250610068,
125.910052630899));
#245787=CARTESIAN_POINT('Ctrl Pts',(-187.932742183925,0.34871221802889,
125.89658551925));
#245788=CARTESIAN_POINT('Ctrl Pts',(-187.940506936872,0.211985954126687,
125.888772485131));
#245789=CARTESIAN_POINT('Ctrl Pts',(-187.948271689819,0.0750286477215531,
125.886682937551));
#245790=CARTESIAN_POINT('Ctrl Pts',(-187.956028730704,-0.0617926307557264,
125.884595465339));
#245791=CARTESIAN_POINT('Ctrl Pts',(-187.963785771589,-0.198844106680892,
125.888220172887));
#245792=CARTESIAN_POINT('Ctrl Pts',(-187.971542812474,-0.33561135775171,
125.897574696105));
#245793=CARTESIAN_POINT('Ctrl Pts',(-187.979294003714,-0.472275471574414,
125.906922165004));
#245794=CARTESIAN_POINT('Ctrl Pts',(-187.987045194954,-0.608655398690284,
125.921990822516));
#245795=CARTESIAN_POINT('Ctrl Pts',(-187.994796386194,-0.744236962088531,
125.942746234795));
#245796=CARTESIAN_POINT('Ctrl Pts',(-188.002544282971,-0.879760899705762,
125.963492825471));
#245797=CARTESIAN_POINT('Ctrl Pts',(-188.010292179749,-1.01448676284468,
125.989921304604));
#245798=CARTESIAN_POINT('Ctrl Pts',(-188.018040076526,-1.14790596186375,
126.021945436382));
#245799=CARTESIAN_POINT('Ctrl Pts',(-188.02578635261,-1.28129725246294,
126.053962869403));
#245800=CARTESIAN_POINT('Ctrl Pts',(-188.033532628694,-1.41338204267613,
126.091573535708));
#245801=CARTESIAN_POINT('Ctrl Pts',(-188.041278904778,-1.54366278809802,
126.134640255581));
#245802=CARTESIAN_POINT('Ctrl Pts',(-188.049025238043,-1.67394449522224,
126.177707293362));
#245803=CARTESIAN_POINT('Ctrl Pts',(-188.056771571308,-1.80242175977307,
126.226230342367));
#245804=CARTESIAN_POINT('Ctrl Pts',(-188.064517904574,-1.928613414739,126.280022725787));
#245805=CARTESIAN_POINT('Ctrl Pts',(-188.072265972577,-2.05483332945198,
126.333827155638));
#245806=CARTESIAN_POINT('Ctrl Pts',(-188.080014040579,-2.17876625648171,
126.392903114748));
#245807=CARTESIAN_POINT('Ctrl Pts',(-188.087762108582,-2.29995254948067,
126.457016447543));
#245808=CARTESIAN_POINT('Ctrl Pts',(-188.095518411324,-2.42126764071347,
126.52119792075));
#245809=CARTESIAN_POINT('Ctrl Pts',(-188.103274714066,-2.53982992045492,
126.590427279275));
#245810=CARTESIAN_POINT('Ctrl Pts',(-188.111031016808,-2.65520535582168,
126.664424919887));
#245811=CARTESIAN_POINT('Ctrl Pts',(-188.118791459322,-2.77064237053186,
126.738462055268));
#245812=CARTESIAN_POINT('Ctrl Pts',(-188.126551901836,-2.88288883183471,
126.817272319268));
#245813=CARTESIAN_POINT('Ctrl Pts',(-188.13431234435,-2.99154193003811,
126.900534296721));
#245814=CARTESIAN_POINT('Ctrl Pts',(-188.142085244616,-3.1003694478408,
126.983929933691));
#245815=CARTESIAN_POINT('Ctrl Pts',(-188.149858144881,-3.20559177519847,
127.071791313939));
#245816=CARTESIAN_POINT('Ctrl Pts',(-188.157631045146,-3.30684059919295,
127.163757877081));
#245817=CARTESIAN_POINT('Ctrl Pts',(-188.165121380909,-3.4044087734147,
127.252381224011));
#245818=CARTESIAN_POINT('Ctrl Pts',(-188.172611716672,-3.49828710288302,
127.344816252083));
#245819=CARTESIAN_POINT('Ctrl Pts',(-188.180102052434,-3.58818134762388,
127.440711159156));
#245820=CARTESIAN_POINT('Ctrl Pts',(-188.187783968033,-3.6803748116775,
127.539058764095));
#245821=CARTESIAN_POINT('Ctrl Pts',(-188.195465883631,-3.76868519027518,
127.641374004402));
#245822=CARTESIAN_POINT('Ctrl Pts',(-188.20314779923,-3.85274535651832,
127.747313630631));
#245823=CARTESIAN_POINT('Ctrl Pts',(-188.210820609535,-3.93670588713396,
127.85312768774));
#245824=CARTESIAN_POINT('Ctrl Pts',(-188.21849341984,-4.01642597523958,
127.962557278402));
#245825=CARTESIAN_POINT('Ctrl Pts',(-188.226166230145,-4.09157506968238,
128.075222198274));
#245826=CARTESIAN_POINT('Ctrl Pts',(-188.233972786232,-4.16803409802803,
128.189850995414));
#245827=CARTESIAN_POINT('Ctrl Pts',(-188.241779342318,-4.23976097868823,
128.307828684763));
#245828=CARTESIAN_POINT('Ctrl Pts',(-188.249585898404,-4.3064496647105,
128.428718736344));
#245829=CARTESIAN_POINT('Ctrl Pts',(-188.257245164482,-4.37188010355881,
128.547327897795));
#245830=CARTESIAN_POINT('Ctrl Pts',(-188.26490443056,-4.43246057085316,
128.668740130964));
#245831=CARTESIAN_POINT('Ctrl Pts',(-188.272563696638,-4.4879455798733,
128.792513820567));
#245832=CARTESIAN_POINT('Ctrl Pts',(-188.280443897728,-4.54503107920871,
128.919857818529));
#245833=CARTESIAN_POINT('Ctrl Pts',(-188.288324098819,-4.59672247009533,
129.049701204745));
#245834=CARTESIAN_POINT('Ctrl Pts',(-188.29620429991,-4.64280362102202,
129.181536659422));
#245835=CARTESIAN_POINT('Ctrl Pts',(-188.304084501,-4.68888477194858,129.3133721141));
#245836=CARTESIAN_POINT('Ctrl Pts',(-188.311964702091,-4.72935551781386,
129.447199204311));
#245837=CARTESIAN_POINT('Ctrl Pts',(-188.319844903182,-4.76405452823404,
129.582490119308));
#245838=CARTESIAN_POINT('Ctrl Pts',(-186.570144995258,-4.76405452823391,
129.582490119308));
#245839=CARTESIAN_POINT('Ctrl Pts',(-186.57840025716,-4.80024267923322,
129.723587170822));
#245840=CARTESIAN_POINT('Ctrl Pts',(-186.586655519063,-4.83019874442568,
129.866450467451));
#245841=CARTESIAN_POINT('Ctrl Pts',(-186.594910780965,-4.8537620318651,
130.010523606257));
#245842=CARTESIAN_POINT('Ctrl Pts',(-186.603145195941,-4.87726581518243,
130.154232918679));
#245843=CARTESIAN_POINT('Ctrl Pts',(-186.611379610917,-4.89440896454415,
130.299145675755));
#245844=CARTESIAN_POINT('Ctrl Pts',(-186.619614025893,-4.90508133671532,
130.444693906975));
#245845=CARTESIAN_POINT('Ctrl Pts',(-186.626362495915,-4.9138278213004,
130.563977168498));
#245846=CARTESIAN_POINT('Ctrl Pts',(-186.633110965936,-4.91822907159551,
130.683686883876));
#245847=CARTESIAN_POINT('Ctrl Pts',(-186.639859435957,-4.91824992550734,
130.803504611091));
#245848=CARTESIAN_POINT('Origin',(213.235140564004,0.,130.804360617566));
#245849=CARTESIAN_POINT('',(-184.819837330039,-4.76405452823405,129.582490119308));
#245850=CARTESIAN_POINT('',(-185.165421073984,-4.76405452823401,129.582490119308));
#245851=CARTESIAN_POINT('',(213.235140564004,-4.76405452823405,129.582490119308));
#245852=CARTESIAN_POINT('',(-185.235140563977,-4.91824999726717,130.804196661748));
#245853=CARTESIAN_POINT('Ctrl Pts',(-185.165421073984,-4.76405452823401,
129.582490119308));
#245854=CARTESIAN_POINT('Ctrl Pts',(-185.17357585509,-4.79982922771808,
129.72197512964));
#245855=CARTESIAN_POINT('Ctrl Pts',(-185.181730636195,-4.82951156155369,
129.863179394967));
#245856=CARTESIAN_POINT('Ctrl Pts',(-185.189885417301,-4.85294732447109,
130.005558183663));
#245857=CARTESIAN_POINT('Ctrl Pts',(-185.198024167137,-4.87633701563996,
130.147657073652));
#245858=CARTESIAN_POINT('Ctrl Pts',(-185.206162916974,-4.89350457056318,
130.29092555989));
#245859=CARTESIAN_POINT('Ctrl Pts',(-185.21430166681,-4.90434637358492,
130.434807224395));
#245860=CARTESIAN_POINT('Ctrl Pts',(-185.221247965866,-4.9135996873744,
130.557608034144));
#245861=CARTESIAN_POINT('Ctrl Pts',(-185.228194264921,-4.91824588552851,
130.680855148721));
#245862=CARTESIAN_POINT('Ctrl Pts',(-185.235140563977,-4.91824999726717,
130.804196661748));
#245863=CARTESIAN_POINT('Ctrl Pts',(-185.235140564012,-4.91824999726719,
130.804196662373));
#245864=CARTESIAN_POINT('Ctrl Pts',(-185.243235275636,-4.91825478877005,
130.947929889419));
#245865=CARTESIAN_POINT('Ctrl Pts',(-185.251329987261,-4.91195447570265,
131.09154808551));
#245866=CARTESIAN_POINT('Ctrl Pts',(-185.259424698885,-4.89940510202952,
131.234491654236));
#245867=CARTESIAN_POINT('Ctrl Pts',(-185.267529366981,-4.88684029266407,
131.377611043127));
#245868=CARTESIAN_POINT('Ctrl Pts',(-185.275634035077,-4.86801111637512,
131.520053813894));
#245869=CARTESIAN_POINT('Ctrl Pts',(-185.283738703172,-4.84302506459005,
131.661268597604));
#245870=CARTESIAN_POINT('Ctrl Pts',(-185.291861849205,-4.8179820467862,
131.802805338704));
#245871=CARTESIAN_POINT('Ctrl Pts',(-185.299984995237,-4.78675414792536,
131.9431081626));
#245872=CARTESIAN_POINT('Ctrl Pts',(-185.308108141269,-4.74949972502816,
132.081637182942));
#245873=CARTESIAN_POINT('Ctrl Pts',(-185.316240943695,-4.71220101591753,
132.220330879723));
#245874=CARTESIAN_POINT('Ctrl Pts',(-185.324373746121,-4.66886158835768,
132.357246244439));
#245875=CARTESIAN_POINT('Ctrl Pts',(-185.332506548547,-4.61968871556572,
132.491861501647));
#245876=CARTESIAN_POINT('Ctrl Pts',(-185.340657905423,-4.57040365811858,
132.626783874656));
#245877=CARTESIAN_POINT('Ctrl Pts',(-185.3488092623,-4.51525867281962,132.759395335421));
#245878=CARTESIAN_POINT('Ctrl Pts',(-185.356960619176,-4.45450870042069,
132.889195215412));
#245879=CARTESIAN_POINT('Ctrl Pts',(-185.363319352166,-4.40711869413288,
132.990449864361));
#245880=CARTESIAN_POINT('Ctrl Pts',(-185.369678085156,-4.35631884409728,
133.08999403756));
#245881=CARTESIAN_POINT('Ctrl Pts',(-185.376036818146,-4.3022485761293,
133.187602160443));
#245882=CARTESIAN_POINT('Ctrl Pts',(-185.383811152265,-4.23614101511718,
133.306940110507));
#245883=CARTESIAN_POINT('Ctrl Pts',(-185.391585486384,-4.16495959670137,
133.423714411295));
#245884=CARTESIAN_POINT('Ctrl Pts',(-185.399359820503,-4.08892792282361,
133.537463525335));
#245885=CARTESIAN_POINT('Ctrl Pts',(-185.40712457345,-4.01298995118897,
133.651072453757));
#245886=CARTESIAN_POINT('Ctrl Pts',(-185.414889326397,-3.93221383272465,
133.761663291662));
#245887=CARTESIAN_POINT('Ctrl Pts',(-185.422654079344,-3.84686924586274,
133.868798586874));
#245888=CARTESIAN_POINT('Ctrl Pts',(-185.430411120229,-3.76160942444742,
133.9758274738));
#245889=CARTESIAN_POINT('Ctrl Pts',(-185.438168161114,-3.67179040642328,
134.079407344235));
#245890=CARTESIAN_POINT('Ctrl Pts',(-185.445925201999,-3.57772519128268,
134.179129575311));
#245891=CARTESIAN_POINT('Ctrl Pts',(-185.453676393239,-3.48373091145266,
134.278776605077));
#245892=CARTESIAN_POINT('Ctrl Pts',(-185.461427584479,-3.38549707525688,
134.37457150257));
#245893=CARTESIAN_POINT('Ctrl Pts',(-185.469178775719,-3.28337675376989,
134.466138895303));
#245894=CARTESIAN_POINT('Ctrl Pts',(-185.476926672496,-3.18129983614355,
134.557667369451));
#245895=CARTESIAN_POINT('Ctrl Pts',(-185.484674569273,-3.07534000912483,
134.644971652084));
#245896=CARTESIAN_POINT('Ctrl Pts',(-185.49242246605,-2.96588681661787,
134.727713578174));
#245897=CARTESIAN_POINT('Ctrl Pts',(-185.500168742134,-2.85645651935925,
134.810438196437));
#245898=CARTESIAN_POINT('Ctrl Pts',(-185.507915018218,-2.74353462176835,
134.888602120789));
#245899=CARTESIAN_POINT('Ctrl Pts',(-185.515661294302,-2.62754301228335,
134.961908065413));
#245900=CARTESIAN_POINT('Ctrl Pts',(-185.523407627568,-2.51155054657478,
135.035214551166));
#245901=CARTESIAN_POINT('Ctrl Pts',(-185.531153960833,-2.39248865425077,
135.103662776763));
#245902=CARTESIAN_POINT('Ctrl Pts',(-185.538900294098,-2.27080706495366,
135.166999536415));
#245903=CARTESIAN_POINT('Ctrl Pts',(-185.546648362101,-2.14909822590848,
135.230350479895));
#245904=CARTESIAN_POINT('Ctrl Pts',(-185.554396430104,-2.02476886923059,
135.288587499175));
#245905=CARTESIAN_POINT('Ctrl Pts',(-185.562144498107,-1.89829174083592,
135.341504160499));
#245906=CARTESIAN_POINT('Ctrl Pts',(-185.569900800848,-1.77168019104392,
135.394477062279));
#245907=CARTESIAN_POINT('Ctrl Pts',(-185.57765710359,-1.64291667088637,
135.442118159409));
#245908=CARTESIAN_POINT('Ctrl Pts',(-185.585413406332,-1.51249277472832,
135.484269662504));
#245909=CARTESIAN_POINT('Ctrl Pts',(-185.593173848846,-1.38199926740991,
135.526443663125));
#245910=CARTESIAN_POINT('Ctrl Pts',(-185.60093429136,-1.24984399481776,
135.563122127009));
#245911=CARTESIAN_POINT('Ctrl Pts',(-185.608694733874,-1.11653102912432,
135.594197934584));
#245912=CARTESIAN_POINT('Ctrl Pts',(-185.61646763414,-0.983004057623368,
135.625323627805));
#245913=CARTESIAN_POINT('Ctrl Pts',(-185.624240534405,-0.848316063641948,
135.650828619293));
#245914=CARTESIAN_POINT('Ctrl Pts',(-185.63201343467,-0.712979458432716,
135.670657295159));
#245915=CARTESIAN_POINT('Ctrl Pts',(-185.639503770433,-0.582562679703454,
135.689765148714));
#245916=CARTESIAN_POINT('Ctrl Pts',(-185.646994106196,-0.451543934645043,
135.703602186016));
#245917=CARTESIAN_POINT('Ctrl Pts',(-185.654484441958,-0.320381836731385,
135.712164458511));
#245918=CARTESIAN_POINT('Ctrl Pts',(-185.662258776077,-0.184246688020785,
135.721051372169));
#245919=CARTESIAN_POINT('Ctrl Pts',(-185.670033110196,-0.047525866190644,
135.72428379084));
#245920=CARTESIAN_POINT('Ctrl Pts',(-185.677807444315,0.0892714619018228,
135.721800364893));
#245921=CARTESIAN_POINT('Ctrl Pts',(-185.685572197262,0.225900199513344,
135.719319999546));
#245922=CARTESIAN_POINT('Ctrl Pts',(-185.69333695021,0.362604868635719,
135.711137812602));
#245923=CARTESIAN_POINT('Ctrl Pts',(-185.701101703157,0.498871660584027,
135.697244238578));
#245924=CARTESIAN_POINT('Ctrl Pts',(-185.708858744042,0.635003110433547,
135.683364463847));
#245925=CARTESIAN_POINT('Ctrl Pts',(-185.716615784927,0.770697162159242,
135.663784630225));
#245926=CARTESIAN_POINT('Ctrl Pts',(-185.724372825812,0.905440845898517,
135.638547202409));
#245927=CARTESIAN_POINT('Ctrl Pts',(-185.732124017052,1.04008291837792,
135.613328806334));
#245928=CARTESIAN_POINT('Ctrl Pts',(-185.739875208292,1.17377566665088,
135.58246137983));
#245929=CARTESIAN_POINT('Ctrl Pts',(-185.747626399532,1.3060124356725,135.546039073595));
#245930=CARTESIAN_POINT('Ctrl Pts',(-185.755374296309,1.43819300053959,
135.509632247811));
#245931=CARTESIAN_POINT('Ctrl Pts',(-185.763122193086,1.56891844082116,
135.46767534169));
#245932=CARTESIAN_POINT('Ctrl Pts',(-185.770870089863,1.69769369070752,
135.420313303094));
#245933=CARTESIAN_POINT('Ctrl Pts',(-185.778616365947,1.82644200358802,
135.372961171615));
#245934=CARTESIAN_POINT('Ctrl Pts',(-185.786362642032,1.95324057078163,
135.320206291428));
#245935=CARTESIAN_POINT('Ctrl Pts',(-185.794108918116,2.07761123630648,
135.262242918981));
#245936=CARTESIAN_POINT('Ctrl Pts',(-185.801855251381,2.20198281990683,
135.204279118662));
#245937=CARTESIAN_POINT('Ctrl Pts',(-185.809601584646,2.32392611170664,
135.141106914518));
#245938=CARTESIAN_POINT('Ctrl Pts',(-185.817347917912,2.44298499264541,
135.072967812918));
#245939=CARTESIAN_POINT('Ctrl Pts',(-185.825095985915,2.56207053599523,
135.004813452038));
#245940=CARTESIAN_POINT('Ctrl Pts',(-185.832844053918,2.67827004387223,
134.931690174513));
#245941=CARTESIAN_POINT('Ctrl Pts',(-185.840592121921,2.79115430699464,
134.853884132382));
#245942=CARTESIAN_POINT('Ctrl Pts',(-185.848348424663,2.9041585448554,134.775995397063));
#245943=CARTESIAN_POINT('Ctrl Pts',(-185.856104727404,3.01384017700653,
134.693414177478));
#245944=CARTESIAN_POINT('Ctrl Pts',(-185.863861030146,3.11980073200734,
134.606468776873));
#245945=CARTESIAN_POINT('Ctrl Pts',(-185.871621472661,3.22581784134676,
134.519476970889));
#245946=CARTESIAN_POINT('Ctrl Pts',(-185.879381915175,3.32810962470852,
134.428116602875));
#245947=CARTESIAN_POINT('Ctrl Pts',(-185.887142357689,3.42631349604209,
134.33275386228));
#245948=CARTESIAN_POINT('Ctrl Pts',(-185.894915257954,3.52467501294806,
134.237238036947));
#245949=CARTESIAN_POINT('Ctrl Pts',(-185.90268815822,3.61893523531003,134.13770728394));
#245950=CARTESIAN_POINT('Ctrl Pts',(-185.910461058485,3.70877040278946,
134.034562648692));
#245951=CARTESIAN_POINT('Ctrl Pts',(-185.917951394247,3.79533983565013,
133.935167580741));
#245952=CARTESIAN_POINT('Ctrl Pts',(-185.925441730009,3.8778001590255,133.832417056538));
#245953=CARTESIAN_POINT('Ctrl Pts',(-185.932932065771,3.9559001591004,133.726694786296));
#245954=CARTESIAN_POINT('Ctrl Pts',(-185.94070639989,4.03696134441601,133.616964024045));
#245955=CARTESIAN_POINT('Ctrl Pts',(-185.948480734009,4.11358181358176,
133.503684125752));
#245956=CARTESIAN_POINT('Ctrl Pts',(-185.956255068128,4.18543473429262,
133.38725030694));
#245957=CARTESIAN_POINT('Ctrl Pts',(-185.964019821076,4.25719910270018,
133.270959982405));
#245958=CARTESIAN_POINT('Ctrl Pts',(-185.971784574023,4.32420740995068,
133.15152380069));
#245959=CARTESIAN_POINT('Ctrl Pts',(-185.97954932697,4.38617388218686,133.029368873219));
#245960=CARTESIAN_POINT('Ctrl Pts',(-185.987306367855,4.44807880844942,
132.907335271742));
#245961=CARTESIAN_POINT('Ctrl Pts',(-185.99506340874,4.50495168936313,132.782588644633));
#245962=CARTESIAN_POINT('Ctrl Pts',(-186.002820449625,4.55655097893896,
132.655583521171));
#245963=CARTESIAN_POINT('Ctrl Pts',(-186.010571640865,4.60811135708892,
132.52867417326));
#245964=CARTESIAN_POINT('Ctrl Pts',(-186.018322832105,4.65440591302887,
132.399510079759));
#245965=CARTESIAN_POINT('Ctrl Pts',(-186.026074023345,4.69523999897835,
132.268568394657));
#245966=CARTESIAN_POINT('Ctrl Pts',(-186.033821920122,4.73605672935219,
132.137682363264));
#245967=CARTESIAN_POINT('Ctrl Pts',(-186.041569816899,4.77141748956988,
132.005020615405));
#245968=CARTESIAN_POINT('Ctrl Pts',(-186.049317713676,4.80117663320995,
131.871078011827));
#245969=CARTESIAN_POINT('Ctrl Pts',(-186.05706398976,4.83092955187871,131.737163426154));
#245970=CARTESIAN_POINT('Ctrl Pts',(-186.064810265844,4.85508309987727,
131.601968899102));
#245971=CARTESIAN_POINT('Ctrl Pts',(-186.072556541928,4.87354225566816,
131.466001717194));
#245972=CARTESIAN_POINT('Ctrl Pts',(-186.080302875194,4.89200154772027,
131.330033531608));
#245973=CARTESIAN_POINT('Ctrl Pts',(-186.088049208459,4.90476631109189,
131.193293067196));
#245974=CARTESIAN_POINT('Ctrl Pts',(-186.095795541724,4.91179318843833,
131.056294609935));
#245975=CARTESIAN_POINT('Ctrl Pts',(-186.103543609727,4.91882163940525,
130.919265472818));
#245976=CARTESIAN_POINT('Ctrl Pts',(-186.11129167773,4.92010962740263,130.781978618262));
#245977=CARTESIAN_POINT('Ctrl Pts',(-186.119039745733,4.91566590214478,
130.644949824358));
#245978=CARTESIAN_POINT('Ctrl Pts',(-186.126796048475,4.91121745404283,
130.507775394621));
#245979=CARTESIAN_POINT('Ctrl Pts',(-186.134552351217,4.90102513648487,
130.370859964803));
#245980=CARTESIAN_POINT('Ctrl Pts',(-186.142308653959,4.88514977674217,
130.234716236135));
#245981=CARTESIAN_POINT('Ctrl Pts',(-186.150069096473,4.86926594384197,
130.09849984346));
#245982=CARTESIAN_POINT('Ctrl Pts',(-186.157829538987,4.84769308629387,
129.963056358551));
#245983=CARTESIAN_POINT('Ctrl Pts',(-186.165589981501,4.82054330303636,
129.828888769663));
#245984=CARTESIAN_POINT('Ctrl Pts',(-186.173362881767,4.79334993653653,
129.694505803051));
#245985=CARTESIAN_POINT('Ctrl Pts',(-186.181135782032,4.76056184779475,
129.561403205215));
#245986=CARTESIAN_POINT('Ctrl Pts',(-186.188908682298,4.72234144732119,
129.430070139751));
#245987=CARTESIAN_POINT('Ctrl Pts',(-186.19639901806,4.68551045467694,129.303511362027));
#245988=CARTESIAN_POINT('Ctrl Pts',(-186.203889353822,4.6436353476091,129.178595988423));
#245989=CARTESIAN_POINT('Ctrl Pts',(-186.211379689583,4.59690316518476,
129.05574277698));
#245990=CARTESIAN_POINT('Ctrl Pts',(-186.219154023703,4.54839911785924,
128.928231548683));
#245991=CARTESIAN_POINT('Ctrl Pts',(-186.226928357822,4.49450876631522,
128.802538025928));
#245992=CARTESIAN_POINT('Ctrl Pts',(-186.234702691941,4.43538795572149,
128.679150805632));
#245993=CARTESIAN_POINT('Ctrl Pts',(-186.242467444888,4.37634000624273,
128.555915649057));
#245994=CARTESIAN_POINT('Ctrl Pts',(-186.250232197835,4.31207459079579,
128.434981488786));
#245995=CARTESIAN_POINT('Ctrl Pts',(-186.257996950782,4.2427965825651,128.316819618613));
#245996=CARTESIAN_POINT('Ctrl Pts',(-186.265753991667,4.17358738222901,
128.198775108475));
#245997=CARTESIAN_POINT('Ctrl Pts',(-186.273511032552,4.09937569316561,
128.083497743981));
#245998=CARTESIAN_POINT('Ctrl Pts',(-186.281268073437,4.02041336222315,
127.971436428789));
#245999=CARTESIAN_POINT('Ctrl Pts',(-186.289019264677,3.94151057738879,
127.859459619907));
#246000=CARTESIAN_POINT('Ctrl Pts',(-186.296770455917,3.85786450570213,
127.750694351319));
#246001=CARTESIAN_POINT('Ctrl Pts',(-186.304521647158,3.76977137844832,
127.645562299102));
#246002=CARTESIAN_POINT('Ctrl Pts',(-186.312269543935,3.68171569312366,
127.540474930812));
#246003=CARTESIAN_POINT('Ctrl Pts',(-186.320017440712,3.58921696210682,
127.439018006611));
#246004=CARTESIAN_POINT('Ctrl Pts',(-186.327765337489,3.49261280031067,
127.341581547281));
#246005=CARTESIAN_POINT('Ctrl Pts',(-186.335511613573,3.39602884602262,
127.244165469557));
#246006=CARTESIAN_POINT('Ctrl Pts',(-186.343257889657,3.29534144418254,
127.15076846138));
#246007=CARTESIAN_POINT('Ctrl Pts',(-186.351004165741,3.19092602784825,
127.061744667819));
#246008=CARTESIAN_POINT('Ctrl Pts',(-186.358750499007,3.08650984074266,
126.972720217104));
#246009=CARTESIAN_POINT('Ctrl Pts',(-186.366496832272,2.97836588174077,
126.888069299076));
#246010=CARTESIAN_POINT('Ctrl Pts',(-186.374243165537,2.86690339849536,
126.808106375629));
#246011=CARTESIAN_POINT('Ctrl Pts',(-186.38199123354,2.75541595399981,126.728125545041));
#246012=CARTESIAN_POINT('Ctrl Pts',(-186.389739301543,2.64060882406983,
126.652835025955));
#246013=CARTESIAN_POINT('Ctrl Pts',(-186.397487369546,2.52292067685579,
126.582506247648));
#246014=CARTESIAN_POINT('Ctrl Pts',(-186.405243672288,2.40510744927854,
126.512102723079));
#246015=CARTESIAN_POINT('Ctrl Pts',(-186.41299997503,2.2844074239254,126.44667167434));
#246016=CARTESIAN_POINT('Ctrl Pts',(-186.420756277772,2.16128482948886,
126.386439053264));
#246017=CARTESIAN_POINT('Ctrl Pts',(-186.428516720286,2.03809652081653,
126.326174284226));
#246018=CARTESIAN_POINT('Ctrl Pts',(-186.4362771628,1.9124834245532,126.271113628271));
#246019=CARTESIAN_POINT('Ctrl Pts',(-186.444037605315,1.78492931117828,
126.221434650829));
#246020=CARTESIAN_POINT('Ctrl Pts',(-186.45181050558,1.65717043661684,126.171675924281));
#246021=CARTESIAN_POINT('Ctrl Pts',(-186.459583405845,1.52746468853852,
126.127316266604));
#246022=CARTESIAN_POINT('Ctrl Pts',(-186.467356306111,1.39631140097754,
126.088483442109));
#246023=CARTESIAN_POINT('Ctrl Pts',(-186.474846641873,1.26992586577211,
126.051062288597));
#246024=CARTESIAN_POINT('Ctrl Pts',(-186.482336977635,1.14219650594113,
126.018773191476));
#246025=CARTESIAN_POINT('Ctrl Pts',(-186.489827313397,1.0135767336687,125.991685138431));
#246026=CARTESIAN_POINT('Ctrl Pts',(-186.497601647516,0.880080303639861,
125.963570033623));
#246027=CARTESIAN_POINT('Ctrl Pts',(-186.505375981635,0.745201731765015,
125.940969093346));
#246028=CARTESIAN_POINT('Ctrl Pts',(-186.513150315754,0.609436326590159,
125.924015299217));
#246029=CARTESIAN_POINT('Ctrl Pts',(-186.520915068702,0.47383824014311,
125.907082399123));
#246030=CARTESIAN_POINT('Ctrl Pts',(-186.528679821649,0.337355879254183,
125.895782845622));
#246031=CARTESIAN_POINT('Ctrl Pts',(-186.536444574596,0.200496495701578,
125.890199018909));
#246032=CARTESIAN_POINT('Ctrl Pts',(-186.544201615481,0.0637730428177244,
125.884620738132));
#246033=CARTESIAN_POINT('Ctrl Pts',(-186.551958656366,-0.0733262994167068,
125.88474690261));
#246034=CARTESIAN_POINT('Ctrl Pts',(-186.559715697251,-0.2102877262663,
125.89060826985));
#246035=CARTESIAN_POINT('Ctrl Pts',(-186.567466888491,-0.34714586943757,
125.896465216988));
#246036=CARTESIAN_POINT('Ctrl Pts',(-186.575218079731,-0.483865915208605,
125.908048741667));
#246037=CARTESIAN_POINT('Ctrl Pts',(-186.582969270971,-0.619932975308011,
125.925337542336));
#246038=CARTESIAN_POINT('Ctrl Pts',(-186.590717167748,-0.755942203277722,
125.942618994804));
#246039=CARTESIAN_POINT('Ctrl Pts',(-186.598465064525,-0.891298610539438,
125.965600851155));
#246040=CARTESIAN_POINT('Ctrl Pts',(-186.606212961302,-1.02549157245746,
125.994209882161));
#246041=CARTESIAN_POINT('Ctrl Pts',(-186.613959237386,-1.15965646410071,
126.022812928774));
#246042=CARTESIAN_POINT('Ctrl Pts',(-186.62170551347,-1.29265801234209,
126.057040727289));
#246043=CARTESIAN_POINT('Ctrl Pts',(-186.629451789554,-1.42399533416772,
126.096768839303));
#246044=CARTESIAN_POINT('Ctrl Pts',(-186.63719812282,-1.55533362549545,
126.136497244581));
#246045=CARTESIAN_POINT('Ctrl Pts',(-186.644944456085,-1.68500729167432,
126.181725931178));
#246046=CARTESIAN_POINT('Ctrl Pts',(-186.65269078935,-1.81253055865413,
126.232280561788));
#246047=CARTESIAN_POINT('Ctrl Pts',(-186.660438857353,-1.94008238358522,
126.282846513757));
#246048=CARTESIAN_POINT('Ctrl Pts',(-186.668186925356,-2.06548248767706,
126.338740639035));
#246049=CARTESIAN_POINT('Ctrl Pts',(-186.675934993359,-2.18826539894326,
126.399740587837));
#246050=CARTESIAN_POINT('Ctrl Pts',(-186.683691296101,-2.31117880534887,
126.460805368111));
#246051=CARTESIAN_POINT('Ctrl Pts',(-186.691447598843,-2.43146911172216,
126.526986637757));
#246052=CARTESIAN_POINT('Ctrl Pts',(-186.699203901585,-2.54869529143897,
126.598015960516));
#246053=CARTESIAN_POINT('Ctrl Pts',(-186.706964344099,-2.66598403829782,
126.669083193762));
#246054=CARTESIAN_POINT('Ctrl Pts',(-186.714724786613,-2.7802050743521,
126.745003419722));
#246055=CARTESIAN_POINT('Ctrl Pts',(-186.722485229127,-2.89094751901861,
126.825465607041));
#246056=CARTESIAN_POINT('Ctrl Pts',(-186.730258129393,-3.00186773728824,
126.906056959406));
#246057=CARTESIAN_POINT('Ctrl Pts',(-186.738031029658,-3.10929789869776,
126.991204600203));
#246058=CARTESIAN_POINT('Ctrl Pts',(-186.745803929924,-3.21286060927254,
127.080557485299));
#246059=CARTESIAN_POINT('Ctrl Pts',(-186.753294265686,-3.31265855445779,
127.166662167953));
#246060=CARTESIAN_POINT('Ctrl Pts',(-186.760784601447,-3.40886512528903,
127.256671450161));
#246061=CARTESIAN_POINT('Ctrl Pts',(-186.768274937209,-3.50117720011197,
127.350241152939));
#246062=CARTESIAN_POINT('Ctrl Pts',(-186.775943029108,-3.5956799694917,
127.446031395543));
#246063=CARTESIAN_POINT('Ctrl Pts',(-186.783611121006,-3.68641809312052,
127.545874838496));
#246064=CARTESIAN_POINT('Ctrl Pts',(-186.791279212905,-3.77301654595831,
127.649439191219));
#246065=CARTESIAN_POINT('Ctrl Pts',(-186.798938310547,-3.85951342349731,
127.75288206856));
#246066=CARTESIAN_POINT('Ctrl Pts',(-186.806597408188,-3.94188002817934,
127.860036873487));
#246067=CARTESIAN_POINT('Ctrl Pts',(-186.81425650583,-4.0197769009932,127.970533394756));
#246068=CARTESIAN_POINT('Ctrl Pts',(-186.821908387342,-4.09760038214203,
128.080925810129));
#246069=CARTESIAN_POINT('Ctrl Pts',(-186.829560268854,-4.17096227552672,
128.194653354138));
#246070=CARTESIAN_POINT('Ctrl Pts',(-186.837212150366,-4.23956264999936,
128.311311961958));
#246071=CARTESIAN_POINT('Ctrl Pts',(-186.844858218946,-4.30811091057845,
128.427881947313));
#246072=CARTESIAN_POINT('Ctrl Pts',(-186.852504287526,-4.37190464719919,
128.547378219883));
#246073=CARTESIAN_POINT('Ctrl Pts',(-186.860150356106,-4.43068697554932,
128.669367412144));
#246074=CARTESIAN_POINT('Ctrl Pts',(-186.867793074609,-4.48944354879428,
128.791303155613));
#246075=CARTESIAN_POINT('Ctrl Pts',(-186.875435793112,-4.54319290765865,
128.915729283918));
#246076=CARTESIAN_POINT('Ctrl Pts',(-186.883078511615,-4.59172410237677,
129.04218785925));
#246077=CARTESIAN_POINT('Ctrl Pts',(-186.890720376631,-4.64024987745937,
129.168632312543));
#246078=CARTESIAN_POINT('Ctrl Pts',(-186.898362241647,-4.68355850002953,
129.297108387139));
#246079=CARTESIAN_POINT('Ctrl Pts',(-186.906004106664,-4.72148732126051,
129.427138581119));
#246080=CARTESIAN_POINT('Ctrl Pts',(-186.909033691086,-4.73652403883128,
129.478688490636));
#246081=CARTESIAN_POINT('Ctrl Pts',(-186.912063275508,-4.75071576216139,
129.530482472835));
#246082=CARTESIAN_POINT('Ctrl Pts',(-186.915092859931,-4.76405452823404,
129.582490119308));
#246083=CARTESIAN_POINT('',(-184.889859436036,-4.91824816211532,130.800108753356));
#246084=CARTESIAN_POINT('Ctrl Pts',(-184.889859436036,-4.91824816211532,
130.800108753357));
#246085=CARTESIAN_POINT('Ctrl Pts',(-184.897506058226,-4.91836465031066,
130.934853849735));
#246086=CARTESIAN_POINT('Ctrl Pts',(-184.905152680416,-4.91293956817794,
131.069789576618));
#246087=CARTESIAN_POINT('Ctrl Pts',(-184.912799302606,-4.90195264080868,
131.204414826104));
#246088=CARTESIAN_POINT('Ctrl Pts',(-184.920439094191,-4.89097552788502,
131.338919817018));
#246089=CARTESIAN_POINT('Ctrl Pts',(-184.928078885776,-4.87444648449873,
131.473114482282));
#246090=CARTESIAN_POINT('Ctrl Pts',(-184.935718677362,-4.85239729067965,
131.60649751106));
#246091=CARTESIAN_POINT('Ctrl Pts',(-184.943353957593,-4.83036111707372,
131.739801776167));
#246092=CARTESIAN_POINT('Ctrl Pts',(-184.950989237825,-4.80281134123516,
131.872294960994));
#246093=CARTESIAN_POINT('Ctrl Pts',(-184.958624518056,-4.76983155314398,
132.003481135751));
#246094=CARTESIAN_POINT('Ctrl Pts',(-184.96625747086,-4.73686181813173,
132.134627321622));
#246095=CARTESIAN_POINT('Ctrl Pts',(-184.973890423664,-4.69846545941638,
132.264466898419));
#246096=CARTESIAN_POINT('Ctrl Pts',(-184.981523376467,-4.65477702326063,
132.392514868961));
#246097=CARTESIAN_POINT('Ctrl Pts',(-184.989155769078,-4.61109179346305,
132.520553441876));
#246098=CARTESIAN_POINT('Ctrl Pts',(-184.996788161688,-4.56211538887205,
132.646800288048));
#246099=CARTESIAN_POINT('Ctrl Pts',(-185.004420554298,-4.50803182670943,
132.770786846));
#246100=CARTESIAN_POINT('Ctrl Pts',(-185.012054153287,-4.45393971608056,
132.89479300131));
#246101=CARTESIAN_POINT('Ctrl Pts',(-185.019687752276,-4.39473900456917,
133.016537788303));
#246102=CARTESIAN_POINT('Ctrl Pts',(-185.027321351264,-4.33066108607502,
133.13557438298));
#246103=CARTESIAN_POINT('Ctrl Pts',(-185.034962554895,-4.26651933273594,
133.254729562698));
#246104=CARTESIAN_POINT('Ctrl Pts',(-185.042603758525,-4.19749086029851,
133.371170805936));
#246105=CARTESIAN_POINT('Ctrl Pts',(-185.050244962156,-4.12385227870567,
133.484477302696));
#246106=CARTESIAN_POINT('Ctrl Pts',(-185.057889999776,-4.05017674879779,
133.597840651233));
#246107=CARTESIAN_POINT('Ctrl Pts',(-185.065535037397,-3.9718867376698,
133.708065792888));
#246108=CARTESIAN_POINT('Ctrl Pts',(-185.073180075017,-3.88930031472982,
133.814763601278));
#246109=CARTESIAN_POINT('Ctrl Pts',(-185.080837121003,-3.80658417000405,
133.921629004168));
#246110=CARTESIAN_POINT('Ctrl Pts',(-185.088494166989,-3.7195583925844,
134.024955697636));
#246111=CARTESIAN_POINT('Ctrl Pts',(-185.096151212975,-3.62857964916102,
134.124389652408));
#246112=CARTESIAN_POINT('Ctrl Pts',(-185.103160205481,-3.54530088447839,
134.215408022297));
#246113=CARTESIAN_POINT('Ctrl Pts',(-185.110169197986,-3.45871056569238,
134.303164978857));
#246114=CARTESIAN_POINT('Ctrl Pts',(-185.117178190492,-3.36910616455944,
134.387418908248));
#246115=CARTESIAN_POINT('Ctrl Pts',(-185.124952524611,-3.26971747889623,
134.480872881472));
#246116=CARTESIAN_POINT('Ctrl Pts',(-185.13272685873,-3.1662800113838,134.570336404582));
#246117=CARTESIAN_POINT('Ctrl Pts',(-185.140501192849,-3.05914760954894,
134.655438254474));
#246118=CARTESIAN_POINT('Ctrl Pts',(-185.148265945796,-2.95214723882493,
134.740435223941));
#246119=CARTESIAN_POINT('Ctrl Pts',(-185.156030698744,-2.84146129743104,
134.821080974734));
#246120=CARTESIAN_POINT('Ctrl Pts',(-185.163795451691,-2.7274801549028,
134.897041287629));
#246121=CARTESIAN_POINT('Ctrl Pts',(-185.171552492576,-2.61361222005217,
134.972926155671));
#246122=CARTESIAN_POINT('Ctrl Pts',(-185.179309533461,-2.4964559204001,
135.044134631363));
#246123=CARTESIAN_POINT('Ctrl Pts',(-185.187066574346,-2.37643407513157,
135.110373175496));
#246124=CARTESIAN_POINT('Ctrl Pts',(-185.194817765586,-2.25650273927002,
135.176561768628));
#246125=CARTESIAN_POINT('Ctrl Pts',(-185.202568956826,-2.13371049990436,
135.237787701952));
#246126=CARTESIAN_POINT('Ctrl Pts',(-185.210320148066,-2.00850818166039,
135.293801334037));
#246127=CARTESIAN_POINT('Ctrl Pts',(-185.218068044844,-1.88335907774139,
135.349791158833));
#246128=CARTESIAN_POINT('Ctrl Pts',(-185.225815941621,-1.75580228842462,
135.400572929258));
#246129=CARTESIAN_POINT('Ctrl Pts',(-185.233563838398,-1.62631200864633,
135.445943570938));
#246130=CARTESIAN_POINT('Ctrl Pts',(-185.241310114482,-1.49684881544309,
135.491304722058));
#246131=CARTESIAN_POINT('Ctrl Pts',(-185.249056390566,-1.36545330497909,
135.531256866629));
#246132=CARTESIAN_POINT('Ctrl Pts',(-185.25680266665,-1.23261799023726,
135.56564573323));
#246133=CARTESIAN_POINT('Ctrl Pts',(-185.264548999916,-1.09978169493548,
135.600034853681));
#246134=CARTESIAN_POINT('Ctrl Pts',(-185.272295333181,-0.965505952635501,
135.628860516231));
#246135=CARTESIAN_POINT('Ctrl Pts',(-185.280041666446,-0.830296328772982,
135.65201892534));
#246136=CARTESIAN_POINT('Ctrl Pts',(-185.287789734449,-0.695056425652861,
135.675182520613));
#246137=CARTESIAN_POINT('Ctrl Pts',(-185.295537802453,-0.558882610093101,
135.692676271008));
#246138=CARTESIAN_POINT('Ctrl Pts',(-185.303285870456,-0.42228808350065,
135.704447947097));
#246139=CARTESIAN_POINT('Ctrl Pts',(-185.311042173197,-0.285548382619655,
135.716232134264));
#246140=CARTESIAN_POINT('Ctrl Pts',(-185.318798475939,-0.148387467644769,
135.722282065073));
#246141=CARTESIAN_POINT('Ctrl Pts',(-185.326554778681,-0.0113216354735307,
135.722597586549));
#246142=CARTESIAN_POINT('Ctrl Pts',(-185.334315221195,0.125817352859683,
135.722913276428));
#246143=CARTESIAN_POINT('Ctrl Pts',(-185.34207566371,0.262860766800342,
135.717488473873));
#246144=CARTESIAN_POINT('Ctrl Pts',(-185.349836106224,0.399295898810333,
135.706375085894));
#246145=CARTESIAN_POINT('Ctrl Pts',(-185.357609006489,0.535950048605996,
135.695243857718));
#246146=CARTESIAN_POINT('Ctrl Pts',(-185.365381906755,0.671993576948554,
135.678405843878));
#246147=CARTESIAN_POINT('Ctrl Pts',(-185.37315480702,0.806921561960867,
135.655964543624));
#246148=CARTESIAN_POINT('Ctrl Pts',(-185.380645142782,0.936944574849048,
135.634339041161));
#246149=CARTESIAN_POINT('Ctrl Pts',(-185.388135478544,1.06593144034985,
135.60751062932));
#246150=CARTESIAN_POINT('Ctrl Pts',(-185.395625814305,1.19344424050067,
135.575615579032));
#246151=CARTESIAN_POINT('Ctrl Pts',(-185.403400148425,1.32579172723165,
135.542511218217));
#246152=CARTESIAN_POINT('Ctrl Pts',(-185.411174482543,1.45697040075332,
135.503843566807));
#246153=CARTESIAN_POINT('Ctrl Pts',(-185.418948816663,1.5864766773227,135.459709671591));
#246154=CARTESIAN_POINT('Ctrl Pts',(-185.42671356961,1.71582334898017,135.415630167457));
#246155=CARTESIAN_POINT('Ctrl Pts',(-185.434478322557,1.84350135810591,
135.366097948359));
#246156=CARTESIAN_POINT('Ctrl Pts',(-185.442243075504,1.9690185123329,135.31126078959));
#246157=CARTESIAN_POINT('Ctrl Pts',(-185.450000116389,2.09441100115318,
135.25647809586));
#246158=CARTESIAN_POINT('Ctrl Pts',(-185.457757157274,2.21764655014518,
135.196401103399));
#246159=CARTESIAN_POINT('Ctrl Pts',(-185.465514198159,2.33824965236156,
135.13122687685));
#246160=CARTESIAN_POINT('Ctrl Pts',(-185.473265389399,2.45876180684023,
135.066101798692));
#246161=CARTESIAN_POINT('Ctrl Pts',(-185.481016580639,2.5766451232984,134.995887322545));
#246162=CARTESIAN_POINT('Ctrl Pts',(-185.488767771879,2.69144588960641,
134.920827802644));
#246163=CARTESIAN_POINT('Ctrl Pts',(-185.496515668657,2.80619786252648,
134.84580018504));
#246164=CARTESIAN_POINT('Ctrl Pts',(-185.504263565434,2.91786956457255,
134.76593183292));
#246165=CARTESIAN_POINT('Ctrl Pts',(-185.512011462211,3.02603382957723,
134.681511933256));
#246166=CARTESIAN_POINT('Ctrl Pts',(-185.519757738295,3.13417546894943,
134.597109692414));
#246167=CARTESIAN_POINT('Ctrl Pts',(-185.527504014379,3.23881082260025,
134.508158038173));
#246168=CARTESIAN_POINT('Ctrl Pts',(-185.535250290463,3.33954388231524,
134.414987948182));
#246169=CARTESIAN_POINT('Ctrl Pts',(-185.542996623729,3.44027768561866,
134.32181717043));
#246170=CARTESIAN_POINT('Ctrl Pts',(-185.550742956994,3.53710885048758,
134.224428160262));
#246171=CARTESIAN_POINT('Ctrl Pts',(-185.558489290259,3.62967678032664,
134.123190160169));
#246172=CARTESIAN_POINT('Ctrl Pts',(-185.566237358262,3.72226544011165,
134.021929488529));
#246173=CARTESIAN_POINT('Ctrl Pts',(-185.573985426265,3.81058870130834,
133.916818400254));
#246174=CARTESIAN_POINT('Ctrl Pts',(-185.581733494268,3.89432522392317,
133.808260434939));
#246175=CARTESIAN_POINT('Ctrl Pts',(-185.58948979701,3.97815074271105,133.699587092927));
#246176=CARTESIAN_POINT('Ctrl Pts',(-185.597246099752,4.05737954572931,
133.58745986594));
#246177=CARTESIAN_POINT('Ctrl Pts',(-185.605002402494,4.13173243319085,
133.472313046493));
#246178=CARTESIAN_POINT('Ctrl Pts',(-185.612762845008,4.20612500502695,
133.357104769722));
#246179=CARTESIAN_POINT('Ctrl Pts',(-185.620523287522,4.27563627770473,
133.238874026014));
#246180=CARTESIAN_POINT('Ctrl Pts',(-185.628283730036,4.3400327911151,133.118080227749));
#246181=CARTESIAN_POINT('Ctrl Pts',(-185.636056630302,4.40453267952583,
132.997092520555));
#246182=CARTESIAN_POINT('Ctrl Pts',(-185.643829530567,4.46390123172262,
132.873533889436));
#246183=CARTESIAN_POINT('Ctrl Pts',(-185.651602430833,4.51795260194687,
132.74788508334));
#246184=CARTESIAN_POINT('Ctrl Pts',(-185.659092766595,4.57003906871526,
132.626803927838));
#246185=CARTESIAN_POINT('Ctrl Pts',(-185.666583102356,4.61718811749639,
132.50378221287));
#246186=CARTESIAN_POINT('Ctrl Pts',(-185.674073438118,4.65927769153067,
132.37926202899));
#246187=CARTESIAN_POINT('Ctrl Pts',(-185.681847772237,4.70296310455798,
132.250020624489));
#246188=CARTESIAN_POINT('Ctrl Pts',(-185.689622106357,4.74133619155718,
132.118755481185));
#246189=CARTESIAN_POINT('Ctrl Pts',(-185.697396440476,4.77420640142745,
131.985942734505));
#246190=CARTESIAN_POINT('Ctrl Pts',(-185.705161193423,4.80703610170175,
131.853293667665));
#246191=CARTESIAN_POINT('Ctrl Pts',(-185.71292594637,4.83437632559071,131.719101168244));
#246192=CARTESIAN_POINT('Ctrl Pts',(-185.720690699317,4.85608535863617,
131.583859207776));
#246193=CARTESIAN_POINT('Ctrl Pts',(-185.728447740202,4.87777282996403,
131.448751571529));
#246194=CARTESIAN_POINT('Ctrl Pts',(-185.736204781087,4.89384017916371,
131.312596932063));
#246195=CARTESIAN_POINT('Ctrl Pts',(-185.743961821972,4.90419617918031,
131.175901865092));
#246196=CARTESIAN_POINT('Ctrl Pts',(-185.751713013212,4.9145443696567,131.039309880935));
#246197=CARTESIAN_POINT('Ctrl Pts',(-185.759464204452,4.91918975430297,
130.902178668729));
#246198=CARTESIAN_POINT('Ctrl Pts',(-185.767215395692,4.91809267276772,
130.76502202877));
#246199=CARTESIAN_POINT('Ctrl Pts',(-185.774963292469,4.91699605752139,
130.627923684042));
#246200=CARTESIAN_POINT('Ctrl Pts',(-185.782711189246,4.91016183358293,
130.490800323191));
#246201=CARTESIAN_POINT('Ctrl Pts',(-185.790459086024,4.89760240839343,
130.354167645832));
#246202=CARTESIAN_POINT('Ctrl Pts',(-185.798205362108,4.88504561036494,
130.217563549084));
#246203=CARTESIAN_POINT('Ctrl Pts',(-185.805951638192,4.86676602891934,
130.081450320748));
#246204=CARTESIAN_POINT('Ctrl Pts',(-185.813697914276,4.84282807281364,
129.946340035256));
#246205=CARTESIAN_POINT('Ctrl Pts',(-185.821444247541,4.81888994000336,
129.81122875241));
#246206=CARTESIAN_POINT('Ctrl Pts',(-185.829190580807,4.78929341739268,
129.677120812149));
#246207=CARTESIAN_POINT('Ctrl Pts',(-185.836936914072,4.75415424788159,
129.54451917919));
#246208=CARTESIAN_POINT('Ctrl Pts',(-185.844684982075,4.71900720919718,
129.411887851015));
#246209=CARTESIAN_POINT('Ctrl Pts',(-185.852433050078,4.67831515382283,
129.280763879231));
#246210=CARTESIAN_POINT('Ctrl Pts',(-185.860181118081,4.63224389893416,
129.151635739286));
#246211=CARTESIAN_POINT('Ctrl Pts',(-185.867937420823,4.5861236789676,129.022370360416));
#246212=CARTESIAN_POINT('Ctrl Pts',(-185.875693723564,4.5346129705982,128.895105419515));
#246213=CARTESIAN_POINT('Ctrl Pts',(-185.883450026306,4.47792624211395,
128.770310560983));
#246214=CARTESIAN_POINT('Ctrl Pts',(-185.89121046882,4.42120925821574,128.645449095676));
#246215=CARTESIAN_POINT('Ctrl Pts',(-185.898970911335,4.35931092585522,
128.52306068839));
#246216=CARTESIAN_POINT('Ctrl Pts',(-185.906731353849,4.29249157078739,
128.403590079339));
#246217=CARTESIAN_POINT('Ctrl Pts',(-185.914504254114,4.22556495135886,
128.28392768546));
#246218=CARTESIAN_POINT('Ctrl Pts',(-185.922277154379,4.15370172825647,
128.167192782885));
#246219=CARTESIAN_POINT('Ctrl Pts',(-185.930050054645,4.07720591501325,
128.053801585463));
#246220=CARTESIAN_POINT('Ctrl Pts',(-185.937540390407,4.00349091726232,
127.944532443683));
#246221=CARTESIAN_POINT('Ctrl Pts',(-185.945030726169,3.92547447684811,
127.838368371698));
#246222=CARTESIAN_POINT('Ctrl Pts',(-185.952521061931,3.84346256241335,
127.73565102006));
#246223=CARTESIAN_POINT('Ctrl Pts',(-185.96029539605,3.75834114131641,127.629039108815));
#246224=CARTESIAN_POINT('Ctrl Pts',(-185.968069730169,3.66864564947082,
127.525802727655));
#246225=CARTESIAN_POINT('Ctrl Pts',(-185.975844064288,3.57467367557063,
127.426359555446));
#246226=CARTESIAN_POINT('Ctrl Pts',(-185.983608817235,3.48081751372976,
127.32703893806));
#246227=CARTESIAN_POINT('Ctrl Pts',(-185.991373570182,3.38269562227221,
127.231502509616));
#246228=CARTESIAN_POINT('Ctrl Pts',(-185.99913832313,3.28064699331261,127.140136502181));
#246229=CARTESIAN_POINT('Ctrl Pts',(-186.006895364015,3.17869972048965,
127.048861240753));
#246230=CARTESIAN_POINT('Ctrl Pts',(-186.0146524049,3.07283376091616,126.961748416427));
#246231=CARTESIAN_POINT('Ctrl Pts',(-186.022409445785,2.96342600063647,
126.879148597655));
#246232=CARTESIAN_POINT('Ctrl Pts',(-186.030160637025,2.85410074559971,
126.79661106805));
#246233=CARTESIAN_POINT('Ctrl Pts',(-186.037911828265,2.74123931688351,
126.718580004569));
#246234=CARTESIAN_POINT('Ctrl Pts',(-186.045663019505,2.6252525518401,126.6453664962));
#246235=CARTESIAN_POINT('Ctrl Pts',(-186.053410916282,2.50931508426635,
126.572184105526));
#246236=CARTESIAN_POINT('Ctrl Pts',(-186.061158813059,2.39025525227261,
126.503815405716));
#246237=CARTESIAN_POINT('Ctrl Pts',(-186.068906709836,2.26851363507625,
126.440528706278));
#246238=CARTESIAN_POINT('Ctrl Pts',(-186.07665298592,2.14679748360143,126.377255245054));
#246239=CARTESIAN_POINT('Ctrl Pts',(-186.084399262004,2.02240100940056,
126.319061849963));
#246240=CARTESIAN_POINT('Ctrl Pts',(-186.092145538088,1.89578984970093,
126.266171120832));
#246241=CARTESIAN_POINT('Ctrl Pts',(-186.099891871354,1.769177755387,126.213280001273));
#246242=CARTESIAN_POINT('Ctrl Pts',(-186.107638204619,1.64035130370563,
126.165691776484));
#246243=CARTESIAN_POINT('Ctrl Pts',(-186.115384537884,1.50979621498143,
126.123580933397));
#246244=CARTESIAN_POINT('Ctrl Pts',(-186.123132605887,1.37921188934978,
126.081460659879));
#246245=CARTESIAN_POINT('Ctrl Pts',(-186.13088067389,1.24689852837551,126.044820328894));
#246246=CARTESIAN_POINT('Ctrl Pts',(-186.138628741893,1.11335672851959,
126.013784466667));
#246247=CARTESIAN_POINT('Ctrl Pts',(-186.146385044635,0.979672998849801,
125.982715619156));
#246248=CARTESIAN_POINT('Ctrl Pts',(-186.154141347377,0.844758603646081,
125.957263227791));
#246249=CARTESIAN_POINT('Ctrl Pts',(-186.161897650119,0.709124593392249,
125.937500708595));
#246250=CARTESIAN_POINT('Ctrl Pts',(-186.169658092633,0.573418191182914,
125.917727641549));
#246251=CARTESIAN_POINT('Ctrl Pts',(-186.177418535147,0.436991797321192,
125.903650537974));
#246252=CARTESIAN_POINT('Ctrl Pts',(-186.185178977661,0.300360296774949,
125.895290771391));
#246253=CARTESIAN_POINT('Ctrl Pts',(-186.192951877927,0.163509463214826,
125.886917584969));
#246254=CARTESIAN_POINT('Ctrl Pts',(-186.200724778192,0.0264532561306669,
125.884280083587));
#246255=CARTESIAN_POINT('Ctrl Pts',(-186.208497678457,-0.110293825237829,
125.887347465803));
#246256=CARTESIAN_POINT('Ctrl Pts',(-186.215988014219,-0.242069805751984,
125.890303340948));
#246257=CARTESIAN_POINT('Ctrl Pts',(-186.223478349981,-0.37355843793483,
125.898556507699));
#246258=CARTESIAN_POINT('Ctrl Pts',(-186.230968685743,-0.504306897976589,
125.91203421644));
#246259=CARTESIAN_POINT('Ctrl Pts',(-186.238743019862,-0.640012725620837,
125.926022936604));
#246260=CARTESIAN_POINT('Ctrl Pts',(-186.246517353981,-0.775351021172049,
125.945684508496));
#246261=CARTESIAN_POINT('Ctrl Pts',(-186.2542916881,-0.909809525613153,
125.970994327949));
#246262=CARTESIAN_POINT('Ctrl Pts',(-186.262056441047,-1.0441023219648,
125.996272955312));
#246263=CARTESIAN_POINT('Ctrl Pts',(-186.269821193994,-1.17751710403923,
126.02718590837));
#246264=CARTESIAN_POINT('Ctrl Pts',(-186.277585946941,-1.3095456903417,
126.063656751323));
#246265=CARTESIAN_POINT('Ctrl Pts',(-186.285342987826,-1.44144314399063,
126.100091370921));
#246266=CARTESIAN_POINT('Ctrl Pts',(-186.293100028711,-1.57195676732722,
126.142072791592));
#246267=CARTESIAN_POINT('Ctrl Pts',(-186.300857069596,-1.7005879010708,
126.189473419245));
#246268=CARTESIAN_POINT('Ctrl Pts',(-186.308608260836,-1.8291220330753,
126.236838301715));
#246269=CARTESIAN_POINT('Ctrl Pts',(-186.316359452076,-1.95577613574888,
126.289614122268));
#246270=CARTESIAN_POINT('Ctrl Pts',(-186.324110643316,-2.08006641349185,
126.347623383));
#246271=CARTESIAN_POINT('Ctrl Pts',(-186.331858540093,-2.20430386455207,
126.40560798825));
#246272=CARTESIAN_POINT('Ctrl Pts',(-186.33960643687,-2.32617913539421,
126.46882144461));
#246273=CARTESIAN_POINT('Ctrl Pts',(-186.347354333647,-2.4452283458019,
126.537038108148));
#246274=CARTESIAN_POINT('Ctrl Pts',(-186.355100609731,-2.56425265368117,
126.605240502231));
#246275=CARTESIAN_POINT('Ctrl Pts',(-186.362846885815,-2.68045173795131,
126.678443827566));
#246276=CARTESIAN_POINT('Ctrl Pts',(-186.370593161899,-2.79338663077894,
126.756376651011));
#246277=CARTESIAN_POINT('Ctrl Pts',(-186.378339495165,-2.90632235726645,
126.834310049738));
#246278=CARTESIAN_POINT('Ctrl Pts',(-186.38608582843,-3.01599352244523,
126.916972794186));
#246279=CARTESIAN_POINT('Ctrl Pts',(-186.393832161695,-3.12199078181559,
127.004050548538));
#246280=CARTESIAN_POINT('Ctrl Pts',(-186.401580229698,-3.2280117785374,
127.091147803349));
#246281=CARTESIAN_POINT('Ctrl Pts',(-186.409328297701,-3.33035693024278,
127.182661787357));
#246282=CARTESIAN_POINT('Ctrl Pts',(-186.417076365704,-3.42865088487751,
127.278238644048));
#246283=CARTESIAN_POINT('Ctrl Pts',(-186.424832668446,-3.52704930749682,
127.373917080959));
#246284=CARTESIAN_POINT('Ctrl Pts',(-186.432588971188,-3.62138765127686,
127.473666743374));
#246285=CARTESIAN_POINT('Ctrl Pts',(-186.440345273929,-3.71132791396644,
127.577097353202));
#246286=CARTESIAN_POINT('Ctrl Pts',(-186.448105716444,-3.8013161804825,
127.680583167061));
#246287=CARTESIAN_POINT('Ctrl Pts',(-186.455866158958,-3.8869014446861,
127.787753537677));
#246288=CARTESIAN_POINT('Ctrl Pts',(-186.463626601472,-3.96778741652845,
127.898186830653));
#246289=CARTESIAN_POINT('Ctrl Pts',(-186.471399501737,-4.04880323371331,
128.008797400955));
#246290=CARTESIAN_POINT('Ctrl Pts',(-186.479172402003,-4.12510446603694,
128.122681035685));
#246291=CARTESIAN_POINT('Ctrl Pts',(-186.486945302268,-4.19643892821958,
128.239388223129));
#246292=CARTESIAN_POINT('Ctrl Pts',(-186.494435638031,-4.26518020302876,
128.351852810354));
#246293=CARTESIAN_POINT('Ctrl Pts',(-186.501925973793,-4.32930939758988,
128.466938958798));
#246294=CARTESIAN_POINT('Ctrl Pts',(-186.509416309556,-4.38864295588559,
128.584226372018));
#246295=CARTESIAN_POINT('Ctrl Pts',(-186.517717331537,-4.45439824205773,
128.714207914373));
#246296=CARTESIAN_POINT('Ctrl Pts',(-186.526018353518,-4.51445011624346,
128.847261066043));
#246297=CARTESIAN_POINT('Ctrl Pts',(-186.534319375498,-4.56852078633726,
128.982877461645));
#246298=CARTESIAN_POINT('Ctrl Pts',(-186.542600349557,-4.62246086954897,
129.118166328066));
#246299=CARTESIAN_POINT('Ctrl Pts',(-186.550881323616,-4.670448438029,129.256005807444));
#246300=CARTESIAN_POINT('Ctrl Pts',(-186.559162297674,-4.71225244919594,
129.39586499544));
#246301=CARTESIAN_POINT('Ctrl Pts',(-186.562823196869,-4.73073339959214,
129.45769472526));
#246302=CARTESIAN_POINT('Ctrl Pts',(-186.566484096064,-4.74800643982495,
129.519918866165));
#246303=CARTESIAN_POINT('Ctrl Pts',(-186.570144995258,-4.76405452823391,
129.582490119308));
#246304=CARTESIAN_POINT('Ctrl Pts',(-184.819837330039,-4.76405452823405,
129.582490119308));
#246305=CARTESIAN_POINT('Ctrl Pts',(-184.826135075586,-4.79157558581711,
129.689794305134));
#246306=CARTESIAN_POINT('Ctrl Pts',(-184.832432821132,-4.8154390765796,
129.797910017712));
#246307=CARTESIAN_POINT('Ctrl Pts',(-184.838730566679,-4.83561259437176,
129.906566710451));
#246308=CARTESIAN_POINT('Ctrl Pts',(-184.850410110173,-4.87302558235891,
130.108077006377));
#246309=CARTESIAN_POINT('Ctrl Pts',(-184.862089653666,-4.89785094753426,
130.311991589822));
#246310=CARTESIAN_POINT('Ctrl Pts',(-184.87376919716,-4.90985019127264,
130.517038217186));
#246311=CARTESIAN_POINT('Ctrl Pts',(-184.879132610105,-4.91536041512924,
130.611198552825));
#246312=CARTESIAN_POINT('Ctrl Pts',(-184.88449602305,-4.9181664561817,130.705597270812));
#246313=CARTESIAN_POINT('Ctrl Pts',(-184.889859435995,-4.9182481621147,
130.800108752638));
#246314=CARTESIAN_POINT('Origin',(213.235140564004,0.,130.804360617566));
#246315=CARTESIAN_POINT('',(-183.069718605797,-4.76405452823406,129.582490119308));
#246316=CARTESIAN_POINT('',(-183.415149158805,-4.76405452823414,129.582490119309));
#246317=CARTESIAN_POINT('',(213.235140564004,-4.76405452823405,129.582490119308));
#246318=CARTESIAN_POINT('',(-183.485140564052,-4.91824798071509,130.799903859564));
#246319=CARTESIAN_POINT('Ctrl Pts',(-183.415149158805,-4.76405452823414,
129.582490119309));
#246320=CARTESIAN_POINT('Ctrl Pts',(-183.419067256354,-4.78116185622988,
129.649191331524));
#246321=CARTESIAN_POINT('Ctrl Pts',(-183.422985353904,-4.79685563415493,
129.716203290357));
#246322=CARTESIAN_POINT('Ctrl Pts',(-183.426903451454,-4.81112741488386,
129.783460984765));
#246323=CARTESIAN_POINT('Ctrl Pts',(-183.437819003722,-4.85088762159933,
129.970836329416));
#246324=CARTESIAN_POINT('Ctrl Pts',(-183.448734555991,-4.87971282541858,
130.160606736013));
#246325=CARTESIAN_POINT('Ctrl Pts',(-183.459650108259,-4.89737607248764,
130.351712114724));
#246326=CARTESIAN_POINT('Ctrl Pts',(-183.468146926843,-4.91112539109944,
130.500471214907));
#246327=CARTESIAN_POINT('Ctrl Pts',(-183.476643745428,-4.91811217802289,
130.650039045172));
#246328=CARTESIAN_POINT('Ctrl Pts',(-183.485140564012,-4.91824798071445,
130.799903858857));
#246329=CARTESIAN_POINT('Ctrl Pts',(-183.485140564052,-4.91824798071509,
130.799903859564));
#246330=CARTESIAN_POINT('Ctrl Pts',(-183.492790120517,-4.91837024179223,
130.934824870645));
#246331=CARTESIAN_POINT('Ctrl Pts',(-183.500439676982,-4.91293645195532,
131.069920615074));
#246332=CARTESIAN_POINT('Ctrl Pts',(-183.508089233447,-4.90193026440357,
131.204688914623));
#246333=CARTESIAN_POINT('Ctrl Pts',(-183.515732635828,-4.89093293135145,
131.339348792808));
#246334=CARTESIAN_POINT('Ctrl Pts',(-183.52337603821,-4.8743721510898,131.473681350422));
#246335=CARTESIAN_POINT('Ctrl Pts',(-183.531019440591,-4.85228364227142,
131.607184706296));
#246336=CARTESIAN_POINT('Ctrl Pts',(-183.538659228572,-4.83020557863537,
131.740624931294));
#246337=CARTESIAN_POINT('Ctrl Pts',(-183.546299016552,-4.80260504893871,
131.873236337474));
#246338=CARTESIAN_POINT('Ctrl Pts',(-183.553938804532,-4.76956954354201,
132.004522869854));
#246339=CARTESIAN_POINT('Ctrl Pts',(-183.561576868312,-4.73654149382951,
132.135779772569));
#246340=CARTESIAN_POINT('Ctrl Pts',(-183.569214932091,-4.69808100518792,
132.265712005344));
#246341=CARTESIAN_POINT('Ctrl Pts',(-183.576852995871,-4.65432642489983,
132.393834930973));
#246342=CARTESIAN_POINT('Ctrl Pts',(-183.584491098882,-4.6105716198721,
132.521958514688));
#246343=CARTESIAN_POINT('Ctrl Pts',(-183.592129201894,-4.56152279959267,
132.648272391449));
#246344=CARTESIAN_POINT('Ctrl Pts',(-183.599767304905,-4.50736762758277,
132.772308821234));
#246345=CARTESIAN_POINT('Ctrl Pts',(-183.607407210404,-4.45319967569707,
132.89637452191));
#246346=CARTESIAN_POINT('Ctrl Pts',(-183.615047115903,-4.39392313754426,
133.018161337874));
#246347=CARTESIAN_POINT('Ctrl Pts',(-183.622687021401,-4.32977284733201,
133.137223698205));
#246348=CARTESIAN_POINT('Ctrl Pts',(-183.63033486744,-4.26555588247997,
133.256409806066));
#246349=CARTESIAN_POINT('Ctrl Pts',(-183.637982713479,-4.19645524369809,
133.372865449847));
#246350=CARTESIAN_POINT('Ctrl Pts',(-183.645630559517,-4.12275070500498,
133.486171514494));
#246351=CARTESIAN_POINT('Ctrl Pts',(-183.653282768779,-4.04900411665295,
133.599542222126));
#246352=CARTESIAN_POINT('Ctrl Pts',(-183.66093497804,-3.97064863261913,
133.709759445809));
#246353=CARTESIAN_POINT('Ctrl Pts',(-183.668587187302,-3.8880051776028,
133.816436114866));
#246354=CARTESIAN_POINT('Ctrl Pts',(-183.676250761655,-3.80523898019318,
133.923271220542));
#246355=CARTESIAN_POINT('Ctrl Pts',(-183.683914336009,-3.71817235596996,
134.026554965782));
#246356=CARTESIAN_POINT('Ctrl Pts',(-183.691577910362,-3.62716431972376,
134.125935855344));
#246357=CARTESIAN_POINT('Ctrl Pts',(-183.696168965331,-3.5726436903536,
134.1854724509));
#246358=CARTESIAN_POINT('Ctrl Pts',(-183.700760020299,-3.51670920889025,
134.243609084722));
#246359=CARTESIAN_POINT('Ctrl Pts',(-183.705351075268,-3.45944366050394,
134.300277181544));
#246360=CARTESIAN_POINT('Ctrl Pts',(-183.713125409387,-3.36247215619332,
134.396236981985));
#246361=CARTESIAN_POINT('Ctrl Pts',(-183.720899743506,-3.26135135780418,
134.488310951084));
#246362=CARTESIAN_POINT('Ctrl Pts',(-183.728674077625,-3.15642552453558,
134.57611895693));
#246363=CARTESIAN_POINT('Ctrl Pts',(-183.736438830572,-3.05162900297956,
134.663818747256));
#246364=CARTESIAN_POINT('Ctrl Pts',(-183.744203583519,-2.94303707393275,
134.74726278652));
#246365=CARTESIAN_POINT('Ctrl Pts',(-183.751968336466,-2.83103145099696,
134.826107002654));
#246366=CARTESIAN_POINT('Ctrl Pts',(-183.759725377351,-2.71913707362488,
134.9048729096));
#246367=CARTESIAN_POINT('Ctrl Pts',(-183.767482418236,-2.60383606730024,
134.979047861564));
#246368=CARTESIAN_POINT('Ctrl Pts',(-183.775239459121,-2.48554362280428,
135.048327625171));
#246369=CARTESIAN_POINT('Ctrl Pts',(-183.782990650361,-2.36734038356073,
135.117555144369));
#246370=CARTESIAN_POINT('Ctrl Pts',(-183.790741841601,-2.24615053231144,
135.181894626134));
#246371=CARTESIAN_POINT('Ctrl Pts',(-183.798493032841,-2.12241837636851,
135.241085005913));
#246372=CARTESIAN_POINT('Ctrl Pts',(-183.806240929618,-1.99873880989235,
135.300250228202));
#246373=CARTESIAN_POINT('Ctrl Pts',(-183.813988826396,-1.87251943979781,
135.354270532912));
#246374=CARTESIAN_POINT('Ctrl Pts',(-183.821736723173,-1.7442291244233,
135.402930811008));
#246375=CARTESIAN_POINT('Ctrl Pts',(-183.829482999257,-1.61596564461714,
135.451580910423));
#246376=CARTESIAN_POINT('Ctrl Pts',(-183.837229275341,-1.48563244650519,
135.494873074791));
#246377=CARTESIAN_POINT('Ctrl Pts',(-183.844975551425,-1.35371794589048,
135.532640514682));
#246378=CARTESIAN_POINT('Ctrl Pts',(-183.85272188469,-1.22180247151308,
135.570408233365));
#246379=CARTESIAN_POINT('Ctrl Pts',(-183.860468217956,-1.08830604720463,
135.602651038582));
#246380=CARTESIAN_POINT('Ctrl Pts',(-183.868214551221,-0.953731425044513,
135.62925226727));
#246381=CARTESIAN_POINT('Ctrl Pts',(-183.875962619224,-0.81912666583066,
135.655859453118));
#246382=CARTESIAN_POINT('Ctrl Pts',(-183.883710687227,-0.683443611768262,
135.676822472633));
#246383=CARTESIAN_POINT('Ctrl Pts',(-183.89145875523,-0.547193964316623,
135.69207601721));
#246384=CARTESIAN_POINT('Ctrl Pts',(-183.899215057972,-0.410799509118467,
135.707345773435));
#246385=CARTESIAN_POINT('Ctrl Pts',(-183.906971360713,-0.273837646764738,
135.716893889475));
#246386=CARTESIAN_POINT('Ctrl Pts',(-183.914727663455,-0.136824502115776,
135.720707037228));
#246387=CARTESIAN_POINT('Ctrl Pts',(-183.922488105969,0.000261770573871722,
135.724522220172));
#246388=CARTESIAN_POINT('Ctrl Pts',(-183.930248548483,0.137398989362215,
135.722596341163));
#246389=CARTESIAN_POINT('Ctrl Pts',(-183.938008990998,0.274073289081115,
135.714968206726));
#246390=CARTESIAN_POINT('Ctrl Pts',(-183.945781891263,0.410966990519299,
135.70732782693));
#246391=CARTESIAN_POINT('Ctrl Pts',(-183.953554791528,0.547395898572235,
135.693966937693));
#246392=CARTESIAN_POINT('Ctrl Pts',(-183.961327691794,0.682852614635353,
135.674976119655));
#246393=CARTESIAN_POINT('Ctrl Pts',(-183.968818027556,0.813385137877262,
135.656675665687));
#246394=CARTESIAN_POINT('Ctrl Pts',(-183.976308363318,0.943014622152609,
135.633147555643));
#246395=CARTESIAN_POINT('Ctrl Pts',(-183.98379869908,1.07129981466353,135.604516841024));
#246396=CARTESIAN_POINT('Ctrl Pts',(-183.991573033199,1.20444897923751,
135.574800584158));
#246397=CARTESIAN_POINT('Ctrl Pts',(-183.999347367318,1.3365716786525,135.539493021914));
#246398=CARTESIAN_POINT('Ctrl Pts',(-184.007121701437,1.46716201666007,
135.49867831872));
#246399=CARTESIAN_POINT('Ctrl Pts',(-184.014886454385,1.5975914137469,135.457913916001));
#246400=CARTESIAN_POINT('Ctrl Pts',(-184.022651207332,1.72649183739355,
135.411655992067));
#246401=CARTESIAN_POINT('Ctrl Pts',(-184.030415960279,1.85336748449725,
135.360039714024));
#246402=CARTESIAN_POINT('Ctrl Pts',(-184.038173001164,1.98011711691926,
135.308474701997));
#246403=CARTESIAN_POINT('Ctrl Pts',(-184.045930042049,2.10484561505189,
135.251562073242));
#246404=CARTESIAN_POINT('Ctrl Pts',(-184.053687082934,2.22707259798284,
135.189486693954));
#246405=CARTESIAN_POINT('Ctrl Pts',(-184.061438274174,2.34920740859568,
135.127458126191));
#246406=CARTESIAN_POINT('Ctrl Pts',(-184.069189465414,2.46884411162038,
135.060274733533));
#246407=CARTESIAN_POINT('Ctrl Pts',(-184.076940656654,2.58552290710035,
134.988169212538));
#246408=CARTESIAN_POINT('Ctrl Pts',(-184.084688553431,2.70215211097956,
134.916094338312));
#246409=CARTESIAN_POINT('Ctrl Pts',(-184.092436450208,2.81582557588218,
134.839101701749));
#246410=CARTESIAN_POINT('Ctrl Pts',(-184.100184346985,2.92610889510012,
134.757469494958));
#246411=CARTESIAN_POINT('Ctrl Pts',(-184.107930623069,3.03636914542542,
134.675854363865));
#246412=CARTESIAN_POINT('Ctrl Pts',(-184.115676899153,3.14324034655068,
134.589601825376));
#246413=CARTESIAN_POINT('Ctrl Pts',(-184.123423175237,3.24631817313421,
134.499032643779));
#246414=CARTESIAN_POINT('Ctrl Pts',(-184.131169508503,3.34939676061442,
134.40846279362));
#246415=CARTESIAN_POINT('Ctrl Pts',(-184.138915841768,3.44868162397767,
134.313576494829));
#246416=CARTESIAN_POINT('Ctrl Pts',(-184.146662175034,3.54380286150397,
134.214733667732));
#246417=CARTESIAN_POINT('Ctrl Pts',(-184.154410243036,3.63894540077176,
134.115868705469));
#246418=CARTESIAN_POINT('Ctrl Pts',(-184.162158311039,3.72992218775639,
134.013045733441));
#246419=CARTESIAN_POINT('Ctrl Pts',(-184.169906379042,3.81640168934142,
133.906659959682));
#246420=CARTESIAN_POINT('Ctrl Pts',(-184.177662681784,3.90297310236997,
133.800161117856));
#246421=CARTESIAN_POINT('Ctrl Pts',(-184.185418984526,3.98503743489305,
133.690092214043));
#246422=CARTESIAN_POINT('Ctrl Pts',(-184.193175287268,4.06230449550591,
133.576880274537));
#246423=CARTESIAN_POINT('Ctrl Pts',(-184.200935729782,4.13961279587571,
133.463607910411));
#246424=CARTESIAN_POINT('Ctrl Pts',(-184.208696172296,4.21211851583949,
133.34718949967));
#246425=CARTESIAN_POINT('Ctrl Pts',(-184.21645661481,4.27957654775137,133.228078347508));
#246426=CARTESIAN_POINT('Ctrl Pts',(-184.224229515076,4.34714286928472,
133.108775987551));
#246427=CARTESIAN_POINT('Ctrl Pts',(-184.232002415341,4.40964513203329,
132.986772596348));
#246428=CARTESIAN_POINT('Ctrl Pts',(-184.239775315607,4.46688528271646,
132.862544023765));
#246429=CARTESIAN_POINT('Ctrl Pts',(-184.247265651369,4.52204460974522,
132.742831472703));
#246430=CARTESIAN_POINT('Ctrl Pts',(-184.254755987131,4.57231764704277,
132.621052998097));
#246431=CARTESIAN_POINT('Ctrl Pts',(-184.262246322894,4.61757109606277,
132.497647431814));
#246432=CARTESIAN_POINT('Ctrl Pts',(-184.270020657013,4.66454034335519,
132.369562905981));
#246433=CARTESIAN_POINT('Ctrl Pts',(-184.277794991132,4.70625063758659,
132.239319737225));
#246434=CARTESIAN_POINT('Ctrl Pts',(-184.285569325251,4.74249933939709,
132.107389043318));
#246435=CARTESIAN_POINT('Ctrl Pts',(-184.293334078198,4.77870336792206,
131.975620942201));
#246436=CARTESIAN_POINT('Ctrl Pts',(-184.301098831145,4.80945909397288,
131.842169827338));
#246437=CARTESIAN_POINT('Ctrl Pts',(-184.308863584092,4.83461224377596,
131.707525893045));
#246438=CARTESIAN_POINT('Ctrl Pts',(-184.316620624977,4.85974041111613,
131.573015689005));
#246439=CARTESIAN_POINT('Ctrl Pts',(-184.324377665862,4.87927700459897,
131.437315405021));
#246440=CARTESIAN_POINT('Ctrl Pts',(-184.332134706747,4.89311789977162,
131.300929123851));
#246441=CARTESIAN_POINT('Ctrl Pts',(-184.339885897987,4.9069483574176,131.164645692637));
#246442=CARTESIAN_POINT('Ctrl Pts',(-184.347637089227,4.91509162671567,
131.027677681317));
#246443=CARTESIAN_POINT('Ctrl Pts',(-184.355388280468,4.91749494876237,
130.89053771079));
#246444=CARTESIAN_POINT('Ctrl Pts',(-184.363136177245,4.91989724933307,
130.75345602841));
#246445=CARTESIAN_POINT('Ctrl Pts',(-184.370884074022,4.9165644480558,130.616202922275));
#246446=CARTESIAN_POINT('Ctrl Pts',(-184.378631970799,4.90749578839558,
130.479294240683));
#246447=CARTESIAN_POINT('Ctrl Pts',(-184.386378246883,4.89842902570346,
130.342414197436));
#246448=CARTESIAN_POINT('Ctrl Pts',(-184.394124522967,4.88362881695607,
130.205878825291));
#246449=CARTESIAN_POINT('Ctrl Pts',(-184.401870799051,4.86314648250967,
130.070201675542));
#246450=CARTESIAN_POINT('Ctrl Pts',(-184.409617132316,4.84266399686724,
129.934523524254));
#246451=CARTESIAN_POINT('Ctrl Pts',(-184.417363465582,4.81649936018953,
129.799703994589));
#246452=CARTESIAN_POINT('Ctrl Pts',(-184.425109798847,4.78475544272591,
129.666248841067));
#246453=CARTESIAN_POINT('Ctrl Pts',(-184.43285786685,4.75300441643203,129.532763801189));
#246454=CARTESIAN_POINT('Ctrl Pts',(-184.440605934853,4.7156717135631,129.400644125729));
#246455=CARTESIAN_POINT('Ctrl Pts',(-184.448354002856,4.67291063208325,
129.270382362484));
#246456=CARTESIAN_POINT('Ctrl Pts',(-184.456110305598,4.6301041036172,129.139982155487));
#246457=CARTESIAN_POINT('Ctrl Pts',(-184.46386660834,4.58185779378596,129.011444177258));
#246458=CARTESIAN_POINT('Ctrl Pts',(-184.471622911082,4.52837411636472,
128.885243392189));
#246459=CARTESIAN_POINT('Ctrl Pts',(-184.479383353596,4.47486189309462,
128.758975249962));
#246460=CARTESIAN_POINT('Ctrl Pts',(-184.48714379611,4.41610689968782,128.635047139604));
#246461=CARTESIAN_POINT('Ctrl Pts',(-184.494904238624,4.35235802797307,
128.513910299651));
#246462=CARTESIAN_POINT('Ctrl Pts',(-184.50267713889,4.28850682091009,128.392579000088));
#246463=CARTESIAN_POINT('Ctrl Pts',(-184.510450039155,4.21964591229296,
128.274048263238));
#246464=CARTESIAN_POINT('Ctrl Pts',(-184.518222939421,4.14606859545448,
128.15874192541));
#246465=CARTESIAN_POINT('Ctrl Pts',(-184.525713275183,4.07516599941415,
128.047627263403));
#246466=CARTESIAN_POINT('Ctrl Pts',(-184.533203610945,3.99988412443292,
127.939506893194));
#246467=CARTESIAN_POINT('Ctrl Pts',(-184.540693946706,3.92052012106803,
127.83473016197));
#246468=CARTESIAN_POINT('Ctrl Pts',(-184.548468280826,3.83814700739212,
127.725980789134));
#246469=CARTESIAN_POINT('Ctrl Pts',(-184.556242614945,3.75111517370212,
127.620489123221));
#246470=CARTESIAN_POINT('Ctrl Pts',(-184.564016949064,3.65971145319893,
127.518680301129));
#246471=CARTESIAN_POINT('Ctrl Pts',(-184.571781702011,3.56842037961253,
127.41699694931));
#246472=CARTESIAN_POINT('Ctrl Pts',(-184.579546454958,3.47276839832737,
127.318987698628));
#246473=CARTESIAN_POINT('Ctrl Pts',(-184.587311207905,3.37308453496028,
127.225047305978));
#246474=CARTESIAN_POINT('Ctrl Pts',(-184.59506824879,3.27349967901132,127.13120021625));
#246475=CARTESIAN_POINT('Ctrl Pts',(-184.602825289675,3.16989119284842,
127.04141420869));
#246476=CARTESIAN_POINT('Ctrl Pts',(-184.61058233056,3.06262689376355,126.956049355194));
#246477=CARTESIAN_POINT('Ctrl Pts',(-184.6183335218,2.95544348352117,126.870748875999));
#246478=CARTESIAN_POINT('Ctrl Pts',(-184.62608471304,2.84461005242828,126.789863157161));
#246479=CARTESIAN_POINT('Ctrl Pts',(-184.63383590428,2.73052936548945,126.713713670358));
#246480=CARTESIAN_POINT('Ctrl Pts',(-184.641583801057,2.61649716588561,
126.637596549119));
#246481=CARTESIAN_POINT('Ctrl Pts',(-184.649331697835,2.49922077998541,
126.566211872763));
#246482=CARTESIAN_POINT('Ctrl Pts',(-184.657079594612,2.37913379664567,
126.499839106392));
#246483=CARTESIAN_POINT('Ctrl Pts',(-184.664825870696,2.25907193291407,
126.433480223773));
#246484=CARTESIAN_POINT('Ctrl Pts',(-184.67257214678,2.13620098310233,126.372131354849));
#246485=CARTESIAN_POINT('Ctrl Pts',(-184.680318422864,2.01098075236442,
126.316026909371));
#246486=CARTESIAN_POINT('Ctrl Pts',(-184.688064756129,1.88575959727938,
126.259922049742));
#246487=CARTESIAN_POINT('Ctrl Pts',(-184.695811089395,1.75818948345372,
126.209061850666));
#246488=CARTESIAN_POINT('Ctrl Pts',(-184.70355742266,1.62875152037251,126.163633137161));
#246489=CARTESIAN_POINT('Ctrl Pts',(-184.711305490663,1.49928457055711,
126.118194250211));
#246490=CARTESIAN_POINT('Ctrl Pts',(-184.719053558666,1.36794930796729,
126.078189398663));
#246491=CARTESIAN_POINT('Ctrl Pts',(-184.726801626669,1.23524298830775,
126.043755842715));
#246492=CARTESIAN_POINT('Ctrl Pts',(-184.734557929411,1.10239562679191,
126.009285690373));
#246493=CARTESIAN_POINT('Ctrl Pts',(-184.742314232153,0.968174676377767,
125.980398760293));
#246494=CARTESIAN_POINT('Ctrl Pts',(-184.750070534895,0.833089147649478,
125.957181485889));
#246495=CARTESIAN_POINT('Ctrl Pts',(-184.757830977409,0.697931519707528,
125.933951819726));
#246496=CARTESIAN_POINT('Ctrl Pts',(-184.765591419923,0.561908781530276,
125.916397888946));
#246497=CARTESIAN_POINT('Ctrl Pts',(-184.773351862437,0.425535104989546,
125.904554199255));
#246498=CARTESIAN_POINT('Ctrl Pts',(-184.781124762703,0.288942509316547,
125.892691497022));
#246499=CARTESIAN_POINT('Ctrl Pts',(-184.788897662968,0.1519982403108,125.886557371142));
#246500=CARTESIAN_POINT('Ctrl Pts',(-184.796670563234,0.0152174156738462,
125.886134159506));
#246501=CARTESIAN_POINT('Ctrl Pts',(-184.804160898996,-0.116591081455591,
125.885726332679));
#246502=CARTESIAN_POINT('Ctrl Pts',(-184.811651234757,-0.248247503329108,
125.89062140511));
#246503=CARTESIAN_POINT('Ctrl Pts',(-184.819141570519,-0.379297317131378,
125.900758206306));
#246504=CARTESIAN_POINT('Ctrl Pts',(-184.826915904638,-0.515315924457791,
125.9112793474));
#246505=CARTESIAN_POINT('Ctrl Pts',(-184.834690238758,-0.651111882649554,
125.92748087175));
#246506=CARTESIAN_POINT('Ctrl Pts',(-184.842464572877,-0.786172471644022,
125.949351255337));
#246507=CARTESIAN_POINT('Ctrl Pts',(-184.850229325824,-0.921066610532533,
125.971194685631));
#246508=CARTESIAN_POINT('Ctrl Pts',(-184.857994078771,-1.05522680121144,
125.998693012488));
#246509=CARTESIAN_POINT('Ctrl Pts',(-184.865758831718,-1.18814307714153,
126.031782793084));
#246510=CARTESIAN_POINT('Ctrl Pts',(-184.873515872603,-1.3209273387533,
126.064839708443));
#246511=CARTESIAN_POINT('Ctrl Pts',(-184.881272913488,-1.45246976733426,
126.103476931965));
#246512=CARTESIAN_POINT('Ctrl Pts',(-184.889029954373,-1.58226860997003,
126.147579636201));
#246513=CARTESIAN_POINT('Ctrl Pts',(-184.896781145613,-1.71196957028905,
126.191649082245));
#246514=CARTESIAN_POINT('Ctrl Pts',(-184.904532336853,-1.83992919311302,
126.241175680014));
#246515=CARTESIAN_POINT('Ctrl Pts',(-184.912283528093,-1.96565931089237,
126.295994335197));
#246516=CARTESIAN_POINT('Ctrl Pts',(-184.92003142487,-2.09133599001719,
126.350789690989));
#246517=CARTESIAN_POINT('Ctrl Pts',(-184.927779321648,-2.21478469116771,
126.410872474649));
#246518=CARTESIAN_POINT('Ctrl Pts',(-184.935527218425,-2.33553592707272,
126.476028953304));
#246519=CARTESIAN_POINT('Ctrl Pts',(-184.943273494509,-2.45626190442228,
126.541171802628));
#246520=CARTESIAN_POINT('Ctrl Pts',(-184.951019770593,-2.57429119500066,
126.611386050408));
#246521=CARTESIAN_POINT('Ctrl Pts',(-184.958766046677,-2.68917804732998,
126.686411553741));
#246522=CARTESIAN_POINT('Ctrl Pts',(-184.966512379942,-2.8040657477281,
126.761437610895));
#246523=CARTESIAN_POINT('Ctrl Pts',(-184.974258713208,-2.9158106362426,
126.8412747807));
#246524=CARTESIAN_POINT('Ctrl Pts',(-184.982005046473,-3.02399548026597,
126.925619275606));
#246525=CARTESIAN_POINT('Ctrl Pts',(-184.989753114476,-3.1322045515355,
127.009982658877));
#246526=CARTESIAN_POINT('Ctrl Pts',(-184.997501182479,-3.2368516836113,
127.098855135468));
#246527=CARTESIAN_POINT('Ctrl Pts',(-185.005249250482,-3.33755261674843,
127.19189254256));
#246528=CARTESIAN_POINT('Ctrl Pts',(-185.013005553224,-3.43836057603525,
127.285028830915));
#246529=CARTESIAN_POINT('Ctrl Pts',(-185.020761855966,-3.53521367065951,
127.382338626523));
#246530=CARTESIAN_POINT('Ctrl Pts',(-185.028518158708,-3.62776404908838,
127.483440403733));
#246531=CARTESIAN_POINT('Ctrl Pts',(-185.036278601222,-3.72036382444085,
127.584596142007));
#246532=CARTESIAN_POINT('Ctrl Pts',(-185.044039043736,-3.80865605608395,
127.689547595635));
#246533=CARTESIAN_POINT('Ctrl Pts',(-185.05179948625,-3.89233379093432,
127.797880828435));
#246534=CARTESIAN_POINT('Ctrl Pts',(-185.059572386516,-3.976145852713,127.906387967359));
#246535=CARTESIAN_POINT('Ctrl Pts',(-185.067345286781,-4.05532838899046,
128.018287414464));
#246536=CARTESIAN_POINT('Ctrl Pts',(-185.075118187046,-4.12961782569921,
128.133136239838));
#246537=CARTESIAN_POINT('Ctrl Pts',(-185.082608522808,-4.20120665425939,
128.243810021123));
#246538=CARTESIAN_POINT('Ctrl Pts',(-185.09009885857,-4.26825180309765,
128.357222203767));
#246539=CARTESIAN_POINT('Ctrl Pts',(-185.097589194332,-4.33055905059273,
128.472957312295));
#246540=CARTESIAN_POINT('Ctrl Pts',(-185.10578677954,-4.39874944774409,
128.599620314307));
#246541=CARTESIAN_POINT('Ctrl Pts',(-185.113984364748,-4.46146195184884,
128.729431206875));
#246542=CARTESIAN_POINT('Ctrl Pts',(-185.122181949956,-4.51841101832934,
128.86190214132));
#246543=CARTESIAN_POINT('Ctrl Pts',(-185.130360998453,-4.57523130928227,
128.994073527142));
#246544=CARTESIAN_POINT('Ctrl Pts',(-185.13854004695,-4.62631401768098,
129.128892662092));
#246545=CARTESIAN_POINT('Ctrl Pts',(-185.146719095448,-4.6714196002999,
129.265847705552));
#246546=CARTESIAN_POINT('Ctrl Pts',(-185.152953088293,-4.70579864566502,
129.370233534949));
#246547=CARTESIAN_POINT('Ctrl Pts',(-185.159187081138,-4.73670625024354,
129.475859598491));
#246548=CARTESIAN_POINT('Ctrl Pts',(-185.165421073984,-4.76405452823401,
129.582490119308));
#246549=CARTESIAN_POINT('',(-183.139859435957,-4.91824917715616,130.807205596086));
#246550=CARTESIAN_POINT('Ctrl Pts',(-183.139859435995,-4.91824917715577,
130.807205596751));
#246551=CARTESIAN_POINT('Ctrl Pts',(-183.149254565264,-4.91815366403183,
130.972323621388));
#246552=CARTESIAN_POINT('Ctrl Pts',(-183.158649694533,-4.90974370090652,
131.137198293807));
#246553=CARTESIAN_POINT('Ctrl Pts',(-183.168044823802,-4.89308820514277,
131.301221643601));
#246554=CARTESIAN_POINT('Ctrl Pts',(-183.175819157921,-4.87930602234573,
131.436948602553));
#246555=CARTESIAN_POINT('Ctrl Pts',(-183.18359349204,-4.85985043506831,
131.572316662951));
#246556=CARTESIAN_POINT('Ctrl Pts',(-183.191367826159,-4.83474526787819,
131.70681352893));
#246557=CARTESIAN_POINT('Ctrl Pts',(-183.199132579106,-4.80967104056291,
131.841144639542));
#246558=CARTESIAN_POINT('Ctrl Pts',(-183.206897332053,-4.77896115788808,
131.974606311377));
#246559=CARTESIAN_POINT('Ctrl Pts',(-183.214662085,-4.74269128219991,132.106690247209));
#246560=CARTESIAN_POINT('Ctrl Pts',(-183.222419125885,-4.70645743026349,
132.238642995413));
#246561=CARTESIAN_POINT('Ctrl Pts',(-183.23017616677,-4.664674677723,132.369220356194));
#246562=CARTESIAN_POINT('Ctrl Pts',(-183.237933207655,-4.61746985964742,
132.497923476673));
#246563=CARTESIAN_POINT('Ctrl Pts',(-183.245684398895,-4.57030063909242,
132.626529541128));
#246564=CARTESIAN_POINT('Ctrl Pts',(-183.253435590136,-4.5177176256354,
132.753263812955));
#246565=CARTESIAN_POINT('Ctrl Pts',(-183.261186781376,-4.45989758071983,
132.877642226993));
#246566=CARTESIAN_POINT('Ctrl Pts',(-183.268934678153,-4.40210211086567,
133.001967776888));
#246567=CARTESIAN_POINT('Ctrl Pts',(-183.27668257493,-4.33907420112053,
133.123939106722));
#246568=CARTESIAN_POINT('Ctrl Pts',(-183.284430471707,-4.27103878920714,
133.243091993423));
#246569=CARTESIAN_POINT('Ctrl Pts',(-183.292176747791,-4.20301760883524,
133.362219955909));
#246570=CARTESIAN_POINT('Ctrl Pts',(-183.299923023875,-4.12999120349208,
133.478530308623));
#246571=CARTESIAN_POINT('Ctrl Pts',(-183.307669299959,-4.05223033797251,
133.591583671165));
#246572=CARTESIAN_POINT('Ctrl Pts',(-183.315415633224,-3.97446889844,133.704637868242));
#246573=CARTESIAN_POINT('Ctrl Pts',(-183.32316196649,-3.89197315055749,
133.814434705049));
#246574=CARTESIAN_POINT('Ctrl Pts',(-183.330908299755,-3.80505680682347,
133.920564359196));
#246575=CARTESIAN_POINT('Ctrl Pts',(-183.338656367758,-3.7181209987768,
134.026717780342));
#246576=CARTESIAN_POINT('Ctrl Pts',(-183.346404435761,-3.62676287263744,
134.129202082239));
#246577=CARTESIAN_POINT('Ctrl Pts',(-183.354152503764,-3.53133571328797,
134.227641374757));
#246578=CARTESIAN_POINT('Ctrl Pts',(-183.361908806506,-3.43580713281808,
134.326185289727));
#246579=CARTESIAN_POINT('Ctrl Pts',(-183.369665109248,-3.33620115280986,
134.420675326271));
#246580=CARTESIAN_POINT('Ctrl Pts',(-183.37742141199,-3.23290753652007,
134.510772888592));
#246581=CARTESIAN_POINT('Ctrl Pts',(-183.385181854504,-3.12955878931717,
134.600918538695));
#246582=CARTESIAN_POINT('Ctrl Pts',(-183.392942297018,-3.02251878900405,
134.686666798853));
#246583=CARTESIAN_POINT('Ctrl Pts',(-183.400702739532,-2.91220871858613,
134.767720737703));
#246584=CARTESIAN_POINT('Ctrl Pts',(-183.408475639798,-2.80172156865031,
134.848904791531));
#246585=CARTESIAN_POINT('Ctrl Pts',(-183.416248540063,-2.68795418328053,
134.925379247005));
#246586=CARTESIAN_POINT('Ctrl Pts',(-183.424021440328,-2.57135568988743,
134.996891235055));
#246587=CARTESIAN_POINT('Ctrl Pts',(-183.43151177609,-2.45899584542431,
135.065803582211));
#246588=CARTESIAN_POINT('Ctrl Pts',(-183.439002111852,-2.34400742397867,
135.130107844031));
#246589=CARTESIAN_POINT('Ctrl Pts',(-183.446492447614,-2.22681044216329,
135.18961982509));
#246590=CARTESIAN_POINT('Ctrl Pts',(-183.454266781733,-2.1051699011596,
135.251388221));
#246591=CARTESIAN_POINT('Ctrl Pts',(-183.462041115852,-1.98076469797066,
135.308189427607));
#246592=CARTESIAN_POINT('Ctrl Pts',(-183.469815449971,-1.85403871937935,
135.359766580764));
#246593=CARTESIAN_POINT('Ctrl Pts',(-183.477580202919,-1.72746891923083,
135.41128016969));
#246594=CARTESIAN_POINT('Ctrl Pts',(-183.485344955866,-1.59858439316792,
135.457582369257));
#246595=CARTESIAN_POINT('Ctrl Pts',(-183.493109708813,-1.467853683391,135.49846208927));
#246596=CARTESIAN_POINT('Ctrl Pts',(-183.500866749698,-1.33725281719802,
135.539301206969));
#246597=CARTESIAN_POINT('Ctrl Pts',(-183.508623790583,-1.204809787081,135.57472844694));
#246598=CARTESIAN_POINT('Ctrl Pts',(-183.516380831468,-1.07101284954884,
135.60458087695));
#246599=CARTESIAN_POINT('Ctrl Pts',(-183.524132022708,-0.937316809328249,
135.634410795011));
#246600=CARTESIAN_POINT('Ctrl Pts',(-183.531883213948,-0.802269273954129,
135.65867418614));
#246601=CARTESIAN_POINT('Ctrl Pts',(-183.539634405188,-0.66637304503378,
135.677258115703));
#246602=CARTESIAN_POINT('Ctrl Pts',(-183.547382301965,-0.530534575635689,
135.695834146601));
#246603=CARTESIAN_POINT('Ctrl Pts',(-183.555130198743,-0.393848516679804,
135.708735464179));
#246604=CARTESIAN_POINT('Ctrl Pts',(-183.56287809552,-0.256827016516643,
135.715900391006));
#246605=CARTESIAN_POINT('Ctrl Pts',(-183.570624371604,-0.119834178297475,
135.723063819085));
#246606=CARTESIAN_POINT('Ctrl Pts',(-183.578370647688,0.01749357137839,
135.724493222735));
#246607=CARTESIAN_POINT('Ctrl Pts',(-183.586116923772,0.15464021435102,
135.720178908207));
#246608=CARTESIAN_POINT('Ctrl Pts',(-183.593863257037,0.291787869708826,
135.715864561833));
#246609=CARTESIAN_POINT('Ctrl Pts',(-183.601609590303,0.42875402492383,
135.705806424969));
#246610=CARTESIAN_POINT('Ctrl Pts',(-183.609355923568,0.565024315543222,
135.690046913814));
#246611=CARTESIAN_POINT('Ctrl Pts',(-183.617103991571,0.701325122949181,
135.674283873426));
#246612=CARTESIAN_POINT('Ctrl Pts',(-183.624852059574,0.836929367365514,
135.652816963002));
#246613=CARTESIAN_POINT('Ctrl Pts',(-183.632600127577,0.971329842672489,
135.625740233323));
#246614=CARTESIAN_POINT('Ctrl Pts',(-183.640356430319,1.10587316040419,
135.598634726173));
#246615=CARTESIAN_POINT('Ctrl Pts',(-183.648112733061,1.23920976945106,
135.565907567004));
#246616=CARTESIAN_POINT('Ctrl Pts',(-183.655869035803,1.37084412301909,
135.527703655382));
#246617=CARTESIAN_POINT('Ctrl Pts',(-183.663629478317,1.50254873380541,
135.489479353182));
#246618=CARTESIAN_POINT('Ctrl Pts',(-183.671389920831,1.63254890835973,
135.445772598521));
#246619=CARTESIAN_POINT('Ctrl Pts',(-183.679150363345,1.76036717021572,
135.396777245936));
#246620=CARTESIAN_POINT('Ctrl Pts',(-183.686923263611,1.88839061729247,
135.347703241661));
#246621=CARTESIAN_POINT('Ctrl Pts',(-183.694696163876,2.01422479326663,
135.293323829465));
#246622=CARTESIAN_POINT('Ctrl Pts',(-183.702469064142,2.13741418789364,
135.233880191051));
#246623=CARTESIAN_POINT('Ctrl Pts',(-183.709959399904,2.25612533772893,
135.176597478624));
#246624=CARTESIAN_POINT('Ctrl Pts',(-183.717449735665,2.37238038492857,
135.114612487253));
#246625=CARTESIAN_POINT('Ctrl Pts',(-183.724940071427,2.48579733142663,
135.048179026684));
#246626=CARTESIAN_POINT('Ctrl Pts',(-183.732714405547,2.60351451592501,
134.979226721265));
#246627=CARTESIAN_POINT('Ctrl Pts',(-183.740488739666,2.71854703082651,
134.905263540102));
#246628=CARTESIAN_POINT('Ctrl Pts',(-183.748263073785,2.83043883740145,
134.826524096371));
#246629=CARTESIAN_POINT('Ctrl Pts',(-183.756027826732,2.94219274732453,
134.747881691967));
#246630=CARTESIAN_POINT('Ctrl Pts',(-183.763792579679,3.05081333368219,
134.664474959851));
#246631=CARTESIAN_POINT('Ctrl Pts',(-183.771557332626,3.15586974181246,
134.57658399844));
#246632=CARTESIAN_POINT('Ctrl Pts',(-183.779314373511,3.26082180643742,
134.488780331571));
#246633=CARTESIAN_POINT('Ctrl Pts',(-183.787071414396,3.36221643965492,
134.396501547914));
#246634=CARTESIAN_POINT('Ctrl Pts',(-183.794828455281,3.45965264739519,
134.300070362649));
#246635=CARTESIAN_POINT('Ctrl Pts',(-183.802579646521,3.55701537773313,
134.203711896892));
#246636=CARTESIAN_POINT('Ctrl Pts',(-183.810330837761,3.65042534745426,
134.103207536208));
#246637=CARTESIAN_POINT('Ctrl Pts',(-183.818082029001,3.73951576490132,
133.998919257903));
#246638=CARTESIAN_POINT('Ctrl Pts',(-183.825829925778,3.82856831654428,
133.894675304899));
#246639=CARTESIAN_POINT('Ctrl Pts',(-183.833577822555,3.91330471401534,
133.786650929633));
#246640=CARTESIAN_POINT('Ctrl Pts',(-183.841325719332,3.99339623765048,
133.675243678859));
#246641=CARTESIAN_POINT('Ctrl Pts',(-183.849071995416,4.07347100786544,
133.56385973208));
#246642=CARTESIAN_POINT('Ctrl Pts',(-183.8568182715,4.14890260875522,133.449094634542));
#246643=CARTESIAN_POINT('Ctrl Pts',(-183.864564547585,4.21940396427489,
133.33137728723));
#246644=CARTESIAN_POINT('Ctrl Pts',(-183.87231088085,4.28990584021965,133.213659070955));
#246645=CARTESIAN_POINT('Ctrl Pts',(-183.880057214115,4.35547719729329,
133.092988896832));
#246646=CARTESIAN_POINT('Ctrl Pts',(-183.887803547381,4.41587569489273,
132.969822441232));
#246647=CARTESIAN_POINT('Ctrl Pts',(-183.895551615384,4.47628771831701,
132.846628403359));
#246648=CARTESIAN_POINT('Ctrl Pts',(-183.903299683387,4.53152440502785,
132.720937322577));
#246649=CARTESIAN_POINT('Ctrl Pts',(-183.911047751389,4.58139072531399,
132.593226762504));
#246650=CARTESIAN_POINT('Ctrl Pts',(-183.918804054131,4.63131004411868,
132.465380470129));
#246651=CARTESIAN_POINT('Ctrl Pts',(-183.926560356873,4.67584745234577,
132.335510775713));
#246652=CARTESIAN_POINT('Ctrl Pts',(-183.934316659615,4.71485700295889,
132.204112918564));
#246653=CARTESIAN_POINT('Ctrl Pts',(-183.942077102129,4.75388737414372,
132.072644930422));
#246654=CARTESIAN_POINT('Ctrl Pts',(-183.949837544643,4.78738391338526,
131.939647533283));
#246655=CARTESIAN_POINT('Ctrl Pts',(-183.957597987157,4.81525162830277,
131.805627224733));
#246656=CARTESIAN_POINT('Ctrl Pts',(-183.965370887423,4.84316407895025,
131.671391774886));
#246657=CARTESIAN_POINT('Ctrl Pts',(-183.973143787688,4.86542958515006,
131.536130518247));
#246658=CARTESIAN_POINT('Ctrl Pts',(-183.980916687954,4.88200484548556,
131.400357053089));
#246659=CARTESIAN_POINT('Ctrl Pts',(-183.988407023716,4.8979775533577,131.269519295378));
#246660=CARTESIAN_POINT('Ctrl Pts',(-183.995897359478,4.90866651731051,
131.138206229746));
#246661=CARTESIAN_POINT('Ctrl Pts',(-184.00338769524,4.91407879538588,131.006876432353));
#246662=CARTESIAN_POINT('Ctrl Pts',(-184.011162029359,4.91969628162939,
130.870567225777));
#246663=CARTESIAN_POINT('Ctrl Pts',(-184.018936363479,4.91964684670001,
130.73380820703));
#246664=CARTESIAN_POINT('Ctrl Pts',(-184.026710697598,4.91388137723509,
130.597109868563));
#246665=CARTESIAN_POINT('Ctrl Pts',(-184.034475450545,4.90812301319603,
130.460579998582));
#246666=CARTESIAN_POINT('Ctrl Pts',(-184.042240203492,4.89666264739697,
130.324111046953));
#246667=CARTESIAN_POINT('Ctrl Pts',(-184.050004956439,4.87950304710029,
130.188216903941));
#246668=CARTESIAN_POINT('Ctrl Pts',(-184.057761997324,4.86236048996048,
130.052457732909));
#246669=CARTESIAN_POINT('Ctrl Pts',(-184.065519038209,4.83953001175498,
129.917272619736));
#246670=CARTESIAN_POINT('Ctrl Pts',(-184.073276079094,4.81106637481358,
129.783173367529));
#246671=CARTESIAN_POINT('Ctrl Pts',(-184.081027270334,4.78262420252226,
129.649175240611));
#246672=CARTESIAN_POINT('Ctrl Pts',(-184.088778461574,4.74855740774753,
129.516261725672));
#246673=CARTESIAN_POINT('Ctrl Pts',(-184.096529652814,4.70897227239641,
129.384937072495));
#246674=CARTESIAN_POINT('Ctrl Pts',(-184.104277549591,4.66940396178373,
129.253668235799));
#246675=CARTESIAN_POINT('Ctrl Pts',(-184.112025446369,4.62432208809752,
129.123987291273));
#246676=CARTESIAN_POINT('Ctrl Pts',(-184.119773343146,4.57388343767266,
128.996385683812));
#246677=CARTESIAN_POINT('Ctrl Pts',(-184.12751961923,4.52345533792613,128.868810767856));
#246678=CARTESIAN_POINT('Ctrl Pts',(-184.135265895314,4.46767283385089,
128.74331468718));
#246679=CARTESIAN_POINT('Ctrl Pts',(-184.143012171398,4.40674160037786,
128.620370798451));
#246680=CARTESIAN_POINT('Ctrl Pts',(-184.150758504663,4.3458099171244,128.497426002177));
#246681=CARTESIAN_POINT('Ctrl Pts',(-184.158504837929,4.2797296022448,128.377033785747));
#246682=CARTESIAN_POINT('Ctrl Pts',(-184.166251171194,4.20875303816093,
128.259644341383));
#246683=CARTESIAN_POINT('Ctrl Pts',(-184.173999239197,4.13776057936755,
128.142228608466));
#246684=CARTESIAN_POINT('Ctrl Pts',(-184.1817473072,4.06186989174729,128.027817320214));
#246685=CARTESIAN_POINT('Ctrl Pts',(-184.189495375203,3.98137734477428,
127.916832695447));
#246686=CARTESIAN_POINT('Ctrl Pts',(-184.197251677945,3.90079924936458,
127.8057301149));
#246687=CARTESIAN_POINT('Ctrl Pts',(-184.205007980687,3.81560975438436,
127.698061789918));
#246688=CARTESIAN_POINT('Ctrl Pts',(-184.212764283429,3.72614663075139,
127.594218198819));
#246689=CARTESIAN_POINT('Ctrl Pts',(-184.220524725943,3.63663575795566,
127.490319183269));
#246690=CARTESIAN_POINT('Ctrl Pts',(-184.228285168457,3.54284697871845,
127.390249254338));
#246691=CARTESIAN_POINT('Ctrl Pts',(-184.236045610971,3.44515507810191,
127.294362106124));
#246692=CARTESIAN_POINT('Ctrl Pts',(-184.243818511237,3.34730635377383,
127.198321031346));
#246693=CARTESIAN_POINT('Ctrl Pts',(-184.251591411502,3.2455422777318,127.106476417236));
#246694=CARTESIAN_POINT('Ctrl Pts',(-184.259364311768,3.14027154927359,
127.01914230691));
#246695=CARTESIAN_POINT('Ctrl Pts',(-184.26685464753,3.03882767695724,126.934983011478));
#246696=CARTESIAN_POINT('Ctrl Pts',(-184.274344983291,2.93412792197492,
126.855012163906));
#246697=CARTESIAN_POINT('Ctrl Pts',(-184.281835319053,2.82656191248064,
126.779471697681));
#246698=CARTESIAN_POINT('Ctrl Pts',(-184.289609653172,2.71491750504099,
126.701067091717));
#246699=CARTESIAN_POINT('Ctrl Pts',(-184.297383987292,2.59983154856586,
126.627187092566));
#246700=CARTESIAN_POINT('Ctrl Pts',(-184.305158321411,2.4817069878406,126.55814895433));
#246701=CARTESIAN_POINT('Ctrl Pts',(-184.312923074358,2.36372800507934,
126.489195899429));
#246702=CARTESIAN_POINT('Ctrl Pts',(-184.320687827305,2.2427182034227,126.425073027955));
#246703=CARTESIAN_POINT('Ctrl Pts',(-184.328452580252,2.11911142907846,
126.366055781973));
#246704=CARTESIAN_POINT('Ctrl Pts',(-184.336209621137,1.99562742272505,
126.307097152752));
#246705=CARTESIAN_POINT('Ctrl Pts',(-184.343966662022,1.8695519272367,126.253234224909));
#246706=CARTESIAN_POINT('Ctrl Pts',(-184.351723702907,1.74134513743703,
126.204697567426));
#246707=CARTESIAN_POINT('Ctrl Pts',(-184.359474894147,1.61323502937467,
126.156197511813));
#246708=CARTESIAN_POINT('Ctrl Pts',(-184.367226085387,1.48299719024648,
126.113015869661));
#246709=CARTESIAN_POINT('Ctrl Pts',(-184.374977276627,1.35111330764339,
126.075335782316));
#246710=CARTESIAN_POINT('Ctrl Pts',(-184.382725173404,1.2192854792087,126.037671710014));
#246711=CARTESIAN_POINT('Ctrl Pts',(-184.390473070181,1.08581337391095,
126.005504648981));
#246712=CARTESIAN_POINT('Ctrl Pts',(-184.398220966959,0.951195205101593,
125.978968328405));
#246713=CARTESIAN_POINT('Ctrl Pts',(-184.405967243043,0.816605195511116,
125.952437558655));
#246714=CARTESIAN_POINT('Ctrl Pts',(-184.413713519127,0.680869982589351,
125.931535262159));
#246715=CARTESIAN_POINT('Ctrl Pts',(-184.421459795211,0.544498987029324,
125.916344259612));
#246716=CARTESIAN_POINT('Ctrl Pts',(-184.429206128476,0.408126984809772,
125.901153144929));
#246717=CARTESIAN_POINT('Ctrl Pts',(-184.436952461741,0.271119579148865,
125.891673451605));
#246718=CARTESIAN_POINT('Ctrl Pts',(-184.444698795007,0.133991948377302,
125.887936183054));
#246719=CARTESIAN_POINT('Ctrl Pts',(-184.45244686301,-0.00316639117658285,
125.884198077567));
#246720=CARTESIAN_POINT('Ctrl Pts',(-184.460194931013,-0.140444618670646,
125.886204966446));
#246721=CARTESIAN_POINT('Ctrl Pts',(-184.467942999016,-0.277327314513638,
125.893935725245));
#246722=CARTESIAN_POINT('Ctrl Pts',(-184.475699301758,-0.41435549091451,
125.901674700386));
#246723=CARTESIAN_POINT('Ctrl Pts',(-184.4834556045,-0.550986904952897,
125.915149675607));
#246724=CARTESIAN_POINT('Ctrl Pts',(-184.491211907241,-0.686710462729283,
125.934287537737));
#246725=CARTESIAN_POINT('Ctrl Pts',(-184.498972349756,-0.822506460255012,
125.95343561432));
#246726=CARTESIAN_POINT('Ctrl Pts',(-184.50673279227,-0.957393251687999,
125.978252529597));
#246727=CARTESIAN_POINT('Ctrl Pts',(-184.514493234784,-1.09087068368609,
126.00861414658));
#246728=CARTESIAN_POINT('Ctrl Pts',(-184.522266135049,-1.22456238550795,
126.039024502726));
#246729=CARTESIAN_POINT('Ctrl Pts',(-184.530039035315,-1.35683982936047,
126.074997244652));
#246730=CARTESIAN_POINT('Ctrl Pts',(-184.53781193558,-1.48721788992002,
126.116358270041));
#246731=CARTESIAN_POINT('Ctrl Pts',(-184.545302271342,-1.61285637957678,
126.156215717975));
#246732=CARTESIAN_POINT('Ctrl Pts',(-184.552792607104,-1.73673089353513,
126.201076390584));
#246733=CARTESIAN_POINT('Ctrl Pts',(-184.560282942866,-1.85842728276808,
126.250743253627));
#246734=CARTESIAN_POINT('Ctrl Pts',(-184.568057639186,-1.98474371230457,
126.302295652556));
#246735=CARTESIAN_POINT('Ctrl Pts',(-184.575832335506,-2.10911352182145,
126.359189682738));
#246736=CARTESIAN_POINT('Ctrl Pts',(-184.583607031826,-2.23105192754482,
126.421257794326));
#246737=CARTESIAN_POINT('Ctrl Pts',(-184.591372063905,-2.35283875923919,
126.483248752913));
#246738=CARTESIAN_POINT('Ctrl Pts',(-184.599137095985,-2.4721998557502,
126.550400819786));
#246739=CARTESIAN_POINT('Ctrl Pts',(-184.606902128064,-2.5886689263795,
126.622497844579));
#246740=CARTESIAN_POINT('Ctrl Pts',(-184.614659365366,-2.70502108178013,
126.694522496164));
#246741=CARTESIAN_POINT('Ctrl Pts',(-184.622416602668,-2.81848665856598,
126.771482022306));
#246742=CARTESIAN_POINT('Ctrl Pts',(-184.63017383997,-2.92862289471845,
126.85311385192));
#246743=CARTESIAN_POINT('Ctrl Pts',(-184.63807648539,-3.0408236162226,126.936275856545));
#246744=CARTESIAN_POINT('Ctrl Pts',(-184.645979130809,-3.1495685597896,
127.02428690553));
#246745=CARTESIAN_POINT('Ctrl Pts',(-184.653881776229,-3.25441882467343,
127.116821983719));
#246746=CARTESIAN_POINT('Ctrl Pts',(-184.66162933114,-3.35721138861581,
127.207541048209));
#246747=CARTESIAN_POINT('Ctrl Pts',(-184.669376886051,-3.45626042849622,
127.30260793449));
#246748=CARTESIAN_POINT('Ctrl Pts',(-184.677124440961,-3.55118486455092,
127.401675042864));
#246749=CARTESIAN_POINT('Ctrl Pts',(-184.684870290526,-3.64608840639422,
127.500720345166));
#246750=CARTESIAN_POINT('Ctrl Pts',(-184.69261614009,-3.73686888073763,
127.603763835403));
#246751=CARTESIAN_POINT('Ctrl Pts',(-184.700361989654,-3.82318206752826,
127.710421067247));
#246752=CARTESIAN_POINT('Ctrl Pts',(-184.708107811659,-3.90949494721215,
127.817077919599));
#246753=CARTESIAN_POINT('Ctrl Pts',(-184.715853633663,-3.99134032571703,
127.927348183657));
#246754=CARTESIAN_POINT('Ctrl Pts',(-184.723599455667,-4.06841453913728,
128.040814670737));
#246755=CARTESIAN_POINT('Ctrl Pts',(-184.731619278531,-4.1482151773007,
128.158294923565));
#246756=CARTESIAN_POINT('Ctrl Pts',(-184.739639101396,-4.22290061394825,
128.279201330047));
#246757=CARTESIAN_POINT('Ctrl Pts',(-184.74765892426,-4.29218348010272,
128.403039307197));
#246758=CARTESIAN_POINT('Ctrl Pts',(-184.755413217867,-4.35917245170187,
128.522777118212));
#246759=CARTESIAN_POINT('Ctrl Pts',(-184.763167511474,-4.42111077918117,
128.645255083161));
#246760=CARTESIAN_POINT('Ctrl Pts',(-184.770921805081,-4.4777865008787,
128.770002951115));
#246761=CARTESIAN_POINT('Ctrl Pts',(-184.779074392574,-4.53737333151672,
128.901158406353));
#246762=CARTESIAN_POINT('Ctrl Pts',(-184.787226980067,-4.59114243408741,
129.034822659559));
#246763=CARTESIAN_POINT('Ctrl Pts',(-184.79537956756,-4.63890608312226,
129.170428729612));
#246764=CARTESIAN_POINT('Ctrl Pts',(-184.803532155053,-4.68666973215712,
129.306034799666));
#246765=CARTESIAN_POINT('Ctrl Pts',(-184.811684742546,-4.72842783798587,
129.443582194741));
#246766=CARTESIAN_POINT('Ctrl Pts',(-184.819837330039,-4.76405452823405,
129.582490119308));
#246767=CARTESIAN_POINT('Ctrl Pts',(-183.069718605797,-4.76405452823406,
129.582490119308));
#246768=CARTESIAN_POINT('Ctrl Pts',(-183.077377441043,-4.79772994797449,
129.71379006978));
#246769=CARTESIAN_POINT('Ctrl Pts',(-183.085036276289,-4.825950394775,129.846394602858));
#246770=CARTESIAN_POINT('Ctrl Pts',(-183.092695111536,-4.84863804824104,
129.97980489498));
#246771=CARTESIAN_POINT('Ctrl Pts',(-183.100555832273,-4.87192374408618,
130.116731857903));
#246772=CARTESIAN_POINT('Ctrl Pts',(-183.10841655301,-4.88938085774212,
130.254507194701));
#246773=CARTESIAN_POINT('Ctrl Pts',(-183.116277273746,-4.90098218359303,
130.392587987825));
#246774=CARTESIAN_POINT('Ctrl Pts',(-183.124137994483,-4.91258350944392,
130.530668780949));
#246775=CARTESIAN_POINT('Ctrl Pts',(-183.13199871522,-4.91832909109846,
130.669054577283));
#246776=CARTESIAN_POINT('Ctrl Pts',(-183.139859435957,-4.91824917715616,
130.807205596086));
#246777=CARTESIAN_POINT('Origin',(213.235140564004,0.,130.804360617566));
#246778=CARTESIAN_POINT('',(-181.320039938991,-4.76405452823418,129.582490119309));
#246779=CARTESIAN_POINT('',(-181.664999290689,-4.76405452823418,129.582490119309));
#246780=CARTESIAN_POINT('',(213.235140564004,-4.76405452823405,129.582490119308));
#246781=CARTESIAN_POINT('',(-181.735140563977,-4.91824950327072,130.806571064885));
#246782=CARTESIAN_POINT('Ctrl Pts',(-181.664999290689,-4.76405452823418,
129.582490119309));
#246783=CARTESIAN_POINT('Ctrl Pts',(-181.672675880478,-4.79779503273996,
129.714043834293));
#246784=CARTESIAN_POINT('Ctrl Pts',(-181.680352470268,-4.82605765331497,
129.846900063432));
#246785=CARTESIAN_POINT('Ctrl Pts',(-181.688029060058,-4.84876606521478,
129.980558027547));
#246786=CARTESIAN_POINT('Ctrl Pts',(-181.695880977377,-4.87199312014276,
130.117268638917));
#246787=CARTESIAN_POINT('Ctrl Pts',(-181.703732894697,-4.88940914158996,
130.254817604855));
#246788=CARTESIAN_POINT('Ctrl Pts',(-181.711584812017,-4.90098872141958,
130.392665809464));
#246789=CARTESIAN_POINT('Ctrl Pts',(-181.719436729337,-4.9125683012492,
130.530514014073));
#246790=CARTESIAN_POINT('Ctrl Pts',(-181.727288646657,-4.91831148526274,
130.668661014282));
#246791=CARTESIAN_POINT('Ctrl Pts',(-181.735140563977,-4.91824950327072,
130.806571064884));
#246792=CARTESIAN_POINT('Ctrl Pts',(-181.735140564012,-4.91824950327044,
130.806571065507));
#246793=CARTESIAN_POINT('Ctrl Pts',(-181.742166278867,-4.91819404319526,
130.929969803894));
#246794=CARTESIAN_POINT('Ctrl Pts',(-181.749191993722,-4.91349490493225,
131.053259845395));
#246795=CARTESIAN_POINT('Ctrl Pts',(-181.756217708576,-4.90417395891944,
131.176195047328));
#246796=CARTESIAN_POINT('Ctrl Pts',(-181.763992042696,-4.89385982717492,
131.312229508533));
#246797=CARTESIAN_POINT('Ctrl Pts',(-181.771766376815,-4.87786497991832,
131.448049965438));
#246798=CARTESIAN_POINT('Ctrl Pts',(-181.779540710934,-4.85620016088216,
131.583143681036));
#246799=CARTESIAN_POINT('Ctrl Pts',(-181.787305463881,-4.83456204179922,
131.718070905703));
#246800=CARTESIAN_POINT('Ctrl Pts',(-181.795070216828,-4.80726791575691,
131.852272788801));
#246801=CARTESIAN_POINT('Ctrl Pts',(-181.802834969775,-4.77438044942487,
131.98523926783));
#246802=CARTESIAN_POINT('Ctrl Pts',(-181.81059201066,-4.74152564738802,
132.118073682678));
#246803=CARTESIAN_POINT('Ctrl Pts',(-181.818349051545,-4.70308865379099,
132.249674758213));
#246804=CARTESIAN_POINT('Ctrl Pts',(-181.82610609243,-4.6591835323683,132.379540567352));
#246805=CARTESIAN_POINT('Ctrl Pts',(-181.833857283671,-4.61531152013915,
132.509308443675));
#246806=CARTESIAN_POINT('Ctrl Pts',(-181.841608474911,-4.56597971248463,
132.637343289375));
#246807=CARTESIAN_POINT('Ctrl Pts',(-181.849359666151,-4.51135246061705,
132.763156686223));
#246808=CARTESIAN_POINT('Ctrl Pts',(-181.857107562928,-4.45674842678867,
132.888916609021));
#246809=CARTESIAN_POINT('Ctrl Pts',(-181.864855459705,-4.39685358061205,
133.012456602989));
#246810=CARTESIAN_POINT('Ctrl Pts',(-181.872603356482,-4.33188094023251,
133.133306856136));
#246811=CARTESIAN_POINT('Ctrl Pts',(-181.880349632566,-4.26692189072869,
133.254131830015));
#246812=CARTESIAN_POINT('Ctrl Pts',(-181.888095908651,-4.19688734474357,
133.372267838051));
#246813=CARTESIAN_POINT('Ctrl Pts',(-181.895842184735,-4.12203676652123,
133.487268733389));
#246814=CARTESIAN_POINT('Ctrl Pts',(-181.903588518,-4.04718563576903,133.602270477636));
#246815=CARTESIAN_POINT('Ctrl Pts',(-181.911334851265,-3.9675186151122,
133.714136735334));
#246816=CARTESIAN_POINT('Ctrl Pts',(-181.919081184531,-3.88333885679162,
133.822449812045));
#246817=CARTESIAN_POINT('Ctrl Pts',(-181.926829252534,-3.79914024699795,
133.930787144718));
#246818=CARTESIAN_POINT('Ctrl Pts',(-181.934577320537,-3.71042712844116,
134.035569404395));
#246819=CARTESIAN_POINT('Ctrl Pts',(-181.94232538854,-3.61754307876341,
134.136411808018));
#246820=CARTESIAN_POINT('Ctrl Pts',(-181.950081691281,-3.52456031081195,
134.237361388148));
#246821=CARTESIAN_POINT('Ctrl Pts',(-181.957837994024,-3.42739802181008,
134.334362459562));
#246822=CARTESIAN_POINT('Ctrl Pts',(-181.965594296765,-3.32643720759424,
134.427066590514));
#246823=CARTESIAN_POINT('Ctrl Pts',(-181.97335473928,-3.22542250755198,
134.519820200452));
#246824=CARTESIAN_POINT('Ctrl Pts',(-181.981115181794,-3.12060554120253,
134.608272048101));
#246825=CARTESIAN_POINT('Ctrl Pts',(-181.988875624308,-3.01239977711739,
134.692114550793));
#246826=CARTESIAN_POINT('Ctrl Pts',(-181.996648524573,-2.90402031153368,
134.776091644914));
#246827=CARTESIAN_POINT('Ctrl Pts',(-182.004421424839,-2.79224149634652,
134.85544438141));
#246828=CARTESIAN_POINT('Ctrl Pts',(-182.012194325104,-2.67750585984077,
134.929908512454));
#246829=CARTESIAN_POINT('Ctrl Pts',(-182.019684660866,-2.5669411527255,
135.001665684771));
#246830=CARTESIAN_POINT('Ctrl Pts',(-182.027174996628,-2.4536311327147,
135.068883350007));
#246831=CARTESIAN_POINT('Ctrl Pts',(-182.03466533239,-2.33799097923109,
135.131366654485));
#246832=CARTESIAN_POINT('Ctrl Pts',(-182.042439666509,-2.21796629417824,
135.196219032444));
#246833=CARTESIAN_POINT('Ctrl Pts',(-182.050214000628,-2.09505109151086,
135.256176389005));
#246834=CARTESIAN_POINT('Ctrl Pts',(-182.057988334747,-1.96968255864387,
135.310970616298));
#246835=CARTESIAN_POINT('Ctrl Pts',(-182.065753087694,-1.84446853128913,
135.365697314603));
#246836=CARTESIAN_POINT('Ctrl Pts',(-182.073517840642,-1.71680754442264,
135.415273389231));
#246837=CARTESIAN_POINT('Ctrl Pts',(-182.081282593589,-1.5871626009352,
135.459475862186));
#246838=CARTESIAN_POINT('Ctrl Pts',(-182.089039634474,-1.45764642263331,
135.503634432622));
#246839=CARTESIAN_POINT('Ctrl Pts',(-182.096796675359,-1.32615057673516,
135.542429897177));
#246840=CARTESIAN_POINT('Ctrl Pts',(-182.104553716244,-1.19315900294414,
135.575686917055));
#246841=CARTESIAN_POINT('Ctrl Pts',(-182.112304907484,-1.06026771913327,
135.608918857555));
#246842=CARTESIAN_POINT('Ctrl Pts',(-182.120056098724,-0.925883330276927,
135.636620572151));
#246843=CARTESIAN_POINT('Ctrl Pts',(-182.127807289964,-0.790505592309228,
135.65866633219));
#246844=CARTESIAN_POINT('Ctrl Pts',(-182.135555186741,-0.655185393491669,
135.680702722192));
#246845=CARTESIAN_POINT('Ctrl Pts',(-182.143303083518,-0.518873070360332,
135.697087876165));
#246846=CARTESIAN_POINT('Ctrl Pts',(-182.151050980295,-0.382079030561141,
135.70774706745));
#246847=CARTESIAN_POINT('Ctrl Pts',(-182.15879725638,-0.245313605126137,
135.718404029062));
#246848=CARTESIAN_POINT('Ctrl Pts',(-182.166543532464,-0.108067052986587,
135.723337380018));
#246849=CARTESIAN_POINT('Ctrl Pts',(-182.174289808548,0.0291450231112156,
135.722524261664));
#246850=CARTESIAN_POINT('Ctrl Pts',(-182.182036141813,0.16635811207758,
135.721711137307));
#246851=CARTESIAN_POINT('Ctrl Pts',(-182.189782475079,0.303536333536031,
135.715151461312));
#246852=CARTESIAN_POINT('Ctrl Pts',(-182.197528808344,0.440164408135673,
135.702874510198));
#246853=CARTESIAN_POINT('Ctrl Pts',(-182.205276876347,0.576823079645122,
135.690594809746));
#246854=CARTESIAN_POINT('Ctrl Pts',(-182.21302494435,0.712930969817092,
135.672595321422));
#246855=CARTESIAN_POINT('Ctrl Pts',(-182.220773012353,0.847978637660013,
135.648957122186));
#246856=CARTESIAN_POINT('Ctrl Pts',(-182.228529315095,0.983169835771588,
135.62529379999));
#246857=CARTESIAN_POINT('Ctrl Pts',(-182.236285617837,1.1172981748916,135.595979862955));
#246858=CARTESIAN_POINT('Ctrl Pts',(-182.244041920579,1.24986457196712,
135.5611475178));
#246859=CARTESIAN_POINT('Ctrl Pts',(-182.251802363093,1.38250172372027,
135.526296581574));
#246860=CARTESIAN_POINT('Ctrl Pts',(-182.259562805607,1.51357489884223,
135.485921483424));
#246861=CARTESIAN_POINT('Ctrl Pts',(-182.267323248121,1.64260182946052,
135.440203830225));
#246862=CARTESIAN_POINT('Ctrl Pts',(-182.275096148387,1.77183588556232,
135.39441278699));
#246863=CARTESIAN_POINT('Ctrl Pts',(-182.282869048652,1.89901677012015,
135.343262196406));
#246864=CARTESIAN_POINT('Ctrl Pts',(-182.290641948918,2.02368296660664,
135.286981537649));
#246865=CARTESIAN_POINT('Ctrl Pts',(-182.298132284679,2.14381723283161,
135.232746822602));
#246866=CARTESIAN_POINT('Ctrl Pts',(-182.305622620441,2.26161619186303,
135.173748683604));
#246867=CARTESIAN_POINT('Ctrl Pts',(-182.313112956203,2.37669149316271,
135.11023109969));
#246868=CARTESIAN_POINT('Ctrl Pts',(-182.320887290322,2.49612990949109,
135.044305227274));
#246869=CARTESIAN_POINT('Ctrl Pts',(-182.328661624441,2.61301240105838,
134.973301601892));
#246870=CARTESIAN_POINT('Ctrl Pts',(-182.33643595856,2.72687709064381,134.897443122845));
#246871=CARTESIAN_POINT('Ctrl Pts',(-182.344200711507,2.84060145217569,
134.821678132594));
#246872=CARTESIAN_POINT('Ctrl Pts',(-182.351965464454,2.9513150895211,134.741070408096));
#246873=CARTESIAN_POINT('Ctrl Pts',(-182.359730217402,3.05858014060573,
134.655888961742));
#246874=CARTESIAN_POINT('Ctrl Pts',(-182.367487258287,3.16573865452946,
134.570792118802));
#246875=CARTESIAN_POINT('Ctrl Pts',(-182.375244299171,3.26945509427675,
134.481130835716));
#246876=CARTESIAN_POINT('Ctrl Pts',(-182.383001340056,3.369320361121,134.387217489761));
#246877=CARTESIAN_POINT('Ctrl Pts',(-182.390752531297,3.46911031879082,
134.29337496459));
#246878=CARTESIAN_POINT('Ctrl Pts',(-182.398503722537,3.56505460053173,
134.195287025673));
#246879=CARTESIAN_POINT('Ctrl Pts',(-182.406254913777,3.6567772969768,134.093306172423));
#246880=CARTESIAN_POINT('Ctrl Pts',(-182.414002810554,3.74846100882897,
133.991368663756));
#246881=CARTESIAN_POINT('Ctrl Pts',(-182.421750707331,3.83592644318413,
133.885541821693));
#246882=CARTESIAN_POINT('Ctrl Pts',(-182.429498604108,3.91883484258758,
133.776214675056));
#246883=CARTESIAN_POINT('Ctrl Pts',(-182.437244880192,4.00172589934117,
133.666910397302));
#246884=CARTESIAN_POINT('Ctrl Pts',(-182.444991156276,4.08006158108549,
133.554107582659));
#246885=CARTESIAN_POINT('Ctrl Pts',(-182.45273743236,4.15354396030729,133.438227666658));
#246886=CARTESIAN_POINT('Ctrl Pts',(-182.460483765626,4.22702688195942,
133.322346895258));
#246887=CARTESIAN_POINT('Ctrl Pts',(-182.468230098891,4.29565622022754,
133.203389307352));
#246888=CARTESIAN_POINT('Ctrl Pts',(-182.475976432157,4.35917808520141,
133.081804246726));
#246889=CARTESIAN_POINT('Ctrl Pts',(-182.48372450016,4.42271417545642,132.960191957968));
#246890=CARTESIAN_POINT('Ctrl Pts',(-182.491472568163,4.48114033541539,
132.83595137209));
#246891=CARTESIAN_POINT('Ctrl Pts',(-182.499220636166,4.53424941212098,
132.709554920303));
#246892=CARTESIAN_POINT('Ctrl Pts',(-182.506976938907,4.58741493378524,
132.583024132863));
#246893=CARTESIAN_POINT('Ctrl Pts',(-182.514733241649,4.63525193190573,
132.45433326345));
#246894=CARTESIAN_POINT('Ctrl Pts',(-182.522489544391,4.67760186915715,
132.323973665732));
#246895=CARTESIAN_POINT('Ctrl Pts',(-182.530249986905,4.71997440984532,
132.193544491172));
#246896=CARTESIAN_POINT('Ctrl Pts',(-182.53801042942,4.75685394908354,132.06144518999));
#246897=CARTESIAN_POINT('Ctrl Pts',(-182.545770871934,4.78813260031306,
131.928179670759));
#246898=CARTESIAN_POINT('Ctrl Pts',(-182.553543772199,4.81946146281031,
131.794700221885));
#246899=CARTESIAN_POINT('Ctrl Pts',(-182.561316672464,4.84517139696213,
131.660051198124));
#246900=CARTESIAN_POINT('Ctrl Pts',(-182.56908957273,4.86520600914096,131.524744925501));
#246901=CARTESIAN_POINT('Ctrl Pts',(-182.576579908492,4.88451231270299,
131.394357376703));
#246902=CARTESIAN_POINT('Ctrl Pts',(-182.584070244254,4.89854872220694,
131.263359840987));
#246903=CARTESIAN_POINT('Ctrl Pts',(-182.591560580016,4.90731059117172,
131.132210925289));
#246904=CARTESIAN_POINT('Ctrl Pts',(-182.599334914135,4.91640466906136,
130.99608945859));
#246905=CARTESIAN_POINT('Ctrl Pts',(-182.607109248254,4.91984514980589,
130.859373714271));
#246906=CARTESIAN_POINT('Ctrl Pts',(-182.614883582373,4.91756990898058,
130.722572765236));
#246907=CARTESIAN_POINT('Ctrl Pts',(-182.62264833532,4.91529747218625,130.585940411145));
#246908=CARTESIAN_POINT('Ctrl Pts',(-182.630413088267,4.90732333595251,
130.449223448429));
#246909=CARTESIAN_POINT('Ctrl Pts',(-182.638177841215,4.89363715287714,
130.31293567062));
#246910=CARTESIAN_POINT('Ctrl Pts',(-182.6459348821,4.87996456311174,130.176783255754));
#246911=CARTESIAN_POINT('Ctrl Pts',(-182.653691922985,4.86059125541069,
130.041059563987));
#246912=CARTESIAN_POINT('Ctrl Pts',(-182.66144896387,4.83555891376832,129.906277629209));
#246913=CARTESIAN_POINT('Ctrl Pts',(-182.66920015511,4.81054544920946,129.771597334537));
#246914=CARTESIAN_POINT('Ctrl Pts',(-182.67695134635,4.77988151605426,129.63785776611));
#246915=CARTESIAN_POINT('Ctrl Pts',(-182.68470253759,4.74366049384699,129.505565721666));
#246916=CARTESIAN_POINT('Ctrl Pts',(-182.692450434367,4.70745486654033,
129.37332990487));
#246917=CARTESIAN_POINT('Ctrl Pts',(-182.700198331144,4.66569695087129,
129.242540764698));
#246918=CARTESIAN_POINT('Ctrl Pts',(-182.707946227921,4.618530941128,129.11369358697));
#246919=CARTESIAN_POINT('Ctrl Pts',(-182.715692504005,4.57137479749729,
128.984873361295));
#246920=CARTESIAN_POINT('Ctrl Pts',(-182.72343878009,4.51881294423457,128.857994656986));
#246921=CARTESIAN_POINT('Ctrl Pts',(-182.731185056174,4.46103890988972,
128.733535925094));
#246922=CARTESIAN_POINT('Ctrl Pts',(-182.738931389439,4.40326444907,128.609076274477));
#246923=CARTESIAN_POINT('Ctrl Pts',(-182.746677722704,4.34027789500933,
128.487036986544));
#246924=CARTESIAN_POINT('Ctrl Pts',(-182.75442405597,4.27232005966242,128.36787454736));
#246925=CARTESIAN_POINT('Ctrl Pts',(-182.762172123973,4.20434700562956,
128.248685422574));
#246926=CARTESIAN_POINT('Ctrl Pts',(-182.769920191976,4.13140064865017,
128.132374768074));
#246927=CARTESIAN_POINT('Ctrl Pts',(-182.777668259979,4.05376648724896,
128.019372228119));
#246928=CARTESIAN_POINT('Ctrl Pts',(-182.78542456272,3.97604981533704,127.906249587719));
#246929=CARTESIAN_POINT('Ctrl Pts',(-182.793180865462,3.89363560815299,
127.796442408019));
#246930=CARTESIAN_POINT('Ctrl Pts',(-182.800937168204,3.80685156215607,
127.69034965962));
#246931=CARTESIAN_POINT('Ctrl Pts',(-182.808697610718,3.72002119690079,
127.584200286326));
#246932=CARTESIAN_POINT('Ctrl Pts',(-182.816458053233,3.62881660536122,
127.481769586489));
#246933=CARTESIAN_POINT('Ctrl Pts',(-182.824218495747,3.5336034247693,127.383420703016));
#246934=CARTESIAN_POINT('Ctrl Pts',(-182.831991396012,3.43823739952725,
127.284913941185));
#246935=CARTESIAN_POINT('Ctrl Pts',(-182.839764296278,3.33885020978783,
127.190502359112));
#246936=CARTESIAN_POINT('Ctrl Pts',(-182.847537196543,3.23584240781202,
127.100510327084));
#246937=CARTESIAN_POINT('Ctrl Pts',(-182.855027532305,3.1365791988993,127.013789732096));
#246938=CARTESIAN_POINT('Ctrl Pts',(-182.862517868067,3.03395428425488,
126.931173135403));
#246939=CARTESIAN_POINT('Ctrl Pts',(-182.870008203829,2.92835099134394,
126.852912334468));
#246940=CARTESIAN_POINT('Ctrl Pts',(-182.877782537948,2.818743717485,126.77168425148));
#246941=CARTESIAN_POINT('Ctrl Pts',(-182.885556872067,2.70558055367971,
126.694891478318));
#246942=CARTESIAN_POINT('Ctrl Pts',(-182.893331206186,2.58925621761079,
126.622861448361));
#246943=CARTESIAN_POINT('Ctrl Pts',(-182.901095959133,2.47307524088987,
126.550920188978));
#246944=CARTESIAN_POINT('Ctrl Pts',(-182.90886071208,2.35374117271796,126.483730197785));
#246945=CARTESIAN_POINT('Ctrl Pts',(-182.916625465027,2.23168068912202,
126.4215778983));
#246946=CARTESIAN_POINT('Ctrl Pts',(-182.924382505912,2.10974143771914,
126.359487329355));
#246947=CARTESIAN_POINT('Ctrl Pts',(-182.932139546797,1.98508150590871,
126.302424671168));
#246948=CARTESIAN_POINT('Ctrl Pts',(-182.939896587682,1.85815505485159,
126.250632161166));
#246949=CARTESIAN_POINT('Ctrl Pts',(-182.947647778922,1.73132432001839,
126.198878708298));
#246950=CARTESIAN_POINT('Ctrl Pts',(-182.955398970163,1.60223082852072,
126.152387640204));
#246951=CARTESIAN_POINT('Ctrl Pts',(-182.963150161403,1.47135143757472,
126.111354330585));
#246952=CARTESIAN_POINT('Ctrl Pts',(-182.97089805818,1.34052767386137,126.070338461217));
#246953=CARTESIAN_POINT('Ctrl Pts',(-182.978645954957,1.20791989268096,
126.034775853349));
#246954=CARTESIAN_POINT('Ctrl Pts',(-182.986393851734,1.07402273255796,
126.004812906328));
#246955=CARTESIAN_POINT('Ctrl Pts',(-182.994140127818,0.940153580834378,
125.97485622691));
#246956=CARTESIAN_POINT('Ctrl Pts',(-183.001886403902,0.804995967924261,
125.950496963824));
#246957=CARTESIAN_POINT('Ctrl Pts',(-183.009632679986,0.669057035157692,
125.931830910504));
#246958=CARTESIAN_POINT('Ctrl Pts',(-183.017379013251,0.533117098920988,
125.913164719394));
#246959=CARTESIAN_POINT('Ctrl Pts',(-183.025125346517,0.39639621864993,
125.900191875094));
#246960=CARTESIAN_POINT('Ctrl Pts',(-183.032871679782,0.259408613742112,
125.892956517554));
#246961=CARTESIAN_POINT('Ctrl Pts',(-183.040619747785,0.122390331409793,
125.885719539705));
#246962=CARTESIAN_POINT('Ctrl Pts',(-183.048367815788,-0.0148944040710403,
125.884222625977));
#246963=CARTESIAN_POINT('Ctrl Pts',(-183.056115883791,-0.151929801890471,
125.888457811591));
#246964=CARTESIAN_POINT('Ctrl Pts',(-183.063872186533,-0.289110842561633,
125.89269749841));
#246965=CARTESIAN_POINT('Ctrl Pts',(-183.071628489275,-0.426041624805545,
125.902681442188));
#246966=CARTESIAN_POINT('Ctrl Pts',(-183.079384792016,-0.562209355415556,
125.918349595967));
#246967=CARTESIAN_POINT('Ctrl Pts',(-183.08714523453,-0.698449762843326,
125.934026112312));
#246968=CARTESIAN_POINT('Ctrl Pts',(-183.094905677045,-0.833925921127289,
125.955392822951));
#246969=CARTESIAN_POINT('Ctrl Pts',(-183.102666119559,-0.968134671998613,
125.982338394538));
#246970=CARTESIAN_POINT('Ctrl Pts',(-183.110439019824,-1.10255886667133,
126.009327221549));
#246971=CARTESIAN_POINT('Ctrl Pts',(-183.11821192009,-1.2357112082651,126.041912712826));
#246972=CARTESIAN_POINT('Ctrl Pts',(-183.125984820355,-1.36710228659016,
126.079933202471));
#246973=CARTESIAN_POINT('Ctrl Pts',(-183.133475156117,-1.49371696826858,
126.116571551551));
#246974=CARTESIAN_POINT('Ctrl Pts',(-183.14096549188,-1.61869592401328,
126.158256510196));
#246975=CARTESIAN_POINT('Ctrl Pts',(-183.148455827642,-1.74162011162668,
126.204801676833));
#246976=CARTESIAN_POINT('Ctrl Pts',(-183.15623038486,-1.86920866845707,
126.253113003952));
#246977=CARTESIAN_POINT('Ctrl Pts',(-183.164004942078,-1.99498761497027,
126.306813704835));
#246978=CARTESIAN_POINT('Ctrl Pts',(-183.171779499296,-2.11846807574788,
126.365748663978));
#246979=CARTESIAN_POINT('Ctrl Pts',(-183.179544423664,-2.24179554147299,
126.424610601388));
#246980=CARTESIAN_POINT('Ctrl Pts',(-183.187309348032,-2.36282983852742,
126.488693725991));
#246981=CARTESIAN_POINT('Ctrl Pts',(-183.195074272399,-2.48109933137568,
126.557793866607));
#246982=CARTESIAN_POINT('Ctrl Pts',(-183.202831433245,-2.59925057609296,
126.626824919564));
#246983=CARTESIAN_POINT('Ctrl Pts',(-183.210588594091,-2.71464218244685,
126.700862809964));
#246984=CARTESIAN_POINT('Ctrl Pts',(-183.218345754937,-2.82682484457249,
126.779656360033));
#246985=CARTESIAN_POINT('Ctrl Pts',(-183.226097014844,-2.93892216838622,
126.858389971173));
#246986=CARTESIAN_POINT('Ctrl Pts',(-183.233848274751,-3.04781508831774,
126.941871817109));
#246987=CARTESIAN_POINT('Ctrl Pts',(-183.241599534659,-3.15308146877894,
127.029806297684));
#246988=CARTESIAN_POINT('Ctrl Pts',(-183.249347240883,-3.25829958826959,
127.11770046336));
#246989=CARTESIAN_POINT('Ctrl Pts',(-183.257094947108,-3.35989417716957,
127.210042951671));
#246990=CARTESIAN_POINT('Ctrl Pts',(-183.264842653332,-3.45747473226868,
127.30649676398));
#246991=CARTESIAN_POINT('Ctrl Pts',(-183.272588665805,-3.55503395496101,
127.402929490203));
#246992=CARTESIAN_POINT('Ctrl Pts',(-183.280334678278,-3.6485806119105,
127.503471477585));
#246993=CARTESIAN_POINT('Ctrl Pts',(-183.28808069075,-3.73776002458828,
127.607747869501));
#246994=CARTESIAN_POINT('Ctrl Pts',(-183.295826687299,-3.82693925393412,
127.71202404705));
#246995=CARTESIAN_POINT('Ctrl Pts',(-183.303572683848,-3.91175100311841,
127.820034316536));
#246996=CARTESIAN_POINT('Ctrl Pts',(-183.311318680397,-3.9918802286738,
127.931369962791));
#246997=CARTESIAN_POINT('Ctrl Pts',(-183.319066338468,-4.07202664200908,
128.042729490627));
#246998=CARTESIAN_POINT('Ctrl Pts',(-183.326813996539,-4.14748830531724,
128.157415497046));
#246999=CARTESIAN_POINT('Ctrl Pts',(-183.33456165461,-4.21799316285316,
128.274989798444));
#247000=CARTESIAN_POINT('Ctrl Pts',(-183.342316556619,-4.28856394132185,
128.392674029965));
#247001=CARTESIAN_POINT('Ctrl Pts',(-183.350071458629,-4.35416845854172,
128.5132516133));
#247002=CARTESIAN_POINT('Ctrl Pts',(-183.357826360638,-4.4145801711371,
128.636258919051));
#247003=CARTESIAN_POINT('Ctrl Pts',(-183.365585372232,-4.47502389793923,
128.759331410527));
#247004=CARTESIAN_POINT('Ctrl Pts',(-183.373344383826,-4.53026917973013,
128.884835832641));
#247005=CARTESIAN_POINT('Ctrl Pts',(-183.38110339542,-4.58013779618434,
129.012288958713));
#247006=CARTESIAN_POINT('Ctrl Pts',(-183.388872575828,-4.63007176950502,
129.139909122444));
#247007=CARTESIAN_POINT('Ctrl Pts',(-183.396641756236,-4.67461487900791,
129.269482721212));
#247008=CARTESIAN_POINT('Ctrl Pts',(-183.404410936644,-4.71363875007996,
129.400511339244));
#247009=CARTESIAN_POINT('Ctrl Pts',(-183.407990344031,-4.73161778069228,
129.460878685434));
#247010=CARTESIAN_POINT('Ctrl Pts',(-183.411569751418,-4.74842600050534,
129.52155472689));
#247011=CARTESIAN_POINT('Ctrl Pts',(-183.415149158805,-4.76405452823414,
129.582490119309));
#247012=CARTESIAN_POINT('',(-181.389859436049,-4.91824915695527,130.807240306567));
#247013=CARTESIAN_POINT('Ctrl Pts',(-181.389859436049,-4.91824915695527,
130.807240306567));
#247014=CARTESIAN_POINT('Ctrl Pts',(-181.398817739788,-4.91815613411647,
130.966114927541));
#247015=CARTESIAN_POINT('Ctrl Pts',(-181.407776043528,-4.91036021059812,
131.124708256897));
#247016=CARTESIAN_POINT('Ctrl Pts',(-181.416734347267,-4.89497108865333,
131.282315744903));
#247017=CARTESIAN_POINT('Ctrl Pts',(-181.425417497863,-4.88005464160356,
131.43508233925));
#247018=CARTESIAN_POINT('Ctrl Pts',(-181.434100648459,-4.8580046953391,
131.58692260436));
#247019=CARTESIAN_POINT('Ctrl Pts',(-181.442783799056,-4.82897206538774,
131.737212081736));
#247020=CARTESIAN_POINT('Ctrl Pts',(-181.451879679367,-4.79855944910979,
131.89464515665));
#247021=CARTESIAN_POINT('Ctrl Pts',(-181.460975559678,-4.76048430540328,
132.050376121223));
#247022=CARTESIAN_POINT('Ctrl Pts',(-181.47007143999,-4.71497645596076,
132.203710495987));
#247023=CARTESIAN_POINT('Ctrl Pts',(-181.479167320301,-4.66946860651813,
132.35704487075));
#247024=CARTESIAN_POINT('Ctrl Pts',(-181.488263200613,-4.61652822818693,
132.507982437687));
#247025=CARTESIAN_POINT('Ctrl Pts',(-181.497359080924,-4.5564403008889,
132.65585591784));
#247026=CARTESIAN_POINT('Ctrl Pts',(-181.505133415044,-4.50508258647963,
132.782244766713));
#247027=CARTESIAN_POINT('Ctrl Pts',(-181.512907749162,-4.44838078293223,
132.906695307599));
#247028=CARTESIAN_POINT('Ctrl Pts',(-181.520682083282,-4.386501677665,133.028722569754));
#247029=CARTESIAN_POINT('Ctrl Pts',(-181.528446836229,-4.32469883286472,
133.150599444214));
#247030=CARTESIAN_POINT('Ctrl Pts',(-181.536211589176,-4.25773155688373,
133.27005863679));
#247031=CARTESIAN_POINT('Ctrl Pts',(-181.543976342123,-4.18581526386889,
133.386633577433));
#247032=CARTESIAN_POINT('Ctrl Pts',(-181.551733383008,-4.11397039913011,
133.503092734203));
#247033=CARTESIAN_POINT('Ctrl Pts',(-181.559490423893,-4.0371865032356,
133.616673009293));
#247034=CARTESIAN_POINT('Ctrl Pts',(-181.567247464778,-3.95572544889312,
133.72693127291));
#247035=CARTESIAN_POINT('Ctrl Pts',(-181.574998656018,-3.87432582496551,
133.837106389913));
#247036=CARTESIAN_POINT('Ctrl Pts',(-181.582749847258,-3.78825629441504,
133.943964168621));
#247037=CARTESIAN_POINT('Ctrl Pts',(-181.590501038498,-3.69782249121197,
134.047089697521));
#247038=CARTESIAN_POINT('Ctrl Pts',(-181.598248935275,-3.60742712478753,
134.150171395321));
#247039=CARTESIAN_POINT('Ctrl Pts',(-181.605996832053,-3.51267143226317,
134.249523705019));
#247040=CARTESIAN_POINT('Ctrl Pts',(-181.61374472883,-3.41390170930395,
134.344764292532));
#247041=CARTESIAN_POINT('Ctrl Pts',(-181.621491004914,-3.31515264684154,
134.439984957767));
#247042=CARTESIAN_POINT('Ctrl Pts',(-181.629237280998,-3.21239150530955,
134.531095340363));
#247043=CARTESIAN_POINT('Ctrl Pts',(-181.636983557082,-3.10600158262843,
134.617749822881));
#247044=CARTESIAN_POINT('Ctrl Pts',(-181.644729890347,-2.99961087460092,
134.704404945062));
#247045=CARTESIAN_POINT('Ctrl Pts',(-181.652476223613,-2.88959163510988,
134.786603854625));
#247046=CARTESIAN_POINT('Ctrl Pts',(-181.660222556878,-2.77636007621668,
134.864041367291));
#247047=CARTESIAN_POINT('Ctrl Pts',(-181.667970624881,-2.66310315990082,
134.941496221552));
#247048=CARTESIAN_POINT('Ctrl Pts',(-181.675718692884,-2.54663281535994,
135.01418733648));
#247049=CARTESIAN_POINT('Ctrl Pts',(-181.683466760887,-2.4273937005275,
135.081853210796));
#247050=CARTESIAN_POINT('Ctrl Pts',(-181.691223063629,-2.30802785694534,
135.149591001208));
#247051=CARTESIAN_POINT('Ctrl Pts',(-181.698979366371,-2.18588770531916,
135.212292688746));
#247052=CARTESIAN_POINT('Ctrl Pts',(-181.706735669113,-2.06144243552465,
135.269742812577));
#247053=CARTESIAN_POINT('Ctrl Pts',(-181.714496111627,-1.93693074554234,
135.327223599268));
#247054=CARTESIAN_POINT('Ctrl Pts',(-181.722256554141,-1.81011184722903,
135.379447088406));
#247055=CARTESIAN_POINT('Ctrl Pts',(-181.730016996655,-1.68147337978646,
135.426246632557));
#247056=CARTESIAN_POINT('Ctrl Pts',(-181.737789896921,-1.55262841045597,
135.473121303491));
#247057=CARTESIAN_POINT('Ctrl Pts',(-181.745562797186,-1.42195840793301,
135.514554511845));
#247058=CARTESIAN_POINT('Ctrl Pts',(-181.753335697452,-1.28996545172147,
135.550429748527));
#247059=CARTESIAN_POINT('Ctrl Pts',(-181.760826033214,-1.16277077193805,
135.585000829992));
#247060=CARTESIAN_POINT('Ctrl Pts',(-181.768316368976,-1.03434795419006,
135.614410947926));
#247061=CARTESIAN_POINT('Ctrl Pts',(-181.775806704738,-0.905151846678698,
135.638601322884));
#247062=CARTESIAN_POINT('Ctrl Pts',(-181.783581038857,-0.771057229483291,
135.663708883261));
#247063=CARTESIAN_POINT('Ctrl Pts',(-181.791355372976,-0.635704754977355,
135.68327260728));
#247064=CARTESIAN_POINT('Ctrl Pts',(-181.799129707095,-0.499592595456683,
135.697170679388));
#247065=CARTESIAN_POINT('Ctrl Pts',(-181.806894460042,-0.363648182007928,
135.711051623364));
#247066=CARTESIAN_POINT('Ctrl Pts',(-181.814659212989,-0.226946331599816,
135.719280769009));
#247067=CARTESIAN_POINT('Ctrl Pts',(-181.822423965936,-0.08999601943478,
135.721787157839));
#247068=CARTESIAN_POINT('Ctrl Pts',(-181.830181006821,0.0468182717495528,
135.724291057289));
#247069=CARTESIAN_POINT('Ctrl Pts',(-181.837938047706,0.18388014522574,
135.721083504079));
#247070=CARTESIAN_POINT('Ctrl Pts',(-181.845695088591,0.320675234751949,
135.712145296657));
#247071=CARTESIAN_POINT('Ctrl Pts',(-181.853446279831,0.457367166036849,
135.703213829606));
#247072=CARTESIAN_POINT('Ctrl Pts',(-181.861197471071,0.593792325261312,
135.688560335476));
#247073=CARTESIAN_POINT('Ctrl Pts',(-181.868948662312,0.7294364329914,135.668217682975));
#247074=CARTESIAN_POINT('Ctrl Pts',(-181.876696559089,0.865022888357463,
135.647883676643));
#247075=CARTESIAN_POINT('Ctrl Pts',(-181.884444455866,0.999828566655742,
135.621865379108));
#247076=CARTESIAN_POINT('Ctrl Pts',(-181.892192352643,1.13334461812831,
135.59024747781));
#247077=CARTESIAN_POINT('Ctrl Pts',(-181.899938628727,1.26683274092118,
135.558636190296));
#247078=CARTESIAN_POINT('Ctrl Pts',(-181.907684904811,1.39903139325775,
135.521427718866));
#247079=CARTESIAN_POINT('Ctrl Pts',(-181.915431180895,1.5294426155094,135.478757728249));
#247080=CARTESIAN_POINT('Ctrl Pts',(-181.92317751416,1.65985480042725,135.436087422652));
#247081=CARTESIAN_POINT('Ctrl Pts',(-181.930923847426,1.78847915735103,
135.387955639));
#247082=CARTESIAN_POINT('Ctrl Pts',(-181.938670180691,1.91483395331802,
135.334547588732));
#247083=CARTESIAN_POINT('Ctrl Pts',(-181.946418248694,2.0412170455653,135.281127578101));
#247084=CARTESIAN_POINT('Ctrl Pts',(-181.954166316697,2.16532920544419,
135.222429101825));
#247085=CARTESIAN_POINT('Ctrl Pts',(-181.9619143847,2.2867100760472,135.158684915388));
#247086=CARTESIAN_POINT('Ctrl Pts',(-181.969670687442,2.40821995168409,
135.094872980871));
#247087=CARTESIAN_POINT('Ctrl Pts',(-181.977426990184,2.52699239260691,
135.026004805807));
#247088=CARTESIAN_POINT('Ctrl Pts',(-181.985183292925,2.64259251692664,
134.952358671083));
#247089=CARTESIAN_POINT('Ctrl Pts',(-181.99294373544,2.75825434051338,134.8786732292));
#247090=CARTESIAN_POINT('Ctrl Pts',(-182.000704177954,2.87074015323274,
134.80020496986));
#247091=CARTESIAN_POINT('Ctrl Pts',(-182.008464620468,2.97964616898119,
134.717274080726));
#247092=CARTESIAN_POINT('Ctrl Pts',(-182.016237520733,3.08872701033434,
134.634210063566));
#247093=CARTESIAN_POINT('Ctrl Pts',(-182.024010420999,3.19421627012777,
134.546669350855));
#247094=CARTESIAN_POINT('Ctrl Pts',(-182.031783321264,3.29574453972754,
134.455011380287));
#247095=CARTESIAN_POINT('Ctrl Pts',(-182.039273657026,3.39358200099335,
134.366685407822));
#247096=CARTESIAN_POINT('Ctrl Pts',(-182.046763992788,3.48774123604373,
134.274536541253));
#247097=CARTESIAN_POINT('Ctrl Pts',(-182.05425432855,3.57792693550293,134.178915685527));
#247098=CARTESIAN_POINT('Ctrl Pts',(-182.062028662669,3.67153205316809,
134.079669335994));
#247099=CARTESIAN_POINT('Ctrl Pts',(-182.069802996788,3.76115288689754,
133.976368136514));
#247100=CARTESIAN_POINT('Ctrl Pts',(-182.077577330907,3.84641767552078,
133.869365369266));
#247101=CARTESIAN_POINT('Ctrl Pts',(-182.085342083855,3.93157738291237,
133.762494473365));
#247102=CARTESIAN_POINT('Ctrl Pts',(-182.093106836802,4.01239148547918,
133.651931389249));
#247103=CARTESIAN_POINT('Ctrl Pts',(-182.100871589749,4.0885251703094,133.538065977375));
#247104=CARTESIAN_POINT('Ctrl Pts',(-182.108628630634,4.16458323809056,
133.424313658233));
#247105=CARTESIAN_POINT('Ctrl Pts',(-182.116385671519,4.23596992326855,
133.307265861425));
#247106=CARTESIAN_POINT('Ctrl Pts',(-182.124142712404,4.30239104351552,
133.187344958928));
#247107=CARTESIAN_POINT('Ctrl Pts',(-182.131893903644,4.36876207507913,
133.067514489717));
#247108=CARTESIAN_POINT('Ctrl Pts',(-182.139645094884,4.43017480638999,
132.944815567991));
#247109=CARTESIAN_POINT('Ctrl Pts',(-182.147396286124,4.48637891022631,
132.819698637943));
#247110=CARTESIAN_POINT('Ctrl Pts',(-182.155144182901,4.54255912581914,
132.694634885927));
#247111=CARTESIAN_POINT('Ctrl Pts',(-182.162892079678,4.59353495715868,
132.56715552553));
#247112=CARTESIAN_POINT('Ctrl Pts',(-182.170639976455,4.639102608463,132.437734442094));
#247113=CARTESIAN_POINT('Ctrl Pts',(-182.178386252539,4.68466072799699,
132.308340430758));
#247114=CARTESIAN_POINT('Ctrl Pts',(-182.186132528623,4.724812787904,132.177005872811));
#247115=CARTESIAN_POINT('Ctrl Pts',(-182.193878804708,4.75940376741928,
132.044223045892));
#247116=CARTESIAN_POINT('Ctrl Pts',(-182.201625137973,4.79399500227735,
131.911439238801));
#247117=CARTESIAN_POINT('Ctrl Pts',(-182.209371471238,4.82302497627006,
131.777207519742));
#247118=CARTESIAN_POINT('Ctrl Pts',(-182.217117804504,4.8463891245921,131.642033295606));
#247119=CARTESIAN_POINT('Ctrl Pts',(-182.224865872507,4.86975850515314,
131.506828800141));
#247120=CARTESIAN_POINT('Ctrl Pts',(-182.23261394051,4.88745946865773,131.370681764779));
#247121=CARTESIAN_POINT('Ctrl Pts',(-182.240362008513,4.89943900473265,
131.234105310848));
#247122=CARTESIAN_POINT('Ctrl Pts',(-182.248118311254,4.91143127280104,
131.097383701837));
#247123=CARTESIAN_POINT('Ctrl Pts',(-182.255874613996,4.91768993216839,
130.960232152658));
#247124=CARTESIAN_POINT('Ctrl Pts',(-182.263630916738,4.91821404414322,
130.823166959378));
#247125=CARTESIAN_POINT('Ctrl Pts',(-182.271391359252,4.9187384358524,130.686028610276));
#247126=CARTESIAN_POINT('Ctrl Pts',(-182.279151801766,4.91352219632619,
130.548977099404));
#247127=CARTESIAN_POINT('Ctrl Pts',(-182.28691224428,4.90261645226236,130.4125252127));
#247128=CARTESIAN_POINT('Ctrl Pts',(-182.294685144546,4.89169320132999,
130.275854281314));
#247129=CARTESIAN_POINT('Ctrl Pts',(-182.302458044811,4.8750622420806,130.139785285917));
#247130=CARTESIAN_POINT('Ctrl Pts',(-182.310230945077,4.85282630523814,
130.004823305311));
#247131=CARTESIAN_POINT('Ctrl Pts',(-182.317721280839,4.83139870070879,
129.874767532648));
#247132=CARTESIAN_POINT('Ctrl Pts',(-182.325211616601,4.80476661598463,
129.74573998823));
#247133=CARTESIAN_POINT('Ctrl Pts',(-182.332701952363,4.77306565540504,
129.618178796894));
#247134=CARTESIAN_POINT('Ctrl Pts',(-182.340476286482,4.74016274326992,
129.485781084218));
#247135=CARTESIAN_POINT('Ctrl Pts',(-182.348250620601,4.70169476824667,
129.354543717016));
#247136=CARTESIAN_POINT('Ctrl Pts',(-182.35602495472,4.65775801064424,129.224970426138));
#247137=CARTESIAN_POINT('Ctrl Pts',(-182.363789707667,4.61387540116881,
129.09555682276));
#247138=CARTESIAN_POINT('Ctrl Pts',(-182.371554460614,4.56453754362383,
128.967803581878));
#247139=CARTESIAN_POINT('Ctrl Pts',(-182.379319213561,4.50989146409757,
128.842203120177));
#247140=CARTESIAN_POINT('Ctrl Pts',(-182.387076254446,4.45529965982786,
128.716727406625));
#247141=CARTESIAN_POINT('Ctrl Pts',(-182.394833295331,4.39541028046255,
128.593400573383));
#247142=CARTESIAN_POINT('Ctrl Pts',(-182.402590336216,4.33041966677546,
128.472698426745));
#247143=CARTESIAN_POINT('Ctrl Pts',(-182.410341527457,4.26547806301561,
128.352087302535));
#247144=CARTESIAN_POINT('Ctrl Pts',(-182.418092718697,4.19544306651655,
128.234097268103));
#247145=CARTESIAN_POINT('Ctrl Pts',(-182.425843909937,4.1205583407563,128.119182406921));
#247146=CARTESIAN_POINT('Ctrl Pts',(-182.433591806714,4.04570544300221,
128.00431638762));
#247147=CARTESIAN_POINT('Ctrl Pts',(-182.441339703491,3.96600712868981,
127.892523268852));
#247148=CARTESIAN_POINT('Ctrl Pts',(-182.449087600268,3.88175193438076,
127.784230656384));
#247149=CARTESIAN_POINT('Ctrl Pts',(-182.456833876352,3.79751436444203,
127.675960696395));
#247150=CARTESIAN_POINT('Ctrl Pts',(-182.464580152436,3.70872205040214,
127.571190094635));
#247151=CARTESIAN_POINT('Ctrl Pts',(-182.47232642852,3.61570536686982,127.470315362551));
#247152=CARTESIAN_POINT('Ctrl Pts',(-182.480072761786,3.52268799670936,
127.369439885832));
#247153=CARTESIAN_POINT('Ctrl Pts',(-182.487819095051,3.42544645986479,
127.272460623597));
#247154=CARTESIAN_POINT('Ctrl Pts',(-182.495565428317,3.32434944963606,
127.179738733948));
#247155=CARTESIAN_POINT('Ctrl Pts',(-182.50331349632,3.22322979943299,127.086996079874));
#247156=CARTESIAN_POINT('Ctrl Pts',(-182.511061564323,3.11825324584275,
126.998512959771));
#247157=CARTESIAN_POINT('Ctrl Pts',(-182.518809632326,3.00982283896963,
126.914611327378));
#247158=CARTESIAN_POINT('Ctrl Pts',(-182.526565935067,2.9012771909699,126.830620523332));
#247159=CARTESIAN_POINT('Ctrl Pts',(-182.534322237809,2.78927066657606,
126.751221173508));
#247160=CARTESIAN_POINT('Ctrl Pts',(-182.542078540551,2.67423713290575,
126.676693138288));
#247161=CARTESIAN_POINT('Ctrl Pts',(-182.549838983065,2.55914220237462,
126.602125325212));
#247162=CARTESIAN_POINT('Ctrl Pts',(-182.557599425579,2.44101737989998,
126.532434205961));
#247163=CARTESIAN_POINT('Ctrl Pts',(-182.565359868094,2.32032172204335,
126.467853939523));
#247164=CARTESIAN_POINT('Ctrl Pts',(-182.573132768359,2.19943231280187,
126.403170003107));
#247165=CARTESIAN_POINT('Ctrl Pts',(-182.580905668624,2.07596417359235,
126.343613484455));
#247166=CARTESIAN_POINT('Ctrl Pts',(-182.58867856889,1.95039776998001,126.289370960728));
#247167=CARTESIAN_POINT('Ctrl Pts',(-182.596168904652,1.82939602142133,
126.237100289366));
#247168=CARTESIAN_POINT('Ctrl Pts',(-182.603659240414,1.70644620173451,
126.189764077074));
#247169=CARTESIAN_POINT('Ctrl Pts',(-182.611149576176,1.5819902152108,126.147485053255));
#247170=CARTESIAN_POINT('Ctrl Pts',(-182.618923910295,1.45281544213099,
126.103603007398));
#247171=CARTESIAN_POINT('Ctrl Pts',(-182.626698244414,1.3216088481364,126.065030201631));
#247172=CARTESIAN_POINT('Ctrl Pts',(-182.634472578533,1.18884627811505,
126.031957911432));
#247173=CARTESIAN_POINT('Ctrl Pts',(-182.64223733148,1.05624732609592,125.998926379875));
#247174=CARTESIAN_POINT('Ctrl Pts',(-182.650002084427,0.922096589234707,
125.971381969506));
#247175=CARTESIAN_POINT('Ctrl Pts',(-182.657766837375,0.786887822827249,
125.949467146357));
#247176=CARTESIAN_POINT('Ctrl Pts',(-182.66552387826,0.651813347672695,
125.92757408932));
#247177=CARTESIAN_POINT('Ctrl Pts',(-182.673280919145,0.515683317642029,
125.911299554543));
#247178=CARTESIAN_POINT('Ctrl Pts',(-182.68103796003,0.379004169031384,
125.900735539896));
#247179=CARTESIAN_POINT('Ctrl Pts',(-182.68878915127,0.242428091229729,
125.890179491655));
#247180=CARTESIAN_POINT('Ctrl Pts',(-182.69654034251,0.105304107303662,
125.885325422026));
#247181=CARTESIAN_POINT('Ctrl Pts',(-182.70429153375,-0.0318540434016616,
125.886213773233));
#247182=CARTESIAN_POINT('Ctrl Pts',(-182.712039430527,-0.168953898234309,
125.887101746867));
#247183=CARTESIAN_POINT('Ctrl Pts',(-182.719787327304,-0.306087500824971,
125.893727284479));
#247184=CARTESIAN_POINT('Ctrl Pts',(-182.727535224081,-0.442739133272749,
125.906078763449));
#247185=CARTESIAN_POINT('Ctrl Pts',(-182.735281500165,-0.579362181144514,
125.918427658756));
#247186=CARTESIAN_POINT('Ctrl Pts',(-182.743027776249,-0.715503070274265,
125.936500077871));
#247187=CARTESIAN_POINT('Ctrl Pts',(-182.750774052334,-0.85064962880552,
125.960232391403));
#247188=CARTESIAN_POINT('Ctrl Pts',(-182.758520385599,-0.985797184958153,
125.98396488012));
#247189=CARTESIAN_POINT('Ctrl Pts',(-182.766266718864,-1.11995001079294,
126.013357279003));
#247190=CARTESIAN_POINT('Ctrl Pts',(-182.77401305213,-1.25260496603569,
126.048294610711));
#247191=CARTESIAN_POINT('Ctrl Pts',(-182.781761120133,-1.38528962843572,
126.083239766392));
#247192=CARTESIAN_POINT('Ctrl Pts',(-182.789509188136,-1.51647537476105,
126.123732226282));
#247193=CARTESIAN_POINT('Ctrl Pts',(-182.797257256139,-1.6456734777856,
126.169606916773));
#247194=CARTESIAN_POINT('Ctrl Pts',(-182.80501355888,-1.7750088940917,126.215530363432));
#247195=CARTESIAN_POINT('Ctrl Pts',(-182.812769861622,-1.902352078152,126.266847336577));
#247196=CARTESIAN_POINT('Ctrl Pts',(-182.820526164364,-2.02723305972525,
126.323344082888));
#247197=CARTESIAN_POINT('Ctrl Pts',(-182.828286606878,-2.15218069403846,
126.379870983214));
#247198=CARTESIAN_POINT('Ctrl Pts',(-182.836047049393,-2.27466315832567,
126.441582989575));
#247199=CARTESIAN_POINT('Ctrl Pts',(-182.843807491907,-2.39423531671549,
126.508220453338));
#247200=CARTESIAN_POINT('Ctrl Pts',(-182.851580392172,-2.51399942294907,
126.574964889473));
#247201=CARTESIAN_POINT('Ctrl Pts',(-182.859353292438,-2.63084355393906,
126.646650378709));
#247202=CARTESIAN_POINT('Ctrl Pts',(-182.867126192703,-2.74435103366134,
126.722973541272));
#247203=CARTESIAN_POINT('Ctrl Pts',(-182.874616528465,-2.85373223058731,
126.796522164628));
#247204=CARTESIAN_POINT('Ctrl Pts',(-182.882106864227,-2.9600149073766,
126.874376951055));
#247205=CARTESIAN_POINT('Ctrl Pts',(-182.889597199989,-3.06285694824154,
126.956232452197));
#247206=CARTESIAN_POINT('Ctrl Pts',(-182.897271718051,-3.16822780545898,
127.040100724848));
#247207=CARTESIAN_POINT('Ctrl Pts',(-182.904946236112,-3.27033860869109,
127.128449457481));
#247208=CARTESIAN_POINT('Ctrl Pts',(-182.912620754173,-3.36877703830128,
127.220992881942));
#247209=CARTESIAN_POINT('Ctrl Pts',(-182.920286491824,-3.46710284456976,
127.313430427532));
#247210=CARTESIAN_POINT('Ctrl Pts',(-182.927952229474,-3.56176434009002,
127.410052852803));
#247211=CARTESIAN_POINT('Ctrl Pts',(-182.935617967125,-3.65237997082311,
127.510532508628));
#247212=CARTESIAN_POINT('Ctrl Pts',(-182.943276696308,-3.74291275542632,
127.610920300052));
#247213=CARTESIAN_POINT('Ctrl Pts',(-182.95093542549,-3.82940676294885,
127.715158013987));
#247214=CARTESIAN_POINT('Ctrl Pts',(-182.958594154673,-3.9115156180739,
127.822879671448));
#247215=CARTESIAN_POINT('Ctrl Pts',(-182.966247640976,-3.99356826453599,
127.930527586676));
#247216=CARTESIAN_POINT('Ctrl Pts',(-182.973901127278,-4.07124148666013,
128.041654383705));
#247217=CARTESIAN_POINT('Ctrl Pts',(-182.98155461358,-4.14422807866773,
128.15585977851));
#247218=CARTESIAN_POINT('Ctrl Pts',(-182.989205542012,-4.2171902778377,
128.270027004747));
#247219=CARTESIAN_POINT('Ctrl Pts',(-182.996856470444,-4.28546874152419,
128.387270447522));
#247220=CARTESIAN_POINT('Ctrl Pts',(-183.004507398876,-4.34879885726115,
128.50715980754));
#247221=CARTESIAN_POINT('Ctrl Pts',(-183.012156622058,-4.41211485788887,
128.627022446441));
#247222=CARTESIAN_POINT('Ctrl Pts',(-183.019805845239,-4.47048452011149,
128.749529472692));
#247223=CARTESIAN_POINT('Ctrl Pts',(-183.027455068421,-4.52368893671273,
128.874225527381));
#247224=CARTESIAN_POINT('Ctrl Pts',(-183.035106947243,-4.57691182470863,
128.998964873778));
#247225=CARTESIAN_POINT('Ctrl Pts',(-183.042758826066,-4.62496572459593,
129.125894397969));
#247226=CARTESIAN_POINT('Ctrl Pts',(-183.050410704888,-4.66767971122647,
129.254538312944));
#247227=CARTESIAN_POINT('Ctrl Pts',(-183.056846671858,-4.7036062873606,
129.362740233909));
#247228=CARTESIAN_POINT('Ctrl Pts',(-183.063282638827,-4.73575598385233,
129.472154524254));
#247229=CARTESIAN_POINT('Ctrl Pts',(-183.069718605797,-4.76405452823406,
129.582490119308));
#247230=CARTESIAN_POINT('Ctrl Pts',(-181.320039938991,-4.76405452823418,
129.582490119309));
#247231=CARTESIAN_POINT('Ctrl Pts',(-181.327866674491,-4.79848591795568,
129.716737585264));
#247232=CARTESIAN_POINT('Ctrl Pts',(-181.33569340999,-4.82725862397902,
129.852519526693));
#247233=CARTESIAN_POINT('Ctrl Pts',(-181.34352014549,-4.8502474171004,129.989325001528));
#247234=CARTESIAN_POINT('Ctrl Pts',(-181.351344753954,-4.8732299626622,
130.126093297362));
#247235=CARTESIAN_POINT('Ctrl Pts',(-181.359169362417,-4.89043165683097,
130.263884199659));
#247236=CARTESIAN_POINT('Ctrl Pts',(-181.366993970881,-4.90177834412933,
130.40217642155));
#247237=CARTESIAN_POINT('Ctrl Pts',(-181.374615792586,-4.91283096458077,
130.536884587887));
#247238=CARTESIAN_POINT('Ctrl Pts',(-181.38223761429,-4.91832830176703,
130.672068059881));
#247239=CARTESIAN_POINT('Ctrl Pts',(-181.389859435995,-4.91824915695583,
130.807240305618));
#247240=CARTESIAN_POINT('Origin',(213.235140564004,0.,130.804360617566));
#247241=CARTESIAN_POINT('',(-179.570054719422,-4.76405452823393,129.582490119308));
#247242=CARTESIAN_POINT('',(-179.915287826822,-4.76405452823417,129.582490119309));
#247243=CARTESIAN_POINT('',(213.235140564004,-4.76405452823405,129.582490119308));
#247244=CARTESIAN_POINT('',(-179.985140564067,-4.91824883331974,130.807748249335));
#247245=CARTESIAN_POINT('Ctrl Pts',(-179.915287826822,-4.76405452823417,
129.582490119309));
#247246=CARTESIAN_POINT('Ctrl Pts',(-179.92306888399,-4.79829769999019,
129.716003726273));
#247247=CARTESIAN_POINT('Ctrl Pts',(-179.930849941158,-4.82693968418732,
129.851018898772));
#247248=CARTESIAN_POINT('Ctrl Pts',(-179.938630998326,-4.84986100741504,
129.987028817588));
#247249=CARTESIAN_POINT('Ctrl Pts',(-179.946411829481,-4.87278166485761,
130.123034785786));
#247250=CARTESIAN_POINT('Ctrl Pts',(-179.954192660636,-4.88998191732996,
130.260035064349));
#247251=CARTESIAN_POINT('Ctrl Pts',(-179.961973491791,-4.90139348051783,
130.397512965935));
#247252=CARTESIAN_POINT('Ctrl Pts',(-179.969695849198,-4.91271928463228,
130.533957706923));
#247253=CARTESIAN_POINT('Ctrl Pts',(-179.977418206605,-4.91834311166686,
130.670872539273));
#247254=CARTESIAN_POINT('Ctrl Pts',(-179.985140564012,-4.91824883332041,
130.807748248363));
#247255=CARTESIAN_POINT('Ctrl Pts',(-179.985140564067,-4.91824883331974,
130.807748249336));
#247256=CARTESIAN_POINT('Ctrl Pts',(-179.993960729007,-4.91814115236676,
130.964082159672));
#247257=CARTESIAN_POINT('Ctrl Pts',(-180.002780893947,-4.91057552406498,
131.120123073993));
#247258=CARTESIAN_POINT('Ctrl Pts',(-180.011601058887,-4.89565957716396,
131.27521130199));
#247259=CARTESIAN_POINT('Ctrl Pts',(-180.020460543816,-4.88067713548981,
131.43099090792));
#247260=CARTESIAN_POINT('Ctrl Pts',(-180.029320028745,-4.85827880522494,
131.585809153203));
#247261=CARTESIAN_POINT('Ctrl Pts',(-180.038179513674,-4.82862329315814,
131.739015717199));
#247262=CARTESIAN_POINT('Ctrl Pts',(-180.047091538771,-4.79879191244734,
131.893130855312));
#247263=CARTESIAN_POINT('Ctrl Pts',(-180.056003563869,-4.7616171115927,
132.045614980022));
#247264=CARTESIAN_POINT('Ctrl Pts',(-180.064915588966,-4.71730902760369,
132.195826966634));
#247265=CARTESIAN_POINT('Ctrl Pts',(-180.071787714544,-4.68314275069523,
132.311656491802));
#247266=CARTESIAN_POINT('Ctrl Pts',(-180.078659840122,-4.64473597477464,
132.426135393135));
#247267=CARTESIAN_POINT('Ctrl Pts',(-180.0855319657,-4.60220406385651,132.538978966691));
#247268=CARTESIAN_POINT('Ctrl Pts',(-180.093306299819,-4.55408834151546,
132.666637234001));
#247269=CARTESIAN_POINT('Ctrl Pts',(-180.101080633938,-4.50058080743443,
132.792494198247));
#247270=CARTESIAN_POINT('Ctrl Pts',(-180.108854968057,-4.44183581893942,
132.916060790433));
#247271=CARTESIAN_POINT('Ctrl Pts',(-180.116619721004,-4.3831632283927,
133.039475097838));
#247272=CARTESIAN_POINT('Ctrl Pts',(-180.124384473951,-4.31926619260353,
133.160604299769));
#247273=CARTESIAN_POINT('Ctrl Pts',(-180.132149226898,-4.25034814935119,
133.27897648105));
#247274=CARTESIAN_POINT('Ctrl Pts',(-180.139906267783,-4.1814985564708,
133.397231093413));
#247275=CARTESIAN_POINT('Ctrl Pts',(-180.147663308668,-4.10763807579476,
133.512733798804));
#247276=CARTESIAN_POINT('Ctrl Pts',(-180.155420349553,-4.02901718669648,
133.62503492911));
#247277=CARTESIAN_POINT('Ctrl Pts',(-180.163171540793,-3.95045558622215,
133.73725137226));
#247278=CARTESIAN_POINT('Ctrl Pts',(-180.170922732034,-3.8671409460421,
133.846270726925));
#247279=CARTESIAN_POINT('Ctrl Pts',(-180.178673923274,-3.77936821263246,
133.951670417354));
#247280=CARTESIAN_POINT('Ctrl Pts',(-180.186421820051,-3.69163278497605,
134.057025310104));
#247281=CARTESIAN_POINT('Ctrl Pts',(-180.194169716828,-3.5994432823843,
134.158763298683));
#247282=CARTESIAN_POINT('Ctrl Pts',(-180.201917613605,-3.50313613111719,
134.256493336533));
#247283=CARTESIAN_POINT('Ctrl Pts',(-180.209663889689,-3.40684912522998,
134.354202931366));
#247284=CARTESIAN_POINT('Ctrl Pts',(-180.217410165773,-3.30644645813239,
134.447905964751));
#247285=CARTESIAN_POINT('Ctrl Pts',(-180.225156441857,-3.20230248324751,
134.537247150571));
#247286=CARTESIAN_POINT('Ctrl Pts',(-180.232902775123,-3.0981577395956,
134.626588995887));
#247287=CARTESIAN_POINT('Ctrl Pts',(-180.240649108388,-2.99027192978512,
134.711568674828));
#247288=CARTESIAN_POINT('Ctrl Pts',(-180.248395441653,-2.8790533424594,
134.79187048135));
#247289=CARTESIAN_POINT('Ctrl Pts',(-180.256143509656,-2.76780984850203,
134.872190270904));
#247290=CARTESIAN_POINT('Ctrl Pts',(-180.263891577659,-2.65323240879196,
134.947829874661));
#247291=CARTESIAN_POINT('Ctrl Pts',(-180.271639645662,-2.53575886331033,
135.018516529447));
#247292=CARTESIAN_POINT('Ctrl Pts',(-180.279395948404,-2.41816046554677,
135.089278310851));
#247293=CARTESIAN_POINT('Ctrl Pts',(-180.287152251146,-2.29766014887279,
135.155076425877));
#247294=CARTESIAN_POINT('Ctrl Pts',(-180.294908553888,-2.17472145211095,
135.215683510784));
#247295=CARTESIAN_POINT('Ctrl Pts',(-180.302668996402,-2.05171713926471,
135.276322943517));
#247296=CARTESIAN_POINT('Ctrl Pts',(-180.310429438916,-1.92627221052881,
135.331765667491));
#247297=CARTESIAN_POINT('Ctrl Pts',(-180.31818988143,-1.79886989369378,
135.381832645669));
#247298=CARTESIAN_POINT('Ctrl Pts',(-180.325962781696,-1.67126305934953,
135.431979995805));
#247299=CARTESIAN_POINT('Ctrl Pts',(-180.333735681961,-1.54169292759772,
135.476734227691));
#247300=CARTESIAN_POINT('Ctrl Pts',(-180.341508582227,-1.41065844128908,
135.515966057808));
#247301=CARTESIAN_POINT('Ctrl Pts',(-180.348998917989,-1.28438738861264,
135.553771712082));
#247302=CARTESIAN_POINT('Ctrl Pts',(-180.356489253751,-1.15675689732088,
135.586449423876));
#247303=CARTESIAN_POINT('Ctrl Pts',(-180.363979589513,-1.02822016752291,
135.613928825794));
#247304=CARTESIAN_POINT('Ctrl Pts',(-180.371753923632,-0.894809928547707,
135.642450117588));
#247305=CARTESIAN_POINT('Ctrl Pts',(-180.379528257751,-0.760000770908441,
135.665461477155));
#247306=CARTESIAN_POINT('Ctrl Pts',(-180.38730259187,-0.624287596106585,
135.682828415948));
#247307=CARTESIAN_POINT('Ctrl Pts',(-180.395067344817,-0.488741675663636,
135.700173951541));
#247308=CARTESIAN_POINT('Ctrl Pts',(-180.402832097764,-0.352294338905479,
135.711888858062));
#247309=CARTESIAN_POINT('Ctrl Pts',(-180.410596850712,-0.215452584523784,
135.717889211797));
#247310=CARTESIAN_POINT('Ctrl Pts',(-180.418353891597,-0.0787467433016716,
135.723883605896));
#247311=CARTESIAN_POINT('Ctrl Pts',(-180.426110932482,0.0583523478990269,
135.72417472524));
#247312=CARTESIAN_POINT('Ctrl Pts',(-180.433867973367,0.195330980338071,
135.718730248619));
#247313=CARTESIAN_POINT('Ctrl Pts',(-180.441619164607,0.332206316124668,
135.713289877721));
#247314=CARTESIAN_POINT('Ctrl Pts',(-180.449370355847,0.468960984882857,
135.702122535486));
#247315=CARTESIAN_POINT('Ctrl Pts',(-180.457121547087,0.605080035891566,
135.685247956223));
#247316=CARTESIAN_POINT('Ctrl Pts',(-180.464869443864,0.741141232672686,
135.668380549107));
#247317=CARTESIAN_POINT('Ctrl Pts',(-180.472617340641,0.876566961838184,
135.645810777549));
#247318=CARTESIAN_POINT('Ctrl Pts',(-180.480365237418,1.01084637823296,
135.617610316274));
#247319=CARTESIAN_POINT('Ctrl Pts',(-180.488111513502,1.14509770626855,
135.589415753928));
#247320=CARTESIAN_POINT('Ctrl Pts',(-180.495857789587,1.27820281610075,
135.555592924915));
#247321=CARTESIAN_POINT('Ctrl Pts',(-180.503604065671,1.40966044828803,
135.516264742549));
#247322=CARTESIAN_POINT('Ctrl Pts',(-180.511350398936,1.54111905086551,
135.476936269871));
#247323=CARTESIAN_POINT('Ctrl Pts',(-180.519096732201,1.67092977696887,
135.432102474804));
#247324=CARTESIAN_POINT('Ctrl Pts',(-180.526843065467,1.7986063241752,135.381936215318));
#247325=CARTESIAN_POINT('Ctrl Pts',(-180.53459113347,1.9263114636592,135.331758721446));
#247326=CARTESIAN_POINT('Ctrl Pts',(-180.542339201473,2.05188110939729,
135.276246529846));
#247327=CARTESIAN_POINT('Ctrl Pts',(-180.550087269476,2.17484911480286,
135.215620572538));
#247328=CARTESIAN_POINT('Ctrl Pts',(-180.557843572218,2.29794781206775,
135.154930181241));
#247329=CARTESIAN_POINT('Ctrl Pts',(-180.56559987496,2.41843899428399,135.089115340456));
#247330=CARTESIAN_POINT('Ctrl Pts',(-180.573356177701,2.53588081984257,
135.018443142868));
#247331=CARTESIAN_POINT('Ctrl Pts',(-180.581116620216,2.65338532763989,
134.9477332254));
#247332=CARTESIAN_POINT('Ctrl Pts',(-180.58887706273,2.76783690968252,134.87216100064));
#247333=CARTESIAN_POINT('Ctrl Pts',(-180.596637505244,2.87882374061796,
134.792036247924));
#247334=CARTESIAN_POINT('Ctrl Pts',(-180.604410405509,2.98998873746736,
134.711782871843));
#247335=CARTESIAN_POINT('Ctrl Pts',(-180.612183305775,3.09767756139703,
134.6269626059));
#247336=CARTESIAN_POINT('Ctrl Pts',(-180.61995620604,3.2015117517228,134.537925343948));
#247337=CARTESIAN_POINT('Ctrl Pts',(-180.627446541802,3.30157130768515,
134.452124810741));
#247338=CARTESIAN_POINT('Ctrl Pts',(-180.634936877564,3.39805139018646,
134.362408765159));
#247339=CARTESIAN_POINT('Ctrl Pts',(-180.642427213326,3.49064783141407,
134.269120461992));
#247340=CARTESIAN_POINT('Ctrl Pts',(-180.650201547445,3.58675509485719,
134.172295104453));
#247341=CARTESIAN_POINT('Ctrl Pts',(-180.657975881564,3.67898284597718,
134.071314544067));
#247342=CARTESIAN_POINT('Ctrl Pts',(-180.665750215683,3.76695042939966,
133.966522461138));
#247343=CARTESIAN_POINT('Ctrl Pts',(-180.67351496863,3.85480960063723,133.861859525086));
#247344=CARTESIAN_POINT('Ctrl Pts',(-180.681279721577,3.93841880170574,
133.75339470941));
#247345=CARTESIAN_POINT('Ctrl Pts',(-180.689044474525,4.01743338003051,
133.64150920365));
#247346=CARTESIAN_POINT('Ctrl Pts',(-180.69680151541,4.09636947996217,133.529734824151));
#247347=CARTESIAN_POINT('Ctrl Pts',(-180.704558556295,4.17071981453642,
133.414546832993));
#247348=CARTESIAN_POINT('Ctrl Pts',(-180.71231559718,4.24017951888239,133.296359957484));
#247349=CARTESIAN_POINT('Ctrl Pts',(-180.72006678842,4.30958684312489,133.178262207617));
#247350=CARTESIAN_POINT('Ctrl Pts',(-180.72781797966,4.37411068070913,133.057170410442));
#247351=CARTESIAN_POINT('Ctrl Pts',(-180.7355691709,4.433489291225,132.933528475461));
#247352=CARTESIAN_POINT('Ctrl Pts',(-180.743317067677,4.4928426642475,132.8099390916));
#247353=CARTESIAN_POINT('Ctrl Pts',(-180.751064964454,4.5470549907979,132.683802077373));
#247354=CARTESIAN_POINT('Ctrl Pts',(-180.758812861231,4.59591044856734,
132.555585963217));
#247355=CARTESIAN_POINT('Ctrl Pts',(-180.766559137315,4.64475568682821,
132.427396669107));
#247356=CARTESIAN_POINT('Ctrl Pts',(-180.774305413399,4.68824614600501,
132.297129505223));
#247357=CARTESIAN_POINT('Ctrl Pts',(-180.782051689483,4.72621429357663,
132.165272632978));
#247358=CARTESIAN_POINT('Ctrl Pts',(-180.789798022749,4.76418272142055,
132.033414787394));
#247359=CARTESIAN_POINT('Ctrl Pts',(-180.797544356014,4.79662864813414,
131.899967585733));
#247360=CARTESIAN_POINT('Ctrl Pts',(-180.80529068928,4.82343464568437,131.765433601949));
#247361=CARTESIAN_POINT('Ctrl Pts',(-180.813038757283,4.85024664625185,
131.630869490213));
#247362=CARTESIAN_POINT('Ctrl Pts',(-180.820786825286,4.87141612800267,
131.495218495417));
#247363=CARTESIAN_POINT('Ctrl Pts',(-180.828534893288,4.88687700368533,
131.358992219038));
#247364=CARTESIAN_POINT('Ctrl Pts',(-180.83629119603,4.90235431137068,131.222621159752));
#247365=CARTESIAN_POINT('Ctrl Pts',(-180.844047498772,4.91211084899382,
131.085673986604));
#247366=CARTESIAN_POINT('Ctrl Pts',(-180.851803801514,4.91613250301284,
130.948666803576));
#247367=CARTESIAN_POINT('Ctrl Pts',(-180.859564244028,4.92015630350971,
130.811586495688));
#247368=CARTESIAN_POINT('Ctrl Pts',(-180.867324686542,4.91843912623242,
130.674446504842));
#247369=CARTESIAN_POINT('Ctrl Pts',(-180.875085129057,4.91101899564668,
130.537760754668));
#247370=CARTESIAN_POINT('Ctrl Pts',(-180.882858029322,4.90358695360859,
130.400855584392));
#247371=CARTESIAN_POINT('Ctrl Pts',(-180.890630929587,4.89043370141627,
130.264406501322));
#247372=CARTESIAN_POINT('Ctrl Pts',(-180.898403829853,4.871649047432,130.128921041323));
#247373=CARTESIAN_POINT('Ctrl Pts',(-180.905894165615,4.85354726293575,
129.998360819063));
#247374=CARTESIAN_POINT('Ctrl Pts',(-180.913384501377,4.83021645414565,
129.86869567912));
#247375=CARTESIAN_POINT('Ctrl Pts',(-180.920874837139,4.80178100090587,
129.74036706409));
#247376=CARTESIAN_POINT('Ctrl Pts',(-180.928649171258,4.77226740881377,
129.607172830616));
#247377=CARTESIAN_POINT('Ctrl Pts',(-180.936423505377,4.73716095571161,
129.474996552097));
#247378=CARTESIAN_POINT('Ctrl Pts',(-180.944197839496,4.69654503604511,
129.344344252281));
#247379=CARTESIAN_POINT('Ctrl Pts',(-180.951962592443,4.65597917186976,
129.213852969748));
#247380=CARTESIAN_POINT('Ctrl Pts',(-180.95972734539,4.60991746600389,129.08488229868));
#247381=CARTESIAN_POINT('Ctrl Pts',(-180.967492098337,4.55849433086872,
128.957928247308));
#247382=CARTESIAN_POINT('Ctrl Pts',(-180.975249139222,4.5071222699163,128.831100288489));
#247383=CARTESIAN_POINT('Ctrl Pts',(-180.983006180107,4.45039952260687,
128.706285323457));
#247384=CARTESIAN_POINT('Ctrl Pts',(-180.990763220992,4.38851022386175,
128.583964013902));
#247385=CARTESIAN_POINT('Ctrl Pts',(-180.998514412233,4.32666759631816,
128.461734947799));
#247386=CARTESIAN_POINT('Ctrl Pts',(-181.006265603473,4.2596663481538,128.341996141624));
#247387=CARTESIAN_POINT('Ctrl Pts',(-181.014016794713,4.18773847591968,
128.225207748928));
#247388=CARTESIAN_POINT('Ctrl Pts',(-181.02176469149,4.11584117494989,128.108468994414));
#247389=CARTESIAN_POINT('Ctrl Pts',(-181.029512588267,4.03902161920529,
127.994678491457));
#247390=CARTESIAN_POINT('Ctrl Pts',(-181.037260485044,3.95755733938158,
127.884271069623));
#247391=CARTESIAN_POINT('Ctrl Pts',(-181.045006761128,3.87611010012927,
127.773886742641));
#247392=CARTESIAN_POINT('Ctrl Pts',(-181.052753037212,3.79002030129498,
127.666884403591));
#247393=CARTESIAN_POINT('Ctrl Pts',(-181.060499313296,3.6996080914805,127.563668865493));
#247394=CARTESIAN_POINT('Ctrl Pts',(-181.068245646562,3.6091952142635,127.460452565482));
#247395=CARTESIAN_POINT('Ctrl Pts',(-181.075991979827,3.51446012000957,
127.361023416295));
#247396=CARTESIAN_POINT('Ctrl Pts',(-181.083738313092,3.41576216570124,
127.26575186696));
#247397=CARTESIAN_POINT('Ctrl Pts',(-181.091486381095,3.3170421086705,127.170458982223));
#247398=CARTESIAN_POINT('Ctrl Pts',(-181.099234449098,3.2143577068925,127.079325821528));
#247399=CARTESIAN_POINT('Ctrl Pts',(-181.106982517101,3.10810366340641,
126.992684519047));
#247400=CARTESIAN_POINT('Ctrl Pts',(-181.114738819843,3.00173669185833,
126.905951133159));
#247401=CARTESIAN_POINT('Ctrl Pts',(-181.122495122585,2.89179280344652,
126.82371938953));
#247402=CARTESIAN_POINT('Ctrl Pts',(-181.130251425327,2.77869858235167,
126.746280129092));
#247403=CARTESIAN_POINT('Ctrl Pts',(-181.138011867841,2.66554399946583,
126.668799536988));
#247404=CARTESIAN_POINT('Ctrl Pts',(-181.145772310355,2.54923606489846,
126.596116731981));
#247405=CARTESIAN_POINT('Ctrl Pts',(-181.153532752869,2.43022771030707,
126.528477511288));
#247406=CARTESIAN_POINT('Ctrl Pts',(-181.161305653134,2.31102831293982,
126.460729710112));
#247407=CARTESIAN_POINT('Ctrl Pts',(-181.1690785534,2.18912018081892,126.398041851348));
#247408=CARTESIAN_POINT('Ctrl Pts',(-181.176851453665,2.06497886185556,
126.340612712208));
#247409=CARTESIAN_POINT('Ctrl Pts',(-181.184341789427,1.94535039252626,
126.285271266929));
#247410=CARTESIAN_POINT('Ctrl Pts',(-181.19183212519,1.82364856594436,126.23481296174));
#247411=CARTESIAN_POINT('Ctrl Pts',(-181.199322460952,1.70031201061043,
126.189371762859));
#247412=CARTESIAN_POINT('Ctrl Pts',(-181.207096795071,1.57229911229676,
126.142207647111));
#247413=CARTESIAN_POINT('Ctrl Pts',(-181.21487112919,1.44211957032787,126.100299193248));
#247414=CARTESIAN_POINT('Ctrl Pts',(-181.222645463309,1.31024419354801,
126.063849757355));
#247415=CARTESIAN_POINT('Ctrl Pts',(-181.230410216256,1.17853134138399,
126.027445242135));
#247416=CARTESIAN_POINT('Ctrl Pts',(-181.238174969203,1.04512718603475,
125.996486461819));
#247417=CARTESIAN_POINT('Ctrl Pts',(-181.24593972215,0.910521686468727,
125.971128435995));
#247418=CARTESIAN_POINT('Ctrl Pts',(-181.253696763035,0.776049878982477,
125.94579559612));
#247419=CARTESIAN_POINT('Ctrl Pts',(-181.26145380392,0.640379483506111,
125.926052512528));
#247420=CARTESIAN_POINT('Ctrl Pts',(-181.269210844805,0.504014423755966,
125.91200407668));
#247421=CARTESIAN_POINT('Ctrl Pts',(-181.276962036045,0.36775219795833,
125.897966234867));
#247422=CARTESIAN_POINT('Ctrl Pts',(-181.284713227285,0.230796737915274,
125.889614533002));
#247423=CARTESIAN_POINT('Ctrl Pts',(-181.292464418526,0.0936605836422182,
125.887002510048));
#247424=CARTESIAN_POINT('Ctrl Pts',(-181.300212315303,-0.0434172841072315,
125.884391597274));
#247425=CARTESIAN_POINT('Ctrl Pts',(-181.30796021208,-0.180675303261666,
125.887515518829));
#247426=CARTESIAN_POINT('Ctrl Pts',(-181.315708108857,-0.317597627272033,
125.89637581628));
#247427=CARTESIAN_POINT('Ctrl Pts',(-181.323454384941,-0.454491310083921,
125.905234260348));
#247428=CARTESIAN_POINT('Ctrl Pts',(-181.331200661025,-0.591049047521525,
125.919826668363));
#247429=CARTESIAN_POINT('Ctrl Pts',(-181.338946937109,-0.726757210785079,
125.940102501566));
#247430=CARTESIAN_POINT('Ctrl Pts',(-181.346693270374,-0.862466375815651,
125.96037848444));
#247431=CARTESIAN_POINT('Ctrl Pts',(-181.35443960364,-0.997325567484876,
125.986337918446));
#247432=CARTESIAN_POINT('Ctrl Pts',(-181.362185936905,-1.13082887530605,
126.017878703125));
#247433=CARTESIAN_POINT('Ctrl Pts',(-181.369934004908,-1.26436208026681,
126.049426551144));
#247434=CARTESIAN_POINT('Ctrl Pts',(-181.377682072911,-1.39653841675175,
126.086558147126));
#247435=CARTESIAN_POINT('Ctrl Pts',(-181.385430140914,-1.52686510424168,
126.12912094286));
#247436=CARTESIAN_POINT('Ctrl Pts',(-181.393186443656,-1.65733030448651,
126.171728974839));
#247437=CARTESIAN_POINT('Ctrl Pts',(-181.400942746398,-1.78594155654096,
126.21977961588));
#247438=CARTESIAN_POINT('Ctrl Pts',(-181.408699049139,-1.91222358852397,
126.273071175256));
#247439=CARTESIAN_POINT('Ctrl Pts',(-181.416459491654,-2.03857302102973,
126.326391177942));
#247440=CARTESIAN_POINT('Ctrl Pts',(-181.424219934168,-2.16259040297888,
126.384957505823));
#247441=CARTESIAN_POINT('Ctrl Pts',(-181.431980376682,-2.28382411758841,
126.448521954068));
#247442=CARTESIAN_POINT('Ctrl Pts',(-181.439753276947,-2.40525244731925,
126.512188441609));
#247443=CARTESIAN_POINT('Ctrl Pts',(-181.447526177213,-2.52388784149363,
126.580868886882));
#247444=CARTESIAN_POINT('Ctrl Pts',(-181.455299077478,-2.63930601795003,
126.654270641901));
#247445=CARTESIAN_POINT('Ctrl Pts',(-181.46278941324,-2.75052845296859,
126.725004058236));
#247446=CARTESIAN_POINT('Ctrl Pts',(-181.470279749002,-2.85876326417252,
126.800121305243));
#247447=CARTESIAN_POINT('Ctrl Pts',(-181.477770084764,-2.96366065256876,
126.879325764356));
#247448=CARTESIAN_POINT('Ctrl Pts',(-181.485571301677,-3.07291173377017,
126.961817549197));
#247449=CARTESIAN_POINT('Ctrl Pts',(-181.493372518591,-3.17890946479242,
127.049020518601));
#247450=CARTESIAN_POINT('Ctrl Pts',(-181.501173735504,-3.28121524436916,
127.140645347158));
#247451=CARTESIAN_POINT('Ctrl Pts',(-181.508855785267,-3.38195825643629,
127.230870564611));
#247452=CARTESIAN_POINT('Ctrl Pts',(-181.516537835029,-3.47912097019819,
127.325383261093));
#247453=CARTESIAN_POINT('Ctrl Pts',(-181.524219884791,-3.57231315162841,
127.423863345092));
#247454=CARTESIAN_POINT('Ctrl Pts',(-181.531894943118,-3.66542051884068,
127.522253802353));
#247455=CARTESIAN_POINT('Ctrl Pts',(-181.539570001446,-3.75456426629303,
127.624604178921));
#247456=CARTESIAN_POINT('Ctrl Pts',(-181.547245059773,-3.83938845729224,
127.730555266456));
#247457=CARTESIAN_POINT('Ctrl Pts',(-181.554914880889,-3.92415476700669,
127.836434056396));
#247458=CARTESIAN_POINT('Ctrl Pts',(-181.562584702005,-4.00460713403721,
127.945908359317));
#247459=CARTESIAN_POINT('Ctrl Pts',(-181.570254523121,-4.08042798415152,
128.058583764169));
#247460=CARTESIAN_POINT('Ctrl Pts',(-181.578149920418,-4.15847879212069,
128.174573051728));
#247461=CARTESIAN_POINT('Ctrl Pts',(-181.586045317716,-4.2316211508202,
128.293954320808));
#247462=CARTESIAN_POINT('Ctrl Pts',(-181.593940715013,-4.29955471667743,
128.416262566648));
#247463=CARTESIAN_POINT('Ctrl Pts',(-181.60160643385,-4.36551208345984,
128.535012844653));
#247464=CARTESIAN_POINT('Ctrl Pts',(-181.609272152686,-4.42655931303819,
128.656521791086));
#247465=CARTESIAN_POINT('Ctrl Pts',(-181.616937871523,-4.48246715571917,
128.780337084996));
#247466=CARTESIAN_POINT('Ctrl Pts',(-181.624948108051,-4.54088764480406,
128.909716965876));
#247467=CARTESIAN_POINT('Ctrl Pts',(-181.632958344578,-4.59369582612956,
129.041614905708));
#247468=CARTESIAN_POINT('Ctrl Pts',(-181.640968581106,-4.6406858403334,
129.175490458889));
#247469=CARTESIAN_POINT('Ctrl Pts',(-181.648978817634,-4.68767585453736,
129.30936601207));
#247470=CARTESIAN_POINT('Ctrl Pts',(-181.656989054161,-4.72884756406629,
129.445218700358));
#247471=CARTESIAN_POINT('Ctrl Pts',(-181.664999290689,-4.76405452823418,
129.582490119309));
#247472=CARTESIAN_POINT('',(-179.639859435944,-4.91824845113006,130.800457355239));
#247473=CARTESIAN_POINT('Ctrl Pts',(-179.639859435995,-4.91824845113077,
130.80045735614));
#247474=CARTESIAN_POINT('Ctrl Pts',(-179.647643348581,-4.91835785303648,
130.938307654795));
#247475=CARTESIAN_POINT('Ctrl Pts',(-179.655427261166,-4.91266728495612,
131.076231294055));
#247476=CARTESIAN_POINT('Ctrl Pts',(-179.663211173751,-4.90118571413701,
131.213703576513));
#247477=CARTESIAN_POINT('Ctrl Pts',(-179.670945887216,-4.88977671391655,
131.350306949481));
#247478=CARTESIAN_POINT('Ctrl Pts',(-179.67868060068,-4.87264975986795,
131.486464261715));
#247479=CARTESIAN_POINT('Ctrl Pts',(-179.686415314144,-4.84986584312386,
131.62166372303));
#247480=CARTESIAN_POINT('Ctrl Pts',(-179.694150299485,-4.82708112551935,
131.75686793664));
#247481=CARTESIAN_POINT('Ctrl Pts',(-179.701885284826,-4.79863911424742,
131.891113845955));
#247482=CARTESIAN_POINT('Ctrl Pts',(-179.709620270168,-4.76465219127589,
132.023898463912));
#247483=CARTESIAN_POINT('Ctrl Pts',(-179.717357210254,-4.73065667930619,
132.156716638506));
#247484=CARTESIAN_POINT('Ctrl Pts',(-179.725094150341,-4.69111356423603,
132.288072407442));
#247485=CARTESIAN_POINT('Ctrl Pts',(-179.732831090427,-4.64618538712646,
132.417476983782));
#247486=CARTESIAN_POINT('Ctrl Pts',(-179.740651277729,-4.6007737959558,
132.54827391556));
#247487=CARTESIAN_POINT('Ctrl Pts',(-179.748471465031,-4.54986071193366,
132.677077031875));
#247488=CARTESIAN_POINT('Ctrl Pts',(-179.756291652332,-4.4936638437746,
132.803402468467));
#247489=CARTESIAN_POINT('Ctrl Pts',(-179.764041702127,-4.43797099273028,
132.928594920532));
#247490=CARTESIAN_POINT('Ctrl Pts',(-179.771791751921,-4.37708898469712,
133.051353633612));
#247491=CARTESIAN_POINT('Ctrl Pts',(-179.779541801716,-4.31127556038019,
133.171233259887));
#247492=CARTESIAN_POINT('Ctrl Pts',(-179.787397057771,-4.24456872447766,
133.292740241798));
#247493=CARTESIAN_POINT('Ctrl Pts',(-179.795252313826,-4.17279583022991,
133.41128904481));
#247494=CARTESIAN_POINT('Ctrl Pts',(-179.803107569882,-4.09626958239033,
133.526447789367));
#247495=CARTESIAN_POINT('Ctrl Pts',(-179.810962825937,-4.01974333455076,
133.641606533924));
#247496=CARTESIAN_POINT('Ctrl Pts',(-179.818818081992,-3.93846402808792,
133.753374925537));
#247497=CARTESIAN_POINT('Ctrl Pts',(-179.826673338047,-3.85278485618213,
133.861357823072));
#247498=CARTESIAN_POINT('Ctrl Pts',(-179.834447672166,-3.76798831934649,
133.968228320824));
#247499=CARTESIAN_POINT('Ctrl Pts',(-179.842222006285,-3.67860745899652,
134.071737226023));
#247500=CARTESIAN_POINT('Ctrl Pts',(-179.849996340404,-3.58493859117706,
134.171465955982));
#247501=CARTESIAN_POINT('Ctrl Pts',(-179.857761093352,-3.491385161866,134.271071779194));
#247502=CARTESIAN_POINT('Ctrl Pts',(-179.865525846299,-3.39355450492741,
134.366906414405));
#247503=CARTESIAN_POINT('Ctrl Pts',(-179.873290599246,-3.29178443534814,
134.458582599562));
#247504=CARTESIAN_POINT('Ctrl Pts',(-179.881047640131,-3.19011544523642,
134.550167730639));
#247505=CARTESIAN_POINT('Ctrl Pts',(-179.888804681016,-3.08451511749853,
134.637602371029));
#247506=CARTESIAN_POINT('Ctrl Pts',(-179.896561721901,-2.97535926942331,
134.720534806792));
#247507=CARTESIAN_POINT('Ctrl Pts',(-179.904312913141,-2.86628573662238,
134.803404702559));
#247508=CARTESIAN_POINT('Ctrl Pts',(-179.912064104381,-2.75366233038859,
134.881778915971));
#247509=CARTESIAN_POINT('Ctrl Pts',(-179.919815295621,-2.63789893932337,
134.955345109035));
#247510=CARTESIAN_POINT('Ctrl Pts',(-179.927563192398,-2.52218475078761,
135.028880034504));
#247511=CARTESIAN_POINT('Ctrl Pts',(-179.935311089175,-2.40333356107528,
135.097610794808));
#247512=CARTESIAN_POINT('Ctrl Pts',(-179.943058985952,-2.28178513072117,
135.161267740712));
#247513=CARTESIAN_POINT('Ctrl Pts',(-179.950805262036,-2.16026212567808,
135.224911370955));
#247514=CARTESIAN_POINT('Ctrl Pts',(-179.958551538121,-2.03604334835015,
135.283483116575));
#247515=CARTESIAN_POINT('Ctrl Pts',(-179.966297814205,-1.9095937562906,
135.336758961538));
#247516=CARTESIAN_POINT('Ctrl Pts',(-179.97404414747,-1.78314323080907,
135.39003519977));
#247517=CARTESIAN_POINT('Ctrl Pts',(-179.981790480735,-1.65446221802928,
135.438015307539));
#247518=CARTESIAN_POINT('Ctrl Pts',(-179.989536814001,-1.5240359049478,
135.480523320352));
#247519=CARTESIAN_POINT('Ctrl Pts',(-179.997284882004,-1.393580383798,135.52304085254));
#247520=CARTESIAN_POINT('Ctrl Pts',(-180.005032950007,-1.26137915625431,
135.560083730166));
#247521=CARTESIAN_POINT('Ctrl Pts',(-180.01278101801,-1.12793243744398,
135.59152590394));
#247522=CARTESIAN_POINT('Ctrl Pts',(-180.020537320752,-0.994343889872685,
135.62300149483));
#247523=CARTESIAN_POINT('Ctrl Pts',(-180.028293623494,-0.859507587907298,
135.648864401312));
#247524=CARTESIAN_POINT('Ctrl Pts',(-180.036049926235,-0.723934356211346,
135.66903965224));
#247525=CARTESIAN_POINT('Ctrl Pts',(-180.04381036875,-0.588288764999606,
135.689225671307));
#247526=CARTESIAN_POINT('Ctrl Pts',(-180.051570811264,-0.45190584891694,
135.703717944691));
#247527=CARTESIAN_POINT('Ctrl Pts',(-180.059331253778,-0.315300425492684,
135.71249353184));
#247528=CARTESIAN_POINT('Ctrl Pts',(-180.067104154043,-0.178475710915488,
135.721283206341));
#247529=CARTESIAN_POINT('Ctrl Pts',(-180.074877054309,-0.0414281663132729,
135.724337847456));
#247530=CARTESIAN_POINT('Ctrl Pts',(-180.082649954574,0.0953276177084138,
135.721686690525));
#247531=CARTESIAN_POINT('Ctrl Pts',(-180.090140290336,0.227111984512766,
135.719131909827));
#247532=CARTESIAN_POINT('Ctrl Pts',(-180.097630626098,0.358625127450248,
135.71127898747));
#247533=CARTESIAN_POINT('Ctrl Pts',(-180.10512096186,0.489414003383709,
135.698199294494));
#247534=CARTESIAN_POINT('Ctrl Pts',(-180.112895295979,0.625161779301939,
135.684623680983));
#247535=CARTESIAN_POINT('Ctrl Pts',(-180.120669630098,0.76055929103879,
135.665374123379));
#247536=CARTESIAN_POINT('Ctrl Pts',(-180.128443964217,0.895094207063287,
135.640473666594));
#247537=CARTESIAN_POINT('Ctrl Pts',(-180.136208717164,1.02946332082715,
135.615603897398));
#247538=CARTESIAN_POINT('Ctrl Pts',(-180.143973470111,1.16297157332996,
135.58509715623));
#247539=CARTESIAN_POINT('Ctrl Pts',(-180.151738223059,1.29511055278657,
135.549028331807));
#247540=CARTESIAN_POINT('Ctrl Pts',(-180.159495263944,1.42711828994595,
135.512995331449));
#247541=CARTESIAN_POINT('Ctrl Pts',(-180.167252304829,1.55775908575723,
135.471411343807));
#247542=CARTESIAN_POINT('Ctrl Pts',(-180.175009345714,1.68653389489693,
135.424402444635));
#247543=CARTESIAN_POINT('Ctrl Pts',(-180.182760536954,1.81521159395151,
135.377428995238));
#247544=CARTESIAN_POINT('Ctrl Pts',(-180.190511728194,1.94202574141753,
135.325038910659));
#247545=CARTESIAN_POINT('Ctrl Pts',(-180.198262919434,2.06649200369359,
135.267408215472));
#247546=CARTESIAN_POINT('Ctrl Pts',(-180.206010816211,2.19090536448777,
135.209802014867));
#247547=CARTESIAN_POINT('Ctrl Pts',(-180.213758712988,2.31297247082939,
135.146959797708));
#247548=CARTESIAN_POINT('Ctrl Pts',(-180.221506609765,2.43222875786826,
135.079105794989));
#247549=CARTESIAN_POINT('Ctrl Pts',(-180.229252885849,2.55146009906276,
135.011265985864));
#247550=CARTESIAN_POINT('Ctrl Pts',(-180.236999161933,2.6678814508488,134.938416669642));
#247551=CARTESIAN_POINT('Ctrl Pts',(-180.244745438018,2.78105302127715,
134.860827942141));
#247552=CARTESIAN_POINT('Ctrl Pts',(-180.252491771283,2.89422542711247,
134.783238641898));
#247553=CARTESIAN_POINT('Ctrl Pts',(-180.260238104548,3.00414768126175,
134.700910081639));
#247554=CARTESIAN_POINT('Ctrl Pts',(-180.267984437814,3.11040948439129,
134.61415534982));
#247555=CARTESIAN_POINT('Ctrl Pts',(-180.275732505817,3.21669508411531,
134.52738118988));
#247556=CARTESIAN_POINT('Ctrl Pts',(-180.28348057382,3.31931829885344,134.436179133193));
#247557=CARTESIAN_POINT('Ctrl Pts',(-180.291228641823,3.41790270127258,
134.340901892192));
#247558=CARTESIAN_POINT('Ctrl Pts',(-180.298984944565,3.51659188036738,
134.245523389406));
#247559=CARTESIAN_POINT('Ctrl Pts',(-180.306741247306,3.61123339083883,
134.146061322491));
#247560=CARTESIAN_POINT('Ctrl Pts',(-180.314497550048,3.70148804412907,
134.042904938966));
#247561=CARTESIAN_POINT('Ctrl Pts',(-180.322257992563,3.79179086904529,
133.939693497773));
#247562=CARTESIAN_POINT('Ctrl Pts',(-180.330018435077,3.87770192656671,
133.832784115665));
#247563=CARTESIAN_POINT('Ctrl Pts',(-180.337778877591,3.95892364470687,
133.722597523282));
#247564=CARTESIAN_POINT('Ctrl Pts',(-180.345551777856,4.04027574715952,
133.612234049598));
#247565=CARTESIAN_POINT('Ctrl Pts',(-180.353324678122,4.1169232486707,133.498583177072));
#247566=CARTESIAN_POINT('Ctrl Pts',(-180.361097578387,4.18861259696973,
133.38209364777));
#247567=CARTESIAN_POINT('Ctrl Pts',(-180.368587914149,4.25769585688294,
133.269838806279));
#247568=CARTESIAN_POINT('Ctrl Pts',(-180.376078249911,4.32217503704249,
133.154948378128));
#247569=CARTESIAN_POINT('Ctrl Pts',(-180.383568585673,4.3818653030435,133.037842099129));
#247570=CARTESIAN_POINT('Ctrl Pts',(-180.391342919792,4.44381874362301,
132.916295699966));
#247571=CARTESIAN_POINT('Ctrl Pts',(-180.399117253911,4.50080920799675,
132.791977082604));
#247572=CARTESIAN_POINT('Ctrl Pts',(-180.40689158803,4.5525791567958,132.665329742406));
#247573=CARTESIAN_POINT('Ctrl Pts',(-180.414656340977,4.60428530375948,
132.538838483737));
#247574=CARTESIAN_POINT('Ctrl Pts',(-180.422421093925,4.65078359001705,
132.410024570987));
#247575=CARTESIAN_POINT('Ctrl Pts',(-180.430185846872,4.69186221257831,
132.27935622457));
#247576=CARTESIAN_POINT('Ctrl Pts',(-180.437942887757,4.73290003527265,
132.148817659796));
#247577=CARTESIAN_POINT('Ctrl Pts',(-180.445699928642,4.76852878996476,
132.016428697274));
#247578=CARTESIAN_POINT('Ctrl Pts',(-180.453456969527,4.79858480156904,
131.882677344994));
#247579=CARTESIAN_POINT('Ctrl Pts',(-180.461208160767,4.8286181477013,131.749026855648));
#247580=CARTESIAN_POINT('Ctrl Pts',(-180.468959352007,4.85308703009387,
131.614016401407));
#247581=CARTESIAN_POINT('Ctrl Pts',(-180.476710543247,4.87187774906408,
131.478148611429));
#247582=CARTESIAN_POINT('Ctrl Pts',(-180.484458440024,4.89066048147738,
131.342338568887));
#247583=CARTESIAN_POINT('Ctrl Pts',(-180.492206336801,4.90376979703001,
131.205672301821));
#247584=CARTESIAN_POINT('Ctrl Pts',(-180.499954233578,4.91114323895842,
131.068661864126));
#247585=CARTESIAN_POINT('Ctrl Pts',(-180.507700509662,4.91851513852172,
130.93168008606));
#247586=CARTESIAN_POINT('Ctrl Pts',(-180.515446785746,4.92015352997405,
130.794354670717));
#247587=CARTESIAN_POINT('Ctrl Pts',(-180.523193061831,4.91604793428645,
130.657201620906));
#247588=CARTESIAN_POINT('Ctrl Pts',(-180.530939395096,4.91194230829228,
130.520047558662));
#247589=CARTESIAN_POINT('Ctrl Pts',(-180.538685728361,4.9020926222485,130.38306625528));
#247590=CARTESIAN_POINT('Ctrl Pts',(-180.546432061627,4.88654050952772,
130.246772139166));
#247591=CARTESIAN_POINT('Ctrl Pts',(-180.55418012963,4.8709849140191,130.110447500929));
#247592=CARTESIAN_POINT('Ctrl Pts',(-180.561928197633,4.84972439502942,
129.974810744557));
#247593=CARTESIAN_POINT('Ctrl Pts',(-180.569676265636,4.82285223134933,
129.84036921871));
#247594=CARTESIAN_POINT('Ctrl Pts',(-180.577432568377,4.795951507614,129.70578480681));
#247595=CARTESIAN_POINT('Ctrl Pts',(-180.585188871119,4.76342730196317,
129.572398547));
#247596=CARTESIAN_POINT('Ctrl Pts',(-180.592945173861,4.72542375965904,
129.440706206012));
#247597=CARTESIAN_POINT('Ctrl Pts',(-180.600705616375,4.68739993372011,
129.308943576857));
#247598=CARTESIAN_POINT('Ctrl Pts',(-180.608466058889,4.64389106780674,
129.178877038601));
#247599=CARTESIAN_POINT('Ctrl Pts',(-180.616226501404,4.59509028959371,
129.050984362171));
#247600=CARTESIAN_POINT('Ctrl Pts',(-180.623999401669,4.54621117203903,
128.922886381063));
#247601=CARTESIAN_POINT('Ctrl Pts',(-180.631772301934,4.49202332100907,
128.796969594594));
#247602=CARTESIAN_POINT('Ctrl Pts',(-180.6395452022,4.43276722471806,128.67368987952));
#247603=CARTESIAN_POINT('Ctrl Pts',(-180.647035537962,4.37566523678433,
128.554891692612));
#247604=CARTESIAN_POINT('Ctrl Pts',(-180.654525873724,4.31385723758189,
128.438542449427));
#247605=CARTESIAN_POINT('Ctrl Pts',(-180.662016209486,4.24759645522655,
128.325024533844));
#247606=CARTESIAN_POINT('Ctrl Pts',(-180.669790543605,4.17882337516859,
128.207202551989));
#247607=CARTESIAN_POINT('Ctrl Pts',(-180.677564877724,4.10503533955871,
128.092057610922));
#247608=CARTESIAN_POINT('Ctrl Pts',(-180.685339211843,4.02646626728858,
127.980046105886));
#247609=CARTESIAN_POINT('Ctrl Pts',(-180.69310396479,3.94799402437853,127.86817264502));
#247610=CARTESIAN_POINT('Ctrl Pts',(-180.700868717737,3.86475269088806,
127.759425253595));
#247611=CARTESIAN_POINT('Ctrl Pts',(-180.708633470684,3.77702170922281,
127.654235212037));
#247612=CARTESIAN_POINT('Ctrl Pts',(-180.71639051157,3.68937786320486,127.54914964671));
#247613=CARTESIAN_POINT('Ctrl Pts',(-180.724147552455,3.59725349177691,
127.447614698306));
#247614=CARTESIAN_POINT('Ctrl Pts',(-180.73190459334,3.50097069949896,127.350031851547));
#247615=CARTESIAN_POINT('Ctrl Pts',(-180.73965578458,3.40476051482377,127.252522592771));
#247616=CARTESIAN_POINT('Ctrl Pts',(-180.74740697582,3.30439842459542,127.158959780689));
#247617=CARTESIAN_POINT('Ctrl Pts',(-180.75515816706,3.20024584750376,127.0697107574));
#247618=CARTESIAN_POINT('Ctrl Pts',(-180.762906063837,3.09613753803588,
126.980499667328));
#247619=CARTESIAN_POINT('Ctrl Pts',(-180.770653960614,2.98824224223235,
126.89559897327));
#247620=CARTESIAN_POINT('Ctrl Pts',(-180.778401857391,2.87695700613077,
126.815337999508));
#247621=CARTESIAN_POINT('Ctrl Pts',(-180.786148133475,2.76569504850156,
126.735093814613));
#247622=CARTESIAN_POINT('Ctrl Pts',(-180.793894409559,2.65104487791537,
126.659487648129));
#247623=CARTESIAN_POINT('Ctrl Pts',(-180.801640685643,2.53343495797927,
126.588807228485));
#247624=CARTESIAN_POINT('Ctrl Pts',(-180.809387018909,2.41582416987298,
126.518126287095));
#247625=CARTESIAN_POINT('Ctrl Pts',(-180.817133352174,2.29525392392618,
126.452371366488));
#247626=CARTESIAN_POINT('Ctrl Pts',(-180.82487968544,2.17217952718222,126.39178550045));
#247627=CARTESIAN_POINT('Ctrl Pts',(-180.832627753443,2.04907756878062,
126.331186066628));
#247628=CARTESIAN_POINT('Ctrl Pts',(-180.840375821446,1.92347069438084,
126.275758163452));
#247629=CARTESIAN_POINT('Ctrl Pts',(-180.848123889449,1.79583617024562,
126.225697547178));
#247630=CARTESIAN_POINT('Ctrl Pts',(-180.855880192191,1.66806599461945,
126.175583725885));
#247631=CARTESIAN_POINT('Ctrl Pts',(-180.863636494932,1.53826422894359,
126.130848729665));
#247632=CARTESIAN_POINT('Ctrl Pts',(-180.871392797674,1.40692588984619,
126.091639259053));
#247633=CARTESIAN_POINT('Ctrl Pts',(-180.879153240188,1.2755174515227,126.052408861167));
#247634=CARTESIAN_POINT('Ctrl Pts',(-180.886913682703,1.14257118442251,
126.018709961316));
#247635=CARTESIAN_POINT('Ctrl Pts',(-180.894674125217,1.00859344098332,
125.990638322574));
#247636=CARTESIAN_POINT('Ctrl Pts',(-180.902447025482,0.874400624576381,
125.962521620745));
#247637=CARTESIAN_POINT('Ctrl Pts',(-180.910219925748,0.739173408878079,
125.940050295721));
#247638=CARTESIAN_POINT('Ctrl Pts',(-180.917992826013,0.603425325667191,
125.923268430479));
#247639=CARTESIAN_POINT('Ctrl Pts',(-180.925483161775,0.472612027210911,
125.907096628309));
#247640=CARTESIAN_POINT('Ctrl Pts',(-180.932973497537,0.341315380425482,
125.896207840602));
#247641=CARTESIAN_POINT('Ctrl Pts',(-180.940463833299,0.20999397167983,
125.890595707199));
#247642=CARTESIAN_POINT('Ctrl Pts',(-180.948238167418,0.0736934718059715,
125.884770788052));
#247643=CARTESIAN_POINT('Ctrl Pts',(-180.956012501537,-0.0630654638079416,
125.884612098978));
#247644=CARTESIAN_POINT('Ctrl Pts',(-180.963786835656,-0.199772418043521,
125.890169530165));
#247645=CARTESIAN_POINT('Ctrl Pts',(-180.971551588603,-0.336310893175113,
125.895720112316));
#247646=CARTESIAN_POINT('Ctrl Pts',(-180.97931634155,-0.472797127501037,
125.90697278233));
#247647=CARTESIAN_POINT('Ctrl Pts',(-180.987081094497,-0.608717227139118,
125.923925555004));
#247648=CARTESIAN_POINT('Ctrl Pts',(-180.994838135382,-0.744502329018101,
125.940861489945));
#247649=CARTESIAN_POINT('Ctrl Pts',(-181.002595176267,-0.87972202974887,
125.963486212983));
#247650=CARTESIAN_POINT('Ctrl Pts',(-181.010352217152,-1.01386444348082,
125.99174574073));
#247651=CARTESIAN_POINT('Ctrl Pts',(-181.018103408392,-1.14790569937564,
126.019983957747));
#247652=CARTESIAN_POINT('Ctrl Pts',(-181.025854599632,-1.28087090426565,
126.053848441329));
#247653=CARTESIAN_POINT('Ctrl Pts',(-181.033605790873,-1.41225564720813,
126.093233677074));
#247654=CARTESIAN_POINT('Ctrl Pts',(-181.04135368765,-1.54358454812987,
126.132602173044));
#247655=CARTESIAN_POINT('Ctrl Pts',(-181.049101584427,-1.67333394942435,
126.177486642203));
#247656=CARTESIAN_POINT('Ctrl Pts',(-181.056849481204,-1.80101216816459,
126.227731046296));
#247657=CARTESIAN_POINT('Ctrl Pts',(-181.064595757288,-1.92866367937423,
126.277964940342));
#247658=CARTESIAN_POINT('Ctrl Pts',(-181.072342033372,-2.05424450620277,
126.333556396151));
#247659=CARTESIAN_POINT('Ctrl Pts',(-181.080088309456,-2.17728097953044,
126.394300459396));
#247660=CARTESIAN_POINT('Ctrl Pts',(-181.087834642722,-2.3003183610849,
126.455044971041));
#247661=CARTESIAN_POINT('Ctrl Pts',(-181.095580975987,-2.42081100109293,
126.520941992941));
#247662=CARTESIAN_POINT('Ctrl Pts',(-181.103327309252,-2.53830832377024,
126.591739828084));
#247663=CARTESIAN_POINT('Ctrl Pts',(-181.111075377255,-2.65583195915813,
126.662553517911));
#247664=CARTESIAN_POINT('Ctrl Pts',(-181.118823445258,-2.77035860763099,
126.738270003146));
#247665=CARTESIAN_POINT('Ctrl Pts',(-181.126571513261,-2.88146559983368,
126.818593557203));
#247666=CARTESIAN_POINT('Ctrl Pts',(-181.134327816003,-2.99269067787002,
126.89900248009));
#247667=CARTESIAN_POINT('Ctrl Pts',(-181.142084118745,-3.1004885220833,
126.984028023559));
#247668=CARTESIAN_POINT('Ctrl Pts',(-181.149840421487,-3.20446814057772,
127.073333011326));
#247669=CARTESIAN_POINT('Ctrl Pts',(-181.157600864001,-3.30850325612586,
127.162685663855));
#247670=CARTESIAN_POINT('Ctrl Pts',(-181.165361306515,-3.40871579973424,
127.25632204509));
#247671=CARTESIAN_POINT('Ctrl Pts',(-181.173121749029,-3.5047515073558,
127.353867908664));
#247672=CARTESIAN_POINT('Ctrl Pts',(-181.180894649295,-3.60094138002062,
127.451570361518));
#247673=CARTESIAN_POINT('Ctrl Pts',(-181.18866754956,-3.69294075537735,
127.55319454785));
#247674=CARTESIAN_POINT('Ctrl Pts',(-181.196440449825,-3.78043496869995,
127.658332246758));
#247675=CARTESIAN_POINT('Ctrl Pts',(-181.203930785587,-3.86474854698411,
127.759647925484));
#247676=CARTESIAN_POINT('Ctrl Pts',(-181.21142112135,-3.94487863715625,
127.864225857211));
#247677=CARTESIAN_POINT('Ctrl Pts',(-181.218911457112,-4.02058271306412,
127.971676782418));
#247678=CARTESIAN_POINT('Ctrl Pts',(-181.226774298583,-4.10005166699623,
128.084471404409));
#247679=CARTESIAN_POINT('Ctrl Pts',(-181.234637140055,-4.174892552443,128.200785850527));
#247680=CARTESIAN_POINT('Ctrl Pts',(-181.242499981526,-4.24478179121977,
128.320208728605));
#247681=CARTESIAN_POINT('Ctrl Pts',(-181.250349252588,-4.31455040877096,
128.439425495782));
#247682=CARTESIAN_POINT('Ctrl Pts',(-181.25819852365,-4.37938421453783,
128.56173968249));
#247683=CARTESIAN_POINT('Ctrl Pts',(-181.266047794713,-4.43900175716958,
128.686709451216));
#247684=CARTESIAN_POINT('Ctrl Pts',(-181.273889191536,-4.49855949261664,
128.811553852646));
#247685=CARTESIAN_POINT('Ctrl Pts',(-181.281730588359,-4.55291121398804,
128.939048195462));
#247686=CARTESIAN_POINT('Ctrl Pts',(-181.289571985181,-4.60182013260226,
129.0687239823));
#247687=CARTESIAN_POINT('Ctrl Pts',(-181.297405522347,-4.65068002839995,
129.198269791365));
#247688=CARTESIAN_POINT('Ctrl Pts',(-181.305239059512,-4.69410785428418,
129.329992335658));
#247689=CARTESIAN_POINT('Ctrl Pts',(-181.313072596677,-4.73191416286347,
129.463401476581));
#247690=CARTESIAN_POINT('Ctrl Pts',(-181.315395044115,-4.74312278581986,
129.502953943239));
#247691=CARTESIAN_POINT('Ctrl Pts',(-181.317717491553,-4.75383761304045,
129.542654522032));
#247692=CARTESIAN_POINT('Ctrl Pts',(-181.320039938991,-4.76405452823418,
129.582490119309));
#247693=CARTESIAN_POINT('Ctrl Pts',(-179.570054719422,-4.76405452823393,
129.582490119308));
#247694=CARTESIAN_POINT('Ctrl Pts',(-179.579197174056,-4.80396699441805,
129.738108219203));
#247695=CARTESIAN_POINT('Ctrl Pts',(-179.58833962869,-4.8362916101084,129.895843536568));
#247696=CARTESIAN_POINT('Ctrl Pts',(-179.597482083324,-4.86082915223956,
130.055012223801));
#247697=CARTESIAN_POINT('Ctrl Pts',(-179.606541047858,-4.88514261430456,
130.212727361621));
#247698=CARTESIAN_POINT('Ctrl Pts',(-179.615600012392,-4.90181051144224,
130.371849719594));
#247699=CARTESIAN_POINT('Ctrl Pts',(-179.624658976926,-4.91068588618086,
130.53169380667));
#247700=CARTESIAN_POINT('Ctrl Pts',(-179.629725796599,-4.91565002122716,
130.621097089119));
#247701=CARTESIAN_POINT('Ctrl Pts',(-179.634792616271,-4.91817723760474,
130.710725797053));
#247702=CARTESIAN_POINT('Ctrl Pts',(-179.639859435944,-4.91824845113006,
130.800457355239));
#247703=CARTESIAN_POINT('Origin',(213.235140564004,0.,130.804360617566));
#247704=CARTESIAN_POINT('',(-177.819765072025,-4.76405452823413,129.582490119309));
#247705=CARTESIAN_POINT('',(-178.165366640417,-4.76405452823403,129.582490119308));
#247706=CARTESIAN_POINT('',(213.235140564004,-4.76405452823405,129.582490119308));
#247707=CARTESIAN_POINT('',(-177.725096247279,-4.0820853165969,128.06104828928));
#247708=CARTESIAN_POINT('Ctrl Pts',(-177.725096247279,-4.08208531659689,
128.06104828928));
#247709=CARTESIAN_POINT('Ctrl Pts',(-177.732985316008,-4.16002539388626,
128.177024163335));
#247710=CARTESIAN_POINT('Ctrl Pts',(-177.740874384737,-4.23303079411445,
128.296341548097));
#247711=CARTESIAN_POINT('Ctrl Pts',(-177.748763453466,-4.30081646430476,
128.418535644341));
#247712=CARTESIAN_POINT('Ctrl Pts',(-177.756510780686,-4.36738424129978,
128.538534300783));
#247713=CARTESIAN_POINT('Ctrl Pts',(-177.764258107907,-4.42891811933753,
128.661306795764));
#247714=CARTESIAN_POINT('Ctrl Pts',(-177.772005435128,-4.48519447304636,
128.786387971207));
#247715=CARTESIAN_POINT('Ctrl Pts',(-177.779965374611,-4.54301523588223,
128.91490178747));
#247716=CARTESIAN_POINT('Ctrl Pts',(-177.787925314094,-4.59528555643844,
129.045852432001));
#247717=CARTESIAN_POINT('Ctrl Pts',(-177.795885253576,-4.64181608494743,
129.178714132003));
#247718=CARTESIAN_POINT('Ctrl Pts',(-177.803845193059,-4.68834661345641,
129.311575832005));
#247719=CARTESIAN_POINT('Ctrl Pts',(-177.811805132542,-4.72913724299794,
129.446348154116));
#247720=CARTESIAN_POINT('Ctrl Pts',(-177.819765072025,-4.76405452823413,
129.582490119309));
#247721=CARTESIAN_POINT('',(-177.981041338087,-3.00808041127123,126.914654376525));
#247722=CARTESIAN_POINT('Ctrl Pts',(-177.981095179098,-3.00961479406227,
126.914450354609));
#247723=CARTESIAN_POINT('Ctrl Pts',(-177.946925114628,-3.17693683926483,
127.043907043471));
#247724=CARTESIAN_POINT('Ctrl Pts',(-177.912218584466,-3.33351065782883,
127.182415422253));
#247725=CARTESIAN_POINT('Ctrl Pts',(-177.8272197828,-3.69621327019491,127.545118034619));
#247726=CARTESIAN_POINT('Ctrl Pts',(-177.774444409595,-3.90151116845466,
127.792249968281));
#247727=CARTESIAN_POINT('Ctrl Pts',(-177.725144769241,-4.08256462727749,
128.061761644584));
#247728=CARTESIAN_POINT('Ctrl Pts',(-177.981095179098,-3.00961479406228,
126.914450354609));
#247729=CARTESIAN_POINT('Ctrl Pts',(-177.988841298821,-3.11812387474683,
126.998403585517));
#247730=CARTESIAN_POINT('Ctrl Pts',(-177.996587418545,-3.22313694139555,
127.086915601532));
#247731=CARTESIAN_POINT('Ctrl Pts',(-178.004333538268,-3.32425823831933,
127.17965508091));
#247732=CARTESIAN_POINT('Ctrl Pts',(-178.012080203021,-3.42538665030451,
127.272401085591));
#247733=CARTESIAN_POINT('Ctrl Pts',(-178.019826867774,-3.52262245944916,
127.36937488135));
#247734=CARTESIAN_POINT('Ctrl Pts',(-178.027573532527,-3.61560540807819,
127.470206962502));
#247735=CARTESIAN_POINT('Ctrl Pts',(-178.035322419979,-3.70861503568729,
127.571067974734));
#247736=CARTESIAN_POINT('Ctrl Pts',(-178.043071307431,-3.79736910967914,
127.675789187946));
#247737=CARTESIAN_POINT('Ctrl Pts',(-178.050820194884,-3.88154670282093,
127.783966892185));
#247738=CARTESIAN_POINT('Ctrl Pts',(-178.058577545204,-3.96581622965968,
127.892262741597));
#247739=CARTESIAN_POINT('Ctrl Pts',(-178.066334895524,-4.04549905361132,
128.004022312041));
#247740=CARTESIAN_POINT('Ctrl Pts',(-178.074092245844,-4.12031647581515,
128.118811287983));
#247741=CARTESIAN_POINT('Ctrl Pts',(-178.081854174614,-4.19517805584832,
128.233668013278));
#247742=CARTESIAN_POINT('Ctrl Pts',(-178.089616103383,-4.2651683139012,
128.351557370489));
#247743=CARTESIAN_POINT('Ctrl Pts',(-178.097378032152,-4.33005433352629,
128.472020048264));
#247744=CARTESIAN_POINT('Ctrl Pts',(-178.10515176728,-4.39503904867666,
128.592665956994));
#247745=CARTESIAN_POINT('Ctrl Pts',(-178.112925502409,-4.45490384678247,
128.715892653527));
#247746=CARTESIAN_POINT('Ctrl Pts',(-178.120699237537,-4.50946352571929,
128.841219824676));
#247747=CARTESIAN_POINT('Ctrl Pts',(-178.125932358028,-4.54619199268115,
128.925587529081));
#247748=CARTESIAN_POINT('Ctrl Pts',(-178.131165478519,-4.58051734944699,
129.010906720745));
#247749=CARTESIAN_POINT('Ctrl Pts',(-178.13639859901,-4.61239592518718,
129.097027348454));
#247750=CARTESIAN_POINT('Ctrl Pts',(-178.145370171086,-4.66704800905346,
129.244671076535));
#247751=CARTESIAN_POINT('Ctrl Pts',(-178.154341743163,-4.71465032755617,
129.395057764512));
#247752=CARTESIAN_POINT('Ctrl Pts',(-178.163313315239,-4.75495695955518,
129.547552209225));
#247753=CARTESIAN_POINT('Ctrl Pts',(-178.163997756965,-4.75803195472055,
129.559186018774));
#247754=CARTESIAN_POINT('Ctrl Pts',(-178.164682198691,-4.7610645102698,
129.570832084646));
#247755=CARTESIAN_POINT('Ctrl Pts',(-178.165366640417,-4.76405452823403,
129.582490119308));
#247756=CARTESIAN_POINT('Ctrl Pts',(210.579426101437,-2.14555810197798,
126.384433368448));
#247757=CARTESIAN_POINT('Ctrl Pts',(210.533016425084,-2.88204635455982,
126.741945114569));
#247758=CARTESIAN_POINT('Ctrl Pts',(210.440198811428,-4.16073755837059,
127.832228156677));
#247759=CARTESIAN_POINT('Ctrl Pts',(210.254565323169,-5.41774734084591,
130.983824311839));
#247760=CARTESIAN_POINT('Ctrl Pts',(210.022525636658,-3.70466367662459,
135.280954889074));
#247761=CARTESIAN_POINT('Ctrl Pts',(209.744078012845,1.77278938863763,136.341871604603));
#247762=CARTESIAN_POINT('Ctrl Pts',(209.465630389032,5.61248518735455,132.305536381355));
#247763=CARTESIAN_POINT('Ctrl Pts',(209.187182765219,4.2990952821384,126.894094626803));
#247764=CARTESIAN_POINT('Ctrl Pts',(208.908735141406,-0.967335548355457,
125.073681250508));
#247765=CARTESIAN_POINT('Ctrl Pts',(208.630287517594,-5.34357155608916,
128.520706403956));
#247766=CARTESIAN_POINT('Ctrl Pts',(208.351839893781,-4.80999390579215,
134.065650134797));
#247767=CARTESIAN_POINT('Ctrl Pts',(208.073392269968,0.144086686833323,
136.613971320579));
#247768=CARTESIAN_POINT('Ctrl Pts',(207.794944646155,4.96557142732685,133.823362329787));
#247769=CARTESIAN_POINT('Ctrl Pts',(207.516497022342,5.22403776314189,128.258534510045));
#247770=CARTESIAN_POINT('Ctrl Pts',(207.238049398529,0.681816090004523,
125.033145533949));
#247771=CARTESIAN_POINT('Ctrl Pts',(206.959601774716,-4.48693345015888,
127.111248278652));
#247772=CARTESIAN_POINT('Ctrl Pts',(206.681154150904,-5.53242507739068,
132.583126545744));
#247773=CARTESIAN_POINT('Ctrl Pts',(206.40270652709,-1.49388053201802,136.420413394932));
#247774=CARTESIAN_POINT('Ctrl Pts',(206.124258903278,3.91746311099657,135.0968180907));
#247775=CARTESIAN_POINT('Ctrl Pts',(205.845811279465,5.72885172159717,129.828666190814));
#247776=CARTESIAN_POINT('Ctrl Pts',(205.567363655652,2.27570431130586,125.457128678938));
#247777=CARTESIAN_POINT('Ctrl Pts',(205.288916031839,-3.26870357308214,
125.999436687584));
#247778=CARTESIAN_POINT('Ctrl Pts',(205.010468408026,-5.80933288384994,
130.9572347388));
#247779=CARTESIAN_POINT('Ctrl Pts',(204.732020784213,-3.01146890392974,
135.774549108008));
#247780=CARTESIAN_POINT('Ctrl Pts',(204.4535731604,2.5537877891123,136.024502973214));
#247781=CARTESIAN_POINT('Ctrl Pts',(204.175125536587,5.77223831170541,131.477401078575));
#247782=CARTESIAN_POINT('Ctrl Pts',(203.896677912775,3.6862837897924,126.311807855303));
#247783=CARTESIAN_POINT('Ctrl Pts',(203.618230288961,-1.78718543642468,
125.274651160291));
#247784=CARTESIAN_POINT('Ctrl Pts',(203.339782665149,-5.61831856260093,
129.319027308227));
#247785=CARTESIAN_POINT('Ctrl Pts',(203.061335041336,-4.28649139606962,
134.728352208566));
#247786=CARTESIAN_POINT('Ctrl Pts',(202.782887417523,0.984411954691954,
136.531720532469));
#247787=CARTESIAN_POINT('Ctrl Pts',(202.50443979371,5.3506888113544,133.071924892697));
#247788=CARTESIAN_POINT('Ctrl Pts',(202.225992169897,4.79994404549834,127.528348460205));
#247789=CARTESIAN_POINT('Ctrl Pts',(201.947544546084,-0.161714807569177,
124.995267158526));
#247790=CARTESIAN_POINT('Ctrl Pts',(201.669096922271,-4.97476565284641,
127.800458955558));
#247791=CARTESIAN_POINT('Ctrl Pts',(201.390649298458,-5.21624989388704,
133.366089631302));
#247792=CARTESIAN_POINT('Ctrl Pts',(201.112201674645,-0.664255310463968,
136.577616490799));
#247793=CARTESIAN_POINT('Ctrl Pts',(200.833754050833,4.49815745262305,134.483803242045));
#247794=CARTESIAN_POINT('Ctrl Pts',(200.55530642702,5.52698326394509,129.008761972148));
#247795=CARTESIAN_POINT('Ctrl Pts',(200.276858803207,1.47678146385132,125.183788137525));
#247796=CARTESIAN_POINT('Ctrl Pts',(199.998411179394,-3.93051035674001,
126.523845831826));
#247797=CARTESIAN_POINT('Ctrl Pts',(199.719963555581,-5.7258551755912,131.79748749945));
#247798=CARTESIAN_POINT('Ctrl Pts',(199.441515931768,-2.25941881165118,
136.158494079568));
#247799=CARTESIAN_POINT('Ctrl Pts',(199.163068307955,3.28331306145151,135.599313572066));
#247800=CARTESIAN_POINT('Ctrl Pts',(198.884620684142,5.80884062984016,130.633805545853));
#247801=CARTESIAN_POINT('Ctrl Pts',(198.606173060329,2.99632743704681,125.825029298466));
#247802=CARTESIAN_POINT('Ctrl Pts',(198.327725436517,-2.56966429165962,
125.592015279473));
#247803=CARTESIAN_POINT('Ctrl Pts',(198.049277812704,-5.77426007141042,
130.148891988961));
#247804=CARTESIAN_POINT('Ctrl Pts',(197.770830188891,-3.6725929338218,135.308112346714));
#247805=CARTESIAN_POINT('Ctrl Pts',(197.492382565078,1.80400769380988,136.328604885883));
#247806=CARTESIAN_POINT('Ctrl Pts',(197.213934941265,5.62281338150559,132.272586816804));
#247807=CARTESIAN_POINT('Ctrl Pts',(196.935487317452,4.27452826130232,126.867340597462));
#247808=CARTESIAN_POINT('Ctrl Pts',(196.657039693639,-1.00183950872307,
125.080023442474));
#247809=CARTESIAN_POINT('Ctrl Pts',(196.378592069827,-5.35756571281285,
128.553092501978));
#247810=CARTESIAN_POINT('Ctrl Pts',(196.100144446013,-4.78995075846325,
134.094966979145));
#247811=CARTESIAN_POINT('Ctrl Pts',(195.821696822201,0.179394940810534,
136.612934965078));
#247812=CARTESIAN_POINT('Ctrl Pts',(195.543249198387,4.98388545340951,133.79310689028));
#247813=CARTESIAN_POINT('Ctrl Pts',(195.264801574575,5.20842871066526,128.22676699923));
#247814=CARTESIAN_POINT('Ctrl Pts',(194.986353950762,0.64668042870769,125.029109720981));
#247815=CARTESIAN_POINT('Ctrl Pts',(194.70790632695,-4.50933557513701,127.138625880003));
#247816=CARTESIAN_POINT('Ctrl Pts',(194.429458703136,-5.52149247872048,
132.616773181746));
#247817=CARTESIAN_POINT('Ctrl Pts',(194.151011079324,-1.4596675342632,136.429401878284));
#247818=CARTESIAN_POINT('Ctrl Pts',(193.87256345551,3.9435205654586,135.072892454764));
#247819=CARTESIAN_POINT('Ctrl Pts',(193.594115831698,5.72280591721378,129.793810802232));
#247820=CARTESIAN_POINT('Ctrl Pts',(193.315668207884,2.24311220566103,125.443375061888));
#247821=CARTESIAN_POINT('Ctrl Pts',(193.037220584072,-3.29789204077089,
126.019423148508));
#247822=CARTESIAN_POINT('Ctrl Pts',(192.758772960259,-5.80829461271728,
130.992595012001));
#247823=CARTESIAN_POINT('Ctrl Pts',(192.480325336446,-2.98115818654302,
135.792788662769));
#247824=CARTESIAN_POINT('Ctrl Pts',(192.201877712633,2.58551697539033,136.008860638253));
#247825=CARTESIAN_POINT('Ctrl Pts',(191.92343008882,5.77622834646622,131.442251348686));
#247826=CARTESIAN_POINT('Ctrl Pts',(191.644982465007,3.658868051582,126.289451639914));
#247827=CARTESIAN_POINT('Ctrl Pts',(191.366534841194,-1.82081323706467,
125.285632716038));
#247828=CARTESIAN_POINT('Ctrl Pts',(191.088087217381,-5.6272561125207,129.35325512882));
#247829=CARTESIAN_POINT('Ctrl Pts',(190.809639593569,-4.26252552731426,
134.754372595315));
#247830=CARTESIAN_POINT('Ctrl Pts',(190.531191969755,1.01925778154541,136.525622023071));
#247831=CARTESIAN_POINT('Ctrl Pts',(190.252744345943,5.36439298267566,133.039311718326));
#247832=CARTESIAN_POINT('Ctrl Pts',(189.974296722129,4.77991309789331,127.499190535413));
#247833=CARTESIAN_POINT('Ctrl Pts',(189.695849098317,-0.197073412116412,
124.996359191464));
#247834=CARTESIAN_POINT('Ctrl Pts',(189.417401474504,-4.99295908396257,
127.830797421458));
#247835=CARTESIAN_POINT('Ctrl Pts',(189.138953850692,-5.20055927725872,
133.397794962038));
#247836=CARTESIAN_POINT('Ctrl Pts',(188.860506226878,-0.629099556198964,
136.581553036358));
#247837=CARTESIAN_POINT('Ctrl Pts',(188.582058603065,4.52047192378579,134.456353509349));
#247838=CARTESIAN_POINT('Ctrl Pts',(188.303610979253,5.51595054314194,128.975150924561));
#247839=CARTESIAN_POINT('Ctrl Pts',(188.02516335544,1.44254008251539,125.174902685784));
#247840=CARTESIAN_POINT('Ctrl Pts',(187.746715731627,-3.95649424194195,
126.547851272005));
#247841=CARTESIAN_POINT('Ctrl Pts',(187.468268107814,-5.71970364354381,
131.832324004755));
#247842=CARTESIAN_POINT('Ctrl Pts',(187.189820484001,-2.22678481978599,
136.172148603481));
#247843=CARTESIAN_POINT('Ctrl Pts',(186.911372860188,3.312440468869,135.579238274173));
#247844=CARTESIAN_POINT('Ctrl Pts',(186.632925236375,5.80769478834652,130.598448644184));
#247845=CARTESIAN_POINT('Ctrl Pts',(186.354477612562,2.96596131899707,125.806882058373));
#247846=CARTESIAN_POINT('Ctrl Pts',(186.076029988749,-2.60134570724499,
125.607754128061));
#247847=CARTESIAN_POINT('Ctrl Pts',(185.797582364937,-5.7781431113317,130.184053693262));
#247848=CARTESIAN_POINT('Ctrl Pts',(185.519134741124,-3.64510927408837,
135.33038501822));
#247849=CARTESIAN_POINT('Ctrl Pts',(185.240687117311,1.83760191255446,136.317521027561));
#247850=CARTESIAN_POINT('Ctrl Pts',(184.962239493498,5.63164671340385,132.238331952975));
#247851=CARTESIAN_POINT('Ctrl Pts',(184.683791869685,4.25048330587202,126.841393274542));
#247852=CARTESIAN_POINT('Ctrl Pts',(184.405344245872,-1.03666661210287,
125.086227982629));
#247853=CARTESIAN_POINT('Ctrl Pts',(184.126896622059,-5.37117055753467,
128.585747235914));
#247854=CARTESIAN_POINT('Ctrl Pts',(183.848448998247,-4.7698311568614,134.124063801647));
#247855=CARTESIAN_POINT('Ctrl Pts',(183.570001374433,0.214750057761129,
136.611735317726));
#247856=CARTESIAN_POINT('Ctrl Pts',(183.291553750621,5.00198646042476,133.762713190383));
#247857=CARTESIAN_POINT('Ctrl Pts',(183.013106126807,5.19264166658148,128.195109572179));
#247858=CARTESIAN_POINT('Ctrl Pts',(182.734658502995,0.611512855797894,
125.025280195685));
#247859=CARTESIAN_POINT('Ctrl Pts',(182.456210879182,-4.53156639540017,
127.166143403126));
#247860=CARTESIAN_POINT('Ctrl Pts',(182.177763255369,-5.5103575085511,132.650350493844));
#247861=CARTESIAN_POINT('Ctrl Pts',(181.899315631556,-1.42539926727337,
136.438183069882));
#247862=CARTESIAN_POINT('Ctrl Pts',(181.620868007743,3.96943126600311,135.048808039769));
#247863=CARTESIAN_POINT('Ctrl Pts',(181.34242038393,5.71654838332065,129.758993181434));
#247864=CARTESIAN_POINT('Ctrl Pts',(181.063972760118,2.21043680528058,125.429819927867));
#247865=CARTESIAN_POINT('Ctrl Pts',(180.785525136304,-3.32695821097111,
126.039587007222));
#247866=CARTESIAN_POINT('Ctrl Pts',(180.507077512492,-5.80704116228462,
131.027948262352));
#247867=CARTESIAN_POINT('Ctrl Pts',(180.228629888679,-2.95073697519064,
135.810843394787));
#247868=CARTESIAN_POINT('Ctrl Pts',(179.950182264866,2.61715034058839,135.993025435236));
#247869=CARTESIAN_POINT('Ctrl Pts',(179.671734641053,5.78000434826875,131.407077988614));
#247870=CARTESIAN_POINT('Ctrl Pts',(179.39328701724,3.63131672880039,126.26726272238));
#247871=CARTESIAN_POINT('Ctrl Pts',(179.114839393428,-1.8543735647511,125.296818772266));
#247872=CARTESIAN_POINT('Ctrl Pts',(178.836391769614,-5.63598514348121,
129.387536719606));
#247873=CARTESIAN_POINT('Ctrl Pts',(178.557944145802,-4.23840170853308,
134.780246613475));
#247874=CARTESIAN_POINT('Ctrl Pts',(178.279496521988,1.05406583912245,136.519311509933));
#247875=CARTESIAN_POINT('Ctrl Pts',(178.001048898175,5.3778983746034,133.006615727177));
#247876=CARTESIAN_POINT('Ctrl Pts',(177.722601274363,4.75970502876524,127.470155084831));
#247877=CARTESIAN_POINT('Ctrl Pts',(177.44415365055,-0.232424713990654,
124.997666442073));
#247878=CARTESIAN_POINT('Ctrl Pts',(177.165706026737,-5.01096749916768,
127.861246073811));
#247879=CARTESIAN_POINT('Ctrl Pts',(176.887258402924,-5.18467595198119,
133.429404192122));
#247880=CARTESIAN_POINT('Ctrl Pts',(176.608810779111,-0.593920490425269,
136.585275505922));
#247881=CARTESIAN_POINT('Ctrl Pts',(176.330363155298,4.54261888720253,134.428768450716));
#247882=CARTESIAN_POINT('Ctrl Pts',(176.051915531486,5.50471342676105,128.941607659011));
#247883=CARTESIAN_POINT('Ctrl Pts',(175.773467907672,1.40824524732727,125.166225835676));
#247884=CARTESIAN_POINT('Ctrl Pts',(175.49502028386,-3.98233151779528,126.572014438702));
#247885=CARTESIAN_POINT('Ctrl Pts',(175.216572660047,-5.7133401657742,131.867122418498));
#247886=CARTESIAN_POINT('Ctrl Pts',(174.938125036234,-2.19406831359054,
136.185604222037));
#247887=CARTESIAN_POINT('Ctrl Pts',(174.659677412421,3.34144513258691,135.558986041432));
#247888=CARTESIAN_POINT('Ctrl Pts',(174.381229788608,5.80633374058666,130.563099372659));
#247889=CARTESIAN_POINT('Ctrl Pts',(174.102782164795,2.93548529615992,125.788920001687));
#247890=CARTESIAN_POINT('Ctrl Pts',(173.824334540982,-2.63293072900865,
125.623685538813));
#247891=CARTESIAN_POINT('Ctrl Pts',(173.54588691717,-5.7818120400351,130.219238383264));
#247892=CARTESIAN_POINT('Ctrl Pts',(173.267439293356,-3.61749054349026,
135.352489976228));
#247893=CARTESIAN_POINT('Ctrl Pts',(172.988991669544,1.87112803828436,136.306232877052));
#247894=CARTESIAN_POINT('Ctrl Pts',(172.71054404573,5.64027136256211,132.204023952811));
#247895=CARTESIAN_POINT('Ctrl Pts',(172.432096421918,4.22628084721974,126.815592800833));
#247896=CARTESIAN_POINT('Ctrl Pts',(172.153648798105,-1.07145530142008,
125.092644410292));
#247897=CARTESIAN_POINT('Ctrl Pts',(171.875201174292,-5.38457637155629,
128.618484181386));
#247898=CARTESIAN_POINT('Ctrl Pts',(171.596753550479,-4.74953480741189,
134.153037611328));
#247899=CARTESIAN_POINT('Ctrl Pts',(171.318305926666,0.25009721706947,136.610320475968));
#247900=CARTESIAN_POINT('Ctrl Pts',(171.039858302853,5.01990211699227,133.732209867644));
#247901=CARTESIAN_POINT('Ctrl Pts',(170.76141067904,5.1766622072511,128.163548831885));
#247902=CARTESIAN_POINT('Ctrl Pts',(170.482963055228,0.576322623054293,
125.021664816339));
#247903=CARTESIAN_POINT('Ctrl Pts',(170.204515431414,-4.55362929680409,
127.193795741725));
#247904=CARTESIAN_POINT('Ctrl Pts',(169.926067807602,-5.4990183500578,132.683859402108));
#247905=CARTESIAN_POINT('Ctrl Pts',(169.647620183788,-1.39107818158956,
136.446755498118));
#247906=CARTESIAN_POINT('Ctrl Pts',(169.369172559976,3.99519487781229,135.024566345214));
#247907=CARTESIAN_POINT('Ctrl Pts',(169.090724936163,5.71007902062496,129.724214297113));
#247908=CARTESIAN_POINT('Ctrl Pts',(168.81227731235,2.17767949635139,125.416463949427));
#247909=CARTESIAN_POINT('Ctrl Pts',(168.533829688537,-3.35590109951139,
126.059927426375));
#247910=CARTESIAN_POINT('Ctrl Pts',(168.255382064725,-5.80557252980615,
131.063293227581));
#247911=CARTESIAN_POINT('Ctrl Pts',(167.976934440911,-2.92020642319446,
135.828712609743));
#247912=CARTESIAN_POINT('Ctrl Pts',(167.698486817099,2.64868672631821,135.976997964335));
#247913=CARTESIAN_POINT('Ctrl Pts',(167.420039193286,5.78356616988455,131.371882294628));
#247914=CARTESIAN_POINT('Ctrl Pts',(167.141591569473,3.60363084624196,126.245241928676));
#247915=CARTESIAN_POINT('Ctrl Pts',(166.86314394566,-1.88786517794308,125.308208912483));
#247916=CARTESIAN_POINT('Ctrl Pts',(166.584696321847,-5.64450533093961,
129.421870811324));
#247917=CARTESIAN_POINT('Ctrl Pts',(166.306248698034,-4.21412083421794,
134.805973303719));
#247918=CARTESIAN_POINT('Ctrl Pts',(166.027801074221,1.08883483790225,136.512789227187));
#247919=CARTESIAN_POINT('Ctrl Pts',(165.749353450409,5.3912044865292,132.973838130654));
#247920=CARTESIAN_POINT('Ctrl Pts',(165.470905826595,4.73932058701693,127.441243184462));
#247921=CARTESIAN_POINT('Ctrl Pts',(165.192458202783,-0.267767403281747,
124.999188861871));
#247922=CARTESIAN_POINT('Ctrl Pts',(164.914010578969,-5.02879023112935,
127.891803784357));
#247923=CARTESIAN_POINT('Ctrl Pts',(164.635562955157,-5.16860050662956,
133.46091615025));
#247924=CARTESIAN_POINT('Ctrl Pts',(164.357115331344,-0.55871941670932,
136.588783761558));
#247925=CARTESIAN_POINT('Ctrl Pts',(164.078667707531,4.56459752220588,134.401049088318));
#247926=CARTESIAN_POINT('Ctrl Pts',(163.800220083718,5.49327233119978,128.908133418456));
#247927=CARTESIAN_POINT('Ctrl Pts',(163.521772459905,1.37389822909362,125.157757908727));
#247928=CARTESIAN_POINT('Ctrl Pts',(163.243324836092,-4.00802122688977,
126.596334436543));
#247929=CARTESIAN_POINT('Ctrl Pts',(162.964877212279,-5.70676497808368,
131.901881451211));
#247930=CARTESIAN_POINT('Ctrl Pts',(162.686429588467,-2.16127050538683,
136.198860436632));
#247931=CARTESIAN_POINT('Ctrl Pts',(162.407981964654,3.37032597782655,135.538557624299));
#247932=CARTESIAN_POINT('Ctrl Pts',(162.129534340841,5.80475753699479,130.527759041158));
#247933=CARTESIAN_POINT('Ctrl Pts',(161.851086717028,2.90490049783562,125.771143793998));
#247934=CARTESIAN_POINT('Ctrl Pts',(161.572639093215,-2.66441818655578,
125.639808921385));
#247935=CARTESIAN_POINT('Ctrl Pts',(161.294191469402,-5.7852667215671,130.254444755185));
#247936=CARTESIAN_POINT('Ctrl Pts',(161.015743845589,-3.58973776544978,
135.37442640163));
#247937=CARTESIAN_POINT('Ctrl Pts',(160.737296221776,1.90458482867669,136.294740852644));
#247938=CARTESIAN_POINT('Ctrl Pts',(160.458848597964,5.64868700939082,132.169664087608));
#247939=CARTESIAN_POINT('Ctrl Pts',(160.18040097415,4.20192178217643,126.789940132385));
#247940=CARTESIAN_POINT('Ctrl Pts',(159.901953350338,-1.10620428756715,
125.099272487699));
#247941=CARTESIAN_POINT('Ctrl Pts',(159.623505726525,-5.39778265812024,
128.651302125312));
#247942=CARTESIAN_POINT('Ctrl Pts',(159.345058102712,-4.72906246220349,
134.18188733455));
#247943=CARTESIAN_POINT('Ctrl Pts',(159.066610478899,0.285435108933367,
136.608690492233));
#247944=CARTESIAN_POINT('Ctrl Pts',(158.788162855086,5.03763175924073,133.701598052375));
#247945=CARTESIAN_POINT('Ctrl Pts',(158.509715231273,5.16049092479898,128.132085947844));
#247946=CARTESIAN_POINT('Ctrl Pts',(158.23126760746,0.541111034464008,125.018263716911));
#247947=CARTESIAN_POINT('Ctrl Pts',(157.952819983648,-4.57552346179978,
127.221581871133));
#247948=CARTESIAN_POINT('Ctrl Pts',(157.674372359834,-5.48747542341729,
132.717298664853));
#247949=CARTESIAN_POINT('Ctrl Pts',(157.395924736022,-1.35670554899215,
136.455118845335));
#247950=CARTESIAN_POINT('Ctrl Pts',(157.117477112209,4.02081044620608,135.000168269382));
#247951=CARTESIAN_POINT('Ctrl Pts',(156.839029488396,5.70339806885126,129.68947543801));
#247952=CARTESIAN_POINT('Ctrl Pts',(156.560581864583,2.1448414927076,125.403307621479));
#247953=CARTESIAN_POINT('Ctrl Pts',(156.28213424077,-3.38471963390224,126.080443652244));
#247954=CARTESIAN_POINT('Ctrl Pts',(156.003686616957,-5.8038887697026,131.098628597966));
#247955=CARTESIAN_POINT('Ctrl Pts',(155.725238993144,-2.88956766187541,
135.846395645489));
#247956=CARTESIAN_POINT('Ctrl Pts',(155.446791369331,2.68012496398725,135.960778819456));
#247957=CARTESIAN_POINT('Ctrl Pts',(155.168343745519,5.78691367932904,131.336665570917));
#247958=CARTESIAN_POINT('Ctrl Pts',(154.889896121706,3.57581142981733,126.223390074792));
#247959=CARTESIAN_POINT('Ctrl Pts',(154.611448497893,-1.92128683559663,
125.319802714623));
#247960=CARTESIAN_POINT('Ctrl Pts',(154.33300087408,-5.65281635917722,129.456256131708));
#247961=CARTESIAN_POINT('Ctrl Pts',(154.054553250267,-4.18968380410554,
134.831551712731));
#247962=CARTESIAN_POINT('Ctrl Pts',(153.776105626454,1.12356348950664,136.50605541652));
#247963=CARTESIAN_POINT('Ctrl Pts',(153.497658002641,5.40431082539012,132.940980143345));
#247964=CARTESIAN_POINT('Ctrl Pts',(153.219210378828,4.71876052800142,127.412455905645));
#247965=CARTESIAN_POINT('Ctrl Pts',(152.940762755016,-0.303100170353132,
125.000926394444));
#247966=CARTESIAN_POINT('Ctrl Pts',(152.662315131202,-5.04642661941966,
127.922469420767));
#247967=CARTESIAN_POINT('Ctrl Pts',(152.38386750739,-5.15233353688545,133.492329668737));
#247968=CARTESIAN_POINT('Ctrl Pts',(152.105419883576,-0.523497639439988,
136.592077673268));
#247969=CARTESIAN_POINT('Ctrl Pts',(151.826972259764,4.58640701436939,134.373196449306));
#247970=CARTESIAN_POINT('Ctrl Pts',(151.548524635951,5.48162768041213,128.874729443297));
#247971=CARTESIAN_POINT('Ctrl Pts',(151.270077012138,1.33950030055583,125.149499218718));
#247972=CARTESIAN_POINT('Ctrl Pts',(150.991629388325,-4.03356241728369,
126.620810364342));
#247973=CARTESIAN_POINT('Ctrl Pts',(150.713181764512,-5.69997832411825,
131.936599814887));
#247974=CARTESIAN_POINT('Ctrl Pts',(150.434734140699,-2.1283926105098,136.211916756054));
#247975=CARTESIAN_POINT('Ctrl Pts',(150.156286516886,3.39908193439765,135.517953779753));
#247976=CARTESIAN_POINT('Ctrl Pts',(149.877838893074,5.8029662359777,130.49242895923));
#247977=CARTESIAN_POINT('Ctrl Pts',(149.599391269261,2.87420805735513,125.753554094008));
#247978=CARTESIAN_POINT('Ctrl Pts',(149.320943645448,-2.69580691310719,
125.65612367832));
#247979=CARTESIAN_POINT('Ctrl Pts',(149.042496021635,-5.7885070279132,130.289671504441));
#247980=CARTESIAN_POINT('Ctrl Pts',(148.764048397822,-3.56185196835627,
135.396193481562));
#247981=CARTESIAN_POINT('Ctrl Pts',(148.485600774009,1.93797104397778,136.283045380177));
#247982=CARTESIAN_POINT('Ctrl Pts',(148.207153150196,5.6568933420451,132.135253630582));
#247983=CARTESIAN_POINT('Ctrl Pts',(147.928705526383,4.17740701337624,126.764436219762));
#247984=CARTESIAN_POINT('Ctrl Pts',(147.65025790257,-1.14091228290746,125.106111969245));
#247985=CARTESIAN_POINT('Ctrl Pts',(147.371810278758,-5.41078892786276,
128.684199851613));
#247986=CARTESIAN_POINT('Ctrl Pts',(147.093362654945,-4.70841487984645,
134.210611902278));
#247987=CARTESIAN_POINT('Ctrl Pts',(146.814915031132,0.320762423894332,
136.60684542692));
#247988=CARTESIAN_POINT('Ctrl Pts',(146.536467407319,5.05517473019176,133.670878878906));
#247989=CARTESIAN_POINT('Ctrl Pts',(146.258019783506,5.14412841845787,128.100722085923));
#247990=CARTESIAN_POINT('Ctrl Pts',(145.979572159693,0.505879394805349,
125.015077023433));
#247991=CARTESIAN_POINT('Ctrl Pts',(145.70112453588,-4.59724807909095,127.249500761725));
#247992=CARTESIAN_POINT('Ctrl Pts',(145.422676912067,-5.47572915635697,
132.750667042976));
#247993=CARTESIAN_POINT('Ctrl Pts',(145.144229288255,-1.32228264317164,
136.463272801628));
#247994=CARTESIAN_POINT('Ctrl Pts',(144.865781664442,4.0462770219901,134.975614716357));
#247995=CARTESIAN_POINT('Ctrl Pts',(144.587334040629,5.69650577556471,129.654777891387));
#247996=CARTESIAN_POINT('Ctrl Pts',(144.308886416816,2.11192401117359,125.390351431538));
#247997=CARTESIAN_POINT('Ctrl Pts',(144.030438793003,-3.41341274626234,
126.101134924595));
#247998=CARTESIAN_POINT('Ctrl Pts',(143.75199116919,-5.80198994436631,131.133953064144));
#247999=CARTESIAN_POINT('Ctrl Pts',(143.473543545377,-2.85882182656403,
135.863891846773));
#248000=CARTESIAN_POINT('Ctrl Pts',(143.195095921564,2.71146388864014,135.944368601604));
#248001=CARTESIAN_POINT('Ctrl Pts',(142.916648297751,5.790046752559,131.301429122451));
#248002=CARTESIAN_POINT('Ctrl Pts',(142.638200673938,3.54785951038517,126.201707970457));
#248003=CARTESIAN_POINT('Ctrl Pts',(142.359753050125,-1.95463729925998,
125.331599749072));
#248004=CARTESIAN_POINT('Ctrl Pts',(142.081305426313,-5.66091792022584,
129.490691406602));
#248005=CARTESIAN_POINT('Ctrl Pts',(141.8028578025,-4.16509152371897,134.856980892698));
#248006=CARTESIAN_POINT('Ctrl Pts',(141.524410178687,1.15825050705268,136.499110327454));
#248007=CARTESIAN_POINT('Ctrl Pts',(141.245962554874,5.41721690552589,132.908042982814));
#248008=CARTESIAN_POINT('Ctrl Pts',(140.967514931061,4.69802561357932,127.383794315106));
#248009=CARTESIAN_POINT('Ctrl Pts',(140.689067307248,-0.338421705936203,
125.002878975406));
#248010=CARTESIAN_POINT('Ctrl Pts',(140.410619683435,-5.06387601051571,
127.953241846716));
#248011=CARTESIAN_POINT('Ctrl Pts',(140.132172059623,-5.13587564552739,
133.523643583541));
#248012=CARTESIAN_POINT('Ctrl Pts',(139.85372443581,-0.48825646377323,136.595157118993));
#248013=CARTESIAN_POINT('Ctrl Pts',(139.575276811997,4.60804655553434,134.34521156577));
#248014=CARTESIAN_POINT('Ctrl Pts',(139.296829188184,5.46977990589493,128.841396971331));
#248015=CARTESIAN_POINT('Ctrl Pts',(139.018381564371,1.30505273634171,125.141450071677));
#248016=CARTESIAN_POINT('Ctrl Pts',(138.739933940558,-4.05895414253892,
126.645441315135));
#248017=CARTESIAN_POINT('Ctrl Pts',(138.461486316745,-5.69298045535984,
131.971276223022));
#248018=CARTESIAN_POINT('Ctrl Pts',(138.183038692932,-2.09543584726193,
136.224772696493));
#248019=CARTESIAN_POINT('Ctrl Pts',(137.904591069119,3.42771193673771,135.49717527128));
#248020=CARTESIAN_POINT('Ctrl Pts',(137.626143445306,5.80095990391266,130.457110436044));
#248021=CARTESIAN_POINT('Ctrl Pts',(137.347695821494,2.84340911203807,125.736151553513));
#248022=CARTESIAN_POINT('Ctrl Pts',(137.069248197681,-2.727095745542,125.672629205068));
#248023=CARTESIAN_POINT('Ctrl Pts',(136.790800573868,-5.7915328390027,130.324917325691));
#248024=CARTESIAN_POINT('Ctrl Pts',(136.512352950055,-3.53383418552815,
135.417790409441));
#248025=CARTESIAN_POINT('Ctrl Pts',(136.233905326242,1.97128544704926,136.271146893031));
#248026=CARTESIAN_POINT('Ctrl Pts',(135.955457702429,5.66489005643625,132.100793856825));
#248027=CARTESIAN_POINT('Ctrl Pts',(135.677010078616,4.15273744922295,126.739082008025));
#248028=CARTESIAN_POINT('Ctrl Pts',(135.398562454803,-1.17557800132362,
125.113162601491));
#248029=CARTESIAN_POINT('Ctrl Pts',(135.12011483099,-5.42359469883174,128.717176141249));
#248030=CARTESIAN_POINT('Ctrl Pts',(134.841667207177,-4.68759282544451,
134.239210250113));
#248031=CARTESIAN_POINT('Ctrl Pts',(134.563219583365,0.356077852885664,
136.604785348398));
#248032=CARTESIAN_POINT('Ctrl Pts',(134.284771959552,5.0725303797842,133.640053485549));
#248033=CARTESIAN_POINT('Ctrl Pts',(134.006324335739,5.12757529454644,128.069458408322));
#248034=CARTESIAN_POINT('Ctrl Pts',(133.727876711926,0.470629009599695,
125.012104853988));
#248035=CARTESIAN_POINT('Ctrl Pts',(133.449429088113,-4.61880234366392,
127.277551378957));
#248036=CARTESIAN_POINT('Ctrl Pts',(133.1709814643,-5.46377998413907,132.783963299997));
#248037=CARTESIAN_POINT('Ctrl Pts',(132.892533840487,-1.28781073968153,
136.47121706485));
#248038=CARTESIAN_POINT('Ctrl Pts',(132.614086216674,4.07159366149105,134.950906595976));
#248039=CARTESIAN_POINT('Ctrl Pts',(132.335638592862,5.68940239616175,129.620122942976));
#248040=CARTESIAN_POINT('Ctrl Pts',(132.057190969048,2.07892827151876,125.377595859696));
#248041=CARTESIAN_POINT('Ctrl Pts',(131.778743345236,-3.44197937335791,
126.122000476702));
#248042=CARTESIAN_POINT('Ctrl Pts',(131.500295721423,-5.79987612415893,
131.169265317152));
#248043=CARTESIAN_POINT('Ctrl Pts',(131.22184809761,-2.82797005655853,135.881200565267));
#248044=CARTESIAN_POINT('Ctrl Pts',(130.943400473797,2.74270233900145,135.927767918864));
#248045=CARTESIAN_POINT('Ctrl Pts',(130.664952849984,5.79296527347731,131.26617425493));
#248046=CARTESIAN_POINT('Ctrl Pts',(130.386505226171,3.51977612371406,126.180196419108));
#248047=CARTESIAN_POINT('Ctrl Pts',(130.108057602358,-1.98791533311939,
125.343599578688));
#248048=CARTESIAN_POINT('Ctrl Pts',(129.829609978546,-5.66880971387908,
129.52517535999));
#248049=CARTESIAN_POINT('Ctrl Pts',(129.551162354732,-4.14034490433441,
134.882259901329));
#248050=CARTESIAN_POINT('Ctrl Pts',(129.27271473092,1.19289460520041,136.491954217345));
#248051=CARTESIAN_POINT('Ctrl Pts',(128.994267107107,5.42992224869717,132.875027869557));
#248052=CARTESIAN_POINT('Ctrl Pts',(128.715819483294,4.67711661209022,127.355259474909));
#248053=CARTESIAN_POINT('Ctrl Pts',(128.437371859481,-0.373730701178542,
125.005046532403));
#248054=CARTESIAN_POINT('Ctrl Pts',(128.158924235668,-5.0811377578241,127.984119921918));
#248055=CARTESIAN_POINT('Ctrl Pts',(127.880476611855,-5.11922744240848,
133.554856734316));
#248056=CARTESIAN_POINT('Ctrl Pts',(127.602028988042,-0.452997195583419,
136.598021984625));
#248057=CARTESIAN_POINT('Ctrl Pts',(127.323581364229,4.62951534383955,134.3170954747));
#248058=CARTESIAN_POINT('Ctrl Pts',(127.045133740417,5.45772944667181,128.808137237705));
#248059=CARTESIAN_POINT('Ctrl Pts',(126.766686116604,1.2705568129186,125.133610765869));
#248060=CARTESIAN_POINT('Ctrl Pts',(126.488238492791,-4.08419546175569,
126.67022637621));
#248061=CARTESIAN_POINT('Ctrl Pts',(126.209790868978,-5.68577163111709,
132.005909390672));
#248062=CARTESIAN_POINT('Ctrl Pts',(125.931343245165,-2.06240143686808,
136.237427781569));
#248063=CARTESIAN_POINT('Ctrl Pts',(125.652895621352,3.45621492395137,135.476222868834));
#248064=CARTESIAN_POINT('Ctrl Pts',(125.374447997539,5.79873861514512,130.421804780342));
#248065=CARTESIAN_POINT('Ctrl Pts',(125.096000373726,2.8125048031507,125.718936817367));
#248066=CARTESIAN_POINT('Ctrl Pts',(124.817552749914,-2.75828352444112,
125.68932489001));
#248067=CARTESIAN_POINT('Ctrl Pts',(124.5391051261,-5.79434404271298,130.36018091289));
#248068=CARTESIAN_POINT('Ctrl Pts',(124.260657502288,-3.50568545517477,
135.439216384981));
#248069=CARTESIAN_POINT('Ctrl Pts',(123.982209878475,2.00452680341345,136.25904583211));
#248070=CARTESIAN_POINT('Ctrl Pts',(123.703762254662,5.67267685624313,132.066286043259));
#248071=CARTESIAN_POINT('Ctrl Pts',(123.425314630849,4.12791400385628,126.71387843668));
#248072=CARTESIAN_POINT('Ctrl Pts',(123.146867007036,-1.21020015826455,
125.120424123171));
#248073=CARTESIAN_POINT('Ctrl Pts',(122.868419383223,-5.43619949650465,
128.750229772276));
#248074=CARTESIAN_POINT('Ctrl Pts',(122.58997175941,-4.66659707056658,134.267681318331));
#248075=CARTESIAN_POINT('Ctrl Pts',(122.311524135597,0.391380087281262,
136.602510333005));
#248076=CARTESIAN_POINT('Ctrl Pts',(122.033076511785,5.08969806489794,133.609123014551));
#248077=CARTESIAN_POINT('Ctrl Pts',(121.754628887972,5.11083216644683,128.038296073528));
#248078=CARTESIAN_POINT('Ctrl Pts',(121.476181264159,0.435361185062875,
125.00934731871));
#248079=CARTESIAN_POINT('Ctrl Pts',(121.197733640346,-4.64018545681751,
127.305732683402));
#248080=CARTESIAN_POINT('Ctrl Pts',(120.919286016533,-5.45162834954452,
132.817186202114));
#248081=CARTESIAN_POINT('Ctrl Pts',(120.64083839272,-1.25329111589093,136.478951340622));
#248082=CARTESIAN_POINT('Ctrl Pts',(120.362390768907,4.09675942659154,134.92604482381));
#248083=CARTESIAN_POINT('Ctrl Pts',(120.083943145094,5.68208819386074,129.585511876926));
#248084=CARTESIAN_POINT('Ctrl Pts',(119.805495521281,2.04585549641223,125.36504137862));
#248085=CARTESIAN_POINT('Ctrl Pts',(119.527047897469,-3.47041845664194,
126.143039535386));
#248086=CARTESIAN_POINT('Ctrl Pts',(119.248600273655,-5.79754738740892,
131.204564048482));
#248087=CARTESIAN_POINT('Ctrl Pts',(118.970152649843,-2.7970134950826,135.898321159589));
#248088=CARTESIAN_POINT('Ctrl Pts',(118.69170502603,2.77383915751901,135.910977386384));
#248089=CARTESIAN_POINT('Ctrl Pts',(118.413257402217,5.795669133937,131.230902274733));
#248090=CARTESIAN_POINT('Ctrl Pts',(118.134809778404,3.49156231044436,126.158856217863));
#248091=CARTESIAN_POINT('Ctrl Pts',(117.856362154591,-2.02111970404504,
125.355801758813));
#248092=CARTESIAN_POINT('Ctrl Pts',(117.577914530778,-5.67649144770371,
129.559706714059));
#248093=CARTESIAN_POINT('Ctrl Pts',(117.299466906965,-4.11544486294674,
134.907387801903));
#248094=CARTESIAN_POINT('Ctrl Pts',(117.021019283153,1.22749450019975,136.484587351363));
#248095=CARTESIAN_POINT('Ctrl Pts',(116.74257165934,5.44242638410263,132.841936026965));
#248096=CARTESIAN_POINT('Ctrl Pts',(116.464124035527,4.65603429832517,127.326852442422));
#248097=CARTESIAN_POINT('Ctrl Pts',(116.185676411714,-0.409025847692317,
125.007428985116));
#248098=CARTESIAN_POINT('Ctrl Pts',(115.907228787901,-5.09821122170419,
128.015102502178));
#248099=CARTESIAN_POINT('Ctrl Pts',(115.628781164088,-5.10238954443416,
133.585967964446));
#248100=CARTESIAN_POINT('Ctrl Pts',(115.350333540275,-0.417721141415912,
136.600672164005));
#248101=CARTESIAN_POINT('Ctrl Pts',(115.071885916462,4.65081258375125,134.288849217947));
#248102=CARTESIAN_POINT('Ctrl Pts',(114.793438292649,5.44547674927697,128.77495147487));
#248103=CARTESIAN_POINT('Ctrl Pts',(114.514990668836,1.23601380854556,125.125981591782));
#248104=CARTESIAN_POINT('Ctrl Pts',(114.236543045024,-4.10928543960769,
126.695164629152));
#248105=CARTESIAN_POINT('Ctrl Pts',(113.958095421211,-5.67835211851559,
132.040498034489));
#248106=CARTESIAN_POINT('Ctrl Pts',(113.679647797398,-2.02929060343055,
136.249881542344));
#248107=CARTESIAN_POINT('Ctrl Pts',(113.401200173585,3.48458983985001,135.455097348814));
#248108=CARTESIAN_POINT('Ctrl Pts',(113.122752549772,5.79630245198571,130.386513300387));
#248109=CARTESIAN_POINT('Ctrl Pts',(112.844304925959,2.78149627586357,125.701910523471));
#248110=CARTESIAN_POINT('Ctrl Pts',(112.565857302146,-2.78936909412988,
125.706210114483));
#248111=CARTESIAN_POINT('Ctrl Pts',(112.287409678333,-5.7969405348739,130.395460959329));
#248112=CARTESIAN_POINT('Ctrl Pts',(112.008962054521,-3.47740682035766,
135.460470614237));
#248113=CARTESIAN_POINT('Ctrl Pts',(111.730514430707,2.03769388129978,136.246742645822));
#248114=CARTESIAN_POINT('Ctrl Pts',(111.452066806895,5.68025345292297,132.031731468582));
#248115=CARTESIAN_POINT('Ctrl Pts',(111.173619183082,4.10293759711819,126.688826439658));
#248116=CARTESIAN_POINT('Ctrl Pts',(110.895171559269,-1.24477747079359,
125.127896265209));
#248117=CARTESIAN_POINT('Ctrl Pts',(110.616723935456,-5.44860285380605,
128.783359519875));
#248118=CARTESIAN_POINT('Ctrl Pts',(110.338276311643,-4.64542839321807,
134.296024051927));
#248119=CARTESIAN_POINT('Ctrl Pts',(110.05982868783,0.426667818943798,136.600020465042));
#248120=CARTESIAN_POINT('Ctrl Pts',(109.781381064017,5.10667714937814,133.57808861205));
#248121=CARTESIAN_POINT('Ctrl Pts',(109.502933440204,5.0938996545818,128.007236236273));
#248122=CARTESIAN_POINT('Ctrl Pts',(109.224485816392,0.400077228057368,
125.006804519781));
#248123=CARTESIAN_POINT('Ctrl Pts',(108.946038192578,-4.66139662619255,
127.334043630792));
#248124=CARTESIAN_POINT('Ctrl Pts',(108.667590568766,-5.43927470285667,
132.850334518237));
#248125=CARTESIAN_POINT('Ctrl Pts',(108.389142944953,-1.21872505093712,
136.486475342347));
#248126=CARTESIAN_POINT('Ctrl Pts',(108.11069532114,4.1217733847649,134.901030321119));
#248127=CARTESIAN_POINT('Ctrl Pts',(107.832247697327,5.67456343969215,129.550945975765));
#248128=CARTESIAN_POINT('Ctrl Pts',(107.553800073514,2.01270691137792,125.352688453517));
#248129=CARTESIAN_POINT('Ctrl Pts',(107.275352449701,-3.49872894229381,
126.164251321038));
#248130=CARTESIAN_POINT('Ctrl Pts',(106.996904825888,-5.7950038204084,131.239847950126));
#248131=CARTESIAN_POINT('Ctrl Pts',(106.718457202076,-2.76595328924301,
135.91525299533));
#248132=CARTESIAN_POINT('Ctrl Pts',(106.440009578262,2.80487319040651,135.893997626342));
#248133=CARTESIAN_POINT('Ctrl Pts',(106.16156195445,5.7981582337456,131.195614488879));
#248134=CARTESIAN_POINT('Ctrl Pts',(105.883114330637,3.46321911604922,126.137688157493));
#248135=CARTESIAN_POINT('Ctrl Pts',(105.604666706824,-2.05424918163679,
125.36820583729));
#248136=CARTESIAN_POINT('Ctrl Pts',(105.326219083011,-5.68396283705021,
129.594284189235));
#248137=CARTESIAN_POINT('Ctrl Pts',(105.047771459198,-4.09039232223623,
134.932363663296));
#248138=CARTESIAN_POINT('Ctrl Pts',(104.769323835385,1.26204890993897,136.47701000249));
#248139=CARTESIAN_POINT('Ctrl Pts',(104.490876211572,5.45472884839698,132.808768681268));
#248140=CARTESIAN_POINT('Ctrl Pts',(104.21242858776,4.63477945349693,127.29857427028));
#248141=CARTESIAN_POINT('Ctrl Pts',(103.933980963947,-0.444305837602887,
125.010026245263));
#248142=CARTESIAN_POINT('Ctrl Pts',(103.655533340134,-5.1150957694926,128.046188439421));
#248143=CARTESIAN_POINT('Ctrl Pts',(103.377085716321,-5.08536257553889,
133.616976121092));
#248144=CARTESIAN_POINT('Ctrl Pts',(103.098638092508,-0.38242960843803,
136.603107558928));
#248145=CARTESIAN_POINT('Ctrl Pts',(102.820190468695,4.6719374860923,134.260473842188));
#248146=CARTESIAN_POINT('Ctrl Pts',(102.541742844882,5.4330222677386,128.741840912539));
#248147=CARTESIAN_POINT('Ctrl Pts',(102.263295221069,1.2014250032263,125.118562832119));
#248148=CARTESIAN_POINT('Ctrl Pts',(101.984847597256,-4.13422314637653,
126.720255149861));
#248149=CARTESIAN_POINT('Ctrl Pts',(101.706399973443,-5.67072219248816,
132.07504087278));
#248150=CARTESIAN_POINT('Ctrl Pts',(101.427952349631,-1.99610457388343,
136.262133517338));
#248151=CARTESIAN_POINT('Ctrl Pts',(101.149504725818,3.51283563299066,135.433799494034));
#248152=CARTESIAN_POINT('Ctrl Pts',(100.871057102005,5.7936515047074,130.351237303918));
#248153=CARTESIAN_POINT('Ctrl Pts',(100.592609478192,2.75038467920892,125.685073302739));
#248154=CARTESIAN_POINT('Ctrl Pts',(100.314161854379,-2.82035130272114,
125.723284252797));
#248155=CARTESIAN_POINT('Ctrl Pts',(100.035714230566,-5.79932221927147,
130.430756157697));
#248156=CARTESIAN_POINT('Ctrl Pts',(99.7572666067534,-3.44899932895201,
135.481552309624));
#248157=CARTESIAN_POINT('Ctrl Pts',(99.4788189829407,2.07078545168999,136.234237790066));
#248158=CARTESIAN_POINT('Ctrl Pts',(99.2003713591278,5.6876195657222,131.997131413226));
#248159=CARTESIAN_POINT('Ctrl Pts',(98.9219237353147,4.07780915451857,126.663926945268));
#248160=CARTESIAN_POINT('Ctrl Pts',(98.6434761115021,-1.27930865763567,
125.13557875072));
#248161=CARTESIAN_POINT('Ctrl Pts',(98.3650284876889,-5.460804311125,128.816564156414));
#248162=CARTESIAN_POINT('Ctrl Pts',(98.0865808638763,-4.62408757781209,
134.324237400649));
#248163=CARTESIAN_POINT('Ctrl Pts',(97.8081332400632,0.461939740273397,
136.597315836771));
#248164=CARTESIAN_POINT('Ctrl Pts',(97.5296856162504,5.12346700405862,133.546951428038));
#248165=CARTESIAN_POINT('Ctrl Pts',(97.2512379924375,5.07677838639178,127.97628004749));
#248166=CARTESIAN_POINT('Ctrl Pts',(96.9727903686245,0.364778446043045,
125.004476551425));
#248167=CARTESIAN_POINT('Ctrl Pts',(96.6943427448119,-4.68243506580139,
127.362483172053));
#248168=CARTESIAN_POINT('Ctrl Pts',(96.4158951209985,-5.42671950184442,
132.883407020047));
#248169=CARTESIAN_POINT('Ctrl Pts',(96.1374474971861,-1.18411382567837,
136.493788791223));
#248170=CARTESIAN_POINT('Ctrl Pts',(95.8589998733729,4.14663460910971,134.875864014826));
#248171=CARTESIAN_POINT('Ctrl Pts',(95.5805522495601,5.66682841248846,129.516426520346));
#248172=CARTESIAN_POINT('Ctrl Pts',(95.3021046257473,1.97948374474885,125.340537542131));
#248173=CARTESIAN_POINT('Ctrl Pts',(95.0236570019342,-3.52690978125809,
126.185635047646));
#248174=CARTESIAN_POINT('Ctrl Pts',(94.7452093781216,-5.79224551741027,
131.275115714627));
#248175=CARTESIAN_POINT('Ctrl Pts',(94.4667617543085,-2.73479058998699,
135.931995445075));
#248176=CARTESIAN_POINT('Ctrl Pts',(94.1883141304955,2.8358032876865,135.876829267928));
#248177=CARTESIAN_POINT('Ctrl Pts',(93.909866506683,5.80043248066857,131.160312204968));
#248178=CARTESIAN_POINT('Ctrl Pts',(93.6314188828698,3.43474759079615,126.116693022386));
#248179=CARTESIAN_POINT('Ctrl Pts',(93.352971259057,-2.08730253826965,125.380811354481));
#248180=CARTESIAN_POINT('Ctrl Pts',(93.0745236352441,-5.69122360506351,
129.628906504239));
#248181=CARTESIAN_POINT('Ctrl Pts',(92.7960760114314,-4.06518821053398,
134.957186560018));
#248182=CARTESIAN_POINT('Ctrl Pts',(92.5176283876181,1.29655655399172,136.469222451509));
#248183=CARTESIAN_POINT('Ctrl Pts',(92.2391807638055,5.46682918570788,132.775527061492));
#248184=CARTESIAN_POINT('Ctrl Pts',(91.9607331399925,4.61335286521161,127.270426006341));
#248185=CARTESIAN_POINT('Ctrl Pts',(91.6822855161797,-0.479569363597252,
125.012838216602));
#248186=CARTESIAN_POINT('Ctrl Pts',(91.4038378923669,-5.13179077552621,
128.077376581749));
#248187=CARTESIAN_POINT('Ctrl Pts',(91.1253902685539,-5.06814716666323,
133.647880055237));
#248188=CARTESIAN_POINT('Ctrl Pts',(90.846942644741,-0.347123904390365,
136.605328079151));
#248189=CARTESIAN_POINT('Ctrl Pts',(90.5684950209282,4.69288926807169,134.231970398883));
#248190=CARTESIAN_POINT('Ctrl Pts',(90.2900473971151,5.42036646356212,128.708806777632));
#248191=CARTESIAN_POINT('Ctrl Pts',(90.0115997733025,1.16679167866171,125.111354761782));
#248192=CARTESIAN_POINT('Ctrl Pts',(89.7331521494893,-4.15900765798632,
126.7454970086));
#248193=CARTESIAN_POINT('Ctrl Pts',(89.4547045256766,-5.66288213576447,
132.109536625546));
#248194=CARTESIAN_POINT('Ctrl Pts',(89.1762569018636,-1.96284457794726,
136.274183252551));
#248195=CARTESIAN_POINT('Ctrl Pts',(88.8978092780507,3.5409512567151,135.412330093694));
#248196=CARTESIAN_POINT('Ctrl Pts',(88.619361654238,5.79078587154194,130.3159780981));
#248197=CARTESIAN_POINT('Ctrl Pts',(88.3409140304249,2.71917116603865,125.668425779081));
#248198=CARTESIAN_POINT('Ctrl Pts',(88.0624664066122,-2.85122900215762,
125.740546672265));
#248199=CARTESIAN_POINT('Ctrl Pts',(87.7840187827991,-5.80148900765152,
130.466065200115));
#248200=CARTESIAN_POINT('Ctrl Pts',(87.5055711589863,-3.42046403360785,
135.502460689953));
#248201=CARTESIAN_POINT('Ctrl Pts',(87.2271235351733,2.10380028836375,136.221531728214));
#248202=CARTESIAN_POINT('Ctrl Pts',(86.9486759113605,5.69477492168681,131.962487159311));
#248203=CARTESIAN_POINT('Ctrl Pts',(86.6702282875477,4.05252960720113,126.63918087617));
#248204=CARTESIAN_POINT('Ctrl Pts',(86.3917806637346,-1.31379243922498,
125.14347129503));
#248205=CARTESIAN_POINT('Ctrl Pts',(86.113333039922,-5.47280341633199,128.849842451481));
#248206=CARTESIAN_POINT('Ctrl Pts',(85.8348854161089,-4.6025754151404,134.352320319043));
#248207=CARTESIAN_POINT('Ctrl Pts',(85.5564377922961,0.497194544256039,
136.594396548415));
#248208=CARTESIAN_POINT('Ctrl Pts',(85.2779901684829,5.1400670067851,133.515712616316));
#248209=CARTESIAN_POINT('Ctrl Pts',(84.9995425446705,5.05946899631168,127.945428654274));
#248210=CARTESIAN_POINT('Ctrl Pts',(84.7210949208572,0.329466147029263,
125.002363499906));
#248211=CARTESIAN_POINT('Ctrl Pts',(84.4426472970446,-4.70329999605691,
127.391050253351));
#248212=CARTESIAN_POINT('Ctrl Pts',(84.1641996732315,-5.41396321174535,
132.916402482027));
#248213=CARTESIAN_POINT('Ctrl Pts',(83.8857520494189,-1.14945872264635,
136.500891416245));
#248214=CARTESIAN_POINT('Ctrl Pts',(83.6073044256056,4.17134217838416,134.850546837477));
#248215=CARTESIAN_POINT('Ctrl Pts',(83.328856801793,5.65888339887398,129.481954789796));
#248216=CARTESIAN_POINT('Ctrl Pts',(83.05040917798,1.94618722762166,125.328589094719));
#248217=CARTESIAN_POINT('Ctrl Pts',(82.7719615541671,-3.5549599292834,126.207189922827));
#248218=CARTESIAN_POINT('Ctrl Pts',(82.4935139303543,-5.78927258062435,
131.310366035126));
#248219=CARTESIAN_POINT('Ctrl Pts',(82.2150663065413,-2.70352655206008,
135.948547888425));
#248220=CARTESIAN_POINT('Ctrl Pts',(81.9366186827285,2.86662830323276,135.859472947324));
#248221=CARTESIAN_POINT('Ctrl Pts',(81.6581710589156,5.80249179043285,131.124996731141));
#248222=CARTESIAN_POINT('Ctrl Pts',(81.3797234351026,3.40614878970799,126.095871590527));
#248223=CARTESIAN_POINT('Ctrl Pts',(81.1012758112897,-2.12027854913937,
125.393617843285));
#248224=CARTESIAN_POINT('Ctrl Pts',(80.822828187477,-5.6982734826932,129.663572376127));
#248225=CARTESIAN_POINT('Ctrl Pts',(80.5443805636639,-4.03983346178761,
134.981855572247));
#248226=CARTESIAN_POINT('Ctrl Pts',(80.2659329398512,1.33101615366455,136.461224986989));
#248227=CARTESIAN_POINT('Ctrl Pts',(79.9874853160382,5.47872694765296,132.742212399419));
#248228=CARTESIAN_POINT('Ctrl Pts',(79.7090376922254,4.59175532743923,127.242408693648));
#248229=CARTESIAN_POINT('Ctrl Pts',(79.4305900684125,-0.514815118972584,
125.015864794932));
#248230=CARTESIAN_POINT('Ctrl Pts',(79.1521424445996,-5.1482956211654,128.108665773475));
#248231=CARTESIAN_POINT('Ctrl Pts',(78.8736948207867,-5.05074395573051,
133.678678621723));
#248232=CARTESIAN_POINT('Ctrl Pts',(78.5952471969738,-0.31180533753877,
136.607333642391));
#248233=CARTESIAN_POINT('Ctrl Pts',(78.3167995731609,4.71366715331346,134.203339944237));
#248234=CARTESIAN_POINT('Ctrl Pts',(78.0383519493481,5.407509805713,128.675850294243));
#248235=CARTESIAN_POINT('Ctrl Pts',(77.7599043255351,1.1321151182024,125.104357647873));
#248236=CARTESIAN_POINT('Ctrl Pts',(77.4814567017223,-4.18363805603787,
126.770889270024));
#248237=CARTESIAN_POINT('Ctrl Pts',(77.2030090779094,-5.65483223886072,
132.143984014535));
#248238=CARTESIAN_POINT('Ctrl Pts',(76.9245614540965,-1.92951184808342,
136.286030301474));
#248239=CARTESIAN_POINT('Ctrl Pts',(76.6461138302835,3.56893566918854,135.390689943351));
#248240=CARTESIAN_POINT('Ctrl Pts',(76.3676662064707,5.78770565867644,130.280736989476));
#248241=CARTESIAN_POINT('Ctrl Pts',(76.0892185826578,2.68785689298084,125.651968569378));
#248242=CARTESIAN_POINT('Ctrl Pts',(75.8107709588449,-2.8820010482549,125.75799673322));
#248243=CARTESIAN_POINT('Ctrl Pts',(75.532323335032,-5.8034408197229,130.501386778194));
#248244=CARTESIAN_POINT('Ctrl Pts',(75.2538757112192,-3.39180199171105,
135.523194980456));
#248245=CARTESIAN_POINT('Ctrl Pts',(74.9754280874062,2.13673716794415,136.208624931095));
#248246=CARTESIAN_POINT('Ctrl Pts',(74.6969804635933,5.70171925567246,131.92779999059));
#248247=CARTESIAN_POINT('Ctrl Pts',(74.4185328397805,4.02709989190878,126.61458914934));
#248248=CARTESIAN_POINT('Ctrl Pts',(74.1400852159675,-1.34822753775231,
125.151573605674));
#248249=CARTESIAN_POINT('Ctrl Pts',(73.8616375921548,-5.48459972479585,
128.883193171938));
#248250=CARTESIAN_POINT('Ctrl Pts',(73.5831899683417,-4.58089270234404,
134.380271766487));
#248251=CARTESIAN_POINT('Ctrl Pts',(73.3047423445289,0.532430924512096,
136.591262708148));
#248252=CARTESIAN_POINT('Ctrl Pts',(73.026294720716,5.15647654243839,133.484373334449));
#248253=CARTESIAN_POINT('Ctrl Pts',(72.7478470969032,5.04197212574731,127.914683199832));
#248254=CARTESIAN_POINT('Ctrl Pts',(72.46939947309,0.294141639526237,125.000465443524));
#248255=CARTESIAN_POINT('Ctrl Pts',(72.1909518492774,-4.72399064380143,
127.419743816117));
#248256=CARTESIAN_POINT('Ctrl Pts',(71.9125042254643,-5.40100630524849,
132.949319681519));
#248257=CARTESIAN_POINT('Ctrl Pts',(71.6340566016516,-1.11476102599866,
136.507782954223));
#248258=CARTESIAN_POINT('Ctrl Pts',(71.3556089778387,4.19589517704018,134.82507972721));
#248259=CARTESIAN_POINT('Ctrl Pts',(71.0771613540258,5.65072869325411,129.447532061481));
#248260=CARTESIAN_POINT('Ctrl Pts',(70.7987137302128,1.91281859381102,125.316843554035));
#248261=CARTESIAN_POINT('Ctrl Pts',(70.5202661064001,-3.58287834696108,
126.22891514786));
#248262=CARTESIAN_POINT('Ctrl Pts',(70.241818482587,-5.78608512021397,131.345597605407));
#248263=CARTESIAN_POINT('Ctrl Pts',(69.9633708587742,-2.67216233396265,
135.964909712024));
#248264=CARTESIAN_POINT('Ctrl Pts',(69.6849232349613,2.89734709481291,135.841929307673));
#248265=CARTESIAN_POINT('Ctrl Pts',(69.4064756111484,5.80433608672999,131.089669376025));
#248266=CARTESIAN_POINT('Ctrl Pts',(69.1280279873355,3.37742377252397,126.07522463346));
#248267=CARTESIAN_POINT('Ctrl Pts',(68.8495803635227,-2.15317599230747,
125.406624829152));
#248268=CARTESIAN_POINT('Ctrl Pts',(68.5711327397097,-5.70511220870344,
129.698280520343));
#248269=CARTESIAN_POINT('Ctrl Pts',(68.2926851158969,-4.01432901552682,
135.006369785865));
#248270=CARTESIAN_POINT('Ctrl Pts',(68.014237492084,1.36542643204398,136.45301790528));
#248271=CARTESIAN_POINT('Ctrl Pts',(67.735789868271,5.49042169335597,132.708825929535));
#248272=CARTESIAN_POINT('Ctrl Pts',(67.4573422444582,4.56998764048497,127.214523370394));
#248273=CARTESIAN_POINT('Ctrl Pts',(67.1788946206453,-0.550041797684044,
125.019105868103));
#248274=CARTESIAN_POINT('Ctrl Pts',(66.9004469968323,-5.164609694817,128.140054855163));
#248275=CARTESIAN_POINT('Ctrl Pts',(66.6219993730196,-5.03315358762317,
133.709370679297));
#248276=CARTESIAN_POINT('Ctrl Pts',(66.3435517492066,-0.2764752166261,136.609124174332));
#248277=CARTESIAN_POINT('Ctrl Pts',(66.0651041253938,4.73427037188528,134.174583539162));
#248278=CARTESIAN_POINT('Ctrl Pts',(65.7866565015808,5.39445277059944,128.642972683589));
#248279=CARTESIAN_POINT('Ctrl Pts',(65.508208877768,1.0973966068015,125.097571749668));
#248280=CARTESIAN_POINT('Ctrl Pts',(65.2297612539551,-4.20811342784249,
126.796430993211));
#248281=CARTESIAN_POINT('Ctrl Pts',(64.9513136301422,-5.64657280006891,
132.178381763287));
#248282=CARTESIAN_POINT('Ctrl Pts',(64.6728660063292,-1.89610761944867,
136.297674225111));
#248283=CARTESIAN_POINT('Ctrl Pts',(64.3944183825164,3.59678783343796,135.368879844889));
#248284=CARTESIAN_POINT('Ctrl Pts',(64.1159707587035,5.78441098024938,130.245515283918));
#248285=CARTESIAN_POINT('Ctrl Pts',(63.8375231348906,2.65644302039782,125.635702283457));
#248286=CARTESIAN_POINT('Ctrl Pts',(63.5590755110777,-2.91266630074331,
125.775633789045));
#248287=CARTESIAN_POINT('Ctrl Pts',(63.2806278872649,-5.80517758316048,
130.53671958308));
#248288=CARTESIAN_POINT('Ctrl Pts',(63.0021802634519,-3.36301426534433,
135.543754412816));
#248289=CARTESIAN_POINT('Ctrl Pts',(62.723732639639,2.16959486994269,136.195517876976));
#248290=CARTESIAN_POINT('Ctrl Pts',(62.4452850158262,5.70845231035428,131.893071192411));
#248291=CARTESIAN_POINT('Ctrl Pts',(62.1668373920132,4.00152095094907,126.590152676031));
#248292=CARTESIAN_POINT('Ctrl Pts',(61.8883897682004,-1.38261267721222,
125.159885382419));
#248293=CARTESIAN_POINT('Ctrl Pts',(61.6099421443874,-5.49619279939966,
128.916615081961));
#248294=CARTESIAN_POINT('Ctrl Pts',(61.3314945205747,-4.55904024288434,
134.408090707227));
#248295=CARTESIAN_POINT('Ctrl Pts',(61.0530468967616,0.567647575344072,
136.587914432096));
#248296=CARTESIAN_POINT('Ctrl Pts',(60.7745992729488,5.17269500295686,133.452934743723));
#248297=CARTESIAN_POINT('Ctrl Pts',(60.496151649136,5.02428842305186,127.884044823451));
#248298=CARTESIAN_POINT('Ctrl Pts',(60.2177040253229,0.258806232497024,
124.998782452612));
#248299=CARTESIAN_POINT('Ctrl Pts',(59.9392564015102,-4.74450624233532,
127.448562797104));
#248300=CARTESIAN_POINT('Ctrl Pts',(59.6608087776971,-5.38784926247686,
132.982157398764));
#248301=CARTESIAN_POINT('Ctrl Pts',(59.3823611538844,-1.08002202147149,
136.514463149789));
#248302=CARTESIAN_POINT('Ctrl Pts',(59.1039135300714,4.22029269525717,134.799463627718));
#248303=CARTESIAN_POINT('Ctrl Pts',(58.8254659062585,5.64236459780459,129.413159610949));
#248304=CARTESIAN_POINT('Ctrl Pts',(58.5470182824457,1.8793790798041,125.305301355313));
#248305=CARTESIAN_POINT('Ctrl Pts',(58.2685706586328,-3.61066399976409,
126.250809917708));
#248306=CARTESIAN_POINT('Ctrl Pts',(57.9901230348199,-5.78268325429153,
131.380809119953));
#248307=CARTESIAN_POINT('Ctrl Pts',(57.711675411007,-2.64069909790739,135.981080309579));
#248308=CARTESIAN_POINT('Ctrl Pts',(57.4332277871941,2.92795852413098,135.824198999061));
#248309=CARTESIAN_POINT('Ctrl Pts',(57.1547801633813,5.80596530121877,131.054331448687));
#248310=CARTESIAN_POINT('Ctrl Pts',(56.8763325395683,3.34857360366007,126.054752916266));
#248311=CARTESIAN_POINT('Ctrl Pts',(56.5978849157555,-2.18599364874745,
125.419831830104));
#248312=CARTESIAN_POINT('Ctrl Pts',(56.3194372919424,-5.71173952968275,
129.733029650764));
#248313=CARTESIAN_POINT('Ctrl Pts',(56.0409896681298,-3.98867581682796,
135.030728292487));
#248314=CARTESIAN_POINT('Ctrl Pts',(55.7625420443167,1.39978611404518,136.444601510497));
#248315=CARTESIAN_POINT('Ctrl Pts',(55.4840944205039,5.50191298946419,132.675368888989));
#248316=CARTESIAN_POINT('Ctrl Pts',(55.2056467966909,4.54805061095778,127.186771069878));
#248317=CARTESIAN_POINT('Ctrl Pts',(54.9271991728781,-0.585248094394635,
125.022561316018));
#248318=CARTESIAN_POINT('Ctrl Pts',(54.6487515490652,-5.18073239195715,
128.171542663682));
#248319=CARTESIAN_POINT('Ctrl Pts',(54.3703039252523,-5.01537671415865,
133.739955090657));
#248320=CARTESIAN_POINT('Ctrl Pts',(54.0918563014394,-0.241134850822232,
136.610699608625));
#248321=CARTESIAN_POINT('Ctrl Pts',(53.8134086776265,4.75469816032759,134.145702249237));
#248322=CARTESIAN_POINT('Ctrl Pts',(53.5349610538137,5.38119584205463,128.610175163959));
#248323=CARTESIAN_POINT('Ctrl Pts',(53.2565134300007,1.06263743096531,125.090997318624));
#248324=CARTESIAN_POINT('Ctrl Pts',(52.9780658061879,-4.23243286645675,
126.822121231705));
#248325=CARTESIAN_POINT('Ctrl Pts',(52.6996181823749,-5.63810412544538,
132.21272859718));
#248326=CARTESIAN_POINT('Ctrl Pts',(52.4211705585621,-1.86263312984859,
136.309114591992));
#248327=CARTESIAN_POINT('Ctrl Pts',(52.1427229347491,3.62450671739182,135.346900606486));
#248328=CARTESIAN_POINT('Ctrl Pts',(51.8642753109363,5.7809019583462,130.210314286579));
#248329=CARTESIAN_POINT('Ctrl Pts',(51.5858276871234,2.62493071234137,125.619627524071));
#248330=CARTESIAN_POINT('Ctrl Pts',(51.3073800633105,-2.94322362331098,
125.793457186192));
#248331=CARTESIAN_POINT('Ctrl Pts',(51.0289324394976,-5.80669923360788,
130.572062305503));
#248332=CARTESIAN_POINT('Ctrl Pts',(50.7504848156848,-3.33410192124705,
135.564138225197));
#248333=CARTESIAN_POINT('Ctrl Pts',(50.4720371918718,2.20237217680579,136.182211051539));
#248334=CARTESIAN_POINT('Ctrl Pts',(50.193589568059,5.71497383623647,131.858302051661));
#248335=CARTESIAN_POINT('Ctrl Pts',(49.915141944246,3.97579373215887,126.565872361749));
#248336=CARTESIAN_POINT('Ctrl Pts',(49.6366943204332,-1.41694658345112,
125.168406317271));
#248337=CARTESIAN_POINT('Ctrl Pts',(49.3582466966203,-5.50758221055828,
128.950106943089));
#248338=CARTESIAN_POINT('Ctrl Pts',(49.0797990728074,-4.53701884651156,
134.435776110423));
#248339=CARTESIAN_POINT('Ctrl Pts',(48.8013514489945,0.602843191786665,
136.584351844331));
#248340=CARTESIAN_POINT('Ctrl Pts',(48.5229038251815,5.18872178735999,133.421398009111));
#248341=CARTESIAN_POINT('Ctrl Pts',(48.2444562013688,5.006418543501,127.853514660444));
#248342=CARTESIAN_POINT('Ctrl Pts',(47.9660085775558,0.223461235307256,
124.997314589534));
#248343=CARTESIAN_POINT('Ctrl Pts',(47.6875609537429,-4.7648460314457,127.477506128414));
#248344=CARTESIAN_POINT('Ctrl Pts',(47.40911332993,-5.37449257096935,133.014914416948));
#248345=CARTESIAN_POINT('Ctrl Pts',(47.1306657061172,-1.04524299633083,
136.520931755405));
#248346=CARTESIAN_POINT('Ctrl Pts',(46.8522180823042,4.24453382897653,134.773699488214));
#248347=CARTESIAN_POINT('Ctrl Pts',(46.5737704584914,5.6337914224598,129.378838711881));
#248348=CARTESIAN_POINT('Ctrl Pts',(46.2953228346785,1.84586992471411,125.293962926255));
#248349=CARTESIAN_POINT('Ctrl Pts',(46.0168752108656,-3.63831585808481,
126.272873421051));
#248350=CARTESIAN_POINT('Ctrl Pts',(45.7384275870526,-5.77906710891461,
131.415999273987));
#248351=CARTESIAN_POINT('Ctrl Pts',(45.4599799632399,-2.60913800977569,
135.997059081882));
#248352=CARTESIAN_POINT('Ctrl Pts',(45.1815323394269,2.95846145686929,135.806282678493));
#248353=CARTESIAN_POINT('Ctrl Pts',(44.903084715614,5.80737937352832,131.018984258588));
#248354=CARTESIAN_POINT('Ctrl Pts',(44.6246370918012,3.31959935216964,126.034457197533));
#248355=CARTESIAN_POINT('Ctrl Pts',(44.3461894679882,-2.21873030238901,
125.43323835675));
#248356=CARTESIAN_POINT('Ctrl Pts',(44.0677418441753,-5.7181552000533,129.767818479747));
#248357=CARTESIAN_POINT('Ctrl Pts',(43.7892942203624,-3.96287481627985,
135.054930189501));
#248358=CARTESIAN_POINT('Ctrl Pts',(43.5108465965496,1.43409392645716,136.435976114513));
#248359=CARTESIAN_POINT('Ctrl Pts',(43.2323989727367,5.51320041016325,132.641842517543));
#248360=CARTESIAN_POINT('Ctrl Pts',(42.9539513489238,4.52594505174265,127.159152820475));
#248361=CARTESIAN_POINT('Ctrl Pts',(42.6755037251109,-0.620432704521861,
125.026231010632));
#248362=CARTESIAN_POINT('Ctrl Pts',(42.397056101298,-5.19666311515333,128.203128032237));
#248363=CARTESIAN_POINT('Ctrl Pts',(42.1186084774851,-4.99741399406557,
133.770430722483));
#248364=CARTESIAN_POINT('Ctrl Pts',(41.8401608536722,-0.205785549677785,
136.612059886891));
#248365=CARTESIAN_POINT('Ctrl Pts',(41.5617132298594,4.77494976168102,134.11669714467));
#248366=CARTESIAN_POINT('Ctrl Pts',(41.2832656060464,5.36773951131901,128.577458950676));
#248367=CARTESIAN_POINT('Ctrl Pts',(41.0048179822336,1.02783887870806,125.084634598359));
#248368=CARTESIAN_POINT('Ctrl Pts',(40.7263703584206,-4.25659547071474,
126.847959033542));
#248369=CARTESIAN_POINT('Ctrl Pts',(40.4479227346078,-5.62942652880005,
132.24702324348));
#248370=CARTESIAN_POINT('Ctrl Pts',(40.1694751107948,-1.82908961969292,
136.320350978189));
#248371=CARTESIAN_POINT('Ctrl Pts',(39.891027486982,3.65209129391637,135.324753042595));
#248372=CARTESIAN_POINT('Ctrl Pts',(39.6125798631691,5.77717872299504,130.175135301845));
#248373=CARTESIAN_POINT('Ctrl Pts',(39.3341322393562,2.59332113651206,125.603744886877));
#248374=CARTESIAN_POINT('Ctrl Pts',(39.0556846155433,-2.97367188364494,
125.811466264208));
#248375=CARTESIAN_POINT('Ctrl Pts',(38.7772369917304,-5.80800571467979,
130.607413635826));
#248376=CARTESIAN_POINT('Ctrl Pts',(38.4987893679175,-3.30506603077697,
135.584345662267));
#248377=CARTESIAN_POINT('Ctrl Pts',(38.2203417441046,2.23506787395795,136.16870494788));
#248378=CARTESIAN_POINT('Ctrl Pts',(37.9418941202917,5.72128359166147,131.823493856722));
#248379=CARTESIAN_POINT('Ctrl Pts',(37.6634464964789,3.94991918886983,126.541749106207));
#248380=CARTESIAN_POINT('Ctrl Pts',(37.3849988726659,-1.45122798421329,
125.177136094481));
#248381=CARTESIAN_POINT('Ctrl Pts',(37.1065512488531,-5.51876753623267,
128.983667514269));
#248382=CARTESIAN_POINT('Ctrl Pts',(36.8281036250402,-4.51482932923697,
134.463326950183));
#248383=CARTESIAN_POINT('Ctrl Pts',(36.5496560012273,0.6380164696531,136.580575076865));
#248384=CARTESIAN_POINT('Ctrl Pts',(36.2712083774144,5.20455630176915,133.389764299214));
#248385=CARTESIAN_POINT('Ctrl Pts',(35.9927607536015,4.9883631492699,127.82309384212));
#248386=CARTESIAN_POINT('Ctrl Pts',(35.7143131297886,0.188107957679239,
124.996061908681));
#248387=CARTESIAN_POINT('Ctrl Pts',(35.4358655059757,-4.78500925743413,
127.50657273754));
#248388=CARTESIAN_POINT('Ctrl Pts',(35.1574178821628,-5.36093672566315,
133.047589522248));
#248389=CARTESIAN_POINT('Ctrl Pts',(34.87897025835,-1.01042523932657,136.527188531377));
#248390=CARTESIAN_POINT('Ctrl Pts',(34.6005226345371,4.26861767993396,134.747788263399));
#248391=CARTESIAN_POINT('Ctrl Pts',(34.3220750107242,5.62500948490202,129.34457063605));
#248392=CARTESIAN_POINT('Ctrl Pts',(34.0436273869112,1.81229237023524,125.282828687009));
#248393=CARTESIAN_POINT('Ctrl Pts',(33.7651797630984,-3.66583289727342,
126.295104840318));
#248394=CARTESIAN_POINT('Ctrl Pts',(33.4867321392855,-5.77523681808073,
131.451166763527));
#248395=CARTESIAN_POINT('Ctrl Pts',(33.2082845154725,-2.57748023907555,
136.012845436834));
#248396=CARTESIAN_POINT('Ctrl Pts',(32.9298368916598,2.98885476273036,135.788181009863));
#248397=CARTESIAN_POINT('Ctrl Pts',(32.6513892678468,5.80857825125962,130.983629115531));
#248398=CARTESIAN_POINT('Ctrl Pts',(32.3729416440339,3.29050209170421,126.014338229324));
#248399=CARTESIAN_POINT('Ctrl Pts',(32.094494020221,-2.25138474016344,125.446843912307));
#248400=CARTESIAN_POINT('Ctrl Pts',(31.8160463964081,-5.72435898208005,
129.802645718181));
#248401=CARTESIAN_POINT('Ctrl Pts',(31.5375987725953,-3.93692696994811,
135.078974580096));
#248402=CARTESIAN_POINT('Ctrl Pts',(31.2591511487823,1.46834859799131,136.427142036947));
#248403=CARTESIAN_POINT('Ctrl Pts',(30.9807035249695,5.52428353719365,132.608248057529));
#248404=CARTESIAN_POINT('Ctrl Pts',(30.7022559011566,4.50367178196922,127.131669645585));
#248405=CARTESIAN_POINT('Ctrl Pts',(30.4238082773436,-0.655594324287056,
125.030114815962));
#248406=CARTESIAN_POINT('Ctrl Pts',(30.1453606535308,-5.21240127408669,
128.234809790423));
#248407=CARTESIAN_POINT('Ctrl Pts',(29.8669130297179,-4.97926609295916,
133.80079644549));
#248408=CARTESIAN_POINT('Ctrl Pts',(29.588465405905,-0.170428623074124,
136.613204958723));
#248409=CARTESIAN_POINT('Ctrl Pts',(29.3100177820921,4.79502442551506,134.087569300254));
#248410=CARTESIAN_POINT('Ctrl Pts',(29.0315701582792,5.35408427702179,128.544825256054));
#248411=CARTESIAN_POINT('Ctrl Pts',(28.7531225344664,0.99300223950345,125.078483824645));
#248412=CARTESIAN_POINT('Ctrl Pts',(28.4746749106534,-4.28060034526213,
126.873943441297));
#248413=CARTESIAN_POINT('Ctrl Pts',(28.1962272868406,-5.6205403316845,132.281264431386));
#248414=CARTESIAN_POINT('Ctrl Pts',(27.9177796630277,-1.79547833194873,
136.331382967337));
#248415=CARTESIAN_POINT('Ctrl Pts',(27.6393320392148,3.67954054085496,135.3024379739));
#248416=CARTESIAN_POINT('Ctrl Pts',(27.3608844154018,5.77324141216173,130.139979633288));
#248417=CARTESIAN_POINT('Ctrl Pts',(27.082436791589,2.56161546421434,125.58805496041));
#248418=CARTESIAN_POINT('Ctrl Pts',(26.8039891677761,-3.00400995347367,
125.82966035576));
#248419=CARTESIAN_POINT('Ctrl Pts',(26.5255415439632,-5.80909697796402,
130.642772264091));
#248420=CARTESIAN_POINT('Ctrl Pts',(26.2470939201503,-3.27590766986969,
135.604375975235));
#248421=CARTESIAN_POINT('Ctrl Pts',(25.9686462963375,2.2676807498481,136.155000066467));
#248422=CARTESIAN_POINT('Ctrl Pts',(25.6901986725246,5.727381342819,131.788647897428));
#248423=CARTESIAN_POINT('Ctrl Pts',(25.4117510487116,3.92389827987267,126.517783803302));
#248424=CARTESIAN_POINT('Ctrl Pts',(25.1333034248988,-1.48545560918882,
125.186074390566));
#248425=CARTESIAN_POINT('Ctrl Pts',(24.8548558010858,-5.5297483619465,129.017295551901));
#248426=CARTESIAN_POINT('Ctrl Pts',(24.576408177273,-4.49247251330123,134.490742205601));
#248427=CARTESIAN_POINT('Ctrl Pts',(24.2979605534601,0.673166105584617,
136.576584269648));
#248428=CARTESIAN_POINT('Ctrl Pts',(24.0195129296472,5.22019795943058,133.358034786234));
#248429=CARTESIAN_POINT('Ctrl Pts',(23.7410653058343,4.97012290940784,127.792783495733));
#248430=CARTESIAN_POINT('Ctrl Pts',(23.4626176820214,0.152747709641667,
124.995024456474));
#248431=CARTESIAN_POINT('Ctrl Pts',(23.1841700582085,-4.80499517314482,
127.53576154741));
#248432=CARTESIAN_POINT('Ctrl Pts',(22.9057224343956,-5.34718222887511,
133.080181503877));
#248433=CARTESIAN_POINT('Ctrl Pts',(22.6272748105827,-0.975570040643468,
136.533233245855));
#248434=CARTESIAN_POINT('Ctrl Pts',(22.3488271867698,4.29254335569345,134.721730913422));
#248435=CARTESIAN_POINT('Ctrl Pts',(22.070379562957,5.61601911054919,129.310356653276));
#248436=CARTESIAN_POINT('Ctrl Pts',(21.791931939144,1.77864766059611,125.27189905016));
#248437=CARTESIAN_POINT('Ctrl Pts',(21.5134843153312,-3.69321409767591,
126.317503351717));
#248438=CARTESIAN_POINT('Ctrl Pts',(21.2350366915183,-5.77119252372273,
131.486310285425));
#248439=CARTESIAN_POINT('Ctrl Pts',(20.9565890677054,-2.54572695889727,
136.028438789465));
#248440=CARTESIAN_POINT('Ctrl Pts',(20.6781414438925,3.01913731547902,135.769894663934));
#248441=CARTESIAN_POINT('Ctrl Pts',(20.3996938200796,5.80956188998761,130.948267329615));
#248442=CARTESIAN_POINT('Ctrl Pts',(20.1212461962667,3.26128290047392,125.994396757156));
#248443=CARTESIAN_POINT('Ctrl Pts',(19.8427985724538,-2.28395575204823,
125.460647992615));
#248444=CARTESIAN_POINT('Ctrl Pts',(19.5643509486409,-5.7303506458796,129.837510075529));
#248445=CARTESIAN_POINT('Ctrl Pts',(19.285903324828,-3.91083323933969,135.102860573299));
#248446=CARTESIAN_POINT('Ctrl Pts',(19.0074557010152,1.50254885932817,136.418099605148));
#248447=CARTESIAN_POINT('Ctrl Pts',(18.7290080772022,5.53516195986603,132.574586753804));
#248448=CARTESIAN_POINT('Ctrl Pts',(18.4505604533894,4.48123162698169,127.104322563612));
#248449=CARTESIAN_POINT('Ctrl Pts',(18.1721128295765,-0.690731650763477,
125.034212588094));
#248450=CARTESIAN_POINT('Ctrl Pts',(17.8936652057636,-5.22794628557398,
128.26658676426));
#248451=CARTESIAN_POINT('Ctrl Pts',(17.6152175819507,-4.96093368331654,
133.831051134467));
#248452=CARTESIAN_POINT('Ctrl Pts',(17.3367699581378,-0.135065381175154,
136.614134781694));
#248453=CARTESIAN_POINT('Ctrl Pts',(17.0583223343249,4.81492140795562,134.058319795333));
#248454=CARTESIAN_POINT('Ctrl Pts',(16.779874710512,5.34023064516271,128.512275289347));
#248455=CARTESIAN_POINT('Ctrl Pts',(16.5014270866992,0.958128804235671,
125.0725452254));
#248456=CARTESIAN_POINT('Ctrl Pts',(16.2229794628862,-4.30444660058956,
126.900073492105));
#248457=CARTESIAN_POINT('Ctrl Pts',(15.9445318390734,-5.61144586338,132.315450892077));
#248458=CARTESIAN_POINT('Ctrl Pts',(15.6660842152604,-1.76180051209467,
136.342210150638));
#248459=CARTESIAN_POINT('Ctrl Pts',(15.3876365914476,3.70685344106567,135.279956227294));
#248460=CARTESIAN_POINT('Ctrl Pts',(15.1091889676347,5.76909017174479,130.104848583611));
#248461=CARTESIAN_POINT('Ctrl Pts',(14.8307413438218,2.52981487031356,125.572558326068));
#248462=CARTESIAN_POINT('Ctrl Pts',(14.5522937200089,-3.03423670860886,
125.848038786661));
#248463=CARTESIAN_POINT('Ctrl Pts',(14.273846096196,-5.80997298302346,130.678136880072));
#248464=CARTESIAN_POINT('Ctrl Pts',(13.9953984723831,-3.24662791899898,
135.624228421867));
#248465=CARTESIAN_POINT('Ctrl Pts',(13.7169508485702,2.30020959599411,136.141096915141));
#248466=CARTESIAN_POINT('Ctrl Pts',(13.4385032247574,5.73326686375462,131.753765465006));
#248467=CARTESIAN_POINT('Ctrl Pts',(13.1600556009444,3.89773196938174,126.493977341077));
#248468=CARTESIAN_POINT('Ctrl Pts',(12.8816079771316,-1.51962819006047,
125.195220874312));
#248469=CARTESIAN_POINT('Ctrl Pts',(12.6031603533186,-5.54052428080121,
129.050989809886));
#248470=CARTESIAN_POINT('Ctrl Pts',(12.3247127295058,-4.46994922714442,
134.518020860792));
#248471=CARTESIAN_POINT('Ctrl Pts',(12.0462651056929,0.708290797098533,
136.572379570561));
#248472=CARTESIAN_POINT('Ctrl Pts',(11.76781748188,5.23564618073708,133.326210645918));
#248473=CARTESIAN_POINT('Ctrl Pts',(11.4893698580671,4.95169849981347,127.762584744442));
#248474=CARTESIAN_POINT('Ctrl Pts',(11.2109222342542,0.117381801481337,
124.994202271355));
#248475=CARTESIAN_POINT('Ctrl Pts',(10.9324746104413,-4.82480303799234,
127.565071476419));
#248476=CARTESIAN_POINT('Ctrl Pts',(10.6540269866284,-5.33322959028317,
133.112689154126));
#248477=CARTESIAN_POINT('Ctrl Pts',(10.3755793628155,-0.940678691853753,
136.539065674851));
#248478=CARTESIAN_POINT('Ctrl Pts',(10.0971317390026,4.31630996968034,134.695528403849));
#248479=CARTESIAN_POINT('Ctrl Pts',(9.81868411518972,5.60682063254294,129.276198031366));
#248480=CARTESIAN_POINT('Ctrl Pts',(9.54023649137686,1.74493704251384,125.261174420708));
#248481=CARTESIAN_POINT('Ctrl Pts',(9.26178886756394,-3.72045844467185,
126.340068125262));
#248482=CARTESIAN_POINT('Ctrl Pts',(8.98334124375105,-5.76693437570339,
131.52142853743));
#248483=CARTESIAN_POINT('Ctrl Pts',(8.70489361993813,-2.51387934587036,
136.043838561958));
#248484=CARTESIAN_POINT('Ctrl Pts',(8.42644599612531,3.0493079929842,135.751424318317));
#248485=CARTESIAN_POINT('Ctrl Pts',(8.14799837231237,5.81033025326331,130.912900211183));
#248486=CARTESIAN_POINT('Ctrl Pts',(7.86955074849947,3.23194286120641,125.974633519968));
#248487=CARTESIAN_POINT('Ctrl Pts',(7.59110312468663,-2.3164421311127,125.47465008616));
#248488=CARTESIAN_POINT('Ctrl Pts',(7.31265550087371,-5.73612996942864,
129.872410259879));
#248489=CARTESIAN_POINT('Ctrl Pts',(7.0342078770608,-3.88459459136738,135.126587284006));
#248490=CARTESIAN_POINT('Ctrl Pts',(6.75576025324794,1.53669344316449,136.408849154185));
#248491=CARTESIAN_POINT('Ctrl Pts',(6.47731262943506,5.54583527507644,132.540859853697));
#248492=CARTESIAN_POINT('Ctrl Pts',(6.19886500562214,4.45862541830825,127.077112587908));
#248493=CARTESIAN_POINT('Ctrl Pts',(5.92041738180924,-0.725843381924555,
125.038524175185));
#248494=CARTESIAN_POINT('Ctrl Pts',(5.64196975799638,-5.24329757358911,
128.29845777624));
#248495=CARTESIAN_POINT('Ctrl Pts',(5.36352213418349,-4.94241744445191,
133.861193668313));
#248496=CARTESIAN_POINT('Ctrl Pts',(5.08507451037056,-0.0996971343788212,
136.614849321347));
#248497=CARTESIAN_POINT('Ctrl Pts',(4.80662688655771,4.83463997171276,134.028949713759));
#248498=CARTESIAN_POINT('Ctrl Pts',(4.5281792627448,5.32617912909322,128.479810256704));
#248499=CARTESIAN_POINT('Ctrl Pts',(4.24973163893191,0.923219865152705,
125.066819020683));
#248500=CARTESIAN_POINT('Ctrl Pts',(3.97128401511898,-4.32813335306523,
126.926348217707));
#248501=CARTESIAN_POINT('Ctrl Pts',(3.69283639130614,-5.60214346088543,
132.349581358763));
#248502=CARTESIAN_POINT('Ctrl Pts',(3.41438876749324,-1.72805740807474,
136.352832126888));
#248503=CARTESIAN_POINT('Ctrl Pts',(3.13594114368033,3.73402898245891,135.257308635848));
#248504=CARTESIAN_POINT('Ctrl Pts',(2.85749351986744,5.76472515556999,130.06974345461));
#248505=CARTESIAN_POINT('Ctrl Pts',(2.5790458960546,2.49792053319242,125.557255558086));
#248506=CARTESIAN_POINT('Ctrl Pts',(2.30059827224166,-3.06435102898697,
125.866600875889));
#248507=CARTESIAN_POINT('Ctrl Pts',(2.02215064842876,-5.81063369739741,
130.713506173321));
#248508=CARTESIAN_POINT('Ctrl Pts',(1.74370302461591,-3.21722786313679,
135.643902266527));
#248509=CARTESIAN_POINT('Ctrl Pts',(1.46525540080302,2.33265320702766,136.12699600909));
#248510=CARTESIAN_POINT('Ctrl Pts',(1.18680777699008,5.73893993637821,131.718847852038));
#248511=CARTESIAN_POINT('Ctrl Pts',(0.908360153177235,3.87142122699929,
126.47033060169));
#248512=CARTESIAN_POINT('Ctrl Pts',(0.629912529364331,-1.55374446055069,
125.204575206795));
#248513=CARTESIAN_POINT('Ctrl Pts',(0.351464905551429,-5.55109489349118,
129.084749039672));
#248514=CARTESIAN_POINT('Ctrl Pts',(0.0730172817385382,-4.44726030537518,
134.545161904937));
#248515=CARTESIAN_POINT('Ctrl Pts',(-0.205430342074321,0.743389242636492,
136.56796113541));
#248516=CARTESIAN_POINT('Ctrl Pts',(-0.48387796588724,5.25090039324876,
133.294293057522));
#248517=CARTESIAN_POINT('Ctrl Pts',(-0.762325589700153,4.93309060321035,
127.732498707276));
#248518=CARTESIAN_POINT('Ctrl Pts',(-1.040773213513,0.0820115436953976,
124.993595383789));
#248519=CARTESIAN_POINT('Ctrl Pts',(-1.3192208373259,-4.84443211798899,
127.594501438479));
#248520=CARTESIAN_POINT('Ctrl Pts',(-1.5976684611388,-5.31907932690746,
133.145111268411));
#248521=CARTESIAN_POINT('Ctrl Pts',(-1.8761160849517,-0.905752485869179,
136.544685602242));
#248522=CARTESIAN_POINT('Ctrl Pts',(-2.15456370876455,4.33991664121397,
134.669181705622));
#248523=CARTESIAN_POINT('Ctrl Pts',(-2.43301133257747,5.59741439173625,
129.242096036083));
#248524=CARTESIAN_POINT('Ctrl Pts',(-2.71145895639038,1.71116176514775,
125.250655196059));
#248525=CARTESIAN_POINT('Ctrl Pts',(-2.98990658020324,-3.74756492871192,
126.362798324807));
#248526=CARTESIAN_POINT('Ctrl Pts',(-3.26835420401613,-5.76246253181,131.556520218218));
#248527=CARTESIAN_POINT('Ctrl Pts',(-3.54680182782904,-2.48193858011979,
136.059044183669));
#248528=CARTESIAN_POINT('Ctrl Pts',(-3.82524945164193,3.0793656772603,135.732770657435));
#248529=CARTESIAN_POINT('Ctrl Pts',(-4.1036970754548,5.81088331261472,130.877529070775));
#248530=CARTESIAN_POINT('Ctrl Pts',(-4.38214469926771,3.20248306110764,
125.955049250094));
#248531=CARTESIAN_POINT('Ctrl Pts',(-4.66059232308062,-2.34884267356213,
125.488849674089));
#248532=CARTESIAN_POINT('Ctrl Pts',(-4.93903994689347,-5.7416967385722,
129.907344977992));
#248533=CARTESIAN_POINT('Ctrl Pts',(-5.21748757070636,-3.85821199831392,
135.150153833014));
#248534=CARTESIAN_POINT('Ctrl Pts',(-5.49593519451928,1.57078108426016,
136.399391026839));
#248535=CARTESIAN_POINT('Ctrl Pts',(-5.77438281833216,5.55630308732125,
132.507068606974));
#248536=CARTESIAN_POINT('Ctrl Pts',(-6.05283044214503,4.43585399363028,
127.050040726751));
#248537=CARTESIAN_POINT('Ctrl Pts',(-6.33127806595794,-0.76092821669219,
125.043049417465));
#248538=CARTESIAN_POINT('Ctrl Pts',(-6.60972568977086,-5.25845456928442,
128.330421645371));
#248539=CARTESIAN_POINT('Ctrl Pts',(-6.88817331358369,-4.92371806249131,
133.891222930087));
#248540=CARTESIAN_POINT('Ctrl Pts',(-7.16662093739661,-0.0643251932685087,
136.615348551203));
#248541=CARTESIAN_POINT('Ctrl Pts',(-7.44506856120951,4.8541793861078,133.999460143849));
#248542=CARTESIAN_POINT('Ctrl Pts',(-7.72351618502242,5.3119302494974,128.44743136113));
#248543=CARTESIAN_POINT('Ctrl Pts',(-8.00196380883526,0.888276715818123,
125.06130542268));
#248544=CARTESIAN_POINT('Ctrl Pts',(-8.28041143264819,-4.35165972496785,
126.952766644486));
#248545=CARTESIAN_POINT('Ctrl Pts',(-8.55885905646108,-5.59263346890473,
132.383654566726));
#248546=CARTESIAN_POINT('Ctrl Pts',(-8.83730668027396,-1.69425027025207,
136.363248502487));
#248547=CARTESIAN_POINT('Ctrl Pts',(-9.11575430408684,3.76106615803527,
135.234496038775));
#248548=CARTESIAN_POINT('Ctrl Pts',(-9.39420192789976,5.7601465253845,130.034665547118));
#248549=CARTESIAN_POINT('Ctrl Pts',(-9.67264955171265,2.4659336347071,125.542147223509));
#248550=CARTESIAN_POINT('Ctrl Pts',(-9.95109717552551,-3.09435179871079,
125.885345935621));
#248551=CARTESIAN_POINT('Ctrl Pts',(-10.2295447993384,-5.81107909660284,
130.748878833214));
#248552=CARTESIAN_POINT('Ctrl Pts',(-10.5079924231513,-3.18770859171301,
135.663396780189));
#248553=CARTESIAN_POINT('Ctrl Pts',(-10.7864400469642,2.36501038073878,
136.112697870828));
#248554=CARTESIAN_POINT('Ctrl Pts',(-11.0648876707771,5.74440035047196,
131.683896352409));
#248555=CARTESIAN_POINT('Ctrl Pts',(-11.34333529459,3.84496702767957,126.446844461378));
#248556=CARTESIAN_POINT('Ctrl Pts',(-11.6217829184029,-1.58780315646856,
125.214137041385));
#248557=CARTESIAN_POINT('Ctrl Pts',(-11.9002305422157,-5.56145980831845,
129.118571990297));
#248558=CARTESIAN_POINT('Ctrl Pts',(-12.1786781660286,-4.42440658873985,
134.572164332316));
#248559=CARTESIAN_POINT('Ctrl Pts',(-12.4571257898416,0.778460141612691,
136.563329127923));
#248560=CARTESIAN_POINT('Ctrl Pts',(-12.7355734136544,5.26596003171537,
133.262283203764));
#248561=CARTESIAN_POINT('Ctrl Pts',(-13.0140210374673,4.91429990912079,
127.702526499083));
#248562=CARTESIAN_POINT('Ctrl Pts',(-13.2924686612802,0.0466382469415425,
124.993203816266));
#248563=CARTESIAN_POINT('Ctrl Pts',(-13.5709162850931,-4.86388168577195,
127.624050343051));
#248564=CARTESIAN_POINT('Ctrl Pts',(-13.849363908906,-5.30473196309121,
133.177446645321));
#248565=CARTESIAN_POINT('Ctrl Pts',(-14.1278115327188,-0.87079271689315,
136.550092819781));
#248566=CARTESIAN_POINT('Ctrl Pts',(-14.4062591565318,4.36336249554048,
134.642691795028));
#248567=CARTESIAN_POINT('Ctrl Pts',(-14.6847067803446,5.58780073668082,
129.20805193109));
#248568=CARTESIAN_POINT('Ctrl Pts',(-14.9631544041576,1.67732308005318,
125.240341766008));
#248569=CARTESIAN_POINT('Ctrl Pts',(-15.2416020279704,-3.77453254535539,
126.385693108075));
#248570=CARTESIAN_POINT('Ctrl Pts',(-15.5200496517834,-5.75777715774833,
131.591584027456));
#248571=CARTESIAN_POINT('Ctrl Pts',(-15.7984972755962,-2.44990584522241,
136.074055091149));
#248572=CARTESIAN_POINT('Ctrl Pts',(-16.0769448994091,3.1093092545088,135.713934372506));
#248573=CARTESIAN_POINT('Ctrl Pts',(-16.355392523222,5.81122104754806,130.842155219084));
#248574=CARTESIAN_POINT('Ctrl Pts',(-16.6338401470349,3.17290459182133,
125.935644673236));
#248575=CARTESIAN_POINT('Ctrl Pts',(-16.9122877708478,-2.38115617878252,
125.50324623023));
#248576=CARTESIAN_POINT('Ctrl Pts',(-17.1907353946607,-5.74705074703162,
129.94231293535));
#248577=CARTESIAN_POINT('Ctrl Pts',(-17.4691830184736,-3.83168643779603,
135.173559347056));
#248578=CARTESIAN_POINT('Ctrl Pts',(-17.7476306422864,1.6048105194851,136.389725573584));
#248579=CARTESIAN_POINT('Ctrl Pts',(-18.0260782660994,5.56656500871184,
132.473214265779));
#248580=CARTESIAN_POINT('Ctrl Pts',(-18.3045258899123,4.4129181967513,127.023107983299));
#248581=CARTESIAN_POINT('Ctrl Pts',(-18.5829735137251,-0.795984854984928,
125.047788147249));
#248582=CARTESIAN_POINT('Ctrl Pts',(-18.861421137538,-5.27341671101187,
128.362477187221));
#248583=CARTESIAN_POINT('Ctrl Pts',(-19.1398687613509,-4.90483623034722,
133.921137807042));
#248584=CARTESIAN_POINT('Ctrl Pts',(-19.4183163851638,-0.0289508685644962,
136.615632452765));
#248585=CARTESIAN_POINT('Ctrl Pts',(-19.6967640089767,4.87353892710056,
133.969852178351));
#248586=CARTESIAN_POINT('Ctrl Pts',(-19.9752116327896,5.29748453437273,
128.415139802436));
#248587=CARTESIAN_POINT('Ctrl Pts',(-20.2536592566025,0.853300651063172,
125.056004635698));
#248588=CARTESIAN_POINT('Ctrl Pts',(-20.5321068804154,-4.37502484451904,
126.979327793496));
#248589=CARTESIAN_POINT('Ctrl Pts',(-20.8105545042282,-5.58291623983416,
132.417669253371));
#248590=CARTESIAN_POINT('Ctrl Pts',(-21.0890021280412,-1.66038035136256,
136.37345889145));
#248591=CARTESIAN_POINT('Ctrl Pts',(-21.367449751854,3.78796396592178,135.211519281404));
#248592=CARTESIAN_POINT('Ctrl Pts',(-21.6458973756669,5.75535445085128,
129.999616160961));
#248593=CARTESIAN_POINT('Ctrl Pts',(-21.9243449994798,2.43385536014432,
125.527233882186));
#248594=CARTESIAN_POINT('Ctrl Pts',(-22.2027926232928,-3.12423790609075,
125.904273271251));
#248595=CARTESIAN_POINT('Ctrl Pts',(-22.4812402471056,-5.81130916413533,
130.784253549004));
#248596=CARTESIAN_POINT('Ctrl Pts',(-22.7596878709185,-3.15807119857507,
135.682711240481));
#248597=CARTESIAN_POINT('Ctrl Pts',(-23.0381354947314,2.39727991812053,
136.098203030175));
#248598=CARTESIAN_POINT('Ctrl Pts',(-23.3165831185443,5.74964790369824,
131.648912261261));
#248599=CARTESIAN_POINT('Ctrl Pts',(-23.5950307423572,3.81837035169266,
126.423519790431));
#248600=CARTESIAN_POINT('Ctrl Pts',(-23.8734783661701,-1.62180301575654,
125.223906023766));
#248601=CARTESIAN_POINT('Ctrl Pts',(-24.151925989983,-5.57161864120731,
129.15245740844));
#248602=CARTESIAN_POINT('Ctrl Pts',(-24.4303736137958,-4.4013889240913,
134.599027142342));
#248603=CARTESIAN_POINT('Ctrl Pts',(-24.7088212376087,0.813502194462058,
136.558483719739));
#248604=CARTESIAN_POINT('Ctrl Pts',(-24.9872688614217,5.28082453809644,
133.230182270781));
#248605=CARTESIAN_POINT('Ctrl Pts',(-25.2657164852345,4.89532711384086,
127.672669230493));
#248606=CARTESIAN_POINT('Ctrl Pts',(-25.5441641090475,0.0112632219902977,
124.993027583295));
#248607=CARTESIAN_POINT('Ctrl Pts',(-25.8226117328602,-4.88315102063038,
127.65371709519));
#248608=CARTESIAN_POINT('Ctrl Pts',(-26.1010593566733,-5.29018803048126,
133.209694086655));
#248609=CARTESIAN_POINT('Ctrl Pts',(-26.3795069804861,-0.835800680372761,
136.555287127099));
#248610=CARTESIAN_POINT('Ctrl Pts',(-26.6579546042989,4.38664666386508,
134.616059653661));
#248611=CARTESIAN_POINT('Ctrl Pts',(-26.9364022281119,5.57798002361419,
129.174066977901));
#248612=CARTESIAN_POINT('Ctrl Pts',(-27.2148498519247,1.64342224113504,
125.23023451272));
#248613=CARTESIAN_POINT('Ctrl Pts',(-27.4932974757377,-3.80136029530733,
126.408751626694));
#248614=CARTESIAN_POINT('Ctrl Pts',(-27.7717450995505,-5.75287842713667,
131.626618665841));
#248615=CARTESIAN_POINT('Ctrl Pts',(-28.0501927233634,-2.41778232816299,
136.088870728161));
#248616=CARTESIAN_POINT('Ctrl Pts',(-28.3286403471763,3.13913761515943,
135.694916161515));
#248617=CARTESIAN_POINT('Ctrl Pts',(-28.6070879709892,5.8113434455484,130.8067799669));
#248618=CARTESIAN_POINT('Ctrl Pts',(-28.8855355948021,3.14320854938853,
125.916420508438));
#248619=CARTESIAN_POINT('Ctrl Pts',(-29.163983218615,-2.41338144938502,
125.517839221114));
#248620=CARTESIAN_POINT('Ctrl Pts',(-29.4424308424279,-5.75219179641212,
129.977312836202));
#248621=CARTESIAN_POINT('Ctrl Pts',(-29.7208784662408,-3.80501889272807,
135.196802958832));
#248622=CARTESIAN_POINT('Ctrl Pts',(-29.9993260900537,1.6387804878663,136.379853152576));
#248623=CARTESIAN_POINT('Ctrl Pts',(-30.2777737138665,5.576620658989,132.439298084597));
#248624=CARTESIAN_POINT('Ctrl Pts',(-30.5562213376795,4.38981887756547,
126.996315355552));
#248625=CARTESIAN_POINT('Ctrl Pts',(-30.8346689614924,-0.831011997766135,
125.052740188944));
#248626=CARTESIAN_POINT('Ctrl Pts',(-31.1131165853052,-5.2881834443438,
128.394623213959));
#248627=CARTESIAN_POINT('Ctrl Pts',(-31.3915642091181,-4.88577264769286,
133.950937190672));
#248628=CARTESIAN_POINT('Ctrl Pts',(-31.670011832931,0.00642452892459172,
136.615701015511));
#248629=CARTESIAN_POINT('Ctrl Pts',(-31.9484594567439,4.89271787731614,
133.940126914399));
#248630=CARTESIAN_POINT('Ctrl Pts',(-32.2269070805568,5.28284251901049,
128.382936777197));
#248631=CARTESIAN_POINT('Ctrl Pts',(-32.5053547043697,0.818292966938792,
125.050916856162));
#248632=CARTESIAN_POINT('Ctrl Pts',(-32.7838023281826,-4.3982278459157,
127.006030680504));
#248633=CARTESIAN_POINT('Ctrl Pts',(-33.0622499519955,-5.57299213374921,
132.451624158271));
#248634=CARTESIAN_POINT('Ctrl Pts',(-33.3406975758084,-1.62644890646854,
136.383462915428));
#248635=CARTESIAN_POINT('Ctrl Pts',(-33.6191451996212,3.81472140941051,
135.188379215148));
#248636=CARTESIAN_POINT('Ctrl Pts',(-33.8975928234342,5.75034910954236,
129.964596594906));
#248637=CARTESIAN_POINT('Ctrl Pts',(-34.176040447247,2.40168689817613,125.512516086734));
#248638=CARTESIAN_POINT('Ctrl Pts',(-34.4544880710599,-3.15400824368619,
125.923382181419));
#248639=CARTESIAN_POINT('Ctrl Pts',(-34.7329356948729,-5.81132389146964,
130.81962900987));
#248640=CARTESIAN_POINT('Ctrl Pts',(-35.0113833186857,-3.1283167819475,
135.701844931696));
#248641=CARTESIAN_POINT('Ctrl Pts',(-35.2898309424986,2.42946062341331,
136.083512024245));
#248642=CARTESIAN_POINT('Ctrl Pts',(-35.5682785663115,5.75468240160701,
131.613896874941));
#248643=CARTESIAN_POINT('Ctrl Pts',(-35.8467261901244,3.79163218458816,
126.400357453152));
#248644=CARTESIAN_POINT('Ctrl Pts',(-36.1251738139373,-1.65574277853735,
125.233881791944));
#248645=CARTESIAN_POINT('Ctrl Pts',(-36.4036214377501,-5.58157101571846,
129.186404038463));
#248646=CARTESIAN_POINT('Ctrl Pts',(-36.6820690615631,-4.37820816435757,
134.625749339604));
#248647=CARTESIAN_POINT('Ctrl Pts',(-36.960516685376,0.848514102688449,
136.553425090409));
#248648=CARTESIAN_POINT('Ctrl Pts',(-37.2389643091888,5.29549336158222,
133.197991448084));
#248649=CARTESIAN_POINT('Ctrl Pts',(-37.5174119330018,4.87617292041449,
127.64292800788));
#248650=CARTESIAN_POINT('Ctrl Pts',(-37.7958595568146,-0.0241122203237842,
124.993066691407));
#248651=CARTESIAN_POINT('Ctrl Pts',(-38.0743071806275,-4.90223940853195,
127.683500595584));
#248652=CARTESIAN_POINT('Ctrl Pts',(-38.3527548044404,-5.27544806800837,
133.241852397473));
#248653=CARTESIAN_POINT('Ctrl Pts',(-38.6312024282533,-0.800777672950798,
136.560268331721));
#248654=CARTESIAN_POINT('Ctrl Pts',(-38.9096500520661,4.40976828338437,
134.589286268384));
#248655=CARTESIAN_POINT('Ctrl Pts',(-39.1880976758791,5.56795261644649,
129.140142435842));
#248656=CARTESIAN_POINT('Ctrl Pts',(-39.4665452996919,1.6094605046014,125.220333810727));
#248657=CARTESIAN_POINT('Ctrl Pts',(-39.7449929235049,-3.82804718445556,
126.43197302622));
#248658=CARTESIAN_POINT('Ctrl Pts',(-40.0234405473177,-5.74776652149929,
131.661622835152));
#248659=CARTESIAN_POINT('Ctrl Pts',(-40.3018881711306,-2.38556921929025,
136.103490545709));
#248660=CARTESIAN_POINT('Ctrl Pts',(-40.5803357949436,3.16884965391132,
135.675716729192));
#248661=CARTESIAN_POINT('Ctrl Pts',(-40.8587834187564,5.81125050208024,
130.771404625066));
#248662=CARTESIAN_POINT('Ctrl Pts',(-41.1372310425694,3.11339603420704,
125.897377468058));
#248663=CARTESIAN_POINT('Ctrl Pts',(-41.4156786663821,-2.4455172912504,
125.532628105994));
#248664=CARTESIAN_POINT('Ctrl Pts',(-41.6941262901951,-5.75711969621025,
130.012343383614));
#248665=CARTESIAN_POINT('Ctrl Pts',(-41.9725739140079,-3.77821035128576,
135.219883807042));
#248666=CARTESIAN_POINT('Ctrl Pts',(-42.2510215378209,1.67268973063362,
136.369774129642));
#248667=CARTESIAN_POINT('Ctrl Pts',(-42.5294691616338,5.58646966553678,
132.405321320208));
#248668=CARTESIAN_POINT('Ctrl Pts',(-42.8079167854466,4.366556892027,126.969663836325));
#248669=CARTESIAN_POINT('Ctrl Pts',(-43.0863644092596,-0.866008347092154,
125.057905359049));
#248670=CARTESIAN_POINT('Ctrl Pts',(-43.3648120330724,-5.3027542220935,
128.426858534403));
#248671=CARTESIAN_POINT('Ctrl Pts',(-43.6432596568854,-4.86652802093628,
133.98061997675));
#248672=CARTESIAN_POINT('Ctrl Pts',(-43.9217072806982,0.0417996883503892,
136.615554236903));
#248673=CARTESIAN_POINT('Ctrl Pts',(-44.2001549045111,4.9117155260715,133.910285453475));
#248674=CARTESIAN_POINT('Ctrl Pts',(-44.478602528324,5.26800474597596,128.350823478709));
#248675=CARTESIAN_POINT('Ctrl Pts',(-44.7570501521369,0.783254960667603,
125.046042272601));
#248676=CARTESIAN_POINT('Ctrl Pts',(-45.0354977759497,-4.42126786936209,
127.032874316024));
#248677=CARTESIAN_POINT('Ctrl Pts',(-45.3139453997627,-5.56286151839129,
132.485518023215));
#248678=CARTESIAN_POINT('Ctrl Pts',(-45.5923930235756,-1.59245719291215,
136.393260203719));
#248679=CARTESIAN_POINT('Ctrl Pts',(-45.8708406473885,3.84133749699455,
135.165076697471));
#248680=CARTESIAN_POINT('Ctrl Pts',(-46.1492882712014,5.74513068693249,
129.929608146614));
#248681=CARTESIAN_POINT('Ctrl Pts',(-46.4277358950142,2.3694294408167,125.497994382526));
#248682=CARTESIAN_POINT('Ctrl Pts',(-46.7061835188271,-3.18366170834627,
125.942671958037));
#248683=CARTESIAN_POINT('Ctrl Pts',(-46.98463114264,-5.81112327806003,130.85500390496));
#248684=CARTESIAN_POINT('Ctrl Pts',(-47.263078766453,-3.09844644439114,
135.720797144829));
#248685=CARTESIAN_POINT('Ctrl Pts',(-47.5415263902657,2.46155130414924,
136.068625397419));
#248686=CARTESIAN_POINT('Ctrl Pts',(-47.8199740140787,5.75950365764311,
131.578851490957));
#248687=CARTESIAN_POINT('Ctrl Pts',(-48.0984216378915,3.76475351715869,
126.377358307829));
#248688=CARTESIAN_POINT('Ctrl Pts',(-48.3768692617045,-1.6896211871606,
125.244063976264));
#248689=CARTESIAN_POINT('Ctrl Pts',(-48.6553168855173,-5.59131656306301,
129.220410622463));
#248690=CARTESIAN_POINT('Ctrl Pts',(-48.9337645093303,-4.35486516851022,
134.652329933902));
#248691=CARTESIAN_POINT('Ctrl Pts',(-49.2122121331431,0.883494568912716,
136.548153427379));
#248692=CARTESIAN_POINT('Ctrl Pts',(-49.4906597569561,5.3099659586141,133.165711928516));
#248693=CARTESIAN_POINT('Ctrl Pts',(-49.7691073807689,4.85683803860733,
127.613303933314));
#248694=CARTESIAN_POINT('Ctrl Pts',(-50.0475550045819,-0.0594867691506708,
124.993321139153));
#248695=CARTESIAN_POINT('Ctrl Pts',(-50.3260026283946,-4.92114614214944,
127.713399740592));
#248696=CARTESIAN_POINT('Ctrl Pts',(-50.6044502522077,-5.26051262186729,
133.273920386136));
#248697=CARTESIAN_POINT('Ctrl Pts',(-50.8828978760204,-0.765724992417492,
136.565036249065));
#248698=CARTESIAN_POINT('Ctrl Pts',(-51.1613454998334,4.4327264973184,134.562372631296));
#248699=CARTESIAN_POINT('Ctrl Pts',(-51.4397931236463,5.55771888674681,
129.106279562002));
#248700=CARTESIAN_POINT('Ctrl Pts',(-51.7182407474591,1.57543912891688,
125.210640026899));
#248701=CARTESIAN_POINT('Ctrl Pts',(-51.9966883712721,-3.85459222390762,
126.455356446176));
#248702=CARTESIAN_POINT('Ctrl Pts',(-52.2751359950849,-5.7424416302597,
131.696595238295));
#248703=CARTESIAN_POINT('Ctrl Pts',(-52.5535836188979,-2.35326771227282,
136.117914002047));
#248704=CARTESIAN_POINT('Ctrl Pts',(-52.8320312427106,3.19844426977395,
135.656336786975));
#248705=CARTESIAN_POINT('Ctrl Pts',(-53.1104788665238,5.81094222058764,
130.736030504428));
#248706=CARTESIAN_POINT('Ctrl Pts',(-53.3889264903363,3.08346815099054,
125.878516257743));
#248707=CARTESIAN_POINT('Ctrl Pts',(-53.6673741141495,-2.47756251357323,
125.547612336859));
#248708=CARTESIAN_POINT('Ctrl Pts',(-53.9458217379622,-5.76183426382087,
130.047403279515));
#248709=CARTESIAN_POINT('Ctrl Pts',(-54.2242693617753,-3.75126180686946,
135.242801036416));
#248710=CARTESIAN_POINT('Ctrl Pts',(-54.502716985588,1.70653699126786,136.359488878264));
#248711=CARTESIAN_POINT('Ctrl Pts',(-54.7811646094011,5.59611166339667,
132.371285231631));
#248712=CARTESIAN_POINT('Ctrl Pts',(-55.0596122332138,4.3431331021171,126.943154413196));
#248713=CARTESIAN_POINT('Ctrl Pts',(-55.3380598570268,-0.900972606160421,
125.063283466166));
#248714=CARTESIAN_POINT('Ctrl Pts',(-55.6165074808396,-5.31712850433539,
128.459181954061));
#248715=CARTESIAN_POINT('Ctrl Pts',(-55.8949551046525,-4.84710306319425,
134.01018506537));
#248716=CARTESIAN_POINT('Ctrl Pts',(-56.1734027284654,0.0771732988733811,
136.615192122377));
#248717=CARTESIAN_POINT('Ctrl Pts',(-56.4518503522783,4.93053116940174,
133.880328901363));
#248718=CARTESIAN_POINT('Ctrl Pts',(-56.7302979760911,5.25297176508825,
128.318801096944));
#248719=CARTESIAN_POINT('Ctrl Pts',(-57.0087455999042,0.748187930595796,
125.041381065643));
#248720=CARTESIAN_POINT('Ctrl Pts',(-57.2871932237169,-4.44414406110167,
127.059857705357));
#248721=CARTESIAN_POINT('Ctrl Pts',(-57.5656408475299,-5.55252476915405,
132.519349592253));
#248722=CARTESIAN_POINT('Ctrl Pts',(-57.8440884713427,-1.55840647026886,
136.402850393281));
#248723=CARTESIAN_POINT('Ctrl Pts',(-58.1225360951557,3.867811242405,135.141612591857));
#248724=CARTESIAN_POINT('Ctrl Pts',(-58.4009837189685,5.73969937639226,
129.894652112598));
#248725=CARTESIAN_POINT('Ctrl Pts',(-58.6794313427815,2.33708418337799,
125.483669307672));
#248726=CARTESIAN_POINT('Ctrl Pts',(-58.9578789665944,-3.21319720125095,
125.962141886319));
#248727=CARTESIAN_POINT('Ctrl Pts',(-59.2363265904072,-5.81070733134035,
130.890376923444));
#248728=CARTESIAN_POINT('Ctrl Pts',(-59.5147742142201,-3.06846129276222,
135.739567177598));
#248729=CARTESIAN_POINT('Ctrl Pts',(-59.793221838033,2.49355077119662,136.053543701326));
#248730=CARTESIAN_POINT('Ctrl Pts',(-60.071669461846,5.76411149315304,131.543777407928));
#248731=CARTESIAN_POINT('Ctrl Pts',(-60.3501170856587,3.73773534540316,
126.354523206705));
#248732=CARTESIAN_POINT('Ctrl Pts',(-60.6285647094717,-1.72343698624942,
125.254452199421));
#248733=CARTESIAN_POINT('Ctrl Pts',(-60.9070123332846,-5.6008549221161,
129.254475900312));
#248734=CARTESIAN_POINT('Ctrl Pts',(-61.1854599570975,-4.33136080153256,
134.678767940282));
#248735=CARTESIAN_POINT('Ctrl Pts',(-61.4639075809103,0.918442296920838,
136.542668925995));
#248736=CARTESIAN_POINT('Ctrl Pts',(-61.7423552047232,5.32424179290464,
133.133344908207));
#248737=CARTESIAN_POINT('Ctrl Pts',(-62.0208028285362,4.83732318488056,
127.583798104527));
#248738=CARTESIAN_POINT('Ctrl Pts',(-62.299250452349,-0.0948591136734494,
124.993790917104));
#248739=CARTESIAN_POINT('Ctrl Pts',(-62.5776980761619,-4.93987052088691,
127.743413422294));
#248740=CARTESIAN_POINT('Ctrl Pts',(-62.8561456999749,-5.24538224549645,
133.305896864355));
#248741=CARTESIAN_POINT('Ctrl Pts',(-63.1345933237877,-0.730643937663188,
136.569590702456));
#248742=CARTESIAN_POINT('Ctrl Pts',(-63.4130409476006,4.45552045494177,
134.53531973969));
#248743=CARTESIAN_POINT('Ctrl Pts',(-63.6914885714135,5.5472792137301,129.072479611178));
#248744=CARTESIAN_POINT('Ctrl Pts',(-63.9699361952264,1.54135937475606,
125.201153520444));
#248745=CARTESIAN_POINT('Ctrl Pts',(-64.2483838190392,-3.88099443002729,
126.478901020081));
#248746=CARTESIAN_POINT('Ctrl Pts',(-64.5268314428522,-5.73690395073373,
131.731534579357));
#248747=CARTESIAN_POINT('Ctrl Pts',(-64.805279066665,-2.32087900405488,
136.132140562712));
#248748=CARTESIAN_POINT('Ctrl Pts',(-65.083726690478,3.22792036610792,135.636777052998));
#248749=CARTESIAN_POINT('Ctrl Pts',(-65.3621743142908,5.81041861249411,
130.700658915789));
#248750=CARTESIAN_POINT('Ctrl Pts',(-65.6406219381037,3.05342600872776,
125.859837576403));
#248751=CARTESIAN_POINT('Ctrl Pts',(-65.9190695619166,-2.50951592890599,
125.562791358466));
#248752=CARTESIAN_POINT('Ctrl Pts',(-66.1975171857295,-5.76633532454392,
130.082491224748));
#248753=CARTESIAN_POINT('Ctrl Pts',(-66.4759648095424,-3.72417425806736,
135.26555379775));
#248754=CARTESIAN_POINT('Ctrl Pts',(-66.7544124333553,1.74032101554631,
136.348997779564));
#248755=CARTESIAN_POINT('Ctrl Pts',(-67.0328600571681,5.60554629528092,
132.337191080086));
#248756=CARTESIAN_POINT('Ctrl Pts',(-67.3113076809811,4.31954837581292,
126.916788068483));
#248757=CARTESIAN_POINT('Ctrl Pts',(-67.5897553047939,-0.935903479357421,
125.068874311009));
#248758=CARTESIAN_POINT('Ctrl Pts',(-67.8682029286069,-5.33130575842519,
128.491592275178));
#248759=CARTESIAN_POINT('Ctrl Pts',(-68.1466505524197,-4.82749849426569,
134.039631360986));
#248760=CARTESIAN_POINT('Ctrl Pts',(-68.4250981762326,0.112544049711387,
136.614614685353));
#248761=CARTESIAN_POINT('Ctrl Pts',(-68.7035458000455,4.94916411008632,
133.850258368115));
#248762=CARTESIAN_POINT('Ctrl Pts',(-68.9819934238584,5.23774413340002,
128.286870818499));
#248763=CARTESIAN_POINT('Ctrl Pts',(-69.2604410476712,0.713093176145084,
125.036933408012));
#248764=CARTESIAN_POINT('Ctrl Pts',(-69.5388886714842,-4.46685557344872,
127.086979848621));
#248765=CARTESIAN_POINT('Ctrl Pts',(-69.8173362952971,-5.54198226906957,
132.553117611744));
#248766=CARTESIAN_POINT('Ctrl Pts',(-70.09578391911,-1.52429800030071,136.412233128746));
#248767=CARTESIAN_POINT('Ctrl Pts',(-70.3742315429229,3.89414166464747,
135.117987767775));
#248768=CARTESIAN_POINT('Ctrl Pts',(-70.6526791667357,5.73405537918087,
129.859729788164));
#248769=CARTESIAN_POINT('Ctrl Pts',(-70.9311267905487,2.3046523244254,125.469541392991));
#248770=CARTESIAN_POINT('Ctrl Pts',(-71.2095744143614,-3.24261362795168,
125.981791244794));
#248771=CARTESIAN_POINT('Ctrl Pts',(-71.4880220381746,-5.81007606672361,
130.925746754563));
#248772=CARTESIAN_POINT('Ctrl Pts',(-71.7664696619872,-3.03836243817177,
135.758154334473));
#248773=CARTESIAN_POINT('Ctrl Pts',(-72.0449172858002,2.52545783880292,
136.038267494822));
#248774=CARTESIAN_POINT('Ctrl Pts',(-72.3233649096131,5.76850573739207,
131.508675925537));
#248775=CARTESIAN_POINT('Ctrl Pts',(-72.601812533426,3.71057867048956,126.331852995942));
#248776=CARTESIAN_POINT('Ctrl Pts',(-72.8802601572389,-1.75718892274731,
125.265046076474));
#248777=CARTESIAN_POINT('Ctrl Pts',(-73.1587077810518,-5.61018573943046,
129.28859860971));
#248778=CARTESIAN_POINT('Ctrl Pts',(-73.4371554048648,-4.30769593438731,
134.705062379074));
#248779=CARTESIAN_POINT('Ctrl Pts',(-73.7156030286775,0.953355991712339,
136.536971789486));
#248780=CARTESIAN_POINT('Ctrl Pts',(-73.9940506524905,5.33832033545752,
133.100891586529));
#248781=CARTESIAN_POINT('Ctrl Pts',(-74.2724982763033,4.81762908236426,
127.554411614868));
#248782=CARTESIAN_POINT('Ctrl Pts',(-74.5509459001162,-0.130227943157576,
124.994476007852));
#248783=CARTESIAN_POINT('Ctrl Pts',(-74.8293935239292,-4.95841185090586,
127.77354052852));
#248784=CARTESIAN_POINT('Ctrl Pts',(-75.107841147742,-5.23005749955717,
133.337780647228));
#248785=CARTESIAN_POINT('Ctrl Pts',(-75.3862887715549,-0.695535808628632,
136.573931523126));
#248786=CARTESIAN_POINT('Ctrl Pts',(-75.6647363953679,4.4781493116164,134.508128596022));
#248787=CARTESIAN_POINT('Ctrl Pts',(-75.9431840191806,5.53663398424198,
129.038743835842));
#248788=CARTESIAN_POINT('Ctrl Pts',(-76.2216316429937,1.50722250495638,
125.191874642891));
#248789=CARTESIAN_POINT('Ctrl Pts',(-76.5000792668064,-3.90725282447187,
126.502605875483));
#248790=CARTESIAN_POINT('Ctrl Pts',(-76.7785268906195,-5.73115368812196,
131.766439563647));
#248791=CARTESIAN_POINT('Ctrl Pts',(-77.0569745144322,-2.28840429481114,
136.146169700531));
#248792=CARTESIAN_POINT('Ctrl Pts',(-77.3354221382452,3.25727685066645,
135.617038252052));
#248793=CARTESIAN_POINT('Ctrl Pts',(-77.613869762058,5.80967969720196,130.665291169852));
#248794=CARTESIAN_POINT('Ctrl Pts',(-77.8923173858709,3.0232707206408,125.841342116181));
#248795=CARTESIAN_POINT('Ctrl Pts',(-78.1707650096839,-2.54137635320382,
125.57816460835));
#248796=CARTESIAN_POINT('Ctrl Pts',(-78.4492126334967,-5.77062271159095,
130.117605919119));
#248797=CARTESIAN_POINT('Ctrl Pts',(-78.7276602573096,-3.69694870861804,
135.288141247929));
#248798=CARTESIAN_POINT('Ctrl Pts',(-79.0061078811224,1.77404055158998,
136.338301222296));
#248799=CARTESIAN_POINT('Ctrl Pts',(-79.2845555049354,5.61477321158579,
132.303040128944));
#248800=CARTESIAN_POINT('Ctrl Pts',(-79.5630031287483,4.29580358705489,
126.8905657792));
#248801=CARTESIAN_POINT('Ctrl Pts',(-79.8414507525611,-0.970799672307275,
125.074677686406));
#248802=CARTESIAN_POINT('Ctrl Pts',(-80.1198983763742,-5.34528545901998,
128.524088296775));
#248803=CARTESIAN_POINT('Ctrl Pts',(-80.3983460001869,-4.80771504060458,
134.068957772455));
#248804=CARTESIAN_POINT('Ctrl Pts',(-80.6767936239998,0.147910630189091,
136.613821947228));
#248805=CARTESIAN_POINT('Ctrl Pts',(-80.9552412478128,4.96761365767528,
133.820074968005));
#248806=CARTESIAN_POINT('Ctrl Pts',(-81.2336888716256,5.22232241517632,
128.255033826564));
#248807=CARTESIAN_POINT('Ctrl Pts',(-81.5121364954386,0.6779719977639,125.032699464516));
#248808=CARTESIAN_POINT('Ctrl Pts',(-81.7905841192513,-4.48940156482041,
127.114239740797));
#248809=CARTESIAN_POINT('Ctrl Pts',(-82.0690317430644,-5.53123440879372,
132.586820830401));
#248810=CARTESIAN_POINT('Ctrl Pts',(-82.3474793668772,-1.490133046909,136.421408062431));
#248811=CARTESIAN_POINT('Ctrl Pts',(-82.62592699069,3.92032778803891,135.094203100652));
#248812=CARTESIAN_POINT('Ctrl Pts',(-82.9043746145031,5.72819890443852,
129.824842467372));
#248813=CARTESIAN_POINT('Ctrl Pts',(-83.1828222383158,2.27213506573304,
125.455611161998));
#248814=CARTESIAN_POINT('Ctrl Pts',(-83.4612698621288,-3.27190989841242,
126.001619305352));
#248815=CARTESIAN_POINT('Ctrl Pts',(-83.7397174859417,-5.80922950760163,
130.961112087674));
#248816=CARTESIAN_POINT('Ctrl Pts',(-84.0181651097544,-3.00815099594316,
135.776557926701));
#248817=CARTESIAN_POINT('Ctrl Pts',(-84.2966127335676,2.55727132464077,
136.022797343974));
#248818=CARTESIAN_POINT('Ctrl Pts',(-84.5750603573801,5.77268622752965,
131.473548344486));
#248819=CARTESIAN_POINT('Ctrl Pts',(-84.8535079811934,3.68328449871872,
126.309348515594));
#248820=CARTESIAN_POINT('Ctrl Pts',(-85.131955605006,-1.79087574596318,
125.275845214866));
#248821=CARTESIAN_POINT('Ctrl Pts',(-85.4104032288191,-5.61930866924928,
129.322777486226));
#248822=CARTESIAN_POINT('Ctrl Pts',(-85.6888508526319,-4.28387144398495,
134.731212275928));
#248823=CARTESIAN_POINT('Ctrl Pts',(-85.9672984764448,0.98823435954663,
136.531062228962));
#248824=CARTESIAN_POINT('Ctrl Pts',(-86.2457461002577,5.35220106458756,
133.068353166051));
#248825=CARTESIAN_POINT('Ctrl Pts',(-86.5241937240705,4.79775646083024,
127.525145553266));
#248826=CARTESIAN_POINT('Ctrl Pts',(-86.8026413478836,-0.165591946996939,
124.995376386011));
#248827=CARTESIAN_POINT('Ctrl Pts',(-87.0810889716963,-4.97676944515001,
127.803779942897));
#248828=CARTESIAN_POINT('Ctrl Pts',(-87.3595365955093,-5.21453895191432,
133.36957055329));
#248829=CARTESIAN_POINT('Ctrl Pts',(-87.6379842193221,-0.660401906259044,
136.578058550223));
#248830=CARTESIAN_POINT('Ctrl Pts',(-87.916431843135,4.50061222882128,134.480800207869));
#248831=CARTESIAN_POINT('Ctrl Pts',(-88.1948794669479,5.52578359274576,
129.005073486085));
#248832=CARTESIAN_POINT('Ctrl Pts',(-88.4733270907608,1.47302978447255,
125.182803738068));
#248833=CARTESIAN_POINT('Ctrl Pts',(-88.7517747145737,-3.93336643422502,
126.526470133988));
#248834=CARTESIAN_POINT('Ctrl Pts',(-89.0302223383866,-5.7251910555031,
131.801308897747));
#248835=CARTESIAN_POINT('Ctrl Pts',(-89.3086699621995,-2.25584478790559,
136.16000089565));
#248836=CARTESIAN_POINT('Ctrl Pts',(-89.5871175860123,3.28651263563227,
135.597121115567));
#248837=CARTESIAN_POINT('Ctrl Pts',(-89.8655652098253,5.80872550209253,
130.629928577187));
#248838=CARTESIAN_POINT('Ctrl Pts',(-90.1440128336381,2.99300340414587,
125.823030562435));
#248839=CARTESIAN_POINT('Ctrl Pts',(-90.4224604574511,-2.57314260586573,
125.593731516848));
#248840=CARTESIAN_POINT('Ctrl Pts',(-90.7009080812639,-5.77469626609129,
130.152746061436));
#248841=CARTESIAN_POINT('Ctrl Pts',(-90.9793557050769,-3.66958616737523,
135.310562549967));
#248842=CARTESIAN_POINT('Ctrl Pts',(-91.2578033288896,1.80769434990835,
136.327399602824));
#248843=CARTESIAN_POINT('Ctrl Pts',(-91.5362509527026,5.62379207040447,
132.268833643682));
#248844=CARTESIAN_POINT('Ctrl Pts',(-91.8146985765155,4.27189961571542,
126.864488517025));
#248845=CARTESIAN_POINT('Ctrl Pts',(-92.0931462003284,-1.00565989191805,
125.080693377311));
#248846=CARTESIAN_POINT('Ctrl Pts',(-92.3715938241412,-5.3590670880956,
128.556668814702));
#248847=CARTESIAN_POINT('Ctrl Pts',(-92.6500414479542,-4.78775343529548,
134.098163213075));
#248848=CARTESIAN_POINT('Ctrl Pts',(-92.928489071767,0.183271729783054,
136.612813937377));
#248849=CARTESIAN_POINT('Ctrl Pts',(-93.2069366955801,4.98587912851244,
133.789779819492));
#248850=CARTESIAN_POINT('Ctrl Pts',(-93.4853843193926,5.2067071818758,128.223291300872));
#248851=CARTESIAN_POINT('Ctrl Pts',(-93.7638319432059,0.642825696881324,
125.028679392048));
#248852=CARTESIAN_POINT('Ctrl Pts',(-94.0422795670186,-4.51178119976554,
127.14163637176));
#248853=CARTESIAN_POINT('Ctrl Pts',(-94.3207271908314,-5.52028158659305,
132.62045799934));
#248854=CARTESIAN_POINT('Ctrl Pts',(-94.5991748146444,-1.45591287608963,
136.430374854359));
#248855=CARTESIAN_POINT('Ctrl Pts',(-94.8776224384574,3.94636864224209,
135.07025947184));
#248856=CARTESIAN_POINT('Ctrl Pts',(-95.1560700622702,5.7221301691794,129.789991442987));
#248857=CARTESIAN_POINT('Ctrl Pts',(-95.4345176860831,2.23953361224044,
125.441879130882));
#248858=CARTESIAN_POINT('Ctrl Pts',(-95.7129653098959,-3.30108492704829,
126.021625333256));
#248859=CARTESIAN_POINT('Ctrl Pts',(-95.9914129337089,-5.80816768534362,
130.996471612301));
#248860=CARTESIAN_POINT('Ctrl Pts',(-96.2698605575217,-2.97782808557417,
135.794777272329));
#248861=CARTESIAN_POINT('Ctrl Pts',(-96.5483081813347,2.58899004984866,
136.007133822036));
#248862=CARTESIAN_POINT('Ctrl Pts',(-96.8267558051475,5.77665280865574,
131.438395966436));
#248863=CARTESIAN_POINT('Ctrl Pts',(-97.1052034289604,3.65585384148698,
126.287010599573));
#248864=CARTESIAN_POINT('Ctrl Pts',(-97.3836510527732,-1.82449620761995,
125.286849214428));
#248865=CARTESIAN_POINT('Ctrl Pts',(-97.6620986765863,-5.62822337351841,
129.35701126335));
#248866=CARTESIAN_POINT('Ctrl Pts',(-97.9405463003989,-4.25988821315111,
134.757216661848));
#248867=CARTESIAN_POINT('Ctrl Pts',(-98.2189939242121,1.02307610799351,
136.524940463405));
#248868=CARTESIAN_POINT('Ctrl Pts',(-98.4974415480248,5.36588346593846,
133.035730852497));
#248869=CARTESIAN_POINT('Ctrl Pts',(-98.7758891718378,4.77770605666655,
127.496001004183));
#248870=CARTESIAN_POINT('Ctrl Pts',(-99.0543367956506,-0.200949814765295,
124.996492018215));
#248871=CARTESIAN_POINT('Ctrl Pts',(-99.3327844194636,-4.99494262337204,
127.834130544897));
#248872=CARTESIAN_POINT('Ctrl Pts',(-99.6112320432764,-5.19882717761281,
133.401265404553));
#248873=CARTESIAN_POINT('Ctrl Pts',(-99.8896796670892,-0.625243532454567,
136.581971630822));
#248874=CARTESIAN_POINT('Ctrl Pts',(-100.168127290903,4.5229083741848,134.453335587896));
#248875=CARTESIAN_POINT('Ctrl Pts',(-100.446574914715,5.51472844130613,
128.971469809575));
#248876=CARTESIAN_POINT('Ctrl Pts',(-100.725022538528,1.43878248032906,
125.173941142103));
#248877=CARTESIAN_POINT('Ctrl Pts',(-101.003470162341,-3.95933429163924,
126.550492911299));
#248878=CARTESIAN_POINT('Ctrl Pts',(-101.281917786154,-5.71901627382367,
131.836141289563));
#248879=CARTESIAN_POINT('Ctrl Pts',(-101.560365409967,-2.22320168984167,
136.17363363555));
#248880=CARTESIAN_POINT('Ctrl Pts',(-101.83881303378,3.31562663766449,135.577026381578));
#248881=CARTESIAN_POINT('Ctrl Pts',(-102.117260657593,5.80755606252295,
130.594572448163));
#248882=CARTESIAN_POINT('Ctrl Pts',(-102.395708281405,2.96262518080941,
125.804903593708));
#248883=CARTESIAN_POINT('Ctrl Pts',(-102.674155905219,-2.60481350978186,
125.609491507123));
#248884=CARTESIAN_POINT('Ctrl Pts',(-102.952603529031,-5.77855583709781,
130.187910349571));
#248885=CARTESIAN_POINT('Ctrl Pts',(-103.231051152844,-3.64208764826766,
135.332816873036));
#248886=CARTESIAN_POINT('Ctrl Pts',(-103.509498776657,1.84128116344741,
136.316293325111));
#248887=CARTESIAN_POINT('Ctrl Pts',(-103.78794640047,5.63260253753978,132.234572891835));
#248888=CARTESIAN_POINT('Ctrl Pts',(-104.066394024283,4.24783734756473,
126.838557248259));
#248889=CARTESIAN_POINT('Ctrl Pts',(-104.344841648096,-1.04048284643121,
125.086921160811));
#248890=CARTESIAN_POINT('Ctrl Pts',(-104.623289271909,-5.3726501349701,
128.589332621676));
#248891=CARTESIAN_POINT('Ctrl Pts',(-104.901736895722,-4.76761441802147,
134.12724660063));
#248892=CARTESIAN_POINT('Ctrl Pts',(-105.180184519534,0.218626038175886,
136.611590693152));
#248893=CARTESIAN_POINT('Ctrl Pts',(-105.458632143348,5.00395984576562,
133.759374045173));
#248894=CARTESIAN_POINT('Ctrl Pts',(-105.73707976716,5.1908990121252,128.191644417652));
#248895=CARTESIAN_POINT('Ctrl Pts',(-106.015527390973,0.607655575856702,
125.024873339572));
#248896=CARTESIAN_POINT('Ctrl Pts',(-106.293975014786,-4.53399364899913,
127.169168726316));
#248897=CARTESIAN_POINT('Ctrl Pts',(-106.572422638599,-5.50912420832816,
132.654027872123));
#248898=CARTESIAN_POINT('Ctrl Pts',(-106.850870262412,-1.42163875588365,
136.43913317226));
#248899=CARTESIAN_POINT('Ctrl Pts',(-107.129317886225,3.97226326230387,
135.046157768576));
#248900=CARTESIAN_POINT('Ctrl Pts',(-107.407765510038,5.71584939828273,
129.755178006424));
#248901=CARTESIAN_POINT('Ctrl Pts',(-107.686213133851,2.20684917200607,
125.428345808491));
#248902=CARTESIAN_POINT('Ctrl Pts',(-107.964660757664,-3.3301376327682,
126.041808587174));
#248903=CARTESIAN_POINT('Ctrl Pts',(-108.243108381476,-5.80689063929651,
131.031824018185));
#248904=CARTESIAN_POINT('Ctrl Pts',(-108.521556005289,-2.94739483068967,
135.812811696231));
#248905=CARTESIAN_POINT('Ctrl Pts',(-108.800003629102,2.62061283907833,
135.991277509423));
#248906=CARTESIAN_POINT('Ctrl Pts',(-109.078451252915,5.7804053337882,131.403220093974));
#248907=CARTESIAN_POINT('Ctrl Pts',(-109.356898876728,3.62828771524594,
126.264840075618));
#248908=CARTESIAN_POINT('Ctrl Pts',(-109.635346500541,-1.85804906189805,
125.298057667405));
#248909=CARTESIAN_POINT('Ctrl Pts',(-109.913794124354,-5.636929521901,129.391298672536));
#248910=CARTESIAN_POINT('Ctrl Pts',(-110.192241748167,-4.2357471305931,
134.783074573235));
#248911=CARTESIAN_POINT('Ctrl Pts',(-110.470689371979,1.05787994597834,
136.518606719657));
#248912=CARTESIAN_POINT('Ctrl Pts',(-110.749136995792,5.37936703250445,
133.003025854698));
#248913=CARTESIAN_POINT('Ctrl Pts',(-111.027584619605,4.75747861284798,
127.466979047582));
#248914=CARTESIAN_POINT('Ctrl Pts',(-111.306032243418,-0.23630023626489,
124.997822863128));
#248915=CARTESIAN_POINT('Ctrl Pts',(-111.584479867231,-5.01293071215839,
127.864591209862));
#248916=CARTESIAN_POINT('Ctrl Pts',(-111.862927491044,-5.18292275885852,
133.432864026556));
#248917=CARTESIAN_POINT('Ctrl Pts',(-112.141375114857,-0.590061990020461,
136.585670619917));
#248918=CARTESIAN_POINT('Ctrl Pts',(-112.41982273867,4.54503692151536,134.425735753813));
#248919=CARTESIAN_POINT('Ctrl Pts',(-112.698270362483,5.50346893957634,
128.937934051507));
#248920=CARTESIAN_POINT('Ctrl Pts',(-112.976717986295,1.40448186157095,
125.165287183403));
#248921=CARTESIAN_POINT('Ctrl Pts',(-113.255165610108,-3.98515543446448,
126.574673317241));
#248922=CARTESIAN_POINT('Ctrl Pts',(-113.533613233921,-5.71262957189362,
131.870935448366));
#248923=CARTESIAN_POINT('Ctrl Pts',(-113.812060857734,-2.19047621022174,
136.187067415062));
#248924=CARTESIAN_POINT('Ctrl Pts',(-114.090508481547,3.34461777793161,
135.556754794705));
#248925=CARTESIAN_POINT('Ctrl Pts',(-114.36895610536,5.80617142182825,130.559224092919));
#248926=CARTESIAN_POINT('Ctrl Pts',(-114.647403729173,2.9321371763071,125.786961881698));
#248927=CARTESIAN_POINT('Ctrl Pts',(-114.925851352986,-2.63638789137572,
125.625443995184));
#248928=CARTESIAN_POINT('Ctrl Pts',(-115.204298976799,-5.78220128159277,
130.223097480497));
#248929=CARTESIAN_POINT('Ctrl Pts',(-115.482746600612,-3.61445417026275,
135.354903392492));
#248930=CARTESIAN_POINT('Ctrl Pts',(-115.761194224424,1.87479974763623,
136.304982800703));
#248931=CARTESIAN_POINT('Ctrl Pts',(-116.039641848237,5.64120428651674,
132.200259142944));
#248932=CARTESIAN_POINT('Ctrl Pts',(-116.31808947205,4.22361767423897,126.812772933795));
#248933=CARTESIAN_POINT('Ctrl Pts',(-116.596537095863,-1.07526724547036,
125.093360806132));
#248934=CARTESIAN_POINT('Ctrl Pts',(-116.874984719676,-5.38603409631742,
128.622078507325));
#248935=CARTESIAN_POINT('Ctrl Pts',(-117.153432343489,-4.7472987350426,
134.156206857421));
#248936=CARTESIAN_POINT('Ctrl Pts',(-117.431879967302,0.253972245300257,
136.610152259881));
#248937=CARTESIAN_POINT('Ctrl Pts',(-117.710327591115,5.02185513944583,
133.728858771743));
#248938=CARTESIAN_POINT('Ctrl Pts',(-117.988775214928,5.17489849170343,
128.160094349593));
#248939=CARTESIAN_POINT('Ctrl Pts',(-118.26722283874,0.572462937930709,
125.021281448121));
#248940=CARTESIAN_POINT('Ctrl Pts',(-118.545670462553,-4.55603808943068,
127.196835784245));
#248941=CARTESIAN_POINT('Ctrl Pts',(-118.824118086366,-5.49776268743969,
132.687529204804));
#248942=CARTESIAN_POINT('Ctrl Pts',(-119.102565710179,-1.38731195633035,
136.447682691592));
#248943=CARTESIAN_POINT('Ctrl Pts',(-119.381013333992,3.99801068868978,
135.021898883958));
#248944=CARTESIAN_POINT('Ctrl Pts',(-119.659460957805,5.70935682448427,
129.720403447709));
#248945=CARTESIAN_POINT('Ctrl Pts',(-119.937908581618,2.17408295616475,
125.415011696306));
#248946=CARTESIAN_POINT('Ctrl Pts',(-120.216356205431,-3.3590669390133,
126.062168319208));
#248947=CARTESIAN_POINT('Ctrl Pts',(-120.494803829244,-5.80539841678086,
131.067167995328));
#248948=CARTESIAN_POINT('Ctrl Pts',(-120.773251453056,-2.91685235900652,
135.830660530138));
#248949=CARTESIAN_POINT('Ctrl Pts',(-121.051699076869,2.65213852053535,
135.975228993696));
#248950=CARTESIAN_POINT('Ctrl Pts',(-121.330146700682,5.78394366387473,
131.368022030553));
#248951=CARTESIAN_POINT('Ctrl Pts',(-121.608594324495,3.60058714147007,
126.242837765265));
#248952=CARTESIAN_POINT('Ctrl Pts',(-121.887041948308,-1.89153306548558,
125.309470158462));
#248953=CARTESIAN_POINT('Ctrl Pts',(-122.165489572121,-5.64542679178685,
129.425638443252));
#248954=CARTESIAN_POINT('Ctrl Pts',(-122.443937195934,-4.21144909086733,
134.808785051914));
#248955=CARTESIAN_POINT('Ctrl Pts',(-122.722384819747,1.09264458383337,
136.512061232418));
#248956=CARTESIAN_POINT('Ctrl Pts',(-123.00083244356,5.39265126464657,132.97023938455));
#248957=CARTESIAN_POINT('Ctrl Pts',(-123.279280067372,4.73707487890982,
127.438080758883));
#248958=CARTESIAN_POINT('Ctrl Pts',(-123.557727691185,-0.27164190157181,
124.999368871432));
#248959=CARTESIAN_POINT('Ctrl Pts',(-123.836175314998,-5.03073304495359,
127.895160809065));
#248960=CARTESIAN_POINT('Ctrl Pts',(-124.114622938811,-5.16682628499523,
133.464365248398));
#248961=CARTESIAN_POINT('Ctrl Pts',(-124.393070562624,-0.554858582622917,
136.589155380447));
#248962=CARTESIAN_POINT('Ctrl Pts',(-124.671518186437,4.56699705083122,
134.398001728342));
#248963=CARTESIAN_POINT('Ctrl Pts',(-124.94996581025,5.49200550478084,128.904467454562));
#248964=CARTESIAN_POINT('Ctrl Pts',(-125.228413434063,1.37012919922165,
125.156842182641));
#248965=CARTESIAN_POINT('Ctrl Pts',(-125.506861057876,-4.0108289058903,
126.599010455801));
#248966=CARTESIAN_POINT('Ctrl Pts',(-125.785308681688,-5.70603118637341,
131.905690084846));
#248967=CARTESIAN_POINT('Ctrl Pts',(-126.063756305501,-2.1576695617001,
136.200301736396));
#248968=CARTESIAN_POINT('Ctrl Pts',(-126.342203929314,3.37348498215772,
135.536307106118));
#248969=CARTESIAN_POINT('Ctrl Pts',(-126.620651553127,5.8045716313158,130.523884821299));
#248970=CARTESIAN_POINT('Ctrl Pts',(-126.89909917694,2.90154052038371,125.769206091244));
#248971=CARTESIAN_POINT('Ctrl Pts',(-127.177546800753,-2.66786458064647,
125.641588389905));
#248972=CARTESIAN_POINT('Ctrl Pts',(-127.455994424566,-5.7856324644928,
130.258306150342));
#248973=CARTESIAN_POINT('Ctrl Pts',(-127.734442048379,-3.5866867573295,
135.376821289913));
#248974=CARTESIAN_POINT('Ctrl Pts',(-128.012889672192,1.90824886043053,
136.293468448719));
#248975=CARTESIAN_POINT('Ctrl Pts',(-128.291337296005,5.64959699859458,
132.16589366852));
#248976=CARTESIAN_POINT('Ctrl Pts',(-128.569784919818,4.19924149320669,
126.787136529081));
#248977=CARTESIAN_POINT('Ctrl Pts',(-128.84823254363,-1.11001180008614,
125.100012074652));
#248978=CARTESIAN_POINT('Ctrl Pts',(-129.126680167443,-5.39921847619124,
128.654905258242));
#248979=CARTESIAN_POINT('Ctrl Pts',(-129.405127791256,-4.72680713916258,
134.185042910317));
#248980=CARTESIAN_POINT('Ctrl Pts',(-129.683575415069,0.289309041389885,
136.608498690867));
#248981=CARTESIAN_POINT('Ctrl Pts',(-129.962023038882,5.03956434643776,
133.69823512996));
#248982=CARTESIAN_POINT('Ctrl Pts',(-130.240470662695,5.15870621351431,
128.128642265792));
#248983=CARTESIAN_POINT('Ctrl Pts',(-130.518918286508,0.537249087180579,
125.017903850796));
#248984=CARTESIAN_POINT('Ctrl Pts',(-130.79736591032,-4.57791370419536,
127.224636520332));
#248985=CARTESIAN_POINT('Ctrl Pts',(-131.075813534134,-5.4861974449331,
132.720960755981));
#248986=CARTESIAN_POINT('Ctrl Pts',(-131.354261157946,-1.35293374942274,
136.456023095549));
#248987=CARTESIAN_POINT('Ctrl Pts',(-131.632708781759,4.02360996731925,
134.99748371691));
#248988=CARTESIAN_POINT('Ctrl Pts',(-131.911156405572,5.7026526883694,129.685669055425));
#248989=CARTESIAN_POINT('Ctrl Pts',(-132.189604029385,2.1412361788793,125.401877288427));
#248990=CARTESIAN_POINT('Ctrl Pts',(-132.468051653198,-3.38787177379785,
126.082703774923));
#248991=CARTESIAN_POINT('Ctrl Pts',(-132.746499277011,-5.80369107309236,
131.102502234048));
#248992=CARTESIAN_POINT('Ctrl Pts',(-133.024946900823,-2.88620180228584,
135.848323112653));
#248993=CARTESIAN_POINT('Ctrl Pts',(-133.303394524637,2.68356592602436,
135.95898886954));
#248994=CARTESIAN_POINT('Ctrl Pts',(-133.581842148449,5.78726766780228,
131.332803080451));
#248995=CARTESIAN_POINT('Ctrl Pts',(-133.860289772262,3.57275314661281,
126.221004483821));
#248996=CARTESIAN_POINT('Ctrl Pts',(-134.138737396075,-1.92494697761906,
125.321086264707));
#248997=CARTESIAN_POINT('Ctrl Pts',(-134.417185019888,-5.65371486830715,
129.460029303025));
#248998=CARTESIAN_POINT('Ctrl Pts',(-134.695632643701,-4.1869949943469,
134.834347145171));
#248999=CARTESIAN_POINT('Ctrl Pts',(-134.974080267514,1.1273687333409,136.505304244234));
#249000=CARTESIAN_POINT('Ctrl Pts',(-135.252527891327,5.40573567011315,
132.937372656969));
#249001=CARTESIAN_POINT('Ctrl Pts',(-135.53097551514,4.71649561092,127.409307208922));
#249002=CARTESIAN_POINT('Ctrl Pts',(-135.809423138953,-0.306973501088704,
125.001129985841));
#249003=CARTESIAN_POINT('Ctrl Pts',(-136.087870762765,-5.04834896208586,
127.925838209736));
#249004=CARTESIAN_POINT('Ctrl Pts',(-136.366318386578,-5.15053835248403,
133.49576790279));
#249005=CARTESIAN_POINT('Ctrl Pts',(-136.644766010391,-0.519634614735935,
136.592425783278));
#249006=CARTESIAN_POINT('Ctrl Pts',(-136.923213634204,4.58878794839197,
134.37013453918));
#249007=CARTESIAN_POINT('Ctrl Pts',(-137.201661258017,5.48033856170195,
128.871071258858));
#249008=CARTESIAN_POINT('Ctrl Pts',(-137.48010888183,1.33572576623031,125.148606452753));
#249009=CARTESIAN_POINT('Ctrl Pts',(-137.758556505643,-4.03635375457527,
126.623503425159));
#249010=CARTESIAN_POINT('Ctrl Pts',(-138.037004129456,-5.69922136176977,
131.940403911158));
#249011=CARTESIAN_POINT('Ctrl Pts',(-138.315451753269,-2.12478295993955,
136.213336109146));
#249012=CARTESIAN_POINT('Ctrl Pts',(-138.593899377082,3.40222718065648,
135.515684073514));
#249013=CARTESIAN_POINT('Ctrl Pts',(-138.872347000894,5.80275675026745,
130.488555942812));
#249014=CARTESIAN_POINT('Ctrl Pts',(-139.150794624707,2.870836346809,125.751636880291));
#249015=CARTESIAN_POINT('Ctrl Pts',(-139.42924224852,-2.69924241121433,
125.65792409305));
#249016=CARTESIAN_POINT('Ctrl Pts',(-139.707689872333,-5.78884925865424,
130.293535054436));
#249017=CARTESIAN_POINT('Ctrl Pts',(-139.986137496146,-3.55878643839929,
135.398569753122));
#249018=CARTESIAN_POINT('Ctrl Pts',(-140.264585119959,1.94162726236197,
136.281750695826));
#249019=CARTESIAN_POINT('Ctrl Pts',(-140.543032743772,5.65778036277742,
132.131477741989));
#249020=CARTESIAN_POINT('Ctrl Pts',(-140.821480367585,4.17470970773734,
126.761648984083));
#249021=CARTESIAN_POINT('Ctrl Pts',(-141.099927991397,-1.14471522280625,
125.106874719905));
#249022=CARTESIAN_POINT('Ctrl Pts',(-141.37837561521,-5.41220278603824,
128.687811658017));
#249023=CARTESIAN_POINT('Ctrl Pts',(-141.656823239023,-4.70614038970644,
134.213753690789));
#249024=CARTESIAN_POINT('Ctrl Pts',(-141.935270862836,0.324635117026387,
136.60663004738));
#249025=CARTESIAN_POINT('Ctrl Pts',(-142.213718486649,5.05708681051884,
133.667504254592));
#249026=CARTESIAN_POINT('Ctrl Pts',(-142.492166110462,5.14232277757003,
128.097289331719));
#249027=CARTESIAN_POINT('Ctrl Pts',(-142.770613734275,0.502015328467386,
125.014740672754));
#249028=CARTESIAN_POINT('Ctrl Pts',(-143.049061358088,-4.59961968268416,
127.252569904414));
#249029=CARTESIAN_POINT('Ctrl Pts',(-143.327508981901,-5.4744289093626,
132.754321286837));
#249030=CARTESIAN_POINT('Ctrl Pts',(-143.605956605714,-1.31850540905707,
136.464154075075));
#249031=CARTESIAN_POINT('Ctrl Pts',(-143.884404229526,4.04906014960179,
134.972913172143));
#249032=CARTESIAN_POINT('Ctrl Pts',(-144.162851853339,5.69573723836169,
129.650976116669));
#249033=CARTESIAN_POINT('Ctrl Pts',(-144.441299477152,2.10831005730047,
125.388943071553));
#249034=CARTESIAN_POINT('Ctrl Pts',(-144.719747100965,-3.41655106974776,
126.103414193369));
#249035=CARTESIAN_POINT('Ctrl Pts',(-144.998194724778,-5.80176867149642,
131.13782542502));
#249036=CARTESIAN_POINT('Ctrl Pts',(-145.276642348591,-2.85544429629671,
135.865798789283));
#249037=CARTESIAN_POINT('Ctrl Pts',(-145.555089972404,2.71489389099137,
135.942557738738));
#249038=CARTESIAN_POINT('Ctrl Pts',(-145.833537596217,5.79037722239768,
131.29756454872));
#249039=CARTESIAN_POINT('Ctrl Pts',(-146.111985220029,3.54478676207412,
126.199341040322));
#249040=CARTESIAN_POINT('Ctrl Pts',(-146.390432843843,-1.95828956013508,
125.332905555698));
#249041=CARTESIAN_POINT('Ctrl Pts',(-146.668880467655,-5.66179344434354,
129.49446997749));
#249042=CARTESIAN_POINT('Ctrl Pts',(-146.947328091469,-4.16238574718705,
134.859759905796));
#249043=CARTESIAN_POINT('Ctrl Pts',(-147.225775715281,1.16205110778606,
136.498336005488));
#249044=CARTESIAN_POINT('Ctrl Pts',(-147.504223339094,5.41861976405632,
132.904426889841));
#249045=CARTESIAN_POINT('Ctrl Pts',(-147.782670962907,4.6957415714508,127.380659463914));
#249046=CARTESIAN_POINT('Ctrl Pts',(-148.06111858672,-0.342293725589094,
125.003106141093));
#249047=CARTESIAN_POINT('Ctrl Pts',(-148.339566210533,-5.06577781079073,
127.956622275114));
#249048=CARTESIAN_POINT('Ctrl Pts',(-148.618013834346,-5.1340595648799,
133.527070826096));
#249049=CARTESIAN_POINT('Ctrl Pts',(-148.896461458158,-0.48439139159784,
136.595481707227));
#249050=CARTESIAN_POINT('Ctrl Pts',(-149.174909081971,4.61040880672808,
134.342135218952));
#249051=CARTESIAN_POINT('Ctrl Pts',(-149.453356705784,5.4684685426618,128.837746701901));
#249052=CARTESIAN_POINT('Ctrl Pts',(-149.731804329597,1.30127283742975,
125.140580298914));
#249053=CARTESIAN_POINT('Ctrl Pts',(-150.01025195341,-4.06172903468827,
126.648151317718));
#249054=CARTESIAN_POINT('Ctrl Pts',(-150.288699577223,-5.69220035042211,
131.975075640969));
#249055=CARTESIAN_POINT('Ctrl Pts',(-150.567147201036,-2.09181762356486,
136.226170050321));
#249056=CARTESIAN_POINT('Ctrl Pts',(-150.845594824849,3.43084330837664,
135.494886461086));
#249057=CARTESIAN_POINT('Ctrl Pts',(-151.124042448661,5.80072684593324,
130.453238766583));
#249058=CARTESIAN_POINT('Ctrl Pts',(-151.402490072475,2.84002579333802,
125.734254899877));
#249059=CARTESIAN_POINT('Ctrl Pts',(-151.680937696287,-2.73052022036177,
125.674450499292));
#249060=CARTESIAN_POINT('Ctrl Pts',(-151.9593853201,-5.79185154487752,130.32878288736));
#249061=CARTESIAN_POINT('Ctrl Pts',(-152.237832943913,-3.53075424732904,
135.420147976222));
#249062=CARTESIAN_POINT('Ctrl Pts',(-152.516280567726,1.97493371658077,
136.269829976228));
#249063=CARTESIAN_POINT('Ctrl Pts',(-152.794728191539,5.66575407582884,
132.097012638644));
#249064=CARTESIAN_POINT('Ctrl Pts',(-153.073175815352,4.15002322686382,
126.736311243251));
#249065=CARTESIAN_POINT('Ctrl Pts',(-153.351623439165,-1.17937622768304,
125.113948487592));
#249066=CARTESIAN_POINT('Ctrl Pts',(-153.630071062978,-5.42498654472129,
128.720796487292));
#249067=CARTESIAN_POINT('Ctrl Pts',(-153.90851868679,-4.6852992524868,134.242338134946));
#249068=CARTESIAN_POINT('Ctrl Pts',(-154.186966310604,0.359949163189457,
136.604546398667));
#249069=CARTESIAN_POINT('Ctrl Pts',(-154.465413934416,5.0744218823891,133.636667284384));
#249070=CARTESIAN_POINT('Ctrl Pts',(-154.743861558229,5.12574879096345,
128.066036709167));
#249071=CARTESIAN_POINT('Ctrl Pts',(-155.022309182042,0.466762967392146,
125.011792031209));
#249072=CARTESIAN_POINT('Ctrl Pts',(-155.300756805855,-4.62115522057418,
127.280634901405));
#249073=CARTESIAN_POINT('Ctrl Pts',(-155.579204429668,-5.46245751681569,
132.787609561181));
#249074=CARTESIAN_POINT('Ctrl Pts',(-155.857652053481,-1.28402821098903,
136.472075328871));
#249075=CARTESIAN_POINT('Ctrl Pts',(-156.136099677293,4.07436029247137,
134.948188160129));
#249076=CARTESIAN_POINT('Ctrl Pts',(-156.414547301107,5.68861073071636,
129.616325916999));
#249077=CARTESIAN_POINT('Ctrl Pts',(-156.692994924919,2.07530581151645,
125.376209524969));
#249078=CARTESIAN_POINT('Ctrl Pts',(-156.971442548732,-3.44510376414151,
126.124298807112));
#249079=CARTESIAN_POINT('Ctrl Pts',(-157.249890172545,-5.79963128322921,
131.173136259331));
#249080=CARTESIAN_POINT('Ctrl Pts',(-157.528337796358,-2.82458098076833,
135.883086912459));
#249081=CARTESIAN_POINT('Ctrl Pts',(-157.806785420171,2.74612125456611,
135.925936210153));
#249082=CARTESIAN_POINT('Ctrl Pts',(-158.085233043984,5.79327221243612,
131.262307741136));
#249083=CARTESIAN_POINT('Ctrl Pts',(-158.363680667797,3.51668902415852,
126.177848237519));
#249084=CARTESIAN_POINT('Ctrl Pts',(-158.64212829161,-1.9915595775106,125.344927593469));
#249085=CARTESIAN_POINT('Ctrl Pts',(-158.920575915422,-5.66966222054205,
129.528959190434));
#249086=CARTESIAN_POINT('Ctrl Pts',(-159.199023539236,-4.13762226129274,
134.885022392109));
#249087=CARTESIAN_POINT('Ctrl Pts',(-159.477471163048,1.19669042199943,
136.491156774389));
#249088=CARTESIAN_POINT('Ctrl Pts',(-159.755918786861,5.43130306905165,
132.871403303985));
#249089=CARTESIAN_POINT('Ctrl Pts',(-160.034366410674,4.67481352955083,
127.352138585409));
#249090=CARTESIAN_POINT('Ctrl Pts',(-160.312814034487,-0.377601266270116,
125.005297263965));
#249091=CARTESIAN_POINT('Ctrl Pts',(-160.5912616583,-5.08301894523598,127.987511864483));
#249092=CARTESIAN_POINT('Ctrl Pts',(-160.869709282113,-5.1173905328107,
133.558272858373));
#249093=CARTESIAN_POINT('Ctrl Pts',(-161.148156905926,-0.449130219157962,
136.598323039052));
#249094=CARTESIAN_POINT('Ctrl Pts',(-161.426604529739,4.63185882466967,
134.314004805186));
#249095=CARTESIAN_POINT('Ctrl Pts',(-161.705052153551,5.45639588750942,
128.804495018547));
#249096=CARTESIAN_POINT('Ctrl Pts',(-161.983499777364,1.26677168948586,
125.13276401854));
#249097=CARTESIAN_POINT('Ctrl Pts',(-162.261947401177,-4.08695380593746,
126.67295322014));
#249098=CARTESIAN_POINT('Ctrl Pts',(-162.54039502499,-5.68496841249774,
132.009703989503));
#249099=CARTESIAN_POINT('Ctrl Pts',(-162.818842648803,-2.05877477411906,
136.238803084352));
#249100=CARTESIAN_POINT('Ctrl Pts',(-163.097290272616,3.45933230493559,
135.473915039499));
#249101=CARTESIAN_POINT('Ctrl Pts',(-163.375737896429,5.79848199353304,
130.417934601304));
#249102=CARTESIAN_POINT('Ctrl Pts',(-163.654185520242,2.80911000166655,
125.717060794092));
#249103=CARTESIAN_POINT('Ctrl Pts',(-163.932633144055,-2.76169684907854,
125.691166996241));
#249104=CARTESIAN_POINT('Ctrl Pts',(-164.211080767867,-5.79463921191188,
130.36404834299));
#249105=CARTESIAN_POINT('Ctrl Pts',(-164.489528391681,-3.50259122286156,
135.441555159625));
#249106=CARTESIAN_POINT('Ctrl Pts',(-164.767976015493,2.00816698890481,
136.257706731653));
#249107=CARTESIAN_POINT('Ctrl Pts',(-165.046423639306,5.67351784227885,
132.062499635604));
#249108=CARTESIAN_POINT('Ctrl Pts',(-165.324871263119,4.12518296535417,
126.711124245485));
#249109=CARTESIAN_POINT('Ctrl Pts',(-165.603318886932,-1.21399353033979,
125.121233115594));
#249110=CARTESIAN_POINT('Ctrl Pts',(-165.881766510745,-5.43756927853226,
128.753858523801));
#249111=CARTESIAN_POINT('Ctrl Pts',(-166.160214134558,-4.66428449978105,
134.270795183582));
#249112=CARTESIAN_POINT('Ctrl Pts',(-166.438661758371,0.395249871304121,
136.602247821935));
#249113=CARTESIAN_POINT('Ctrl Pts',(-166.717109382183,5.09156891968999,
133.60572536201));
#249114=CARTESIAN_POINT('Ctrl Pts',(-166.995557005996,5.10898486785074,
128.034885556215));
#249115=CARTESIAN_POINT('Ctrl Pts',(-167.274004629809,0.431493310242956,
125.009058035423));
#249116=CARTESIAN_POINT('Ctrl Pts',(-167.552452253622,-4.64251951985801,
127.30883047135));
#249117=CARTESIAN_POINT('Ctrl Pts',(-167.830899877435,-5.45028371089662,
132.820824345507));
#249118=CARTESIAN_POINT('Ctrl Pts',(-168.109347501248,-1.24950343278299,
136.479786563416));
#249119=CARTESIAN_POINT('Ctrl Pts',(-168.387795125061,4.09950945842204,
134.923309597059));
#249120=CARTESIAN_POINT('Ctrl Pts',(-168.666242748874,5.68127342950807,
129.581719740392));
#249121=CARTESIAN_POINT('Ctrl Pts',(-168.944690372687,2.04222466451309,
125.36367712052));
#249122=CARTESIAN_POINT('Ctrl Pts',(-169.223137996499,-3.47352879894819,
126.145356842267));
#249123=CARTESIAN_POINT('Ctrl Pts',(-169.501585620313,-5.79727898749155,
131.208433428525));
#249124=CARTESIAN_POINT('Ctrl Pts',(-169.780033244125,-2.79361299935373,
135.900186841566));
#249125=CARTESIAN_POINT('Ctrl Pts',(-170.058480867939,2.77724685960862,
135.909124899701));
#249126=CARTESIAN_POINT('Ctrl Pts',(-170.336928491751,5.79595253064181,
131.227033964152));
#249127=CARTESIAN_POINT('Ctrl Pts',(-170.615376115564,3.48846097403773,
126.156526871832));
#249128=CARTESIAN_POINT('Ctrl Pts',(-170.893823739377,-2.02475579691427,
125.357151932539));
#249129=CARTESIAN_POINT('Ctrl Pts',(-171.17227136319,-5.67732090532164,
129.563495663847));
#249130=CARTESIAN_POINT('Ctrl Pts',(-171.450718987003,-4.11270545428381,
134.910133667999));
#249131=CARTESIAN_POINT('Ctrl Pts',(-171.729166610815,1.23128539240979,
136.483766816968));
#249132=CARTESIAN_POINT('Ctrl Pts',(-172.007614234629,5.44378511511418,
132.838303123102));
#249133=CARTESIAN_POINT('Ctrl Pts',(-172.286061858441,4.65371226071637,
127.323745630264));
#249134=CARTESIAN_POINT('Ctrl Pts',(-172.564509482254,-0.412894814796852,
125.00770327326));
#249135=CARTESIAN_POINT('Ctrl Pts',(-172.842957106067,-5.10007172654484,
128.018505833219));
#249136=CARTESIAN_POINT('Ctrl Pts',(-173.12140472988,-5.10053187395325,
133.589372843419));
#249137=CARTESIAN_POINT('Ctrl Pts',(-173.399852353693,-0.413852404033268,
136.600949673471));
#249138=CARTESIAN_POINT('Ctrl Pts',(-173.678299977506,4.65313720737985,
134.285744340263));
#249139=CARTESIAN_POINT('Ctrl Pts',(-173.956747601319,5.44412104360021,
128.771317440947));
#249140=CARTESIAN_POINT('Ctrl Pts',(-174.235195225131,1.23222360085094,
125.125157901261));
#249141=CARTESIAN_POINT('Ctrl Pts',(-174.513642848945,-4.11202713361109,
126.697908213384));
#249142=CARTESIAN_POINT('Ctrl Pts',(-174.792090472757,-5.67752581597763,
132.044287673595));
#249143=CARTESIAN_POINT('Ctrl Pts',(-175.070538096571,-2.02565563601667,
136.251234743121));
#249144=CARTESIAN_POINT('Ctrl Pts',(-175.348985720383,3.48769311466452,
135.452770585855));
#249145=CARTESIAN_POINT('Ctrl Pts',(-175.627433344196,5.79602227624969,
130.382644755183));
#249146=CARTESIAN_POINT('Ctrl Pts',(-175.905880968009,2.77809011739122,
125.700055200075));
#249147=CARTESIAN_POINT('Ctrl Pts',(-176.184328591822,-2.79277114210269,
125.708072964459));
#249148=CARTESIAN_POINT('Ctrl Pts',(-176.462776215635,-5.79721215645926,
130.399330114555));
#249149=CARTESIAN_POINT('Ctrl Pts',(-176.741223839448,-3.47429840858841,
135.462790510077));
#249150=CARTESIAN_POINT('Ctrl Pts',(-177.019671463261,2.04132584786218,
136.245381411334));
#249151=CARTESIAN_POINT('Ctrl Pts',(-177.298119087073,5.68107137443935,
132.02794001176));
#249152=CARTESIAN_POINT('Ctrl Pts',(-177.576566710886,4.10018984367198,
126.686088924097));
#249153=CARTESIAN_POINT('Ctrl Pts',(-177.855014334699,-1.24856584802001,
125.128728333976));
#249154=CARTESIAN_POINT('Ctrl Pts',(-178.133461958512,-5.4499505212146,
128.786996542421));
#249155=CARTESIAN_POINT('Ctrl Pts',(-178.411909582325,-4.64309691029714,
134.29912378221));
#249156=CARTESIAN_POINT('Ctrl Pts',(-178.690357206138,0.430535933288815,
136.599734402363));
#249157=CARTESIAN_POINT('Ctrl Pts',(-178.968804829951,5.10852728703229,
133.574679634036));
#249158=CARTESIAN_POINT('Ctrl Pts',(-179.247252453763,5.09203162942501,
128.00383702718));
#249159=CARTESIAN_POINT('Ctrl Pts',(-179.525700077576,0.396207663951002,
125.006538786706));
#249160=CARTESIAN_POINT('Ctrl Pts',(-179.80414770139,-4.66371178887382,
127.337155569449));
#249161=CARTESIAN_POINT('Ctrl Pts',(-180.082595325202,-5.43790794271038,
132.853964409027));
#249162=CARTESIAN_POINT('Ctrl Pts',(-180.361042949015,-1.2149323537682,
136.487287492965));
#249163=CARTESIAN_POINT('Ctrl Pts',(-180.639490572828,4.12450671554208,
134.898278404822));
#249164=CARTESIAN_POINT('Ctrl Pts',(-180.917938196641,5.67372560662389,
129.547158869193));
#249165=CARTESIAN_POINT('Ctrl Pts',(-181.196385820454,2.00906784212309,
125.351346322599));
#249166=CARTESIAN_POINT('Ctrl Pts',(-181.474833444267,-3.50182512086801,
126.166587518521));
#249167=CARTESIAN_POINT('Ctrl Pts',(-181.75328106808,-5.79471187144949,
131.243715624654));
#249168=CARTESIAN_POINT('Ctrl Pts',(-182.031728691892,-2.76254149958135,
135.917097942958));
#249169=CARTESIAN_POINT('Ctrl Pts',(-182.310176315705,2.80826955274668,
135.892124430331));
#249170=CARTESIAN_POINT('Ctrl Pts',(-182.588623939518,5.79841807769547,
131.191744524852));
#249171=CARTESIAN_POINT('Ctrl Pts',(-182.867071563331,3.46010365771282,
126.135377733334));
#249172=CARTESIAN_POINT('Ctrl Pts',(-183.145519187144,-2.05787698824661,
125.369578119929));
#249173=CARTESIAN_POINT('Ctrl Pts',(-183.423966810957,-5.68476921488759,
129.598078117967));
#249174=CARTESIAN_POINT('Ctrl Pts',(-183.70241443477,-4.08763624946197,
134.93509280296));
#249175=CARTESIAN_POINT('Ctrl Pts',(-183.980862058583,1.26583473708647,
136.476166407061));
#249176=CARTESIAN_POINT('Ctrl Pts',(-184.259309682396,5.45606543971754,
132.805127573733));
#249177=CARTESIAN_POINT('Ctrl Pts',(-184.537757306209,4.63243854686269,
127.295481650585));
#249178=CARTESIAN_POINT('Ctrl Pts',(-184.816204930021,-0.448173063354899,
125.010324079826));
#249179=CARTESIAN_POINT('Ctrl Pts',(-185.094652553834,-5.11693552282041,
128.049603032828));
#249180=CARTESIAN_POINT('Ctrl Pts',(-185.373100177647,-5.08348421301165,
133.620369628814));
#249181=CARTESIAN_POINT('Ctrl Pts',(-185.65154780146,-0.378559253454916,
136.60336151315));
#249182=CARTESIAN_POINT('Ctrl Pts',(-185.929995425273,4.67424316637891,
134.257354871388));
#249183=CARTESIAN_POINT('Ctrl Pts',(-186.208443049086,5.4316444657843,128.73821519851));
#249184=CARTESIAN_POINT('Ctrl Pts',(-186.486890672899,1.19762985171755,
125.117762228929));
#249185=CARTESIAN_POINT('Ctrl Pts',(-186.765338296712,-4.13694808860639,
126.72301537273));
#249186=CARTESIAN_POINT('Ctrl Pts',(-187.043785920525,-5.66987283665109,
132.078825411735));
#249187=CARTESIAN_POINT('Ctrl Pts',(-187.322233544337,-1.99246143649967,
136.263464565965));
#249188=CARTESIAN_POINT('Ctrl Pts',(-187.600681168151,3.51592468664221,
135.43145388367));
#249189=CARTESIAN_POINT('Ctrl Pts',(-187.879128791963,5.79334778522967,
130.347370535898));
#249190=CARTESIAN_POINT('Ctrl Pts',(-188.157576415776,2.74696728996466,
125.683238747971));
#249191=CARTESIAN_POINT('Ctrl Pts',(-188.436024039589,-2.82374194796541,
125.72516777749));
#249192=CARTESIAN_POINT('Ctrl Pts',(-188.714471663402,-5.79957028317828,
130.434626894674));
#249193=CARTESIAN_POINT('Ctrl Pts',(-188.992919287215,-3.44587685290989,
135.483853240698));
#249194=CARTESIAN_POINT('Ctrl Pts',(-189.271366911028,2.07440906473995,
136.232854471987));
#249195=CARTESIAN_POINT('Ctrl Pts',(-189.54981453484,5.68841439241029,131.993335047731));
#249196=CARTESIAN_POINT('Ctrl Pts',(-189.828262158654,4.07504478794802,
126.661206206783));
#249197=CARTESIAN_POINT('Ctrl Pts',(-190.106709782466,-1.28309189963338,
125.136433864998));
#249198=CARTESIAN_POINT('Ctrl Pts',(-190.385157406279,-5.46212981397553,
128.820209315208));
#249199=CARTESIAN_POINT('Ctrl Pts',(-190.663605030092,-4.62173726915045,
134.327322881104));
#249200=CARTESIAN_POINT('Ctrl Pts',(-190.942052653905,0.465806041606811,
136.597006233083));
#249201=CARTESIAN_POINT('Ctrl Pts',(-191.220500277718,5.12529635601715,
133.543531250871));
#249202=CARTESIAN_POINT('Ctrl Pts',(-191.49894790153,5.07488970389458,127.972892272577));
#249203=CARTESIAN_POINT('Ctrl Pts',(-191.777395525344,0.360907336037817,
125.004234378408));
#249204=CARTESIAN_POINT('Ctrl Pts',(-192.055843149156,-4.68473124233415,
127.365609146106));
#249205=CARTESIAN_POINT('Ctrl Pts',(-192.33429077297,-5.42533067084548,
132.887028523726));
#249206=CARTESIAN_POINT('Ctrl Pts',(-192.612738396782,-1.1803162549878,
136.494577839569));
#249207=CARTESIAN_POINT('Ctrl Pts',(-192.891186020595,4.14935113754904,
134.873095510955));
#249208=CARTESIAN_POINT('Ctrl Pts',(-193.169633644408,5.66596754175055,
129.512644584067));
#249209=CARTESIAN_POINT('Ctrl Pts',(-193.448081268221,1.97583657298603,
125.339217588127));
#249210=CARTESIAN_POINT('Ctrl Pts',(-193.726528892034,-3.52999168137001,
126.187990049162));
#249211=CARTESIAN_POINT('Ctrl Pts',(-194.004976515847,-5.79193003022761,
131.27898154032));
#249212=CARTESIAN_POINT('Ctrl Pts',(-194.28342413966,-2.73136763281852,
135.933819589987));
#249213=CARTESIAN_POINT('Ctrl Pts',(-194.561871763472,2.83918818442447,
135.874935432001));
#249214=CARTESIAN_POINT('Ctrl Pts',(-194.840319387286,5.80066876223446,
131.156440730899));
#249215=CARTESIAN_POINT('Ctrl Pts',(-195.118767011098,3.43161812597426,
126.114401605713));
#249216=CARTESIAN_POINT('Ctrl Pts',(-195.397214634911,-2.09092192419104,
125.382205695184));
#249217=CARTESIAN_POINT('Ctrl Pts',(-195.675662258724,-5.69200687323938,
129.63270527133));
#249218=CARTESIAN_POINT('Ctrl Pts',(-195.954109882537,-4.06241557577554,
134.95989887212));
#249219=CARTESIAN_POINT('Ctrl Pts',(-196.23255750635,1.30033717579212,136.468355826305));
#249220=CARTESIAN_POINT('Ctrl Pts',(-196.511005130163,5.46814358780935,
132.771877885207));
#249221=CARTESIAN_POINT('Ctrl Pts',(-196.789452753976,4.61099317629508,
127.267347693709));
#249222=CARTESIAN_POINT('Ctrl Pts',(-197.067900377789,-0.483434704694746,
125.013159586548));
#249223=CARTESIAN_POINT('Ctrl Pts',(-197.346348001602,-5.13360970916836,
128.080802310993));
#249224=CARTESIAN_POINT('Ctrl Pts',(-197.624795625414,-5.06624818169292,
133.651262065958));
#249225=CARTESIAN_POINT('Ctrl Pts',(-197.903243249227,-0.343252075224855,
136.605558468718));
#249226=CARTESIAN_POINT('Ctrl Pts',(-198.18169087304,4.69517591957924,134.228837450539));
#249227=CARTESIAN_POINT('Ctrl Pts',(-198.460138496853,5.41896661638458,
128.705189517851));
#249228=CARTESIAN_POINT('Ctrl Pts',(-198.738586120666,1.1629917239694,125.110577275591));
#249229=CARTESIAN_POINT('Ctrl Pts',(-199.017033744479,-4.16171574746965,
126.748273767825));
#249230=CARTESIAN_POINT('Ctrl Pts',(-199.295481368292,-5.6620097581009,
132.113315924113));
#249231=CARTESIAN_POINT('Ctrl Pts',(-199.573928992105,-1.95919340559182,
136.275492099704));
#249232=CARTESIAN_POINT('Ctrl Pts',(-199.852376615917,3.54402597473752,
135.409965722843));
#249233=CARTESIAN_POINT('Ctrl Pts',(-200.13082423973,5.79045861957696,130.312113250549));
#249234=CARTESIAN_POINT('Ctrl Pts',(-200.409271863544,2.71574267265526,
125.666612060922));
#249235=CARTESIAN_POINT('Ctrl Pts',(-200.687719487356,-2.85460811903155,
125.742450801881));
#249236=CARTESIAN_POINT('Ctrl Pts',(-200.966167111169,-5.80171350468764,
130.469937375411));
#249237=CARTESIAN_POINT('Ctrl Pts',(-201.244614734982,-3.41732760899753,
135.504742570997));
#249238=CARTESIAN_POINT('Ctrl Pts',(-201.523062358795,2.10741541362659,
136.220126377805));
#249239=CARTESIAN_POINT('Ctrl Pts',(-201.801509982608,5.69554662409457,
131.958686025817));
#249240=CARTESIAN_POINT('Ctrl Pts',(-202.079957606421,4.04974872994014,
126.636477015578));
#249241=CARTESIAN_POINT('Ctrl Pts',(-202.358405230234,-1.31757040580477,
125.144349423131));
#249242=CARTESIAN_POINT('Ctrl Pts',(-202.636852854047,-5.47410670550813,
128.853495611451));
#249243=CARTESIAN_POINT('Ctrl Pts',(-202.915300477859,-4.6002063678289,
134.355391435336));
#249244=CARTESIAN_POINT('Ctrl Pts',(-203.193748101672,0.501058889310003,
136.594063415189));
#249245=CARTESIAN_POINT('Ctrl Pts',(-203.472195725485,5.14187550526088,
133.512281366733));
#249246=CARTESIAN_POINT('Ctrl Pts',(-203.750643349298,5.05755972645996,
127.942052439074));
#249247=CARTESIAN_POINT('Ctrl Pts',(-204.029090973111,0.325593634571106,
125.002144895921));
#249248=CARTESIAN_POINT('Ctrl Pts',(-204.307538596924,-4.70557710135553,
127.394190146963));
#249249=CARTESIAN_POINT('Ctrl Pts',(-204.585986220737,-5.41255236135747,
132.920015464399));
#249250=CARTESIAN_POINT('Ctrl Pts',(-204.864433844549,-1.14565641915494,
136.50165733308));
#249251=CARTESIAN_POINT('Ctrl Pts',(-205.142881468362,4.17404180382362,
134.847761848621));
#249252=CARTESIAN_POINT('Ctrl Pts',(-205.421329092175,5.6579995223666,129.478178163952));
#249253=CARTESIAN_POINT('Ctrl Pts',(-205.699776715988,1.94253208849746,
125.327291366541));
#249254=CARTESIAN_POINT('Ctrl Pts',(-205.978224339801,-3.55802743673226,
126.209563641112));
#249255=CARTESIAN_POINT('Ctrl Pts',(-206.256671963614,-5.78893356690891,
131.314229868733));
#249256=CARTESIAN_POINT('Ctrl Pts',(-206.535119587427,-2.70009255422283,
135.950351163029));
#249257=CARTESIAN_POINT('Ctrl Pts',(-206.81356721124,2.87000160893922,135.857558541658));
#249258=CARTESIAN_POINT('Ctrl Pts',(-207.092014835053,5.80270450085972,
131.121123890489));
#249259=CARTESIAN_POINT('Ctrl Pts',(-207.370462458865,3.40300543436423,
126.09359926625));
#249260=CARTESIAN_POINT('Ctrl Pts',(-207.648910082679,-2.12388938025395,
125.395034190384));
#249261=CARTESIAN_POINT('Ctrl Pts',(-207.927357706491,-5.69903361218359,
129.667375840811));
#249262=CARTESIAN_POINT('Ctrl Pts',(-208.205805330304,-4.03704436778601,
134.984550956282));
#249263=CARTESIAN_POINT('Ctrl Pts',(-208.484252954117,1.33479143002538,
136.460335364123));
#249264=CARTESIAN_POINT('Ctrl Pts',(-208.76270057793,5.48001911182977,132.738555289606));
#249265=CARTESIAN_POINT('Ctrl Pts',(-209.041148201743,4.58937694367963,
127.239344802146));
#249266=CARTESIAN_POINT('Ctrl Pts',(-209.319595825556,-0.518678432184342,
125.016209688352));
#249267=CARTESIAN_POINT('Ctrl Pts',(-209.598043449369,-5.15009366772074,
128.112102511612));
#249268=CARTESIAN_POINT('Ctrl Pts',(-209.876491073182,-5.04882441868487,
133.682049010123));
#249269=CARTESIAN_POINT('Ctrl Pts',(-210.154938696994,-0.307932177662294,
136.607540458767));
#249270=CARTESIAN_POINT('Ctrl Pts',(-210.433386320807,4.71593469130848,
134.200193134443));
#249271=CARTESIAN_POINT('Ctrl Pts',(-210.71183394462,5.40608796518471,128.672241622749));
#249272=CARTESIAN_POINT('Ctrl Pts',(-210.990281568433,1.12831050113542,
125.103603307488));
#249273=CARTESIAN_POINT('Ctrl Pts',(-211.268729192246,-4.18632919242468,
126.773682462711));
#249274=CARTESIAN_POINT('Ctrl Pts',(-211.547176816059,-5.65393687169752,
132.14775793267));
#249275=CARTESIAN_POINT('Ctrl Pts',(-211.825624439872,-1.92585277605142,
136.287316898656));
#249276=CARTESIAN_POINT('Ctrl Pts',(-212.104072063685,3.57199593764717,
135.388306899624));
#249277=CARTESIAN_POINT('Ctrl Pts',(-212.382519687498,5.78735488635066,
130.276874205606));
#249278=CARTESIAN_POINT('Ctrl Pts',(-212.660967311311,2.68441742250212,
125.650175755035));
#249279=CARTESIAN_POINT('Ctrl Pts',(-212.939414935123,-2.88536851154432,
125.759921397201));
#249280=CARTESIAN_POINT('Ctrl Pts',(-213.217862558936,-5.80364174156953,
130.505260248325));
#249281=CARTESIAN_POINT('Ctrl Pts',(-213.496310182749,-3.38865173475374,
135.525457726916));
#249282=CARTESIAN_POINT('Ctrl Pts',(-213.774757806562,2.14034367146046,
136.20719760043));
#249283=CARTESIAN_POINT('Ctrl Pts',(-214.053205430375,5.7024678052036,131.923994229952));
#249284=CARTESIAN_POINT('Ctrl Pts',(-214.331653054188,4.02430260700449,
126.611902266833));
#249285=CARTESIAN_POINT('Ctrl Pts',(-214.610100678001,-1.35200008892003,
125.152474715061));
#249286=CARTESIAN_POINT('Ctrl Pts',(-214.888548301814,-5.48588075200302,
128.886854197714));
#249287=CARTESIAN_POINT('Ctrl Pts',(-215.166995925626,-4.5785050041694,
134.383328404815));
#249288=CARTESIAN_POINT('Ctrl Pts',(-215.445443549439,0.536293170092427,
136.59090605773));
#249289=CARTESIAN_POINT('Ctrl Pts',(-215.723891173253,5.15826412041666,
133.480931139593));
#249290=CARTESIAN_POINT('Ctrl Pts',(-216.002338797065,5.04004233928969,
127.911318669453));
#249291=CARTESIAN_POINT('Ctrl Pts',(-216.280786420879,0.290267868112,125.000270416672));
#249292=CARTESIAN_POINT('Ctrl Pts',(-216.559234044691,-4.72624859348692,
127.422897512942));
#249293=CARTESIAN_POINT('Ctrl Pts',(-216.837681668504,-5.39957348775117,
132.952924008705));
#249294=CARTESIAN_POINT('Ctrl Pts',(-217.116129292317,-1.11095413060172,
136.508525711168));
#249295=CARTESIAN_POINT('Ctrl Pts',(-217.39457691613,4.19857779944424,134.822278356567));
#249296=CARTESIAN_POINT('Ctrl Pts',(-217.673024539943,5.64982184372931,
129.443760886018));
#249297=CARTESIAN_POINT('Ctrl Pts',(-217.951472163756,1.90915562276867,
125.315568099769));
#249298=CARTESIAN_POINT('Ctrl Pts',(-218.229919787568,-3.58593134807924,
126.231307494954));
#249299=CARTESIAN_POINT('Ctrl Pts',(-218.508367411381,-5.78572259252759,
131.349459303753));
#249300=CARTESIAN_POINT('Ctrl Pts',(-218.786815035194,-2.66871742270537,
135.966692049498));
#249301=CARTESIAN_POINT('Ctrl Pts',(-219.065262659007,2.90070868448967,
135.839994403207));
#249302=CARTESIAN_POINT('Ctrl Pts',(-219.34371028282,5.80452521813531,131.085795312298));
#249303=CARTESIAN_POINT('Ctrl Pts',(-219.622157906633,3.37426664313623,
126.07297148578));
#249304=CARTESIAN_POINT('Ctrl Pts',(-219.900605530446,-2.15677813481551,
125.408063130162));
#249305=CARTESIAN_POINT('Ctrl Pts',(-220.179053154259,-5.70584917134113,
129.702088541682));
#249306=CARTESIAN_POINT('Ctrl Pts',(-220.457500778071,-4.01152356563293,
135.009048141953));
#249307=CARTESIAN_POINT('Ctrl Pts',(-220.735948401884,1.36919622307095,
136.452105317718));
#249308=CARTESIAN_POINT('Ctrl Pts',(-221.014396025697,5.49169157172664,
132.705161021709));
#249309=CARTESIAN_POINT('Ctrl Pts',(-221.29284364951,4.56759065001379,127.211474013555));
#249310=CARTESIAN_POINT('Ctrl Pts',(-221.571291273323,-0.553902939853376,
125.019474272218));
#249311=CARTESIAN_POINT('Ctrl Pts',(-221.849738897136,-5.16638678765824,
128.143502474846));
#249312=CARTESIAN_POINT('Ctrl Pts',(-222.128186520948,-5.03121356963114,
133.712729320486));
#249313=CARTESIAN_POINT('Ctrl Pts',(-222.406634144762,-0.272600869560251,
136.609307409853));
#249314=CARTESIAN_POINT('Ctrl Pts',(-222.685081768574,4.73651871234416,
134.171422984523));
#249315=CARTESIAN_POINT('Ctrl Pts',(-222.963529392388,5.39300898940659,
128.639372734101));
#249316=CARTESIAN_POINT('Ctrl Pts',(-223.2419770162,1.09358746834067,125.096840583045));
#249317=CARTESIAN_POINT('Ctrl Pts',(-223.520424640014,-4.21078751141269,
126.799240515859));
#249318=CARTESIAN_POINT('Ctrl Pts',(-223.798872263826,-5.64565447658353,
132.182150161146));
#249319=CARTESIAN_POINT('Ctrl Pts',(-224.077319887639,-1.89244078332859,
136.298938524645));
#249320=CARTESIAN_POINT('Ctrl Pts',(-224.355767511452,3.59983353893359,
135.366478216591));
#249321=CARTESIAN_POINT('Ctrl Pts',(-224.634215135265,5.78403670056078,
130.241654706868));
#249322=CARTESIAN_POINT('Ctrl Pts',(-224.912662759078,2.65299270027449,
125.633930439363));
#249323=CARTESIAN_POINT('Ctrl Pts',(-225.191110382891,-2.91602198566553,
125.77757891607));
#249324=CARTESIAN_POINT('Ctrl Pts',(-225.469558006704,-5.8053549223724,
130.540594204513));
#249325=CARTESIAN_POINT('Ctrl Pts',(-225.748005630516,-3.35985029277391,
135.545997940844));
#249326=CARTESIAN_POINT('Ctrl Pts',(-226.026453254329,2.17319261807209,
136.194068618944));
#249327=CARTESIAN_POINT('Ctrl Pts',(-226.304900878142,5.7091776792716,131.88926094565));
#249328=CARTESIAN_POINT('Ctrl Pts',(-226.583348501955,3.99870736205508,
126.587482871174));
#249329=CARTESIAN_POINT('Ctrl Pts',(-226.861796125768,-1.38637967317499,
125.160809439701));
#249330=CARTESIAN_POINT('Ctrl Pts',(-227.140243749581,-5.49745151716988,
128.920283837883));
#249331=CARTESIAN_POINT('Ctrl Pts',(-227.418691373394,-4.55663398232247,
134.411132754326));
#249332=CARTESIAN_POINT('Ctrl Pts',(-227.697138997207,0.571507578333558,
136.5875342777));
#249333=CARTESIAN_POINT('Ctrl Pts',(-227.97558662102,5.17446159419872,133.44948173115));
#249334=CARTESIAN_POINT('Ctrl Pts',(-228.254034244832,5.02233819149715,
127.880692102567));
#249335=CARTESIAN_POINT('Ctrl Pts',(-228.532481868645,0.254931345670833,
124.998611010119));
#249336=CARTESIAN_POINT('Ctrl Pts',(-228.810929492458,-4.74674495273865,
127.451730180279));
#249337=CARTESIAN_POINT('Ctrl Pts',(-229.089377116271,-5.38639453096373,
132.985752937203));
#249338=CARTESIAN_POINT('Ctrl Pts',(-229.367824740084,-1.07621067523457,
136.515182719319));
#249339=CARTESIAN_POINT('Ctrl Pts',(-229.646272363897,4.22295821522052,
134.796645979094));
#249340=CARTESIAN_POINT('Ctrl Pts',(-229.92471998771,5.64143480886619,129.409394025606));
#249341=CARTESIAN_POINT('Ctrl Pts',(-230.203167611523,1.87570841257552,
125.304048222223));
#249342=CARTESIAN_POINT('Ctrl Pts',(-230.481615235336,-3.61370238142155,
126.25322080496));
#249343=CARTESIAN_POINT('Ctrl Pts',(-230.760062859148,-5.78229722606833,
131.384668539942));
#249344=CARTESIAN_POINT('Ctrl Pts',(-231.038510482961,-2.63724340088164,
135.982841643878));
#249345=CARTESIAN_POINT('Ctrl Pts',(-231.316958106774,2.93130827321233,
135.822243667495));
#249346=CARTESIAN_POINT('Ctrl Pts',(-231.595405730587,5.80613084659478,
131.050456305442));
#249347=CARTESIAN_POINT('Ctrl Pts',(-231.8738533544,3.34540281721704,126.052519028673));
#249348=CARTESIAN_POINT('Ctrl Pts',(-232.152300978213,-2.18958696916944,
125.42129203173));
#249349=CARTESIAN_POINT('Ctrl Pts',(-232.430748602025,-5.71245329815966,
129.736842087648));
#249350=CARTESIAN_POINT('Ctrl Pts',(-232.709196225839,-3.98585411499877,
135.033389521383));
#249351=CARTESIAN_POINT('Ctrl Pts',(-232.987643849651,1.40355028004735,
136.443665992055));
#249352=CARTESIAN_POINT('Ctrl Pts',(-233.266091473464,5.50316053497282,
132.671696318956));
#249353=CARTESIAN_POINT('Ctrl Pts',(-233.544539097277,4.5456351025967,127.183736360699));
#249354=CARTESIAN_POINT('Ctrl Pts',(-233.82298672109,-0.589106922445798,
125.022953217175));
#249355=CARTESIAN_POINT('Ctrl Pts',(-234.101434344904,-5.18248846523346,
128.175001037157));
#249356=CARTESIAN_POINT('Ctrl Pts',(-234.379881968716,-5.01341628710851,
133.743301860178));
#249357=CARTESIAN_POINT('Ctrl Pts',(-234.658329592529,-0.237259460132118,
136.610859256499));
#249358=CARTESIAN_POINT('Ctrl Pts',(-234.936777216342,4.75692721993639,
134.14252806687));
#249359=CARTESIAN_POINT('Ctrl Pts',(-235.215224840155,5.37973017369771,
128.606584069875));
#249360=CARTESIAN_POINT('Ctrl Pts',(-235.493672463967,1.05882391226032,
125.090289352854));
#249361=CARTESIAN_POINT('Ctrl Pts',(-235.772120087781,-4.23508979812022,
126.824946980203));
#249362=CARTESIAN_POINT('Ctrl Pts',(-236.050567711593,-5.63716287966734,
132.216491335124));
#249363=CARTESIAN_POINT('Ctrl Pts',(-236.329015335406,-1.85895866551617,
136.310356547029));
#249364=CARTESIAN_POINT('Ctrl Pts',(-236.607462959219,3.62753774706455,
135.344480482612));
#249365=CARTESIAN_POINT('Ctrl Pts',(-236.885910583032,5.78050418516386,
130.206456059403));
#249366=CARTESIAN_POINT('Ctrl Pts',(-237.164358206845,2.62146967042642,
125.617876715884));
#249367=CARTESIAN_POINT('Ctrl Pts',(-237.442805830658,-2.94656740551997,
125.795422704185));
#249368=CARTESIAN_POINT('Ctrl Pts',(-237.72125345447,-5.80685298361372,
130.575937934662));
#249369=CARTESIAN_POINT('Ctrl Pts',(-237.999701078284,-3.33092435030571,
135.566362451659));
#249370=CARTESIAN_POINT('Ctrl Pts',(-238.278148702096,2.20596103623244,
136.180739919846));
#249371=CARTESIAN_POINT('Ctrl Pts',(-238.55659632591,5.7156759976606,131.854487459968));
#249372=CARTESIAN_POINT('Ctrl Pts',(-238.835043949722,3.97296394353457,
126.56321973347));
#249373=CARTESIAN_POINT('Ctrl Pts',(-239.113491573535,-1.42070788462113,
125.169353288205));
#249374=CARTESIAN_POINT('Ctrl Pts',(-239.391939197348,-5.50881857224844,
128.95378329321));
#249375=CARTESIAN_POINT('Ctrl Pts',(-239.670386821161,-4.53459411272838,
134.438803453569));
#249376=CARTESIAN_POINT('Ctrl Pts',(-239.948834444974,0.606700809151854,
136.583948200045));
#249377=CARTESIAN_POINT('Ctrl Pts',(-240.227282068787,5.1904673264033,133.417934306771));
#249378=CARTESIAN_POINT('Ctrl Pts',(-240.5057296926,5.00444793911587,127.850173873291));
#249379=CARTESIAN_POINT('Ctrl Pts',(-240.784177316413,0.21958537665436,
124.997166737753));
#249380=CARTESIAN_POINT('Ctrl Pts',(-241.062624940225,-4.76706541961049,
127.48068708057));
#249381=CARTESIAN_POINT('Ctrl Pts',(-241.341072564039,-5.37301597934592,
133.018501033406));
#249382=CARTESIAN_POINT('Ctrl Pts',(-241.619520187851,-1.04142734048567,
136.521628110858));
#249383=CARTESIAN_POINT('Ctrl Pts',(-241.897967811664,4.24718214772698,
134.770865666018));
#249384=CARTESIAN_POINT('Ctrl Pts',(-242.176415435477,5.63283872856131,
129.375078856195));
#249385=CARTESIAN_POINT('Ctrl Pts',(-242.45486305929,1.84219169731802,125.292732160775));
#249386=CARTESIAN_POINT('Ctrl Pts',(-242.733310683103,-3.64133950769301,
126.275302759127));
#249387=CARTESIAN_POINT('Ctrl Pts',(-243.011758306915,-5.77865759445851,
131.419856272607));
#249388=CARTESIAN_POINT('Ctrl Pts',(-243.290205930729,-2.60567165503458,
135.998799347738));
#249389=CARTESIAN_POINT('Ctrl Pts',(-243.568653554541,2.96179924122969,
135.80430699228));
#249390=CARTESIAN_POINT('Ctrl Pts',(-243.847101178355,5.80752132674009,
131.015108179419));
#249391=CARTESIAN_POINT('Ctrl Pts',(-244.125548802166,3.31641502616601,
126.032242652805));
#249392=CARTESIAN_POINT('Ctrl Pts',(-244.403996425981,-2.22231466757369,
125.434720404883));
#249393=CARTESIAN_POINT('Ctrl Pts',(-244.682444049792,-5.71884574792013,
129.771635190908));
#249394=CARTESIAN_POINT('Ctrl Pts',(-244.960891673606,-3.96003696707471,
135.05757419259));
#249395=CARTESIAN_POINT('Ctrl Pts',(-245.239339297418,1.43785232795156,
136.435017699859));
#249396=CARTESIAN_POINT('Ctrl Pts',(-245.517786921232,5.51442557658153,
132.638162421391));
#249397=CARTESIAN_POINT('Ctrl Pts',(-245.796234545044,4.52351111499922,
127.156132871406));
#249398=CARTESIAN_POINT('Ctrl Pts',(-246.074682168857,-0.624289075464052,
125.026646394309));
#249399=CARTESIAN_POINT('Ctrl Pts',(-246.353129792671,-5.19839810379266,
128.206597031353));
#249400=CARTESIAN_POINT('Ctrl Pts',(-246.631577416483,-4.99543323060155,
133.773765496319));
#249401=CARTESIAN_POINT('Ctrl Pts',(-246.910025040296,-0.201909258968066,
136.612195941205));
#249402=CARTESIAN_POINT('Ctrl Pts',(-247.188472664109,4.77715945784187,
134.113509452194));
#249403=CARTESIAN_POINT('Ctrl Pts',(-247.466920287922,5.36625201010822,
128.573876845067));
#249404=CARTESIAN_POINT('Ctrl Pts',(-247.745367911734,1.02402112107033,
125.083949859676));
#249405=CARTESIAN_POINT('Ctrl Pts',(-248.023815535548,-4.25923515201858,
126.850800903184));
#249406=CARTESIAN_POINT('Ctrl Pts',(-248.30226315936,-5.62846239560694,
132.250780182078));
#249407=CARTESIAN_POINT('Ctrl Pts',(-248.580710783174,-1.82540766330725,
136.32157054271));
#249408=CARTESIAN_POINT('Ctrl Pts',(-248.859158406986,3.65510753545023,
135.322314512822));
#249409=CARTESIAN_POINT('Ctrl Pts',(-249.137606030799,5.7767574710584,130.171279567513));
#249410=CARTESIAN_POINT('Ctrl Pts',(-249.416053654612,2.58984950105633,
125.602015179472));
#249411=CARTESIAN_POINT('Ctrl Pts',(-249.694501278425,-2.97700363923603,
125.813452100338));
#249412=CARTESIAN_POINT('Ctrl Pts',(-249.972948902238,-5.80813586978118,
130.611290129096));
#249413=CARTESIAN_POINT('Ctrl Pts',(-250.251396526051,-3.30187497921299,
135.586550504748));
#249414=CARTESIAN_POINT('Ctrl Pts',(-250.529844149864,2.23864771169993,
136.167211997028));
#249415=CARTESIAN_POINT('Ctrl Pts',(-250.808291773676,5.72196251956533,
131.819675061465));
#249416=CARTESIAN_POINT('Ctrl Pts',(-251.08673939749,3.94707330538994,126.539113752772));
#249417=CARTESIAN_POINT('Ctrl Pts',(-251.365187021302,-1.45498345124562,
125.178105944033));
#249418=CARTESIAN_POINT('Ctrl Pts',(-251.643634645115,-5.5199814959705,
128.987351322257));
#249419=CARTESIAN_POINT('Ctrl Pts',(-251.922082268928,-4.51238621219265,
134.466339477392));
#249420=CARTESIAN_POINT('Ctrl Pts',(-252.200529892741,0.641871558658502,
136.580147957277));
#249421=CARTESIAN_POINT('Ctrl Pts',(-252.478977516554,5.20628072353487,
133.386290036154));
#249422=CARTESIAN_POINT('Ctrl Pts',(-252.757425140367,4.98637224582674,
127.819765111179));
#249423=CARTESIAN_POINT('Ctrl Pts',(-253.035872764179,0.184231269403876,
124.995937655572));
#249424=CARTESIAN_POINT('Ctrl Pts',(-253.314320387993,-4.78720923844335,
127.509767136124));
#249425=CARTESIAN_POINT('Ctrl Pts',(-253.592768011806,-5.35943833369967,
133.051167092665));
#249426=CARTESIAN_POINT('Ctrl Pts',(-253.871215635618,-1.00660540571931,
136.527861630253));
#249427=CARTESIAN_POINT('Ctrl Pts',(-254.149663259431,4.27124868131666,
134.744938404161));
#249428=CARTESIAN_POINT('Ctrl Pts',(-254.428110883244,5.62403395537261,
129.340816589823));
#249429=CARTESIAN_POINT('Ctrl Pts',(-254.706558507057,1.80860665472018,
125.281620447135));
#249430=CARTESIAN_POINT('Ctrl Pts',(-254.98500613087,-3.66884158147516,
126.297552326988));
#249431=CARTESIAN_POINT('Ctrl Pts',(-255.263453754682,-5.77480406163408,
131.45502159855));
#249432=CARTESIAN_POINT('Ctrl Pts',(-255.541901378496,-2.57400292253984,
136.014563813166));
#249433=CARTESIAN_POINT('Ctrl Pts',(-255.820349002309,2.99217964199006,
135.78618647082));
#249434=CARTESIAN_POINT('Ctrl Pts',(-256.098796626121,5.80869814913581,
130.979749546569));
#249435=CARTESIAN_POINT('Ctrl Pts',(-256.377244249934,3.28730143236016,
126.01214820295));
#249436=CARTESIAN_POINT('Ctrl Pts',(-256.655691873747,-2.25495451926359,
125.448338134603));
#249437=CARTESIAN_POINT('Ctrl Pts',(-256.93413949756,-5.72503666514098,
129.806484721847));
#249438=CARTESIAN_POINT('Ctrl Pts',(-257.212587121373,-3.93405347634203,
135.081566970265));
#249439=CARTESIAN_POINT('Ctrl Pts',(-257.491034745186,1.47206408278265,
136.426225506557));
#249440=CARTESIAN_POINT('Ctrl Pts',(-257.769482368999,5.52555616721843,
132.604438319186));
#249441=CARTESIAN_POINT('Ctrl Pts',(-258.047929992812,4.50108754276566,
127.128895412351));
#249442=CARTESIAN_POINT('Ctrl Pts',(-258.326377616624,-0.659198908970111,
125.030117734768));
#249443=CARTESIAN_POINT('Ctrl Pts',(-258.604825240438,-5.21458571703409,
128.239112839452));
#249444=CARTESIAN_POINT('Ctrl Pts',(-258.883272864251,-4.97637574492231,
133.802560593787));
#249445=CARTESIAN_POINT('Ctrl Pts',(-259.161720488063,-0.168236736403017,
136.616288572087));
#249446=CARTESIAN_POINT('Ctrl Pts',(-259.440168111876,4.80044487344316,
134.078525892203));
#249447=CARTESIAN_POINT('Ctrl Pts',(-259.672207798387,5.25516631655033,
129.4749169549));
#249448=CARTESIAN_POINT('Ctrl Pts',(-259.857849473896,3.17366342871357,
126.795179433485));
#249449=CARTESIAN_POINT('Ctrl Pts',(-259.9506752748,1.64266665146648,126.102093112095));
#249450=CARTESIAN_POINT('Ctrl Pts',(-259.997093138402,0.835778587061721,
125.962806053044));
#249451=CARTESIAN_POINT('Ctrl Pts',(210.385579563201,-2.29217962691353,
126.082387726892));
#249452=CARTESIAN_POINT('Ctrl Pts',(210.339169886847,-3.0789974560272,126.464330840008));
#249453=CARTESIAN_POINT('Ctrl Pts',(210.246352273192,-4.44507089109247,
127.629120819077));
#249454=CARTESIAN_POINT('Ctrl Pts',(210.060718784933,-5.78798125627161,
130.996088365878));
#249455=CARTESIAN_POINT('Ctrl Pts',(209.828679098422,-3.95783017776954,
135.586872998689));
#249456=CARTESIAN_POINT('Ctrl Pts',(209.550231474609,1.89393692750204,136.720289837399));
#249457=CARTESIAN_POINT('Ctrl Pts',(209.271783850796,5.99602695027556,132.40812259401));
#249458=CARTESIAN_POINT('Ctrl Pts',(208.993336226983,4.59288360023261,126.626877830413));
#249459=CARTESIAN_POINT('Ctrl Pts',(208.71488860317,-1.03344059257722,124.682062423228));
#249460=CARTESIAN_POINT('Ctrl Pts',(208.436440979357,-5.70873650289865,
128.364647771496));
#249461=CARTESIAN_POINT('Ctrl Pts',(208.157993355544,-5.13869562717284,
134.288517668348));
#249462=CARTESIAN_POINT('Ctrl Pts',(207.879545731732,0.153933173725622,
137.010984097728));
#249463=CARTESIAN_POINT('Ctrl Pts',(207.601098107919,5.30490488755997,134.029672582798));
#249464=CARTESIAN_POINT('Ctrl Pts',(207.322650484106,5.58103410012833,128.084559773234));
#249465=CARTESIAN_POINT('Ctrl Pts',(207.044202860293,0.728409521696789,
124.638756607567));
#249466=CARTESIAN_POINT('Ctrl Pts',(206.76575523648,-4.79355811073501,126.858871164077));
#249467=CARTESIAN_POINT('Ctrl Pts',(206.487307612667,-5.91049575314416,
132.704682504842));
#249468=CARTESIAN_POINT('Ctrl Pts',(206.208859988854,-1.59596820864792,
136.804198957117));
#249469=CARTESIAN_POINT('Ctrl Pts',(205.930412365042,4.1851717387407,135.390152799229));
#249470=CARTESIAN_POINT('Ctrl Pts',(205.651964741228,6.12034565262566,129.76198992389));
#249471=CARTESIAN_POINT('Ctrl Pts',(205.373517117416,2.43121966936229,125.091713591677));
#249472=CARTESIAN_POINT('Ctrl Pts',(205.095069493603,-3.49207776276838,
125.671081434371));
#249473=CARTESIAN_POINT('Ctrl Pts',(204.81662186979,-6.20632667560231,130.96768173473));
#249474=CARTESIAN_POINT('Ctrl Pts',(204.538174245977,-3.21726438559061,
136.114198085604));
#249475=CARTESIAN_POINT('Ctrl Pts',(204.259726622164,2.72830660529182,136.381233108793));
#249476=CARTESIAN_POINT('Ctrl Pts',(203.981278998351,6.16669716267351,131.523394807979));
#249477=CARTESIAN_POINT('Ctrl Pts',(203.702831374538,3.9381942601484,126.004799186432));
#249478=CARTESIAN_POINT('Ctrl Pts',(203.424383750725,-1.909316761502,124.896766062528));
#249479=CARTESIAN_POINT('Ctrl Pts',(203.145936126912,-6.00225896230248,
129.217523725228));
#249480=CARTESIAN_POINT('Ctrl Pts',(202.867488503099,-4.57941839934143,
134.996506974633));
#249481=CARTESIAN_POINT('Ctrl Pts',(202.589040879287,1.05168395343957,136.923112517541));
#249482=CARTESIAN_POINT('Ctrl Pts',(202.310593255474,5.71634013176502,133.226883983125));
#249483=CARTESIAN_POINT('Ctrl Pts',(202.032145631661,5.12795898713612,127.30447482202));
#249484=CARTESIAN_POINT('Ctrl Pts',(201.753698007848,-0.172765951628197,
124.598289728405));
#249485=CARTESIAN_POINT('Ctrl Pts',(201.475250384035,-5.31472742110118,
127.595180598346));
#249486=CARTESIAN_POINT('Ctrl Pts',(201.196802760222,-5.57271402936141,
133.541151128878));
#249487=CARTESIAN_POINT('Ctrl Pts',(200.918355136409,-0.709648686901125,
136.972144879116));
#249488=CARTESIAN_POINT('Ctrl Pts',(200.639907512596,4.80554913058071,134.735246206027));
#249489=CARTESIAN_POINT('Ctrl Pts',(200.361459888783,5.90468206117194,128.886055711564));
#249490=CARTESIAN_POINT('Ctrl Pts',(200.083012264971,1.57770063730838,124.799693711321));
#249491=CARTESIAN_POINT('Ctrl Pts',(199.804564641158,-4.19911059728431,
126.231327253625));
#249492=CARTESIAN_POINT('Ctrl Pts',(199.526117017345,-6.11714433092778,
131.865355052293));
#249493=CARTESIAN_POINT('Ctrl Pts',(199.247669393532,-2.4138212635637,136.524380797905));
#249494=CARTESIAN_POINT('Ctrl Pts',(198.969221769719,3.50768562329156,135.926987436306));
#249495=CARTESIAN_POINT('Ctrl Pts',(198.690774145906,6.20580078231077,130.622150282517));
#249496=CARTESIAN_POINT('Ctrl Pts',(198.412326522093,3.20108819260905,125.484755525167));
#249497=CARTESIAN_POINT('Ctrl Pts',(198.13387889828,-2.74526806424844,125.235817970576));
#249498=CARTESIAN_POINT('Ctrl Pts',(197.855431274468,-6.16885708386238,
130.104099070135));
#249499=CARTESIAN_POINT('Ctrl Pts',(197.576983650655,-3.92356780882929,
135.615886322105));
#249500=CARTESIAN_POINT('Ctrl Pts',(197.298536026841,1.92728860557448,136.706116507701));
#249501=CARTESIAN_POINT('Ctrl Pts',(197.020088403029,6.00706094473797,132.372921347066));
#249502=CARTESIAN_POINT('Ctrl Pts',(196.741640779216,4.56663773692898,126.598295504472));
#249503=CARTESIAN_POINT('Ctrl Pts',(196.463193155403,-1.07030245846182,
124.688838023107));
#249504=CARTESIAN_POINT('Ctrl Pts',(196.184745531591,-5.72368698170812,
128.399247046161));
#249505=CARTESIAN_POINT('Ctrl Pts',(195.906297907777,-5.11728278641862,
134.319837945007));
#249506=CARTESIAN_POINT('Ctrl Pts',(195.627850283965,0.191654296427489,
137.009876920548));
#249507=CARTESIAN_POINT('Ctrl Pts',(195.349402660151,5.32447044368961,133.997349569974));
#249508=CARTESIAN_POINT('Ctrl Pts',(195.070955036339,5.56435836804288,128.050621358318));
#249509=CARTESIAN_POINT('Ctrl Pts',(194.792507412526,0.690872786183208,
124.634444998269));
#249510=CARTESIAN_POINT('Ctrl Pts',(194.514059788713,-4.81749113516689,
126.888119675218));
#249511=CARTESIAN_POINT('Ctrl Pts',(194.2356121649,-5.89881605082435,132.740628459178));
#249512=CARTESIAN_POINT('Ctrl Pts',(193.957164541087,-1.55941718895885,
136.81380168864));
#249513=CARTESIAN_POINT('Ctrl Pts',(193.678716917274,4.21300988779493,135.364592151301));
#249514=CARTESIAN_POINT('Ctrl Pts',(193.400269293461,6.11388669464029,129.724752614155));
#249515=CARTESIAN_POINT('Ctrl Pts',(193.121821669648,2.39640030908087,125.077020090361));
#249516=CARTESIAN_POINT('Ctrl Pts',(192.843374045836,-3.52326088986039,
125.692433714928));
#249517=CARTESIAN_POINT('Ctrl Pts',(192.564926422022,-6.20521745188322,
131.005458431507));
#249518=CARTESIAN_POINT('Ctrl Pts',(192.28647879821,-3.1848823173506,136.133684081248));
#249519=CARTESIAN_POINT('Ctrl Pts',(192.008031174397,2.76220407667619,136.36452181979));
#249520=CARTESIAN_POINT('Ctrl Pts',(191.729583550584,6.17095986540858,131.485843042463));
#249521=CARTESIAN_POINT('Ctrl Pts',(191.451135926771,3.90890500597959,125.980915208923));
#249522=CARTESIAN_POINT('Ctrl Pts',(191.172688302958,-1.94524259331895,
124.908498067517));
#249523=CARTESIAN_POINT('Ctrl Pts',(190.894240679145,-6.01180727974115,
129.254090580708));
#249524=CARTESIAN_POINT('Ctrl Pts',(190.615793055332,-4.5538147691942,135.024305522869));
#249525=CARTESIAN_POINT('Ctrl Pts',(190.337345431519,1.08891104802307,136.916597252826));
#249526=CARTESIAN_POINT('Ctrl Pts',(190.058897807707,5.73098080836918,133.192042114338));
#249527=CARTESIAN_POINT('Ctrl Pts',(189.780450183893,5.10655917980125,127.273324325042));
#249528=CARTESIAN_POINT('Ctrl Pts',(189.502002560081,-0.210540865719208,
124.599456387862));
#249529=CARTESIAN_POINT('Ctrl Pts',(189.223554936268,-5.33416414113684,
127.627592311355));
#249530=CARTESIAN_POINT('Ctrl Pts',(188.945107312455,-5.55595115925501,
133.575023114497));
#249531=CARTESIAN_POINT('Ctrl Pts',(188.666659688642,-0.672090485321342,
136.976350437346));
#249532=CARTESIAN_POINT('Ctrl Pts',(188.388212064829,4.82938851117716,134.705920634282));
#249533=CARTESIAN_POINT('Ctrl Pts',(188.109764441016,5.89289539464864,128.850147777659));
#249534=CARTESIAN_POINT('Ctrl Pts',(187.831316817203,1.54111929438253,124.790201052305));
#249535=CARTESIAN_POINT('Ctrl Pts',(187.552869193391,-4.22687014955807,
126.256973159398));
#249536=CARTESIAN_POINT('Ctrl Pts',(187.274421569578,-6.11057242014135,
131.902572188318));
#249537=CARTESIAN_POINT('Ctrl Pts',(186.995973945765,-2.37895715467313,
136.538968434335));
#249538=CARTESIAN_POINT('Ctrl Pts',(186.717526321952,3.53880351742172,135.905540247907));
#249539=CARTESIAN_POINT('Ctrl Pts',(186.439078698139,6.20457663716883,130.584377187674));
#249540=CARTESIAN_POINT('Ctrl Pts',(186.160631074326,3.16864693777749,125.465368152723));
#249541=CARTESIAN_POINT('Ctrl Pts',(185.882183450513,-2.77911450042273,
125.25263236868));
#249542=CARTESIAN_POINT('Ctrl Pts',(185.6037358267,-6.17300548002561,130.14166362836));
#249543=CARTESIAN_POINT('Ctrl Pts',(185.325288202887,-3.89420599156785,
135.639681046572));
#249544=CARTESIAN_POINT('Ctrl Pts',(185.046840579075,1.96317856060187,136.694275209062));
#249545=CARTESIAN_POINT('Ctrl Pts',(184.768392955261,6.0164979221829,132.336325600291));
#249546=CARTESIAN_POINT('Ctrl Pts',(184.489945331449,4.54094961554151,126.570575013045));
#249547=CARTESIAN_POINT('Ctrl Pts',(184.211497707636,-1.10750955006109,
124.695466564429));
#249548=CARTESIAN_POINT('Ctrl Pts',(183.933050083823,-5.73822154400692,
128.434133314579));
#249549=CARTESIAN_POINT('Ctrl Pts',(183.65460246001,-5.09578826671723,134.350923164133));
#249550=CARTESIAN_POINT('Ctrl Pts',(183.376154836197,0.229425484589131,
137.008595292604));
#249551=CARTESIAN_POINT('Ctrl Pts',(183.097707212384,5.34380842361613,133.964878848429));
#249552=CARTESIAN_POINT('Ctrl Pts',(182.819259588571,5.54749248089459,128.016800549989));
#249553=CARTESIAN_POINT('Ctrl Pts',(182.540811964758,0.653301958305029,
124.630353773773));
#249554=CARTESIAN_POINT('Ctrl Pts',(182.262364340946,-4.84124114839195,
126.917517669999));
#249555=CARTESIAN_POINT('Ctrl Pts',(181.983916717133,-5.88692014749505,
132.776500352206));
#249556=CARTESIAN_POINT('Ctrl Pts',(181.70546909332,-1.52280712308763,136.82318296266));
#249557=CARTESIAN_POINT('Ctrl Pts',(181.427021469507,4.24069125417353,135.33886187379));
#249558=CARTESIAN_POINT('Ctrl Pts',(181.148573845694,6.10720153813428,129.687555653153));
#249559=CARTESIAN_POINT('Ctrl Pts',(180.870126221881,2.36149196193127,125.062538635854));
#249560=CARTESIAN_POINT('Ctrl Pts',(180.591678598068,-3.55431336199069,
125.713975516152));
#249561=CARTESIAN_POINT('Ctrl Pts',(180.313230974255,-6.20387834410407,
131.04322762551));
#249562=CARTESIAN_POINT('Ctrl Pts',(180.034783350442,-3.15238220429199,
136.15297262387));
#249563=CARTESIAN_POINT('Ctrl Pts',(179.75633572663,2.79599917883219,136.347604482659));
#249564=CARTESIAN_POINT('Ctrl Pts',(179.477888102817,6.17499390876314,131.448266031944));
#249565=CARTESIAN_POINT('Ctrl Pts',(179.199440479004,3.8794709017638,125.957209961944));
#249566=CARTESIAN_POINT('Ctrl Pts',(178.920992855191,-1.98109634126673,
124.920448547985));
#249567=CARTESIAN_POINT('Ctrl Pts',(178.642545231378,-6.02113282860982,
129.290714880887));
#249568=CARTESIAN_POINT('Ctrl Pts',(178.364097607565,-4.52804239515191,
135.051947700091));
#249569=CARTESIAN_POINT('Ctrl Pts',(178.085649983752,1.12609779228193,136.909855496619));
#249570=CARTESIAN_POINT('Ctrl Pts',(177.807202359939,5.74540912154417,133.157111769304));
#249571=CARTESIAN_POINT('Ctrl Pts',(177.528754736127,5.08497014694685,127.242304671825));
#249572=CARTESIAN_POINT('Ctrl Pts',(177.250307112313,-0.248307978092709,
124.600852972375));
#249573=CARTESIAN_POINT('Ctrl Pts',(176.971859488501,-5.35340320178418,
127.660121740658));
#249574=CARTESIAN_POINT('Ctrl Pts',(176.693411864688,-5.53898241132168,
133.608792432211));
#249575=CARTESIAN_POINT('Ctrl Pts',(176.414964240875,-0.634507379188621,
136.980327290216));
#249576=CARTESIAN_POINT('Ctrl Pts',(176.136516617062,4.85304893701009,134.676450488799));
#249577=CARTESIAN_POINT('Ctrl Pts',(175.858068993249,5.88089036471739,128.814312257825));
#249578=CARTESIAN_POINT('Ctrl Pts',(175.579621369436,1.50448084471559,124.780931250186));
#249579=CARTESIAN_POINT('Ctrl Pts',(175.301173745623,-4.25447307360455,
126.282787570284));
#249580=CARTESIAN_POINT('Ctrl Pts',(175.02272612181,-6.10377407984646,131.939748629711));
#249581=CARTESIAN_POINT('Ctrl Pts',(174.744278497998,-2.34400489265046,
136.553343572764));
#249582=CARTESIAN_POINT('Ctrl Pts',(174.465830874185,3.56979027988629,135.883904033421));
#249583=CARTESIAN_POINT('Ctrl Pts',(174.187383250372,6.20312257915782,130.546612244398));
#249584=CARTESIAN_POINT('Ctrl Pts',(173.908935626559,3.13608826756835,125.446178618609));
#249585=CARTESIAN_POINT('Ctrl Pts',(173.630488002746,-2.81285795548731,
125.269652488117));
#249586=CARTESIAN_POINT('Ctrl Pts',(173.352040378933,-6.17692513320066,
130.179252743065));
#249587=CARTESIAN_POINT('Ctrl Pts',(173.07359275512,-3.86469987307124,135.663296596462));
#249588=CARTESIAN_POINT('Ctrl Pts',(172.795145131307,1.99899576932572,136.682215657471));
#249589=CARTESIAN_POINT('Ctrl Pts',(172.516697507494,6.02571195608475,132.29967308599));
#249590=CARTESIAN_POINT('Ctrl Pts',(172.238249883681,4.51509322759614,126.543011406101));
#249591=CARTESIAN_POINT('Ctrl Pts',(171.959802259869,-1.14467560248665,
124.702321473066));
#249592=CARTESIAN_POINT('Ctrl Pts',(171.681354636056,-5.75254347439624,
128.469107412642));
#249593=CARTESIAN_POINT('Ctrl Pts',(171.402907012243,-5.07410492070761,
134.38187696408));
#249594=CARTESIAN_POINT('Ctrl Pts',(171.12445938843,0.267188171305193,137.007083764462));
#249595=CARTESIAN_POINT('Ctrl Pts',(170.846011764617,5.36294838675633,133.932291012718));
#249596=CARTESIAN_POINT('Ctrl Pts',(170.567564140804,5.53042102937231,127.983083035723));
#249597=CARTESIAN_POINT('Ctrl Pts',(170.289116516991,0.615706922082464,
124.62649132937));
#249598=CARTESIAN_POINT('Ctrl Pts',(170.010668893178,-4.86481176764585,
126.947059693175));
#249599=CARTESIAN_POINT('Ctrl Pts',(169.732221269365,-5.87480610217478,
132.812299166869));
#249600=CARTESIAN_POINT('Ctrl Pts',(169.453773645553,-1.48614062903852,
136.832341207004));
#249601=CARTESIAN_POINT('Ctrl Pts',(169.17532602174,4.26821548017818,135.312963568669));
#249602=CARTESIAN_POINT('Ctrl Pts',(168.896878397927,6.10029007702938,129.650400075769));
#249603=CARTESIAN_POINT('Ctrl Pts',(168.618430774114,2.32649610882855,125.048269946673));
#249604=CARTESIAN_POINT('Ctrl Pts',(168.339983150301,-3.58523412773234,
125.735705943466));
#249605=CARTESIAN_POINT('Ctrl Pts',(168.061535526488,-6.2023093493314,131.08098796821));
#249606=CARTESIAN_POINT('Ctrl Pts',(167.783087902675,-3.11976527855146,
136.172062971709));
#249607=CARTESIAN_POINT('Ctrl Pts',(167.504640278862,2.82969067421049,136.330481738588));
#249608=CARTESIAN_POINT('Ctrl Pts',(167.22619265505,6.17879913544756,131.410665161273));
#249609=CARTESIAN_POINT('Ctrl Pts',(166.947745031236,3.84989304232704,125.933684327914));
#249610=CARTESIAN_POINT('Ctrl Pts',(166.669297407424,-2.01687667896098,
124.93261705898));
#249611=CARTESIAN_POINT('Ctrl Pts',(166.39084978361,-6.03023526218728,129.327395269766));
#249612=CARTESIAN_POINT('Ctrl Pts',(166.112402159798,-4.50210223283349,
135.079432481411));
#249613=CARTESIAN_POINT('Ctrl Pts',(165.833954535985,1.16324280857304,136.902887499053));
#249614=CARTESIAN_POINT('Ctrl Pts',(165.555506912173,5.75962453647134,133.122094242209));
#249615=CARTESIAN_POINT('Ctrl Pts',(165.277059288359,5.06319268865361,127.2114170119));
#249616=CARTESIAN_POINT('Ctrl Pts',(164.998611664547,-0.286065889322858,
124.602479430144));
#249617=CARTESIAN_POINT('Ctrl Pts',(164.720164040733,-5.37244389010723,
127.692767680889));
#249618=CARTESIAN_POINT('Ctrl Pts',(164.441716416921,-5.52180841435808,
133.642457830674));
#249619=CARTESIAN_POINT('Ctrl Pts',(164.163268793108,-0.596900761151562,
136.984075290369));
#249620=CARTESIAN_POINT('Ctrl Pts',(163.884821169295,4.87652953132996,134.646836861603));
#249621=CARTESIAN_POINT('Ctrl Pts',(163.606373545482,5.86866741623098,128.778550479967));
#249622=CARTESIAN_POINT('Ctrl Pts',(163.327925921669,1.46778664595768,124.771884648456));
#249623=CARTESIAN_POINT('Ctrl Pts',(163.049478297856,-4.28191834658676,
126.308769529723));
#249624=CARTESIAN_POINT('Ctrl Pts',(162.771030674043,-6.09674956195837,
131.976882998882));
#249625=CARTESIAN_POINT('Ctrl Pts',(162.49258305023,-2.30896577266445,136.567505680515));
#249626=CARTESIAN_POINT('Ctrl Pts',(162.214135426418,3.60064476245918,135.862079594585));
#249627=CARTESIAN_POINT('Ctrl Pts',(161.935687802605,6.20143866215845,130.508856852083));
#249628=CARTESIAN_POINT('Ctrl Pts',(161.657240178792,3.10341338845521,125.427187633898));
#249629=CARTESIAN_POINT('Ctrl Pts',(161.378792554979,-2.84649717906582,
125.2868776982));
#249630=CARTESIAN_POINT('Ctrl Pts',(161.100344931166,-6.18061589814333,
130.216865021372));
#249631=CARTESIAN_POINT('Ctrl Pts',(160.821897307353,-3.83505054669964,
135.686732096692));
#249632=CARTESIAN_POINT('Ctrl Pts',(160.54344968354,2.0347389045262,136.6699382998));
#249633=CARTESIAN_POINT('Ctrl Pts',(160.265002059727,6.03470270501411,132.262965162335));
#249634=CARTESIAN_POINT('Ctrl Pts',(159.986554435914,4.48906953121078,126.51560570502));
#249635=CARTESIAN_POINT('Ctrl Pts',(159.708106812101,-1.18179923853688,
124.709402495009));
#249636=CARTESIAN_POINT('Ctrl Pts',(159.429659188289,-5.76665224217155,
128.50416804437));
#249637=CARTESIAN_POINT('Ctrl Pts',(159.151211564475,-5.05223355187421,
134.412698197843));
#249638=CARTESIAN_POINT('Ctrl Pts',(158.872763940663,0.304940957265202,
137.005342392132));
#249639=CARTESIAN_POINT('Ctrl Pts',(158.59431631685,5.38188962387183,133.899587270395));
#249640=CARTESIAN_POINT('Ctrl Pts',(158.315868693037,5.51314464606502,127.949470064936));
#249641=CARTESIAN_POINT('Ctrl Pts',(158.037421069224,0.57808907061355,124.622857808186));
#249642=CARTESIAN_POINT('Ctrl Pts',(157.758973445411,-4.88820211951067,
126.976744650055));
#249643=CARTESIAN_POINT('Ctrl Pts',(157.480525821598,-5.86247436375394,
132.848023576631));
#249644=CARTESIAN_POINT('Ctrl Pts',(157.202078197785,-1.44941906550188,
136.841276082311));
#249645=CARTESIAN_POINT('Ctrl Pts',(156.923630573973,4.29558154588865,135.286898195607));
#249646=CARTESIAN_POINT('Ctrl Pts',(156.645182950159,6.09315256743229,129.613287258817));
#249647=CARTESIAN_POINT('Ctrl Pts',(156.366735326347,2.29141404655692,125.034214551549));
#249648=CARTESIAN_POINT('Ctrl Pts',(156.088287702534,-3.61602204130483,
125.757624191644));
#249649=CARTESIAN_POINT('Ctrl Pts',(155.809840078721,-6.2005105257049,131.11873806038));
#249650=CARTESIAN_POINT('Ctrl Pts',(155.531392454908,-3.08703274876129,
136.190954417361));
#249651=CARTESIAN_POINT('Ctrl Pts',(155.252944831095,2.86327731436015,136.313154222067));
#249652=CARTESIAN_POINT('Ctrl Pts',(154.974497207282,6.18237540445775,131.373041823765));
#249653=CARTESIAN_POINT('Ctrl Pts',(154.696049583469,3.82017252368788,125.910339178587));
#249654=CARTESIAN_POINT('Ctrl Pts',(154.417601959656,-2.05258228054818,
124.945003149591));
#249655=CARTESIAN_POINT('Ctrl Pts',(154.139154335844,-6.03911424317947,
129.364130388138));
#249656=CARTESIAN_POINT('Ctrl Pts',(153.860706712031,-4.47599524346119,
135.106758848372));
#249657=CARTESIAN_POINT('Ctrl Pts',(153.582259088218,1.20034472047403,136.895693518332));
#249658=CARTESIAN_POINT('Ctrl Pts',(153.303811464405,5.77362652639317,133.086990830643));
#249659=CARTESIAN_POINT('Ctrl Pts',(153.025363840592,5.04122761189337,127.180662489822));
#249660=CARTESIAN_POINT('Ctrl Pts',(152.746916216779,-0.323813200276178,
124.604335700902));
#249661=CARTESIAN_POINT('Ctrl Pts',(152.468468592966,-5.39128550054617,
127.725528922339));
#249662=CARTESIAN_POINT('Ctrl Pts',(152.190020969154,-5.5044298047531,133.6760180624));
#249663=CARTESIAN_POINT('Ctrl Pts',(151.91157334534,-0.55927202473736,136.987594298923));
#249664=CARTESIAN_POINT('Ctrl Pts',(151.633125721528,4.89982942405471,134.617080850036));
#249665=CARTESIAN_POINT('Ctrl Pts',(151.354678097715,5.85622700211526,128.742863769248));
#249666=CARTESIAN_POINT('Ctrl Pts',(151.076230473902,1.43103805782584,124.763061582343));
#249667=CARTESIAN_POINT('Ctrl Pts',(150.797782850089,-4.3092049515099,126.334918074943));
#249668=CARTESIAN_POINT('Ctrl Pts',(150.519335226276,-6.0894991267732,132.013973919806));
#249669=CARTESIAN_POINT('Ctrl Pts',(150.240887602463,-2.27384109310269,
136.581454232806));
#249670=CARTESIAN_POINT('Ctrl Pts',(149.96243997865,3.63136582181627,135.840067740113));
#249671=CARTESIAN_POINT('Ctrl Pts',(149.683992354837,6.19952494856889,130.471112409769));
#249672=CARTESIAN_POINT('Ctrl Pts',(149.405544731024,3.0706235112177,125.40839590231));
#249673=CARTESIAN_POINT('Ctrl Pts',(149.127097107212,-2.88003092464457,
125.30430736064));
#249674=CARTESIAN_POINT('Ctrl Pts',(148.848649483398,-6.18407763809098,
130.254499069545));
#249675=CARTESIAN_POINT('Ctrl Pts',(148.570201859586,-3.80525911111971,
135.709986678852));
#249676=CARTESIAN_POINT('Ctrl Pts',(148.291754235773,2.07040664172831,136.657443590992));
#249677=CARTESIAN_POINT('Ctrl Pts',(148.01330661196,6.04346983581547,132.226203189553));
#249678=CARTESIAN_POINT('Ctrl Pts',(147.734858988147,4.46287949070312,126.488358925329));
#249679=CARTESIAN_POINT('Ctrl Pts',(147.456411364334,-1.21887908258166,
124.716709367866));
#249680=CARTESIAN_POINT('Ctrl Pts',(147.177963740522,-5.78054732452736,
128.53931391058));
#249681=CARTESIAN_POINT('Ctrl Pts',(146.899516116708,-5.03017497066859,
134.44338572333));
#249682=CARTESIAN_POINT('Ctrl Pts',(146.621068492896,0.342682443525903,
137.003371240143));
#249683=CARTESIAN_POINT('Ctrl Pts',(146.342620869082,5.40063143308812,133.866768833311));
#249684=CARTESIAN_POINT('Ctrl Pts',(146.06417324527,5.49566397115542,127.915962883168));
#249685=CARTESIAN_POINT('Ctrl Pts',(145.785725621457,0.540449797841529,
124.619453344862));
#249686=CARTESIAN_POINT('Ctrl Pts',(145.507277997644,-4.91141133724831,
127.006571440652));
#249687=CARTESIAN_POINT('Ctrl Pts',(145.228830373831,-5.84992538918966,
132.883672257711));
#249688=CARTESIAN_POINT('Ctrl Pts',(144.950382750018,-1.41264379320865,
136.849987257496));
#249689=CARTESIAN_POINT('Ctrl Pts',(144.671935126205,4.32278843724517,135.260666720466));
#249690=CARTESIAN_POINT('Ctrl Pts',(144.393487502392,6.08578927382608,129.576218577526));
#249691=CARTESIAN_POINT('Ctrl Pts',(144.11503987858,2.25624707509518,125.020372971309));
#249692=CARTESIAN_POINT('Ctrl Pts',(143.836592254767,-3.64667596185081,
125.779729448496));
#249693=CARTESIAN_POINT('Ctrl Pts',(143.558144630954,-6.19848193988065,
131.156476503179));
#249694=CARTESIAN_POINT('Ctrl Pts',(143.279697007141,-3.05418582783736,
136.209646260801));
#249695=CARTESIAN_POINT('Ctrl Pts',(143.001249383328,2.89675785471595,136.295622575173));
#249696=CARTESIAN_POINT('Ctrl Pts',(142.722801759515,6.18572258327378,131.335397413564));
#249697=CARTESIAN_POINT('Ctrl Pts',(142.444354135702,3.79031044715096,125.887175379022));
#249698=CARTESIAN_POINT('Ctrl Pts',(142.165906511889,-2.0882118229442,124.957606360848));
#249699=CARTESIAN_POINT('Ctrl Pts',(141.887458888076,-6.04776944257254,
129.400918874772));
#249700=CARTESIAN_POINT('Ctrl Pts',(141.609011264264,-4.44972239443904,
135.133925788383));
#249701=CARTESIAN_POINT('Ctrl Pts',(141.33056364045,1.2374021531599,136.888273821029));
#249702=CARTESIAN_POINT('Ctrl Pts',(141.052116016638,5.78741457246075,133.051802835376));
#249703=CARTESIAN_POINT('Ctrl Pts',(140.773668392825,5.01907573059014,127.15004224521));
#249704=CARTESIAN_POINT('Ctrl Pts',(140.495220769012,-0.361548512212229,
124.606421715863));
#249705=CARTESIAN_POINT('Ctrl Pts',(140.216773145199,-5.4099273349182,127.758404251031));
#249706=CARTESIAN_POINT('Ctrl Pts',(139.938325521386,-5.48684722647749,
133.709471883804));
#249707=CARTESIAN_POINT('Ctrl Pts',(139.659877897573,-0.521622564292735,
136.990884185479));
#249708=CARTESIAN_POINT('Ctrl Pts',(139.38143027376,4.92294775179823,134.58718355672));
#249709=CARTESIAN_POINT('Ctrl Pts',(139.102982649947,5.84356958335437,128.707253448052));
#249710=CARTESIAN_POINT('Ctrl Pts',(138.824535026135,1.39423644205237,124.754462378786));
#249711=CARTESIAN_POINT('Ctrl Pts',(138.546087402322,-4.33633187725888,
126.361232236999));
#249712=CARTESIAN_POINT('Ctrl Pts',(138.267639778509,-6.08202304295846,
132.051020018064));
#249713=CARTESIAN_POINT('Ctrl Pts',(137.989192154696,-2.23863215552307,
136.595188712768));
#249714=CARTESIAN_POINT('Ctrl Pts',(137.710744530883,3.66195231957746,135.817869285661));
#249715=CARTESIAN_POINT('Ctrl Pts',(137.43229690707,6.19738150930245,130.433380316089));
#249716=CARTESIAN_POINT('Ctrl Pts',(137.153849283257,3.03771985089675,125.389804120178));
#249717=CARTESIAN_POINT('Ctrl Pts',(136.875401659444,-2.91345794961824,
125.321940829576));
#249718=CARTESIAN_POINT('Ctrl Pts',(136.596954035631,-6.1873102247676,130.29215349304));
#249719=CARTESIAN_POINT('Ctrl Pts',(136.318506411819,-3.77532667026395,
135.733059481234));
#249720=CARTESIAN_POINT('Ctrl Pts',(136.040058788006,2.10599765925102,136.644731994041));
#249721=CARTESIAN_POINT('Ctrl Pts',(135.761611164193,6.05201302361958,132.189388529871));
#249722=CARTESIAN_POINT('Ctrl Pts',(135.48316354038,4.4365240765547,126.461272076668));
#249723=CARTESIAN_POINT('Ctrl Pts',(135.204715916567,-1.25591376061384,
124.724241820878));
#249724=CARTESIAN_POINT('Ctrl Pts',(134.926268292754,-5.79422820657625,
128.574543708929));
#249725=CARTESIAN_POINT('Ctrl Pts',(134.647820668941,-5.00792999447956,
134.473938403405));
#249726=CARTESIAN_POINT('Ctrl Pts',(134.369373045128,0.380411231562576,
137.001170381535));
#249727=CARTESIAN_POINT('Ctrl Pts',(134.090925421316,5.41917311992063,133.833836917565));
#249728=CARTESIAN_POINT('Ctrl Pts',(133.812477797503,5.4779796523963,127.88256273204));
#249729=CARTESIAN_POINT('Ctrl Pts',(133.53403017369,0.502790498503515,124.616278065551));
#249730=CARTESIAN_POINT('Ctrl Pts',(133.255582549877,-4.93443856083268,
127.036538959725));
#249731=CARTESIAN_POINT('Ctrl Pts',(132.977134926064,-5.83715964348875,
132.919243889133));
#249732=CARTESIAN_POINT('Ctrl Pts',(132.698687302251,-1.37581617488021,
136.858474409763));
#249733=CARTESIAN_POINT('Ctrl Pts',(132.420239678438,4.34983514608645,135.234270115264));
#249734=CARTESIAN_POINT('Ctrl Pts',(132.141792054625,6.07820046906025,129.539195405491));
#249735=CARTESIAN_POINT('Ctrl Pts',(131.863344430812,2.22099649756843,125.006745718858));
#249736=CARTESIAN_POINT('Ctrl Pts',(131.584896806999,-3.67719475347803,
125.802020894903));
#249737=CARTESIAN_POINT('Ctrl Pts',(131.306449183186,-6.1962236670286,131.194201898194));
#249738=CARTESIAN_POINT('Ctrl Pts',(131.028001559374,-3.02122573293442,
136.228137809392));
#249739=CARTESIAN_POINT('Ctrl Pts',(130.749553935561,2.93013105464412,136.277887447547));
#249740=CARTESIAN_POINT('Ctrl Pts',(130.471106311748,6.18884054786473,131.2977333256));
#249741=CARTESIAN_POINT('Ctrl Pts',(130.192658687935,3.76030791926647,125.864193787566));
#249742=CARTESIAN_POINT('Ctrl Pts',(129.914211064122,-2.12376398588317,
124.970426225734));
#249743=CARTESIAN_POINT('Ctrl Pts',(129.635763440309,-6.05620053964477,
129.437759366456));
#249744=CARTESIAN_POINT('Ctrl Pts',(129.357315816496,-4.42328465931731,
135.160932294765));
#249745=CARTESIAN_POINT('Ctrl Pts',(129.078868192683,1.27441373345414,136.880628682086));
#249746=CARTESIAN_POINT('Ctrl Pts',(128.800420568871,5.80098816375315,133.01653156031));
#249747=CARTESIAN_POINT('Ctrl Pts',(128.521972945058,4.99673786558976,127.11955741271));
#249748=CARTESIAN_POINT('Ctrl Pts',(128.243525321245,-0.399270426835251,
124.608737397728));
#249749=CARTESIAN_POINT('Ctrl Pts',(127.965077697432,-5.42836870244348,
127.791392448756));
#249750=CARTESIAN_POINT('Ctrl Pts',(127.686630073619,-5.46906133106002,
133.742818055242));
#249751=CARTESIAN_POINT('Ctrl Pts',(127.408182449806,-0.483953774931917,
136.993944828129));
#249752=CARTESIAN_POINT('Ctrl Pts',(127.129734825993,4.9458836579024,134.557146089508));
#249753=CARTESIAN_POINT('Ctrl Pts',(126.85128720218,5.8306956289736,128.671720835934));
#249754=CARTESIAN_POINT('Ctrl Pts',(126.572839578367,1.35738316233494,124.746087356435));
#249755=CARTESIAN_POINT('Ctrl Pts',(126.294391954555,-4.36329811863544,
126.387711040812));
#249756=CARTESIAN_POINT('Ctrl Pts',(126.015944330741,-6.07432158754323,
132.088019920899));
#249757=CARTESIAN_POINT('Ctrl Pts',(125.737496706929,-2.20334026460562,
136.608708611466));
#249758=CARTESIAN_POINT('Ctrl Pts',(125.459049083116,3.69240312234872,135.795485053802));
#249759=CARTESIAN_POINT('Ctrl Pts',(125.180601459303,6.19500842378515,130.39566196922));
#249760=CARTESIAN_POINT('Ctrl Pts',(124.90215383549,3.00470362674961,125.371412976429));
#249761=CARTESIAN_POINT('Ctrl Pts',(124.623706211677,-2.9467770153362,125.339777451594));
#249762=CARTESIAN_POINT('Ctrl Pts',(124.345258587864,-6.19031353838844,
130.329826896558));
#249763=CARTESIAN_POINT('Ctrl Pts',(124.066810964051,-3.74525433329013,
135.755949648866));
#249764=CARTESIAN_POINT('Ctrl Pts',(123.788363340238,2.14151063825588,136.631803979981));
#249765=CARTESIAN_POINT('Ctrl Pts',(123.509915716426,6.0603319518555,132.152522547471));
#249766=CARTESIAN_POINT('Ctrl Pts',(123.231468092613,4.4100042653751,126.43434616275));
#249767=CARTESIAN_POINT('Ctrl Pts',(122.9530204688,-1.29290190029971,124.731999574929));
#249768=CARTESIAN_POINT('Ctrl Pts',(122.674572844987,-5.80769438136815,
128.609856133963));
#249769=CARTESIAN_POINT('Ctrl Pts',(122.396125221174,-4.98549944760296,
134.504355105923));
#249770=CARTESIAN_POINT('Ctrl Pts',(122.117677597361,0.418125923321227,
136.998739897863));
#249771=CARTESIAN_POINT('Ctrl Pts',(121.839229973548,5.43751399730024,133.80079274346));
#249772=CARTESIAN_POINT('Ctrl Pts',(121.560782349735,5.46009234508668,127.849270849208));
#249773=CARTESIAN_POINT('Ctrl Pts',(121.282334725922,0.465112568078527,
124.613332087916));
#249774=CARTESIAN_POINT('Ctrl Pts',(121.00388710211,-4.95728293698158,127.066646096814));
#249775=CARTESIAN_POINT('Ctrl Pts',(120.725439478297,-5.82417759969065,
132.954737152777));
#249776=CARTESIAN_POINT('Ctrl Pts',(120.446991854484,-1.33893757517749,
136.866737224615));
#249777=CARTESIAN_POINT('Ctrl Pts',(120.168544230671,4.37672067018674,135.207709358136));
#249778=CARTESIAN_POINT('Ctrl Pts',(119.890096606858,6.07038643434081,129.502219114618));
#249779=CARTESIAN_POINT('Ctrl Pts',(119.611648983045,2.18566362019961,124.993333299159));
#249780=CARTESIAN_POINT('Ctrl Pts',(119.333201359232,-3.7075772853013,125.82449770485));
#249781=CARTESIAN_POINT('Ctrl Pts',(119.054753735419,-6.19373579082994,
131.231912847497));
#249782=CARTESIAN_POINT('Ctrl Pts',(118.776306111606,-2.98815368540088,
136.246428377926));
#249783=CARTESIAN_POINT('Ctrl Pts',(118.497858487794,2.96339567748857,136.259949496373));
#249784=CARTESIAN_POINT('Ctrl Pts',(118.219410863981,6.1917291826932,131.26005095553));
#249785=CARTESIAN_POINT('Ctrl Pts',(117.940963240168,3.73016605178927,125.841395255808));
#249786=CARTESIAN_POINT('Ctrl Pts',(117.662515616355,-2.15923745196658,
124.983462269205));
#249787=CARTESIAN_POINT('Ctrl Pts',(117.384067992542,-6.06440722197891,
129.474650498052));
#249788=CARTESIAN_POINT('Ctrl Pts',(117.105620368729,-4.39668301775581,
135.187777366781));
#249789=CARTESIAN_POINT('Ctrl Pts',(116.827172744916,1.31137808987868,136.872758384795));
#249790=CARTESIAN_POINT('Ctrl Pts',(116.548725121103,5.81434679729579,132.981178312436));
#249791=CARTESIAN_POINT('Ctrl Pts',(116.27027749729,4.97421484463032,127.089209121948));
#249792=CARTESIAN_POINT('Ctrl Pts',(115.991829873478,-0.436977546345769,
124.611282660692));
#249793=CARTESIAN_POINT('Ctrl Pts',(115.713382249665,-5.44660891977013,
127.824492293124));
#249794=CARTESIAN_POINT('Ctrl Pts',(115.434934625852,-5.45107277756375,
133.776055341058));
#249795=CARTESIAN_POINT('Ctrl Pts',(115.156487002039,-0.446267052485976,
136.99677611346));
#249796=CARTESIAN_POINT('Ctrl Pts',(114.878039378226,4.9686362924688,134.526969561451));
#249797=CARTESIAN_POINT('Ctrl Pts',(114.599591754413,5.81760561602206,128.636267249567));
#249798=CARTESIAN_POINT('Ctrl Pts',(114.3211441306,1.32047958428524,124.737936825626));
#249799=CARTESIAN_POINT('Ctrl Pts',(114.042696506787,-4.39010267639563,
126.414353505198));
#249800=CARTESIAN_POINT('Ctrl Pts',(113.764248882975,-6.06639504590774,
132.124972257267));
#249801=CARTESIAN_POINT('Ctrl Pts',(113.485801259161,-2.16796672810439,
136.622013427915));
#249802=CARTESIAN_POINT('Ctrl Pts',(113.207353635349,3.72271710176439,135.772915873991));
#249803=CARTESIAN_POINT('Ctrl Pts',(112.928906011536,6.19240577995249,130.357958766832));
#249804=CARTESIAN_POINT('Ctrl Pts',(112.650458387723,2.97157606220462,125.353223152553));
#249805=CARTESIAN_POINT('Ctrl Pts',(112.37201076391,-2.9799868871482,125.357816565752));
#249806=CARTESIAN_POINT('Ctrl Pts',(112.093563140097,-6.19308746766462,
130.367517884098));
#249807=CARTESIAN_POINT('Ctrl Pts',(111.815115516284,-3.71504321453968,
135.778656333547));
#249808=CARTESIAN_POINT('Ctrl Pts',(111.536667892471,2.1769442627965,136.618660027865));
#249809=CARTESIAN_POINT('Ctrl Pts',(111.258220268658,6.06842631226225,132.115606608435));
#249810=CARTESIAN_POINT('Ctrl Pts',(110.979772644846,4.38332103986566,126.407582181323));
#249811=CARTESIAN_POINT('Ctrl Pts',(110.701325021032,-1.32984213103019,
124.739982342551));
#249812=CARTESIAN_POINT('Ctrl Pts',(110.42287739722,-5.82094534990898,128.645249877167));
#249813=CARTESIAN_POINT('Ctrl Pts',(110.144429773407,-4.96288416121089,
134.534634703787));
#249814=CARTESIAN_POINT('Ctrl Pts',(109.865982149594,0.455825121270016,
136.996079879188));
#249815=CARTESIAN_POINT('Ctrl Pts',(109.587534525781,5.45565338559904,133.767637535461));
#249816=CARTESIAN_POINT('Ctrl Pts',(109.309086901968,5.44200271204727,127.816088468313));
#249817=CARTESIAN_POINT('Ctrl Pts',(109.030639278155,0.427417402736423,
124.610615521118));
#249818=CARTESIAN_POINT('Ctrl Pts',(108.752191654342,-4.97994361918818,
127.096891736289));
#249819=CARTESIAN_POINT('Ctrl Pts',(108.473744030529,-5.81097973884976,
132.990150733429));
#249820=CARTESIAN_POINT('Ctrl Pts',(108.195296406717,-1.30200936065053,
136.874775395874));
#249821=CARTESIAN_POINT('Ctrl Pts',(107.916848782904,4.40344401329306,135.180985433302));
#249822=CARTESIAN_POINT('Ctrl Pts',(107.638401159091,6.06234745921968,129.465291075077));
#249823=CARTESIAN_POINT('Ctrl Pts',(107.359953535278,2.15024975226158,124.980136209215));
#249824=CARTESIAN_POINT('Ctrl Pts',(107.081505911465,-3.73782243148481,
125.847159045447));
#249825=CARTESIAN_POINT('Ctrl Pts',(106.803058287652,-6.19101840347381,
131.269607953695));
#249826=CARTESIAN_POINT('Ctrl Pts',(106.524610663839,-2.95497091073364,
136.264517288637));
#249827=CARTESIAN_POINT('Ctrl Pts',(106.246163040026,2.99655049061638,136.241809386346));
#249828=CARTESIAN_POINT('Ctrl Pts',(105.967715416213,6.1943883807198,131.222351699685));
#249829=CARTESIAN_POINT('Ctrl Pts',(105.689267792401,3.69988596163724,125.818780628557));
#249830=CARTESIAN_POINT('Ctrl Pts',(105.410820168588,-2.19463090671215,
124.996714008204));
#249831=CARTESIAN_POINT('Ctrl Pts',(105.132372544775,-6.07238918547325,
129.511590902545));
#249832=CARTESIAN_POINT('Ctrl Pts',(104.853924920962,-4.36991845548819,
135.214460009678));
#249833=CARTESIAN_POINT('Ctrl Pts',(104.575477297149,1.34829385270585,136.864663220793));
#249834=CARTESIAN_POINT('Ctrl Pts',(104.297029673336,5.82748997807964,132.945744401783));
#249835=CARTESIAN_POINT('Ctrl Pts',(104.018582049523,4.95150750231056,127.058998497491));
#249836=CARTESIAN_POINT('Ctrl Pts',(103.74013442571,-0.474668473492613,
124.614057410436));
#249837=CARTESIAN_POINT('Ctrl Pts',(103.461686801897,-5.46464731100027,
127.857702557609));
#249838=CARTESIAN_POINT('Ctrl Pts',(103.183239178085,-5.43288223256107,
133.809182509633));
#249839=CARTESIAN_POINT('Ctrl Pts',(102.904791554272,-0.408563793450433,
136.999377936557));
#249840=CARTESIAN_POINT('Ctrl Pts',(102.626343930459,4.99120481239017,134.496655090749));
#249841=CARTESIAN_POINT('Ctrl Pts',(102.347896306646,5.80430002955499,128.600894002697));
#249842=CARTESIAN_POINT('Ctrl Pts',(102.069448682833,1.28352707537895,124.730011088381));
#249843=CARTESIAN_POINT('Ctrl Pts',(101.79100105902,-4.41674455728669,126.441158642913));
#249844=CARTESIAN_POINT('Ctrl Pts',(101.512553435207,-6.05824371177293,
132.161875657885));
#249845=CARTESIAN_POINT('Ctrl Pts',(101.234105811394,-2.13251285679878,
136.635102669099));
#249846=CARTESIAN_POINT('Ctrl Pts',(100.955658187581,3.75289313452884,135.750162582539));
#249847=CARTESIAN_POINT('Ctrl Pts',(100.677210563769,6.18957367424645,130.320272106026));
#249848=CARTESIAN_POINT('Ctrl Pts',(100.398762939956,2.93833838481571,125.33523532258));
#249849=CARTESIAN_POINT('Ctrl Pts',(100.120315316143,-3.01308633445025,
125.376057503601));
#249850=CARTESIAN_POINT('Ctrl Pts',(99.8418676923298,-6.19563190980719,
130.405225059005));
#249851=CARTESIAN_POINT('Ctrl Pts',(99.5634200685172,-3.68469443349671,
135.801178693871));
#249852=CARTESIAN_POINT('Ctrl Pts',(99.2849724447041,2.2122972198669,136.605300624745));
#249853=CARTESIAN_POINT('Ctrl Pts',(99.0065248208913,6.07629580490035,132.078642080696));
#249854=CARTESIAN_POINT('Ctrl Pts',(98.7280771970783,4.35647538878314,126.380981124141));
#249855=CARTESIAN_POINT('Ctrl Pts',(98.4496295732656,-1.36673308397146,
124.748189827941));
#249856=CARTESIAN_POINT('Ctrl Pts',(98.1711819494526,-5.8339806211792,128.680723627015));
#249857=CARTESIAN_POINT('Ctrl Pts',(97.8927343256397,-4.94008497332115,
134.564776074971));
#249858=CARTESIAN_POINT('Ctrl Pts',(97.6142867018267,0.493507428451318,
136.993190424079));
#249859=CARTESIAN_POINT('Ctrl Pts',(97.3358390780141,5.47359061265531,133.734372522146));
#249860=CARTESIAN_POINT('Ctrl Pts',(97.0573914542009,5.42371142359607,127.783016818942));
#249861=CARTESIAN_POINT('Ctrl Pts',(96.7789438303882,0.389706399285272,
124.608128465823));
#249862=CARTESIAN_POINT('Ctrl Pts',(96.5004962065753,-5.0024197677526,127.127274757387));
#249863=CARTESIAN_POINT('Ctrl Pts',(96.2220485827623,-5.79756655001767,
133.025483318824));
#249864=CARTESIAN_POINT('Ctrl Pts',(95.9436009589496,-1.26503289968789,
136.882588625681));
#249865=CARTESIAN_POINT('Ctrl Pts',(95.6651533351365,4.4300041851621,135.154099331026));
#249866=CARTESIAN_POINT('Ctrl Pts',(95.3867057113237,6.05408384158403,129.428412655251));
#249867=CARTESIAN_POINT('Ctrl Pts',(95.1082580875108,2.11475620602821,124.967154938047));
#249868=CARTESIAN_POINT('Ctrl Pts',(94.8298104636979,-3.76792907128354,
125.870004076972));
#249869=CARTESIAN_POINT('Ctrl Pts',(94.5513628398851,-6.18807160565406,
131.307285819983));
#249870=CARTESIAN_POINT('Ctrl Pts',(94.2729152160721,-2.92167863853249,
136.282403871234));
#249871=CARTESIAN_POINT('Ctrl Pts',(93.9944675922592,3.02959426546386,136.223467789656));
#249872=CARTESIAN_POINT('Ctrl Pts',(93.7160199684464,6.19681804340696,131.184636955029));
#249873=CARTESIAN_POINT('Ctrl Pts',(93.4375723446334,3.66946877085029,125.796350743805));
#249874=CARTESIAN_POINT('Ctrl Pts',(93.1591247208205,-2.22994303860241,
125.010180951684));
#249875=CARTESIAN_POINT('Ctrl Pts',(92.8806770970077,-6.08014613435319,
129.548579211095));
#249876=CARTESIAN_POINT('Ctrl Pts',(92.6022294731947,-4.3429919642852,135.24097923472));
#249877=CARTESIAN_POINT('Ctrl Pts',(92.323781849382,1.38515965400848,136.856343490049));
#249878=CARTESIAN_POINT('Ctrl Pts',(92.045334225569,5.84041721907928,132.910231141365));
#249879=CARTESIAN_POINT('Ctrl Pts',(91.7668866017561,4.9286166800594,127.028926658805));
#249880=CARTESIAN_POINT('Ctrl Pts',(91.4884389779432,-0.512341811624615,
124.617061544141));
#249881=CARTESIAN_POINT('Ctrl Pts',(91.2099913541303,-5.48248320771468,
127.891022011592));
#249882=CARTESIAN_POINT('Ctrl Pts',(90.9315437303175,-5.41449037010934,
133.842198333429));
#249883=CARTESIAN_POINT('Ctrl Pts',(90.6530961065044,-0.370845394933272,
137.00175020101));
#249884=CARTESIAN_POINT('Ctrl Pts',(90.3746484826917,5.01358838138169,134.466203800718));
#249885=CARTESIAN_POINT('Ctrl Pts',(90.0962008588786,5.79077936261581,128.565602406094));
#249886=CARTESIAN_POINT('Ctrl Pts',(89.817753235066,1.24652700490487,124.722310438393));
#249887=CARTESIAN_POINT('Ctrl Pts',(89.5393056112528,-4.44322277408392,
126.468125460682));
#249888=CARTESIAN_POINT('Ctrl Pts',(89.2608579874402,-6.04986788718945,
132.198728755283));
#249889=CARTESIAN_POINT('Ctrl Pts',(88.9824103636271,-2.09697996444503,
136.647975849991));
#249890=CARTESIAN_POINT('Ctrl Pts',(88.7039627398144,3.78293010245805,135.727226022576));
#249891=CARTESIAN_POINT('Ctrl Pts',(88.4255151160013,6.18651221161165,130.282603383299));
#249892=CARTESIAN_POINT('Ctrl Pts',(88.1470674921886,2.9049918262175,125.317450153056));
#249893=CARTESIAN_POINT('Ctrl Pts',(87.8686198683756,-3.04607413073006,
125.394499589218));
#249894=CARTESIAN_POINT('Ctrl Pts',(87.5901722445627,-6.19794677053091,
130.442947024027));
#249895=CARTESIAN_POINT('Ctrl Pts',(87.3117246207499,-3.65420911474647,
135.823515895262));
#249896=CARTESIAN_POINT('Ctrl Pts',(87.033276996937,2.24756819945024,136.59172626566));
#249897=CARTESIAN_POINT('Ctrl Pts',(86.754829373124,6.08394013816284,132.041630333989));
#249898=CARTESIAN_POINT('Ctrl Pts',(86.4763817493112,4.32946830690299,126.35454397691));
#249899=CARTESIAN_POINT('Ctrl Pts',(86.1979341254982,-1.40357339211569,
124.756621726966));
#249900=CARTESIAN_POINT('Ctrl Pts',(85.9194865016854,-5.84679971215209,
128.716276069012));
#249901=CARTESIAN_POINT('Ctrl Pts',(85.6410388778725,-4.91710272876601,
134.594778102578));
#249902=CARTESIAN_POINT('Ctrl Pts',(85.3625912540596,0.531171448533366,
136.990071639606));
#249903=CARTESIAN_POINT('Ctrl Pts',(85.0841436302467,5.49132501379855,133.700998936161));
#249904=CARTESIAN_POINT('Ctrl Pts',(84.8056960064338,5.4052191575235,127.750057126576));
#249905=CARTESIAN_POINT('Ctrl Pts',(84.527248382621,0.351980955120191,124.60587101419));
#249906=CARTESIAN_POINT('Ctrl Pts',(84.2488007588079,-5.02471054981291,
127.157794034254));
#249907=CARTESIAN_POINT('Ctrl Pts',(83.9703531349953,-5.78393853022499,
133.0607335997));
#249908=CARTESIAN_POINT('Ctrl Pts',(83.6919055111822,-1.22800956246596,
136.890176624513));
#249909=CARTESIAN_POINT('Ctrl Pts',(83.4134578873695,4.45640020159694,135.127052047582));
#249910=CARTESIAN_POINT('Ctrl Pts',(83.1350102635564,6.04559588764522,129.391585221682));
#249911=CARTESIAN_POINT('Ctrl Pts',(82.8565626397436,2.07918429672594,124.954389966684));
#249912=CARTESIAN_POINT('Ctrl Pts',(82.5781150159307,-3.79789608908488,
125.893031952893));
#249913=CARTESIAN_POINT('Ctrl Pts',(82.2996673921181,-6.18489550656524,
131.344945050191));
#249914=CARTESIAN_POINT('Ctrl Pts',(82.0212197683047,-2.88827810245507,
136.300087462925));
#249915=CARTESIAN_POINT('Ctrl Pts',(81.7427721444922,3.06252577758164,136.204925385956));
#249916=CARTESIAN_POINT('Ctrl Pts',(81.464324520679,6.19901808072266,131.146908119091));
#249917=CARTESIAN_POINT('Ctrl Pts',(81.1858768968663,3.6389156065486,125.774106432701));
#249918=CARTESIAN_POINT('Ctrl Pts',(80.9074292730533,-2.26517253913331,
125.023862600622));
#249919=CARTESIAN_POINT('Ctrl Pts',(80.6289816492404,-6.08767778118217,
129.585614053086));
#249920=CARTESIAN_POINT('Ctrl Pts',(80.3505340254275,-4.31590454191782,
135.267334059228));
#249921=CARTESIAN_POINT('Ctrl Pts',(80.0720864016147,1.42197412771073,136.847799500855));
#249922=CARTESIAN_POINT('Ctrl Pts',(79.7936387778018,5.85312804127117,132.874639847142));
#249923=CARTESIAN_POINT('Ctrl Pts',(79.5151911539889,4.90554322610457,126.998994720211));
#249924=CARTESIAN_POINT('Ctrl Pts',(79.236743530176,-0.54999616474248,124.62029495049));
#249925=CARTESIAN_POINT('Ctrl Pts',(78.9582959063631,-5.50011594899764,
127.924449420408));
#249926=CARTESIAN_POINT('Ctrl Pts',(78.6798482825503,-5.39589787172579,
133.87510158903));
#249927=CARTESIAN_POINT('Ctrl Pts',(78.4014006587372,-0.333113254603616,
137.003892818912));
#249928=CARTESIAN_POINT('Ctrl Pts',(78.1229530349246,5.035786170012,134.435616819741));
#249929=CARTESIAN_POINT('Ctrl Pts',(77.8445054111114,5.77704411621779,128.530393767498));
#249930=CARTESIAN_POINT('Ctrl Pts',(77.5660577872988,1.20948074391421,124.71483516101));
#249931=CARTESIAN_POINT('Ctrl Pts',(77.2876101634857,-4.46953634562727,
126.49525295924));
#249932=CARTESIAN_POINT('Ctrl Pts',(77.009162539673,-6.04126788252658,132.235530183857));
#249933=CARTESIAN_POINT('Ctrl Pts',(76.73071491586,-2.06136936772754,136.660632493573));
#249934=CARTESIAN_POINT('Ctrl Pts',(76.4522672920471,3.81282689252116,135.704107044024));
#249935=CARTESIAN_POINT('Ctrl Pts',(76.1738196682342,6.18322150549176,130.244953994479));
#249936=CARTESIAN_POINT('Ctrl Pts',(75.8953720444213,2.87153762207887,125.299868303017));
#249937=CARTESIAN_POINT('Ctrl Pts',(75.6169244206085,-3.07894905361277,
125.413142139227));
#249938=CARTESIAN_POINT('Ctrl Pts',(75.3384767967955,-6.20003196405775,
130.480682381363));
#249939=CARTESIAN_POINT('Ctrl Pts',(75.0600291729826,-3.62358838793365,
135.84566711001));
#249940=CARTESIAN_POINT('Ctrl Pts',(74.7815815491698,2.28275589456742,136.577937453613));
#249941=CARTESIAN_POINT('Ctrl Pts',(74.5031339253568,6.09135902878616,132.004572739798));
#249942=CARTESIAN_POINT('Ctrl Pts',(74.224686301544,4.30230079498258,126.328271719272));
#249943=CARTESIAN_POINT('Ctrl Pts',(73.946238677731,-1.44036169033171,124.76527772718));
#249944=CARTESIAN_POINT('Ctrl Pts',(73.6677910539182,-5.85940214781156,
128.75190588575));
#249945=CARTESIAN_POINT('Ctrl Pts',(73.3893434301052,-4.89393827916089,
134.624639674871));
#249946=CARTESIAN_POINT('Ctrl Pts',(73.1108958062924,0.56881578586215,136.986723641335));
#249947=CARTESIAN_POINT('Ctrl Pts',(72.8324481824796,5.50885593187395,133.66751801418));
#249948=CARTESIAN_POINT('Ctrl Pts',(72.5540005586665,5.38652659906729,127.717210612549));
#249949=CARTESIAN_POINT('Ctrl Pts',(72.2755529348538,0.314242468171368,
124.603843249867));
#249950=CARTESIAN_POINT('Ctrl Pts',(71.9971053110409,-5.04681513937595,
127.188448435987));
#249951=CARTESIAN_POINT('Ctrl Pts',(71.7186576872279,-5.77009618446306,
133.095900269846));
#249952=CARTESIAN_POINT('Ctrl Pts',(71.4402100634152,-1.19094072089807,
136.897539111196));
#249953=CARTESIAN_POINT('Ctrl Pts',(71.1617624396021,4.48263108448347,135.099844585217));
#249954=CARTESIAN_POINT('Ctrl Pts',(70.8833148157894,6.03688391192757,129.354810139024));
#249955=CARTESIAN_POINT('Ctrl Pts',(70.6048671919763,2.04353534248492,124.941841768133));
#249956=CARTESIAN_POINT('Ctrl Pts',(70.3264195681636,-3.82772237444985,
125.916241819903));
#249957=CARTESIAN_POINT('Ctrl Pts',(70.0479719443506,-6.18149022389895,
131.382584248845));
#249958=CARTESIAN_POINT('Ctrl Pts',(69.7695243205378,-2.85477054017052,
136.317567408437));
#249959=CARTESIAN_POINT('Ctrl Pts',(69.4910766967249,3.09534380668036,136.186182862342));
#249960=CARTESIAN_POINT('Ctrl Pts',(69.2126290729119,6.20098841114368,131.109166589932));
#249961=CARTESIAN_POINT('Ctrl Pts',(68.934181449099,3.60822760089105,125.752048519516));
#249962=CARTESIAN_POINT('Ctrl Pts',(68.6557338252862,-2.30031810286251,
125.037758448041));
#249963=CARTESIAN_POINT('Ctrl Pts',(68.3772862014732,-6.09498384687224,
129.622694056181));
#249964=CARTESIAN_POINT('Ctrl Pts',(68.0988385776604,-4.28865719212064,
135.293523506613));
#249965=CARTESIAN_POINT('Ctrl Pts',(67.8203909538475,1.45873590963839,136.83903156981));
#249966=CARTESIAN_POINT('Ctrl Pts',(67.5419433300346,5.86562197365073,132.83897183796));
#249967=CARTESIAN_POINT('Ctrl Pts',(67.2634957062218,4.88228799544191,126.969203790852));
#249968=CARTESIAN_POINT('Ctrl Pts',(66.9850480824087,-0.587630137549865,
124.623757509667));
#249969=CARTESIAN_POINT('Ctrl Pts',(66.706600458596,-5.51754488146136,127.957983545393));
#249970=CARTESIAN_POINT('Ctrl Pts',(66.428152834783,-5.37710542636232,133.907891057196));
#249971=CARTESIAN_POINT('Ctrl Pts',(66.1497052109702,-0.295368770640213,
137.00580571087));
#249972=CARTESIAN_POINT('Ctrl Pts',(65.8712575871573,5.05779735573374,134.404895281231));
#249973=CARTESIAN_POINT('Ctrl Pts',(65.5928099633443,5.76309479932555,128.495269391582));
#249974=CARTESIAN_POINT('Ctrl Pts',(65.3143623395316,1.17238966517029,124.707585533234));
#249975=CARTESIAN_POINT('Ctrl Pts',(65.0359147157185,-4.49568429685739,
126.522540133366));
#249976=CARTESIAN_POINT('Ctrl Pts',(64.7574670919057,-6.03244401646077,
132.272278579917));
#249977=CARTESIAN_POINT('Ctrl Pts',(64.4790194680927,-2.02568238621027,
136.673072130848));
#249978=CARTESIAN_POINT('Ctrl Pts',(64.20057184428,3.84258239688126,135.680806503568));
#249979=CARTESIAN_POINT('Ctrl Pts',(63.922124220467,6.17970167782515,130.207325334677));
#249980=CARTESIAN_POINT('Ctrl Pts',(63.6436765966542,2.8379770120581,125.282490423967));
#249981=CARTESIAN_POINT('Ctrl Pts',(63.3652289728412,-3.11170988490585,
125.431984462817));
#249982=CARTESIAN_POINT('Ctrl Pts',(63.0867813490283,-6.20188741312008,
130.518429732716));
#249983=CARTESIAN_POINT('Ctrl Pts',(62.8083337252156,-3.59283338772076,
135.86763151729));
#249984=CARTESIAN_POINT('Ctrl Pts',(62.5298861014024,2.31785900132509,136.563934699553));
#249985=CARTESIAN_POINT('Ctrl Pts',(62.2514384775899,6.09855220186056,131.967470671305));
#249986=CARTESIAN_POINT('Ctrl Pts',(61.9729908537767,4.27497385972414,126.302165324755));
#249987=CARTESIAN_POINT('Ctrl Pts',(61.6945432299639,-1.47709661541541,
124.774157507831));
#249988=CARTESIAN_POINT('Ctrl Pts',(61.416095606151,-5.87178746116934,128.787611756953));
#249989=CARTESIAN_POINT('Ctrl Pts',(61.1376479823382,-4.8705924828735,134.65435968532));
#249990=CARTESIAN_POINT('Ctrl Pts',(60.8592003585251,0.606439045512412,
136.983146553331));
#249991=CARTESIAN_POINT('Ctrl Pts',(60.5807527347125,5.52618271726667,133.633930996847));
#249992=CARTESIAN_POINT('Ctrl Pts',(60.3023051108993,5.36763444088732,127.684478494003));
#249993=CARTESIAN_POINT('Ctrl Pts',(60.0238574870866,0.276492336852797,
124.602045247997));
#249994=CARTESIAN_POINT('Ctrl Pts',(59.7454098632736,-5.06873271734795,
127.219236826675));
#249995=CARTESIAN_POINT('Ctrl Pts',(59.4669622394608,-5.75604002566515,
133.130982026147));
#249996=CARTESIAN_POINT('Ctrl Pts',(59.1885146156479,-1.15382774858414,
136.904675812908));
#249997=CARTESIAN_POINT('Ctrl Pts',(58.9100669918351,4.50869586182645,135.072477952114));
#249998=CARTESIAN_POINT('Ctrl Pts',(58.6316193680221,6.02794823725661,129.318088769994));
#249999=CARTESIAN_POINT('Ctrl Pts',(58.3531717442092,2.00781066429043,124.929510807376));
#250000=CARTESIAN_POINT('Ctrl Pts',(58.0747241203963,-3.85740682215468,
125.939632817953));
#250001=CARTESIAN_POINT('Ctrl Pts',(57.7962764965834,-6.17785588383907,
131.42020202121));
#250002=CARTESIAN_POINT('Ctrl Pts',(57.5178288727705,-2.82115719331391,
136.334843060042));
#250003=CARTESIAN_POINT('Ctrl Pts',(57.2393812489577,3.12804713667602,136.167240913326));
#250004=CARTESIAN_POINT('Ctrl Pts',(56.9609336251447,6.20272896165862,131.071413766074));
#250005=CARTESIAN_POINT('Ctrl Pts',(56.6824860013319,3.57740589103289,125.730177821614));
#250006=CARTESIAN_POINT('Ctrl Pts',(56.404038377519,-2.33537842745856,125.051867979023));
#250007=CARTESIAN_POINT('Ctrl Pts',(56.125590753706,-6.10206406069443,129.659817846364));
#250008=CARTESIAN_POINT('Ctrl Pts',(55.8471431298932,-4.26125092455389,
135.319546606417));
#250009=CARTESIAN_POINT('Ctrl Pts',(55.5686955060803,1.49544363757083,136.830040021814));
#250010=CARTESIAN_POINT('Ctrl Pts',(55.2902478822675,5.87789855325116,132.80322843551));
#250011=CARTESIAN_POINT('Ctrl Pts',(55.0118002584545,4.85885184980179,126.939554974638));
#250012=CARTESIAN_POINT('Ctrl Pts',(54.7333526346416,-0.625242335506623,
124.627449093364));
#250013=CARTESIAN_POINT('Ctrl Pts',(54.4549050108287,-5.53476935927053,
127.991623143927));
#250014=CARTESIAN_POINT('Ctrl Pts',(54.1764573870159,-5.35811373037978,
133.9405655229));
#250015=CARTESIAN_POINT('Ctrl Pts',(53.8980097632029,-0.257613341678002,
137.007488805997));
#250016=CARTESIAN_POINT('Ctrl Pts',(53.61956213939,5.07962112291461,134.374040323585));
#250017=CARTESIAN_POINT('Ctrl Pts',(53.3411145155772,5.74893192883615,128.460230579889));
#250018=CARTESIAN_POINT('Ctrl Pts',(53.0626668917642,1.13525514309568,124.7005618237));
#250019=CARTESIAN_POINT('Ctrl Pts',(52.7842192679514,-4.52166565885288,
126.549985971924));
#250020=CARTESIAN_POINT('Ctrl Pts',(52.5057716441385,-6.0233966159634,132.308972581737));
#250021=CARTESIAN_POINT('Ctrl Pts',(52.2273240203255,-1.98992034228702,
136.685294300858));
#250022=CARTESIAN_POINT('Ctrl Pts',(51.9488763965128,3.87219551293788,135.657325264614));
#250023=CARTESIAN_POINT('Ctrl Pts',(51.6704287726998,6.17595285904027,130.169718798237));
#250024=CARTESIAN_POINT('Ctrl Pts',(51.391981148887,2.80431123975502,125.265317159845));
#250025=CARTESIAN_POINT('Ctrl Pts',(51.113533525074,-3.14435541064497,125.451025861782));
#250026=CARTESIAN_POINT('Ctrl Pts',(50.8350859012611,-6.20351304896362,
130.556187679343));
#250027=CARTESIAN_POINT('Ctrl Pts',(50.5566382774483,-3.5619452537452,135.889408303207));
#250028=CARTESIAN_POINT('Ctrl Pts',(50.2781906536353,2.35287621896542,136.549718522358));
#250029=CARTESIAN_POINT('Ctrl Pts',(49.9997430298226,6.10551939084041,131.930325503341));
#250030=CARTESIAN_POINT('Ctrl Pts',(49.7212954060095,4.2474885137371,126.27622576074));
#250031=CARTESIAN_POINT('Ctrl Pts',(49.4428477821967,-1.51377680614101,
124.783260739875));
#250032=CARTESIAN_POINT('Ctrl Pts',(49.1644001583838,-5.88395519328364,
128.823392359526));
#250033=CARTESIAN_POINT('Ctrl Pts',(48.8859525345709,-4.84706620499019,
134.683937032636));
#250034=CARTESIAN_POINT('Ctrl Pts',(48.607504910758,0.644039833341117,136.97934050814));
#250035=CARTESIAN_POINT('Ctrl Pts',(48.3290572869451,5.54330472792681,133.600239128744));
#250036=CARTESIAN_POINT('Ctrl Pts',(48.0506096631323,5.34854338303893,127.651861983834));
#250037=CARTESIAN_POINT('Ctrl Pts',(47.7721620393193,0.23873196000854,124.600477075203));
#250038=CARTESIAN_POINT('Ctrl Pts',(47.4937144155065,-5.09046247156518,
127.250158065443));
#250039=CARTESIAN_POINT('Ctrl Pts',(47.2152667916935,-5.74177057468722,
133.165977568637));
#250040=CARTESIAN_POINT('Ctrl Pts',(46.9368191678807,-1.11667202075834,
136.911586465198));
#250041=CARTESIAN_POINT('Ctrl Pts',(46.6583715440677,4.53459356778643,135.044953162355));
#250042=CARTESIAN_POINT('Ctrl Pts',(46.379923920255,6.01878919474683,129.281422475313));
#250043=CARTESIAN_POINT('Ctrl Pts',(46.101476296442,1.97201158593325,124.917397541337));
#250044=CARTESIAN_POINT('Ctrl Pts',(45.8230286726291,-3.88694833223118,
125.963204080281));
#250045=CARTESIAN_POINT('Ctrl Pts',(45.5445810488162,-6.17399262105761,
131.457796973343));
#250046=CARTESIAN_POINT('Ctrl Pts',(45.2661334250033,-2.78743930743976,
136.351913777587));
#250047=CARTESIAN_POINT('Ctrl Pts',(44.9876858011905,3.16063455573481,136.148100240809));
#250048=CARTESIAN_POINT('Ctrl Pts',(44.7092381773775,6.20423966777097,131.033651046464));
#250049=CARTESIAN_POINT('Ctrl Pts',(44.4307905535647,3.54645161908363,125.708495149421));
#250050=CARTESIAN_POINT('Ctrl Pts',(44.1523429297517,-2.37035221374829,
125.066190670735));
#250051=CARTESIAN_POINT('Ctrl Pts',(43.8738953059389,-6.10891816028884,
129.696984048001));
#250052=CARTESIAN_POINT('Ctrl Pts',(43.5954476821259,-4.23368675476706,
135.345402394343));
#250053=CARTESIAN_POINT('Ctrl Pts',(43.3170000583131,1.53209595128933,136.820825190051));
#250054=CARTESIAN_POINT('Ctrl Pts',(43.0385524345002,5.88995732515911,132.767410964279));
#250055=CARTESIAN_POINT('Ctrl Pts',(42.7601048106873,4.83523565761953,126.910049370218));
#250056=CARTESIAN_POINT('Ctrl Pts',(42.4816571868744,-0.662831364878718,
124.631369564788));
#250057=CARTESIAN_POINT('Ctrl Pts',(42.2032095630615,-5.55178874416567,
128.025366969483));
#250058=CARTESIAN_POINT('Ctrl Pts',(41.9247619392486,-5.33892348752252,
133.973123775378));
#250059=CARTESIAN_POINT('Ctrl Pts',(41.6463143154357,-0.219848366758665,
137.008942041929));
#250060=CARTESIAN_POINT('Ctrl Pts',(41.3678666916229,5.10125666286673,134.343053090145));
#250061=CARTESIAN_POINT('Ctrl Pts',(41.0894190678099,5.73455602955998,128.425278630796));
#250062=CARTESIAN_POINT('Ctrl Pts',(40.8109714439971,1.09807855372398,124.693764292674));
#250063=CARTESIAN_POINT('Ctrl Pts',(40.5325238201841,-4.5474794688646,126.5775894579));
#250064=CARTESIAN_POINT('Ctrl Pts',(40.2540761963713,-6.01412601628932,
132.345610829607));
#250065=CARTESIAN_POINT('Ctrl Pts',(39.9756285725584,-1.95408456113369,
136.697298550707));
#250066=CARTESIAN_POINT('Ctrl Pts',(39.6971809487455,3.90166514336576,135.633664197272));
#250067=CARTESIAN_POINT('Ctrl Pts',(39.4187333249326,6.171975188051,130.132135778682));
#250068=CARTESIAN_POINT('Ctrl Pts',(39.1402857011198,2.77054155266769,125.248349147017));
#250069=CARTESIAN_POINT('Ctrl Pts',(38.8618380773068,-3.17688442113803,
125.470265630536));
#250070=CARTESIAN_POINT('Ctrl Pts',(38.583390453494,-6.20490881134979,130.593954822108));
#250071=CARTESIAN_POINT('Ctrl Pts',(38.304942829681,-3.53092513057837,135.910996660811));
#250072=CARTESIAN_POINT('Ctrl Pts',(38.0264952058682,2.38780624991219,136.535289448812));
#250073=CARTESIAN_POINT('Ctrl Pts',(37.7480475820552,6.11226033755391,131.893138612335));
#250074=CARTESIAN_POINT('Ctrl Pts',(37.4695999582424,4.21984577550119,126.250453988427));
#250075=CARTESIAN_POINT('Ctrl Pts',(37.1911523344295,-1.55040090331038,
124.792587085991));
#250076=CARTESIAN_POINT('Ctrl Pts',(36.9127047106166,-5.89590489327443,
128.859246367608));
#250077=CARTESIAN_POINT('Ctrl Pts',(36.6342570868037,-4.82336031728617,
134.713370620821));
#250078=CARTESIAN_POINT('Ctrl Pts',(36.3558094629908,0.681616756036961,
136.975305646799));
#250079=CARTESIAN_POINT('Ctrl Pts',(36.0773618391779,5.56022132939171,133.566443658335));
#250080=CARTESIAN_POINT('Ctrl Pts',(35.798914215365,5.32925413294858,127.619362290662));
#250081=CARTESIAN_POINT('Ctrl Pts',(35.5204665915522,0.200962736863706,
124.599138789596));
#250082=CARTESIAN_POINT('Ctrl Pts',(35.2420189677392,-5.11200359682353,
127.281211006494));
#250083=CARTESIAN_POINT('Ctrl Pts',(34.9635713439263,-5.72728836028912,
133.200885600541));
#250084=CARTESIAN_POINT('Ctrl Pts',(34.6851237201134,-1.07947491424015,
136.918270811987));
#250085=CARTESIAN_POINT('Ctrl Pts',(34.4066760963006,4.56032324271418,135.017271235878));
#250086=CARTESIAN_POINT('Ctrl Pts',(34.1282284724876,6.00940712379002,129.244812613665));
#250087=CARTESIAN_POINT('Ctrl Pts',(33.8497808486748,1.93613943396156,124.905502418881));
#250088=CARTESIAN_POINT('Ctrl Pts',(33.5713332248619,-3.91634581000783,
125.986954733445));
#250089=CARTESIAN_POINT('Ctrl Pts',(33.292885601049,-6.16990057870911,131.495367712155));
#250090=CARTESIAN_POINT('Ctrl Pts',(33.0144379772361,-2.753618131977,136.368778928511));
#250091=CARTESIAN_POINT('Ctrl Pts',(32.7359903534233,3.19310485631782,136.128761554055));
#250092=CARTESIAN_POINT('Ctrl Pts',(32.4575427296103,6.20552047350092,130.995879830412));
#250093=CARTESIAN_POINT('Ctrl Pts',(32.1790951057975,3.51536593206519,125.687001306397));
#250094=CARTESIAN_POINT('Ctrl Pts',(31.9006474819845,-2.40523816576522,
125.080725992446));
#250095=CARTESIAN_POINT('Ctrl Pts',(31.6221998581717,-6.11554589167424,
129.734191283883));
#250096=CARTESIAN_POINT('Ctrl Pts',(31.3437522343588,-4.20596570416061,
135.371089912296));
#250097=CARTESIAN_POINT('Ctrl Pts',(31.0653046105458,1.56869149262894,136.811387415981));
#250098=CARTESIAN_POINT('Ctrl Pts',(30.786856986733,5.90179784253235,132.731520751495));
#250099=CARTESIAN_POINT('Ctrl Pts',(30.5084093629201,4.81144029400183,126.880688070935));
#250100=CARTESIAN_POINT('Ctrl Pts',(30.2299617391072,-0.700395832790832,
124.635518778667));
#250101=CARTESIAN_POINT('Ctrl Pts',(29.9515141152943,-5.56860240548724,
128.05921377167));
#250102=CARTESIAN_POINT('Ctrl Pts',(29.6730664914815,-5.31953540889204,
134.005564608172));
#250103=CARTESIAN_POINT('Ctrl Pts',(29.3946188676685,-0.182075245277261,
137.010165364815));
#250104=CARTESIAN_POINT('Ctrl Pts',(29.1161712438556,5.12270317387725,134.311934729152));
#250105=CARTESIAN_POINT('Ctrl Pts',(28.8377236200427,5.71996763420123,128.390414839463));
#250106=CARTESIAN_POINT('Ctrl Pts',(28.5592759962298,1.06086127464794,124.687193192043));
#250107=CARTESIAN_POINT('Ctrl Pts',(28.280828372417,-4.57312477035222,126.605349568435));
#250108=CARTESIAN_POINT('Ctrl Pts',(28.0023807486041,-6.00463256096402,
132.382191965885));
#250109=CARTESIAN_POINT('Ctrl Pts',(27.7239331247912,-1.91817637065835,
136.709084435575));
#250110=CARTESIAN_POINT('Ctrl Pts',(27.4454855009783,3.93099019615694,135.60982417831));
#250111=CARTESIAN_POINT('Ctrl Pts',(27.1670378771654,6.16776881225138,130.094577668667));
#250112=CARTESIAN_POINT('Ctrl Pts',(26.8885902533525,2.73666920214424,125.231587014236));
#250113=CARTESIAN_POINT('Ctrl Pts',(26.6101426295396,-3.20929571101057,
125.48970305614));
#250114=CARTESIAN_POINT('Ctrl Pts',(26.3316950057267,-6.2060746485581,130.631729761538));
#250115=CARTESIAN_POINT('Ctrl Pts',(26.0532473819138,-3.49977416768234,
135.932395790139));
#250116=CARTESIAN_POINT('Ctrl Pts',(25.774799758101,2.42264779982026,136.52064801359));
#250117=CARTESIAN_POINT('Ctrl Pts',(25.4963521342881,6.11877479221284,131.85591137626));
#250118=CARTESIAN_POINT('Ctrl Pts',(25.2179045104751,4.19204666932822,126.224850962798));
#250119=CARTESIAN_POINT('Ctrl Pts',(24.9394568866623,-1.58696754980412,
124.802136200585));
#250120=CARTESIAN_POINT('Ctrl Pts',(24.6610092628494,-5.90763611834117,
128.895172452612));
#250121=CARTESIAN_POINT('Ctrl Pts',(24.3825616390365,-4.79947569819179,
134.742659359205));
#250122=CARTESIAN_POINT('Ctrl Pts',(24.1041140152236,0.719168421173241,
136.97104211882));
#250123=CARTESIAN_POINT('Ctrl Pts',(23.8256663914108,5.57693189481048,133.532545837923));
#250124=CARTESIAN_POINT('Ctrl Pts',(23.5472187675978,5.3097674053865,127.586980618775));
#250125=CARTESIAN_POINT('Ctrl Pts',(23.2687711437849,0.163186066970757,
124.598030440764));
#250126=CARTESIAN_POINT('Ctrl Pts',(22.990323519972,-5.13335529490864,127.312394499151));
#250127=CARTESIAN_POINT('Ctrl Pts',(22.7118758961592,-5.71259391911463,
133.235704828331));
#250128=CARTESIAN_POINT('Ctrl Pts',(22.4334282723462,-1.04223780738205,
136.924728605587));
#250129=CARTESIAN_POINT('Ctrl Pts',(22.1549806485334,4.58588393318709,134.98943319845));
#250130=CARTESIAN_POINT('Ctrl Pts',(21.8765330247205,5.9998023720423,129.208260541641));
#250131=CARTESIAN_POINT('Ctrl Pts',(21.5980854009075,1.90019553763114,124.893825880784));
#250132=CARTESIAN_POINT('Ctrl Pts',(21.3196377770947,-3.94559816615024,
126.010883897355));
#250133=CARTESIAN_POINT('Ctrl Pts',(21.0411901532818,-6.16557990842568,
131.532912845442));
#250134=CARTESIAN_POINT('Ctrl Pts',(20.7627425294689,-2.71969492018171,
136.385437887866));
#250135=CARTESIAN_POINT('Ctrl Pts',(20.484294905656,3.22545683522612,136.109225569666));
#250136=CARTESIAN_POINT('Ctrl Pts',(20.2058472818431,6.20657133138755,130.958101517545));
#250137=CARTESIAN_POINT('Ctrl Pts',(19.9273996580302,3.48414998186958,125.665697089004));
#250138=CARTESIAN_POINT('Ctrl Pts',(19.6489520342174,-2.44003499079723,
125.095473405541));
#250139=CARTESIAN_POINT('Ctrl Pts',(19.3705044104044,-6.12194700925765,
129.771438175283));
#250140=CARTESIAN_POINT('Ctrl Pts',(19.0920567865916,-4.17808879994825,
135.396608208416));
#250141=CARTESIAN_POINT('Ctrl Pts',(18.8136091627787,1.60522890552839,136.801727049323));
#250142=CARTESIAN_POINT('Ctrl Pts',(18.5351615389658,5.91341966661616,132.695559127084));
#250143=CARTESIAN_POINT('Ctrl Pts',(18.2567139151529,4.78746664069464,126.85147216478));
#250144=CARTESIAN_POINT('Ctrl Pts',(17.97826629134,-0.737934347277788,124.63989658125));
#250145=CARTESIAN_POINT('Ctrl Pts',(17.6998186675271,-5.58520972019883,
128.093162296283));
#250146=CARTESIAN_POINT('Ctrl Pts',(17.4213710437142,-5.29995021292075,
134.037886819174));
#250147=CARTESIAN_POINT('Ctrl Pts',(17.1429234199013,-0.144295376930669,
137.011158729324));
#250148=CARTESIAN_POINT('Ctrl Pts',(16.8644757960885,5.14395986123776,134.280686393713));
#250149=CARTESIAN_POINT('Ctrl Pts',(16.5860281722755,5.70516728333829,128.355640497777));
#250150=CARTESIAN_POINT('Ctrl Pts',(16.3075805484627,1.02360468496723,124.6808487653));
#250151=CARTESIAN_POINT('Ctrl Pts',(16.0291329246498,-4.5986006130197,126.633265274869));
#250152=CARTESIAN_POINT('Ctrl Pts',(15.7506853008369,-5.99491660177097,
132.418714635041));
#250153=CARTESIAN_POINT('Ctrl Pts',(15.472237677024,-1.88219710145218,136.720651518731));
#250154=CARTESIAN_POINT('Ctrl Pts',(15.1937900532111,3.96016958466077,135.585806091128));
#250155=CARTESIAN_POINT('Ctrl Pts',(14.9153424293982,6.16333388751023,130.057045859918));
#250156=CARTESIAN_POINT('Ctrl Pts',(14.6368948055853,2.70269544333712,125.215031382631));
#250157=CARTESIAN_POINT('Ctrl Pts',(14.3584471817724,-3.24158807925031,
125.509337418335));
#250158=CARTESIAN_POINT('Ctrl Pts',(14.0799995579596,-6.20701051738803,
130.669511097867));
#250159=CARTESIAN_POINT('Ctrl Pts',(13.8015519341466,-3.46849351936748,
135.953604898237));
#250160=CARTESIAN_POINT('Ctrl Pts',(13.5231043103337,2.45739957762318,136.505794759238));
#250161=CARTESIAN_POINT('Ctrl Pts',(13.2446566865208,6.12506251342167,131.818645174584));
#250162=CARTESIAN_POINT('Ctrl Pts',(12.966209062708,4.16409222532429,126.199417632585));
#250163=CARTESIAN_POINT('Ctrl Pts',(12.687761438895,-1.62347539063169,124.811907729812));
#250164=CARTESIAN_POINT('Ctrl Pts',(12.4093138150822,-5.91914843377905,
128.931169283287));
#250165=CARTESIAN_POINT('Ctrl Pts',(12.1308661912693,-4.77541323276041,
134.771802162479));
#250166=CARTESIAN_POINT('Ctrl Pts',(11.8524185674564,0.756693437259193,
136.96655008219));
#250167=CARTESIAN_POINT('Ctrl Pts',(11.5739709436435,5.59343580496719,133.498546923603));
#250168=CARTESIAN_POINT('Ctrl Pts',(11.2955233198306,5.2900839224404,127.554718168085));
#250169=CARTESIAN_POINT('Ctrl Pts',(11.0170756960177,0.125403350157864,
124.597152069781));
#250170=CARTESIAN_POINT('Ctrl Pts',(10.7386280722048,-5.15451677462551,
127.343707387895));
#250171=CARTESIAN_POINT('Ctrl Pts',(10.460180448392,-5.69768779567166,133.270433961767));
#250172=CARTESIAN_POINT('Ctrl Pts',(10.1817328245791,-1.0049620800187,136.930959606699));
#250173=CARTESIAN_POINT('Ctrl Pts',(9.90328520076621,4.61127469204443,134.961440081617));
#250174=CARTESIAN_POINT('Ctrl Pts',(9.62483757695328,5.98997529541125,129.171767613693));
#250175=CARTESIAN_POINT('Ctrl Pts',(9.34638995314043,1.86418122885626,124.882368359726));
#250176=CARTESIAN_POINT('Ctrl Pts',(9.0679423293275,-3.97470431670162,126.034990685308));
#250177=CARTESIAN_POINT('Ctrl Pts',(8.78949470551463,-6.16103077031137,
131.57043098196));
#250178=CARTESIAN_POINT('Ctrl Pts',(8.5110470817017,-2.68567092909101,136.401890038352));
#250179=CARTESIAN_POINT('Ctrl Pts',(8.2325994578889,3.25768929364524,136.089493011555));
#250180=CARTESIAN_POINT('Ctrl Pts',(7.95415183407592,6.20739220249103,130.920317507753));
#250181=CARTESIAN_POINT('Ctrl Pts',(7.67570421026306,3.45280492521512,125.644583286679));
#250182=CARTESIAN_POINT('Ctrl Pts',(7.39725658645018,-2.47474139943534,
125.110432363552));
#250183=CARTESIAN_POINT('Ctrl Pts',(7.11880896263729,-6.1281212758433,129.808723342005));
#250184=CARTESIAN_POINT('Ctrl Pts',(6.84036133882437,-4.15005707511893,
135.421956337113));
#250185=CARTESIAN_POINT('Ctrl Pts',(6.56191371501151,1.64170683608044,136.791844448048));
#250186=CARTESIAN_POINT('Ctrl Pts',(6.28346609119863,5.92482236675955,132.659527423617));
#250187=CARTESIAN_POINT('Ctrl Pts',(6.00501846738572,4.76331558605049,126.822402734361));
#250188=CARTESIAN_POINT('Ctrl Pts',(5.72657084357281,-0.775445517336138,
124.644502810313));
#250189=CARTESIAN_POINT('Ctrl Pts',(5.44812321975995,-5.60161007291028,
128.127211285347));
#250190=CARTESIAN_POINT('Ctrl Pts',(5.16967559594705,-5.28016862534525,
134.070089210674));
#250191=CARTESIAN_POINT('Ctrl Pts',(4.89122797213414,-0.106510161665837,
137.011922098645));
#250192=CARTESIAN_POINT('Ctrl Pts',(4.6127803483213,5.16502593727395,134.249309241742));
#250193=CARTESIAN_POINT('Ctrl Pts',(4.33433272450837,5.69015552540359,128.320956894316));
#250194=CARTESIAN_POINT('Ctrl Pts',(4.05588510069549,0.986310165238503,
124.674731247541));
#250195=CARTESIAN_POINT('Ctrl Pts',(3.77743747688256,-4.62390605285035,
126.661335542776));
#250196=CARTESIAN_POINT('Ctrl Pts',(3.49898985306972,-5.98497849873861,
132.455177483715));
#250197=CARTESIAN_POINT('Ctrl Pts',(3.22054222925682,-1.84614808674025,
136.731999371551));
#250198=CARTESIAN_POINT('Ctrl Pts',(2.94209460544391,3.9892022276243,135.561610825727));
#250199=CARTESIAN_POINT('Ctrl Pts',(2.66364698163102,6.15867057816533,130.019541743194));
#250200=CARTESIAN_POINT('Ctrl Pts',(2.38519935781816,2.66862153515642,125.198682865676));
#250201=CARTESIAN_POINT('Ctrl Pts',(2.10675173400524,-3.27376032925169,
125.529167989562));
#250202=CARTESIAN_POINT('Ctrl Pts',(1.82830411019233,-6.20771638316062,
130.707297431096));
#250203=CARTESIAN_POINT('Ctrl Pts',(1.54985648637947,-3.43708434474973,
135.974623199195));
#250204=CARTESIAN_POINT('Ctrl Pts',(1.27140886256659,2.49206029558105,136.490730236146));
#250205=CARTESIAN_POINT('Ctrl Pts',(0.992961238753657,6.13112326818657,
131.78134138822));
#250206=CARTESIAN_POINT('Ctrl Pts',(0.714513614940807,4.13598347935162,
126.174154940227));
#250207=CARTESIAN_POINT('Ctrl Pts',(0.436065991127901,-1.65992307298164,
124.821901311585));
#250208=CARTESIAN_POINT('Ctrl Pts',(0.157618367314999,-5.93044141299494,
128.967235525755));
#250209=CARTESIAN_POINT('Ctrl Pts',(-0.120829256497892,-4.75117381263555,
134.800797950748));
#250210=CARTESIAN_POINT('Ctrl Pts',(-0.399276880310752,0.794190413791566,
136.961829703365));
#250211=CARTESIAN_POINT('Ctrl Pts',(-0.67772450412367,5.60973244830296,
133.464448175219));
#250212=CARTESIAN_POINT('Ctrl Pts',(-0.956172127936585,5.27020441348929,
127.522576134092));
#250213=CARTESIAN_POINT('Ctrl Pts',(-1.23461975174943,0.0876159864779326,
124.596503709192));
#250214=CARTESIAN_POINT('Ctrl Pts',(-1.51306737556233,-5.17548725182775,
127.375148512417));
#250215=CARTESIAN_POINT('Ctrl Pts',(-1.79151499937523,-5.6825705423121,
133.305071713949));
#250216=CARTESIAN_POINT('Ctrl Pts',(-2.06996262318813,-0.967649113415911,
136.936963584433));
#250217=CARTESIAN_POINT('Ctrl Pts',(-2.34841024700098,4.63649457842225,
134.933292922676));
#250218=CARTESIAN_POINT('Ctrl Pts',(-2.62685787081389,5.97992625804282,
129.13533518208));
#250219=CARTESIAN_POINT('Ctrl Pts',(-2.90530549462681,1.82809784216042,
124.871130280269));
#250220=CARTESIAN_POINT('Ctrl Pts',(-3.18375311843967,-4.00366318312286,
126.059274204017));
#250221=CARTESIAN_POINT('Ctrl Pts',(-3.46220074225256,-6.15625333293613,
131.607920731459));
#250222=CARTESIAN_POINT('Ctrl Pts',(-3.74064836606547,-2.65154741947636,
136.418134770325));
#250223=CARTESIAN_POINT('Ctrl Pts',(-4.01909598987837,3.28980103718956,
136.06956461092));
#250224=CARTESIAN_POINT('Ctrl Pts',(-4.29754361369122,6.20798305639367,
130.882529201136));
#250225=CARTESIAN_POINT('Ctrl Pts',(-4.57599123750414,3.42133192360438,
125.623660681799));
#250226=CARTESIAN_POINT('Ctrl Pts',(-4.85443886131705,-2.5093561056208,
125.125602312169));
#250227=CARTESIAN_POINT('Ctrl Pts',(-5.13288648512991,-6.13406846264146,
129.846045402432));
#250228=CARTESIAN_POINT('Ctrl Pts',(-5.41133410894279,-4.12187156839848,
135.447133359102));
#250229=CARTESIAN_POINT('Ctrl Pts',(-5.68978173275571,1.67812393258193,
136.781739978358));
#250230=CARTESIAN_POINT('Ctrl Pts',(-5.9682293565686,5.93600552043131,132.623426976261));
#250231=CARTESIAN_POINT('Ctrl Pts',(-6.24667698038146,4.73898802499559,
126.793480856855));
#250232=CARTESIAN_POINT('Ctrl Pts',(-6.52512460419438,-0.812927952975666,
124.649337295173));
#250233=CARTESIAN_POINT('Ctrl Pts',(-6.80357222800728,-5.61780285590049,
128.161359477164));
#250234=CARTESIAN_POINT('Ctrl Pts',(-7.08201985182013,-5.26019137917956,
134.1021705894));
#250235=CARTESIAN_POINT('Ctrl Pts',(-7.36046747563304,-0.0687209996277829,
137.012455444495));
#250236=CARTESIAN_POINT('Ctrl Pts',(-7.63891509944595,5.18590062137458,
134.217804435933));
#250237=CARTESIAN_POINT('Ctrl Pts',(-7.91736272325884,5.67493291666336,
128.286365314294));
#250238=CARTESIAN_POINT('Ctrl Pts',(-8.1958103470717,0.948979097423875,
124.668840865451));
#250239=CARTESIAN_POINT('Ctrl Pts',(-8.47425797088461,-4.64904015214177,
126.689559331999));
#250240=CARTESIAN_POINT('Ctrl Pts',(-8.75270559469752,-5.97481862012702,
132.491579160764));
#250241=CARTESIAN_POINT('Ctrl Pts',(-9.03115321851038,-1.81003066233205,
136.743127573537));
#250242=CARTESIAN_POINT('Ctrl Pts',(-9.30960084232328,4.0180870492325,135.537239278668));
#250243=CARTESIAN_POINT('Ctrl Pts',(-9.58804846613619,6.15377905701727,
129.982066708221));
#250244=CARTESIAN_POINT('Ctrl Pts',(-9.86649608994908,2.63444874022312,
125.182542069172));
#250245=CARTESIAN_POINT('Ctrl Pts',(-10.144943713762,-3.30581126886015,
125.549194034992));
#250246=CARTESIAN_POINT('Ctrl Pts',(-10.4233913375749,-6.20819221971975,
130.745087361036));
#250247=CARTESIAN_POINT('Ctrl Pts',(-10.7018389613878,-3.40554780770759,
135.995449914173));
#250248=CARTESIAN_POINT('Ctrl Pts',(-10.9802865852006,2.52662866932821,
136.475455002538));
#250249=CARTESIAN_POINT('Ctrl Pts',(-11.2587342090136,6.13695683192405,
131.744001399476));
#250250=CARTESIAN_POINT('Ctrl Pts',(-11.5371818328265,4.10772147299012,
126.149063821843));
#250251=CARTESIAN_POINT('Ctrl Pts',(-11.8156294566394,-1.69630924627168,
124.832116575588));
#250252=CARTESIAN_POINT('Ctrl Pts',(-12.0940770804522,-5.94151463752335,
129.003369843568));
#250253=CARTESIAN_POINT('Ctrl Pts',(-12.3725247042651,-4.72675833601782,
134.829645649562));
#250254=CARTESIAN_POINT('Ctrl Pts',(-12.6509723280781,0.83165796130609,
136.956881157257));
#250255=CARTESIAN_POINT('Ctrl Pts',(-12.9294199518909,5.62582122093989,
133.430250856313));
#250256=CARTESIAN_POINT('Ctrl Pts',(-13.2078675757038,5.25012961517551,
127.490555707831));
#250257=CARTESIAN_POINT('Ctrl Pts',(-13.4863151995167,0.0498253761554086,
124.596085383024));
#250258=CARTESIAN_POINT('Ctrl Pts',(-13.7647628233296,-5.19626594944658,
127.406716707655));
#250259=CARTESIAN_POINT('Ctrl Pts',(-14.0432104471424,-5.66724271921134,
133.339616801361));
#250260=CARTESIAN_POINT('Ctrl Pts',(-14.3216580709554,-0.930300290219375,
136.942740316309));
#250261=CARTESIAN_POINT('Ctrl Pts',(-14.6001056947683,4.6615426577884,134.904992764631));
#250262=CARTESIAN_POINT('Ctrl Pts',(-14.8785533185811,5.96965563230779,
129.098964596818));
#250263=CARTESIAN_POINT('Ctrl Pts',(-15.157000942394,1.79194671462675,124.860112058844));
#250264=CARTESIAN_POINT('Ctrl Pts',(-15.4354485662069,-4.03247369233249,
126.08373355365));
#250265=CARTESIAN_POINT('Ctrl Pts',(-15.7138961900198,-6.15124777332969,
131.645380704742));
#250266=CARTESIAN_POINT('Ctrl Pts',(-15.9923438138327,-2.61732565579698,
136.434171481834));
#250267=CARTESIAN_POINT('Ctrl Pts',(-16.2707914376456,3.32179087594663,
136.049441106215));
#250268=CARTESIAN_POINT('Ctrl Pts',(-16.5492390614585,6.2083438712012,130.844737997954));
#250269=CARTESIAN_POINT('Ctrl Pts',(-16.8276866852714,3.38973214328102,
125.602930049661));
#250270=CARTESIAN_POINT('Ctrl Pts',(-17.1061343090842,-2.54387782669295,
125.140982689263));
#250271=CARTESIAN_POINT('Ctrl Pts',(-17.3845819328972,-6.13978834927694,
129.883402973582));
#250272=CARTESIAN_POINT('Ctrl Pts',(-17.66302955671,-4.09353332421128,135.47213834144));
#250273=CARTESIAN_POINT('Ctrl Pts',(-17.9414771805229,1.71447884558397,
136.771414014676));
#250274=CARTESIAN_POINT('Ctrl Pts',(-18.2199248043358,5.94696871323555,
132.587259122732));
#250275=CARTESIAN_POINT('Ctrl Pts',(-18.4983724281487,4.71448485899666,
126.764707603974));
#250276=CARTESIAN_POINT('Ctrl Pts',(-18.7768200519616,-0.850380265270943,
124.654399856686));
#250277=CARTESIAN_POINT('Ctrl Pts',(-19.0552676757745,-5.63378746913994,
128.19560560636));
#250278=CARTESIAN_POINT('Ctrl Pts',(-19.3337152995874,-5.24001921468789,
134.134129766565));
#250279=CARTESIAN_POINT('Ctrl Pts',(-19.6121629234003,-0.0309292911078312,
137.012758747106));
#250280=CARTESIAN_POINT('Ctrl Pts',(-19.8906105472132,5.2065831400206,134.18617314371));
#250281=CARTESIAN_POINT('Ctrl Pts',(-20.1690581710261,5.65950002119693,
128.251867039513));
#250282=CARTESIAN_POINT('Ctrl Pts',(-20.447505794839,0.911612864839816,
124.663177837304));
#250283=CARTESIAN_POINT('Ctrl Pts',(-20.7259534186518,-4.67400197954067,
126.717935596697));
#250284=CARTESIAN_POINT('Ctrl Pts',(-21.0044010424647,-5.96443734241423,
132.527918317308));
#250285=CARTESIAN_POINT('Ctrl Pts',(-21.2828486662776,-1.77384616657202,
136.754035712331));
#250286=CARTESIAN_POINT('Ctrl Pts',(-21.5612962900905,4.0468229791472,135.512692353051));
#250287=CARTESIAN_POINT('Ctrl Pts',(-21.8397439139034,6.14865950532324,
129.944622143653));
#250288=CARTESIAN_POINT('Ctrl Pts',(-22.1181915377163,2.60017832482316,
125.166609591221));
#250289=CARTESIAN_POINT('Ctrl Pts',(-22.3966391615293,-3.33773971041633,
125.569414812551));
#250290=CARTESIAN_POINT('Ctrl Pts',(-22.6750867853421,-6.20843800943312,
130.782879487369));
#250291=CARTESIAN_POINT('Ctrl Pts',(-22.953534409155,-3.37388507683905,
136.016084271426));
#250292=CARTESIAN_POINT('Ctrl Pts',(-23.2319820329679,2.56110341792085,
136.45996962444));
#250293=CARTESIAN_POINT('Ctrl Pts',(-23.5104296567807,6.14256298846929,
131.706626591997));
#250294=CARTESIAN_POINT('Ctrl Pts',(-23.7888772805937,4.07930725349882,
126.124145207193));
#250295=CARTESIAN_POINT('Ctrl Pts',(-24.0673249044065,-1.73263256219878,
124.842553143289));
#250296=CARTESIAN_POINT('Ctrl Pts',(-24.3457725282195,-5.95236769704188,
129.039570897758));
#250297=CARTESIAN_POINT('Ctrl Pts',(-24.6242201520323,-4.70216770763169,
134.858344189959));
#250298=CARTESIAN_POINT('Ctrl Pts',(-24.9026677758452,0.86909469142902,
136.951704627238));
#250299=CARTESIAN_POINT('Ctrl Pts',(-25.1811153996581,5.64170152670257,
133.395956234079));
#250300=CARTESIAN_POINT('Ctrl Pts',(-25.459563023471,5.22986027137813,127.458658075828));
#250301=CARTESIAN_POINT('Ctrl Pts',(-25.7380106472839,0.0120329195352371,
124.595897106778));
#250302=CARTESIAN_POINT('Ctrl Pts',(-26.0164582710968,-5.21685209751974,
127.438410803838));
#250303=CARTESIAN_POINT('Ctrl Pts',(-26.2949058949097,-5.6517048943475,
133.374067943923));
#250304=CARTESIAN_POINT('Ctrl Pts',(-26.5733535187226,-0.892916994403456,
136.948289588268));
#250305=CARTESIAN_POINT('Ctrl Pts',(-26.8518011425354,4.68641800197708,
134.876540656153));
#250306=CARTESIAN_POINT('Ctrl Pts',(-27.1302487663484,5.95916379878798,
129.062657205632));
#250307=CARTESIAN_POINT('Ctrl Pts',(-27.4086963901612,1.75572918584856,
124.849314103734));
#250308=CARTESIAN_POINT('Ctrl Pts',(-27.6871440139742,-4.06113477674652,
126.108367827853));
#250309=CARTESIAN_POINT('Ctrl Pts',(-27.965591637787,-6.1460142769749,131.682809513716));
#250310=CARTESIAN_POINT('Ctrl Pts',(-28.2440392616,-2.5830069061529,136.449999578631));
#250311=CARTESIAN_POINT('Ctrl Pts',(-28.5224868854127,3.3536576245212,136.029123243122));
#250312=CARTESIAN_POINT('Ctrl Pts',(-28.8009345092257,6.20847463354345,
130.806945298572));
#250313=CARTESIAN_POINT('Ctrl Pts',(-29.0793821330386,3.35800675518651,
125.582392158445));
#250314=CARTESIAN_POINT('Ctrl Pts',(-29.3578297568515,-2.57830528343674,
125.156572924908));
#250315=CARTESIAN_POINT('Ctrl Pts',(-29.6362773806644,-6.14528072379723,
129.920794671155));
#250316=CARTESIAN_POINT('Ctrl Pts',(-29.9147250044772,-4.06504339264135,
135.496970357558));
#250317=CARTESIAN_POINT('Ctrl Pts',(-30.1931726282902,1.75077022794215,
136.760866939637));
#250318=CARTESIAN_POINT('Ctrl Pts',(-30.471620252103,5.95771153892721,132.551025203244));
#250319=CARTESIAN_POINT('Ctrl Pts',(-30.750067875916,4.68980699602731,126.736084041921));
#250320=CARTESIAN_POINT('Ctrl Pts',(-31.0285154997288,-0.887801066412759,
124.659690307256));
#250321=CARTESIAN_POINT('Ctrl Pts',(-31.3069631235417,-5.6495633203129,
128.229948403933));
#250322=CARTESIAN_POINT('Ctrl Pts',(-31.5854107473546,-5.21965287935721,
134.16596555791));
#250323=CARTESIAN_POINT('Ctrl Pts',(-31.8638583711675,0.00686356350839004,
137.012831995241));
#250324=CARTESIAN_POINT('Ctrl Pts',(-32.1423059949804,5.22707272681363,
134.154416537178));
#250325=CARTESIAN_POINT('Ctrl Pts',(-32.4207536187933,5.64385741087595,
128.217463348321));
#250326=CARTESIAN_POINT('Ctrl Pts',(-32.6992012426062,0.874212852105795,
124.657742372942));
#250327=CARTESIAN_POINT('Ctrl Pts',(-32.9776488664191,-4.69879061007736,
126.746463285377));
#250328=CARTESIAN_POINT('Ctrl Pts',(-33.2560964902319,-5.9538350502823,
132.564193606789));
#250329=CARTESIAN_POINT('Ctrl Pts',(-33.5345441140448,-1.73759594028995,
136.764723383724));
#250330=CARTESIAN_POINT('Ctrl Pts',(-33.8129917378578,4.07540895254819,
135.487970958469));
#250331=CARTESIAN_POINT('Ctrl Pts',(-34.0914393616706,6.14331211279008,
129.907209437008));
#250332=CARTESIAN_POINT('Ctrl Pts',(-34.3698869854835,2.56581155885918,
125.150886022208));
#250333=CARTESIAN_POINT('Ctrl Pts',(-34.6483346092964,-3.3695444708001,
125.589829572953));
#250334=CARTESIAN_POINT('Ctrl Pts',(-34.9267822331094,-6.2084537431929,
130.820672409693));
#250335=CARTESIAN_POINT('Ctrl Pts',(-35.2052298569221,-3.34209732541825,
136.036525506343));
#250336=CARTESIAN_POINT('Ctrl Pts',(-35.4836774807351,2.59548326388451,
136.444274675672));
#250337=CARTESIAN_POINT('Ctrl Pts',(-35.7621251045479,6.14794153008404,
131.66921835072));
#250338=CARTESIAN_POINT('Ctrl Pts',(-36.0405727283609,4.05074187377708,
126.099400019648));
#250339=CARTESIAN_POINT('Ctrl Pts',(-36.3190203521737,-1.76889167478912,
124.85321062796));
#250340=CARTESIAN_POINT('Ctrl Pts',(-36.5974679759867,-5.96300018938643,
129.075837346879));
#250341=CARTESIAN_POINT('Ctrl Pts',(-36.8759155997995,-4.67740283869194,
134.886892508504));
#250342=CARTESIAN_POINT('Ctrl Pts',(-37.1543632236125,0.906499216928551,
136.946300305126));
#250343=CARTESIAN_POINT('Ctrl Pts',(-37.4328108474252,5.65737277714046,
133.361565579315));
#250344=CARTESIAN_POINT('Ctrl Pts',(-37.7112584712383,5.2093971331851,127.426884420063));
#250345=CARTESIAN_POINT('Ctrl Pts',(-37.9897060950511,-0.0257599829691867,
124.595938887431));
#250346=CARTESIAN_POINT('Ctrl Pts',(-38.268153718864,-5.23724493321992,
127.470229626529));
#250347=CARTESIAN_POINT('Ctrl Pts',(-38.5466013426768,-5.63595764348039,
133.408423865036));
#250348=CARTESIAN_POINT('Ctrl Pts',(-38.8250489664898,-0.855500611219946,
136.953611194679));
#250349=CARTESIAN_POINT('Ctrl Pts',(-39.1034965903026,4.71111968922328,
134.847937651547));
#250350=CARTESIAN_POINT('Ctrl Pts',(-39.3819442141156,5.94845114626212,
129.026414353905));
#250351=CARTESIAN_POINT('Ctrl Pts',(-39.6603918379284,1.71944659787975,
124.838736815064));
#250352=CARTESIAN_POINT('Ctrl Pts',(-39.9388394617414,-4.08964537431793,
126.133176113797));
#250353=CARTESIAN_POINT('Ctrl Pts',(-40.2172870855541,-6.14055303780089,
131.720205771443));
#250354=CARTESIAN_POINT('Ctrl Pts',(-40.495734709367,-2.54859244223803,
136.465618474199));
#250355=CARTESIAN_POINT('Ctrl Pts',(-40.7741823331801,3.3854001020792,136.008611774531));
#250356=CARTESIAN_POINT('Ctrl Pts',(-41.0526299569928,6.20837533857501,
130.769152503414));
#250357=CARTESIAN_POINT('Ctrl Pts',(-41.3310775808058,3.3261569349168,125.562047769191));
#250358=CARTESIAN_POINT('Ctrl Pts',(-41.6095252046187,-2.61263720013008,
125.172372441404));
#250359=CARTESIAN_POINT('Ctrl Pts',(-41.8879728284316,-6.15054538268038,
129.958219109591));
#250360=CARTESIAN_POINT('Ctrl Pts',(-42.1664204522444,-4.03640282939359,
135.521628487296));
#250361=CARTESIAN_POINT('Ctrl Pts',(-42.4448680760573,1.78699673486542,
136.750099144066));
#250362=CARTESIAN_POINT('Ctrl Pts',(-42.7233156998703,5.96823359942677,
132.514726560457));
#250363=CARTESIAN_POINT('Ctrl Pts',(-43.0017633236831,4.66495535053527,
126.707611231352));
#250364=CARTESIAN_POINT('Ctrl Pts',(-43.2802109474961,-0.925188969759574,
124.665208450844));
#250365=CARTESIAN_POINT('Ctrl Pts',(-43.5586585713089,-5.6651298248394,
128.264386597296));
#250366=CARTESIAN_POINT('Ctrl Pts',(-43.8371061951219,-5.19909312786956,
134.197676783747));
#250367=CARTESIAN_POINT('Ctrl Pts',(-44.1155538189346,0.0446561637927345,
137.012675186187));
#250368=CARTESIAN_POINT('Ctrl Pts',(-44.3940014427476,5.24736862250453,
134.122535793092));
#250369=CARTESIAN_POINT('Ctrl Pts',(-44.6724490665605,5.62800566534308,
128.183155515557));
#250370=CARTESIAN_POINT('Ctrl Pts',(-44.9508966903734,0.836780445093053,
124.65253467378));
#250371=CARTESIAN_POINT('Ctrl Pts',(-45.2293443141862,-4.72340512520001,
126.775141340936));
#250372=CARTESIAN_POINT('Ctrl Pts',(-45.5077919379991,-5.94301213660306,
132.600403685011));
#250373=CARTESIAN_POINT('Ctrl Pts',(-45.7862395618121,-1.7012813267513,
136.775190191685));
#250374=CARTESIAN_POINT('Ctrl Pts',(-46.0646871856249,4.10384391017172,
135.463076010984));
#250375=CARTESIAN_POINT('Ctrl Pts',(-46.3431348094379,6.13773707756737,
129.869829974632));
#250376=CARTESIAN_POINT('Ctrl Pts',(-46.6215824332507,2.5313497158043,125.135371944775));
#250377=CARTESIAN_POINT('Ctrl Pts',(-46.9000300570636,-3.40122437147435,
125.610437559721));
#250378=CARTESIAN_POINT('Ctrl Pts',(-47.1784776808764,-6.20823942041608,
130.858464727578));
#250379=CARTESIAN_POINT('Ctrl Pts',(-47.4569253046894,-3.31018573135201,
136.056772861467));
#250380=CARTESIAN_POINT('Ctrl Pts',(-47.7353729285023,2.62976693326135,
136.428370737814));
#250381=CARTESIAN_POINT('Ctrl Pts',(-48.0138205523151,6.15309225746451,
131.631778061822));
#250382=CARTESIAN_POINT('Ctrl Pts',(-48.2922681761281,4.02202639232555,
126.074829176147));
#250383=CARTESIAN_POINT('Ctrl Pts',(-48.570715799941,-1.80508524044794,
124.864088634681));
#250384=CARTESIAN_POINT('Ctrl Pts',(-48.8491634237538,-5.97341172056607,
129.112167847066));
#250385=CARTESIAN_POINT('Ctrl Pts',(-49.1276110475668,-4.65246464686987,
134.915289547327));
#250386=CARTESIAN_POINT('Ctrl Pts',(-49.4060586713796,0.943870151766231,
136.940668391181));
#250387=CARTESIAN_POINT('Ctrl Pts',(-49.6845062951925,5.6728343915496,133.327080166382));
#250388=CARTESIAN_POINT('Ctrl Pts',(-49.9629539190054,5.18874095886556,
127.395235917922));
#250389=CARTESIAN_POINT('Ctrl Pts',(-50.2414015428183,-0.0635519309279763,
124.596210723434));
#250390=CARTESIAN_POINT('Ctrl Pts',(-50.5198491666312,-5.25744370088312,
127.50217199667));
#250391=CARTESIAN_POINT('Ctrl Pts',(-50.798296790444,-5.6200015501302,133.442683291627));
#250392=CARTESIAN_POINT('Ctrl Pts',(-51.076744414257,-0.818052527146474,
136.958704938348));
#250393=CARTESIAN_POINT('Ctrl Pts',(-51.3551920380699,4.73564680419706,
134.819184810706));
#250394=CARTESIAN_POINT('Ctrl Pts',(-51.6336396618827,5.93751807169133,
128.990237384633));
#250395=CARTESIAN_POINT('Ctrl Pts',(-51.9120872856956,1.68310029518491,
124.828380584778));
#250396=CARTESIAN_POINT('Ctrl Pts',(-52.1905349095086,-4.11800442857602,
126.1581574922));
#250397=CARTESIAN_POINT('Ctrl Pts',(-52.4689825333214,-6.13486425817587,
131.757568092191));
#250398=CARTESIAN_POINT('Ctrl Pts',(-52.7474301571343,-2.51408353929296,
136.481027589776));
#250399=CARTESIAN_POINT('Ctrl Pts',(-53.0258777809472,3.41701713239144,
135.987907460498));
#250400=CARTESIAN_POINT('Ctrl Pts',(-53.3043254047601,6.20804598997526,
130.731361012906));
#250401=CARTESIAN_POINT('Ctrl Pts',(-53.5827730285729,3.29418386267868,
125.541897635768));
#250402=CARTESIAN_POINT('Ctrl Pts',(-53.8612206523859,-2.64687230459117,
125.188380653292));
#250403=CARTESIAN_POINT('Ctrl Pts',(-54.1396682761987,-6.15558213084251,
129.995674902111));
#250404=CARTESIAN_POINT('Ctrl Pts',(-54.4181159000117,-4.0076126957546,
135.546111816938));
#250405=CARTESIAN_POINT('Ctrl Pts',(-54.6965635238244,1.82315702396754,
136.739111026966));
#250406=CARTESIAN_POINT('Ctrl Pts',(-54.9750111476374,5.97853450483549,
132.478364539431));
#250407=CARTESIAN_POINT('Ctrl Pts',(-55.2534587714502,4.63993084340721,
126.679290227339));
#250408=CARTESIAN_POINT('Ctrl Pts',(-55.5319063952633,-0.962542589888887,
124.670954082973));
#250409=CARTESIAN_POINT('Ctrl Pts',(-55.810354019076,-5.68048640589689,
128.298918910331));
#250410=CARTESIAN_POINT('Ctrl Pts',(-56.088801642889,-5.1783407220741,134.229262269005));
#250411=CARTESIAN_POINT('Ctrl Pts',(-56.3672492667019,0.0824471093265141,
137.012288325754));
#250412=CARTESIAN_POINT('Ctrl Pts',(-56.6456968905149,5.26747007502141,
134.090532092806));
#250413=CARTESIAN_POINT('Ctrl Pts',(-56.9241445143275,5.6119453719906,128.148944812513));
#250414=CARTESIAN_POINT('Ctrl Pts',(-57.2025921381407,0.799317030873196,
124.64755493279));
#250415=CARTESIAN_POINT('Ctrl Pts',(-57.4810397619534,-4.74784461280872,
126.803968700697));
#250416=CARTESIAN_POINT('Ctrl Pts',(-57.7594873857663,-5.93196900242356,
132.636547210196));
#250417=CARTESIAN_POINT('Ctrl Pts',(-58.0379350095792,-1.66490367160747,
136.785435748359));
#250418=CARTESIAN_POINT('Ctrl Pts',(-58.3163826333922,4.13212679834998,
135.438008433087));
#250419=CARTESIAN_POINT('Ctrl Pts',(-58.5948302572049,6.13193460624012,
129.832485141631));
#250420=CARTESIAN_POINT('Ctrl Pts',(-58.873277881018,2.49679407265481,125.120067933803));
#250421=CARTESIAN_POINT('Ctrl Pts',(-59.1517255048308,-3.43277823852872,
125.631238009216));
#250422=CARTESIAN_POINT('Ctrl Pts',(-59.4301731286437,-6.20779504904446,
130.896255040614));
#250423=CARTESIAN_POINT('Ctrl Pts',(-59.7086207524566,-3.27815147713605,
136.076825586523));
#250424=CARTESIAN_POINT('Ctrl Pts',(-59.9870683762695,2.66395315565763,
136.412258400192));
#250425=CARTESIAN_POINT('Ctrl Pts',(-60.2655160000824,6.15801497974849,
131.594307112665));
#250426=CARTESIAN_POINT('Ctrl Pts',(-60.5439636238952,3.99316187320697,
126.050433587173));
#250427=CARTESIAN_POINT('Ctrl Pts',(-60.8224112477081,-1.84121191800936,
124.875186760365));
#250428=CARTESIAN_POINT('Ctrl Pts',(-61.1008588715211,-5.98360190477769,
129.148561052078));
#250429=CARTESIAN_POINT('Ctrl Pts',(-61.3793064953339,-4.62735405625939,
134.943534254169));
#250430=CARTESIAN_POINT('Ctrl Pts',(-61.6577541191468,0.981206111148332,
136.934809094094));
#250431=CARTESIAN_POINT('Ctrl Pts',(-61.9362017429597,5.68808579699418,
133.292501273148));
#250432=CARTESIAN_POINT('Ctrl Pts',(-62.2146493667725,5.16789251384163,
127.36371374215));
#250433=CARTESIAN_POINT('Ctrl Pts',(-62.4930969905855,-0.10134152394658,
124.596712604715));
#250434=CARTESIAN_POINT('Ctrl Pts',(-62.7715446143984,-5.27744765203657,
127.534236730624));
#250435=CARTESIAN_POINT('Ctrl Pts',(-63.0499922382113,-5.60383720555579,
133.476844954201));
#250436=CARTESIAN_POINT('Ctrl Pts',(-63.3284398620242,-0.780574129835986,
136.963570630527));
#250437=CARTESIAN_POINT('Ctrl Pts',(-63.606887485837,4.75999843803683,134.790283199078));
#250438=CARTESIAN_POINT('Ctrl Pts',(-63.88533510965,5.92636498020503,128.954127638363));
#250439=CARTESIAN_POINT('Ctrl Pts',(-64.1637827334628,1.64669162458969,
124.818245796629));
#250440=CARTESIAN_POINT('Ctrl Pts',(-64.4422303572757,-4.14621088866563,
126.183311037368));
#250441=CARTESIAN_POINT('Ctrl Pts',(-64.7206779810887,-6.12894814889968,
131.794895091487));
#250442=CARTESIAN_POINT('Ctrl Pts',(-64.9991256049015,-2.47948147605779,
136.49622635437));
#250443=CARTESIAN_POINT('Ctrl Pts',(-65.2775732287142,3.44850754387722,
135.967011068231));
#250444=CARTESIAN_POINT('Ctrl Pts',(-65.5560208525274,6.20748659994837,
130.693572227424));
#250445=CARTESIAN_POINT('Ctrl Pts',(-65.83446847634,3.26208872324607,125.521942504845));
#250446=CARTESIAN_POINT('Ctrl Pts',(-66.1129161001531,-2.68100932822562,
125.204596967384));
#250447=CARTESIAN_POINT('Ctrl Pts',(-66.3913637239659,-6.1603907816451,
130.033160660777));
#250448=CARTESIAN_POINT('Ctrl Pts',(-66.6698113477789,-3.97867405855336,
135.570419439246));
#250449=CARTESIAN_POINT('Ctrl Pts',(-66.9482589715917,1.85924975531565,
136.727902995508));
#250450=CARTESIAN_POINT('Ctrl Pts',(-67.2267065954047,5.98861387344954,
132.441940487574));
#250451=CARTESIAN_POINT('Ctrl Pts',(-67.5051542192175,4.61473440193538,
126.651122079325));
#250452=CARTESIAN_POINT('Ctrl Pts',(-67.7836018430304,-0.999860542648545,
124.676926990737));
#250453=CARTESIAN_POINT('Ctrl Pts',(-68.0620494668433,-5.69563249444164,
128.33354406343));
#250454=CARTESIAN_POINT('Ctrl Pts',(-68.3404970906562,-5.15739643095884,
134.260720843274));
#250455=CARTESIAN_POINT('Ctrl Pts',(-68.618944714469,0.120234999752325,
137.011671428276));
#250456=CARTESIAN_POINT('Ctrl Pts',(-68.8973923382821,5.28737633949755,
134.058406622227));
#250457=CARTESIAN_POINT('Ctrl Pts',(-69.1758399620947,5.59567712593856,
128.114832506878));
#250458=CARTESIAN_POINT('Ctrl Pts',(-69.4542875859078,0.761823997666808,
124.642803334499));
#250459=CARTESIAN_POINT('Ctrl Pts',(-69.7327352097205,-4.77210816728929,
126.832944296451));
#250460=CARTESIAN_POINT('Ctrl Pts',(-70.0111828335336,-5.92070605695121,
132.672622843033));
#250461=CARTESIAN_POINT('Ctrl Pts',(-70.2896304573463,-1.62846432284579,
136.795459674095));
#250462=CARTESIAN_POINT('Ctrl Pts',(-70.5680780811594,4.16025656905012,
135.412769153666));
#250463=CARTESIAN_POINT('Ctrl Pts',(-70.8465257049722,6.12590491382102,
129.795176321834));
#250464=CARTESIAN_POINT('Ctrl Pts',(-71.1249733287852,2.46214590988275,
125.104974556385));
#250465=CARTESIAN_POINT('Ctrl Pts',(-71.4034209525978,-3.46420490272305,
125.652230150673));
#250466=CARTESIAN_POINT('Ctrl Pts',(-71.681868576411,-6.20712064554441,
130.93404194847));
#250467=CARTESIAN_POINT('Ctrl Pts',(-71.9603162002238,-3.24599574981168,
136.09668293845));
#250468=CARTESIAN_POINT('Ctrl Pts',(-72.2387638240367,2.69804066428979,
136.395938259856));
#250469=CARTESIAN_POINT('Ctrl Pts',(-72.5172114478495,6.16270951452303,
131.556806891751));
#250470=CARTESIAN_POINT('Ctrl Pts',(-72.7956590716624,3.96414938600637,
126.026214156713));
#250471=CARTESIAN_POINT('Ctrl Pts',(-73.0741066954753,-1.87727036878649,
124.886504593767));
#250472=CARTESIAN_POINT('Ctrl Pts',(-73.3525543192881,-5.99357036442037,
129.185015613353));
#250473=CARTESIAN_POINT('Ctrl Pts',(-73.6310019431012,-4.60207199734241,
134.971625582408));
#250474=CARTESIAN_POINT('Ctrl Pts',(-73.909449566914,1.01850571157763,136.928722630985));
#250475=CARTESIAN_POINT('Ctrl Pts',(-74.187897190727,5.70312642832773,133.257830180947));
#250476=CARTESIAN_POINT('Ctrl Pts',(-74.4663448145398,5.14685257066011,
127.332319060812));
#250477=CARTESIAN_POINT('Ctrl Pts',(-74.7447924383527,-0.139127361718492,
124.597444512675));
#250478=CARTESIAN_POINT('Ctrl Pts',(-75.0232400621657,-5.29725604542678,
127.566422640223));
#250479=CARTESIAN_POINT('Ctrl Pts',(-75.3016876859784,-5.58746520873256,
133.510907586884));
#250480=CARTESIAN_POINT('Ctrl Pts',(-75.5801353097915,-0.743066808063574,
136.968208090913));
#250481=CARTESIAN_POINT('Ctrl Pts',(-75.8585829336042,4.7841736883842,134.761233887624));
#250482=CARTESIAN_POINT('Ctrl Pts',(-76.1370305574171,5.91499228508486,
128.918086453158));
#250483=CARTESIAN_POINT('Ctrl Pts',(-76.41547818123,1.61022193523031,124.808332826166));
#250484=CARTESIAN_POINT('Ctrl Pts',(-76.693925805043,-4.17426370938676,
126.208635817229));
#250485=CARTESIAN_POINT('Ctrl Pts',(-76.9723734288558,-6.12280492919574,
131.832185386163));
#250486=CARTESIAN_POINT('Ctrl Pts',(-77.2508210526686,-2.44478753472383,
136.511214204787));
#250487=CARTESIAN_POINT('Ctrl Pts',(-77.5292686764817,3.47987016964863,
135.945923372052));
#250488=CARTESIAN_POINT('Ctrl Pts',(-77.8077163002943,6.20669718922256,
130.655787547247));
#250489=CARTESIAN_POINT('Ctrl Pts',(-78.0861639241075,3.22987270591563,
125.502183115868));
#250490=CARTESIAN_POINT('Ctrl Pts',(-78.3646115479203,-2.71504700607423,
125.221020782777));
#250491=CARTESIAN_POINT('Ctrl Pts',(-78.6430591717333,-6.16497115690175,
130.070674996542));
#250492=CARTESIAN_POINT('Ctrl Pts',(-78.921506795546,-3.94958799012119,
135.594550453492));
#250493=CARTESIAN_POINT('Ctrl Pts',(-79.199954419359,1.89527359148086,136.71647546501));
#250494=CARTESIAN_POINT('Ctrl Pts',(-79.4784020431719,5.9984713317742,132.405455754592));
#250495=CARTESIAN_POINT('Ctrl Pts',(-79.7568496669848,4.58936695978296,
126.623107831093));
#250496=CARTESIAN_POINT('Ctrl Pts',(-80.0352972907976,-1.0371414452086,
124.683126952807));
#250497=CARTESIAN_POINT('Ctrl Pts',(-80.3137449146107,-5.71056752923021,
128.368260773546));
#250498=CARTESIAN_POINT('Ctrl Pts',(-80.5921925384234,-5.13626103062165,
134.292051340844));
#250499=CARTESIAN_POINT('Ctrl Pts',(-80.8706401622364,0.158018434826916,
137.010824516613));
#250500=CARTESIAN_POINT('Ctrl Pts',(-81.1490877860493,5.30708667829958,
134.026160571776));
#250501=CARTESIAN_POINT('Ctrl Pts',(-81.4275354098621,5.57920153001237,
128.080819862696));
#250502=CARTESIAN_POINT('Ctrl Pts',(-81.705983033675,0.724302734791404,
124.63828005498));
#250503=CARTESIAN_POINT('Ctrl Pts',(-81.984430657488,-4.79619488954742,
126.862067054498));
#250504=CARTESIAN_POINT('Ctrl Pts',(-82.2628782813007,-5.90922371753823,
132.708629246728));
#250505=CARTESIAN_POINT('Ctrl Pts',(-82.5413259051138,-1.59196463073914,
136.805261597452));
#250506=CARTESIAN_POINT('Ctrl Pts',(-82.8197735289264,4.18823217991362,
135.387359107972));
#250507=CARTESIAN_POINT('Ctrl Pts',(-83.0982211527395,6.11964822374235,
129.757904897731));
#250508=CARTESIAN_POINT('Ctrl Pts',(-83.3766687765523,2.42740651138818,
125.090092371815));
#250509=CARTESIAN_POINT('Ctrl Pts',(-83.6551164003652,-3.49550319953123,
125.67341320622));
#250510=CARTESIAN_POINT('Ctrl Pts',(-83.9335640241781,-6.20621623490623,
130.971824050937));
#250511=CARTESIAN_POINT('Ctrl Pts',(-84.2120116479911,-3.21371974092037,
136.116344181428));
#250512=CARTESIAN_POINT('Ctrl Pts',(-84.4904592718038,2.73202819603347,
136.379410921554));
#250513=CARTESIAN_POINT('Ctrl Pts',(-84.7689068956169,6.16717568783019,
131.519278788663));
#250514=CARTESIAN_POINT('Ctrl Pts',(-85.0473545194296,3.9349900057924,126.002171782228));
#250515=CARTESIAN_POINT('Ctrl Pts',(-85.3258021432425,-1.91325925661942,
124.898041715501));
#250516=CARTESIAN_POINT('Ctrl Pts',(-85.6042497670555,-6.00331673010926,
129.221530180052));
#250517=CARTESIAN_POINT('Ctrl Pts',(-85.8826973908683,-4.57661940695503,
134.999562491112));
#250518=CARTESIAN_POINT('Ctrl Pts',(-86.1611450146813,1.05576757090286,
136.922409227389));
#250519=CARTESIAN_POINT('Ctrl Pts',(-86.4395926384942,5.71795572821454,
133.223068174528));
#250520=CARTESIAN_POINT('Ctrl Pts',(-86.718040262307,5.12562190896342,127.301053037252));
#250521=CARTESIAN_POINT('Ctrl Pts',(-86.9964878861199,-0.176908044074368,
124.598406420195));
#250522=CARTESIAN_POINT('Ctrl Pts',(-87.2749355099329,-5.31686814704595,
127.598728532803));
#250523=CARTESIAN_POINT('Ctrl Pts',(-87.5533831337457,-5.57088616633168,
133.544869927476));
#250524=CARTESIAN_POINT('Ctrl Pts',(-87.8318307575586,-0.70553195167748,
136.972617147663));
#250525=CARTESIAN_POINT('Ctrl Pts',(-88.1102783813713,4.80817165941601,
134.732037952774));
#250526=CARTESIAN_POINT('Ctrl Pts',(-88.3887260051845,5.90340040775061,
128.882115164534));
#250527=CARTESIAN_POINT('Ctrl Pts',(-88.6671736289971,1.57369257850503,
124.798642040718));
#250528=CARTESIAN_POINT('Ctrl Pts',(-88.9456212528103,-4.20216185122988,
126.234130893362));
#250529=CARTESIAN_POINT('Ctrl Pts',(-89.2240688766231,-6.11643482670397,
131.869437594414));
#250530=CARTESIAN_POINT('Ctrl Pts',(-89.5025165004358,-2.41000300088966,
136.525990585645));
#250531=CARTESIAN_POINT('Ctrl Pts',(-89.7809641242489,3.51110384754994,
135.924645153375));
#250532=CARTESIAN_POINT('Ctrl Pts',(-90.0594117480617,6.20567778705031,
130.618008372501));
#250533=CARTESIAN_POINT('Ctrl Pts',(-90.3378593718745,3.19753700446471,
125.482620201028));
#250534=CARTESIAN_POINT('Ctrl Pts',(-90.6163069956876,-2.74898407685696,
125.237651490881));
#250535=CARTESIAN_POINT('Ctrl Pts',(-90.8947546195002,-6.16932308688508,
130.108216519297));
#250536=CARTESIAN_POINT('Ctrl Pts',(-91.1732022433134,-3.92035556825405,
135.618503965492));
#250537=CARTESIAN_POINT('Ctrl Pts',(-91.4516498671261,1.93122719758584,
136.70482885892));
#250538=CARTESIAN_POINT('Ctrl Pts',(-91.7300974909391,6.00810651453776,
132.368911692441));
#250539=CARTESIAN_POINT('Ctrl Pts',(-92.0085451147519,4.56382945695037,
126.595248520721));
#250540=CARTESIAN_POINT('Ctrl Pts',(-92.2869927385648,-1.07438391611076,
124.689553739443));
#250541=CARTESIAN_POINT('Ctrl Pts',(-92.5654403623776,-5.72529095683809,
128.403067754236));
#250542=CARTESIAN_POINT('Ctrl Pts',(-92.8438879861907,-5.11493530424405,
134.323252600751));
#250543=CARTESIAN_POINT('Ctrl Pts',(-93.1223356100035,0.195796014469281,
137.009747622148));
#250544=CARTESIAN_POINT('Ctrl Pts',(-93.4007832338166,5.32660036105212,
133.993795136343));
#250545=CARTESIAN_POINT('Ctrl Pts',(-93.6792308576291,5.56251919472255,
128.046908140318));
#250546=CARTESIAN_POINT('Ctrl Pts',(-93.9576784814422,0.686754632612129,
124.633985261843));
#250547=CARTESIAN_POINT('Ctrl Pts',(-94.2361261052551,-4.82010388703947,
126.891335895681));
#250548=CARTESIAN_POINT('Ctrl Pts',(-94.5145737290679,-5.8975224096676,
132.744565087048));
#250549=CARTESIAN_POINT('Ctrl Pts',(-94.7930213528811,-1.55540594779807,
136.814841155217));
#250550=CARTESIAN_POINT('Ctrl Pts',(-95.0714689766937,4.21605259429308,
135.361779237583));
#250551=CARTESIAN_POINT('Ctrl Pts',(-95.3499166005066,6.11316476784841,
129.720672250431));
#250552=CARTESIAN_POINT('Ctrl Pts',(-95.6283642243196,2.39257716445285,
125.075421931555));
#250553=CARTESIAN_POINT('Ctrl Pts',(-95.9068118481323,-3.52667196918255,
125.694786390909));
#250554=CARTESIAN_POINT('Ctrl Pts',(-96.1852594719453,-6.20508185064282,
131.009599947983));
#250555=CARTESIAN_POINT('Ctrl Pts',(-96.4637070957582,-3.18132464646333,
136.135808586901));
#250556=CARTESIAN_POINT('Ctrl Pts',(-96.742154719571,2.76591449146702,136.362676997713));
#250557=CARTESIAN_POINT('Ctrl Pts',(-97.020602343384,6.17141333417382,131.481724194021));
#250558=CARTESIAN_POINT('Ctrl Pts',(-97.299049967197,3.90568481307747,125.978307354616));
#250559=CARTESIAN_POINT('Ctrl Pts',(-97.5774975910097,-1.94917724792726,
124.909797698053));
#250560=CARTESIAN_POINT('Ctrl Pts',(-97.8559452148228,-6.01284064068852,
129.258103399115));
#250561=CARTESIAN_POINT('Ctrl Pts',(-98.1343928386354,-4.55099722825276,
135.027343945068));
#250562=CARTESIAN_POINT('Ctrl Pts',(-98.4128404624484,1.09299030837272,
136.915869117251));
#250563=CARTESIAN_POINT('Ctrl Pts',(-98.6912880862614,5.73257314714861,
133.188216542011));
#250564=CARTESIAN_POINT('Ctrl Pts',(-98.9697357100741,5.10420131546234,
127.269916830042));
#250565=CARTESIAN_POINT('Ctrl Pts',(-99.2481833338871,-0.214682171037078,
124.599598291628));
#250566=CARTESIAN_POINT('Ctrl Pts',(-99.5266309576999,-5.33628323016052,
127.631153211259));
#250567=CARTESIAN_POINT('Ctrl Pts',(-99.8050785815131,-5.55410069269506,
133.578730717485));
#250568=CARTESIAN_POINT('Ctrl Pts',(-100.083526205326,-0.667970951546107,
136.976797637399));
#250569=CARTESIAN_POINT('Ctrl Pts',(-100.361973829139,4.83199146187865,
134.702696476397));
#250570=CARTESIAN_POINT('Ctrl Pts',(-100.640421452952,5.89158977774298,
128.846215105423));
#250571=CARTESIAN_POINT('Ctrl Pts',(-100.918869076765,1.53710490802326,
124.789173799381));
#250572=CARTESIAN_POINT('Ctrl Pts',(-101.197316700577,-4.22990428042106,
126.259795321038));
#250573=CARTESIAN_POINT('Ctrl Pts',(-101.47576432439,-6.10983807746976,
131.906650335846));
#250574=CARTESIAN_POINT('Ctrl Pts',(-101.754211948203,-2.37512916350784,
136.540554949401));
#250575=CARTESIAN_POINT('Ctrl Pts',(-102.032659572016,3.54220742020778,
135.903177200671));
#250576=CARTESIAN_POINT('Ctrl Pts',(-102.311107195829,6.20442843120499,
130.580236103105));
#250577=CARTESIAN_POINT('Ctrl Pts',(-102.589554819642,3.16508281710451,
125.463254485237));
#250578=CARTESIAN_POINT('Ctrl Pts',(-102.868002443455,-2.78281928302352,
125.254488475437));
#250579=CARTESIAN_POINT('Ctrl Pts',(-103.146450067268,-6.1734464103326,
130.145783837928));
#250580=CARTESIAN_POINT('Ctrl Pts',(-103.424897691081,-3.8909778761698,
135.642279087639));
#250581=CARTESIAN_POINT('Ctrl Pts',(-103.703345314893,1.96710924135641,
136.69296360881));
#250582=CARTESIAN_POINT('Ctrl Pts',(-103.981792938706,6.01751906470488,
132.332309655276));
#250583=CARTESIAN_POINT('Ctrl Pts',(-104.260240562519,4.53812283973896,
126.567545180546));
#250584=CARTESIAN_POINT('Ctrl Pts',(-104.538688186332,-1.11158657532129,
124.696207112496));
#250585=CARTESIAN_POINT('Ctrl Pts',(-104.817135810145,-5.73980223168479,
128.437963715717));
#250586=CARTESIAN_POINT('Ctrl Pts',(-105.095583433958,-5.093420042057,134.354323466822));
#250587=CARTESIAN_POINT('Ctrl Pts',(-105.374031057771,0.233566338818549,
137.008440784786));
#250588=CARTESIAN_POINT('Ctrl Pts',(-105.652478681584,5.34591666467016,
133.961311515241));
#250589=CARTESIAN_POINT('Ctrl Pts',(-105.930926305397,5.54563073823764,
128.013098596357));
#250590=CARTESIAN_POINT('Ctrl Pts',(-106.20937392921,0.649181082487974,
124.629919114234));
#250591=CARTESIAN_POINT('Ctrl Pts',(-106.487821553022,-4.84383427380942,
126.920749735436));
#250592=CARTESIAN_POINT('Ctrl Pts',(-106.766269176835,-5.88560256693534,
132.780429032376));
#250593=CARTESIAN_POINT('Ctrl Pts',(-107.044716800648,-1.51878962871805,
136.824197992414));
#250594=CARTESIAN_POINT('Ctrl Pts',(-107.323164424461,4.2437167812931,135.336030490371));
#250595=CARTESIAN_POINT('Ctrl Pts',(-107.601612048274,6.10645478638612,
129.683479759601));
#250596=CARTESIAN_POINT('Ctrl Pts',(-107.880059672087,2.35765915969063,
125.060963779225));
#250597=CARTESIAN_POINT('Ctrl Pts',(-108.1585072959,-3.55771005670707,125.716348912751));
#250598=CARTESIAN_POINT('Ctrl Pts',(-108.436954919713,-6.20371753478999,
131.04736823981));
#250599=CARTESIAN_POINT('Ctrl Pts',(-108.715402543526,-3.14881166685081,
136.155075433609));
#250600=CARTESIAN_POINT('Ctrl Pts',(-108.993850167338,2.79969829492213,
136.345737108415));
#250601=CARTESIAN_POINT('Ctrl Pts',(-109.272297791151,6.17542229652738,
131.444144499421));
#250602=CARTESIAN_POINT('Ctrl Pts',(-109.550745414964,3.87623489377466,
125.954621758183));
#250603=CARTESIAN_POINT('Ctrl Pts',(-109.829193038777,-1.98502301175461,
124.921772105802));
#250604=CARTESIAN_POINT('Ctrl Pts',(-110.10764066259,-6.02214174324697,
129.294733915307));
#250605=CARTESIAN_POINT('Ctrl Pts',(-110.386088286403,-4.52520641067474,
135.054968914823));
#250606=CARTESIAN_POINT('Ctrl Pts',(-110.664535910216,1.13017254468408,
136.909102542919));
#250607=CARTESIAN_POINT('Ctrl Pts',(-110.942983534029,5.74697814347679,
133.153276574838));
#250608=CARTESIAN_POINT('Ctrl Pts',(-111.221431157841,5.08259158390449,
127.238911592946));
#250609=CARTESIAN_POINT('Ctrl Pts',(-111.499878781655,-0.252448342873548,
124.601020082813));
#250610=CARTESIAN_POINT('Ctrl Pts',(-111.778326405467,-5.3555005753377,
127.663695474083));
#250611=CARTESIAN_POINT('Ctrl Pts',(-112.05677402928,-5.53710940981492,
133.612488702192));
#250612=CARTESIAN_POINT('Ctrl Pts',(-112.335221653093,-0.630385199504834,
136.980749405212));
#250613=CARTESIAN_POINT('Ctrl Pts',(-112.613669276906,4.85563221312083,
134.673210545752));
#250614=CARTESIAN_POINT('Ctrl Pts',(-112.892116900719,5.8795608327098,128.810387606114));
#250615=CARTESIAN_POINT('Ctrl Pts',(-113.170564524532,1.50046027955312,
124.779928453004));
#250616=CARTESIAN_POINT('Ctrl Pts',(-113.449012148345,-4.25748996895278,
126.285628149252));
#250617=CARTESIAN_POINT('Ctrl Pts',(-113.727459772158,-6.10301492593933,
131.943822231527));
#250618=CARTESIAN_POINT('Ctrl Pts',(-114.00590739597,-2.3401673148416,136.554906756366));
#250619=CARTESIAN_POINT('Ctrl Pts',(-114.284355019783,3.57317973506622,
135.881520309444));
#250620=CARTESIAN_POINT('Ctrl Pts',(-114.562802643596,6.202949167983,130.542472138726));
#250621=CARTESIAN_POINT('Ctrl Pts',(-114.841250267409,3.13251134643626,
125.444086686097));
#250622=CARTESIAN_POINT('Ctrl Pts',(-115.119697891222,-2.81655137079845,
125.271531112549));
#250623=CARTESIAN_POINT('Ctrl Pts',(-115.398145515035,-6.17734097445314,
130.183375560363));
#250624=CARTESIAN_POINT('Ctrl Pts',(-115.676593138848,-3.86145600246928,
135.665874938939));
#250625=CARTESIAN_POINT('Ctrl Pts',(-115.955040762661,2.00291839317105,
136.680880154352));
#250626=CARTESIAN_POINT('Ctrl Pts',(-116.233488386474,6.02670863349017,
132.295650999397));
#250627=CARTESIAN_POINT('Ctrl Pts',(-116.511936010287,4.51224806071678,
126.539998837124));
#250628=CARTESIAN_POINT('Ctrl Pts',(-116.790383634099,-1.14874804428301,
124.703086825424));
#250629=CARTESIAN_POINT('Ctrl Pts',(-117.068831257912,-5.75410081604829,
128.472947364906));
#250630=CARTESIAN_POINT('Ctrl Pts',(-117.347278881725,-5.07171604131793,
134.385262787713));
#250631=CARTESIAN_POINT('Ctrl Pts',(-117.625726505538,0.271328008281021,
137.006904052952));
#250632=CARTESIAN_POINT('Ctrl Pts',(-117.904174129351,5.3650348733795,133.928710912162));
#250633=CARTESIAN_POINT('Ctrl Pts',(-118.182621753164,5.52853678636705,
127.979392483636));
#250634=CARTESIAN_POINT('Ctrl Pts',(-118.461069376977,0.611583476719488,
124.626081762825));
#250635=CARTESIAN_POINT('Ctrl Pts',(-118.73951700079,-4.86738517051901,
126.95030748382));
#250636=CARTESIAN_POINT('Ctrl Pts',(-119.017964624603,-5.87346463103546,
132.816219753764));
#250637=CARTESIAN_POINT('Ctrl Pts',(-119.296412248415,-1.48211703032935,
136.833331762325));
#250638=CARTESIAN_POINT('Ctrl Pts',(-119.574859872228,4.27122371580729,
135.310113820466));
#250639=CARTESIAN_POINT('Ctrl Pts',(-119.853307496041,6.09951852799569,
129.646328803424));
#250640=CARTESIAN_POINT('Ctrl Pts',(-120.131755119854,2.32265379100196,
125.046718450578));
#250641=CARTESIAN_POINT('Ctrl Pts',(-120.410202743667,-3.58861631197691,
125.738099972737));
#250642=CARTESIAN_POINT('Ctrl Pts',(-120.68865036748,-6.20212333790203,
131.085127526901));
#250643=CARTESIAN_POINT('Ctrl Pts',(-120.967097991293,-3.11618200686478,
136.174144007612));
#250644=CARTESIAN_POINT('Ctrl Pts',(-121.245545615105,2.83337835452712,
136.328591881372));
#250645=CARTESIAN_POINT('Ctrl Pts',(-121.523993238919,6.17920242633619,
131.406541097396));
#250646=CARTESIAN_POINT('Ctrl Pts',(-121.802440862731,3.84664133916317,
125.931115870606));
#250647=CARTESIAN_POINT('Ctrl Pts',(-122.080888486544,-2.02079521982502,
124.933964495032));
#250648=CARTESIAN_POINT('Ctrl Pts',(-122.359336110357,-6.03121969312815,
129.331420371272));
#250649=CARTESIAN_POINT('Ctrl Pts',(-122.63778373417,-4.49924790990888,
135.082436376724));
#250650=CARTESIAN_POINT('Ctrl Pts',(-122.916231357983,1.16731290203685,
136.90210975513));
#250651=CARTESIAN_POINT('Ctrl Pts',(-123.194678981796,5.76117018341619,
133.118249567719));
#250652=CARTESIAN_POINT('Ctrl Pts',(-123.473126605609,5.06079351504635,
127.208038474877));
#250653=CARTESIAN_POINT('Ctrl Pts',(-123.751574229422,-0.290205160143283,
124.602671741062));
#250654=CARTESIAN_POINT('Ctrl Pts',(-124.030021853235,-5.37451947047147,
127.696354115408));
#250655=CARTESIAN_POINT('Ctrl Pts',(-124.308469477047,-5.51991294730918,
133.646142630679));
#250656=CARTESIAN_POINT('Ctrl Pts',(-124.58691710086,-0.592776088308802,
136.984472304668));
#250657=CARTESIAN_POINT('Ctrl Pts',(-124.865364724673,4.87909303712557,
134.64358125345));
#250658=CARTESIAN_POINT('Ctrl Pts',(-125.143812348486,5.86731401838748,
128.774633994209));
#250659=CARTESIAN_POINT('Ctrl Pts',(-125.422259972299,1.46376005097626,
124.770906344175));
#250660=CARTESIAN_POINT('Ctrl Pts',(-125.700707596112,-4.28491789462882,
126.311628420759));
#250661=CARTESIAN_POINT('Ctrl Pts',(-125.979155219925,-6.09596562494584,
131.980951904039));
#250662=CARTESIAN_POINT('Ctrl Pts',(-126.257602843738,-2.30511875041471,
136.569045474729));
#250663=CARTESIAN_POINT('Ctrl Pts',(-126.536050467551,3.60401964443632,
135.859675282198));
#250664=CARTESIAN_POINT('Ctrl Pts',(-126.814498091363,6.20124005219796,
130.50471787872));
#250665=CARTESIAN_POINT('Ctrl Pts',(-127.092945715177,3.09982379940838,
125.42511751388));
#250666=CARTESIAN_POINT('Ctrl Pts',(-127.371393338989,-2.85017909022625,
125.288778770691));
#250667=CARTESIAN_POINT('Ctrl Pts',(-127.649840962802,-6.18100663493216,
130.220990293627));
#250668=CARTESIAN_POINT('Ctrl Pts',(-127.928288586615,-3.83179104109667,
135.689290645038));
#250669=CARTESIAN_POINT('Ctrl Pts',(-128.206736210428,2.03865332610762,
136.6685789433));
#250670=CARTESIAN_POINT('Ctrl Pts',(-128.485183834241,6.03567488037103,
132.258937083203));
#250671=CARTESIAN_POINT('Ctrl Pts',(-128.763631458054,4.48620607868298,
126.512610511197));
#250672=CARTESIAN_POINT('Ctrl Pts',(-129.042079081867,-1.18586694596332,
124.710192623294));
#250673=CARTESIAN_POINT('Ctrl Pts',(-129.32052670568,-5.76818618009069,
128.508017405469));
#250674=CARTESIAN_POINT('Ctrl Pts',(-129.598974329492,-5.04982410627509,
134.416069416958));
#250675=CARTESIAN_POINT('Ctrl Pts',(-129.877421953305,0.30907962358457,
137.005137483589));
#250676=CARTESIAN_POINT('Ctrl Pts',(-130.155869577118,5.38395427874936,
133.895994535135));
#250677=CARTESIAN_POINT('Ctrl Pts',(-130.434317200931,5.51123797253198,
127.945791051148));
#250678=CARTESIAN_POINT('Ctrl Pts',(-130.712764824744,0.573963208500954,
124.622473349811));
#250679=CARTESIAN_POINT('Ctrl Pts',(-130.991212448557,-4.89075570448117,
126.980008045559));
#250680=CARTESIAN_POINT('Ctrl Pts',(-131.26966007237,-5.8611090517438,132.851935924971));
#250681=CARTESIAN_POINT('Ctrl Pts',(-131.548107696183,-1.44538951154951,
136.842242126491));
#250682=CARTESIAN_POINT('Ctrl Pts',(-131.826555319995,4.29857237855583,
135.28403018822));
#250683=CARTESIAN_POINT('Ctrl Pts',(-132.105002943808,6.09235624970348,
129.609220758541));
#250684=CARTESIAN_POINT('Ctrl Pts',(-132.383450567622,2.28756235552218,
125.032686473479));
#250685=CARTESIAN_POINT('Ctrl Pts',(-132.661898191434,-3.6193895897498,
125.760038764874));
#250686=CARTESIAN_POINT('Ctrl Pts',(-132.940345815247,-6.20029931905343,
131.122876410071));
#250687=CARTESIAN_POINT('Ctrl Pts',(-133.21879343906,-3.08343687560774,
136.193013602317));
#250688=CARTESIAN_POINT('Ctrl Pts',(-133.497241062873,2.86695342225543,
136.311241951909));
#250689=CARTESIAN_POINT('Ctrl Pts',(-133.775688686686,6.18275358352724,
131.368915381349));
#250690=CARTESIAN_POINT('Ctrl Pts',(-134.054136310499,3.81690524584148,
125.907790562906));
#250691=CARTESIAN_POINT('Ctrl Pts',(-134.332583934311,-2.05649254658467,
124.946374413949));
#250692=CARTESIAN_POINT('Ctrl Pts',(-134.611031558124,-6.04007415394596,
129.36816140758));
#250693=CARTESIAN_POINT('Ctrl Pts',(-134.889479181937,-4.47312268785726,
135.109745312956));
#250694=CARTESIAN_POINT('Ctrl Pts',(-135.16792680575,1.20441000418008,136.894891013003));
#250695=CARTESIAN_POINT('Ctrl Pts',(-135.446374429563,5.775148741076,133.083136818595));
#250696=CARTESIAN_POINT('Ctrl Pts',(-135.724822053376,5.03880791662344,
127.177298619846));
#250697=CARTESIAN_POINT('Ctrl Pts',(-136.003269677189,-0.327951223754644,
124.604553205172));
#250698=CARTESIAN_POINT('Ctrl Pts',(-136.281717301002,-5.39333921080989,
127.729127925058));
#250699=CARTESIAN_POINT('Ctrl Pts',(-136.560164924815,-5.50251194239939,
133.679691255889));
#250700=CARTESIAN_POINT('Ctrl Pts',(-136.838612548628,-0.555145011576188,
136.987966197812));
#250701=CARTESIAN_POINT('Ctrl Pts',(-137.117060172441,4.90237306454367,
134.613809697415));
#250702=CARTESIAN_POINT('Ctrl Pts',(-137.395507796253,5.8548497885868,128.73895559457));
#250703=CARTESIAN_POINT('Ctrl Pts',(-137.673955420066,1.42700558223168,
124.762107807213));
#250704=CARTESIAN_POINT('Ctrl Pts',(-137.952403043879,-4.3121870410957,
126.33779517211));
#250705=CARTESIAN_POINT('Ctrl Pts',(-138.230850667692,-6.08869043570493,
132.018037977528));
#250706=CARTESIAN_POINT('Ctrl Pts',(-138.509298291505,-2.26998476896503,
136.582970580575));
#250707=CARTESIAN_POINT('Ctrl Pts',(-138.787745915318,3.63472600553235,
135.837642928407));
#250708=CARTESIAN_POINT('Ctrl Pts',(-139.066193539131,6.1993011471828,130.466974722087));
#250709=CARTESIAN_POINT('Ctrl Pts',(-139.344641162943,3.06702138726935,
125.406347671494));
#250710=CARTESIAN_POINT('Ctrl Pts',(-139.623088786757,-2.88370119522,125.306230810748));
#250711=CARTESIAN_POINT('Ctrl Pts',(-139.901536410569,-6.18444325593727,
130.258626643894));
#250712=CARTESIAN_POINT('Ctrl Pts',(-140.179984034382,-3.80198409129777,
135.712525338258));
#250713=CARTESIAN_POINT('Ctrl Pts',(-140.458431658195,2.07431271599591,
136.656060431482));
#250714=CARTESIAN_POINT('Ctrl Pts',(-140.736879282008,6.04441747309895,
132.222169267145));
#250715=CARTESIAN_POINT('Ctrl Pts',(-141.015326905821,4.45999785863389,
126.485381217648));
#250716=CARTESIAN_POINT('Ctrl Pts',(-141.293774529634,-1.22294190490765,
124.717524242802));
#250717=CARTESIAN_POINT('Ctrl Pts',(-141.572222153447,-5.78205780187226,
128.543172537875));
#250718=CARTESIAN_POINT('Ctrl Pts',(-141.85066977726,-5.02774504814366,
134.446742213005));
#250719=CARTESIAN_POINT('Ctrl Pts',(-142.129117401072,0.346819785828787,
137.003141142159));
#250720=CARTESIAN_POINT('Ctrl Pts',(-142.407565024885,5.40267417971275,
133.863163596476));
#250721=CARTESIAN_POINT('Ctrl Pts',(-142.686012648698,5.49373493774783,
127.912295544006));
#250722=CARTESIAN_POINT('Ctrl Pts',(-142.964460272511,0.536321671864061,
124.619094008905));
#250723=CARTESIAN_POINT('Ctrl Pts',(-143.242907896324,-4.91394500969209,
127.00985032009));
#250724=CARTESIAN_POINT('Ctrl Pts',(-143.521355520137,-5.84853628690073,
132.887576222521));
#250725=CARTESIAN_POINT('Ctrl Pts',(-143.79980314395,-1.40860843332932,
136.850928754739));
#250726=CARTESIAN_POINT('Ctrl Pts',(-144.078250767763,4.32576175612421,
135.257780560169));
#250727=CARTESIAN_POINT('Ctrl Pts',(-144.356698391576,6.08496821690962,
129.572157000006));
#250728=CARTESIAN_POINT('Ctrl Pts',(-144.635146015388,2.2523861535788,125.018868367886));
#250729=CARTESIAN_POINT('Ctrl Pts',(-144.913593639201,-3.65002874971022,
125.782164476213));
#250730=CARTESIAN_POINT('Ctrl Pts',(-145.192041263014,-6.19824554583293,
131.160613490521));
#250731=CARTESIAN_POINT('Ctrl Pts',(-145.470488886827,-3.05057748646412,
136.211683518503));
#250732=CARTESIAN_POINT('Ctrl Pts',(-145.74893651064,2.90042225397064,136.293687962933));
#250733=CARTESIAN_POINT('Ctrl Pts',(-146.027384134453,6.18607563651005,
131.33126874552));
#250734=CARTESIAN_POINT('Ctrl Pts',(-146.305831758266,3.78702771569254,
125.884646699409));
#250735=CARTESIAN_POINT('Ctrl Pts',(-146.584279382079,-2.09211366925746,
124.959001402698));
#250736=CARTESIAN_POINT('Ctrl Pts',(-146.862727005891,-6.04870479759444,
129.404955662777));
#250737=CARTESIAN_POINT('Ctrl Pts',(-147.141174629705,-4.4468317125993,
135.136894711575));
#250738=CARTESIAN_POINT('Ctrl Pts',(-147.419622253517,1.24146247646836,
136.887446584034));
#250739=CARTESIAN_POINT('Ctrl Pts',(-147.69806987733,5.78891329847519,133.04793962858));
#250740=CARTESIAN_POINT('Ctrl Pts',(-147.976517501143,5.01663560332014,
127.146693166932));
#250741=CARTESIAN_POINT('Ctrl Pts',(-148.254965124956,-0.365685135012239,
124.606664405427));
#250742=CARTESIAN_POINT('Ctrl Pts',(-148.533412748769,-5.41195909898036,
127.762015688586));
#250743=CARTESIAN_POINT('Ctrl Pts',(-148.811860372582,-5.48490703988586,
133.713133334664));
#250744=CARTESIAN_POINT('Ctrl Pts',(-149.090307996395,-0.517493363741682,
136.991230955176));
#250745=CARTESIAN_POINT('Ctrl Pts',(-149.368755620208,4.92547143272535,
134.583896980843));
#250746=CARTESIAN_POINT('Ctrl Pts',(-149.647203244021,5.84216860517359,
128.703353729273));
#250747=CARTESIAN_POINT('Ctrl Pts',(-149.925650867833,1.39019823527075,
124.753533168151));
#250748=CARTESIAN_POINT('Ctrl Pts',(-150.204098491647,-4.33929639788676,
126.364127433687));
#250749=CARTESIAN_POINT('Ctrl Pts',(-150.482546115459,-6.08118962780021,
132.055079077756));
#250750=CARTESIAN_POINT('Ctrl Pts',(-150.760993739272,-2.23476667239474,
136.596681557904));
#250751=CARTESIAN_POINT('Ctrl Pts',(-151.039441363085,3.66529768052036,
135.81542406449));
#250752=CARTESIAN_POINT('Ctrl Pts',(-151.317888986898,6.19713252478332,
130.429244067412));
#250753=CARTESIAN_POINT('Ctrl Pts',(-151.596336610711,3.03410532552526,
125.387777854462));
#250754=CARTESIAN_POINT('Ctrl Pts',(-151.874784234524,-2.91711644360522,
125.323886586026));
#250755=CARTESIAN_POINT('Ctrl Pts',(-152.153231858337,-6.18765071012318,
130.296283216534));
#250756=CARTESIAN_POINT('Ctrl Pts',(-152.431679482149,-3.77203625758034,
135.735578157629));
#250757=CARTESIAN_POINT('Ctrl Pts',(-152.710127105962,2.10989524146327,
136.643325082775));
#250758=CARTESIAN_POINT('Ctrl Pts',(-152.988574729775,6.0529360877152,132.185348913665));
#250759=CARTESIAN_POINT('Ctrl Pts',(-153.267022353588,4.43362437172323,
126.458311965469));
#250760=CARTESIAN_POINT('Ctrl Pts',(-153.545469977401,-1.25997154729018,
124.725081412269));
#250761=CARTESIAN_POINT('Ctrl Pts',(-153.823917601214,-5.79571516737629,
128.578411459437));
#250762=CARTESIAN_POINT('Ctrl Pts',(-154.102365225027,-5.00547968506979,
134.477280039263));
#250763=CARTESIAN_POINT('Ctrl Pts',(-154.38081284884,0.38454709653853,137.000915102638));
#250764=CARTESIAN_POINT('Ctrl Pts',(-154.659260472653,5.4211938825983,133.830219312748));
#250765=CARTESIAN_POINT('Ctrl Pts',(-154.937708096465,5.47602833059452,
127.8789072034));
#250766=CARTESIAN_POINT('Ctrl Pts',(-155.216155720278,0.498660261630971,
124.615943865326));
#250767=CARTESIAN_POINT('Ctrl Pts',(-155.494603344091,-4.93695222686361,
127.039833201595));
#250768=CARTESIAN_POINT('Ctrl Pts',(-155.773050967904,-5.83574680239484,
132.923139325752));
#250769=CARTESIAN_POINT('Ctrl Pts',(-156.051498591717,-1.37177515860606,
136.85939132518));
#250770=CARTESIAN_POINT('Ctrl Pts',(-156.32994621553,4.3527908409998,135.231365909006));
#250771=CARTESIAN_POINT('Ctrl Pts',(-156.608393839343,6.0773547033811,129.535138901228));
#250772=CARTESIAN_POINT('Ctrl Pts',(-156.886841463156,2.21712648863745,
125.005264645838));
#250773=CARTESIAN_POINT('Ctrl Pts',(-157.165289086968,-3.68053265651321,
125.804476286877));
#250774=CARTESIAN_POINT('Ctrl Pts',(-157.443736710782,-6.19596209434481,
131.19833736989));
#250775=CARTESIAN_POINT('Ctrl Pts',(-157.722184334594,-3.0176050570491,
136.230153064351));
#250776=CARTESIAN_POINT('Ctrl Pts',(-158.000631958407,2.93378360947182,
136.275930564914));
#250777=CARTESIAN_POINT('Ctrl Pts',(-158.27907958222,6.18916846218569,131.293602584915));
#250778=CARTESIAN_POINT('Ctrl Pts',(-158.557527206033,3.7570098558391,125.861685137721));
#250779=CARTESIAN_POINT('Ctrl Pts',(-158.835974829846,-2.12765726788813,
124.971844993383));
#250780=CARTESIAN_POINT('Ctrl Pts',(-159.114422453659,-6.05711130426257,
129.44180177344));
#250781=CARTESIAN_POINT('Ctrl Pts',(-159.392870077472,-4.42037595835707,
135.163883566548));
#250782=CARTESIAN_POINT('Ctrl Pts',(-159.671317701285,1.27846894590735,
136.879776744077));
#250783=CARTESIAN_POINT('Ctrl Pts',(-159.949765325097,5.80246334556346,
133.01265930192));
#250784=CARTESIAN_POINT('Ctrl Pts',(-160.22821294891,4.9942773967397,127.116223250229));
#250785=CARTESIAN_POINT('Ctrl Pts',(-160.506660572723,-0.403405495673234,
124.609005263594));
#250786=CARTESIAN_POINT('Ctrl Pts',(-160.785108196536,-5.43037844501628,
127.795016187323));
#250787=CARTESIAN_POINT('Ctrl Pts',(-161.063555820349,-5.46709889212507,
133.746467627798));
#250788=CARTESIAN_POINT('Ctrl Pts',(-161.342003444162,-0.479822539999598,
136.994266455786));
#250789=CARTESIAN_POINT('Ctrl Pts',(-161.620451067975,4.94838728575097,
134.553844212161));
#250790=CARTESIAN_POINT('Ctrl Pts',(-161.898898691787,5.82927093805496,
128.66782971756));
#250791=CARTESIAN_POINT('Ctrl Pts',(-162.177346315601,1.35333937400316,
124.745182744726));
#250792=CARTESIAN_POINT('Ctrl Pts',(-162.455793939413,-4.36624496045326,
126.390624229737));
#250793=CARTESIAN_POINT('Ctrl Pts',(-162.734241563226,-6.07346347917808,
132.092073832152));
#250794=CARTESIAN_POINT('Ctrl Pts',(-163.012689187039,-2.19946576572379,
136.61017789865));
#250795=CARTESIAN_POINT('Ctrl Pts',(-163.291136810852,3.69573353655413,
135.793019513774));
#250796=CARTESIAN_POINT('Ctrl Pts',(-163.569584434665,6.19473426535967,
130.391527312818));
#250797=CARTESIAN_POINT('Ctrl Pts',(-163.848032058478,3.0010768338922,125.369408750896));
#250798=CARTESIAN_POINT('Ctrl Pts',(-164.126479682291,-2.95042359716811,
125.341745442286));
#250799=CARTESIAN_POINT('Ctrl Pts',(-164.404927306104,-6.19062887863655,
130.333958616169));
#250800=CARTESIAN_POINT('Ctrl Pts',(-164.683374929917,-3.74194864967208,
135.758448248921));
#250801=CARTESIAN_POINT('Ctrl Pts',(-164.961822553729,2.14539958398697,
136.630373369092));
#250802=CARTESIAN_POINT('Ctrl Pts',(-165.240270177542,6.06123040855813,
132.148477387157));
#250803=CARTESIAN_POINT('Ctrl Pts',(-165.518717801355,4.40708659523179,
126.431403757722));
#250804=CARTESIAN_POINT('Ctrl Pts',(-165.797165425168,-1.29695450096345,
124.732863851664));
#250805=CARTESIAN_POINT('Ctrl Pts',(-166.075613048981,-5.80915777052276,
128.613732864363));
#250806=CARTESIAN_POINT('Ctrl Pts',(-166.354060672794,-4.98302884210618,
134.50768176414));
#250807=CARTESIAN_POINT('Ctrl Pts',(-166.632508296607,0.422260157714416,
136.998459447511));
#250808=CARTESIAN_POINT('Ctrl Pts',(-166.91095592042,5.43951270115045,133.797162904712));
#250809=CARTESIAN_POINT('Ctrl Pts',(-167.189403544233,5.45811880719792,
127.845627266545));
#250810=CARTESIAN_POINT('Ctrl Pts',(-167.467851168046,0.460980373357943,
124.613023035806));
#250811=CARTESIAN_POINT('Ctrl Pts',(-167.746298791858,-4.95977650345479,
127.069955579048));
#250812=CARTESIAN_POINT('Ctrl Pts',(-168.024746415672,-5.822741072145,132.958623916859));
#250813=CARTESIAN_POINT('Ctrl Pts',(-168.303194039484,-1.33489105224939,
136.867629524233));
#250814=CARTESIAN_POINT('Ctrl Pts',(-168.581641663297,4.37965863161014,
135.204787213532));
#250815=CARTESIAN_POINT('Ctrl Pts',(-168.86008928711,6.06951599123876,129.498167833929));
#250816=CARTESIAN_POINT('Ctrl Pts',(-169.138536910923,2.18178466725943,
124.991875811423));
#250817=CARTESIAN_POINT('Ctrl Pts',(-169.416984534736,-3.71090017982492,
125.826973370093));
#250818=CARTESIAN_POINT('Ctrl Pts',(-169.695432158549,-6.19344904920226,
131.236046650305));
#250819=CARTESIAN_POINT('Ctrl Pts',(-169.973879782361,-2.98452080916978,
136.248421555465));
#250820=CARTESIAN_POINT('Ctrl Pts',(-170.252327406175,2.96703625254325,
136.257970415857));
#250821=CARTESIAN_POINT('Ctrl Pts',(-170.530775029987,6.19203194594742,
131.25591829527));
#250822=CARTESIAN_POINT('Ctrl Pts',(-170.8092226538,3.72685277860365,125.838906728691));
#250823=CARTESIAN_POINT('Ctrl Pts',(-171.087670277614,-2.16312202539704,
124.984904710079));
#250824=CARTESIAN_POINT('Ctrl Pts',(-171.366117901426,-6.06529336244348,
129.478698374222));
#250825=CARTESIAN_POINT('Ctrl Pts',(-171.644565525239,-4.39375640545797,
135.190710877796));
#250826=CARTESIAN_POINT('Ctrl Pts',(-171.923013149052,1.31542804121008,
136.871881777341));
#250827=CARTESIAN_POINT('Ctrl Pts',(-172.201460772865,5.81579838023838,
132.977297145939));
#250828=CARTESIAN_POINT('Ctrl Pts',(-172.479908396678,4.97173412537368,
127.085889998814));
#250829=CARTESIAN_POINT('Ctrl Pts',(-172.75835602049,-0.441110907994683,
124.611575692932));
#250830=CARTESIAN_POINT('Ctrl Pts',(-173.036803644304,-5.4485965663818,
127.828128198426));
#250831=CARTESIAN_POINT('Ctrl Pts',(-173.315251268116,-5.44908815900415,
133.779692900072));
#250832=CARTESIAN_POINT('Ctrl Pts',(-173.593698891929,-0.442133936257506,
136.997072587158));
#250833=CARTESIAN_POINT('Ctrl Pts',(-173.872146515742,4.97111977446672,
134.523652504987));
#250834=CARTESIAN_POINT('Ctrl Pts',(-174.150594139555,5.81615726515733,
128.632384875785));
#250835=CARTESIAN_POINT('Ctrl Pts',(-174.429041763368,1.31643036424716,
124.737056846366));
#250836=CARTESIAN_POINT('Ctrl Pts',(-174.707489387181,-4.39303173020782,
126.417284578411));
#250837=CARTESIAN_POINT('Ctrl Pts',(-174.985937010994,-6.06551227613263,
132.129020869861));
#250838=CARTESIAN_POINT('Ctrl Pts',(-175.264384634806,-2.16408335703982,
136.623459102702));
#250839=CARTESIAN_POINT('Ctrl Pts',(-175.542832258619,3.72603244582337,
135.770430106468));
#250840=CARTESIAN_POINT('Ctrl Pts',(-175.821279882432,6.19210645777918,
130.353825855915));
#250841=CARTESIAN_POINT('Ctrl Pts',(-176.099727506245,2.96793713625374,
125.351241041473));
#250842=CARTESIAN_POINT('Ctrl Pts',(-176.378175130058,-2.98362142169932,
125.359806717758));
#250843=CARTESIAN_POINT('Ctrl Pts',(-176.656622753871,-6.19337765112022,
130.371651446723));
#250844=CARTESIAN_POINT('Ctrl Pts',(-176.935070377684,-3.71172238248064,
135.781134764673));
#250845=CARTESIAN_POINT('Ctrl Pts',(-177.213518001496,2.18082442793968,
136.617205770365));
#250846=CARTESIAN_POINT('Ctrl Pts',(-177.49196562531,6.06930012827989,132.111556053907));
#250847=CARTESIAN_POINT('Ctrl Pts',(-177.770413249122,4.38038551252508,
126.404657591498));
#250848=CARTESIAN_POINT('Ctrl Pts',(-178.048860872936,-1.33388939551094,
124.740871272604));
#250849=CARTESIAN_POINT('Ctrl Pts',(-178.327308496748,-5.82238511319243,
128.649135443807));
#250850=CARTESIAN_POINT('Ctrl Pts',(-178.605756120561,-4.96039335117553,
134.537946261091));
#250851=CARTESIAN_POINT('Ctrl Pts',(-178.884203744374,0.459957571884186,
136.995774267775));
#250852=CARTESIAN_POINT('Ctrl Pts',(-179.162651368187,5.45762995655925,
133.763995597288));
#250853=CARTESIAN_POINT('Ctrl Pts',(-179.441098991999,5.44000703120181,
127.812456966643));
#250854=CARTESIAN_POINT('Ctrl Pts',(-179.719546615813,0.423283403288203,
124.610331628578));
#250855=CARTESIAN_POINT('Ctrl Pts',(-179.997994239625,-4.98241699370369,
127.100216336253));
#250856=CARTESIAN_POINT('Ctrl Pts',(-180.276441863438,-5.80951957808352,
132.994028680947));
#250857=CARTESIAN_POINT('Ctrl Pts',(-180.554889487251,-1.29795748101432,
136.875643046625));
#250858=CARTESIAN_POINT('Ctrl Pts',(-180.833337111064,4.40636413235919,
135.178045458633));
#250859=CARTESIAN_POINT('Ctrl Pts',(-181.111784734877,6.06145237094964,
129.461245168083));
#250860=CARTESIAN_POINT('Ctrl Pts',(-181.39023235869,2.14636199904753,124.97870236077));
#250861=CARTESIAN_POINT('Ctrl Pts',(-181.668679982503,-3.74113019436597,
125.849654892224));
#250862=CARTESIAN_POINT('Ctrl Pts',(-181.947127606316,-6.19070650352801,
131.273739934436));
#250863=CARTESIAN_POINT('Ctrl Pts',(-182.225575230128,-2.95132596877351,
136.266488314898));
#250864=CARTESIAN_POINT('Ctrl Pts',(-182.504022853942,3.00017895099442,
136.239808181284));
#250865=CARTESIAN_POINT('Ctrl Pts',(-182.782470477755,6.19466598168877,
131.218217272988));
#250866=CARTESIAN_POINT('Ctrl Pts',(-183.060918101567,3.6965576014681,125.81631231638));
#250867=CARTESIAN_POINT('Ctrl Pts',(-183.33936572538,-2.19850662762309,
124.998180068855));
#250868=CARTESIAN_POINT('Ctrl Pts',(-183.617813349193,-6.07325066894868,
129.515644097905));
#250869=CARTESIAN_POINT('Ctrl Pts',(-183.896260973006,-4.36697404029963,
135.217375651221));
#250870=CARTESIAN_POINT('Ctrl Pts',(-184.174708596819,1.35233839284232,
136.863761976378));
#250871=CARTESIAN_POINT('Ctrl Pts',(-184.453156220632,5.8289179083658,132.941854470998));
#250872=CARTESIAN_POINT('Ctrl Pts',(-184.731603844444,4.94900662457131,
127.055694536694));
#250873=CARTESIAN_POINT('Ctrl Pts',(-185.010051468258,-0.478799974789776,
124.614375598192));
#250874=CARTESIAN_POINT('Ctrl Pts',(-185.28849909207,-5.46661278799793,
127.861350494915));
#250875=CARTESIAN_POINT('Ctrl Pts',(-185.566946715884,-5.43087550791776,
133.812807920317));
#250876=CARTESIAN_POINT('Ctrl Pts',(-185.845394339696,-0.404428949079144,
136.999649245311));
#250877=CARTESIAN_POINT('Ctrl Pts',(-186.123841963509,4.99366805651034,
134.493322978084));
#250878=CARTESIAN_POINT('Ctrl Pts',(-186.402289587322,5.80282807241402,
128.59702051737));
#250879=CARTESIAN_POINT('Ctrl Pts',(-186.680737211135,1.27947257368013,
124.729155774178));
#250880=CARTESIAN_POINT('Ctrl Pts',(-186.959184834948,-4.41965571455532,
126.444107491802));
#250881=CARTESIAN_POINT('Ctrl Pts',(-187.237632458761,-6.0573363132998,
132.165918821797));
#250882=CARTESIAN_POINT('Ctrl Pts',(-187.516080082574,-2.12862075745111,
136.636524677919));
#250883=CARTESIAN_POINT('Ctrl Pts',(-187.794527706387,3.75619328558978,
135.74765667963));
#250884=CARTESIAN_POINT('Ctrl Pts',(-188.072975330199,6.18924919941703,
130.316141093742));
#250885=CARTESIAN_POINT('Ctrl Pts',(-188.351422954013,2.93468746061294,
125.333275399398));
#250886=CARTESIAN_POINT('Ctrl Pts',(-188.629870577825,-3.01670868704181,
125.378069743179));
#250887=CARTESIAN_POINT('Ctrl Pts',(-188.908318201638,-6.19589692571743,
130.409360311474));
#250888=CARTESIAN_POINT('Ctrl Pts',(-189.186765825451,-3.68135857605119,
135.80363686423));
#250889=CARTESIAN_POINT('Ctrl Pts',(-189.465213449264,2.21616846064164,
136.603822774524));
#250890=CARTESIAN_POINT('Ctrl Pts',(-189.743661073077,6.07714494785282,
132.07458628205));
#250891=CARTESIAN_POINT('Ctrl Pts',(-190.02210869689,4.35352211302309,126.378074457888));
#250892=CARTESIAN_POINT('Ctrl Pts',(-190.300556320702,-1.37077486229612,
124.749103378371));
#250893=CARTESIAN_POINT('Ctrl Pts',(-190.579003944516,-5.83539670523986,
128.684617885911));
#250894=CARTESIAN_POINT('Ctrl Pts',(-190.857451568328,-4.93757405104588,
134.568072408653));
#250895=CARTESIAN_POINT('Ctrl Pts',(-191.135899192141,0.497637942157669,
136.992859662928));
#250896=CARTESIAN_POINT('Ctrl Pts',(-191.414346815954,5.47554497748281,
133.730718619501));
#250897=CARTESIAN_POINT('Ctrl Pts',(-191.692794439767,5.42169367374449,
127.779397532831));
#250898=CARTESIAN_POINT('Ctrl Pts',(-191.97124206358,0.385570748295746,
124.60786974337));
#250899=CARTESIAN_POINT('Ctrl Pts',(-192.249689687393,-5.00487285865859,
127.130614351886));
#250900=CARTESIAN_POINT('Ctrl Pts',(-192.528137311206,-5.79608281013753,
133.029352306079));
#250901=CARTESIAN_POINT('Ctrl Pts',(-192.806584935019,-1.26097581348702,
136.883431595415));
#250902=CARTESIAN_POINT('Ctrl Pts',(-193.085032558831,4.43290635366497,
135.151141635234));
#250903=CARTESIAN_POINT('Ctrl Pts',(-193.363480182644,6.05316414131348,
129.424372271875));
#250904=CARTESIAN_POINT('Ctrl Pts',(-193.641927806457,2.11085979660312,
124.965744782026));
#250905=CARTESIAN_POINT('Ctrl Pts',(-193.92037543027,-3.77122157995168,
125.872520012798));
#250906=CARTESIAN_POINT('Ctrl Pts',(-194.198823054083,-6.1877345589472,
131.311415825543));
#250907=CARTESIAN_POINT('Ctrl Pts',(-194.477270677896,-2.91802176590892,
136.284352673182));
#250908=CARTESIAN_POINT('Ctrl Pts',(-194.755718301709,3.03321047671203,
136.221444534203));
#250909=CARTESIAN_POINT('Ctrl Pts',(-195.034165925522,6.19707047180361,
131.180500915096));
#250910=CARTESIAN_POINT('Ctrl Pts',(-195.312613549334,3.66612544703105,
125.793902738034));
#250911=CARTESIAN_POINT('Ctrl Pts',(-195.591061173148,-2.23380976337827,
125.011670577786));
#250912=CARTESIAN_POINT('Ctrl Pts',(-195.86950879696,-6.08098292891658,
129.552637575454));
#250913=CARTESIAN_POINT('Ctrl Pts',(-196.147956420774,-4.3400298553121,
135.243876898752));
#250914=CARTESIAN_POINT('Ctrl Pts',(-196.426404044586,1.38919863307876,
136.855417642068));
#250915=CARTESIAN_POINT('Ctrl Pts',(-196.704851668399,5.84182144379631,
132.906332590435));
#250916=CARTESIAN_POINT('Ctrl Pts',(-196.983299292212,4.92609573650846,
127.025637982775));
#250917=CARTESIAN_POINT('Ctrl Pts',(-197.261746916025,-0.516471299475173,
124.617404875624));
#250918=CARTESIAN_POINT('Ctrl Pts',(-197.540194539838,-5.48442644226676,
127.894681845726));
#250919=CARTESIAN_POINT('Ctrl Pts',(-197.81864216365,-5.41246161374207,
133.845811461438));
#250920=CARTESIAN_POINT('Ctrl Pts',(-198.097089787464,-0.36670897563802,
137.001996334766));
#250921=CARTESIAN_POINT('Ctrl Pts',(-198.375537411276,5.01603129634849,
134.462856755322));
#250922=CARTESIAN_POINT('Ctrl Pts',(-198.65398503509,5.78928385374183,128.561737952753));
#250923=CARTESIAN_POINT('Ctrl Pts',(-198.932432658902,1.24246737178614,
124.721479820939));
#250924=CARTESIAN_POINT('Ctrl Pts',(-199.210880282716,-4.44611592693577,
126.471091975977));
#250925=CARTESIAN_POINT('Ctrl Pts',(-199.489327906528,-6.04893589364168,
132.202766320694));
#250926=CARTESIAN_POINT('Ctrl Pts',(-199.767775530341,-2.09307928103787,
136.649374140152));
#250927=CARTESIAN_POINT('Ctrl Pts',(-200.046223154153,3.7862149382325,135.724700077139));
#250928=CARTESIAN_POINT('Ctrl Pts',(-200.324670777967,6.18616259614969,
130.278474422724));
#250929=CARTESIAN_POINT('Ctrl Pts',(-200.603118401779,2.90132903904936,
125.315512490399));
#250930=CARTESIAN_POINT('Ctrl Pts',(-200.881566025592,-3.04968416713424,
125.396533841802));
#250931=CARTESIAN_POINT('Ctrl Pts',(-201.160013649405,-6.1981866090755,
130.447083813107));
#250932=CARTESIAN_POINT('Ctrl Pts',(-201.438461273218,-3.65085835552605,
135.825953713766));
#250933=CARTESIAN_POINT('Ctrl Pts',(-201.716908897031,2.2514303724059,136.590224877478));
#250934=CARTESIAN_POINT('Ctrl Pts',(-201.995356520844,6.08476457658541,
132.037569441512));
#250935=CARTESIAN_POINT('Ctrl Pts',(-202.273804144657,4.32649739215744,
126.35165534194));
#250936=CARTESIAN_POINT('Ctrl Pts',(-202.55225176847,-1.40760953451491,
124.757559863922));
#250937=CARTESIAN_POINT('Ctrl Pts',(-202.830699392283,-5.84819206451709,
128.720178875862));
#250938=CARTESIAN_POINT('Ctrl Pts',(-203.109147016096,-4.91457178729319,
134.59805909049));
#250939=CARTESIAN_POINT('Ctrl Pts',(-203.387594639908,0.535299872273523,
136.989715740974));
#250940=CARTESIAN_POINT('Ctrl Pts',(-203.666042263721,5.49325710007376,
133.697333204442));
#250941=CARTESIAN_POINT('Ctrl Pts',(-203.944489887534,5.40317941343439,
127.746450190138));
#250942=CARTESIAN_POINT('Ctrl Pts',(-204.222937511347,0.347843805837959,
124.605637471411));
#250943=CARTESIAN_POINT('Ctrl Pts',(-204.50138513516,-5.0271432662092,127.161148499539));
#250944=CARTESIAN_POINT('Ctrl Pts',(-204.779832758973,-5.78243126621161,
133.064593483327));
#250945=CARTESIAN_POINT('Ctrl Pts',(-205.058280382786,-1.22394742003769,
136.890994881994));
#250946=CARTESIAN_POINT('Ctrl Pts',(-205.336728006599,4.45928431199552,
135.124076740266));
#250947=CARTESIAN_POINT('Ctrl Pts',(-205.615175630412,6.04465160945437,
129.387550511641));
#250948=CARTESIAN_POINT('Ctrl Pts',(-205.893623254225,2.07527937547198,
124.953003555339));
#250949=CARTESIAN_POINT('Ctrl Pts',(-206.172070878037,-3.80117322153507,
125.89556788454));
#250950=CARTESIAN_POINT('Ctrl Pts',(-206.45051850185,-6.18453332558722,
131.349072927534));
#250951=CARTESIAN_POINT('Ctrl Pts',(-206.728966125663,-2.8846094346739,
136.302013968343));
#250952=CARTESIAN_POINT('Ctrl Pts',(-207.007413749476,3.06612960569919,
136.202880155086));
#250953=CARTESIAN_POINT('Ctrl Pts',(-207.285861373289,6.19924532719362,
131.142770619188));
#250954=CARTESIAN_POINT('Ctrl Pts',(-207.564308997102,3.63555744296752,
125.771678824048));
#250955=CARTESIAN_POINT('Ctrl Pts',(-207.842756620915,-2.26903012449045,
125.025375736976));
#250956=CARTESIAN_POINT('Ctrl Pts',(-208.121204244728,-6.08848985582611,
129.58967743606));
#250957=CARTESIAN_POINT('Ctrl Pts',(-208.399651868541,-4.31292484892225,
135.270213638376));
#250958=CARTESIAN_POINT('Ctrl Pts',(-208.678099492353,1.42600739604885,
136.846849083615));
#250959=CARTESIAN_POINT('Ctrl Pts',(-208.956547116166,5.85450850838505,
132.870732820528));
#250960=CARTESIAN_POINT('Ctrl Pts',(-209.234994739979,4.90300231015654,
126.995721450812));
#250961=CARTESIAN_POINT('Ctrl Pts',(-209.513442363792,-0.554123486127181,
124.620663412976));
#250962=CARTESIAN_POINT('Ctrl Pts',(-209.791889987605,-5.50203686909699,
127.928121015754));
#250963=CARTESIAN_POINT('Ctrl Pts',(-210.070337611418,-5.393847158811,133.878702300482));
#250964=CARTESIAN_POINT('Ctrl Pts',(-210.348785235231,-0.328975413660277,
137.004113768549));
#250965=CARTESIAN_POINT('Ctrl Pts',(-210.627232859043,5.03820866530154,
134.432254965643));
#250966=CARTESIAN_POINT('Ctrl Pts',(-210.905680482857,5.77552511102812,
128.526538489345));
#250967=CARTESIAN_POINT('Ctrl Pts',(-211.184128106669,1.20541612980698,
124.714029271085));
#250968=CARTESIAN_POINT('Ctrl Pts',(-211.462575730482,-4.47241138685473,
126.498237031013));
#250969=CARTESIAN_POINT('Ctrl Pts',(-211.741023354295,-6.04031132844015,
132.239562001151));
#250970=CARTESIAN_POINT('Ctrl Pts',(-212.019470978108,-2.05746024480169,
136.66200701326));
#250971=CARTESIAN_POINT('Ctrl Pts',(-212.297918601921,3.81609629128846,
135.701561149659));
#250972=CARTESIAN_POINT('Ctrl Pts',(-212.576366225734,6.1828467623524,130.240827238612));
#250973=CARTESIAN_POINT('Ctrl Pts',(-212.854813849547,2.86786310767097,
125.297952972686));
#250974=CARTESIAN_POINT('Ctrl Pts',(-213.133261473359,-3.0825466400586,
125.415198329437));
#250975=CARTESIAN_POINT('Ctrl Pts',(-213.411709097173,-6.20024661634941,
130.484820553763));
#250976=CARTESIAN_POINT('Ctrl Pts',(-213.690156720985,-3.62022285110177,
135.848084486325));
#250977=CARTESIAN_POINT('Ctrl Pts',(-213.968604344798,2.28660885659016,
136.576412583105));
#250978=CARTESIAN_POINT('Ctrl Pts',(-214.247051968611,6.09215873212836,
132.00050690397));
#250979=CARTESIAN_POINT('Ctrl Pts',(-214.525499592424,4.29931235134063,
126.325401222624));
#250980=CARTESIAN_POINT('Ctrl Pts',(-214.803947216237,-1.44439204724454,
124.766240415898));
#250981=CARTESIAN_POINT('Ctrl Pts',(-215.08239484005,-5.86077071688603,
128.755817095934));
#250982=CARTESIAN_POINT('Ctrl Pts',(-215.360842463863,-4.89138741227638,
134.627905195436));
#250983=CARTESIAN_POINT('Ctrl Pts',(-215.639290087675,0.572941966656434,
136.986342618411));
#250984=CARTESIAN_POINT('Ctrl Pts',(-215.917737711489,5.51076566800256,
133.66384058922));
#250985=CARTESIAN_POINT('Ctrl Pts',(-216.196185335301,5.38446493632399,
127.713616159441));
#250986=CARTESIAN_POINT('Ctrl Pts',(-216.474632959115,0.310103973899474,
124.603634895418));
#250987=CARTESIAN_POINT('Ctrl Pts',(-216.753080582927,-5.04922739111732,
127.191817647757));
#250988=CARTESIAN_POINT('Ctrl Pts',(-217.031528206741,-5.76856545216855,
133.099750906814));
#250989=CARTESIAN_POINT('Ctrl Pts',(-217.309975830553,-1.18687367276612,
136.898332626102));
#250990=CARTESIAN_POINT('Ctrl Pts',(-217.588423454366,4.48549702990607,
135.096851776628));
#250991=CARTESIAN_POINT('Ctrl Pts',(-217.866871078179,6.03591509080661,
129.350781251827));
#250992=CARTESIAN_POINT('Ctrl Pts',(-218.145318701992,2.03962205410111,
124.94047915284));
#250993=CARTESIAN_POINT('Ctrl Pts',(-218.423766325804,-3.83098400924668,
125.9187976534));
#250994=CARTESIAN_POINT('Ctrl Pts',(-218.702213949618,-6.18110292207006,
131.386709845009));
#250995=CARTESIAN_POINT('Ctrl Pts',(-218.98066157343,-2.85109021317626,
136.319471545938));
#250996=CARTESIAN_POINT('Ctrl Pts',(-219.259109197243,3.09893511812703,
136.18411573184));
#250997=CARTESIAN_POINT('Ctrl Pts',(-219.537556821056,6.20119046726778,
131.105027783371));
#250998=CARTESIAN_POINT('Ctrl Pts',(-219.816004444869,3.6048547219858,125.749641397935));
#250999=CARTESIAN_POINT('Ctrl Pts',(-220.094452068682,-2.30416640585769,
125.039295038577));
#251000=CARTESIAN_POINT('Ctrl Pts',(-220.372899692494,-6.09577117150464,
129.626762307198));
#251001=CARTESIAN_POINT('Ctrl Pts',(-220.651347316308,-4.28566002551621,
135.296384894171));
#251002=CARTESIAN_POINT('Ctrl Pts',(-220.929794940121,1.46276331779004,
136.83805661853));
#251003=CARTESIAN_POINT('Ctrl Pts',(-221.208242563933,5.86697863200795,
132.835056480438));
#251004=CARTESIAN_POINT('Ctrl Pts',(-221.486690187747,4.87972720125093,
126.965946049375));
#251005=CARTESIAN_POINT('Ctrl Pts',(-221.765137811559,-0.591755139529082,
124.624151089502));
#251006=CARTESIAN_POINT('Ctrl Pts',(-222.043585435373,-5.51944341592756,
127.961666765899));
#251007=CARTESIAN_POINT('Ctrl Pts',(-222.322033059185,-5.37503283288975,
133.911479218663));
#251008=CARTESIAN_POINT('Ctrl Pts',(-222.600480682998,-0.29122966137826,
137.006001468201));
#251009=CARTESIAN_POINT('Ctrl Pts',(-222.878928306811,5.06019934158045,
134.401518743003));
#251010=CARTESIAN_POINT('Ctrl Pts',(-223.157375930624,5.7615523541068,128.491423431472));
#251011=CARTESIAN_POINT('Ctrl Pts',(-223.435823554437,1.16832022068962,
124.706804400699));
#251012=CARTESIAN_POINT('Ctrl Pts',(-223.71427117825,-4.49854111992577,
126.525541651043));
#251013=CARTESIAN_POINT('Ctrl Pts',(-223.992718802062,-6.03146293728042,
132.276304499695));
#251014=CARTESIAN_POINT('Ctrl Pts',(-224.271166425875,-2.02176496861996,
136.674422829126));
#251015=CARTESIAN_POINT('Ctrl Pts',(-224.549614049688,3.84583623749284,
135.678240754614));
#251016=CARTESIAN_POINT('Ctrl Pts',(-224.828061673501,6.1793018208946,130.203200936436));
#251017=CARTESIAN_POINT('Ctrl Pts',(-225.106509297314,2.83429090657077,
125.280597496933));
#251018=CARTESIAN_POINT('Ctrl Pts',(-225.384956921127,-3.11529488808334,
125.434062514461));
#251019=CARTESIAN_POINT('Ctrl Pts',(-225.66340454494,-6.20207687120481,
130.522569135094));
#251020=CARTESIAN_POINT('Ctrl Pts',(-225.941852168753,-3.5894531979886,
135.87002836184));
#251021=CARTESIAN_POINT('Ctrl Pts',(-226.220299792565,2.32170260964191,
136.562386403224));
#251022=CARTESIAN_POINT('Ctrl Pts',(-226.498747416378,6.09932714048972,
131.963400042786));
#251023=CARTESIAN_POINT('Ctrl Pts',(-226.777195040191,4.27196799792278,
126.299313072794));
#251024=CARTESIAN_POINT('Ctrl Pts',(-227.055642664004,-1.48112103749588,
124.775144712639));
#251025=CARTESIAN_POINT('Ctrl Pts',(-227.334090287817,-5.87313219624144,
128.79153122554));
#251026=CARTESIAN_POINT('Ctrl Pts',(-227.61253791163,-4.8680217850994,134.65760961753));
#251027=CARTESIAN_POINT('Ctrl Pts',(-227.890985535443,0.610562830463375,
136.982740420231));
#251028=CARTESIAN_POINT('Ctrl Pts',(-228.169433159256,5.52807003248314,
133.630242014917));
#251029=CARTESIAN_POINT('Ctrl Pts',(-228.447880783069,5.36555093588535,
127.680896657417));
#251030=CARTESIAN_POINT('Ctrl Pts',(-228.726328406882,0.272352650944771,
124.601862089598));
#251031=CARTESIAN_POINT('Ctrl Pts',(-229.004776030695,-5.07112441504767,
127.222620660081));
#251032=CARTESIAN_POINT('Ctrl Pts',(-229.283223654507,-5.75448588181141,
133.134823273769));
#251033=CARTESIAN_POINT('Ctrl Pts',(-229.561671278321,-1.14975594545406,
136.905444555836));
#251034=CARTESIAN_POINT('Ctrl Pts',(-229.840118902133,4.51154353607471,
135.069467753152));
#251035=CARTESIAN_POINT('Ctrl Pts',(-230.118566525947,6.0269549091058,129.314065854931));
#251036=CARTESIAN_POINT('Ctrl Pts',(-230.397014149759,2.00388915378425,
124.928172038625));
#251037=CARTESIAN_POINT('Ctrl Pts',(-230.675461773572,-3.86065283843716,
125.942208458593));
#251038=CARTESIAN_POINT('Ctrl Pts',(-230.953909397385,-6.17744347551146,
131.424325183319));
#251039=CARTESIAN_POINT('Ctrl Pts',(-231.232357021197,-2.81746534348149,
136.33672475907));
#251040=CARTESIAN_POINT('Ctrl Pts',(-231.510804645011,3.13162579837364,
136.165151959792));
#251041=CARTESIAN_POINT('Ctrl Pts',(-231.789252268823,6.20290581994918,
131.067273806224));
#251042=CARTESIAN_POINT('Ctrl Pts',(-232.067699892636,3.57401842178686,
125.727791276302));
#251043=CARTESIAN_POINT('Ctrl Pts',(-232.346147516449,-2.33921730549066,
125.053427966802));
#251044=CARTESIAN_POINT('Ctrl Pts',(-232.624595140262,-6.10282660614105,
129.663890814674));
#251045=CARTESIAN_POINT('Ctrl Pts',(-232.903042764075,-4.25823639540172,
135.322389696357));
#251046=CARTESIAN_POINT('Ctrl Pts',(-233.181490387888,1.499465036299,136.829040572621));
#251047=CARTESIAN_POINT('Ctrl Pts',(-233.459938011701,5.87923135258013,
132.799304892167));
#251048=CARTESIAN_POINT('Ctrl Pts',(-233.738385635514,4.85627127225937,
126.9363128818));
#251049=CARTESIAN_POINT('Ctrl Pts',(-234.016833259326,-0.629364865227224,
124.627867775965));
#251050=CARTESIAN_POINT('Ctrl Pts',(-234.29528088314,-5.53664543775268,
127.99531785311));
#251051=CARTESIAN_POINT('Ctrl Pts',(-234.573728506952,-5.35601933315035,
133.944141001422));
#251052=CARTESIAN_POINT('Ctrl Pts',(-234.852176130765,-0.253473117473377,
137.007659363768));
#251053=CARTESIAN_POINT('Ctrl Pts',(-235.130623754578,5.08200251031112,
134.370649226346));
#251054=CARTESIAN_POINT('Ctrl Pts',(-235.409071378391,5.74736610074488,
128.456394080338));
#251055=CARTESIAN_POINT('Ctrl Pts',(-235.687519002204,1.13118101903705,
124.699805477501));
#251056=CARTESIAN_POINT('Ctrl Pts',(-235.965966626017,-4.52450415790052,
126.553004824284));
#251057=CARTESIAN_POINT('Ctrl Pts',(-236.24441424983,-6.0223910480441,132.312992454817));
#251058=CARTESIAN_POINT('Ctrl Pts',(-236.522861873642,-1.98599477519336,
136.686621127679));
#251059=CARTESIAN_POINT('Ctrl Pts',(-236.801309497456,3.87543367482126,
135.654739756147));
#251060=CARTESIAN_POINT('Ctrl Pts',(-237.079757121268,6.1755279031354,130.165596910454));
#251061=CARTESIAN_POINT('Ctrl Pts',(-237.358204745081,2.80061367977841,
125.263446706254));
#251062=CARTESIAN_POINT('Ctrl Pts',(-237.636652368894,-3.14792769771062,
125.453125697856));
#251063=CARTESIAN_POINT('Ctrl Pts',(-237.915099992707,-6.20367730582095,
130.560328158313));
#251064=CARTESIAN_POINT('Ctrl Pts',(-238.19354761652,-3.55855053636696,
135.891784527174));
#251065=CARTESIAN_POINT('Ctrl Pts',(-238.471995240333,2.35671033115007,
136.54814685758));
#251066=CARTESIAN_POINT('Ctrl Pts',(-238.750442864146,6.10626953604027,
131.92625023297));
#251067=CARTESIAN_POINT('Ctrl Pts',(-239.028890487959,4.24446534516054,
126.273391859158));
#251068=CARTESIAN_POINT('Ctrl Pts',(-239.307338111771,-1.51779514426229,
124.784272424193));
#251069=CARTESIAN_POINT('Ctrl Pts',(-239.585785735585,-5.88527604452282,
128.827319941278));
#251070=CARTESIAN_POINT('Ctrl Pts',(-239.864233359397,-4.84447577158576,
134.687171256065));
#251071=CARTESIAN_POINT('Ctrl Pts',(-240.14268098321,0.648161069640796,
136.978909279916));
#251072=CARTESIAN_POINT('Ctrl Pts',(-240.421128607023,5.54516955229552,
133.596538726537));
#251073=CARTESIAN_POINT('Ctrl Pts',(-240.699576230836,5.34643811298351,
127.648292896498));
#251074=CARTESIAN_POINT('Ctrl Pts',(-240.978023854649,0.234591235861842,
124.600319119639));
#251075=CARTESIAN_POINT('Ctrl Pts',(-241.256471478461,-5.09283352659785,
127.253556395099));
#251076=CARTESIAN_POINT('Ctrl Pts',(-241.534919102275,-5.74019307686353,
133.169809284574));
#251077=CARTESIAN_POINT('Ctrl Pts',(-241.813366726087,-1.11259561351327,
136.912330407661));
#251078=CARTESIAN_POINT('Ctrl Pts',(-242.0918143499,4.53742286533832,135.041925684563));
#251079=CARTESIAN_POINT('Ctrl Pts',(-242.370261973713,6.01777139637409,
129.277405681456));
#251080=CARTESIAN_POINT('Ctrl Pts',(-242.648709597526,1.96808199861856,
124.916082668738));
#251081=CARTESIAN_POINT('Ctrl Pts',(-242.927157221339,-3.89017860971679,
125.965799432623));
#251082=CARTESIAN_POINT('Ctrl Pts',(-243.205604845152,-6.1735551215127,
131.461917548614));
#251083=CARTESIAN_POINT('Ctrl Pts',(-243.484052468965,-2.78373607157309,
136.353772968415));
#251084=CARTESIAN_POINT('Ctrl Pts',(-243.762500092778,3.16420043507544,
136.145989541648));
#251085=CARTESIAN_POINT('Ctrl Pts',(-244.040947716591,6.20439132167383,
131.029510086731));
#251086=CARTESIAN_POINT('Ctrl Pts',(-244.319395340403,3.54304968502077,
125.706129268813));
#251087=CARTESIAN_POINT('Ctrl Pts',(-244.597842964216,-2.37418152456686,
125.067773997952));
#251088=CARTESIAN_POINT('Ctrl Pts',(-244.876290588029,-6.10965589829292,
129.701061582678));
#251089=CARTESIAN_POINT('Ctrl Pts',(-245.154738211842,-4.23065497477177,
135.348227081313));
#251090=CARTESIAN_POINT('Ctrl Pts',(-245.433185835655,1.53611119157916,
136.819801279981));
#251091=CARTESIAN_POINT('Ctrl Pts',(-245.711633459468,5.89126621607239,
132.763479380503));
#251092=CARTESIAN_POINT('Ctrl Pts',(-245.990081083281,4.83263539234992,
126.906823046158));
#251093=CARTESIAN_POINT('Ctrl Pts',(-246.268528707094,-0.666951269578287,
124.631813334641));
#251094=CARTESIAN_POINT('Ctrl Pts',(-246.546976330906,-5.55364229714491,
128.029073030433));
#251095=CARTESIAN_POINT('Ctrl Pts',(-246.825423954719,-5.33680736414475,
133.976686438464));
#251096=CARTESIAN_POINT('Ctrl Pts',(-247.103871578532,-0.215707181029578,
137.009087393821));
#251097=CARTESIAN_POINT('Ctrl Pts',(-247.382319202345,5.10361736357064,
134.339647559554));
#251098=CARTESIAN_POINT('Ctrl Pts',(-247.660766826158,5.73296687661779,
128.421451733968));
#251099=CARTESIAN_POINT('Ctrl Pts',(-247.939214449971,1.09399990105564,
124.693032760838));
#251100=CARTESIAN_POINT('Ctrl Pts',(-248.217662073784,-4.55029953871062,
126.580625533077));
#251101=CARTESIAN_POINT('Ctrl Pts',(-248.496109697597,-6.01309599689209,
132.349624507031));
#251102=CARTESIAN_POINT('Ctrl Pts',(-248.77455732141,-1.95015099000055,
136.698601456905));
#251103=CARTESIAN_POINT('Ctrl Pts',(-249.053004945222,3.90488750652966,
135.631059025098));
#251104=CARTESIAN_POINT('Ctrl Pts',(-249.331452569036,6.17152514891849,
130.128016554096));
#251105=CARTESIAN_POINT('Ctrl Pts',(-249.609900192848,2.76683267521693,
125.246501236177));
#251106=CARTESIAN_POINT('Ctrl Pts',(-249.888347816661,-3.18044385971988,
125.472387173231));
#251107=CARTESIAN_POINT('Ctrl Pts',(-250.166795440474,-6.20504786089197,
130.598096224241));
#251108=CARTESIAN_POINT('Ctrl Pts',(-250.445243064287,-3.5275160113489,
135.913352176149));
#251109=CARTESIAN_POINT('Ctrl Pts',(-250.7236906881,2.39163072389511,136.533694473816));
#251110=CARTESIAN_POINT('Ctrl Pts',(-251.002138311913,6.11298566151878,
131.889058851139));
#251111=CARTESIAN_POINT('Ctrl Pts',(-251.280585935725,4.21680541219097,
126.247638542206));
#251112=CARTESIAN_POINT('Ctrl Pts',(-251.559033559539,-1.5544130086051,
124.793623212388));
#251113=CARTESIAN_POINT('Ctrl Pts',(-251.837481183351,-5.89720181167361,
128.863181916876));
#251114=CARTESIAN_POINT('Ctrl Pts',(-252.115928807165,-4.82075024435922,
134.716589015834));
#251115=CARTESIAN_POINT('Ctrl Pts',(-252.394376430977,0.685735291195708,
136.974849339035));
#251116=CARTESIAN_POINT('Ctrl Pts',(-252.67282405479,5.56206359338632,133.562731973716));
#251117=CARTESIAN_POINT('Ctrl Pts',(-252.951271678603,5.32712717665345,
127.615806083426));
#251118=CARTESIAN_POINT('Ctrl Pts',(-253.229719302416,0.196821126400439,
124.599006045371));
#251119=CARTESIAN_POINT('Ctrl Pts',(-253.508166926229,-5.11435391846912,
127.284623701469));
#251120=CARTESIAN_POINT('Ctrl Pts',(-253.786614550041,-5.72568757235024,
133.204707652256));
#251121=CARTESIAN_POINT('Ctrl Pts',(-254.065062173855,-1.07539404373626,
136.918989908584));
#251122=CARTESIAN_POINT('Ctrl Pts',(-254.343509797667,4.56313403947717,
135.014226625117));
#251123=CARTESIAN_POINT('Ctrl Pts',(-254.621957421481,6.00836492926231,
129.240802026269));
#251124=CARTESIAN_POINT('Ctrl Pts',(-254.900405045293,1.9322018468105,124.904211611225));
#251125=CARTESIAN_POINT('Ctrl Pts',(-255.178852669106,-3.91956009939235,
125.989569474605));
#251126=CARTESIAN_POINT('Ctrl Pts',(-255.457300292919,-6.16943824888009,
131.499485975975));
#251127=CARTESIAN_POINT('Ctrl Pts',(-255.735747916732,-2.74990318521692,
136.370614733943));
#251128=CARTESIAN_POINT('Ctrl Pts',(-256.014195540545,3.19665694865877,
136.126630713714));
#251129=CARTESIAN_POINT('Ctrl Pts',(-256.292643164358,6.20564856486739,
130.991735142402));
#251130=CARTESIAN_POINT('Ctrl Pts',(-256.571090788171,3.51194654848645,
125.68466161966));
#251131=CARTESIAN_POINT('Ctrl Pts',(-256.849538411983,-2.40905189372645,
125.082322325773));
#251132=CARTESIAN_POINT('Ctrl Pts',(-257.127986035797,-6.11626988572704,
129.738292634474));
#251133=CARTESIAN_POINT('Ctrl Pts',(-257.406433659609,-4.20289584392431,
135.373859459261));
#251134=CARTESIAN_POINT('Ctrl Pts',(-257.684881283423,1.57266088340656,
136.810408252432));
#251135=CARTESIAN_POINT('Ctrl Pts',(-257.963328907235,5.90315744058412,
132.727450666138));
#251136=CARTESIAN_POINT('Ctrl Pts',(-258.241776531048,4.80867945501638,
126.87772425425));
#251137=CARTESIAN_POINT('Ctrl Pts',(-258.520224154861,-0.704246744852541,
124.635521896935));
#251138=CARTESIAN_POINT('Ctrl Pts',(-258.798671778674,-5.5709361272427,
128.063810879205));
#251139=CARTESIAN_POINT('Ctrl Pts',(-259.077119402487,-5.31644754243966,
134.007449313497));
#251140=CARTESIAN_POINT('Ctrl Pts',(-259.355567026299,-0.179733571114533,
137.013459703814));
#251141=CARTESIAN_POINT('Ctrl Pts',(-259.634014650113,5.12849404027147,
134.30227331953));
#251142=CARTESIAN_POINT('Ctrl Pts',(-259.866054336623,5.61428989304695,
129.384066440553));
#251143=CARTESIAN_POINT('Ctrl Pts',(-260.051696012132,3.39054283699284,
126.521203045511));
#251144=CARTESIAN_POINT('Ctrl Pts',(-260.144521813036,1.754921961264,125.780753115897));
#251145=CARTESIAN_POINT('Ctrl Pts',(-260.190939676638,0.892893391295023,
125.631947563271));
#251146=CARTESIAN_POINT('Ctrl Pts',(210.191733024964,-2.43880115184907,
125.780342085335));
#251147=CARTESIAN_POINT('Ctrl Pts',(210.145323348611,-3.27594855749458,
126.186716565447));
#251148=CARTESIAN_POINT('Ctrl Pts',(210.052505734956,-4.72940422381435,
127.426013481475));
#251149=CARTESIAN_POINT('Ctrl Pts',(209.866872246696,-6.15821517169733,
131.008352419918));
#251150=CARTESIAN_POINT('Ctrl Pts',(209.634832560185,-4.21099667891447,
135.892791108304));
#251151=CARTESIAN_POINT('Ctrl Pts',(209.356384936373,2.01508446636645,137.098708070195));
#251152=CARTESIAN_POINT('Ctrl Pts',(209.07793731256,6.37956871319657,132.510708806665));
#251153=CARTESIAN_POINT('Ctrl Pts',(208.799489688747,4.8866719183268,126.359661034021));
#251154=CARTESIAN_POINT('Ctrl Pts',(208.521042064934,-1.09954563679898,
124.290443595948));
#251155=CARTESIAN_POINT('Ctrl Pts',(208.242594441121,-6.07390144970816,
128.208589139036));
#251156=CARTESIAN_POINT('Ctrl Pts',(207.964146817309,-5.46739734855352,
134.511385201899));
#251157=CARTESIAN_POINT('Ctrl Pts',(207.685699193495,0.163779660617915,
137.407996874876));
#251158=CARTESIAN_POINT('Ctrl Pts',(207.407251569682,5.6442383477931,134.235982835808));
#251159=CARTESIAN_POINT('Ctrl Pts',(207.128803945869,5.93803043711477,127.910585036422));
#251160=CARTESIAN_POINT('Ctrl Pts',(206.850356322057,0.775002953389061,
124.244367681185));
#251161=CARTESIAN_POINT('Ctrl Pts',(206.571908698243,-5.10018277131114,
126.606494049502));
#251162=CARTESIAN_POINT('Ctrl Pts',(206.293461074431,-6.28856642889766,
132.82623846394));
#251163=CARTESIAN_POINT('Ctrl Pts',(206.015013450618,-1.69805588527783,
137.187984519302));
#251164=CARTESIAN_POINT('Ctrl Pts',(205.736565826805,4.45288036648484,135.683487507757));
#251165=CARTESIAN_POINT('Ctrl Pts',(205.458118202992,6.51183958365415,129.695313656966));
#251166=CARTESIAN_POINT('Ctrl Pts',(205.179670579179,2.58673502741873,124.726298504418));
#251167=CARTESIAN_POINT('Ctrl Pts',(204.901222955366,-3.71545195245463,
125.342726181157));
#251168=CARTESIAN_POINT('Ctrl Pts',(204.622775331554,-6.60332046735468,
130.978128730661));
#251169=CARTESIAN_POINT('Ctrl Pts',(204.344327707741,-3.42305986725146,
136.4538470632));
#251170=CARTESIAN_POINT('Ctrl Pts',(204.065880083927,2.90282542147133,136.737963244372));
#251171=CARTESIAN_POINT('Ctrl Pts',(203.787432460115,6.56115601364161,131.569388537382));
#251172=CARTESIAN_POINT('Ctrl Pts',(203.508984836302,4.1901047305044,125.69779051756));
#251173=CARTESIAN_POINT('Ctrl Pts',(203.230537212489,-2.03144808657932,
124.518880964767));
#251174=CARTESIAN_POINT('Ctrl Pts',(202.952089588676,-6.38619936200403,
129.116020142231));
#251175=CARTESIAN_POINT('Ctrl Pts',(202.673641964863,-4.87234540261322,
135.2646617407));
#251176=CARTESIAN_POINT('Ctrl Pts',(202.39519434105,1.1189559521872,137.314504502614));
#251177=CARTESIAN_POINT('Ctrl Pts',(202.116746717238,6.08199145217563,133.381843073553));
#251178=CARTESIAN_POINT('Ctrl Pts',(201.838299093424,5.45597392877388,127.080601183836));
#251179=CARTESIAN_POINT('Ctrl Pts',(201.559851469612,-0.183817095687214,
124.201312298284));
#251180=CARTESIAN_POINT('Ctrl Pts',(201.281403845799,-5.65468918935595,
127.389902241135));
#251181=CARTESIAN_POINT('Ctrl Pts',(201.002956221986,-5.92917816483575,
133.716212626452));
#251182=CARTESIAN_POINT('Ctrl Pts',(200.724508598173,-0.755042063338292,
137.366673267433));
#251183=CARTESIAN_POINT('Ctrl Pts',(200.44606097436,5.11294080853837,134.986689170007));
#251184=CARTESIAN_POINT('Ctrl Pts',(200.167613350547,6.2823808583988,128.763349450982));
#251185=CARTESIAN_POINT('Ctrl Pts',(199.889165726734,1.67861981076543,124.415599285115));
#251186=CARTESIAN_POINT('Ctrl Pts',(199.610718102921,-4.46771083782862,
125.938808675424));
#251187=CARTESIAN_POINT('Ctrl Pts',(199.332270479108,-6.50843348626435,
131.933222605136));
#251188=CARTESIAN_POINT('Ctrl Pts',(199.053822855296,-2.56822371547623,
136.890267516244));
#251189=CARTESIAN_POINT('Ctrl Pts',(198.775375231483,3.73205818513161,136.254661300547));
#251190=CARTESIAN_POINT('Ctrl Pts',(198.49692760767,6.60276093478139,130.610495019181));
#251191=CARTESIAN_POINT('Ctrl Pts',(198.218479983857,3.4058489481713,125.14448175187));
#251192=CARTESIAN_POINT('Ctrl Pts',(197.940032360044,-2.92087183683725,
124.879620661678));
#251193=CARTESIAN_POINT('Ctrl Pts',(197.661584736231,-6.56345409631434,
130.05930615131));
#251194=CARTESIAN_POINT('Ctrl Pts',(197.383137112418,-4.1745426838368,135.923660297497));
#251195=CARTESIAN_POINT('Ctrl Pts',(197.104689488605,2.05056951733907,137.083628129519));
#251196=CARTESIAN_POINT('Ctrl Pts',(196.826241864792,6.39130850797037,132.473255877329));
#251197=CARTESIAN_POINT('Ctrl Pts',(196.54779424098,4.85874721255563,126.329250411482));
#251198=CARTESIAN_POINT('Ctrl Pts',(196.269346617166,-1.13876540820057,
124.297652603739));
#251199=CARTESIAN_POINT('Ctrl Pts',(195.990898993354,-6.0898082506034,128.245401590344));
#251200=CARTESIAN_POINT('Ctrl Pts',(195.712451369541,-5.44461481437399,
134.544708910868));
#251201=CARTESIAN_POINT('Ctrl Pts',(195.434003745728,0.203913652044436,
137.406818876019));
#251202=CARTESIAN_POINT('Ctrl Pts',(195.155556121915,5.66505543396973,134.201592249669));
#251203=CARTESIAN_POINT('Ctrl Pts',(194.877108498102,5.92028802542049,127.874475717408));
#251204=CARTESIAN_POINT('Ctrl Pts',(194.59866087429,0.735065143658737,124.239780275557));
#251205=CARTESIAN_POINT('Ctrl Pts',(194.320213250476,-5.1256466951968,126.637613470433));
#251206=CARTESIAN_POINT('Ctrl Pts',(194.041765626664,-6.2761396229282,132.86448373661));
#251207=CARTESIAN_POINT('Ctrl Pts',(193.763318002851,-1.6591668436545,137.198201498994));
#251208=CARTESIAN_POINT('Ctrl Pts',(193.484870379038,4.48249921013125,135.656291847837));
#251209=CARTESIAN_POINT('Ctrl Pts',(193.206422755225,6.50496747206681,129.655694426079));
#251210=CARTESIAN_POINT('Ctrl Pts',(192.927975131412,2.54968841250072,124.710665118833));
#251211=CARTESIAN_POINT('Ctrl Pts',(192.649527507599,-3.74862973894988,
125.365444281348));
#251212=CARTESIAN_POINT('Ctrl Pts',(192.371079883787,-6.60214029104917,
131.018321851013));
#251213=CARTESIAN_POINT('Ctrl Pts',(192.092632259973,-3.38860644815819,
136.474579499726));
#251214=CARTESIAN_POINT('Ctrl Pts',(191.814184636161,2.93889117796205,136.720183001327));
#251215=CARTESIAN_POINT('Ctrl Pts',(191.535737012347,6.56569138435095,131.529434736241));
#251216=CARTESIAN_POINT('Ctrl Pts',(191.257289388535,4.15894196037717,125.672378777932));
#251217=CARTESIAN_POINT('Ctrl Pts',(190.978841764722,-2.06967194957323,
124.531363418996));
#251218=CARTESIAN_POINT('Ctrl Pts',(190.700394140909,-6.3963584469616,129.154926032595));
#251219=CARTESIAN_POINT('Ctrl Pts',(190.421946517096,-4.84510401107414,
135.294238450423));
#251220=CARTESIAN_POINT('Ctrl Pts',(190.143498893283,1.15856431450073,137.307572482581));
#251221=CARTESIAN_POINT('Ctrl Pts',(189.86505126947,6.09756863406271,133.344772510351));
#251222=CARTESIAN_POINT('Ctrl Pts',(189.586603645657,5.4332052617092,127.047458114672));
#251223=CARTESIAN_POINT('Ctrl Pts',(189.308156021844,-0.224008319322015,
124.202553584261));
#251224=CARTESIAN_POINT('Ctrl Pts',(189.029708398032,-5.67536919831109,
127.424387201254));
#251225=CARTESIAN_POINT('Ctrl Pts',(188.751260774218,-5.91134304125131,
133.752251266956));
#251226=CARTESIAN_POINT('Ctrl Pts',(188.472813150406,-0.71508141444371,
137.371147838333));
#251227=CARTESIAN_POINT('Ctrl Pts',(188.194365526593,5.13830509856852,134.955487759214));
#251228=CARTESIAN_POINT('Ctrl Pts',(187.91591790278,6.26984024615536,128.725144630756));
#251229=CARTESIAN_POINT('Ctrl Pts',(187.637470278967,1.63969850624965,124.405499418827));
#251230=CARTESIAN_POINT('Ctrl Pts',(187.359022655154,-4.49724605717418,
125.966095046791));
#251231=CARTESIAN_POINT('Ctrl Pts',(187.080575031341,-6.5014411967389,131.972820371883));
#251232=CARTESIAN_POINT('Ctrl Pts',(186.802127407528,-2.53112948956026,
136.905788265189));
#251233=CARTESIAN_POINT('Ctrl Pts',(186.523679783716,3.76516656597443,136.231842221641));
#251234=CARTESIAN_POINT('Ctrl Pts',(186.245232159903,6.60145848599114,130.570305731164));
#251235=CARTESIAN_POINT('Ctrl Pts',(185.96678453609,3.3713325565579,125.123854247073));
#251236=CARTESIAN_POINT('Ctrl Pts',(185.688336912277,-2.95688329360047,
124.897510609301));
#251237=CARTESIAN_POINT('Ctrl Pts',(185.409889288464,-6.5678678487195,130.099273563458));
#251238=CARTESIAN_POINT('Ctrl Pts',(185.131441664651,-4.14330270904733,
135.948977074923));
#251239=CARTESIAN_POINT('Ctrl Pts',(184.852994040838,2.08875520864929,137.071029390563));
#251240=CARTESIAN_POINT('Ctrl Pts',(184.574546417025,6.40134913096194,132.434319247607));
#251241=CARTESIAN_POINT('Ctrl Pts',(184.296098793212,4.831415925211,126.299756751549));
#251242=CARTESIAN_POINT('Ctrl Pts',(184.017651169399,-1.17835248801931,
124.304705146227));
#251243=CARTESIAN_POINT('Ctrl Pts',(183.739203545587,-6.10527253047917,
128.282519393244));
#251244=CARTESIAN_POINT('Ctrl Pts',(183.460755921774,-5.42174537657308,
134.577782526619));
#251245=CARTESIAN_POINT('Ctrl Pts',(183.182308297961,0.244100911417136,
137.405455267482));
#251246=CARTESIAN_POINT('Ctrl Pts',(182.903860674148,5.68563038680749,134.167044506474));
#251247=CARTESIAN_POINT('Ctrl Pts',(182.625413050335,5.90234329520773,127.838491527799));
#251248=CARTESIAN_POINT('Ctrl Pts',(182.346965426522,0.695091060812155,
124.23542735186));
#251249=CARTESIAN_POINT('Ctrl Pts',(182.068517802709,-5.15091590138369,
126.668891936874));
#251250=CARTESIAN_POINT('Ctrl Pts',(181.790070178896,-6.263482786439,132.902650210566));
#251251=CARTESIAN_POINT('Ctrl Pts',(181.511622555083,-1.62021497890189,
137.208182855437));
#251252=CARTESIAN_POINT('Ctrl Pts',(181.233174931271,4.51195124234396,135.628915707812));
#251253=CARTESIAN_POINT('Ctrl Pts',(180.954727307458,6.49785469294791,129.61611812487));
#251254=CARTESIAN_POINT('Ctrl Pts',(180.676279683645,2.51254711858197,124.695257343842));
#251255=CARTESIAN_POINT('Ctrl Pts',(180.397832059832,-3.78166851301026,
125.388364025079));
#251256=CARTESIAN_POINT('Ctrl Pts',(180.119384436019,-6.60071552592353,
131.058506988669));
#251257=CARTESIAN_POINT('Ctrl Pts',(179.840936812206,-3.35402743339335,
136.495101852955));
#251258=CARTESIAN_POINT('Ctrl Pts',(179.562489188393,2.97484801707599,136.702183530083));
#251259=CARTESIAN_POINT('Ctrl Pts',(179.28404156458,6.56998346925752,131.489454075275));
#251260=CARTESIAN_POINT('Ctrl Pts',(179.005593940767,4.12762507472721,125.647157201507));
#251261=CARTESIAN_POINT('Ctrl Pts',(178.727146316955,-2.10781911778238,
124.544078323705));
#251262=CARTESIAN_POINT('Ctrl Pts',(178.448698693142,-6.40628051373842,
129.193893042167));
#251263=CARTESIAN_POINT('Ctrl Pts',(178.170251069329,-4.81768308177075,
135.323648786705));
#251264=CARTESIAN_POINT('Ctrl Pts',(177.891803445516,1.19812974544141,137.300399483306));
#251265=CARTESIAN_POINT('Ctrl Pts',(177.613355821703,6.11291986848493,133.307607811431));
#251266=CARTESIAN_POINT('Ctrl Pts',(177.33490819789,5.41023526512845,127.014454258818));
#251267=CARTESIAN_POINT('Ctrl Pts',(177.056460574078,-0.264191242194762,
124.204039502676));
#251268=CARTESIAN_POINT('Ctrl Pts',(176.778012950264,-5.69583890440069,
127.458997407505));
#251269=CARTESIAN_POINT('Ctrl Pts',(176.499565326452,-5.89328887066216,
133.788180672302));
#251270=CARTESIAN_POINT('Ctrl Pts',(176.221117702638,-0.675094267951971,
137.375379074508));
#251271=CARTESIAN_POINT('Ctrl Pts',(175.942670078826,5.16347898681764,134.924132526884));
#251272=CARTESIAN_POINT('Ctrl Pts',(175.664222455013,6.25706730267374,128.687016856641));
#251273=CARTESIAN_POINT('Ctrl Pts',(175.3857748312,1.60071644210391,124.395636664696));
#251274=CARTESIAN_POINT('Ctrl Pts',(175.107327207387,-4.5266146294138,125.993560701866));
#251275=CARTESIAN_POINT('Ctrl Pts',(174.828879583574,-6.49420799391872,
132.012374840923));
#251276=CARTESIAN_POINT('Ctrl Pts',(174.550431959762,-2.49394147171037,
136.92108292349));
#251277=CARTESIAN_POINT('Ctrl Pts',(174.271984335948,3.79813542718566,136.208822025409));
#251278=CARTESIAN_POINT('Ctrl Pts',(173.993536712136,6.59991141772898,130.530125116137));
#251279=CARTESIAN_POINT('Ctrl Pts',(173.715089088322,3.33669123897678,125.103437235529));
#251280=CARTESIAN_POINT('Ctrl Pts',(173.43664146451,-2.99278518196597,124.915619437422));
#251281=CARTESIAN_POINT('Ctrl Pts',(173.158193840697,-6.5720382263662,130.139267102866));
#251282=CARTESIAN_POINT('Ctrl Pts',(172.879746216884,-4.11190920265221,
135.974103216695));
#251283=CARTESIAN_POINT('Ctrl Pts',(172.601298593071,2.12686350036709,137.058198437889));
#251284=CARTESIAN_POINT('Ctrl Pts',(172.322850969258,6.41115254960738,132.395322219168));
#251285=CARTESIAN_POINT('Ctrl Pts',(172.044403345445,4.80390560797255,126.270430011369));
#251286=CARTESIAN_POINT('Ctrl Pts',(171.765955721632,-1.21789590355323,
124.31199853584));
#251287=CARTESIAN_POINT('Ctrl Pts',(171.487508097819,-6.12051057723618,
128.319730643897));
#251288=CARTESIAN_POINT('Ctrl Pts',(171.209060474007,-5.39867503400336,
134.610716316833));
#251289=CARTESIAN_POINT('Ctrl Pts',(170.930612850193,0.284279125540913,
137.403847052956));
#251290=CARTESIAN_POINT('Ctrl Pts',(170.652165226381,5.70599465652041,134.13237215779));
#251291=CARTESIAN_POINT('Ctrl Pts',(170.373717602568,5.88417985149351,127.802617239562));
#251292=CARTESIAN_POINT('Ctrl Pts',(170.095269978755,0.655091221110643,
124.231317842401));
#251293=CARTESIAN_POINT('Ctrl Pts',(169.816822354942,-5.17599423848763,
126.700323644626));
#251294=CARTESIAN_POINT('Ctrl Pts',(169.538374731129,-6.25059385429175,
132.940738931629));
#251295=CARTESIAN_POINT('Ctrl Pts',(169.259927107316,-1.58120307648749,
137.217926915891));
#251296=CARTESIAN_POINT('Ctrl Pts',(168.981479483503,4.54123608254409,135.601360792124));
#251297=CARTESIAN_POINT('Ctrl Pts',(168.703031859691,6.49050113343381,129.576585854424));
#251298=CARTESIAN_POINT('Ctrl Pts',(168.424584235878,2.47531272130571,124.680075943919));
#251299=CARTESIAN_POINT('Ctrl Pts',(168.146136612065,-3.81456715595326,
125.411484460556));
#251300=CARTESIAN_POINT('Ctrl Pts',(167.867688988252,-6.59904616885666,
131.098682708838));
#251301=CARTESIAN_POINT('Ctrl Pts',(167.589241364439,-3.31932413390846,
136.515413333674));
#251302=CARTESIAN_POINT('Ctrl Pts',(167.310793740626,3.01069462210276,136.683965512842));
#251303=CARTESIAN_POINT('Ctrl Pts',(167.032346116813,6.57403210101054,131.449448027918));
#251304=CARTESIAN_POINT('Ctrl Pts',(166.753898493,4.09615523841214,125.622126727152));
#251305=CARTESIAN_POINT('Ctrl Pts',(166.475450869187,-2.14588817997888,
124.557025205477));
#251306=CARTESIAN_POINT('Ctrl Pts',(166.197003245374,-6.41596519343492,
129.232919728208));
#251307=CARTESIAN_POINT('Ctrl Pts',(165.918555621562,-4.79008363144905,
135.352891659104));
#251308=CARTESIAN_POINT('Ctrl Pts',(165.640107997748,1.23765077924384,137.292985770921));
#251309=CARTESIAN_POINT('Ctrl Pts',(165.361660373936,6.12804458641347,133.270350353765));
#251310=CARTESIAN_POINT('Ctrl Pts',(165.083212750123,5.38706479029029,126.981590839339));
#251311=CARTESIAN_POINT('Ctrl Pts',(164.80476512631,-0.304364375363971,
124.205769998417));
#251312=CARTESIAN_POINT('Ctrl Pts',(164.526317502497,-5.71609754908509,
127.493731577419));
#251313=CARTESIAN_POINT('Ctrl Pts',(164.247869878684,-5.8750163220866,133.823999511097));
#251314=CARTESIAN_POINT('Ctrl Pts',(163.969422254871,-0.635082105593798,
137.37936681918));
#251315=CARTESIAN_POINT('Ctrl Pts',(163.690974631059,5.18846154045405,134.892624634889));
#251316=CARTESIAN_POINT('Ctrl Pts',(163.412527007245,6.24406250126218,128.648967541478));
#251317=CARTESIAN_POINT('Ctrl Pts',(163.134079383433,1.56167506282176,124.386011388187));
#251318=CARTESIAN_POINT('Ctrl Pts',(162.85563175962,-4.55581546628373,126.021204622902));
#251319=CARTESIAN_POINT('Ctrl Pts',(162.577184135807,-6.48673414583306,
132.051884546553));
#251320=CARTESIAN_POINT('Ctrl Pts',(162.298736511994,-2.45666103994207,
136.936150924396));
#251321=CARTESIAN_POINT('Ctrl Pts',(162.020288888181,3.83096354709181,136.185601564872));
#251322=CARTESIAN_POINT('Ctrl Pts',(161.741841264368,6.59811978732212,130.489954663008));
#251323=CARTESIAN_POINT('Ctrl Pts',(161.463393640556,3.30192627907479,125.083231473798));
#251324=CARTESIAN_POINT('Ctrl Pts',(161.184946016742,-3.02857617157586,
124.933946475014));
#251325=CARTESIAN_POINT('Ctrl Pts',(160.90649839293,-6.57596507471956,130.179285287561));
#251326=CARTESIAN_POINT('Ctrl Pts',(160.628050769116,-4.08036332794952,
135.999037791754));
#251327=CARTESIAN_POINT('Ctrl Pts',(160.349603145304,2.16489298037573,137.045135746957));
#251328=CARTESIAN_POINT('Ctrl Pts',(160.07115552149,6.42071840063739,132.356266237063));
#251329=CARTESIAN_POINT('Ctrl Pts',(159.792707897678,4.77621728024515,126.241271277656));
#251330=CARTESIAN_POINT('Ctrl Pts',(159.514260273865,-1.25739418950663,
124.319532502318));
#251331=CARTESIAN_POINT('Ctrl Pts',(159.235812650052,-6.13552182622286,
128.357033963427));
#251332=CARTESIAN_POINT('Ctrl Pts',(158.957365026239,-5.37540464154493,
134.643509061136));
#251333=CARTESIAN_POINT('Ctrl Pts',(158.678917402427,0.324446805597038,
137.401994292032));
#251334=CARTESIAN_POINT('Ctrl Pts',(158.400469778613,5.72614748850293,134.097576488416));
#251335=CARTESIAN_POINT('Ctrl Pts',(158.122022154801,5.86579836733105,127.766854182028));
#251336=CARTESIAN_POINT('Ctrl Pts',(157.843574530988,0.615067106763091,
124.22745189946));
#251337=CARTESIAN_POINT('Ctrl Pts',(157.565126907175,-5.20088077722156,
126.731907428977));
#251338=CARTESIAN_POINT('Ctrl Pts',(157.286679283362,-6.23747330409059,
132.978748488409));
#251339=CARTESIAN_POINT('Ctrl Pts',(157.008231659549,-1.54213258201158,
137.227433319288));
#251340=CARTESIAN_POINT('Ctrl Pts',(156.729784035736,4.5703526455712,135.57362812183));
#251341=CARTESIAN_POINT('Ctrl Pts',(156.451336411923,6.48290706601333,129.537099079623));
#251342=CARTESIAN_POINT('Ctrl Pts',(156.172888788111,2.43798660040623,124.665121481617));
#251343=CARTESIAN_POINT('Ctrl Pts',(155.894441164297,-3.84732444870741,
125.434804731043));
#251344=CARTESIAN_POINT('Ctrl Pts',(155.615993540485,-6.59713228170722,
131.138847522794));
#251345=CARTESIAN_POINT('Ctrl Pts',(155.337545916672,-3.28449783564716,
136.535513189234));
#251346=CARTESIAN_POINT('Ctrl Pts',(155.059098292859,3.04642966473303,136.665529624679));
#251347=CARTESIAN_POINT('Ctrl Pts',(154.780650669046,6.57783712958646,131.409418076611));
#251348=CARTESIAN_POINT('Ctrl Pts',(154.502203045233,4.06453361755842,125.597288282381));
#251349=CARTESIAN_POINT('Ctrl Pts',(154.22375542142,-2.18387772549973,124.57020358456));
#251350=CARTESIAN_POINT('Ctrl Pts',(153.945307797607,-6.42541212718171,
129.272004644569));
#251351=CARTESIAN_POINT('Ctrl Pts',(153.666860173794,-4.76230668281685,
135.381965984011));
#251352=CARTESIAN_POINT('Ctrl Pts',(153.388412549982,1.27712595144142,137.285331620145));
#251353=CARTESIAN_POINT('Ctrl Pts',(153.109964926169,6.14294222739622,133.233001517943));
#251354=CARTESIAN_POINT('Ctrl Pts',(152.831517302356,5.36369469578529,126.948869073999));
#251355=CARTESIAN_POINT('Ctrl Pts',(152.553069678543,-0.344526230199219,
124.207745007359));
#251356=CARTESIAN_POINT('Ctrl Pts',(152.27462205473,-5.73614438167267,127.528588423912));
#251357=CARTESIAN_POINT('Ctrl Pts',(151.996174430917,-5.85652607262075,
133.859706456064));
#251358=CARTESIAN_POINT('Ctrl Pts',(151.717726807104,-0.595046410034728,
137.383110924578));
#251359=CARTESIAN_POINT('Ctrl Pts',(151.439279183291,5.21325183374003,134.860965250768));
#251360=CARTESIAN_POINT('Ctrl Pts',(151.160831559478,6.23082632381839,128.610998095198));
#251361=CARTESIAN_POINT('Ctrl Pts',(150.882383935665,1.52257581509584,124.376623945969));
#251362=CARTESIAN_POINT('Ctrl Pts',(150.603936311853,-4.58484748573611,
126.049025785542));
#251363=CARTESIAN_POINT('Ctrl Pts',(150.32548868804,-6.47901992942814,132.091348024725));
#251364=CARTESIAN_POINT('Ctrl Pts',(150.047041064227,-2.41928957569559,
136.950991709558));
#251365=CARTESIAN_POINT('Ctrl Pts',(149.768593440414,3.8636497092349,136.162181700472));
#251366=CARTESIAN_POINT('Ctrl Pts',(149.490145816601,6.59608366116008,130.449795860306));
#251367=CARTESIAN_POINT('Ctrl Pts',(149.211698192788,3.26703896508027,125.06323771061));
#251368=CARTESIAN_POINT('Ctrl Pts',(148.933250568975,-3.06425493618196,
124.95249104296));
#251369=CARTESIAN_POINT('Ctrl Pts',(148.654802945162,-6.57964824826877,
130.219326634649));
#251370=CARTESIAN_POINT('Ctrl Pts',(148.376355321349,-4.04866625388314,
136.02377987614));
#251371=CARTESIAN_POINT('Ctrl Pts',(148.097907697537,2.20284223947883,137.031841801807));
#251372=CARTESIAN_POINT('Ctrl Pts',(147.819460073724,6.43004632958585,132.317152748525));
#251373=CARTESIAN_POINT('Ctrl Pts',(147.541012449911,4.74835196802999,126.212281630895));
#251374=CARTESIAN_POINT('Ctrl Pts',(147.262564826098,-1.29684588225586,
124.327306766486));
#251375=CARTESIAN_POINT('Ctrl Pts',(146.984117202285,-6.15030572119196,
128.394427969547));
#251376=CARTESIAN_POINT('Ctrl Pts',(146.705669578472,-5.35193506149072,
134.676159544383));
#251377=CARTESIAN_POINT('Ctrl Pts',(146.427221954659,0.364602463157475,
137.399897053366));
#251378=CARTESIAN_POINT('Ctrl Pts',(146.148774330846,5.74608813598446,134.062658787717));
#251379=CARTESIAN_POINT('Ctrl Pts',(145.870326707034,5.84719952385297,127.731203680413));
#251380=CARTESIAN_POINT('Ctrl Pts',(145.59187908322,0.575020200877703,124.22382966629));
#251381=CARTESIAN_POINT('Ctrl Pts',(145.313431459408,-5.22557459540567,
126.76364211958));
#251382=CARTESIAN_POINT('Ctrl Pts',(145.034983835595,-6.22412162202233,
133.016677472446));
#251383=CARTESIAN_POINT('Ctrl Pts',(144.756536211782,-1.50300494324566,
137.236701713364));
#251384=CARTESIAN_POINT('Ctrl Pts',(144.478088587969,4.59929985250025,135.545718724575));
#251385=CARTESIAN_POINT('Ctrl Pts',(144.199640964156,6.47507277208744,129.497659263665));
#251386=CARTESIAN_POINT('Ctrl Pts',(143.921193340343,2.40057013901678,124.65039451108));
#251387=CARTESIAN_POINT('Ctrl Pts',(143.64274571653,-3.87993917743928,125.458323972397));
#251388=CARTESIAN_POINT('Ctrl Pts',(143.364298092718,-6.594973935395,131.178999942215));
#251389=CARTESIAN_POINT('Ctrl Pts',(143.085850468904,-3.2495498291107,136.555400674828));
#251390=CARTESIAN_POINT('Ctrl Pts',(142.807402845092,3.08205182079176,136.646876548744));
#251391=CARTESIAN_POINT('Ctrl Pts',(142.528955221279,6.58139841398854,131.369365704677));
#251392=CARTESIAN_POINT('Ctrl Pts',(142.250507597466,4.03276138391676,125.572642787588));
#251393=CARTESIAN_POINT('Ctrl Pts',(141.972059973653,-2.2217863466284,124.583612972623));
#251394=CARTESIAN_POINT('Ctrl Pts',(141.69361234984,-6.43462096491922,129.311146342943));
#251395=CARTESIAN_POINT('Ctrl Pts',(141.415164726027,-4.7343532651591,135.410870684068));
#251396=CARTESIAN_POINT('Ctrl Pts',(141.136717102214,1.31655379926713,137.277437314604));
#251397=CARTESIAN_POINT('Ctrl Pts',(140.858269478402,6.15761223939561,133.195562687939));
#251398=CARTESIAN_POINT('Ctrl Pts',(140.579821854588,5.34012584760095,126.916290175316));
#251399=CARTESIAN_POINT('Ctrl Pts',(140.301374230776,-0.384675318488256,
124.20996445632));
#251400=CARTESIAN_POINT('Ctrl Pts',(140.022926606963,-5.75597865932068,
127.563566655346));
#251401=CARTESIAN_POINT('Ctrl Pts',(139.74447898315,-5.83781880742758,133.895300184066));
#251402=CARTESIAN_POINT('Ctrl Pts',(139.466031359337,-0.554988664812238,
137.386611251964));
#251403=CARTESIAN_POINT('Ctrl Pts',(139.187583735524,5.23784894806212,134.829155547671));
#251404=CARTESIAN_POINT('Ctrl Pts',(138.909136111711,6.21735926081381,128.573109924773));
#251405=CARTESIAN_POINT('Ctrl Pts',(138.630688487898,1.48342014776303,124.367474685896));
#251406=CARTESIAN_POINT('Ctrl Pts',(138.352240864086,-4.61370961197883,
126.077023158863));
#251407=CARTESIAN_POINT('Ctrl Pts',(138.073793240272,-6.47106563055709,
132.130763813104));
#251408=CARTESIAN_POINT('Ctrl Pts',(137.79534561646,-2.38182846378423,136.965604729043));
#251409=CARTESIAN_POINT('Ctrl Pts',(137.516897992647,3.89619270241722,136.138563300043));
#251410=CARTESIAN_POINT('Ctrl Pts',(137.238450368834,6.59380311469226,130.409650196134));
#251411=CARTESIAN_POINT('Ctrl Pts',(136.960002745021,3.23203058975544,125.043456686844));
#251412=CARTESIAN_POINT('Ctrl Pts',(136.681555121208,-3.09982015369448,
124.971252454085));
#251413=CARTESIAN_POINT('Ctrl Pts',(136.403107497395,-6.58308761053252,
130.259389660389));
#251414=CARTESIAN_POINT('Ctrl Pts',(136.124659873582,-4.01681915499975,
136.048328553027));
#251415=CARTESIAN_POINT('Ctrl Pts',(135.846212249769,2.24070987145278,137.018317095051));
#251416=CARTESIAN_POINT('Ctrl Pts',(135.567764625956,6.43913599080291,132.277983202917));
#251417=CARTESIAN_POINT('Ctrl Pts',(135.289317002144,4.72031070388647,126.183462145311));
#251418=CARTESIAN_POINT('Ctrl Pts',(135.010869378331,-1.33624951990408,
124.335321040266));
#251419=CARTESIAN_POINT('Ctrl Pts',(134.732421754518,-6.16486171432077,
128.431911276607));
#251420=CARTESIAN_POINT('Ctrl Pts',(134.453974130705,-5.32826716351462,
134.708666556695));
#251421=CARTESIAN_POINT('Ctrl Pts',(134.175526506892,0.404744610239488,
137.397555414672));
#251422=CARTESIAN_POINT('Ctrl Pts',(133.897078883079,5.76581586005707,134.027620349581));
#251423=CARTESIAN_POINT('Ctrl Pts',(133.618631259266,5.82838401024617,127.695667055759));
#251424=CARTESIAN_POINT('Ctrl Pts',(133.340183635453,0.534951987407334,
124.220451277114));
#251425=CARTESIAN_POINT('Ctrl Pts',(133.06173601164,-5.25007477800144,126.795526540492));
#251426=CARTESIAN_POINT('Ctrl Pts',(132.783288387828,-6.21053930283845,
133.054524478268));
#251427=CARTESIAN_POINT('Ctrl Pts',(132.504840764015,-1.46382161007886,
137.245731754674));
#251428=CARTESIAN_POINT('Ctrl Pts',(132.226393140202,4.62807663068185,135.517633634551));
#251429=CARTESIAN_POINT('Ctrl Pts',(131.947945516389,6.46699854195874,129.458267868007));
#251430=CARTESIAN_POINT('Ctrl Pts',(131.669497892576,2.3630647236181,124.635895578019));
#251431=CARTESIAN_POINT('Ctrl Pts',(131.391050268763,-3.91241013359816,
125.482041313105));
#251432=CARTESIAN_POINT('Ctrl Pts',(131.11260264495,-6.59257120989826,131.219138479237));
#251433=CARTESIAN_POINT('Ctrl Pts',(130.834155021138,-3.2144814093103,136.575075053519));
#251434=CARTESIAN_POINT('Ctrl Pts',(130.555707397324,3.1175597702868,136.628006976231));
#251435=CARTESIAN_POINT('Ctrl Pts',(130.277259773512,6.58471582225214,131.329292396271));
#251436=CARTESIAN_POINT('Ctrl Pts',(129.998812149698,4.0008397148189,125.548191156024));
#251437=CARTESIAN_POINT('Ctrl Pts',(129.720364525886,-2.25961263864694,
124.59725287278));
#251438=CARTESIAN_POINT('Ctrl Pts',(129.441916902073,-6.44359136541048,
129.350343372922));
#251439=CARTESIAN_POINT('Ctrl Pts',(129.16346927826,-4.70622441430021,135.439604688201));
#251440=CARTESIAN_POINT('Ctrl Pts',(128.885021654447,1.35593286170785,137.269303146827));
#251441=CARTESIAN_POINT('Ctrl Pts',(128.606574030634,6.17205407880915,133.158035251063));
#251442=CARTESIAN_POINT('Ctrl Pts',(128.328126406821,5.31635911908928,126.883855350513));
#251443=CARTESIAN_POINT('Ctrl Pts',(128.049678783009,-0.424810152491945,
124.212428263054));
#251444=CARTESIAN_POINT('Ctrl Pts',(127.771231159195,-5.77559964706288,
127.598664975593));
#251445=CARTESIAN_POINT('Ctrl Pts',(127.492783535383,-5.81889521971155,
133.930779376167));
#251446=CARTESIAN_POINT('Ctrl Pts',(127.21433591157,-0.514910354280421,
137.389867671632));
#251447=CARTESIAN_POINT('Ctrl Pts',(126.935888287757,5.26225197196523,134.797196704317));
#251448=CARTESIAN_POINT('Ctrl Pts',(126.657440663944,6.20366181127538,128.535304434163));
#251449=CARTESIAN_POINT('Ctrl Pts',(126.378993040131,1.44420951175126,124.358563947));
#251450=CARTESIAN_POINT('Ctrl Pts',(126.100545416318,-4.64240077551519,
126.105195705413));
#251451=CARTESIAN_POINT('Ctrl Pts',(125.822097792505,-6.46287154396936,
132.170130451126));
#251452=CARTESIAN_POINT('Ctrl Pts',(125.543650168692,-2.34427909234318,
136.979989441362));
#251453=CARTESIAN_POINT('Ctrl Pts',(125.26520254488,3.92859132074607,136.114747238771));
#251454=CARTESIAN_POINT('Ctrl Pts',(124.986754921067,6.59127823242518,130.369519158099));
#251455=CARTESIAN_POINT('Ctrl Pts',(124.708307297254,3.19690245034852,125.023889135492));
#251456=CARTESIAN_POINT('Ctrl Pts',(124.429859673441,-3.13527050623128,
124.990230013179));
#251457=CARTESIAN_POINT('Ctrl Pts',(124.151412049628,-6.58628303406391,
130.299472880227));
#251458=CARTESIAN_POINT('Ctrl Pts',(123.872964425815,-3.98482321140548,
136.072682912751));
#251459=CARTESIAN_POINT('Ctrl Pts',(123.594516802002,2.2784944730983,137.004562127853));
#251460=CARTESIAN_POINT('Ctrl Pts',(123.316069178189,6.44798704746787,132.238759051683));
#251461=CARTESIAN_POINT('Ctrl Pts',(123.037621554376,4.6920945268939,126.154813888819));
#251462=CARTESIAN_POINT('Ctrl Pts',(122.759173930564,-1.37560364233486,
124.343575026687));
#251463=CARTESIAN_POINT('Ctrl Pts',(122.480726306751,-6.17918926623166,
128.46948249565));
#251464=CARTESIAN_POINT('Ctrl Pts',(122.202278682938,-5.30440182463932,
134.741028893516));
#251465=CARTESIAN_POINT('Ctrl Pts',(121.923831059125,0.444871759361186,
137.394969462721));
#251466=CARTESIAN_POINT('Ctrl Pts',(121.645383435312,5.78532992970255,133.992462472369));
#251467=CARTESIAN_POINT('Ctrl Pts',(121.366935811499,5.80935252372653,127.660245624887));
#251468=CARTESIAN_POINT('Ctrl Pts',(121.088488187686,0.494863951094175,
124.21731685712));
#251469=CARTESIAN_POINT('Ctrl Pts',(120.810040563873,-5.27438041714564,
126.827559510225));
#251470=CARTESIAN_POINT('Ctrl Pts',(120.53159294006,-6.19672684983677,133.092288103441));
#251471=CARTESIAN_POINT('Ctrl Pts',(120.253145316248,-1.42458403446405,
137.254523108609));
#251472=CARTESIAN_POINT('Ctrl Pts',(119.974697692435,4.65668191378195,135.489373892464));
#251473=CARTESIAN_POINT('Ctrl Pts',(119.696250068622,6.45868467482089,129.418926352309));
#251474=CARTESIAN_POINT('Ctrl Pts',(119.417802444809,2.32547174398699,124.621625219699));
#251475=CARTESIAN_POINT('Ctrl Pts',(119.139354820996,-3.94473611396066,
125.505955874312));
#251476=CARTESIAN_POINT('Ctrl Pts',(118.860907197183,-6.58992419425096,
131.259261646514));
#251477=CARTESIAN_POINT('Ctrl Pts',(118.58245957337,-3.17929387571916,136.594535596262));
#251478=CARTESIAN_POINT('Ctrl Pts',(118.304011949557,3.15295219745811,136.608921606362));
#251479=CARTESIAN_POINT('Ctrl Pts',(118.025564325744,6.58778923144938,131.289199636326));
#251480=CARTESIAN_POINT('Ctrl Pts',(117.747116701932,3.96876979313418,125.523934293753));
#251481=CARTESIAN_POINT('Ctrl Pts',(117.468669078118,-2.29735519988813,
124.611122779595));
#251482=CARTESIAN_POINT('Ctrl Pts',(117.190221454306,-6.45232299625411,
129.389594282045));
#251483=CARTESIAN_POINT('Ctrl Pts',(116.911773830493,-4.67792117256487,
135.468166931659));
#251484=CARTESIAN_POINT('Ctrl Pts',(116.63332620668,1.39526167955762,137.260929418227));
#251485=CARTESIAN_POINT('Ctrl Pts',(116.354878582867,6.18626721048894,133.120420597908));
#251486=CARTESIAN_POINT('Ctrl Pts',(116.076430959054,5.29239539093549,126.851565801475));
#251487=CARTESIAN_POINT('Ctrl Pts',(115.797983335241,-0.464929244999223,
124.215136336267));
#251488=CARTESIAN_POINT('Ctrl Pts',(115.519535711428,-5.79500661783607,
127.633882084071));
#251489=CARTESIAN_POINT('Ctrl Pts',(115.241088087616,-5.79975601069334,
133.96614271767));
#251490=CARTESIAN_POINT('Ctrl Pts',(114.962640463802,-0.474812963556037,
137.392880062915));
#251491=CARTESIAN_POINT('Ctrl Pts',(114.68419283999,5.28646000118636,134.765089904953));
#251492=CARTESIAN_POINT('Ctrl Pts',(114.405745216177,6.18973448276714,128.497583024264));
#251493=CARTESIAN_POINT('Ctrl Pts',(114.127297592364,1.40494536002493,124.349892059469));
#251494=CARTESIAN_POINT('Ctrl Pts',(113.848849968551,-4.67091991318358,
126.133542381245));
#251495=CARTESIAN_POINT('Ctrl Pts',(113.570402344738,-6.45443797329988,
132.209446480045));
#251496=CARTESIAN_POINT('Ctrl Pts',(113.291954720925,-2.30664285277824,
136.994145313484));
#251497=CARTESIAN_POINT('Ctrl Pts',(113.013507097112,3.96084436367879,136.09073439917));
#251498=CARTESIAN_POINT('Ctrl Pts',(112.735059473299,6.58850910791926,130.329404233275));
#251499=CARTESIAN_POINT('Ctrl Pts',(112.456611849487,3.16165584854565,125.004535781636));
#251500=CARTESIAN_POINT('Ctrl Pts',(112.178164225674,-3.1706046801665,125.00942301702));
#251501=CARTESIAN_POINT('Ctrl Pts',(111.899716601861,-6.58923440045535,
130.339574808866));
#251502=CARTESIAN_POINT('Ctrl Pts',(111.621268978048,-3.9526796087217,136.096842052857));
#251503=CARTESIAN_POINT('Ctrl Pts',(111.342821354235,2.31619464429322,136.990577409908));
#251504=CARTESIAN_POINT('Ctrl Pts',(111.064373730422,6.45659917160154,132.199481748287));
#251505=CARTESIAN_POINT('Ctrl Pts',(110.785926106609,4.66370448261314,126.12633792299));
#251506=CARTESIAN_POINT('Ctrl Pts',(110.507478482796,-1.41490679126679,
124.352068419894));
#251507=CARTESIAN_POINT('Ctrl Pts',(110.229030858983,-6.19328784601188,
128.50714023446));
#251508=CARTESIAN_POINT('Ctrl Pts',(109.950583235171,-5.28033992920373,
134.773245355646));
#251509=CARTESIAN_POINT('Ctrl Pts',(109.672135611358,0.484982423596243,
137.392139293334));
#251510=CARTESIAN_POINT('Ctrl Pts',(109.393687987545,5.80462962181993,133.957186458871));
#251511=CARTESIAN_POINT('Ctrl Pts',(109.115240363732,5.79010576951274,127.624940700352));
#251512=CARTESIAN_POINT('Ctrl Pts',(108.836792739919,0.454757577415474,
124.214426522456));
#251513=CARTESIAN_POINT('Ctrl Pts',(108.558345116106,-5.29849061218381,
126.859739841786));
#251514=CARTESIAN_POINT('Ctrl Pts',(108.279897492293,-6.18268477484283,
133.12996694862));
#251515=CARTESIAN_POINT('Ctrl Pts',(108.00144986848,-1.38529367036394,137.2630754494));
#251516=CARTESIAN_POINT('Ctrl Pts',(107.723002244667,4.68511464182123,135.460940545486));
#251517=CARTESIAN_POINT('Ctrl Pts',(107.444554620855,6.45013147874722,129.379636174388));
#251518=CARTESIAN_POINT('Ctrl Pts',(107.166106997042,2.28779259314522,124.607583964913));
#251519=CARTESIAN_POINT('Ctrl Pts',(106.887659373229,-3.97691592067581,
125.530066769856));
#251520=CARTESIAN_POINT('Ctrl Pts',(106.609211749416,-6.58703298653922,
131.299367957265));
#251521=CARTESIAN_POINT('Ctrl Pts',(106.330764125603,-3.14398853222427,
136.613781581943));
#251522=CARTESIAN_POINT('Ctrl Pts',(106.05231650179,3.18822779082625,136.589621146351));
#251523=CARTESIAN_POINT('Ctrl Pts',(105.773868877977,6.59061852769399,131.249088910493));
#251524=CARTESIAN_POINT('Ctrl Pts',(105.495421254164,3.93655280722527,125.49987309962));
#251525=CARTESIAN_POINT('Ctrl Pts',(105.216973630351,-2.33501263178752,
124.625222179118));
#251526=CARTESIAN_POINT('Ctrl Pts',(104.938526006539,-6.46081553389627,
129.428897615854));
#251527=CARTESIAN_POINT('Ctrl Pts',(104.660078382726,-4.64944458874018,
135.49655635606));
#251528=CARTESIAN_POINT('Ctrl Pts',(104.381630758913,1.43453879547275,137.252316439095));
#251529=CARTESIAN_POINT('Ctrl Pts',(104.1031831351,6.20025110776228,133.082720122298));
#251530=CARTESIAN_POINT('Ctrl Pts',(103.824735511287,5.26823555112421,126.819422724701));
#251531=CARTESIAN_POINT('Ctrl Pts',(103.546287887474,-0.505031109382345,
124.218088575609));
#251532=CARTESIAN_POINT('Ctrl Pts',(103.267840263661,-5.81419885250792,
127.669216675797));
#251533=CARTESIAN_POINT('Ctrl Pts',(102.989392639848,-5.78040188958328,
134.001388898174));
#251534=CARTESIAN_POINT('Ctrl Pts',(102.710945016035,-0.434697978462825,
137.395648314187));
#251535=CARTESIAN_POINT('Ctrl Pts',(102.432497392222,5.31047213868803,134.732836339309));
#251536=CARTESIAN_POINT('Ctrl Pts',(102.15404976841,6.17557779137139,128.459947092858));
#251537=CARTESIAN_POINT('Ctrl Pts',(101.875602144597,1.3656291475316,124.341459344644));
#251538=CARTESIAN_POINT('Ctrl Pts',(101.597154520784,-4.69926596819684,
126.162062135967));
#251539=CARTESIAN_POINT('Ctrl Pts',(101.318706896971,-6.44576523105769,
132.248710442988));
#251540=CARTESIAN_POINT('Ctrl Pts',(101.040259273158,-2.26892113971413,
137.008071820859));
#251541=CARTESIAN_POINT('Ctrl Pts',(100.761811649345,3.99295063606701,136.066525671043));
#251542=CARTESIAN_POINT('Ctrl Pts',(100.483364025532,6.58549584378548,130.289306908136));
#251543=CARTESIAN_POINT('Ctrl Pts',(100.204916401719,3.12629209042249,124.985397342422));
#251544=CARTESIAN_POINT('Ctrl Pts',(99.9264687779064,-3.20582136617937,
125.028830754405));
#251545=CARTESIAN_POINT('Ctrl Pts',(99.6480211540935,-6.5919416003429,130.379693960313));
#251546=CARTESIAN_POINT('Ctrl Pts',(99.3695735302808,-3.92038953804142,
136.120805078117));
#251547=CARTESIAN_POINT('Ctrl Pts',(99.0911259064677,2.35380898804382,136.976363459425));
#251548=CARTESIAN_POINT('Ctrl Pts',(98.812678282655,6.46497204407849,132.160152748165));
#251549=CARTESIAN_POINT('Ctrl Pts',(98.5342306588419,4.63514162304771,126.098035303012));
#251550=CARTESIAN_POINT('Ctrl Pts',(98.2557830350292,-1.45415751030726,
124.36080090516));
#251551=CARTESIAN_POINT('Ctrl Pts',(97.9773354112161,-6.20715693123341,
128.544883097616));
#251552=CARTESIAN_POINT('Ctrl Pts',(97.6988877874034,-5.25608236883021,
134.805314749293));
#251553=CARTESIAN_POINT('Ctrl Pts',(97.4204401635904,0.525075116629235,
137.389065011387));
#251554=CARTESIAN_POINT('Ctrl Pts',(97.1419925397775,5.82371422125203,133.921793616252));
#251555=CARTESIAN_POINT('Ctrl Pts',(96.8635449159648,5.77064446080036,127.589753590393));
#251556=CARTESIAN_POINT('Ctrl Pts',(96.5850972921516,0.414634352527504,
124.211780380221));
#251557=CARTESIAN_POINT('Ctrl Pts',(96.306649668339,-5.32240446970382,126.89206634272));
#251558=CARTESIAN_POINT('Ctrl Pts',(96.0282020445258,-6.16841359819089,
133.1675596176));
#251559=CARTESIAN_POINT('Ctrl Pts',(95.7497544207132,-1.34595197369742,
137.271388460138));
#251560=CARTESIAN_POINT('Ctrl Pts',(95.4713067969001,4.7133737612145,135.432334647225));
#251561=CARTESIAN_POINT('Ctrl Pts',(95.1928591730874,6.44133927067958,129.340398790155));
#251562=CARTESIAN_POINT('Ctrl Pts',(94.9144115492744,2.25002866730758,124.593772333964));
#251563=CARTESIAN_POINT('Ctrl Pts',(94.6359639254615,-4.008948361309,125.554373106298));
#251564=CARTESIAN_POINT('Ctrl Pts',(94.3575163016487,-6.58389769389783,
131.339455925338));
#251565=CARTESIAN_POINT('Ctrl Pts',(94.0790686778357,-3.10856668707799,
136.632812297395));
#251566=CARTESIAN_POINT('Ctrl Pts',(93.8006210540229,3.22338524324122,136.570106311383));
#251567=CARTESIAN_POINT('Ctrl Pts',(93.52217343021,6.59320360614536,131.208961705089));
#251568=CARTESIAN_POINT('Ctrl Pts',(93.2437258063971,3.90418995090443,125.476008465224));
#251569=CARTESIAN_POINT('Ctrl Pts',(92.9652781825842,-2.37258353893516,
124.639550548886));
#251570=CARTESIAN_POINT('Ctrl Pts',(92.6868305587713,-6.46906866364288,
129.468251917951));
#251571=CARTESIAN_POINT('Ctrl Pts',(92.4083829349583,-4.62079571803641,
135.524771909422));
#251572=CARTESIAN_POINT('Ctrl Pts',(92.1299353111456,1.47376275402524,137.24346452859));
#251573=CARTESIAN_POINT('Ctrl Pts',(91.8514876873325,6.21400525245068,133.04493522124));
#251574=CARTESIAN_POINT('Ctrl Pts',(91.5730400635199,5.24388049490719,126.787427311268));
#251575=CARTESIAN_POINT('Ctrl Pts',(91.2945924397067,-0.545114259651984,
124.221284871682));
#251576=CARTESIAN_POINT('Ctrl Pts',(91.016144815894,-5.83317563990314,127.704667441434));
#251577=CARTESIAN_POINT('Ctrl Pts',(90.7376971920811,-5.76083357355547,
134.036516611621));
#251578=CARTESIAN_POINT('Ctrl Pts',(90.4592495682681,-0.394566885476172,
137.398172322869));
#251579=CARTESIAN_POINT('Ctrl Pts',(90.1808019444553,5.33428749469169,134.700437202553));
#251580=CARTESIAN_POINT('Ctrl Pts',(89.9023543206424,6.16119226166949,128.422398034556));
#251581=CARTESIAN_POINT('Ctrl Pts',(89.6239066968295,1.32626233114802,124.333266115003));
#251582=CARTESIAN_POINT('Ctrl Pts',(89.3454590730166,-4.72743789018152,
126.190753912764));
#251583=CARTESIAN_POINT('Ctrl Pts',(89.0670114492037,-6.43685363861442,
132.28792088502));
#251584=CARTESIAN_POINT('Ctrl Pts',(88.7885638253908,-2.23111535094281,
137.021768447433));
#251585=CARTESIAN_POINT('Ctrl Pts',(88.5101162015778,4.02490894820102,136.042121951457));
#251586=CARTESIAN_POINT('Ctrl Pts',(88.2316685777651,6.58223855168135,130.2492286685));
#251587=CARTESIAN_POINT('Ctrl Pts',(87.9532209539521,3.09081248639635,124.966474527032));
#251588=CARTESIAN_POINT('Ctrl Pts',(87.6747733301392,-3.2409192593025,125.048452506173));
#251589=CARTESIAN_POINT('Ctrl Pts',(87.3963257063264,-6.59440453341028,
130.41982884794));
#251590=CARTESIAN_POINT('Ctrl Pts',(87.1178780825135,-3.88795419588509,
136.144571100572));
#251591=CARTESIAN_POINT('Ctrl Pts',(86.8394304587006,2.39133611053674,136.961920803106));
#251592=CARTESIAN_POINT('Ctrl Pts',(86.5609828348878,6.47310535463887,132.120773508667));
#251593=CARTESIAN_POINT('Ctrl Pts',(86.2825352110747,4.60640700660486,126.06990707765));
#251594=CARTESIAN_POINT('Ctrl Pts',(86.004087587262,-1.49335434500641,124.369772158902));
#251595=CARTESIAN_POINT('Ctrl Pts',(85.725639963449,-6.22079600797217,128.582709686544));
#251596=CARTESIAN_POINT('Ctrl Pts',(85.4471923396362,-5.23163004239161,
134.837235886113));
#251597=CARTESIAN_POINT('Ctrl Pts',(85.1687447158232,0.565148352810691,
137.385746730796));
#251598=CARTESIAN_POINT('Ctrl Pts',(84.8902970920103,5.842583020812,133.886285256006));
#251599=CARTESIAN_POINT('Ctrl Pts',(84.6118494681974,5.75096931873532,127.554685598878));
#251600=CARTESIAN_POINT('Ctrl Pts',(84.3334018443846,0.374495763211118,
124.209378528473));
#251601=CARTESIAN_POINT('Ctrl Pts',(84.0549542205716,-5.34612110356891,
126.924537815158));
#251602=CARTESIAN_POINT('Ctrl Pts',(83.7765065967588,-6.15391384870464,
133.205064717373));
#251603=CARTESIAN_POINT('Ctrl Pts',(83.498058972946,-1.30656040228555,137.279461832782));
#251604=CARTESIAN_POINT('Ctrl Pts',(83.2196113491328,4.74145822480973,135.403557257686));
#251605=CARTESIAN_POINT('Ctrl Pts',(82.9411637253203,6.43230837641647,129.301215653567));
#251606=CARTESIAN_POINT('Ctrl Pts',(82.6627161015071,2.21218136583022,124.580190838648));
#251607=CARTESIAN_POINT('Ctrl Pts',(82.3842684776944,-4.04083224888638,
125.578873982957));
#251608=CARTESIAN_POINT('Ctrl Pts',(82.1058208538814,-6.58051843250612,
131.379524065257));
#251609=CARTESIAN_POINT('Ctrl Pts',(81.8273732300686,-3.07302965285007,
136.651627037425));
#251610=CARTESIAN_POINT('Ctrl Pts',(81.5489256062556,3.25842325193051,136.550377824588));
#251611=CARTESIAN_POINT('Ctrl Pts',(81.270477982443,6.59554437101248,131.168819507043));
#251612=CARTESIAN_POINT('Ctrl Pts',(80.9920303586297,3.87168242338918,125.452341274876));
#251613=CARTESIAN_POINT('Ctrl Pts',(80.713582734817,-2.41006652912724,124.654107357959));
#251614=CARTESIAN_POINT('Ctrl Pts',(80.435135111004,-6.47708207967116,129.507655730047));
#251615=CARTESIAN_POINT('Ctrl Pts',(80.1566874871913,-4.59197562204804,
135.552812546207));
#251616=CARTESIAN_POINT('Ctrl Pts',(79.8782398633782,1.51293210175691,137.234374014721));
#251617=CARTESIAN_POINT('Ctrl Pts',(79.5997922395654,6.22752913488936,133.007067294864));
#251618=CARTESIAN_POINT('Ctrl Pts',(79.3213446157525,5.2193311247699,126.755580746775));
#251619=CARTESIAN_POINT('Ctrl Pts',(79.0428969919396,-0.585177210512381,
124.224725106049));
#251620=CARTESIAN_POINT('Ctrl Pts',(78.7644493681267,-5.85193627682986,
127.740233067343));
#251621=CARTESIAN_POINT('Ctrl Pts',(78.4860017443139,-5.74105178772106,
134.071524556339));
#251622=CARTESIAN_POINT('Ctrl Pts',(78.2075541205009,-0.354421171668466,
137.400451995434));
#251623=CARTESIAN_POINT('Ctrl Pts',(77.9291064966881,5.35790518671055,134.667893695246));
#251624=CARTESIAN_POINT('Ctrl Pts',(77.6506588728751,6.14657842672258,128.384937240753));
#251625=CARTESIAN_POINT('Ctrl Pts',(77.3722112490624,1.28684636962602,124.325312674148));
#251626=CARTESIAN_POINT('Ctrl Pts',(77.0937636252493,-4.75543463521666,
126.219616648455));
#251627=CARTESIAN_POINT('Ctrl Pts',(76.8153160014366,-6.42770352619243,
132.327076353179));
#251628=CARTESIAN_POINT('Ctrl Pts',(76.5368683776235,-2.19322688737167,
137.035234685673));
#251629=CARTESIAN_POINT('Ctrl Pts',(76.2584207538107,4.05671811585379,136.017524144697));
#251630=CARTESIAN_POINT('Ctrl Pts',(75.9799731299978,6.57873735230709,130.209170999483));
#251631=CARTESIAN_POINT('Ctrl Pts',(75.7015255061849,3.05521835117689,124.947768036657));
#251632=CARTESIAN_POINT('Ctrl Pts',(75.423077882372,-3.27589705897064,125.068287545233));
#251633=CARTESIAN_POINT('Ctrl Pts',(75.1446302585591,-6.5966231083926,130.459977984534));
#251634=CARTESIAN_POINT('Ctrl Pts',(74.8661826347462,-3.85537478415624,
136.168139239563));
#251635=CARTESIAN_POINT('Ctrl Pts',(74.5877350109334,2.42877462119068,136.94724997613));
#251636=CARTESIAN_POINT('Ctrl Pts',(74.3092873871204,6.48099880189986,132.081345489005));
#251637=CARTESIAN_POINT('Ctrl Pts',(74.0308397633076,4.57750169805637,126.041954289206));
#251638=CARTESIAN_POINT('Ctrl Pts',(73.7523921394947,-1.53249584291112,
124.378981848686));
#251639=CARTESIAN_POINT('Ctrl Pts',(73.4739445156818,-6.23420457082727,
128.620618599563));
#251640=CARTESIAN_POINT('Ctrl Pts',(73.1954968918689,-5.20698385597775,
134.869007583256));
#251641=CARTESIAN_POINT('Ctrl Pts',(72.917049268056,0.605200647212208,137.382184574524));
#251642=CARTESIAN_POINT('Ctrl Pts',(72.6386016442432,5.86123532130951,133.850662693911));
#251643=CARTESIAN_POINT('Ctrl Pts',(72.3601540204302,5.73108107238729,127.519738025268));
#251644=CARTESIAN_POINT('Ctrl Pts',(72.0817063966174,0.334343296816498,
124.207221056211));
#251645=CARTESIAN_POINT('Ctrl Pts',(71.8032587728044,-5.36963963495047,
126.957153055855));
#251646=CARTESIAN_POINT('Ctrl Pts',(71.5248111489915,-6.13918606367764,
133.242480858172));
#251647=CARTESIAN_POINT('Ctrl Pts',(71.2463635251787,-1.26712041579749,
137.287295268168));
#251648=CARTESIAN_POINT('Ctrl Pts',(70.9679159013657,4.76936699192676,135.374609443224));
#251649=CARTESIAN_POINT('Ctrl Pts',(70.689468277553,6.423039130601,129.262088216567));
#251650=CARTESIAN_POINT('Ctrl Pts',(70.4110206537399,2.17425209115883,124.566839982233));
#251651=CARTESIAN_POINT('Ctrl Pts',(70.1325730299272,-4.07256640193864,
125.603568491945));
#251652=CARTESIAN_POINT('Ctrl Pts',(69.8541254061142,-6.57689532758393,
131.419570892283));
#251653=CARTESIAN_POINT('Ctrl Pts',(69.5756777823013,-3.03737874637841,
136.670225104848));
#251654=CARTESIAN_POINT('Ctrl Pts',(69.2972301584884,3.2933405185478,136.530436417012));
#251655=CARTESIAN_POINT('Ctrl Pts',(69.0187825346755,6.5976407355574,131.128663803839));
#251656=CARTESIAN_POINT('Ctrl Pts',(68.7403349108627,3.83903142925813,125.428872405572));
#251657=CARTESIAN_POINT('Ctrl Pts',(68.4618872870498,-2.44746021341752,
124.668892066929));
#251658=CARTESIAN_POINT('Ctrl Pts',(68.1834396632368,-6.48485548504104,
129.547107592018));
#251659=CARTESIAN_POINT('Ctrl Pts',(67.904992039424,-4.56298536871445,135.580677227361));
#251660=CARTESIAN_POINT('Ctrl Pts',(67.6265444156111,1.55204538723279,137.225045234339));
#251661=CARTESIAN_POINT('Ctrl Pts',(67.3480967917982,6.2408222539455,132.969117746385));
#251662=CARTESIAN_POINT('Ctrl Pts',(67.0696491679854,5.19458835039884,126.723884211309));
#251663=CARTESIAN_POINT('Ctrl Pts',(66.7912015441724,-0.625218477415679,
124.228409151229));
#251664=CARTESIAN_POINT('Ctrl Pts',(66.5127539203596,-5.87048006810572,
127.775912235624));
#251665=CARTESIAN_POINT('Ctrl Pts',(66.2343062965465,-5.72105726510147,
134.106411435094));
#251666=CARTESIAN_POINT('Ctrl Pts',(65.9558586727338,-0.314262324654327,
137.402487247406));
#251667=CARTESIAN_POINT('Ctrl Pts',(65.6774110489208,5.3813243395822,134.6352070233));
#251668=CARTESIAN_POINT('Ctrl Pts',(65.398963425108,6.13173682805169,128.347566099575));
#251669=CARTESIAN_POINT('Ctrl Pts',(65.120515801295,1.24738272353907,124.317599316798));
#251670=CARTESIAN_POINT('Ctrl Pts',(64.8420681774823,-4.78325516587229,
126.248649273519));
#251671=CARTESIAN_POINT('Ctrl Pts',(64.5636205536692,-6.41831523285262,
132.366175396547));
#251672=CARTESIAN_POINT('Ctrl Pts',(64.2851729298565,-2.15525715297185,
137.048470036584));
#251673=CARTESIAN_POINT('Ctrl Pts',(64.0067253060435,4.08837696032456,135.992733162246));
#251674=CARTESIAN_POINT('Ctrl Pts',(63.7282776822307,6.57499237540094,130.169135385437));
#251675=CARTESIAN_POINT('Ctrl Pts',(63.4498300584178,3.01951100371835,124.929278564476));
#251676=CARTESIAN_POINT('Ctrl Pts',(63.1713824346048,-3.31075346906837,
125.088335136589));
#251677=CARTESIAN_POINT('Ctrl Pts',(62.892934810792,-6.59859724307971,130.500139882352));
#251678=CARTESIAN_POINT('Ctrl Pts',(62.614487186979,-3.82265251009718,136.191508621766));
#251679=CARTESIAN_POINT('Ctrl Pts',(62.3360395631662,2.46612313270748,136.932351522132));
#251680=CARTESIAN_POINT('Ctrl Pts',(62.0575919393533,6.48865209336687,132.041870150199));
#251681=CARTESIAN_POINT('Ctrl Pts',(61.7791443155403,4.5484267684992,126.014177973478));
#251682=CARTESIAN_POINT('Ctrl Pts',(61.5006966917276,-1.57158055361859,
124.388429633243));
#251683=CARTESIAN_POINT('Ctrl Pts',(61.2222490679146,-6.24738212293903,
128.658608431946));
#251684=CARTESIAN_POINT('Ctrl Pts',(60.9438014441017,-5.18214472286266,
134.900628663412));
#251685=CARTESIAN_POINT('Ctrl Pts',(60.6653538202889,0.645230515680748,
137.378378674564));
#251686=CARTESIAN_POINT('Ctrl Pts',(60.3869061964759,5.87967043157647,133.814927249971));
#251687=CARTESIAN_POINT('Ctrl Pts',(60.108458572663,5.71098045872276,127.484912164554));
#251688=CARTESIAN_POINT('Ctrl Pts',(59.8300109488502,0.294178441208572,
124.205308043382));
#251689=CARTESIAN_POINT('Ctrl Pts',(59.5515633250373,-5.39295919236059,
126.989910856244));
#251690=CARTESIAN_POINT('Ctrl Pts',(59.2731157012244,-6.12423078885343,
133.27980665353));
#251691=CARTESIAN_POINT('Ctrl Pts',(58.9946680774115,-1.2276334756968,137.294888476026));
#251692=CARTESIAN_POINT('Ctrl Pts',(58.7162204535986,4.79709902839574,135.345492276511));
#251693=CARTESIAN_POINT('Ctrl Pts',(58.4377728297857,6.41353187670863,129.223017929039));
#251694=CARTESIAN_POINT('Ctrl Pts',(58.1593252059728,2.13624224877676,124.553720259438));
#251695=CARTESIAN_POINT('Ctrl Pts',(57.8808775821599,-4.10414964454526,
125.628455718198));
#251696=CARTESIAN_POINT('Ctrl Pts',(57.602429958347,-6.57302851338661,131.459594922466));
#251697=CARTESIAN_POINT('Ctrl Pts',(57.3239823345341,-3.00161528872044,
136.688605810505));
#251698=CARTESIAN_POINT('Ctrl Pts',(57.0455347107212,3.32813574922106,136.510282827592));
#251699=CARTESIAN_POINT('Ctrl Pts',(56.7670870869083,6.59949262209846,131.088496083461));
#251700=CARTESIAN_POINT('Ctrl Pts',(56.4886394630955,3.80623817840574,125.405602726962));
#251701=CARTESIAN_POINT('Ctrl Pts',(56.2101918392826,-2.48476320616966,
124.683904127941));
#251702=CARTESIAN_POINT('Ctrl Pts',(55.9317442154696,-6.49238859170611,
129.586606041964));
#251703=CARTESIAN_POINT('Ctrl Pts',(55.6532965916568,-4.53382603227983,
135.608364920346));
#251704=CARTESIAN_POINT('Ctrl Pts',(55.3748489678439,1.59110116109648,137.215478533129));
#251705=CARTESIAN_POINT('Ctrl Pts',(55.096401344031,6.25388411703813,132.931087982032));
#251706=CARTESIAN_POINT('Ctrl Pts',(54.8179537202181,5.1696530886458,126.692338879397));
#251707=CARTESIAN_POINT('Ctrl Pts',(54.5395060964052,-0.665236576618623,
124.23233687071));
#251708=CARTESIAN_POINT('Ctrl Pts',(54.2610584725923,-5.88880632658389,
127.811703624173));
#251709=CARTESIAN_POINT('Ctrl Pts',(53.9826108487795,-5.70085074660091,
134.141175955143));
#251710=CARTESIAN_POINT('Ctrl Pts',(53.7041632249665,-0.274091832533765,
137.40427800337));
#251711=CARTESIAN_POINT('Ctrl Pts',(53.4257156011537,5.40454408550164,134.602378397932));
#251712=CARTESIAN_POINT('Ctrl Pts',(53.1472679773408,6.11666801561766,128.310285995821));
#251713=CARTESIAN_POINT('Ctrl Pts',(52.8688203535278,1.20787285522606,124.310126328773));
#251714=CARTESIAN_POINT('Ctrl Pts',(52.590372729715,-4.81089845124901,126.277850712144));
#251715=CARTESIAN_POINT('Ctrl Pts',(52.3119251059021,-6.40868910648141,
132.405216566294));
#251716=CARTESIAN_POINT('Ctrl Pts',(52.0334774820892,-2.11720755472543,
137.061474009724));
#251717=CARTESIAN_POINT('Ctrl Pts',(51.7550298582764,4.11988430848393,135.967749922743));
#251718=CARTESIAN_POINT('Ctrl Pts',(51.4765822344634,6.57100375973434,130.129123309894));
#251719=CARTESIAN_POINT('Ctrl Pts',(51.1981346106506,2.98369176716867,124.91100679562));
#251720=CARTESIAN_POINT('Ctrl Pts',(50.9196869868376,-3.34548719797895,
125.108594537373));
#251721=CARTESIAN_POINT('Ctrl Pts',(50.6412393630248,-6.60032686431936,
130.540313053181));
#251722=CARTESIAN_POINT('Ctrl Pts',(50.3627917392119,-3.78978858624336,
136.214678381218));
#251723=CARTESIAN_POINT('Ctrl Pts',(50.0843441153989,2.50338026112505,136.917225993175));
#251724=CARTESIAN_POINT('Ctrl Pts',(49.8058964915862,6.49606494544435,132.002348955022));
#251725=CARTESIAN_POINT('Ctrl Pts',(49.5274488677731,4.51918329531533,125.986579159731));
#251726=CARTESIAN_POINT('Ctrl Pts',(49.2490012439603,-1.6106070288309,124.39811516248));
#251727=CARTESIAN_POINT('Ctrl Pts',(48.9705536201474,-6.26032817600901,
128.696677775965));
#251728=CARTESIAN_POINT('Ctrl Pts',(48.6921059963345,-5.15711356346882,
134.932097954848));
#251729=CARTESIAN_POINT('Ctrl Pts',(48.4136583725217,0.685236474895564,
137.374329171949));
#251730=CARTESIAN_POINT('Ctrl Pts',(48.1352107487087,5.89788766849362,133.779080248378));
#251731=CARTESIAN_POINT('Ctrl Pts',(47.8567631248959,5.69066822257687,127.450209307224));
#251732=CARTESIAN_POINT('Ctrl Pts',(47.578315501083,0.254002684709825,124.203639560873));
#251733=CARTESIAN_POINT('Ctrl Pts',(47.29986787727,-5.41607891168467,127.022810002472));
#251734=CARTESIAN_POINT('Ctrl Pts',(47.0214202534572,-6.10904857840509,
133.317040720324));
#251735=CARTESIAN_POINT('Ctrl Pts',(46.7429726296443,-1.18810104518584,
137.302241174989));
#251736=CARTESIAN_POINT('Ctrl Pts',(46.4645250058313,4.82465330659632,135.316206836494));
#251737=CARTESIAN_POINT('Ctrl Pts',(46.1860773820186,6.40378696703385,129.184006238746));
#251738=CARTESIAN_POINT('Ctrl Pts',(45.9076297582056,2.09815324715241,124.54083215642));
#251739=CARTESIAN_POINT('Ctrl Pts',(45.6291821343927,-4.13558080637756,
125.653534739511));
#251740=CARTESIAN_POINT('Ctrl Pts',(45.3507345105798,-6.56891813320061,
131.499594672701));
#251741=CARTESIAN_POINT('Ctrl Pts',(45.072286886767,-2.96574060510383,136.706768473292));
#251742=CARTESIAN_POINT('Ctrl Pts',(44.793839262954,3.36280765460034,136.489917803126));
#251743=CARTESIAN_POINT('Ctrl Pts',(44.5153916391412,6.60109996201359,131.048317834339));
#251744=CARTESIAN_POINT('Ctrl Pts',(44.2369440153282,3.77330388599763,125.38253310131));
#251745=CARTESIAN_POINT('Ctrl Pts',(43.9584963915154,-2.52197412510756,
124.699142984721));
#251746=CARTESIAN_POINT('Ctrl Pts',(43.6800487677024,-6.49968112052436,
129.626149616253));
#251747=CARTESIAN_POINT('Ctrl Pts',(43.4016011438896,-4.50449869325427,
135.635874599185));
#251748=CARTESIAN_POINT('Ctrl Pts',(43.1231535200766,1.6300979761215,137.205674265588));
#251749=CARTESIAN_POINT('Ctrl Pts',(42.8447058962639,6.26671424015497,132.892979411015));
#251750=CARTESIAN_POINT('Ctrl Pts',(42.5662582724509,5.14452626349642,126.660945919963));
#251751=CARTESIAN_POINT('Ctrl Pts',(42.287810648638,-0.705230025235587,
124.236508118946));
#251752=CARTESIAN_POINT('Ctrl Pts',(42.0093630248251,-5.90691437317801,
127.847605906729));
#251753=CARTESIAN_POINT('Ctrl Pts',(41.7309154010123,-5.68043298097947,
134.175816828272));
#251754=CARTESIAN_POINT('Ctrl Pts',(41.4524677771993,-0.233911183839542,
137.405824196969));
#251755=CARTESIAN_POINT('Ctrl Pts',(41.1740201533865,5.42756356405245,134.569409035618));
#251756=CARTESIAN_POINT('Ctrl Pts',(40.8955725295735,6.10137254780096,128.273098310918));
#251757=CARTESIAN_POINT('Ctrl Pts',(40.6171249057607,1.1683182287399,124.302893986988));
#251758=CARTESIAN_POINT('Ctrl Pts',(40.3386772819477,-4.83836346701448,
126.307219882257));
#251759=CARTESIAN_POINT('Ctrl Pts',(40.060229658135,-6.39882550377857,132.444198415735));
#251760=CARTESIAN_POINT('Ctrl Pts',(39.781782034322,-2.07907950257448,137.074246123225));
#251761=CARTESIAN_POINT('Ctrl Pts',(39.5033344105091,4.15123899281517,135.94257535195));
#251762=CARTESIAN_POINT('Ctrl Pts',(39.2248867866962,6.56677165310695,130.089136255519));
#251763=CARTESIAN_POINT('Ctrl Pts',(38.9464391628834,2.94776196882331,124.892953407157));
#251764=CARTESIAN_POINT('Ctrl Pts',(38.6679915390704,-3.38009695863112,
125.129064996863));
#251765=CARTESIAN_POINT('Ctrl Pts',(38.3895439152575,-6.6018119080198,130.58049600839));
#251766=CARTESIAN_POINT('Ctrl Pts',(38.1110962914447,-3.75678423037978,
136.237647659355));
#251767=CARTESIAN_POINT('Ctrl Pts',(37.8326486676317,2.54054462586645,136.901873949744));
#251768=CARTESIAN_POINT('Ctrl Pts',(37.5542010438189,6.50323708344635,131.962783367948));
#251769=CARTESIAN_POINT('Ctrl Pts',(37.275753420006,4.48977236213255,125.959158870647));
#251770=CARTESIAN_POINT('Ctrl Pts',(36.9973057961931,-1.64957382240749,
124.4080380775));
#251771=CARTESIAN_POINT('Ctrl Pts',(36.7188581723802,-6.27304225031618,
128.734825220947));
#251772=CARTESIAN_POINT('Ctrl Pts',(36.4404105485673,-5.13189130533538,
134.96341429146));
#251773=CARTESIAN_POINT('Ctrl Pts',(36.1619629247544,0.725217042420823,
137.370036216732));
#251774=CARTESIAN_POINT('Ctrl Pts',(35.8835153009416,5.91588635701427,133.743123017455));
#251775=CARTESIAN_POINT('Ctrl Pts',(35.6050676771286,5.67014511662727,127.415630739204));
#251776=CARTESIAN_POINT('Ctrl Pts',(35.3266200533158,0.213817516048174,
124.202215670509));
#251777=CARTESIAN_POINT('Ctrl Pts',(35.0481724295028,-5.43899793621292,
127.055849275448));
#251778=CARTESIAN_POINT('Ctrl Pts',(34.76972480569,-6.09363999491508,133.354181678833));
#251779=CARTESIAN_POINT('Ctrl Pts',(34.4912771818771,-1.14852458915375,
137.309353092597));
#251780=CARTESIAN_POINT('Ctrl Pts',(34.2128295580642,4.85202880549439,135.286754208357));
#251781=CARTESIAN_POINT('Ctrl Pts',(33.9343819342512,6.393804762678,129.145054591279));
#251782=CARTESIAN_POINT('Ctrl Pts',(33.6559343104384,2.05998649768791,124.528176150753));
#251783=CARTESIAN_POINT('Ctrl Pts',(33.3774866866255,-4.16685872274224,
125.678804626571));
#251784=CARTESIAN_POINT('Ctrl Pts',(33.0990390628127,-6.56456433933747,
131.539568660782));
#251785=CARTESIAN_POINT('Ctrl Pts',(32.8205914389997,-2.92975602487846,
136.724712420187));
#251786=CARTESIAN_POINT('Ctrl Pts',(32.5421438151868,3.39735494990529,136.469342098247));
#251787=CARTESIAN_POINT('Ctrl Pts',(32.263696191374,6.60246269574222,131.008130545292));
#251788=CARTESIAN_POINT('Ctrl Pts',(31.985248567561,3.74022977242616,125.359664383471));
#251789=CARTESIAN_POINT('Ctrl Pts',(31.7068009437482,-2.55909159136699,
124.714608072585));
#251790=CARTESIAN_POINT('Ctrl Pts',(31.4283533199352,-6.50673280126843,
129.665736849585));
#251791=CARTESIAN_POINT('Ctrl Pts',(31.1499056961224,-4.47500443837311,
135.663205244496));
#251792=CARTESIAN_POINT('Ctrl Pts',(30.8714580723094,1.66903438726656,137.195632795014));
#251793=CARTESIAN_POINT('Ctrl Pts',(30.5930104484966,6.27931214787105,132.854793445461));
#251794=CARTESIAN_POINT('Ctrl Pts',(30.3145628246837,5.11920880603445,126.629706496284));
#251795=CARTESIAN_POINT('Ctrl Pts',(30.0361152008708,-0.745197341294603,
124.240922741373));
#251796=CARTESIAN_POINT('Ctrl Pts',(29.7576675770579,-5.9248035368878,127.883617752917));
#251797=CARTESIAN_POINT('Ctrl Pts',(29.4792199532451,-5.65980472482494,
134.210332770852));
#251798=CARTESIAN_POINT('Ctrl Pts',(29.2007723294321,-0.193721867480399,
137.407125770907));
#251799=CARTESIAN_POINT('Ctrl Pts',(28.9223247056193,5.45038192223944,134.536300158051));
#251800=CARTESIAN_POINT('Ctrl Pts',(28.6438770818064,6.08585099138068,128.236004422871));
#251801=CARTESIAN_POINT('Ctrl Pts',(28.3654294579935,1.12872030979243,124.29590255944));
#251802=CARTESIAN_POINT('Ctrl Pts',(28.0869818341806,-4.86564919544231,
126.336755695574));
#251803=CARTESIAN_POINT('Ctrl Pts',(27.8085342103677,-6.38872479024353,
132.483119500384));
#251804=CARTESIAN_POINT('Ctrl Pts',(27.5300865865548,-2.04087440936798,
137.086785903815));
#251805=CARTESIAN_POINT('Ctrl Pts',(27.2516389627419,4.18243985145892,135.91721038272));
#251806=CARTESIAN_POINT('Ctrl Pts',(26.973191338929,6.56229621234102,130.049175704046));
#251807=CARTESIAN_POINT('Ctrl Pts',(26.6947437151162,2.91172294007416,124.875119068062));
#251808=CARTESIAN_POINT('Ctrl Pts',(26.4162960913032,-3.41458146854746,
125.149745756519));
#251809=CARTESIAN_POINT('Ctrl Pts',(26.1378484674903,-6.60305231915217,
130.620687258984));
#251810=CARTESIAN_POINT('Ctrl Pts',(25.8594008436774,-3.72364066549499,
136.260415605043));
#251811=CARTESIAN_POINT('Ctrl Pts',(25.5809532198646,2.57761484979243,136.886295960714));
#251812=CARTESIAN_POINT('Ctrl Pts',(25.3025055960517,6.51016824160669,131.92317485509));
#251813=CARTESIAN_POINT('Ctrl Pts',(25.0240579722387,4.46019505878377,125.931918122295));
#251814=CARTESIAN_POINT('Ctrl Pts',(24.7456103484259,-1.68847949041943,
124.418198010604));
#251815=CARTESIAN_POINT('Ctrl Pts',(24.467162724613,-6.28552387473587,128.773049353324));
#251816=CARTESIAN_POINT('Ctrl Pts',(24.1887151008001,-5.10647888308236,
134.994576512808));
#251817=CARTESIAN_POINT('Ctrl Pts',(23.9102674769872,0.765170736761864,
137.365499967992));
#251818=CARTESIAN_POINT('Ctrl Pts',(23.6318198531744,5.93366583019039,133.707056889611));
#251819=CARTESIAN_POINT('Ctrl Pts',(23.3533722293614,5.64941190136517,127.381177741815));
#251820=CARTESIAN_POINT('Ctrl Pts',(23.0749246055485,0.173624424299845,
124.201036425055));
#251821=CARTESIAN_POINT('Ctrl Pts',(22.7964769817356,-5.46171541667246,
127.08902745089));
#251822=CARTESIAN_POINT('Ctrl Pts',(22.5180293579228,-6.07800560935413,
133.391228152785));
#251823=CARTESIAN_POINT('Ctrl Pts',(22.2395817341099,-1.10890557412062,
137.316223965318));
#251824=CARTESIAN_POINT('Ctrl Pts',(21.9611341102969,4.87922451068073,135.257135483476));
#251825=CARTESIAN_POINT('Ctrl Pts',(21.6826864864842,6.38358563353538,129.106164430008));
#251826=CARTESIAN_POINT('Ctrl Pts',(21.4042388626712,2.02174341466617,124.515752711409));
#251827=CARTESIAN_POINT('Ctrl Pts',(21.1257912388583,-4.19798223462457,
125.704264442993));
#251828=CARTESIAN_POINT('Ctrl Pts',(20.8473436150454,-6.55996729312864,
131.579515405459));
#251829=CARTESIAN_POINT('Ctrl Pts',(20.5688959912325,-2.89366288146616,
136.742436986267));
#251830=CARTESIAN_POINT('Ctrl Pts',(20.2904483674196,3.43177635497322,136.448556475397));
#251831=CARTESIAN_POINT('Ctrl Pts',(20.0120007436067,6.60358077278748,130.967935705476));
#251832=CARTESIAN_POINT('Ctrl Pts',(19.7335531197938,3.70701706326526,125.336997420853));
#251833=CARTESIAN_POINT('Ctrl Pts',(19.455105495981,-2.59611422954622,124.730298818468));
#251834=CARTESIAN_POINT('Ctrl Pts',(19.176657872168,-6.51354337263571,129.705366275038));
#251835=CARTESIAN_POINT('Ctrl Pts',(18.8982102483552,-4.4453443605568,135.690355843533));
#251836=CARTESIAN_POINT('Ctrl Pts',(18.6197626245423,1.70790895172861,137.1853544935));
#251837=CARTESIAN_POINT('Ctrl Pts',(18.3413150007294,6.29167737336628,132.816531500364));
#251838=CARTESIAN_POINT('Ctrl Pts',(18.0628673769165,5.09370165440758,126.598621765949));
#251839=CARTESIAN_POINT('Ctrl Pts',(17.7844197531036,-0.785137043792105,
124.245580574404));
#251840=CARTESIAN_POINT('Ctrl Pts',(17.5059721292907,-5.94247315482366,
127.919737828307));
#251841=CARTESIAN_POINT('Ctrl Pts',(17.2275245054778,-5.63896674252494,
134.244722503881));
#251842=CARTESIAN_POINT('Ctrl Pts',(16.949076881665,-0.15352537268619,137.408182676953));
#251843=CARTESIAN_POINT('Ctrl Pts',(16.6706292578521,5.47299831451989,134.503052992091));
#251844=CARTESIAN_POINT('Ctrl Pts',(16.3921816340391,6.07010392151387,128.199005706208));
#251845=CARTESIAN_POINT('Ctrl Pts',(16.1137340102263,1.08908056569879,124.289152305198));
#251846=CARTESIAN_POINT('Ctrl Pts',(15.8352863864134,-4.89275462544986,
126.366457057635));
#251847=CARTESIAN_POINT('Ctrl Pts',(15.5568387626005,-6.37838734016194,
132.521978378005));
#251848=CARTESIAN_POINT('Ctrl Pts',(15.2783911387876,-2.00259369080969,
137.099092886824));
#251849=CARTESIAN_POINT('Ctrl Pts',(14.9999435149747,4.21348572825588,135.891655954962));
#251850=CARTESIAN_POINT('Ctrl Pts',(14.7214958911618,6.55757760327567,130.009243136227));
#251851=CARTESIAN_POINT('Ctrl Pts',(14.4430482673489,2.87557601636067,124.857504439193));
#251852=CARTESIAN_POINT('Ctrl Pts',(14.164600643536,-3.44893944989177,125.170636050008));
#251853=CARTESIAN_POINT('Ctrl Pts',(13.8861530197231,-6.60404805175259,
130.660885315664));
#251854=CARTESIAN_POINT('Ctrl Pts',(13.6077053959103,-3.69035911973598,
136.282981374608));
#251855=CARTESIAN_POINT('Ctrl Pts',(13.3292577720973,2.61458955925225,136.870492603333));
#251856=CARTESIAN_POINT('Ctrl Pts',(13.0508101482845,6.5168581630887,131.883524884162));
#251857=CARTESIAN_POINT('Ctrl Pts',(12.7723625244716,4.43045248126686,125.904857924092));
#251858=CARTESIAN_POINT('Ctrl Pts',(12.4939149006587,-1.72732259120293,
124.428594585312));
#251859=CARTESIAN_POINT('Ctrl Pts',(12.2154672768458,-6.29777258675688,
128.811348756686));
#251860=CARTESIAN_POINT('Ctrl Pts',(11.9370196530329,-5.08087723837641,
135.025583464166));
#251861=CARTESIAN_POINT('Ctrl Pts',(11.65857202922,0.805096077419857,137.36072059382));
#251862=CARTESIAN_POINT('Ctrl Pts',(11.3801244054071,5.95122542919731,133.670883201288));
#251863=CARTESIAN_POINT('Ctrl Pts',(11.1016767815943,5.62846934506734,127.346851591727));
#251864=CARTESIAN_POINT('Ctrl Pts',(10.8232291577813,0.13342489883439,124.200101868207));
#251865=CARTESIAN_POINT('Ctrl Pts',(10.5447815339684,-5.4842305112587,127.12234329937));
#251866=CARTESIAN_POINT('Ctrl Pts',(10.2663339101556,-6.06214600106014,
133.428178769409));
#251867=CARTESIAN_POINT('Ctrl Pts',(9.98788628634267,-1.06924546818365,
137.322853538546));
#251868=CARTESIAN_POINT('Ctrl Pts',(9.70943866252976,4.90623941440849,135.227351759386));
#251869=CARTESIAN_POINT('Ctrl Pts',(9.43099103871685,6.37312995827954,129.067337196021));
#251870=CARTESIAN_POINT('Ctrl Pts',(9.15254341490403,1.98342541519871,124.503562298745));
#251871=CARTESIAN_POINT('Ctrl Pts',(8.87409579109107,-4.22895018873139,
125.729913245354));
#251872=CARTESIAN_POINT('Ctrl Pts',(8.59564816727821,-6.55512716491932,
131.61943342649));
#251873=CARTESIAN_POINT('Ctrl Pts',(8.31720054346528,-2.85746251231165,
136.759941514744));
#251874=CARTESIAN_POINT('Ctrl Pts',(8.03875291965246,3.46607059430627,136.427561704794));
#251875=CARTESIAN_POINT('Ctrl Pts',(7.76030529583951,6.60445415171875,130.927734804324));
#251876=CARTESIAN_POINT('Ctrl Pts',(7.48185767202662,3.67366698922382,125.314533053388));
#251877=CARTESIAN_POINT('Ctrl Pts',(7.20341004821377,-2.63304066775796,
124.746214640945));
#251878=CARTESIAN_POINT('Ctrl Pts',(6.92496242440086,-6.52011258225796,
129.745036424131));
#251879=CARTESIAN_POINT('Ctrl Pts',(6.64651480058794,-4.41551955887045,
135.71732539022));
#251880=CARTESIAN_POINT('Ctrl Pts',(6.36806717677509,1.74672022899638,137.174839741911));
#251881=CARTESIAN_POINT('Ctrl Pts',(6.08961955296221,6.30380945844269,132.778194993536));
#251882=CARTESIAN_POINT('Ctrl Pts',(5.81117192914928,5.06800575379271,126.567692880813));
#251883=CARTESIAN_POINT('Ctrl Pts',(5.53272430533639,-0.825047652747706,
124.250481445441));
#251884=CARTESIAN_POINT('Ctrl Pts',(5.25427668152353,-5.95992257223146,
127.955964794454));
#251885=CARTESIAN_POINT('Ctrl Pts',(4.97582905771062,-5.61791980623858,
134.278984753035));
#251886=CARTESIAN_POINT('Ctrl Pts',(4.69738143389771,-0.113323188952861,
137.408994875945));
#251887=CARTESIAN_POINT('Ctrl Pts',(4.41893381008486,5.49541190283514,134.469668769726));
#251888=CARTESIAN_POINT('Ctrl Pts',(4.14048618627195,6.05413192171396,128.162103531929));
#251889=CARTESIAN_POINT('Ctrl Pts',(3.86203856245905,1.0494004653243,124.282643474398));
#251890=CARTESIAN_POINT('Ctrl Pts',(3.58359093864613,-4.91967875263547,
126.396322867843));
#251891=CARTESIAN_POINT('Ctrl Pts',(3.30514331483329,-6.36781353659179,
132.560773608667));
#251892=CARTESIAN_POINT('Ctrl Pts',(3.02669569102039,-1.96423876540577,
137.111166616214));
#251893=CARTESIAN_POINT('Ctrl Pts',(2.74824806720748,4.24437547278969,135.865913015604));
#251894=CARTESIAN_POINT('Ctrl Pts',(2.46980044339459,6.55261600076067,129.969340031779));
#251895=CARTESIAN_POINT('Ctrl Pts',(2.19135281958173,2.83932253712042,124.840110173268));
#251896=CARTESIAN_POINT('Ctrl Pts',(1.91290519576881,-3.48316962951642,
125.191735103234));
#251897=CARTESIAN_POINT('Ctrl Pts',(1.6344575719559,-6.60479906892382,130.701088688872));
#251898=CARTESIAN_POINT('Ctrl Pts',(1.35600994814304,-3.65694082636265,
136.305344131865));
#251899=CARTESIAN_POINT('Ctrl Pts',(1.07756232433016,2.65146738413444,136.854464463202));
#251900=CARTESIAN_POINT('Ctrl Pts',(0.799114700517227,6.52330659999492,
131.843834924404));
#251901=CARTESIAN_POINT('Ctrl Pts',(0.520667076704378,4.40054573170394,
125.877979278764));
#251902=CARTESIAN_POINT('Ctrl Pts',(0.242219452891471,-1.76610168541259,
124.439227416375));
#251903=CARTESIAN_POINT('Ctrl Pts',(-0.03622817092143,-6.30978793249869,
128.849722011837));
#251904=CARTESIAN_POINT('Ctrl Pts',(-0.314675794734322,-5.05508731989592,
135.056433996558));
#251905=CARTESIAN_POINT('Ctrl Pts',(-0.593123418547181,0.844991584946641,
137.355698271319));
#251906=CARTESIAN_POINT('Ctrl Pts',(-0.871571042360099,5.96856450335716,
133.634603292916));
#251907=CARTESIAN_POINT('Ctrl Pts',(-1.15001866617301,5.60731822376822,
127.312653560908));
#251908=CARTESIAN_POINT('Ctrl Pts',(-1.42846628998586,0.0932204292604712,
124.199412034595));
#251909=CARTESIAN_POINT('Ctrl Pts',(-1.70691391379876,-5.50654238566651,
127.155795586355));
#251910=CARTESIAN_POINT('Ctrl Pts',(-1.98536153761166,-6.04606175771675,
133.465032159487));
#251911=CARTESIAN_POINT('Ctrl Pts',(-2.26380916142456,-1.02954574096264,
137.329241566624));
#251912=CARTESIAN_POINT('Ctrl Pts',(-2.5422567852374,4.9330725156305,135.197404139731));
#251913=CARTESIAN_POINT('Ctrl Pts',(-2.82070440905033,6.36243812434939,
129.028574328076));
#251914=CARTESIAN_POINT('Ctrl Pts',(-3.09915203286324,1.94503391917308,
124.491605364478));
#251915=CARTESIAN_POINT('Ctrl Pts',(-3.3775996566761,-4.25976143753379,
125.755750083229));
#251916=CARTESIAN_POINT('Ctrl Pts',(-3.65604728048899,-6.55004413406227,
131.659321244699));
#251917=CARTESIAN_POINT('Ctrl Pts',(-3.9344949043019,-2.82115625883292,
136.777225356981));
#251918=CARTESIAN_POINT('Ctrl Pts',(-4.2129425281148,3.50023639711881,136.406358564405));
#251919=CARTESIAN_POINT('Ctrl Pts',(-4.49139015192765,6.60508280017262,
130.887529331496));
#251920=CARTESIAN_POINT('Ctrl Pts',(-4.76983777574057,3.64018078610111,
125.292272113504));
#251921=CARTESIAN_POINT('Ctrl Pts',(-5.04828539955349,-2.66986953767946,
124.762354950249));
#251922=CARTESIAN_POINT('Ctrl Pts',(-5.32673302336633,-6.52644018671072,
129.784745826872));
#251923=CARTESIAN_POINT('Ctrl Pts',(-5.60518064717923,-4.38553113848304,
135.74411288519));
#251924=CARTESIAN_POINT('Ctrl Pts',(-5.88362827099213,1.7854667809037,137.164088929876));
#251925=CARTESIAN_POINT('Ctrl Pts',(-6.16207589480503,6.31570795354138,
132.739785345549));
#251926=CARTESIAN_POINT('Ctrl Pts',(-6.44052351861788,5.04212205636089,
126.536920986959));
#251927=CARTESIAN_POINT('Ctrl Pts',(-6.71897114243081,-0.864927689259141,
124.255625172881));
#251928=CARTESIAN_POINT('Ctrl Pts',(-6.99741876624371,-5.97715114251656,
127.992297308957));
#251929=CARTESIAN_POINT('Ctrl Pts',(-7.27586639005655,-5.59666469586782,
134.313118248714));
#251930=CARTESIAN_POINT('Ctrl Pts',(-7.55431401386947,-0.0731168059870705,
137.409562337785));
#251931=CARTESIAN_POINT('Ctrl Pts',(-7.83276163768236,5.51762185664139,
134.436148728019));
#251932=CARTESIAN_POINT('Ctrl Pts',(-8.11120926149529,6.03793558382929,
128.125299267457));
#251933=CARTESIAN_POINT('Ctrl Pts',(-8.38965688530811,1.00968147902963,
124.276376308223));
#251934=CARTESIAN_POINT('Ctrl Pts',(-8.66810450912106,-4.94642057931569,
126.426352019512));
#251935=CARTESIAN_POINT('Ctrl Pts',(-8.94655213293394,-6.3570037713493,
132.599503754801));
#251936=CARTESIAN_POINT('Ctrl Pts',(-9.22499975674682,-1.92581105441205,
137.123006644589));
#251937=CARTESIAN_POINT('Ctrl Pts',(-9.50344738055969,4.27510794042973,
135.839982518561));
#251938=CARTESIAN_POINT('Ctrl Pts',(-9.78189500437264,6.54741158865002,
129.929467869325));
#251939=CARTESIAN_POINT('Ctrl Pts',(-10.0603426281855,2.80296384573913,
124.822936914835));
#251940=CARTESIAN_POINT('Ctrl Pts',(-10.3387902519984,-3.51727073900952,
125.213042134361));
#251941=CARTESIAN_POINT('Ctrl Pts',(-10.6172378758113,-6.60530534283666,
130.74129588886));
#251942=CARTESIAN_POINT('Ctrl Pts',(-10.8956854996242,-3.62338702370218,
136.327503048155));
#251943=CARTESIAN_POINT('Ctrl Pts',(-11.174133123437,2.68824695791763,136.838212134247));
#251944=CARTESIAN_POINT('Ctrl Pts',(-11.4525807472499,6.52951331337615,
131.804106446543));
#251945=CARTESIAN_POINT('Ctrl Pts',(-11.7310283710628,4.37047591830066,
125.851283182307));
#251946=CARTESIAN_POINT('Ctrl Pts',(-12.0094759948757,-1.80481533607482,
124.450096109789));
#251947=CARTESIAN_POINT('Ctrl Pts',(-12.2879236186886,-6.32156946672825,
128.88816769684));
#251948=CARTESIAN_POINT('Ctrl Pts',(-12.5663712425015,-5.02911008329581,
135.087126966809));
#251949=CARTESIAN_POINT('Ctrl Pts',(-12.8448188663144,0.884855780999501,
137.350433186591));
#251950=CARTESIAN_POINT('Ctrl Pts',(-13.1232664901273,5.98568241016441,
133.598218508862));
#251951=CARTESIAN_POINT('Ctrl Pts',(-13.4017141139402,5.58595932123025,
127.278584916578));
#251952=CARTESIAN_POINT('Ctrl Pts',(-13.6801617377531,0.0530125053692662,
124.198966949783));
#251953=CARTESIAN_POINT('Ctrl Pts',(-13.958609361566,-5.5286502131212,127.189383072259));
#251954=CARTESIAN_POINT('Ctrl Pts',(-14.2370569853788,-6.02975347533148,
133.501786957402));
#251955=CARTESIAN_POINT('Ctrl Pts',(-14.5155046091917,-0.989807863545592,
137.335387812837));
#251956=CARTESIAN_POINT('Ctrl Pts',(-14.7939522330047,4.95972282003631,
135.167293734234));
#251957=CARTESIAN_POINT('Ctrl Pts',(-15.0723998568175,6.35151052793477,
128.989877262545));
#251958=CARTESIAN_POINT('Ctrl Pts',(-15.3508474806304,1.9065703492003,124.479882351679));
#251959=CARTESIAN_POINT('Ctrl Pts',(-15.6292951044433,-4.29041483930959,
125.781773999224));
#251960=CARTESIAN_POINT('Ctrl Pts',(-15.9077427282562,-6.54471838891106,
131.699177382027));
#251961=CARTESIAN_POINT('Ctrl Pts',(-16.186190352069,-2.78474546637155,
136.794287872519));
#251962=CARTESIAN_POINT('Ctrl Pts',(-16.464637975882,3.53427249738445,136.384947839923));
#251963=CARTESIAN_POINT('Ctrl Pts',(-16.7430855996949,6.60546669485434,
130.847320776822));
#251964=CARTESIAN_POINT('Ctrl Pts',(-17.0215332235078,3.6065596947407,125.270215426085));
#251965=CARTESIAN_POINT('Ctrl Pts',(-17.2999808473206,-2.7065994746034,
124.778719148295));
#251966=CARTESIAN_POINT('Ctrl Pts',(-17.5784284711336,-6.53252595152224,
129.824493011814));
#251967=CARTESIAN_POINT('Ctrl Pts',(-17.8568760949464,-4.35538021062653,
135.770717335825));
#251968=CARTESIAN_POINT('Ctrl Pts',(-18.1353237187593,1.82414717168286,
137.153102455769));
#251969=CARTESIAN_POINT('Ctrl Pts',(-18.4137713425722,6.32737241775927,
132.701303979686));
#251970=CARTESIAN_POINT('Ctrl Pts',(-18.6922189663851,5.01605152124203,
126.506307224649));
#251971=CARTESIAN_POINT('Ctrl Pts',(-18.9706665901979,-0.904775675556959,
124.261011566121));
#251972=CARTESIAN_POINT('Ctrl Pts',(-19.2491142140109,-5.99415822726801,
128.028734025499));
#251973=CARTESIAN_POINT('Ctrl Pts',(-19.5275618378238,-5.57520219902858,
134.347121726088));
#251974=CARTESIAN_POINT('Ctrl Pts',(-19.8060094616367,-0.0329077136511566,
137.409885041447));
#251975=CARTESIAN_POINT('Ctrl Pts',(-20.0844570854496,5.53962735294063,
134.402494109067));
#251976=CARTESIAN_POINT('Ctrl Pts',(-20.3629047092624,6.02151550802112,
128.08859427659));
#251977=CARTESIAN_POINT('Ctrl Pts',(-20.6413523330754,0.969925078616457,
124.270351038909));
#251978=CARTESIAN_POINT('Ctrl Pts',(-20.9197999568882,-4.9729791145623,
126.456543399899));
#251979=CARTESIAN_POINT('Ctrl Pts',(-21.1982475807011,-6.34595844499429,
132.638167381246));
#251980=CARTESIAN_POINT('Ctrl Pts',(-21.476695204514,-1.88731198178147,
137.134612533211));
#251981=CARTESIAN_POINT('Ctrl Pts',(-21.7551428283269,4.30568199237261,
135.813865424697));
#251982=CARTESIAN_POINT('Ctrl Pts',(-22.0335904521398,6.54196455979519,
129.889628126344));
#251983=CARTESIAN_POINT('Ctrl Pts',(-22.3120380759527,2.766501289502,124.805985300257));
#251984=CARTESIAN_POINT('Ctrl Pts',(-22.5904856997656,-3.5512415147419,
125.234556353852));
#251985=CARTESIAN_POINT('Ctrl Pts',(-22.8689333235784,-6.60556685473091,
130.781505425734));
#251986=CARTESIAN_POINT('Ctrl Pts',(-23.1473809473914,-3.58969895510304,
136.349457302372));
#251987=CARTESIAN_POINT('Ctrl Pts',(-23.4258285712042,2.7249269177212,136.821736218705));
#251988=CARTESIAN_POINT('Ctrl Pts',(-23.7042761950172,6.53547807324032,
131.764340922733));
#251989=CARTESIAN_POINT('Ctrl Pts',(-23.98272381883,4.34024415530499,125.824770623956));
#251990=CARTESIAN_POINT('Ctrl Pts',(-24.2611714426429,-1.84346210864104,
124.461200262812));
#251991=CARTESIAN_POINT('Ctrl Pts',(-24.5396190664558,-6.33311675287646,
128.926684387076));
#251992=CARTESIAN_POINT('Ctrl Pts',(-24.8180666902687,-5.00294649117208,
135.117661237576));
#251993=CARTESIAN_POINT('Ctrl Pts',(-25.0965143140816,0.924687188395989,
137.344925534737));
#251994=CARTESIAN_POINT('Ctrl Pts',(-25.3749619378945,6.00257851530871,
133.561730197376));
#251995=CARTESIAN_POINT('Ctrl Pts',(-25.6534095617074,5.56439342891538,
127.244646921163));
#251996=CARTESIAN_POINT('Ctrl Pts',(-25.9318571855203,0.0128026170801758,
124.198766630261));
#251997=CARTESIAN_POINT('Ctrl Pts',(-26.2103048093331,-5.5505531744091,
127.223104512485));
#251998=CARTESIAN_POINT('Ctrl Pts',(-26.4887524331461,-6.01322175821376,
133.538441801192));
#251999=CARTESIAN_POINT('Ctrl Pts',(-26.7672000569589,-0.950033308434149,
137.341292049436));
#252000=CARTESIAN_POINT('Ctrl Pts',(-27.0456476807718,4.98618934008908,
135.137021658645));
#252001=CARTESIAN_POINT('Ctrl Pts',(-27.3240953045847,6.34034757396176,
128.951247433362));
#252002=CARTESIAN_POINT('Ctrl Pts',(-27.6025429283976,1.86803613056208,
124.468393694749));
#252003=CARTESIAN_POINT('Ctrl Pts',(-27.8809905522105,-4.32090925818572,
125.807984029013));
#252004=CARTESIAN_POINT('Ctrl Pts',(-28.1594381760234,-6.53915012681315,
131.739000361591));
#252005=CARTESIAN_POINT('Ctrl Pts',(-28.4378857998363,-2.74823148414282,
136.811128429099));
#252006=CARTESIAN_POINT('Ctrl Pts',(-28.7163334236492,3.56817763388296,
136.36333032473));
#252007=CARTESIAN_POINT('Ctrl Pts',(-28.994781047462,6.60560582153853,130.807110630244));
#252008=CARTESIAN_POINT('Ctrl Pts',(-29.273228671275,3.5728049609845,125.248363808452));
#252009=CARTESIAN_POINT('Ctrl Pts',(-29.5516762950878,-2.74322911748845,
124.795306628702));
#252010=CARTESIAN_POINT('Ctrl Pts',(-29.8301239189007,-6.53836965118233,
129.86427650611));
#252011=CARTESIAN_POINT('Ctrl Pts',(-30.1085715427137,-4.32506789255462,
135.797137756284));
#252012=CARTESIAN_POINT('Ctrl Pts',(-30.3870191665265,1.862759968018,137.141880726698));
#252013=CARTESIAN_POINT('Ctrl Pts',(-30.6654667903394,6.33880241886542,
132.662752321889));
#252014=CARTESIAN_POINT('Ctrl Pts',(-30.9439144141524,4.98979511448915,
126.475852728289));
#252015=CARTESIAN_POINT('Ctrl Pts',(-31.2223620379652,-0.944590135059391,
124.266640425567));
#252016=CARTESIAN_POINT('Ctrl Pts',(-31.5008096617781,-6.01094319628198,
128.065273593905));
#252017=CARTESIAN_POINT('Ctrl Pts',(-31.7792572855909,-5.55353311102158,
134.380993925146));
#252018=CARTESIAN_POINT('Ctrl Pts',(-32.0577049094039,0.00730259809219468,
137.409962974972));
#252019=CARTESIAN_POINT('Ctrl Pts',(-32.3361525332168,5.56142757631112,
134.368706159956));
#252020=CARTESIAN_POINT('Ctrl Pts',(-32.6146001570296,6.0048723027414,128.051989919443));
#252021=CARTESIAN_POINT('Ctrl Pts',(-32.8930477808425,0.930132737272799,
124.264567889721));
#252022=CARTESIAN_POINT('Ctrl Pts',(-33.1714954046555,-4.99935337423901,
126.486895890252));
#252023=CARTESIAN_POINT('Ctrl Pts',(-33.4499430284683,-6.33467796681538,
132.676763055306));
#252024=CARTESIAN_POINT('Ctrl Pts',(-33.7283906522812,-1.84874297411136,
137.145983852021));
#252025=CARTESIAN_POINT('Ctrl Pts',(-34.0068382760941,4.33609649568588,
135.787562701789));
#252026=CARTESIAN_POINT('Ctrl Pts',(-34.285285899907,6.53627511603778,129.849822279112));
#252027=CARTESIAN_POINT('Ctrl Pts',(-34.5637335237199,2.72993621954223,
124.789255957683));
#252028=CARTESIAN_POINT('Ctrl Pts',(-34.8421811475328,-3.58508069791401,
125.256276964487));
#252029=CARTESIAN_POINT('Ctrl Pts',(-35.1206287713457,-6.60558359491616,
130.821715809516));
#252030=CARTESIAN_POINT('Ctrl Pts',(-35.3990763951586,-3.55587786888901,
136.37120608099));
#252031=CARTESIAN_POINT('Ctrl Pts',(-35.6775240189714,2.76150590435573,
136.805037327097));
#252032=CARTESIAN_POINT('Ctrl Pts',(-35.9559716427844,6.54120065856107,
131.724539826499));
#252033=CARTESIAN_POINT('Ctrl Pts',(-36.2344192665972,4.30985156296601,
125.798442586144));
#252034=CARTESIAN_POINT('Ctrl Pts',(-36.5128668904101,-1.8820405710409,
124.472539463974));
#252035=CARTESIAN_POINT('Ctrl Pts',(-36.791314514223,-6.3444293630544,128.965270655295));
#252036=CARTESIAN_POINT('Ctrl Pts',(-37.0697621380359,-4.9765975130263,
135.148035677403));
#252037=CARTESIAN_POINT('Ctrl Pts',(-37.3482097618488,0.964484331168655,
137.339175519844));
#252038=CARTESIAN_POINT('Ctrl Pts',(-37.6266573856617,6.0192521926987,133.525139710547));
#252039=CARTESIAN_POINT('Ctrl Pts',(-37.9051050094746,5.54262134595571,
127.210840832248));
#252040=CARTESIAN_POINT('Ctrl Pts',(-38.1835526332875,-0.0274077456145885,
124.198811083455));
#252041=CARTESIAN_POINT('Ctrl Pts',(-38.4620002571004,-5.5722504579079,
127.256958657474));
#252042=CARTESIAN_POINT('Ctrl Pts',(-38.7404478809132,-5.99646721895241,
133.574995332598));
#252043=CARTESIAN_POINT('Ctrl Pts',(-39.0188955047262,-0.910223549489097,
137.346954057637));
#252044=CARTESIAN_POINT('Ctrl Pts',(-39.297343128539,5.0124710950622,135.106589034709));
#252045=CARTESIAN_POINT('Ctrl Pts',(-39.5757907523519,6.32894967607775,
128.912686271968));
#252046=CARTESIAN_POINT('Ctrl Pts',(-39.8542383761648,1.82943269115809,
124.457139819403));
#252047=CARTESIAN_POINT('Ctrl Pts',(-40.1326859999777,-4.35124356418029,
125.834379201373));
#252048=CARTESIAN_POINT('Ctrl Pts',(-40.4111336237906,-6.53333955410249,
131.778788707735));
#252049=CARTESIAN_POINT('Ctrl Pts',(-40.6895812476035,-2.7116156651858,
136.827746402689));
#252050=CARTESIAN_POINT('Ctrl Pts',(-40.9680288714165,3.60195055024708,
136.34150681987));
#252051=CARTESIAN_POINT('Ctrl Pts',(-41.2464764952292,6.60550017506977,
130.766900381762));
#252052=CARTESIAN_POINT('Ctrl Pts',(-41.5249241190422,3.53891783562657,
125.226718070324));
#252053=CARTESIAN_POINT('Ctrl Pts',(-41.803371742855,-2.77975710900975,
124.812116776814));
#252054=CARTESIAN_POINT('Ctrl Pts',(-42.081819366668,-6.5439710691505,129.904094835568));
#252055=CARTESIAN_POINT('Ctrl Pts',(-42.3602669904808,-4.2945953075014,
135.82337316755));
#252056=CARTESIAN_POINT('Ctrl Pts',(-42.6387146142937,1.90130373909722,
137.130424158489));
#252057=CARTESIAN_POINT('Ctrl Pts',(-42.9171622381066,6.34999753331677,
132.624131800705));
#252058=CARTESIAN_POINT('Ctrl Pts',(-43.1956098619195,4.96335380904355,
126.44555862638));
#252059=CARTESIAN_POINT('Ctrl Pts',(-43.4740574857324,-0.984369592426984,
124.272511542639));
#252060=CARTESIAN_POINT('Ctrl Pts',(-43.7525051095453,-6.02750542758532,
128.101914660188));
#252061=CARTESIAN_POINT('Ctrl Pts',(-44.0309527333582,-5.53165823480283,
134.414733590743));
#252062=CARTESIAN_POINT('Ctrl Pts',(-44.3094003571711,0.0475126392350714,
137.409796135472));
#252063=CARTESIAN_POINT('Ctrl Pts',(-44.5878479809839,5.58302171893757,
134.334786132711));
#252064=CARTESIAN_POINT('Ctrl Pts',(-44.8662956047969,5.98800658471021,
128.015487552405));
#252065=CARTESIAN_POINT('Ctrl Pts',(-45.1447432286098,0.890305929518511,
124.259027074959));
#252066=CARTESIAN_POINT('Ctrl Pts',(-45.4231908524226,-5.02554238103793,
126.517408365848));
#252067=CARTESIAN_POINT('Ctrl Pts',(-45.7016384762356,-6.32316275481482,
132.715289346806));
#252068=CARTESIAN_POINT('Ctrl Pts',(-45.9800861000484,-1.81010546059046,
137.15712017965));
#252069=CARTESIAN_POINT('Ctrl Pts',(-46.2585337238614,4.36635032334889,
135.761075324496));
#252070=CARTESIAN_POINT('Ctrl Pts',(-46.5369813476741,6.53034346820225,
129.810051802649));
#252071=CARTESIAN_POINT('Ctrl Pts',(-46.8154289714873,2.6932699907919,124.772749507024));
#252072=CARTESIAN_POINT('Ctrl Pts',(-47.0938765952999,-3.61878703460243,
125.278203161403));
#252073=CARTESIAN_POINT('Ctrl Pts',(-47.3723242191129,-6.60535556277213,
130.861925550195));
#252074=CARTESIAN_POINT('Ctrl Pts',(-47.6507718429257,-3.52192501831287,
136.392748578105));
#252075=CARTESIAN_POINT('Ctrl Pts',(-47.9292194667387,2.79798256237344,
136.788116078208));
#252076=CARTESIAN_POINT('Ctrl Pts',(-48.2076670905515,6.54668085728591,
131.684704632686));
#252077=CARTESIAN_POINT('Ctrl Pts',(-48.4861147143645,4.27929926749242,
125.772300044465));
#252078=CARTESIAN_POINT('Ctrl Pts',(-48.7645623381774,-1.92054929373528,
124.484113293097));
#252079=CARTESIAN_POINT('Ctrl Pts',(-49.0430099619902,-6.35550687806913,
129.003925071669));
#252080=CARTESIAN_POINT('Ctrl Pts',(-49.3214575858032,-4.95006412522954,
135.178249160753));
#252081=CARTESIAN_POINT('Ctrl Pts',(-49.5999052096159,1.00424573461974,
137.333183354982));
#252082=CARTESIAN_POINT('Ctrl Pts',(-49.878352833429,6.03570282448511,133.488448404247));
#252083=CARTESIAN_POINT('Ctrl Pts',(-50.1568004572417,5.52064387912377,
127.17716790253));
#252084=CARTESIAN_POINT('Ctrl Pts',(-50.4352480810547,-0.0676170927052693,
124.199100307716));
#252085=CARTESIAN_POINT('Ctrl Pts',(-50.7136957048675,-5.5937412596168,
127.290944252747));
#252086=CARTESIAN_POINT('Ctrl Pts',(-50.9921433286805,-5.97949047839309,
133.611446197116));
#252087=CARTESIAN_POINT('Ctrl Pts',(-51.2705909524933,-0.870380061875472,
137.352373627632));
#252088=CARTESIAN_POINT('Ctrl Pts',(-51.5490385763063,5.03856711107574,
135.075996990117));
#252089=CARTESIAN_POINT('Ctrl Pts',(-51.8274862001192,6.31731725663583,
128.874195207264));
#252090=CARTESIAN_POINT('Ctrl Pts',(-52.105933823932,1.79076146145295,124.446121142656));
#252091=CARTESIAN_POINT('Ctrl Pts',(-52.3843814477449,-4.38141663324442,
125.860958538224));
#252092=CARTESIAN_POINT('Ctrl Pts',(-52.6628290715579,-6.52728688609205,
131.818540946088));
#252093=CARTESIAN_POINT('Ctrl Pts',(-52.9412766953706,-2.67489936631311,
136.844141177504));
#252094=CARTESIAN_POINT('Ctrl Pts',(-53.2197243191836,3.63558999500893,
136.319478134021));
#252095=CARTESIAN_POINT('Ctrl Pts',(-53.4981719429964,6.60514975936288,
130.726691521383));
#252096=CARTESIAN_POINT('Ctrl Pts',(-53.7766195668094,3.50489957436681,
125.205279013792));
#252097=CARTESIAN_POINT('Ctrl Pts',(-54.0550671906223,-2.8161820956091,
124.829148969725));
#252098=CARTESIAN_POINT('Ctrl Pts',(-54.3335148144351,-6.54932999786417,
129.943946524707));
#252099=CARTESIAN_POINT('Ctrl Pts',(-54.6119624382481,-4.26396358463975,
135.849422597461));
#252100=CARTESIAN_POINT('Ctrl Pts',(-54.890410062061,1.93977705666721,137.11873317567));
#252101=CARTESIAN_POINT('Ctrl Pts',(-55.1688576858738,6.3609573462743,132.58544384723));
#252102=CARTESIAN_POINT('Ctrl Pts',(-55.4473053096868,4.93672858469731,
126.415426041482));
#252103=CARTESIAN_POINT('Ctrl Pts',(-55.7257529334997,-1.02411257361735,
124.278624699781));
#252104=CARTESIAN_POINT('Ctrl Pts',(-56.0042005573125,-6.0438443074584,
128.138655866601));
#252105=CARTESIAN_POINT('Ctrl Pts',(-56.2826481811254,-5.50957838095395,
134.448339472641));
#252106=CARTESIAN_POINT('Ctrl Pts',(-56.5610958049383,0.0877209197796484,
137.40938452913));
#252107=CARTESIAN_POINT('Ctrl Pts',(-56.8395434287512,5.60440898064107,
134.300735284249));
#252108=CARTESIAN_POINT('Ctrl Pts',(-57.117991052564,5.97091897889293,127.979088528083));
#252109=CARTESIAN_POINT('Ctrl Pts',(-57.396438676377,0.850446131150592,
124.253728799937));
#252110=CARTESIAN_POINT('Ctrl Pts',(-57.6748863001899,-5.05154516451579,
126.548079696037));
#252111=CARTESIAN_POINT('Ctrl Pts',(-57.9533339240027,-6.31141323569307,
132.753744828139));
#252112=CARTESIAN_POINT('Ctrl Pts',(-58.2317815478157,-1.77140087294607,
137.168021103437));
#252113=CARTESIAN_POINT('Ctrl Pts',(-58.5102291716285,4.39644235429495,
135.734404274317));
#252114=CARTESIAN_POINT('Ctrl Pts',(-58.7886767954414,6.52416983608798,
129.770318170665));
#252115=CARTESIAN_POINT('Ctrl Pts',(-59.0671244192543,2.65650396193163,
124.756466559932));
#252116=CARTESIAN_POINT('Ctrl Pts',(-59.3455720430672,-3.6523592758065,
125.300334132115));
#252117=CARTESIAN_POINT('Ctrl Pts',(-59.62401966688,-6.60488276674858,130.902133157784));
#252118=CARTESIAN_POINT('Ctrl Pts',(-59.902467290693,-3.48784166150989,
136.414083995446));
#252119=CARTESIAN_POINT('Ctrl Pts',(-60.1809149145059,2.83435554011865,
136.770973099059));
#252120=CARTESIAN_POINT('Ctrl Pts',(-60.4593625383188,6.55191846634393,
131.644836817403));
#252121=CARTESIAN_POINT('Ctrl Pts',(-60.7378101621316,4.24858840101079,
125.746343967642));
#252122=CARTESIAN_POINT('Ctrl Pts',(-61.0162577859445,-1.95898684976931,
124.49592132131));
#252123=CARTESIAN_POINT('Ctrl Pts',(-61.2947054097575,-6.36634888743926,
129.042646203845));
#252124=CARTESIAN_POINT('Ctrl Pts',(-61.5731530335703,-4.92334731098624,
135.208300568055));
#252125=CARTESIAN_POINT('Ctrl Pts',(-61.8516006573832,1.04396992537583,
137.326949262193));
#252126=CARTESIAN_POINT('Ctrl Pts',(-62.1300482811962,6.05192980108374,
133.451657638088));
#252127=CARTESIAN_POINT('Ctrl Pts',(-62.408495905009,5.49846184280268,127.143629379772));
#252128=CARTESIAN_POINT('Ctrl Pts',(-62.6869435288219,-0.107823934219708,
124.199634292325));
#252129=CARTESIAN_POINT('Ctrl Pts',(-62.9653911526347,-5.61502478318622,
127.325060038955));
#252130=CARTESIAN_POINT('Ctrl Pts',(-63.2438387764477,-5.96229216561512,
133.647793044045));
#252131=CARTESIAN_POINT('Ctrl Pts',(-63.5222864002605,-0.830504322008783,
137.357550558596));
#252132=CARTESIAN_POINT('Ctrl Pts',(-63.8007340240734,5.06447642113188,
135.045246658467));
#252133=CARTESIAN_POINT('Ctrl Pts',(-64.0791816478864,6.30545074667997,
128.835775665549));
#252134=CARTESIAN_POINT('Ctrl Pts',(-64.3576292716992,1.75202387442331,
124.435338072814));
#252135=CARTESIAN_POINT('Ctrl Pts',(-64.6360768955121,-4.41142734730395,
125.887721054655));
#252136=CARTESIAN_POINT('Ctrl Pts',(-64.914524519325,-6.52099234706562,
131.858255603616));
#252137=CARTESIAN_POINT('Ctrl Pts',(-65.1929721431379,-2.63808394806071,
136.860312146029));
#252138=CARTESIAN_POINT('Ctrl Pts',(-65.4714197669508,3.66909472164654,
136.297245083462));
#252139=CARTESIAN_POINT('Ctrl Pts',(-65.7498673907637,6.60455458740261,
130.686485539062));
#252140=CARTESIAN_POINT('Ctrl Pts',(-66.0283150145766,3.4707514377644,125.184047433287));
#252141=CARTESIAN_POINT('Ctrl Pts',(-66.3067626383895,-2.85250272754526,
124.846402576302));
#252142=CARTESIAN_POINT('Ctrl Pts',(-66.5852102622024,-6.55444623874626,
129.983830096806));
#252143=CARTESIAN_POINT('Ctrl Pts',(-66.8636578860152,-4.23317385903938,
135.875285080744));
#252144=CARTESIAN_POINT('Ctrl Pts',(-67.1421055098281,1.978178495085,137.106808211453));
#252145=CARTESIAN_POINT('Ctrl Pts',(-67.4205531336411,6.37168145161813,
132.546689895061));
#252146=CARTESIAN_POINT('Ctrl Pts',(-67.6990007574539,4.90992042805787,
126.385456090168));
#252147=CARTESIAN_POINT('Ctrl Pts',(-67.9774483812669,-1.06381760593968,
124.284979670466));
#252148=CARTESIAN_POINT('Ctrl Pts',(-68.2558960050797,-6.05995923045808,
128.175495851683));
#252149=CARTESIAN_POINT('Ctrl Pts',(-68.5343436288926,-5.48729436765201,
134.481810325563));
#252150=CARTESIAN_POINT('Ctrl Pts',(-68.8127912527054,0.12792594979327,
137.408728171199));
#252151=CARTESIAN_POINT('Ctrl Pts',(-69.0912388765185,5.62558856890878,
134.266554876337));
#252152=CARTESIAN_POINT('Ctrl Pts',(-69.3696865003312,5.9536101184771,127.942794195258));
#252153=CARTESIAN_POINT('Ctrl Pts',(-69.6481341241442,0.810554819188534,
124.248673260987));
#252154=CARTESIAN_POINT('Ctrl Pts',(-69.9265817479571,-5.07736076112986,
126.578908744281));
#252155=CARTESIAN_POINT('Ctrl Pts',(-70.2050293717699,-6.29942984483285,
132.792128074323));
#252156=CARTESIAN_POINT('Ctrl Pts',(-70.4834769955829,-1.73263064539088,
137.178686219444));
#252157=CARTESIAN_POINT('Ctrl Pts',(-70.7619246193956,4.42637147345276,
135.707550539556));
#252158=CARTESIAN_POINT('Ctrl Pts',(-71.0403722432087,6.51775444846118,
129.730622855503));
#252159=CARTESIAN_POINT('Ctrl Pts',(-71.3188198670216,2.6196394953401,124.740407719779));
#252160=CARTESIAN_POINT('Ctrl Pts',(-71.5972674908343,-3.68579617749442,
125.322669056552));
#252161=CARTESIAN_POINT('Ctrl Pts',(-71.8757151146474,-6.6041652243652,
130.942337142376));
#252162=CARTESIAN_POINT('Ctrl Pts',(-72.1541627384602,-3.45362906145158,
136.435211542427));
#252163=CARTESIAN_POINT('Ctrl Pts',(-72.4326103622731,2.87062348977667,
136.753609024891));
#252164=CARTESIAN_POINT('Ctrl Pts',(-72.711057986086,6.55691329165398,131.604937857965));
#252165=CARTESIAN_POINT('Ctrl Pts',(-72.9895056098989,4.21772010152317,
125.720575317484));
#252166=CARTESIAN_POINT('Ctrl Pts',(-73.2679532337117,-1.99735181482566,
124.50796311106));
#252167=CARTESIAN_POINT('Ctrl Pts',(-73.5464008575247,-6.37695498941029,
129.081432616995));
#252168=CARTESIAN_POINT('Ctrl Pts',(-73.8248484813376,-4.89644806029751,
135.238188785743));
#252169=CARTESIAN_POINT('Ctrl Pts',(-74.1032961051504,1.08365543144292,
137.320473472483));
#252170=CARTESIAN_POINT('Ctrl Pts',(-74.3817437289633,6.06793252119795,
133.414768775364));
#252171=CARTESIAN_POINT('Ctrl Pts',(-74.6601913527762,5.47607605895596,
127.110226506756));
#252172=CARTESIAN_POINT('Ctrl Pts',(-74.9386389765891,-0.148026780279403,
124.200413017498));
#252173=CARTESIAN_POINT('Ctrl Pts',(-75.217086600402,-5.63610023994771,
127.359304751927));
#252174=CARTESIAN_POINT('Ctrl Pts',(-75.4955342242149,-5.94487291790794,
133.684034526541));
#252175=CARTESIAN_POINT('Ctrl Pts',(-75.7739818480278,-0.790597807498519,
137.362484658699));
#252176=CARTESIAN_POINT('Ctrl Pts',(-76.0524294718406,5.09019806515201,
135.014339179226));
#252177=CARTESIAN_POINT('Ctrl Pts',(-76.3308770956536,6.29335058592772,
128.797429070474));
#252178=CARTESIAN_POINT('Ctrl Pts',(-76.6093247194664,1.71322136550425,
124.424791009442));
#252179=CARTESIAN_POINT('Ctrl Pts',(-76.8877723432794,-4.44127459430165,
125.914665758975));
#252180=CARTESIAN_POINT('Ctrl Pts',(-77.1662199670922,-6.51445617026952,
131.89793120868));
#252181=CARTESIAN_POINT('Ctrl Pts',(-77.4446675909052,-2.60117077463652,
136.876258709042));
#252182=CARTESIAN_POINT('Ctrl Pts',(-77.7231152147181,3.7024634886308,136.274808492052));
#252183=CARTESIAN_POINT('Ctrl Pts',(-78.0015628385308,6.60371468124315,
130.646283924643));
#252184=CARTESIAN_POINT('Ctrl Pts',(-78.2800104623438,3.43647469119047,
125.163024115555));
#252185=CARTESIAN_POINT('Ctrl Pts',(-78.5584580861567,-2.88871765894464,
124.863876957204));
#252186=CARTESIAN_POINT('Ctrl Pts',(-78.8369057099696,-6.55931960221255,
130.023744073965));
#252187=CARTESIAN_POINT('Ctrl Pts',(-79.1153533337825,-4.20222727162433,
135.900959659057));
#252188=CARTESIAN_POINT('Ctrl Pts',(-79.3938009575953,2.01650663137172,
137.094649707722));
#252189=CARTESIAN_POINT('Ctrl Pts',(-79.6722485814083,6.38216945196263,
132.507871380239));
#252190=CARTESIAN_POINT('Ctrl Pts',(-79.9506962052212,4.88293033251105,
126.355649882987));
#252191=CARTESIAN_POINT('Ctrl Pts',(-80.229143829034,-1.10348321810992,
124.29157621921));
#252192=CARTESIAN_POINT('Ctrl Pts',(-80.507591452847,-6.07584959944043,
128.212433250316));
#252193=CARTESIAN_POINT('Ctrl Pts',(-80.7860390766598,-5.46480702063872,
134.515144909234));
#252194=CARTESIAN_POINT('Ctrl Pts',(-81.0644867004727,0.168126239464741,
137.407827085998));
#252195=CARTESIAN_POINT('Ctrl Pts',(-81.3429343242857,5.64655969892388,
134.232246175545));
#252196=CARTESIAN_POINT('Ctrl Pts',(-81.6213819480984,5.93608064484842,
127.906605898828));
#252197=CARTESIAN_POINT('Ctrl Pts',(-81.8998295719115,0.770633471818905,
124.243860645443));
#252198=CARTESIAN_POINT('Ctrl Pts',(-82.1782771957242,-5.10298821427442,
126.609894368197));
#252199=CARTESIAN_POINT('Ctrl Pts',(-82.4567248195372,-6.28721302628274,
132.830437663053));
#252200=CARTESIAN_POINT('Ctrl Pts',(-82.7351724433501,-1.69379621456928,
137.189115132473));
#252201=CARTESIAN_POINT('Ctrl Pts',(-83.0136200671628,4.45613657178832,
135.680515115291));
#252202=CARTESIAN_POINT('Ctrl Pts',(-83.2920676909759,6.51109754304618,
129.690967328089));
#252203=CARTESIAN_POINT('Ctrl Pts',(-83.5705153147887,2.58267795704331,
124.724573581631));
#252204=CARTESIAN_POINT('Ctrl Pts',(-83.8489629386017,-3.71909650065006,
125.345207107088));
#252205=CARTESIAN_POINT('Ctrl Pts',(-84.1274105624144,-6.60320296221082,
130.982536014198));
#252206=CARTESIAN_POINT('Ctrl Pts',(-84.4058581862275,-3.41928848589759,
136.456130436155));
#252207=CARTESIAN_POINT('Ctrl Pts',(-84.6843058100402,2.90678506742617,
136.736024499134));
#252208=CARTESIAN_POINT('Ctrl Pts',(-84.9627534338533,6.56166514813073,
131.565009232842));
#252209=CARTESIAN_POINT('Ctrl Pts',(-85.241201057666,4.1866955128661,125.694995048862));
#252210=CARTESIAN_POINT('Ctrl Pts',(-85.519648681479,-2.03564276727566,
124.520238216135));
#252211=CARTESIAN_POINT('Ctrl Pts',(-85.7980963052919,-6.38732479096924,
129.120282873878));
#252212=CARTESIAN_POINT('Ctrl Pts',(-86.0765439291047,-4.8693673699251,
135.267912706297));
#252213=CARTESIAN_POINT('Ctrl Pts',(-86.3549915529177,1.12330078225909,
137.313756225814));
#252214=CARTESIAN_POINT('Ctrl Pts',(-86.6334391767305,6.08371039184151,
133.377783183006));
#252215=CARTESIAN_POINT('Ctrl Pts',(-86.9118868005434,5.45348735709659,
127.076960521238));
#252216=CARTESIAN_POINT('Ctrl Pts',(-87.1903344243564,-0.188224141151809,
124.201436454379));
#252217=CARTESIAN_POINT('Ctrl Pts',(-87.4687820481692,-5.65696684894189,
127.39367712271));
#252218=CARTESIAN_POINT('Ctrl Pts',(-87.7472296719821,-5.92723338074904,
133.720169301662));
#252219=CARTESIAN_POINT('Ctrl Pts',(-88.0256772957949,-0.750661997095914,
137.367175745102));
#252220=CARTESIAN_POINT('Ctrl Pts',(-88.3041249196079,5.11573109001074,
134.983275697681));
#252221=CARTESIAN_POINT('Ctrl Pts',(-88.5825725434208,6.28101722275544,
128.759156842984));
#252222=CARTESIAN_POINT('Ctrl Pts',(-88.8610201672337,1.67435537253749,
124.414480343369));
#252223=CARTESIAN_POINT('Ctrl Pts',(-89.1394677910466,-4.47095726823472,
125.941791652735));
#252224=CARTESIAN_POINT('Ctrl Pts',(-89.4179154148595,-6.50767859790483,
131.93756629108));
#252225=CARTESIAN_POINT('Ctrl Pts',(-89.6963630386723,-2.56416121387375,
136.891980275641));
#252226=CARTESIAN_POINT('Ctrl Pts',(-89.9748106624853,3.73569505946763,
136.252169191183));
#252227=CARTESIAN_POINT('Ctrl Pts',(-90.253258286298,6.60263007200808,130.606088167816));
#252228=CARTESIAN_POINT('Ctrl Pts',(-90.5317059101111,3.40207060478355,
125.142209839621));
#252229=CARTESIAN_POINT('Ctrl Pts',(-90.8101535339238,-2.9248255478482,
124.881571464914));
#252230=CARTESIAN_POINT('Ctrl Pts',(-91.0886011577368,-6.56394990767886,
130.063686977158));
#252231=CARTESIAN_POINT('Ctrl Pts',(-91.3670487815497,-4.17112496913288,
135.926445381018));
#252232=CARTESIAN_POINT('Ctrl Pts',(-91.6454964053626,2.05476004526333,
137.082258115016));
#252233=CARTESIAN_POINT('Ctrl Pts',(-91.9239440291755,6.39242095867105,
132.468989741201));
#252234=CARTESIAN_POINT('Ctrl Pts',(-92.2023916529884,4.85575929818535,
126.326008524418));
#252235=CARTESIAN_POINT('Ctrl Pts',(-92.4808392768012,-1.14310794030347,
124.298414101576));
#252236=CARTESIAN_POINT('Ctrl Pts',(-92.7592869006141,-6.09151482558059,
128.249466693771));
#252237=CARTESIAN_POINT('Ctrl Pts',(-93.0377345244271,-5.44211717319261,
134.548341988427));
#252238=CARTESIAN_POINT('Ctrl Pts',(-93.3161821482399,0.208320299155509,
137.406681306919));
#252239=CARTESIAN_POINT('Ctrl Pts',(-93.5946297720528,5.6673215935918,134.197810453193));
#252240=CARTESIAN_POINT('Ctrl Pts',(-93.8730773958657,5.91833120756931,
127.870524979765));
#252241=CARTESIAN_POINT('Ctrl Pts',(-94.1515250196785,0.730683568342929,
124.239291131637));
#252242=CARTESIAN_POINT('Ctrl Pts',(-94.4299726434915,-5.12842657431339,
126.641035419604));
#252243=CARTESIAN_POINT('Ctrl Pts',(-94.7084202673044,-6.27476323274215,
132.868672174754));
#252244=CARTESIAN_POINT('Ctrl Pts',(-94.9868678911172,-1.6548990195065,
137.199307456074));
#252245=CARTESIAN_POINT('Ctrl Pts',(-95.2653155149302,4.48573654634406,
135.653299003326));
#252246=CARTESIAN_POINT('Ctrl Pts',(-95.543763138743,6.50419936651746,129.651353057874));
#252247=CARTESIAN_POINT('Ctrl Pts',(-95.822210762556,2.54562071666526,124.708964732227));
#252248=CARTESIAN_POINT('Ctrl Pts',(-96.1006583863688,-3.75225901131679,
125.367947448562));
#252249=CARTESIAN_POINT('Ctrl Pts',(-96.3791060101818,-6.60199601594203,
131.022728283664));
#252250=CARTESIAN_POINT('Ctrl Pts',(-96.6575536339946,-3.38482120735248,
136.476839901474));
#252251=CARTESIAN_POINT('Ctrl Pts',(-96.9360012578075,2.94283893308538,
136.718220173391));
#252252=CARTESIAN_POINT('Ctrl Pts',(-97.2144488816204,6.5661738596919,131.525052421605));
#252253=CARTESIAN_POINT('Ctrl Pts',(-97.4928965054334,4.15551578466796,
125.669604109659));
#252254=CARTESIAN_POINT('Ctrl Pts',(-97.771344129246,-2.07385828823457,
124.532746181678));
#252255=CARTESIAN_POINT('Ctrl Pts',(-98.0497917530593,-6.39745790785863,
129.15919553488));
#252256=CARTESIAN_POINT('Ctrl Pts',(-98.3282393768718,-4.84210624335443,
135.297471228287));
#252257=CARTESIAN_POINT('Ctrl Pts',(-98.606687000685,1.16290450875192,137.306797771098));
#252258=CARTESIAN_POINT('Ctrl Pts',(-98.8851346244975,6.09926282835875,
133.340702231527));
#252259=CARTESIAN_POINT('Ctrl Pts',(-99.1635822483109,5.43069657425812,
127.043832655902));
#252260=CARTESIAN_POINT('Ctrl Pts',(-99.4420298721233,-0.228414527308866,
124.202704565042));
#252261=CARTESIAN_POINT('Ctrl Pts',(-99.7204774959365,-5.67762383694899,
127.428175877623));
#252262=CARTESIAN_POINT('Ctrl Pts',(-99.9989251197493,-5.90937420777732,
133.756196030418));
#252263=CARTESIAN_POINT('Ctrl Pts',(-100.277372743562,-0.710698370637635,
137.371623643978));
#252264=CARTESIAN_POINT('Ctrl Pts',(-100.555820367375,5.14107454957247,
134.9520573649));
#252265=CARTESIAN_POINT('Ctrl Pts',(-100.834267991188,6.26845111417983,
128.720960401273));
#252266=CARTESIAN_POINT('Ctrl Pts',(-101.112715615001,1.63542733571746,
124.404406456659));
#252267=CARTESIAN_POINT('Ctrl Pts',(-101.391163238814,-4.50047426920288,
125.969097730777));
#252268=CARTESIAN_POINT('Ctrl Pts',(-101.669610862627,-6.50065988111587,
131.977159382129));
#252269=CARTESIAN_POINT('Ctrl Pts',(-101.94805848644,-2.52705663717401,
136.907476263252));
#252270=CARTESIAN_POINT('Ctrl Pts',(-102.226506110253,3.76878820275105,
136.229328019765));
#252271=CARTESIAN_POINT('Ctrl Pts',(-102.504953734065,6.60130079988703,
130.565899758046));
#252272=CARTESIAN_POINT('Ctrl Pts',(-102.783401357878,3.36754045339959,
125.121605376767));
#252273=CARTESIAN_POINT('Ctrl Pts',(-103.061848981691,-2.96082505626518,
124.899485443752));
#252274=CARTESIAN_POINT('Ctrl Pts',(-103.340296605504,-6.56833698356739,
130.103657326284));
#252275=CARTESIAN_POINT('Ctrl Pts',(-103.618744229317,-4.13986810407194,
135.951741302244));
#252276=CARTESIAN_POINT('Ctrl Pts',(-103.89719185313,2.0929373192654,137.06963389251));
#252277=CARTESIAN_POINT('Ctrl Pts',(-104.175639476943,6.40243559186997,
132.430046418718));
#252278=CARTESIAN_POINT('Ctrl Pts',(-104.454087100755,4.82840833191319,
126.296533112833));
#252279=CARTESIAN_POINT('Ctrl Pts',(-104.732534724569,-1.18269030421136,
124.305493064181));
#252280=CARTESIAN_POINT('Ctrl Pts',(-105.010982348381,-6.10695432839948,
128.286594809759));
#252281=CARTESIAN_POINT('Ctrl Pts',(-105.289429972194,-5.41922566609253,
134.581400333014));
#252282=CARTESIAN_POINT('Ctrl Pts',(-105.567877596007,0.248506639461218,
137.40529087642));
#252283=CARTESIAN_POINT('Ctrl Pts',(-105.84632521982,5.68787348357469,134.163248985309));
#252284=CARTESIAN_POINT('Ctrl Pts',(-106.124772843633,5.90036246435008,
127.834552775061));
#252285=CARTESIAN_POINT('Ctrl Pts',(-106.403220467446,0.690706589119241,
124.234964888896));
#252286=CARTESIAN_POINT('Ctrl Pts',(-106.681668091259,-5.1536748986197,
126.672330744555));
#252287=CARTESIAN_POINT('Ctrl Pts',(-106.960115715072,-6.26208092554253,
132.906830192629));
#252288=CARTESIAN_POINT('Ctrl Pts',(-107.238563338885,-1.61594050155245,
137.209262812568));
#252289=CARTESIAN_POINT('Ctrl Pts',(-107.517010962697,4.51517030028232,
135.625903212168));
#252290=CARTESIAN_POINT('Ctrl Pts',(-107.79545858651,6.49706017448951,129.611781512777));
#252291=CARTESIAN_POINT('Ctrl Pts',(-108.073906210323,2.50846914737518,
124.69358174996));
#252292=CARTESIAN_POINT('Ctrl Pts',(-108.352353834136,-3.78528248064593,
125.390889238328));
#252293=CARTESIAN_POINT('Ctrl Pts',(-108.630801457949,-6.60054443028347,
131.062912461436));
#252294=CARTESIAN_POINT('Ctrl Pts',(-108.909249081762,-3.35022850301195,
136.497339170987));
#252295=CARTESIAN_POINT('Ctrl Pts',(-109.187696705575,2.97878375076591,
136.700196707408));
#252296=CARTESIAN_POINT('Ctrl Pts',(-109.466144329388,6.57043925926657,
131.485068904869));
#252297=CARTESIAN_POINT('Ctrl Pts',(-109.7445919532,4.12418207230337,125.644403440746));
#252298=CARTESIAN_POINT('Ctrl Pts',(-110.023039577014,-2.11199696161116,
124.5454865442));
#252299=CARTESIAN_POINT('Ctrl Pts',(-110.301487200826,-6.40735396459295,
129.198169158078));
#252300=CARTESIAN_POINT('Ctrl Pts',(-110.579934824639,-4.81466569075636,
135.326863256411));
#252301=CARTESIAN_POINT('Ctrl Pts',(-110.858382448452,1.20246514338981,
137.299598366182));
#252302=CARTESIAN_POINT('Ctrl Pts',(-111.136830072265,6.11458925444912,
133.303527294979));
#252303=CARTESIAN_POINT('Ctrl Pts',(-111.415277696078,5.407704554961,127.010844138312));
#252304=CARTESIAN_POINT('Ctrl Pts',(-111.693725319891,-0.268596449482207,
124.204217302498));
#252305=CARTESIAN_POINT('Ctrl Pts',(-111.972172943703,-5.69807043851701,
127.462799738304));
#252306=CARTESIAN_POINT('Ctrl Pts',(-112.250620567517,-5.89129606077132,
133.792113377828));
#252307=CARTESIAN_POINT('Ctrl Pts',(-112.529068191329,-0.670708408989202,
137.375828190507));
#252308=CARTESIAN_POINT('Ctrl Pts',(-112.807515815142,5.16622750472631,
134.920685337692));
#252309=CARTESIAN_POINT('Ctrl Pts',(-113.085963438955,6.25565272584325,
128.682841160722));
#252310=CARTESIAN_POINT('Ctrl Pts',(-113.364411062768,1.5964386975353,124.394569722605));
#252311=CARTESIAN_POINT('Ctrl Pts',(-113.642858686581,-4.52982450344111,
125.996582981263));
#252312=CARTESIAN_POINT('Ctrl Pts',(-113.921306310394,-6.49340027998504,
132.016709014688));
#252313=CARTESIAN_POINT('Ctrl Pts',(-114.199753934207,-2.48985841946147,
136.922746097669));
#252314=CARTESIAN_POINT('Ctrl Pts',(-114.47820155802,3.80174169220082,136.206285824184));
#252315=CARTESIAN_POINT('Ctrl Pts',(-114.756649181833,6.59972691413776,
130.525720184532));
#252316=CARTESIAN_POINT('Ctrl Pts',(-115.035096805645,3.3328855165654,125.101211490497));
#252317=CARTESIAN_POINT('Ctrl Pts',(-115.313544429458,-2.99671485022117,
124.917618229914));
#252318=CARTESIAN_POINT('Ctrl Pts',(-115.591992053271,-6.57248066731354,
130.143653640229));
#252319=CARTESIAN_POINT('Ctrl Pts',(-115.870439677084,-4.10845783467579,
135.976846485386));
#252320=CARTESIAN_POINT('Ctrl Pts',(-116.148887300897,2.13103703870585,
137.056777507999));
#252321=CARTESIAN_POINT('Ctrl Pts',(-116.42733492471,6.41221298046361,132.391042855849));
#252322=CARTESIAN_POINT('Ctrl Pts',(-116.705782548523,4.8008784471946,126.267224740454));
#252323=CARTESIAN_POINT('Ctrl Pts',(-116.984230172336,-1.22222884309565,
124.312812844714));
#252324=CARTESIAN_POINT('Ctrl Pts',(-117.262677796149,-6.12216753577917,
128.323816222486));
#252325=CARTESIAN_POINT('Ctrl Pts',(-117.541125419961,-5.39613334759327,
134.614318718005));
#252326=CARTESIAN_POINT('Ctrl Pts',(-117.819573043774,0.288683771261777,
137.403655846021));
#252327=CARTESIAN_POINT('Ctrl Pts',(-118.098020667587,5.70821460731317,
134.128563052582));
#252328=CARTESIAN_POINT('Ctrl Pts',(-118.3764682914,5.88217508103065,127.79869061768));
#252329=CARTESIAN_POINT('Ctrl Pts',(-118.654915915213,0.650704015508265,
124.230882077529));
#252330=CARTESIAN_POINT('Ctrl Pts',(-118.933363539026,-5.17873225160735,
126.703779183394));
#252331=CARTESIAN_POINT('Ctrl Pts',(-119.211811162839,-6.24916657463125,
132.944910302722));
#252332=CARTESIAN_POINT('Ctrl Pts',(-119.490258786652,-1.57692210432836,
137.218980833058));
#252333=CARTESIAN_POINT('Ctrl Pts',(-119.768706410464,4.54443674292479,
135.598328756974));
#252334=CARTESIAN_POINT('Ctrl Pts',(-120.047154034278,6.48968023150711,
129.572254159139));
#252335=CARTESIAN_POINT('Ctrl Pts',(-120.32560165809,2.47122462583917,124.67842520485));
#252336=CARTESIAN_POINT('Ctrl Pts',(-120.604049281903,-3.81816568494053,
125.414031626265));
#252337=CARTESIAN_POINT('Ctrl Pts',(-120.882496905716,-6.59884825902321,
131.103087058474));
#252338=CARTESIAN_POINT('Ctrl Pts',(-121.160944529529,-3.31551165472302,
136.517627485086));
#252339=CARTESIAN_POINT('Ctrl Pts',(-121.439392153342,3.0146181885189,136.68195476905));
#252340=CARTESIAN_POINT('Ctrl Pts',(-121.717839777155,6.57446118879764,
131.445060164237));
#252341=CARTESIAN_POINT('Ctrl Pts',(-121.996287400968,4.0926955368563,125.619393975946));
#252342=CARTESIAN_POINT('Ctrl Pts',(-122.274735024781,-2.15005737416446,
124.5584588316));
#252343=CARTESIAN_POINT('Ctrl Pts',(-122.553182648593,-6.41701259446945,
129.237202299292));
#252344=CARTESIAN_POINT('Ctrl Pts',(-122.831630272406,-4.7870467289504,
135.356087701536));
#252345=CARTESIAN_POINT('Ctrl Pts',(-123.110077896219,1.24198122024032,
137.292158277842));
#252346=CARTESIAN_POINT('Ctrl Pts',(-123.388525520032,6.1296891021858,133.266259750888));
#252347=CARTESIAN_POINT('Ctrl Pts',(-123.666973143845,5.38451215118288,
126.97799619087));
#252348=CARTESIAN_POINT('Ctrl Pts',(-123.945420767658,-0.30876841871475,
124.20597461069));
#252349=CARTESIAN_POINT('Ctrl Pts',(-124.223868391471,-5.71830589598935,
127.497547421752));
#252350=CARTESIAN_POINT('Ctrl Pts',(-124.502316015284,-5.87299960962311,
133.827920012961));
#252351=CARTESIAN_POINT('Ctrl Pts',(-124.780763639097,-0.630693593994696,
137.379789228888));
#252352=CARTESIAN_POINT('Ctrl Pts',(-125.059211262909,5.19118902341993,
134.889160778557));
#252353=CARTESIAN_POINT('Ctrl Pts',(-125.337658886723,6.24262253199412,
128.644800533857));
#252354=CARTESIAN_POINT('Ctrl Pts',(-125.616106510535,1.55739090273089,
124.384970505708));
#252355=CARTESIAN_POINT('Ctrl Pts',(-125.894554134348,-4.55900688336737,
126.024246385717));
#252356=CARTESIAN_POINT('Ctrl Pts',(-126.173001758161,-6.48590006351826,
132.056213723232));
#252357=CARTESIAN_POINT('Ctrl Pts',(-126.451449381974,-2.45256793912933,
136.937789213063));
#252358=CARTESIAN_POINT('Ctrl Pts',(-126.729897005787,3.83455430671493,
136.183043458277));
#252359=CARTESIAN_POINT('Ctrl Pts',(-127.0083446296,6.5979084730801,130.485550936142));
#252360=CARTESIAN_POINT('Ctrl Pts',(-127.286792253413,3.29810707843306,
125.081028936517));
#252361=CARTESIAN_POINT('Ctrl Pts',(-127.565239877225,-3.03249359980603,
124.935969151478));
#252362=CARTESIAN_POINT('Ctrl Pts',(-127.843687501038,-6.57638080537151,
130.183674436914));
#252363=CARTESIAN_POINT('Ctrl Pts',(-128.122135124851,-4.07689532486387,
136.001760000162));
#252364=CARTESIAN_POINT('Ctrl Pts',(-128.400582748664,2.1690577917847,137.043689437881));
#252365=CARTESIAN_POINT('Ctrl Pts',(-128.679030372477,6.42175276214748,
132.351980497887));
#252366=CARTESIAN_POINT('Ctrl Pts',(-128.95747799629,4.77317066415926,126.238084493312));
#252367=CARTESIAN_POINT('Ctrl Pts',(-129.235925620103,-1.26172209184052,
124.320373171937));
#252368=CARTESIAN_POINT('Ctrl Pts',(-129.514373243916,-6.13715388399014,
128.361129552696));
#252369=CARTESIAN_POINT('Ctrl Pts',(-129.792820867728,-5.37284107338758,
134.647095923599));
#252370=CARTESIAN_POINT('Ctrl Pts',(-130.071268491542,0.328850205779251,
137.401776276312));
#252371=CARTESIAN_POINT('Ctrl Pts',(-130.349716115354,5.72834421106097,
134.093753940311));
#252372=CARTESIAN_POINT('Ctrl Pts',(-130.628163739167,5.86376973154965,
127.762939836503));
#252373=CARTESIAN_POINT('Ctrl Pts',(-130.90661136298,0.610677329821333,
124.227042848828));
#252374=CARTESIAN_POINT('Ctrl Pts',(-131.185058986793,-5.20359770476699,
126.735379570785));
#252375=CARTESIAN_POINT('Ctrl Pts',(-131.463506610606,-6.23602065855449,
132.982911093959));
#252376=CARTESIAN_POINT('Ctrl Pts',(-131.741954234419,-1.53784527367628,
137.228461157434));
#252377=CARTESIAN_POINT('Ctrl Pts',(-132.020401858232,4.57353478979242,
135.57057665953));
#252378=CARTESIAN_POINT('Ctrl Pts',(-132.298849482045,6.48205981103755,
129.532772461657));
#252379=CARTESIAN_POINT('Ctrl Pts',(-132.577297105858,2.43388853216508,
124.66349565853));
#252380=CARTESIAN_POINT('Ctrl Pts',(-132.85574472967,-3.85090740570176,
125.437373754826));
#252381=CARTESIAN_POINT('Ctrl Pts',(-133.134192353483,-6.59690756501448,
131.143250586095));
#252382=CARTESIAN_POINT('Ctrl Pts',(-133.412639977296,-3.28067194892964,
136.53770409198));
#252383=CARTESIAN_POINT('Ctrl Pts',(-133.691087601109,3.0503409184865,136.663495034279));
#252384=CARTESIAN_POINT('Ctrl Pts',(-133.969535224922,6.5782394992522,131.405027682246));
#252385=CARTESIAN_POINT('Ctrl Pts',(-134.247982848735,4.06105734507014,
125.59457664199));
#252386=CARTESIAN_POINT('Ctrl Pts',(-134.526430472548,-2.18803811555026,
124.57166256319));
#252387=CARTESIAN_POINT('Ctrl Pts',(-134.804878096361,-6.42643343958478,
129.276293512134));
#252388=CARTESIAN_POINT('Ctrl Pts',(-135.083325720174,-4.75925038136761,
135.385143480741));
#252389=CARTESIAN_POINT('Ctrl Pts',(-135.361773343986,1.28145127501926,
137.284477781773));
#252390=CARTESIAN_POINT('Ctrl Pts',(-135.640220967799,6.14456181203885,
133.228900980221));
#252391=CARTESIAN_POINT('Ctrl Pts',(-135.918668591612,5.36112022232688,
126.945290030769));
#252392=CARTESIAN_POINT('Ctrl Pts',(-136.197116215425,-0.348928946420584,
124.207976424505));
#252393=CARTESIAN_POINT('Ctrl Pts',(-136.475563839238,-5.73832945953392,
127.53241764038));
#252394=CARTESIAN_POINT('Ctrl Pts',(-136.754011463051,-5.85448553231475,
133.863614608987));
#252395=CARTESIAN_POINT('Ctrl Pts',(-137.032459086864,-0.590655408416443,
137.383506612345));
#252396=CARTESIAN_POINT('Ctrl Pts',(-137.310906710677,5.21595818069537,
134.857484855651));
#252397=CARTESIAN_POINT('Ctrl Pts',(-137.58935433449,6.22936101547165,128.606839930282));
#252398=CARTESIAN_POINT('Ctrl Pts',(-137.867801958302,1.51828539823306,
124.375609161675));
#252399=CARTESIAN_POINT('Ctrl Pts',(-138.146249582115,-4.58802032761614,
126.052086919061));
#252400=CARTESIAN_POINT('Ctrl Pts',(-138.424697205928,-6.47815950964009,
132.095672043897));
#252401=CARTESIAN_POINT('Ctrl Pts',(-138.703144829741,-2.41518657799051,
136.952605052004));
#252402=CARTESIAN_POINT('Ctrl Pts',(-138.981592453554,3.86722483040823,
136.159601783301));
#252403=CARTESIAN_POINT('Ctrl Pts',(-139.260040077367,6.59584554409815,
130.445393501362));
#252404=CARTESIAN_POINT('Ctrl Pts',(-139.53848770118,3.26320642772972,125.061058462695));
#252405=CARTESIAN_POINT('Ctrl Pts',(-139.816935324993,-3.06815997922566,
124.954537528447));
#252406=CARTESIAN_POINT('Ctrl Pts',(-140.095382948806,-6.58003725322031,
130.223718233352));
#252407=CARTESIAN_POINT('Ctrl Pts',(-140.373830572619,-4.04518174419624,
136.026480923393));
#252408=CARTESIAN_POINT('Ctrl Pts',(-140.652278196431,2.20699816962987,
137.030370167137));
#252409=CARTESIAN_POINT('Ctrl Pts',(-140.930725820244,6.43105458342049,
132.312860792301));
#252410=CARTESIAN_POINT('Ctrl Pts',(-141.209173444057,4.74528600953044,
126.209113451214));
#252411=CARTESIAN_POINT('Ctrl Pts',(-141.48762106787,-1.30116858700904,
124.328173765698));
#252412=CARTESIAN_POINT('Ctrl Pts',(-141.766068691683,-6.15191281770628,
128.398533417733));
#252413=CARTESIAN_POINT('Ctrl Pts',(-142.044516315496,-5.34934970658085,
134.679730735221));
#252414=CARTESIAN_POINT('Ctrl Pts',(-142.322963939309,0.369004454631186,
137.399652236939));
#252415=CARTESIAN_POINT('Ctrl Pts',(-142.601411563122,5.74826154890666,
134.058822938361));
#252416=CARTESIAN_POINT('Ctrl Pts',(-142.879859186934,5.84514709792562,
127.727301756295));
#252417=CARTESIAN_POINT('Ctrl Pts',(-143.158306810748,0.570628015260733,
124.223447345055));
#252418=CARTESIAN_POINT('Ctrl Pts',(-143.43675443456,-5.22827033670001,
126.767130735766));
#252419=CARTESIAN_POINT('Ctrl Pts',(-143.715202058373,-6.22264366443886,
133.020831158207));
#252420=CARTESIAN_POINT('Ctrl Pts',(-143.993649682186,-1.49871145760156,
137.237703434405));
#252421=CARTESIAN_POINT('Ctrl Pts',(-144.272097305999,4.60246336264661,
135.542647948195));
#252422=CARTESIAN_POINT('Ctrl Pts',(-144.550544929812,6.47419919545755,
129.493337883343));
#252423=CARTESIAN_POINT('Ctrl Pts',(-144.828992553625,2.39646224985712,
124.648793664219));
#252424=CARTESIAN_POINT('Ctrl Pts',(-145.107440177438,-3.8835064296727,
125.460914759058));
#252425=CARTESIAN_POINT('Ctrl Pts',(-145.38588780125,-6.59472242016944,
131.183401556022));
#252426=CARTESIAN_POINT('Ctrl Pts',(-145.664335425064,-3.24571067663155,
136.557568247724));
#252427=CARTESIAN_POINT('Ctrl Pts',(-145.942783048876,3.08595061694992,
136.644818187128));
#252428=CARTESIAN_POINT('Ctrl Pts',(-146.221230672689,6.58177405062243,
131.364972942318));
#252429=CARTESIAN_POINT('Ctrl Pts',(-146.499678296502,4.02926866931097,
125.569952358496));
#252430=CARTESIAN_POINT('Ctrl Pts',(-146.778125920315,-2.22593777837984,
124.585097249699));
#252431=CARTESIAN_POINT('Ctrl Pts',(-147.056573544128,-6.43561615084533,
129.315441348065));
#252432=CARTESIAN_POINT('Ctrl Pts',(-147.335021167941,-4.73127767801157,
135.414029517352));
#252433=CARTESIAN_POINT('Ctrl Pts',(-147.613468791753,1.32087384515067,
137.276557162581));
#252434=CARTESIAN_POINT('Ctrl Pts',(-147.891916415567,6.15920683289404,
133.191452367319));
#252435=CARTESIAN_POINT('Ctrl Pts',(-148.170364039379,5.33752963518947,
126.91272686995));
#252436=CARTESIAN_POINT('Ctrl Pts',(-148.448811663193,-0.389076544435395,
124.210222669761));
#252437=CARTESIAN_POINT('Ctrl Pts',(-148.727259287005,-5.75814038716998,
127.567409102056));
#252438=CARTESIAN_POINT('Ctrl Pts',(-149.005706910818,-5.83575451489182,
133.899195843233));
#252439=CARTESIAN_POINT('Ctrl Pts',(-149.284154534631,-0.550595335885521,
137.386980203127));
#252440=CARTESIAN_POINT('Ctrl Pts',(-149.562602158444,5.24053405872261,
134.825658742734));
#252441=CARTESIAN_POINT('Ctrl Pts',(-149.841049782257,6.21586866768539,
128.568960756646));
#252442=CARTESIAN_POINT('Ctrl Pts',(-150.119497406069,1.47912363311174,
124.366486037389));
#252443=CARTESIAN_POINT('Ctrl Pts',(-150.397945029883,-4.61686376108527,
126.080103549656));
#252444=CARTESIAN_POINT('Ctrl Pts',(-150.676392653695,-6.4701789051783,
132.135082514543));
#252445=CARTESIAN_POINT('Ctrl Pts',(-150.954840277509,-2.37771572122463,
136.967193065487));
#252446=CARTESIAN_POINT('Ctrl Pts',(-151.233287901321,3.89975205266408,
136.135961667893));
#252447=CARTESIAN_POINT('Ctrl Pts',(-151.511735525134,6.59353820363339,
130.405249368239));
#252448=CARTESIAN_POINT('Ctrl Pts',(-151.790183148947,3.22818485771248,
125.041300809049));
#252449=CARTESIAN_POINT('Ctrl Pts',(-152.06863077276,-3.10371266684865,
124.97332267276));
#252450=CARTESIAN_POINT('Ctrl Pts',(-152.347078396573,-6.58344987536885,
130.263783545709));
#252451=CARTESIAN_POINT('Ctrl Pts',(-152.625526020386,-4.01331826783166,
136.051008339035));
#252452=CARTESIAN_POINT('Ctrl Pts',(-152.903973644199,2.24485676634579,
137.016820189321));
#252453=CARTESIAN_POINT('Ctrl Pts',(-153.182421268012,6.44011809960154,
132.273685188686));
#252454=CARTESIAN_POINT('Ctrl Pts',(-153.460868891824,4.71722551658265,
126.180312687687));
#252455=CARTESIAN_POINT('Ctrl Pts',(-153.739316515637,-1.34056686689732,
124.336214336947));
#252456=CARTESIAN_POINT('Ctrl Pts',(-154.01776413945,-6.16644379003131,
128.436026431582));
#252457=CARTESIAN_POINT('Ctrl Pts',(-154.296211763263,-5.32566011765276,
134.712221943579));
#252458=CARTESIAN_POINT('Ctrl Pts',(-154.574659387076,0.409145029887599,
137.397283806609));
#252459=CARTESIAN_POINT('Ctrl Pts',(-154.853107010889,5.7679658828075,134.023771341112));
#252460=CARTESIAN_POINT('Ctrl Pts',(-155.131554634702,5.82630787022557,
127.691777697632));
#252461=CARTESIAN_POINT('Ctrl Pts',(-155.410002258515,0.530557555869813,
124.220095699443));
#252462=CARTESIAN_POINT('Ctrl Pts',(-155.688449882327,-5.25274923315307,
126.799031501784));
#252463=CARTESIAN_POINT('Ctrl Pts',(-155.96689750614,-6.20903608797397,
133.058669090323));
#252464=CARTESIAN_POINT('Ctrl Pts',(-156.245345129953,-1.4595221062231,
137.246707321489));
#252465=CARTESIAN_POINT('Ctrl Pts',(-156.523792753766,4.63122138952822,
135.514543657883));
#252466=CARTESIAN_POINT('Ctrl Pts',(-156.802240377579,6.46609867604585,
129.453951885458));
#252467=CARTESIAN_POINT('Ctrl Pts',(-157.080688001392,2.35894716575843,
124.634319766706));
#252468=CARTESIAN_POINT('Ctrl Pts',(-157.359135625205,-3.9159615488849,
125.484653766641));
#252469=CARTESIAN_POINT('Ctrl Pts',(-157.637583249018,-6.59229290546042,
131.223538480449));
#252470=CARTESIAN_POINT('Ctrl Pts',(-157.916030872831,-3.21062913332988,
136.577219216243));
#252471=CARTESIAN_POINT('Ctrl Pts',(-158.194478496644,3.12144596437753,
136.625924919674));
#252472=CARTESIAN_POINT('Ctrl Pts',(-158.472926120456,6.58506471193526,
131.324897428694));
#252473=CARTESIAN_POINT('Ctrl Pts',(-158.751373744269,3.99733068751967,
125.545522037924));
#252474=CARTESIAN_POINT('Ctrl Pts',(-159.029821368082,-2.26375495826568,
124.598762393297));
#252475=CARTESIAN_POINT('Ctrl Pts',(-159.308268991895,-6.44456038798308,
129.354644356446));
#252476=CARTESIAN_POINT('Ctrl Pts',(-159.586716615708,-4.7031296554214,
135.442744740987));
#252477=CARTESIAN_POINT('Ctrl Pts',(-159.865164239521,1.36024746981527,
137.268396713766));
#252478=CARTESIAN_POINT('Ctrl Pts',(-160.143611863334,6.17362362207528,
133.153915299856));
#252479=CARTESIAN_POINT('Ctrl Pts',(-160.422059487147,5.31374126392856,
126.880307915048));
#252480=CARTESIAN_POINT('Ctrl Pts',(-160.70050711096,-0.429209725076344,
124.212713263223));
#252481=CARTESIAN_POINT('Ctrl Pts',(-160.978954734773,-5.77773794479658,
127.602520510164));
#252482=CARTESIAN_POINT('Ctrl Pts',(-161.257402358585,-5.81680725143943,
133.934662397221));
#252483=CARTESIAN_POINT('Ctrl Pts',(-161.535849982398,-0.51051486084124,
137.390209872519));
#252484=CARTESIAN_POINT('Ctrl Pts',(-161.814297606211,5.26491574683228,
134.793683619137));
#252485=CARTESIAN_POINT('Ctrl Pts',(-162.092745230024,6.20214598860049,
128.531164416574));
#252486=CARTESIAN_POINT('Ctrl Pts',(-162.371192853837,1.43990705852047,
124.357601470914));
#252487=CARTESIAN_POINT('Ctrl Pts',(-162.64964047765,-4.64553611496906,
126.108295239334));
#252488=CARTESIAN_POINT('Ctrl Pts',(-162.928088101462,-6.46195854585841,
132.1744436748));
#252489=CARTESIAN_POINT('Ctrl Pts',(-163.206535725276,-2.34015675732853,
136.981552712947));
#252490=CARTESIAN_POINT('Ctrl Pts',(-163.484983349088,3.93213476817268,
136.112123988049));
#252491=CARTESIAN_POINT('Ctrl Pts',(-163.763430972902,6.5909865371863,130.365120024332));
#252492=CARTESIAN_POINT('Ctrl Pts',(-164.041878596714,3.19304366611785,
125.021756707701));
#252493=CARTESIAN_POINT('Ctrl Pts',(-164.320326220527,-3.13915034525769,
124.99232388833));
#252494=CARTESIAN_POINT('Ctrl Pts',(-164.59877384434,-6.58661854536123,
130.303868889347));
#252495=CARTESIAN_POINT('Ctrl Pts',(-164.877221468153,-3.98130607648258,
136.075341338217));
#252496=CARTESIAN_POINT('Ctrl Pts',(-165.155669091966,2.28263217906914,
137.003040006531));
#252497=CARTESIAN_POINT('Ctrl Pts',(-165.434116715779,6.44894297483741,
132.23445513871));
#252498=CARTESIAN_POINT('Ctrl Pts',(-165.712564339591,4.6889902251094,126.151683269957));
#252499=CARTESIAN_POINT('Ctrl Pts',(-165.991011963405,-1.37991547158711,
124.344494587733));
#252500=CARTESIAN_POINT('Ctrl Pts',(-166.269459587217,-6.18074626251326,
128.473607204924));
#252501=CARTESIAN_POINT('Ctrl Pts',(-166.54790721103,-5.3017731844313,134.744568344699));
#252502=CARTESIAN_POINT('Ctrl Pts',(-166.826354834843,0.449270444124704,
137.394671073086));
#252503=CARTESIAN_POINT('Ctrl Pts',(-167.104802458656,5.78745648261092,
133.988600447415));
#252504=CARTESIAN_POINT('Ctrl Pts',(-167.383250082469,5.8072527465451,127.656368976875));
#252505=CARTESIAN_POINT('Ctrl Pts',(-167.661697706282,0.490467436472931,
124.216988036188));
#252506=CARTESIAN_POINT('Ctrl Pts',(-167.940145330095,-5.27703348705155,
126.831080686747));
#252507=CARTESIAN_POINT('Ctrl Pts',(-168.218592953908,-6.19519843339338,
133.096423488211));
#252508=CARTESIAN_POINT('Ctrl Pts',(-168.49704057772,-1.42027867171577,
137.255472485049));
#252509=CARTESIAN_POINT('Ctrl Pts',(-168.775488201534,4.65980780479824,
135.486264830004));
#252510=CARTESIAN_POINT('Ctrl Pts',(-169.053935825346,6.45775855296945,
129.414615927465));
#252511=CARTESIAN_POINT('Ctrl Pts',(-169.332383449159,2.32134467000579,
124.620074502325));
#252512=CARTESIAN_POINT('Ctrl Pts',(-169.610831072972,-3.94827156070164,
125.508589897919));
#252513=CARTESIAN_POINT('Ctrl Pts',(-169.889278696785,-6.58961911091297,
131.263659872085));
#252514=CARTESIAN_POINT('Ctrl Pts',(-170.167726320598,-3.17542861898582,
136.596656269364));
#252515=CARTESIAN_POINT('Ctrl Pts',(-170.446173944411,3.15682564547787,
136.606815932013));
#252516=CARTESIAN_POINT('Ctrl Pts',(-170.724621568223,6.58811136125304,
131.284802626386));
#252517=CARTESIAN_POINT('Ctrl Pts',(-171.003069192037,3.96524458316956,
125.521286585549));
#252518=CARTESIAN_POINT('Ctrl Pts',(-171.28151681585,-2.30148825387982,
124.612657487621));
#252519=CARTESIAN_POINT('Ctrl Pts',(-171.559964439662,-6.45326581956532,
129.393901084596));
#252520=CARTESIAN_POINT('Ctrl Pts',(-171.838412063475,-4.67480735663214,
135.471288087592));
#252521=CARTESIAN_POINT('Ctrl Pts',(-172.116859687288,1.39957069001038,
137.259996737715));
#252522=CARTESIAN_POINT('Ctrl Pts',(-172.395307311101,6.18781164536257,
133.116291168777));
#252523=CARTESIAN_POINT('Ctrl Pts',(-172.673754934914,5.289755990031,126.848034367363));
#252524=CARTESIAN_POINT('Ctrl Pts',(-172.952202558727,-0.469327001192524,
124.215448112602));
#252525=CARTESIAN_POINT('Ctrl Pts',(-173.23065018254,-5.79712140621875,
127.637750563632));
#252526=CARTESIAN_POINT('Ctrl Pts',(-173.509097806352,-5.79764444405506,
133.970012956726));
#252527=CARTESIAN_POINT('Ctrl Pts',(-173.787545430165,-0.470415468481743,
137.393195500846));
#252528=CARTESIAN_POINT('Ctrl Pts',(-174.065993053978,5.28910234155359,
134.76156066971));
#252529=CARTESIAN_POINT('Ctrl Pts',(-174.344440677791,6.18819348671444,
128.493452310623));
#252530=CARTESIAN_POINT('Ctrl Pts',(-174.622888301604,1.40063712764339,
124.34895579147));
#252531=CARTESIAN_POINT('Ctrl Pts',(-174.901335925417,-4.67403632680454,
126.13666094344));
#252532=CARTESIAN_POINT('Ctrl Pts',(-175.17978354923,-6.45349873628761,
132.213754066126));
#252533=CARTESIAN_POINT('Ctrl Pts',(-175.458231173043,-2.30251107806296,
136.995683462282));
#252534=CARTESIAN_POINT('Ctrl Pts',(-175.736678796856,3.96437177698222,
136.088089627079));
#252535=CARTESIAN_POINT('Ctrl Pts',(-176.015126420669,6.58819063930867,
130.325006956645));
#252536=CARTESIAN_POINT('Ctrl Pts',(-176.293574044481,3.15778415511627,
125.002426882869));
#252537=CARTESIAN_POINT('Ctrl Pts',(-176.572021668294,-3.17447170129595,
125.011540471058));
#252538=CARTESIAN_POINT('Ctrl Pts',(-176.850469292107,-6.58954314578118,
130.343972778891));
#252539=CARTESIAN_POINT('Ctrl Pts',(-177.12891691592,-3.94914635637289,
136.099479019269));
#252540=CARTESIAN_POINT('Ctrl Pts',(-177.407364539733,2.32032300801719,
136.989030129397));
#252541=CARTESIAN_POINT('Ctrl Pts',(-177.685812163546,6.45752888212044,
132.195172096054));
#252542=CARTESIAN_POINT('Ctrl Pts',(-177.964259787359,4.66058118137817,
126.123226258898));
#252543=CARTESIAN_POINT('Ctrl Pts',(-178.242707411172,-1.41921294300185,
124.353014211231));
#252544=CARTESIAN_POINT('Ctrl Pts',(-178.521155034985,-6.19481970517025,
128.511274345191));
#252545=CARTESIAN_POINT('Ctrl Pts',(-178.799602658797,-5.27768979205393,
134.776768739972));
#252546=CARTESIAN_POINT('Ctrl Pts',(-179.078050282611,0.489379210479558,
137.391814133187));
#252547=CARTESIAN_POINT('Ctrl Pts',(-179.356497906423,5.80673262608622,
133.95331156054));
#252548=CARTESIAN_POINT('Ctrl Pts',(-179.634945530236,5.7879824329786,127.621076906106));
#252549=CARTESIAN_POINT('Ctrl Pts',(-179.913393154049,0.450359142625426,
124.214124470449));
#252550=CARTESIAN_POINT('Ctrl Pts',(-180.191840777862,-5.30112219853358,
126.863277103057));
#252551=CARTESIAN_POINT('Ctrl Pts',(-180.470288401675,-6.18113121345664,
133.134092952866));
#252552=CARTESIAN_POINT('Ctrl Pts',(-180.748736025488,-1.38098260826046,
137.263998600285));
#252553=CARTESIAN_POINT('Ctrl Pts',(-181.0271836493,4.68822154917632,135.457812512445));
#252554=CARTESIAN_POINT('Ctrl Pts',(-181.305631273113,6.44917913527537,
129.375331466973));
#252555=CARTESIAN_POINT('Ctrl Pts',(-181.584078896926,2.28365615597197,
124.606058398942));
#252556=CARTESIAN_POINT('Ctrl Pts',(-181.862526520739,-3.98043526786393,
125.532722265928));
#252557=CARTESIAN_POINT('Ctrl Pts',(-182.140974144552,-6.58670113560653,
131.303764244219));
#252558=CARTESIAN_POINT('Ctrl Pts',(-182.419421768365,-3.14011043796568,
136.615878686839));
#252559=CARTESIAN_POINT('Ctrl Pts',(-182.697869392178,3.19208834924215,
136.587491932238));
#252560=CARTESIAN_POINT('Ctrl Pts',(-182.976317015991,6.59091388568205,
131.244690021124));
#252561=CARTESIAN_POINT('Ctrl Pts',(-183.254764639804,3.93301154522339,
125.497246899427));
#252562=CARTESIAN_POINT('Ctrl Pts',(-183.533212263617,-2.33913626699958,
124.626782017781));
#252563=CARTESIAN_POINT('Ctrl Pts',(-183.811659887429,-6.46173212300977,
129.433210077844));
#252564=CARTESIAN_POINT('Ctrl Pts',(-184.090107511242,-4.64631183113728,
135.499658499484));
#252565=CARTESIAN_POINT('Ctrl Pts',(-184.368555135055,1.43884204859816,
137.251357545694));
#252566=CARTESIAN_POINT('Ctrl Pts',(-184.647002758868,6.20177037701405,
133.078581368264));
#252567=CARTESIAN_POINT('Ctrl Pts',(-184.925450382681,5.26557470227994,
126.815907422802));
#252568=CARTESIAN_POINT('Ctrl Pts',(-185.203898006494,-0.50942688622466,
124.218427116558));
#252569=CARTESIAN_POINT('Ctrl Pts',(-185.482345630307,-5.81629005317544,
127.673097957001));
#252570=CARTESIAN_POINT('Ctrl Pts',(-185.76079325412,-5.77826680282389,
134.005246211819));
#252571=CARTESIAN_POINT('Ctrl Pts',(-186.039240877932,-0.430298644703365,
137.395936977472));
#252572=CARTESIAN_POINT('Ctrl Pts',(-186.317688501746,5.31309294664177,
134.729291084778));
#252573=CARTESIAN_POINT('Ctrl Pts',(-186.596136125558,6.17401167904375,
128.455825836229));
#252574=CARTESIAN_POINT('Ctrl Pts',(-186.874583749371,1.36131529564269,
124.340549319425));
#252575=CARTESIAN_POINT('Ctrl Pts',(-187.153031373184,-4.70236334050424,
126.165199610876));
#252576=CARTESIAN_POINT('Ctrl Pts',(-187.431478996997,-6.44479978994851,
132.253012231859));
#252577=CARTESIAN_POINT('Ctrl Pts',(-187.70992662081,-2.26478007840253,
137.009584789872));
#252578=CARTESIAN_POINT('Ctrl Pts',(-187.988374244623,3.99646188453734,
136.063859475589));
#252579=CARTESIAN_POINT('Ctrl Pts',(-188.266821868436,6.58515061360439,
130.284911651585));
#252580=CARTESIAN_POINT('Ctrl Pts',(-188.545269492249,3.12240763126122,
124.983312050825));
#252581=CARTESIAN_POINT('Ctrl Pts',(-188.823717116061,-3.20967542611822,
125.030971708867));
#252582=CARTESIAN_POINT('Ctrl Pts',(-189.102164739874,-6.59222356825658,
130.384093728275));
#252583=CARTESIAN_POINT('Ctrl Pts',(-189.380612363687,-3.91684029919248,
136.123420487763));
#252584=CARTESIAN_POINT('Ctrl Pts',(-189.6590599875,2.35792785654334,136.974791077059));
#252585=CARTESIAN_POINT('Ctrl Pts',(-189.937507611313,6.46587550329532,
132.155837516369));
#252586=CARTESIAN_POINT('Ctrl Pts',(-190.215955235126,4.63199943809816,
126.094942708994));
#252587=CARTESIAN_POINT('Ctrl Pts',(-190.494402858939,-1.45845782495887,
124.361772891742));
#252588=CARTESIAN_POINT('Ctrl Pts',(-190.772850482752,-6.2086635965042,
128.549026456613));
#252589=CARTESIAN_POINT('Ctrl Pts',(-191.051298106565,-5.25341083294129,
134.808821936201));
#252590=CARTESIAN_POINT('Ctrl Pts',(-191.329745730377,0.529469842708527,
137.388713092773));
#252591=CARTESIAN_POINT('Ctrl Pts',(-191.60819335419,5.82579359894846,133.91790598813));
#252592=CARTESIAN_POINT('Ctrl Pts',(-191.886640978003,5.76849764359442,
127.585902793086));
#252593=CARTESIAN_POINT('Ctrl Pts',(-192.165088601816,0.410234160553658,
124.211505108333));
#252594=CARTESIAN_POINT('Ctrl Pts',(-192.443536225629,-5.32501447498302,
126.895619557667));
#252595=CARTESIAN_POINT('Ctrl Pts',(-192.721983849442,-6.16683494942961,
133.171676088433));
#252596=CARTESIAN_POINT('Ctrl Pts',(-193.000431473255,-1.34163537198624,
137.272285351261));
#252597=CARTESIAN_POINT('Ctrl Pts',(-193.278879097068,4.71646156978089,
135.429187759513));
#252598=CARTESIAN_POINT('Ctrl Pts',(-193.557326720881,6.44036074087642,
129.336099959682));
#252599=CARTESIAN_POINT('Ctrl Pts',(-193.835774344694,2.24588302022023,
124.592271975924));
#252600=CARTESIAN_POINT('Ctrl Pts',(-194.114221968506,-4.01245147853337,
125.557049976435));
#252601=CARTESIAN_POINT('Ctrl Pts',(-194.392669592319,-6.58353908766677,
131.343850110767));
#252602=CARTESIAN_POINT('Ctrl Pts',(-194.671117216133,-3.10467589899933,
136.634885756375));
#252603=CARTESIAN_POINT('Ctrl Pts',(-194.949564839945,3.22723276899961,
136.567953636405));
#252604=CARTESIAN_POINT('Ctrl Pts',(-195.228012463758,6.59347218137276,
131.204561099293));
#252605=CARTESIAN_POINT('Ctrl Pts',(-195.506460087571,3.90063276808784,
125.473403870355));
#252606=CARTESIAN_POINT('Ctrl Pts',(-195.784907711384,-2.3766976025655,
124.641135460387));
#252607=CARTESIAN_POINT('Ctrl Pts',(-196.063355335197,-6.46995898459376,
129.472569879579));
#252608=CARTESIAN_POINT('Ctrl Pts',(-196.34180295901,-4.61764413484867,
135.527854925386));
#252609=CARTESIAN_POINT('Ctrl Pts',(-196.620250582823,1.47806009036541,
137.242479457832));
#252610=CARTESIAN_POINT('Ctrl Pts',(-196.898698206635,6.21549929978325,
133.040787295662));
#252611=CARTESIAN_POINT('Ctrl Pts',(-197.177145830448,5.24119829672186,
126.783928271841));
#252612=CARTESIAN_POINT('Ctrl Pts',(-197.455593454261,-0.5495078942556,
124.2216501647));
#252613=CARTESIAN_POINT('Ctrl Pts',(-197.734041078074,-5.83524317536515,
127.708561380459));
#252614=CARTESIAN_POINT('Ctrl Pts',(-198.012488701887,-5.75867504579123,
134.040360856918));
#252615=CARTESIAN_POINT('Ctrl Pts',(-198.2909363257,-0.390165876051177,
137.398434200813));
#252616=CARTESIAN_POINT('Ctrl Pts',(-198.569383949513,5.33688667311775,
134.696876060105));
#252617=CARTESIAN_POINT('Ctrl Pts',(-198.847831573325,6.15960109109908,
128.418286387655));
#252618=CARTESIAN_POINT('Ctrl Pts',(-199.126279197139,1.32194301960288,
124.332382366286));
#252619=CARTESIAN_POINT('Ctrl Pts',(-199.404726820951,-4.73051610640191,
126.193910184127));
#252620=CARTESIAN_POINT('Ctrl Pts',(-199.683174444764,-6.43586202918244,
132.292216717274));
#252621=CARTESIAN_POINT('Ctrl Pts',(-199.961622068577,-2.22696515648391,
137.023256180599));
#252622=CARTESIAN_POINT('Ctrl Pts',(-200.24006969239,4.02840390172748,136.039434431435));
#252623=CARTESIAN_POINT('Ctrl Pts',(-200.518517316203,6.58186657272242,
130.244835594899));
#252624=CARTESIAN_POINT('Ctrl Pts',(-200.796964940016,3.08691540544346,
124.964412919876));
#252625=CARTESIAN_POINT('Ctrl Pts',(-201.075412563829,-3.24476021523692,
125.050616881724));
#252626=CARTESIAN_POINT('Ctrl Pts',(-201.353860187642,-6.59465971346335,
130.424230250803));
#252627=CARTESIAN_POINT('Ctrl Pts',(-201.632307811455,-3.88438910205457,
136.147164856536));
#252628=CARTESIAN_POINT('Ctrl Pts',(-201.910755435267,2.39544533118521,
136.960323377152));
#252629=CARTESIAN_POINT('Ctrl Pts',(-202.18920305908,6.47398252907625,132.116452857208));
#252630=CARTESIAN_POINT('Ctrl Pts',(-202.467650682893,4.60324605437475,
126.066833668302));
#252631=CARTESIAN_POINT('Ctrl Pts',(-202.746098306706,-1.49764866322506,
124.370770304711));
#252632=CARTESIAN_POINT('Ctrl Pts',(-203.024545930519,-6.22227742352606,
128.586862140274));
#252633=CARTESIAN_POINT('Ctrl Pts',(-203.302993554332,-5.22893720675747,
134.840726745644));
#252634=CARTESIAN_POINT('Ctrl Pts',(-203.581441178145,0.569540855237039,
137.385368066758));
#252635=CARTESIAN_POINT('Ctrl Pts',(-203.859888801958,5.84463869488665,
133.882385042152));
#252636=CARTESIAN_POINT('Ctrl Pts',(-204.138336425771,5.7487991004088,127.550847941203));
#252637=CARTESIAN_POINT('Ctrl Pts',(-204.416784049583,0.370093977104817,
124.209130046901));
#252638=CARTESIAN_POINT('Ctrl Pts',(-204.695231673396,-5.34870943106288,
126.928106852114));
#252639=CARTESIAN_POINT('Ctrl Pts',(-204.973679297209,-6.15231017106575,
133.209171502253));
#252640=CARTESIAN_POINT('Ctrl Pts',(-205.252126921022,-1.30223842092043,
137.280332430907));
#252641=CARTESIAN_POINT('Ctrl Pts',(-205.530574544835,4.74452682016742,
135.400391631911));
#252642=CARTESIAN_POINT('Ctrl Pts',(-205.809022168648,6.43130369654214,
129.296922859329));
#252643=CARTESIAN_POINT('Ctrl Pts',(-206.087469792461,2.20802666244648,
124.578715744137));
#252644=CARTESIAN_POINT('Ctrl Pts',(-206.365917416273,-4.04431900633787,
125.581572127967));
#252645=CARTESIAN_POINT('Ctrl Pts',(-206.644365040087,-6.58013308426553,
131.383915986335));
#252646=CARTESIAN_POINT('Ctrl Pts',(-206.922812663899,-3.06912631512495,
136.653676773657));
#252647=CARTESIAN_POINT('Ctrl Pts',(-207.201260287713,3.26225760245914,
136.548201768512));
#252648=CARTESIAN_POINT('Ctrl Pts',(-207.479707911525,6.59578615352751,
131.164417347887));
#252649=CARTESIAN_POINT('Ctrl Pts',(-207.758155535338,3.86810945157081,
125.449758381845));
#252650=CARTESIAN_POINT('Ctrl Pts',(-208.036603159151,-2.41417086872696,
124.655717283569));
#252651=CARTESIAN_POINT('Ctrl Pts',(-208.315050782964,-6.47794609946865,
129.511979031309));
#252652=CARTESIAN_POINT('Ctrl Pts',(-208.593498406777,-4.58880533005852,
135.555876320469));
#252653=CARTESIAN_POINT('Ctrl Pts',(-208.87194603059,1.51722336207232,137.233362803106));
#252654=CARTESIAN_POINT('Ctrl Pts',(-209.150393654402,6.22899790494034,
133.00291035145));
#252655=CARTESIAN_POINT('Ctrl Pts',(-209.428841278216,5.21662767663345,
126.752098099478));
#252656=CARTESIAN_POINT('Ctrl Pts',(-209.707288902028,-0.589568540070009,
124.225117137599));
#252657=CARTESIAN_POINT('Ctrl Pts',(-209.985736525842,-5.85398007047323,
127.744139519898));
#252658=CARTESIAN_POINT('Ctrl Pts',(-210.264184149654,-5.73886989893714,
134.07535559084));
#252659=CARTESIAN_POINT('Ctrl Pts',(-210.542631773467,-0.350018649658268,
137.400687078332));
#252660=CARTESIAN_POINT('Ctrl Pts',(-210.82107939728,5.36048263929459,134.664316796842));
#252661=CARTESIAN_POINT('Ctrl Pts',(-211.099527021093,6.14496225687153,
128.38083535594));
#252662=CARTESIAN_POINT('Ctrl Pts',(-211.377974644906,1.28252175847855,
124.324455234681));
#252663=CARTESIAN_POINT('Ctrl Pts',(-211.656422268719,-4.75849358128477,
126.222791599316));
#252664=CARTESIAN_POINT('Ctrl Pts',(-211.934869892531,-6.4266857851828,
132.331366069634));
#252665=CARTESIAN_POINT('Ctrl Pts',(-212.213317516344,-2.18906771355195,
137.036697127864));
#252666=CARTESIAN_POINT('Ctrl Pts',(-212.491765140157,4.06019664492976,
136.014815399695));
#252667=CARTESIAN_POINT('Ctrl Pts',(-212.770212763971,6.57833863835413,
130.204780271616));
#252668=CARTESIAN_POINT('Ctrl Pts',(-213.048660387783,3.05130879283982,
124.945730190337));
#252669=CARTESIAN_POINT('Ctrl Pts',(-213.327108011596,-3.27972476857289,
125.070475261673));
#252670=CARTESIAN_POINT('Ctrl Pts',(-213.605555635409,-6.59685149112928,
130.464380859201));
#252671=CARTESIAN_POINT('Ctrl Pts',(-213.884003259222,-3.85179396744981,
136.170711245733));
#252672=CARTESIAN_POINT('Ctrl Pts',(-214.162450883035,2.43287404171984,
136.94562756578));
#252673=CARTESIAN_POINT('Ctrl Pts',(-214.440898506847,6.48184965905313,
132.077019577989));
#252674=CARTESIAN_POINT('Ctrl Pts',(-214.71934613066,4.57432209567675,126.038900178414));
#252675=CARTESIAN_POINT('Ctrl Pts',(-214.997793754473,-1.53678400556905,
124.380006116735));
#252676=CARTESIAN_POINT('Ctrl Pts',(-215.276241378286,-6.23566068176903,
128.624779994154));
#252677=CARTESIAN_POINT('Ctrl Pts',(-215.554689002099,-5.20426982038336,
134.872481986055));
#252678=CARTESIAN_POINT('Ctrl Pts',(-215.833136625912,0.609590763220439,
137.381779179092));
#252679=CARTESIAN_POINT('Ctrl Pts',(-216.111584249725,5.86326721558844,
133.846750038845));
#252680=CARTESIAN_POINT('Ctrl Pts',(-216.390031873537,5.72888753335829,
127.51591364943));
#252681=CARTESIAN_POINT('Ctrl Pts',(-216.668479497351,0.329940079686948,
124.206999374164));
#252682=CARTESIAN_POINT('Ctrl Pts',(-216.946927121163,-5.37220618874772,
126.960737782571));
#252683=CARTESIAN_POINT('Ctrl Pts',(-217.225374744977,-6.13755741658593,
133.246577804923));
#252684=CARTESIAN_POINT('Ctrl Pts',(-217.503822368789,-1.26279321493052,
137.288139541036));
#252685=CARTESIAN_POINT('Ctrl Pts',(-217.782269992602,4.77241626036792,
135.37142519669));
#252686=CARTESIAN_POINT('Ctrl Pts',(-218.060717616415,6.4220083378839,129.257801617636));
#252687=CARTESIAN_POINT('Ctrl Pts',(-218.339165240228,2.17008848543354,
124.565390205911));
#252688=CARTESIAN_POINT('Ctrl Pts',(-218.617612864041,-4.07603667041411,
125.606287811847));
#252689=CARTESIAN_POINT('Ctrl Pts',(-218.896060487854,-6.57648325161253,
131.423960386264));
#252690=CARTESIAN_POINT('Ctrl Pts',(-219.174508111666,-3.03346300364714,
136.672251042379));
#252691=CARTESIAN_POINT('Ctrl Pts',(-219.45295573548,3.29716155176439,136.528237060474));
#252692=CARTESIAN_POINT('Ctrl Pts',(-219.731403359293,6.59785571640026,
131.124260254445));
#252693=CARTESIAN_POINT('Ctrl Pts',(-220.009850983105,3.83544280083539,
125.426311310091));
#252694=CARTESIAN_POINT('Ctrl Pts',(-220.288298606918,-2.45155467689987,
124.67052694699));
#252695=CARTESIAN_POINT('Ctrl Pts',(-220.566746230731,-6.48569317166813,
129.551436072715));
#252696=CARTESIAN_POINT('Ctrl Pts',(-220.845193854544,-4.55979648539947,
135.58372164639));
#252697=CARTESIAN_POINT('Ctrl Pts',(-221.123641478357,1.55633041250914,
137.224007919343));
#252698=CARTESIAN_POINT('Ctrl Pts',(-221.40208910217,6.24226569228925,132.964951939167));
#252699=CARTESIAN_POINT('Ctrl Pts',(-221.680536725983,5.19186375248807,
126.720418085194));
#252700=CARTESIAN_POINT('Ctrl Pts',(-221.958984349796,-0.629607339204784,
124.228827906785));
#252701=CARTESIAN_POINT('Ctrl Pts',(-222.237431973609,-5.87250004419688,
127.779831056953));
#252702=CARTESIAN_POINT('Ctrl Pts',(-222.515879597421,-5.71885209614835,
134.110229116839));
#252703=CARTESIAN_POINT('Ctrl Pts',(-222.794327221234,-0.309858453196267,
137.402695526548));
#252704=CARTESIAN_POINT('Ctrl Pts',(-223.072774845047,5.38387997081673,
134.631614501482));
#252705=CARTESIAN_POINT('Ctrl Pts',(-223.35122246886,6.13009571880702,128.343474128844));
#252706=CARTESIAN_POINT('Ctrl Pts',(-223.629670092673,1.24305297303857,
124.316768218352));
#252707=CARTESIAN_POINT('Ctrl Pts',(-223.908117716486,-4.78629472843886,
126.25184278623));
#252708=CARTESIAN_POINT('Ctrl Pts',(-224.186565340298,-6.41727139797729,
132.370458838244));
#252709=CARTESIAN_POINT('Ctrl Pts',(-224.465012964112,-2.15108915391133,
137.049907133607));
#252710=CARTESIAN_POINT('Ctrl Pts',(-224.743460587925,4.09183893605206,
135.990003292637));
#252711=CARTESIAN_POINT('Ctrl Pts',(-225.021908211737,6.57456694122844,
130.164747166004));
#252712=CARTESIAN_POINT('Ctrl Pts',(-225.300355835551,3.01558911286705,
124.927264554503));
#252713=CARTESIAN_POINT('Ctrl Pts',(-225.578803459363,-3.31456779050113,
125.090546112851));
#252714=CARTESIAN_POINT('Ctrl Pts',(-225.857251083176,-6.5987988200372,
130.504544065675));
#252715=CARTESIAN_POINT('Ctrl Pts',(-226.135698706989,-3.8190561032033,
136.194058782834));
#252716=CARTESIAN_POINT('Ctrl Pts',(-226.414146330802,2.47021260121173,
136.930704187504));
#252717=CARTESIAN_POINT('Ctrl Pts',(-226.692593954615,6.48947660170784,
132.037539139922));
#252718=CARTESIAN_POINT('Ctrl Pts',(-226.971041578427,4.54522863379049,
126.011143274415));
#252719=CARTESIAN_POINT('Ctrl Pts',(-227.24948920224,-1.57586240181677,
124.389479985577));
#252720=CARTESIAN_POINT('Ctrl Pts',(-227.527936826054,-6.24881287531301,
128.662778613197));
#252721=CARTESIAN_POINT('Ctrl Pts',(-227.806384449866,-5.17940958787633,
134.904086480733));
#252722=CARTESIAN_POINT('Ctrl Pts',(-228.084832073679,0.649618082593193,
137.377946562762));
#252723=CARTESIAN_POINT('Ctrl Pts',(-228.363279697492,5.88167847076755,
133.811002298682));
#252724=CARTESIAN_POINT('Ctrl Pts',(-228.641727321305,5.70876368027354,
127.481101212267));
#252725=CARTESIAN_POINT('Ctrl Pts',(-228.920174945118,0.289773956218704,
124.205113169075));
#252726=CARTESIAN_POINT('Ctrl Pts',(-229.198622568931,-5.39550387735667,
126.993511139885));
#252727=CARTESIAN_POINT('Ctrl Pts',(-229.477070192744,-6.12257723265909,
133.283893610337));
#252728=CARTESIAN_POINT('Ctrl Pts',(-229.755517816557,-1.22330121567356,
137.295706392352));
#252729=CARTESIAN_POINT('Ctrl Pts',(-230.033965440369,4.80012885692891,
135.34228952721));
#252730=CARTESIAN_POINT('Ctrl Pts',(-230.312413064183,6.41247500934538,
129.218737684256));
#252731=CARTESIAN_POINT('Ctrl Pts',(-230.590860687995,2.13206989499296,
124.552295855027));
#252732=CARTESIAN_POINT('Ctrl Pts',(-230.869308311808,-4.10760329545278,
125.631196112227));
#252733=CARTESIAN_POINT('Ctrl Pts',(-231.147755935621,-6.5725897249546,
131.463981826697));
#252734=CARTESIAN_POINT('Ctrl Pts',(-231.426203559434,-2.99768728608136,
136.690607874263));
#252735=CARTESIAN_POINT('Ctrl Pts',(-231.704651183247,3.33194332353496,
136.508060252089));
#252736=CARTESIAN_POINT('Ctrl Pts',(-231.98309880706,6.59968079330357,131.084091307006));
#252737=CARTESIAN_POINT('Ctrl Pts',(-232.261546430872,3.80263402635669,
125.403063523931));
#252738=CARTESIAN_POINT('Ctrl Pts',(-232.539994054686,-2.48884764181187,
124.685563901874));
#252739=CARTESIAN_POINT('Ctrl Pts',(-232.818441678498,-6.49319991412244,
129.5909395417));
#252740=CARTESIAN_POINT('Ctrl Pts',(-233.096889302311,-4.53061867580467,
135.611389871331));
#252741=CARTESIAN_POINT('Ctrl Pts',(-233.375336926124,1.59537979255065,
137.214415153187));
#252742=CARTESIAN_POINT('Ctrl Pts',(-233.653784549937,6.25530217018742,
132.926913465378));
#252743=CARTESIAN_POINT('Ctrl Pts',(-233.93223217375,5.16690744192206,126.688889402902));
#252744=CARTESIAN_POINT('Ctrl Pts',(-234.210679797563,-0.669622808008655,
124.232782334755));
#252745=CARTESIAN_POINT('Ctrl Pts',(-234.489127421376,-5.89080241027189,
127.815634669064));
#252746=CARTESIAN_POINT('Ctrl Pts',(-234.767575045188,-5.69862237919218,
134.144980142666));
#252747=CARTESIAN_POINT('Ctrl Pts',(-235.046022669002,-0.269686774814632,
137.404459471037));
#252748=CARTESIAN_POINT('Ctrl Pts',(-235.324470292814,5.40707780068583,
134.598770385822));
#252749=CARTESIAN_POINT('Ctrl Pts',(-235.602917916627,6.11500202779203,
128.306204090801));
#252750=CARTESIAN_POINT('Ctrl Pts',(-235.88136554044,1.20353812581378,124.309321602146));
#252751=CARTESIAN_POINT('Ctrl Pts',(-236.159813164253,-4.81391851768082,
126.281062668365));
#252752=CARTESIAN_POINT('Ctrl Pts',(-236.438260788066,-6.40761921642086,
132.40949357451));
#252753=CARTESIAN_POINT('Ctrl Pts',(-236.716708411879,-2.11303088487057,
137.062885708328));
#252754=CARTESIAN_POINT('Ctrl Pts',(-236.995156035692,4.12332960257798,
135.964999029683));
#252755=CARTESIAN_POINT('Ctrl Pts',(-237.273603659505,6.57055162110693,
130.124737761504));
#252756=CARTESIAN_POINT('Ctrl Pts',(-237.552051283318,2.97975768913041,
124.909016696624));
#252757=CARTESIAN_POINT('Ctrl Pts',(-237.83049890713,-3.34928798990126,
125.110828691528));
#252758=CARTESIAN_POINT('Ctrl Pts',(-238.108946530943,-6.60050162802816,
130.544718381962));
#252759=CARTESIAN_POINT('Ctrl Pts',(-238.387394154756,-3.7861767224282,
136.217206602688));
#252760=CARTESIAN_POINT('Ctrl Pts',(-238.665841778569,2.5074596260677,136.915553795314));
#252761=CARTESIAN_POINT('Ctrl Pts',(-238.944289402382,6.49686307441993,
131.998013005973));
#252762=CARTESIAN_POINT('Ctrl Pts',(-239.222737026195,4.51596674678651,
125.983563984846));
#252763=CARTESIAN_POINT('Ctrl Pts',(-239.501184650008,-1.61488240390346,
124.399191560181));
#252764=CARTESIAN_POINT('Ctrl Pts',(-239.77963227382,-6.26173351679718,
128.700856589348));
#252765=CARTESIAN_POINT('Ctrl Pts',(-240.058079897633,-5.15435743044315,
134.935539058562));
#252766=CARTESIAN_POINT('Ctrl Pts',(-240.336527521446,0.689621330129741,
137.373870359787));
#252767=CARTESIAN_POINT('Ctrl Pts',(-240.614975145259,5.89987177818775,
133.775143146303));
#252768=CARTESIAN_POINT('Ctrl Pts',(-240.893422769072,5.68842828685113,
127.446411919705));
#252769=CARTESIAN_POINT('Ctrl Pts',(-241.171870392886,0.249597095069331,
124.203471501526));
#252770=CARTESIAN_POINT('Ctrl Pts',(-241.450318016698,-5.41860163358522,
127.026425709627));
#252771=CARTESIAN_POINT('Ctrl Pts',(-241.728765640511,-6.10737017438111,
133.321117535742));
#252772=CARTESIAN_POINT('Ctrl Pts',(-242.007213264324,-1.18376388654087,
137.303032704464));
#252773=CARTESIAN_POINT('Ctrl Pts',(-242.285660888137,4.82766358294966,
135.312985703106));
#252774=CARTESIAN_POINT('Ctrl Pts',(-242.56410851195,6.40270406418687,129.179732506718));
#252775=CARTESIAN_POINT('Ctrl Pts',(-242.842556135762,2.09397229991911,
124.539433176702));
#252776=CARTESIAN_POINT('Ctrl Pts',(-243.121003759575,-4.13901771174057,
125.65629610612));
#252777=CARTESIAN_POINT('Ctrl Pts',(-243.399451383388,-6.56845264856689,
131.503978824623));
#252778=CARTESIAN_POINT('Ctrl Pts',(-243.677899007202,-2.9618004881116,
136.70874658909));
#252779=CARTESIAN_POINT('Ctrl Pts',(-243.956346631013,3.36660162892119,
136.487672091016));
#252780=CARTESIAN_POINT('Ctrl Pts',(-244.234794254827,6.60126131660758,
131.043911994042));
#252781=CARTESIAN_POINT('Ctrl Pts',(-244.513241878639,3.76968434387551,
125.380015884821));
#252782=CARTESIAN_POINT('Ctrl Pts',(-244.791689502453,-2.52604838156001,
124.70082759102));
#252783=CARTESIAN_POINT('Ctrl Pts',(-245.070137126265,-6.50046604866569,
129.630487974449));
#252784=CARTESIAN_POINT('Ctrl Pts',(-245.348584750079,-4.50127298246883,
135.638879970036));
#252785=CARTESIAN_POINT('Ctrl Pts',(-245.627032373891,1.63437005520677,
137.204584860103));
#252786=CARTESIAN_POINT('Ctrl Pts',(-245.905479997704,6.26810685556324,
132.888796339615));
#252787=CARTESIAN_POINT('Ctrl Pts',(-246.183927621517,5.14175966970064,
126.65751322091));
#252788=CARTESIAN_POINT('Ctrl Pts',(-246.46237524533,-0.709613463692526,
124.236980274974));
#252789=CARTESIAN_POINT('Ctrl Pts',(-246.740822869143,-5.90888649049716,
127.851549029514));
#252790=CARTESIAN_POINT('Ctrl Pts',(-247.019270492956,-5.67818149768794,
134.179607380607));
#252791=CARTESIAN_POINT('Ctrl Pts',(-247.297718116769,-0.229505103091092,
137.405978846438));
#252792=CARTESIAN_POINT('Ctrl Pts',(-247.576165740581,5.43007526929941,
134.565785666913));
#252793=CARTESIAN_POINT('Ctrl Pts',(-247.854613364394,6.09968174312738,
128.269026622868));
#252794=CARTESIAN_POINT('Ctrl Pts',(-248.133060988207,1.16397868104094,
124.302115661998));
#252795=CARTESIAN_POINT('Ctrl Pts',(-248.41150861202,-4.84136392540264,
126.31045016297));
#252796=CARTESIAN_POINT('Ctrl Pts',(-248.689956235833,-6.39772959817725,
132.448468831983));
#252797=CARTESIAN_POINT('Ctrl Pts',(-248.968403859646,-2.07489431669385,
137.075632371099));
#252798=CARTESIAN_POINT('Ctrl Pts',(-249.246851483459,4.15466747760909,
135.939803537374));
#252799=CARTESIAN_POINT('Ctrl Pts',(-249.525299107272,6.56629282677857,
130.08475354068));
#252800=CARTESIAN_POINT('Ctrl Pts',(-249.803746731085,2.94381584937754,
124.890987292882));
#252801=CARTESIAN_POINT('Ctrl Pts',(-250.082194354898,-3.38388408020374,
125.131322246124));
#252802=CARTESIAN_POINT('Ctrl Pts',(-250.36064197871,-6.60195985200274,
130.584902319384));
#252803=CARTESIAN_POINT('Ctrl Pts',(-250.639089602524,-3.75315704348482,
136.240153847548));
#252804=CARTESIAN_POINT('Ctrl Pts',(-250.917537226336,2.54461373609029,
136.900176950603));
#252805=CARTESIAN_POINT('Ctrl Pts',(-251.19598485015,6.50400880347224,131.958442640812));
#252806=CARTESIAN_POINT('Ctrl Pts',(-251.474432473962,4.48653751899202,
125.956163331638));
#252807=CARTESIAN_POINT('Ctrl Pts',(-251.752880097775,-1.65384256596459,
124.409140480742));
#252808=CARTESIAN_POINT('Ctrl Pts',(-252.031327721588,-6.27442212737671,
128.739012511497));
#252809=CARTESIAN_POINT('Ctrl Pts',(-252.309775345401,-5.12911427652582,
134.966838554275));
#252810=CARTESIAN_POINT('Ctrl Pts',(-252.588222969213,0.729599023732927,
137.369550720794));
#252811=CARTESIAN_POINT('Ctrl Pts',(-252.866670593027,5.91784646323776,
133.739173911277));
#252812=CARTESIAN_POINT('Ctrl Pts',(-253.145118216839,5.66788210748017,
127.411847055674));
#252813=CARTESIAN_POINT('Ctrl Pts',(-253.423565840652,0.209410983396998,
124.20207443517));
#252814=CARTESIAN_POINT('Ctrl Pts',(-253.702013464465,-5.44149859849489,
127.059480266814));
#252815=CARTESIAN_POINT('Ctrl Pts',(-253.980461088278,-6.0919368110008,
133.358248211846));
#252816=CARTESIAN_POINT('Ctrl Pts',(-254.258908712091,-1.1441826817532,
137.310118186916));
#252817=CARTESIAN_POINT('Ctrl Pts',(-254.537356335904,4.85501939763767,
135.283514846073));
#252818=CARTESIAN_POINT('Ctrl Pts',(-254.815803959717,6.39269590315201,
129.140787462715));
#252819=CARTESIAN_POINT('Ctrl Pts',(-255.09425158353,2.05579703890082,124.526802775315));
#252820=CARTESIAN_POINT('Ctrl Pts',(-255.372699207342,-4.17027861730954,
125.681586622223));
#252821=CARTESIAN_POINT('Ctrl Pts',(-255.651146831155,-6.5640724361261,
131.5439503534));
#252822=CARTESIAN_POINT('Ctrl Pts',(-255.929594454968,-2.925803447894,136.726665654721));
#252823=CARTESIAN_POINT('Ctrl Pts',(-256.208042078781,3.40113425532747,
136.467074956607));
#252824=CARTESIAN_POINT('Ctrl Pts',(-256.486489702594,6.60259898059897,
131.003720738236));
#252825=CARTESIAN_POINT('Ctrl Pts',(-256.764937326407,3.73659166461274,
125.357175036369));
#252826=CARTESIAN_POINT('Ctrl Pts',(-257.04338495022,-2.56314926818932,
124.716306516944));
#252827=CARTESIAN_POINT('Ctrl Pts',(-257.321832574033,-6.5075031063131,
129.670100547101));
#252828=CARTESIAN_POINT('Ctrl Pts',(-257.600280197845,-4.47173821150659,
135.666151948257));
#252829=CARTESIAN_POINT('Ctrl Pts',(-257.878727821659,1.67325768403046,
137.194590998305));
#252830=CARTESIAN_POINT('Ctrl Pts',(-258.157175445471,6.28075871394982,
132.850463013089));
#252831=CARTESIAN_POINT('Ctrl Pts',(-258.435623069284,5.1162713672671,126.626553096149));
#252832=CARTESIAN_POINT('Ctrl Pts',(-258.714070693097,-0.749294580734974,
124.240926059104));
#252833=CARTESIAN_POINT('Ctrl Pts',(-258.99251831691,-5.92728653745133,
127.888508918958));
#252834=CARTESIAN_POINT('Ctrl Pts',(-259.270965940723,-5.656519339957,134.212338033208));
#252835=CARTESIAN_POINT('Ctrl Pts',(-259.549413564536,-0.191230405826049,
137.41063083554));
#252836=CARTESIAN_POINT('Ctrl Pts',(-259.827861188349,5.45654320709978,
134.526020746857));
#252837=CARTESIAN_POINT('Ctrl Pts',(-260.059900874859,5.97341346954355,
129.293215926205));
#252838=CARTESIAN_POINT('Ctrl Pts',(-260.245542550368,3.60742224527213,
126.247226657536));
#252839=CARTESIAN_POINT('Ctrl Pts',(-260.338368351272,1.86717727106152,
125.459413119698));
#252840=CARTESIAN_POINT('Ctrl Pts',(-260.384786214875,0.950008195528324,
125.301089073499));
#252841=CARTESIAN_POINT('Ctrl Pts',(209.997886486728,-2.58542267678463,
125.478296443779));
#252842=CARTESIAN_POINT('Ctrl Pts',(209.951476810375,-3.47289965896197,
125.909102290886));
#252843=CARTESIAN_POINT('Ctrl Pts',(209.85865919672,-5.01373755653622,127.222906143875));
#252844=CARTESIAN_POINT('Ctrl Pts',(209.67302570846,-6.52844908712303,131.020616473957));
#252845=CARTESIAN_POINT('Ctrl Pts',(209.440986021949,-4.4641631800594,136.198709217918));
#252846=CARTESIAN_POINT('Ctrl Pts',(209.162538398136,2.13623200523086,137.47712630299));
#252847=CARTESIAN_POINT('Ctrl Pts',(208.884090774324,6.76311047611758,132.61329501932));
#252848=CARTESIAN_POINT('Ctrl Pts',(208.60564315051,5.180460236421,126.09244423763));
#252849=CARTESIAN_POINT('Ctrl Pts',(208.327195526698,-1.16565068102074,
123.898824768668));
#252850=CARTESIAN_POINT('Ctrl Pts',(208.048747902884,-6.43906639651766,
128.052530506575));
#252851=CARTESIAN_POINT('Ctrl Pts',(207.770300279072,-5.79609906993421,
134.734252735451));
#252852=CARTESIAN_POINT('Ctrl Pts',(207.491852655259,0.173626147510206,
137.805009652024));
#252853=CARTESIAN_POINT('Ctrl Pts',(207.213405031446,5.98357180802623,134.442293088818));
#252854=CARTESIAN_POINT('Ctrl Pts',(206.934957407633,6.29502677410122,127.736610299611));
#252855=CARTESIAN_POINT('Ctrl Pts',(206.65650978382,0.821596385081328,123.849978754804));
#252856=CARTESIAN_POINT('Ctrl Pts',(206.378062160007,-5.40680743188727,
126.354116934927));
#252857=CARTESIAN_POINT('Ctrl Pts',(206.099614536195,-6.66663710465116,
132.947794423038));
#252858=CARTESIAN_POINT('Ctrl Pts',(205.821166912381,-1.80014356190772,
137.571770081489));
#252859=CARTESIAN_POINT('Ctrl Pts',(205.542719288569,4.72058899422897,135.976822216287));
#252860=CARTESIAN_POINT('Ctrl Pts',(205.264271664756,6.90333351468265,129.628637390042));
#252861=CARTESIAN_POINT('Ctrl Pts',(204.985824040943,2.74225038547515,124.360883417158));
#252862=CARTESIAN_POINT('Ctrl Pts',(204.70737641713,-3.93882614214087,125.014370927945));
#252863=CARTESIAN_POINT('Ctrl Pts',(204.428928793317,-7.00031425910704,
130.988575726592));
#252864=CARTESIAN_POINT('Ctrl Pts',(204.150481169504,-3.62885534891233,
136.793496040797));
#252865=CARTESIAN_POINT('Ctrl Pts',(203.872033545692,3.07734423765085,137.09469337995));
#252866=CARTESIAN_POINT('Ctrl Pts',(203.593585921878,6.95561486460971,131.615382266785));
#252867=CARTESIAN_POINT('Ctrl Pts',(203.315138298066,4.44201520086038,125.390781848689));
#252868=CARTESIAN_POINT('Ctrl Pts',(203.036690674253,-2.15357941165663,
124.140995867004));
#252869=CARTESIAN_POINT('Ctrl Pts',(202.75824305044,-6.77013976170558,129.014516559232));
#252870=CARTESIAN_POINT('Ctrl Pts',(202.479795426627,-5.16527240588502,
135.532816506767));
#252871=CARTESIAN_POINT('Ctrl Pts',(202.201347802814,1.18622795093483,137.705896487686));
#252872=CARTESIAN_POINT('Ctrl Pts',(201.922900179001,6.44764277258624,133.536802163981));
#252873=CARTESIAN_POINT('Ctrl Pts',(201.644452555188,5.78398887041165,126.856727545651));
#252874=CARTESIAN_POINT('Ctrl Pts',(201.366004931376,-0.194868239746226,
123.804334868162));
#252875=CARTESIAN_POINT('Ctrl Pts',(201.087557307562,-5.99465095761073,
127.184623883922));
#252876=CARTESIAN_POINT('Ctrl Pts',(200.80910968375,-6.2856423003101,133.891274124028));
#252877=CARTESIAN_POINT('Ctrl Pts',(200.530662059936,-0.80043543977546,
137.76120165575));
#252878=CARTESIAN_POINT('Ctrl Pts',(200.252214436124,5.42033248649604,135.238132133988));
#252879=CARTESIAN_POINT('Ctrl Pts',(199.973766812311,6.66007965562565,128.640643190398));
#252880=CARTESIAN_POINT('Ctrl Pts',(199.695319188498,1.77953898422249,124.031504858911));
#252881=CARTESIAN_POINT('Ctrl Pts',(199.416871564685,-4.73631107837294,
125.646290097223));
#252882=CARTESIAN_POINT('Ctrl Pts',(199.138423940872,-6.89972264160091,
132.00109015798));
#252883=CARTESIAN_POINT('Ctrl Pts',(198.859976317059,-2.72262616738874,
137.256154234582));
#252884=CARTESIAN_POINT('Ctrl Pts',(198.581528693247,3.95643074697165,136.582335164788));
#252885=CARTESIAN_POINT('Ctrl Pts',(198.303081069434,6.999721087252,130.598839755845));
#252886=CARTESIAN_POINT('Ctrl Pts',(198.024633445621,3.61060970373355,124.804207978572));
#252887=CARTESIAN_POINT('Ctrl Pts',(197.746185821808,-3.09647560942607,
124.523423352781));
#252888=CARTESIAN_POINT('Ctrl Pts',(197.467738197995,-6.9580511087663,130.014513232485));
#252889=CARTESIAN_POINT('Ctrl Pts',(197.189290574182,-4.4255175588443,136.231434272887));
#252890=CARTESIAN_POINT('Ctrl Pts',(196.910842950369,2.17385042910367,137.461139751337));
#252891=CARTESIAN_POINT('Ctrl Pts',(196.632395326556,6.77555607120273,132.573590407591));
#252892=CARTESIAN_POINT('Ctrl Pts',(196.353947702743,5.15085668818228,126.060205318492));
#252893=CARTESIAN_POINT('Ctrl Pts',(196.07550007893,-1.20722835793932,123.90646718437));
#252894=CARTESIAN_POINT('Ctrl Pts',(195.797052455118,-6.45592951949867,
128.091556134528));
#252895=CARTESIAN_POINT('Ctrl Pts',(195.518604831305,-5.77194684232935,
134.769579876729));
#252896=CARTESIAN_POINT('Ctrl Pts',(195.240157207492,0.216173007661386,
137.80376083149));
#252897=CARTESIAN_POINT('Ctrl Pts',(194.961709583679,6.00564042424985,134.405834929363));
#252898=CARTESIAN_POINT('Ctrl Pts',(194.683261959866,6.2762176827981,127.698330076496));
#252899=CARTESIAN_POINT('Ctrl Pts',(194.404814336053,0.779257501134259,
123.845115552844));
#252900=CARTESIAN_POINT('Ctrl Pts',(194.12636671224,-5.43380225522669,126.387107265649));
#252901=CARTESIAN_POINT('Ctrl Pts',(193.847919088427,-6.65346319503207,
132.988339014042));
#252902=CARTESIAN_POINT('Ctrl Pts',(193.569471464615,-1.75891649835014,
137.58260130935));
#252903=CARTESIAN_POINT('Ctrl Pts',(193.291023840801,4.75198853246758,135.947991544374));
#252904=CARTESIAN_POINT('Ctrl Pts',(193.012576216989,6.89604824949333,129.586636238002));
#252905=CARTESIAN_POINT('Ctrl Pts',(192.734128593176,2.70297651592057,124.344310147306));
#252906=CARTESIAN_POINT('Ctrl Pts',(192.455680969363,-3.97399858803937,
125.038454847768));
#252907=CARTESIAN_POINT('Ctrl Pts',(192.17723334555,-6.99906313021511,131.031185270517));
#252908=CARTESIAN_POINT('Ctrl Pts',(191.898785721737,-3.59233057896577,
136.815474918205));
#252909=CARTESIAN_POINT('Ctrl Pts',(191.620338097924,3.11557827924791,137.075844182864));
#252910=CARTESIAN_POINT('Ctrl Pts',(191.341890474111,6.96042290329331,131.573026430018));
#252911=CARTESIAN_POINT('Ctrl Pts',(191.063442850298,4.40897891477476,125.363842346942));
#252912=CARTESIAN_POINT('Ctrl Pts',(190.784995226486,-2.19410130582752,
124.154228770475));
#252913=CARTESIAN_POINT('Ctrl Pts',(190.506547602672,-6.78090961418206,
129.055761484483));
#252914=CARTESIAN_POINT('Ctrl Pts',(190.22809997886,-5.13639325295408,135.564171377977));
#252915=CARTESIAN_POINT('Ctrl Pts',(189.949652355047,1.22821758097839,137.698547712335));
#252916=CARTESIAN_POINT('Ctrl Pts',(189.671204731234,6.46415645975623,133.497502906364));
#252917=CARTESIAN_POINT('Ctrl Pts',(189.392757107421,5.75985134361714,126.821591904301));
#252918=CARTESIAN_POINT('Ctrl Pts',(189.114309483608,-0.237475772924818,
123.80565078066));
#252919=CARTESIAN_POINT('Ctrl Pts',(188.835861859795,-6.01657425548534,
127.221182091151));
#252920=CARTESIAN_POINT('Ctrl Pts',(188.557414235982,-6.2667349232476,133.929479419415));
#252921=CARTESIAN_POINT('Ctrl Pts',(188.278966612169,-0.758072343566082,
137.76594523932));
#252922=CARTESIAN_POINT('Ctrl Pts',(188.000518988357,5.44722168595988,135.205054884148));
#252923=CARTESIAN_POINT('Ctrl Pts',(187.722071364544,6.64678509766207,128.600141483854));
#252924=CARTESIAN_POINT('Ctrl Pts',(187.443623740731,1.73827771811677,124.02079778535));
#252925=CARTESIAN_POINT('Ctrl Pts',(187.165176116918,-4.76762196479028,
125.675216934184));
#252926=CARTESIAN_POINT('Ctrl Pts',(186.886728493105,-6.89230997333645,
132.043068555446));
#252927=CARTESIAN_POINT('Ctrl Pts',(186.608280869292,-2.68330182444739,
137.272608096043));
#252928=CARTESIAN_POINT('Ctrl Pts',(186.329833245479,3.99152961452714,136.558144195375));
#252929=CARTESIAN_POINT('Ctrl Pts',(186.051385621667,6.99834033481346,130.556234274655));
#252930=CARTESIAN_POINT('Ctrl Pts',(185.772937997853,3.5740181753383,124.782340341422));
#252931=CARTESIAN_POINT('Ctrl Pts',(185.494490374041,-3.13465208677821,
124.542388849921));
#252932=CARTESIAN_POINT('Ctrl Pts',(185.216042750227,-6.96273021741339,
130.056883498557));
#252933=CARTESIAN_POINT('Ctrl Pts',(184.937595126415,-4.39239942652681,
136.258273103275));
#252934=CARTESIAN_POINT('Ctrl Pts',(184.659147502602,2.21433185669671,137.447783572063));
#252935=CARTESIAN_POINT('Ctrl Pts',(184.380699878789,6.78620033974098,132.532312894923));
#252936=CARTESIAN_POINT('Ctrl Pts',(184.102252254976,5.12188223488049,126.028938490053));
#252937=CARTESIAN_POINT('Ctrl Pts',(183.823804631163,-1.24919542597752,
123.913943728027));
#252938=CARTESIAN_POINT('Ctrl Pts',(183.54535700735,-6.47232351695142,128.130905471908));
#252939=CARTESIAN_POINT('Ctrl Pts',(183.266909383538,-5.74770248642891,
134.804641889104));
#252940=CARTESIAN_POINT('Ctrl Pts',(182.988461759724,0.258776338245136,
137.80231524236));
#252941=CARTESIAN_POINT('Ctrl Pts',(182.710014135912,6.02745234999885,134.369210164519));
#252942=CARTESIAN_POINT('Ctrl Pts',(182.431566512099,6.25719410952084,127.66018250561));
#252943=CARTESIAN_POINT('Ctrl Pts',(182.153118888286,0.73688016331929,123.840500929948));
#252944=CARTESIAN_POINT('Ctrl Pts',(181.874671264473,-5.46059065437546,
126.420266203747));
#252945=CARTESIAN_POINT('Ctrl Pts',(181.59622364066,-6.64004542538295,133.028800068927));
#252946=CARTESIAN_POINT('Ctrl Pts',(181.317776016847,-1.71762283471616,
137.593182748215));
#252947=CARTESIAN_POINT('Ctrl Pts',(181.039328393035,4.78321123051439,135.918969541833));
#252948=CARTESIAN_POINT('Ctrl Pts',(180.760880769221,6.88850784776155,129.544680596588));
#252949=CARTESIAN_POINT('Ctrl Pts',(180.482433145409,2.66360227523266,124.32797605183));
#252950=CARTESIAN_POINT('Ctrl Pts',(180.203985521595,-4.00902366402984,
125.062752534008));
#252951=CARTESIAN_POINT('Ctrl Pts',(179.925537897783,-6.99755270774298,
131.073786351827));
#252952=CARTESIAN_POINT('Ctrl Pts',(179.64709027397,-3.5556726624947,136.837231082039));
#252953=CARTESIAN_POINT('Ctrl Pts',(179.368642650157,3.15369685531979,137.056762577506));
#252954=CARTESIAN_POINT('Ctrl Pts',(179.090195026344,6.96497302975191,131.530642118605));
#252955=CARTESIAN_POINT('Ctrl Pts',(178.811747402531,4.37577924769062,125.337104441072));
#252956=CARTESIAN_POINT('Ctrl Pts',(178.533299778718,-2.23454189429802,
124.167708099424));
#252957=CARTESIAN_POINT('Ctrl Pts',(178.254852154906,-6.79142819886702,
129.097071203448));
#252958=CARTESIAN_POINT('Ctrl Pts',(177.976404531092,-5.10732376838957,
135.595349873321));
#252959=CARTESIAN_POINT('Ctrl Pts',(177.69795690728,1.27016169860089,137.690943469992));
#252960=CARTESIAN_POINT('Ctrl Pts',(177.419509283467,6.48043061542571,133.458103853558));
#252961=CARTESIAN_POINT('Ctrl Pts',(177.141061659654,5.73550038331004,126.786603845811));
#252962=CARTESIAN_POINT('Ctrl Pts',(176.862614035841,-0.280074506296806,
123.807226032976));
#252963=CARTESIAN_POINT('Ctrl Pts',(176.584166412028,-6.0382746070172,127.257873074351));
#252964=CARTESIAN_POINT('Ctrl Pts',(176.305718788215,-6.24759533000263,
133.967568912391));
#252965=CARTESIAN_POINT('Ctrl Pts',(176.027271164402,-0.71568115671533,
137.770430858802));
#252966=CARTESIAN_POINT('Ctrl Pts',(175.748823540589,5.4739090366252,135.171814564968));
#252967=CARTESIAN_POINT('Ctrl Pts',(175.470375916777,6.63324424063007,128.559721455457));
#252968=CARTESIAN_POINT('Ctrl Pts',(175.191928292964,1.69695203949225,124.010342079205));
#252969=CARTESIAN_POINT('Ctrl Pts',(174.913480669151,-4.79875618522306,
125.704333833448));
#252970=CARTESIAN_POINT('Ctrl Pts',(174.635033045338,-6.88464190799096,
132.085001052137));
#252971=CARTESIAN_POINT('Ctrl Pts',(174.356585421525,-2.64387805077028,
137.288822274217));
#252972=CARTESIAN_POINT('Ctrl Pts',(174.078137797712,4.02648057448505,136.533740017397));
#252973=CARTESIAN_POINT('Ctrl Pts',(173.799690173899,6.99670025630013,130.513637987877));
#252974=CARTESIAN_POINT('Ctrl Pts',(173.521242550086,3.53729421038521,124.76069585245));
#252975=CARTESIAN_POINT('Ctrl Pts',(173.242794926273,-3.17271240844464,
124.561586386726));
#252976=CARTESIAN_POINT('Ctrl Pts',(172.96434730246,-6.96715131953175,130.099281462668));
#252977=CARTESIAN_POINT('Ctrl Pts',(172.685899678648,-4.35911853223319,
136.284909836929));
#252978=CARTESIAN_POINT('Ctrl Pts',(172.407452054835,2.25473123140845,137.434181218309));
#252979=CARTESIAN_POINT('Ctrl Pts',(172.129004431022,6.79659314313001,132.490971352347));
#252980=CARTESIAN_POINT('Ctrl Pts',(171.850556807209,5.09271798834896,125.997848616637));
#252981=CARTESIAN_POINT('Ctrl Pts',(171.572109183396,-1.29111620461978,
123.921675598615));
#252982=CARTESIAN_POINT('Ctrl Pts',(171.293661559583,-6.48847768007612,
128.170353875152));
#252983=CARTESIAN_POINT('Ctrl Pts',(171.01521393577,-5.72324514729908,134.839555669585));
#252984=CARTESIAN_POINT('Ctrl Pts',(170.736766311957,0.301370079776633,
137.800610341449));
#252985=CARTESIAN_POINT('Ctrl Pts',(170.458318688145,6.04904092628448,134.332453302864));
#252986=CARTESIAN_POINT('Ctrl Pts',(170.179871064331,6.23793867361471,127.6221514434));
#252987=CARTESIAN_POINT('Ctrl Pts',(169.901423440519,0.694475520138818,
123.836144355433));
#252988=CARTESIAN_POINT('Ctrl Pts',(169.622975816706,-5.4871767093294,126.453587596077));
#252989=CARTESIAN_POINT('Ctrl Pts',(169.344528192893,-6.62638160640872,
133.06917869639));
#252990=CARTESIAN_POINT('Ctrl Pts',(169.06608056908,-1.67626552393645,137.603512624779));
#252991=CARTESIAN_POINT('Ctrl Pts',(168.787632945267,4.81425668490999,135.88975801558));
#252992=CARTESIAN_POINT('Ctrl Pts',(168.509185321454,6.88071218983824,129.50277163308));
#252993=CARTESIAN_POINT('Ctrl Pts',(168.230737697641,2.62412933378287,124.311881941165));
#252994=CARTESIAN_POINT('Ctrl Pts',(167.952290073828,-4.0439001841742,125.087262977647));
#252995=CARTESIAN_POINT('Ctrl Pts',(167.673842450016,-6.99578298838191,
131.116377449467));
#252996=CARTESIAN_POINT('Ctrl Pts',(167.395394826203,-3.51888298926545,
136.858763695638));
#252997=CARTESIAN_POINT('Ctrl Pts',(167.11694720239,3.19169856999505,137.037449287095));
#252998=CARTESIAN_POINT('Ctrl Pts',(166.838499578577,6.96926506657354,131.488230894564));
#252999=CARTESIAN_POINT('Ctrl Pts',(166.560051954764,4.34241743449723,125.310569126392));
#253000=CARTESIAN_POINT('Ctrl Pts',(166.281604330951,-2.27489968099678,
124.181433351974));
#253001=CARTESIAN_POINT('Ctrl Pts',(166.003156707138,-6.80169512468258,
129.13844418665));
#253002=CARTESIAN_POINT('Ctrl Pts',(165.724709083325,-5.0780650300646,135.626350836796));
#253003=CARTESIAN_POINT('Ctrl Pts',(165.446261459512,1.31205874991464,137.683084042787));
#253004=CARTESIAN_POINT('Ctrl Pts',(165.1678138357,6.49646463635559,133.418606465321));
#253005=CARTESIAN_POINT('Ctrl Pts',(164.889366211887,5.71093689192698,126.751764666776));
#253006=CARTESIAN_POINT('Ctrl Pts',(164.610918588074,-0.322662861405092,
123.809060566689));
#253007=CARTESIAN_POINT('Ctrl Pts',(164.332470964261,-6.05975120806294,
127.29469547395));
#253008=CARTESIAN_POINT('Ctrl Pts',(164.054023340448,-6.22822422981513,
134.00554119152));
#253009=CARTESIAN_POINT('Ctrl Pts',(163.775575716635,-0.673263450036036,
137.774658347991));
#253010=CARTESIAN_POINT('Ctrl Pts',(163.497128092822,5.50039354957815,135.138412408175));
#253011=CARTESIAN_POINT('Ctrl Pts',(163.218680469009,6.61945758629338,128.51938460299));
#253012=CARTESIAN_POINT('Ctrl Pts',(162.940232845196,1.65556347968583,124.000138127916));
#253013=CARTESIAN_POINT('Ctrl Pts',(162.661785221384,-4.82971258598073,
125.733639716082));
#253014=CARTESIAN_POINT('Ctrl Pts',(162.383337597571,-6.87671872970774,
132.126886094224));
#253015=CARTESIAN_POINT('Ctrl Pts',(162.104889973758,-2.60435630721971,
137.304796168278));
#253016=CARTESIAN_POINT('Ctrl Pts',(161.826442349945,4.06128233172446,136.509123535159));
#253017=CARTESIAN_POINT('Ctrl Pts',(161.547994726132,6.99480091248578,130.471052473933));
#253018=CARTESIAN_POINT('Ctrl Pts',(161.269547102319,3.50043916969439,124.739275313697));
#253019=CARTESIAN_POINT('Ctrl Pts',(160.991099478506,-3.21065516408591,
124.581015251828));
#253020=CARTESIAN_POINT('Ctrl Pts',(160.712651854693,-6.97131425129578,
130.141705553748));
#253021=CARTESIAN_POINT('Ctrl Pts',(160.434204230881,-4.32567610919938,
136.311343486817));
#253022=CARTESIAN_POINT('Ctrl Pts',(160.155756607067,2.29504705622523,137.420333194114));
#253023=CARTESIAN_POINT('Ctrl Pts',(159.877308983254,6.80673409626067,132.449567311792));
#253024=CARTESIAN_POINT('Ctrl Pts',(159.598861359442,5.06336502927952,125.966936850291));
#253025=CARTESIAN_POINT('Ctrl Pts',(159.320413735629,-1.33298914047637,
123.929662509627));
#253026=CARTESIAN_POINT('Ctrl Pts',(159.041966111816,-6.50439141027418,
128.209899882485));
#253027=CARTESIAN_POINT('Ctrl Pts',(158.763518488003,-5.69857573121565,
134.874319924428));
#253028=CARTESIAN_POINT('Ctrl Pts',(158.48507086419,0.343952653928878,137.798646191931));
#253029=CARTESIAN_POINT('Ctrl Pts',(158.206623240377,6.07040535313402,134.295565706438));
#253030=CARTESIAN_POINT('Ctrl Pts',(157.928175616564,6.2184520885971,127.584238299121));
#253031=CARTESIAN_POINT('Ctrl Pts',(157.649727992752,0.652045142912632,
123.832045990734));
#253032=CARTESIAN_POINT('Ctrl Pts',(157.371280368939,-5.51355943493244,
126.487070207899));
#253033=CARTESIAN_POINT('Ctrl Pts',(157.092832745126,-6.61247224442723,
133.109473400187));
#253034=CARTESIAN_POINT('Ctrl Pts',(156.814385121313,-1.63484609852131,
137.613590556265));
#253035=CARTESIAN_POINT('Ctrl Pts',(156.5359374975,4.84512374525377,135.860358048054));
#253036=CARTESIAN_POINT('Ctrl Pts',(156.257489873687,6.87266156459436,129.46091090043));
#253037=CARTESIAN_POINT('Ctrl Pts',(155.979042249874,2.58455915425555,124.296028411687));
#253038=CARTESIAN_POINT('Ctrl Pts',(155.700594626061,-4.07862685611001,
125.111985270442));
#253039=CARTESIAN_POINT('Ctrl Pts',(155.422147002248,-6.99375403770952,
131.158956985208));
#253040=CARTESIAN_POINT('Ctrl Pts',(155.143699378435,-3.48196292253304,
136.880071961106));
#253041=CARTESIAN_POINT('Ctrl Pts',(154.865251754623,3.22958201510593,137.017905027291));
#253042=CARTESIAN_POINT('Ctrl Pts',(154.58680413081,6.97329885471516,131.445794329457));
#253043=CARTESIAN_POINT('Ctrl Pts',(154.308356506997,4.30889471142897,125.284237386175));
#253044=CARTESIAN_POINT('Ctrl Pts',(154.029908883184,-2.31517317045128,
124.195404019528));
#253045=CARTESIAN_POINT('Ctrl Pts',(153.751461259371,-6.81171001118396,
129.179878900999));
#253046=CARTESIAN_POINT('Ctrl Pts',(153.473013635558,-5.04861812217248,
135.65717311965));
#253047=CARTESIAN_POINT('Ctrl Pts',(153.194566011745,1.3539071824088,137.674969721956));
#253048=CARTESIAN_POINT('Ctrl Pts',(152.916118387933,6.51225792839928,133.379012205241));
#253049=CARTESIAN_POINT('Ctrl Pts',(152.637670764119,5.68616177967723,126.717075658174));
#253050=CARTESIAN_POINT('Ctrl Pts',(152.359223140307,-0.365239260122265,
123.811154313817));
#253051=CARTESIAN_POINT('Ctrl Pts',(152.080775516494,-6.08100326279917,
127.331647925483));
#253052=CARTESIAN_POINT('Ctrl Pts',(151.802327892681,-6.20862234048841,
134.043394849727));
#253053=CARTESIAN_POINT('Ctrl Pts',(151.523880268868,-0.630820795332096,
137.778627550233));
#253054=CARTESIAN_POINT('Ctrl Pts',(151.245432645055,5.52667424342534,135.104849651499));
#253055=CARTESIAN_POINT('Ctrl Pts',(150.966985021242,6.60542564552152,128.479132421149));
#253056=CARTESIAN_POINT('Ctrl Pts',(150.688537397429,1.61411357236584,123.990186309594));
#253057=CARTESIAN_POINT('Ctrl Pts',(150.410089773616,-4.86049001996232,
125.763133496143));
#253058=CARTESIAN_POINT('Ctrl Pts',(150.131642149803,-6.8685407320831,132.168722129643));
#253059=CARTESIAN_POINT('Ctrl Pts',(149.853194525991,-2.56473805828847,
137.32052918631));
#253060=CARTESIAN_POINT('Ctrl Pts',(149.574746902178,4.09593359665354,136.484295660832));
#253061=CARTESIAN_POINT('Ctrl Pts',(149.296299278365,6.99264237375128,130.428479310845));
#253062=CARTESIAN_POINT('Ctrl Pts',(149.017851654552,3.46345441894284,124.718079518912));
#253063=CARTESIAN_POINT('Ctrl Pts',(148.739404030739,-3.24847894771935,
124.600674725279));
#253064=CARTESIAN_POINT('Ctrl Pts',(148.460956406926,-6.97521885844655,
130.184154199754));
#253065=CARTESIAN_POINT('Ctrl Pts',(148.182508783113,-4.29207339664657,
136.337573073429));
#253066=CARTESIAN_POINT('Ctrl Pts',(147.9040611593,2.33527783722936,137.406240012622));
#253067=CARTESIAN_POINT('Ctrl Pts',(147.625613535487,6.81662282335624,132.408102307496));
#253068=CARTESIAN_POINT('Ctrl Pts',(147.347165911675,5.03382444535687,125.936204336462));
#253069=CARTESIAN_POINT('Ctrl Pts',(147.068718287862,-1.37481268193005,
123.937904165105));
#253070=CARTESIAN_POINT('Ctrl Pts',(146.790270664049,-6.52006411785656,
128.249542028514));
#253071=CARTESIAN_POINT('Ctrl Pts',(146.511823040236,-5.67369515231286,
134.908933365434));
#253072=CARTESIAN_POINT('Ctrl Pts',(146.233375416423,0.386522482789046,
137.796422866589));
#253073=CARTESIAN_POINT('Ctrl Pts',(145.95492779261,6.09154483888081,134.258548742122));
#253074=CARTESIAN_POINT('Ctrl Pts',(145.676480168797,6.19873507655051,127.546444477659));
#253075=CARTESIAN_POINT('Ctrl Pts',(145.398032544984,0.609590603913882,
123.828205987717));
#253076=CARTESIAN_POINT('Ctrl Pts',(145.119584921171,-5.53973785356302,
126.520712798507));
#253077=CARTESIAN_POINT('Ctrl Pts',(144.841137297358,-6.59831785485502,
133.149682687181));
#253078=CARTESIAN_POINT('Ctrl Pts',(144.562689673546,-1.59336609328267,
137.623416169231));
#253079=CARTESIAN_POINT('Ctrl Pts',(144.284242049733,4.87581126775532,135.830770728684));
#253080=CARTESIAN_POINT('Ctrl Pts',(144.00579442592,6.86435627034879,129.419099949804));
#253081=CARTESIAN_POINT('Ctrl Pts',(143.727346802107,2.54489320293839,124.280416050852));
#253082=CARTESIAN_POINT('Ctrl Pts',(143.448899178294,-4.11320239302776,
125.136918496298));
#253083=CARTESIAN_POINT('Ctrl Pts',(143.170451554481,-6.99146593090932,
131.201523381251));
#253084=CARTESIAN_POINT('Ctrl Pts',(142.892003930668,-3.44491383038404,
136.901155088855));
#253085=CARTESIAN_POINT('Ctrl Pts',(142.613556306855,3.26734578686757,136.998130522314));
#253086=CARTESIAN_POINT('Ctrl Pts',(142.335108683042,6.97707424470332,131.403333995789));
#253087=CARTESIAN_POINT('Ctrl Pts',(142.05666105923,4.27521232068256,125.258110196154));
#253088=CARTESIAN_POINT('Ctrl Pts',(141.778213435417,-2.35536087031262,
124.209619584399));
#253089=CARTESIAN_POINT('Ctrl Pts',(141.499765811604,-6.8214724872659,129.221373811115));
#253090=CARTESIAN_POINT('Ctrl Pts',(141.221318187791,-5.01898413587917,
135.687815579753));
#253091=CARTESIAN_POINT('Ctrl Pts',(140.942870563978,1.39570544537436,137.666600808179));
#253092=CARTESIAN_POINT('Ctrl Pts',(140.664422940165,6.52780990633047,133.339322540502));
#253093=CARTESIAN_POINT('Ctrl Pts',(140.385975316352,5.66117596461176,126.68253810542));
#253094=CARTESIAN_POINT('Ctrl Pts',(140.10752769254,-0.407802124764288,
123.813507196776));
#253095=CARTESIAN_POINT('Ctrl Pts',(139.829080068726,-6.10202998372316,
127.368729059661));
#253096=CARTESIAN_POINT('Ctrl Pts',(139.550632444914,-6.18879038837768,
134.081128484328));
#253097=CARTESIAN_POINT('Ctrl Pts',(139.272184821101,-0.588354765331746,
137.78233831845));
#253098=CARTESIAN_POINT('Ctrl Pts',(138.993737197288,5.55275014432601,135.071127538621));
#253099=CARTESIAN_POINT('Ctrl Pts',(138.715289573475,6.59114893827324,128.438966401494));
#253100=CARTESIAN_POINT('Ctrl Pts',(138.436841949662,1.57260385347371,123.980486993006));
#253101=CARTESIAN_POINT('Ctrl Pts',(138.158394325849,-4.8910873466988,125.792814080728));
#253102=CARTESIAN_POINT('Ctrl Pts',(137.879946702036,-6.86010821815569,
132.210507608145));
#253103=CARTESIAN_POINT('Ctrl Pts',(137.601499078223,-2.52502477204539,
137.336020745319));
#253104=CARTESIAN_POINT('Ctrl Pts',(137.32305145441,4.13043308525698,136.459257314423));
#253105=CARTESIAN_POINT('Ctrl Pts',(137.044603830598,6.99022472008204,130.385920076178));
#253106=CARTESIAN_POINT('Ctrl Pts',(136.766156206785,3.42634132861412,124.69710925351));
#253107=CARTESIAN_POINT('Ctrl Pts',(136.487708582972,-3.28618235777073,
124.620564078594));
#253108=CARTESIAN_POINT('Ctrl Pts',(136.209260959159,-6.97886499629743,
130.226625827737));
#253109=CARTESIAN_POINT('Ctrl Pts',(135.930813335346,-4.25831163973555,
136.363597624819));
#253110=CARTESIAN_POINT('Ctrl Pts',(135.652365711533,2.37542208365453,137.391902196061));
#253111=CARTESIAN_POINT('Ctrl Pts',(135.37391808772,6.82625895798624,132.366577875963));
#253112=CARTESIAN_POINT('Ctrl Pts',(135.095470463907,5.00409733121823,125.905652213954));
#253113=CARTESIAN_POINT('Ctrl Pts',(134.817022840094,-1.4165852791943,123.946400259653));
#253114=CARTESIAN_POINT('Ctrl Pts',(134.538575216282,-6.53549522206528,
128.289278844285));
#253115=CARTESIAN_POINT('Ctrl Pts',(134.260127592469,-5.64860433254967,
134.943394709987));
#253116=CARTESIAN_POINT('Ctrl Pts',(133.981679968656,0.429077988916399,
137.793940447809));
#253117=CARTESIAN_POINT('Ctrl Pts',(133.703232344843,6.1124586001935,134.221403781595));
#253118=CARTESIAN_POINT('Ctrl Pts',(133.42478472103,6.17878836809604,127.508771379477));
#253119=CARTESIAN_POINT('Ctrl Pts',(133.146337097217,0.567113476311158,
123.824624488677));
#253120=CARTESIAN_POINT('Ctrl Pts',(132.867889473404,-5.5657109951702,126.554514121259));
#253121=CARTESIAN_POINT('Ctrl Pts',(132.589441849591,-6.58391896218814,
133.189805067404));
#253122=CARTESIAN_POINT('Ctrl Pts',(132.310994225778,-1.55182704527753,
137.632989099587));
#253123=CARTESIAN_POINT('Ctrl Pts',(132.032546601965,4.90631811527725,135.800997153839));
#253124=CARTESIAN_POINT('Ctrl Pts',(131.754098978153,6.85579661485726,129.377340330521));
#253125=CARTESIAN_POINT('Ctrl Pts',(131.47565135434,2.50513294966777,124.265045437181));
#253126=CARTESIAN_POINT('Ctrl Pts',(131.197203730527,-4.14762551371829,
125.162061731307));
#253127=CARTESIAN_POINT('Ctrl Pts',(130.918756106714,-6.98891875276791,
131.244075060281));
#253128=CARTESIAN_POINT('Ctrl Pts',(130.640308482901,-3.4077370856862,136.922012297644));
#253129=CARTESIAN_POINT('Ctrl Pts',(130.361860859088,3.30498848592948,136.978126504915));
#253130=CARTESIAN_POINT('Ctrl Pts',(130.083413235275,6.98059109663955,131.360851466943));
#253131=CARTESIAN_POINT('Ctrl Pts',(129.804965611462,4.24137151037132,125.232188524482));
#253132=CARTESIAN_POINT('Ctrl Pts',(129.526517987649,-2.39546129141071,
124.224079519825));
#253133=CARTESIAN_POINT('Ctrl Pts',(129.248070363836,-6.83098219117618,
129.262927379388));
#253134=CARTESIAN_POINT('Ctrl Pts',(128.969622740024,-4.98916416928312,
135.718277081636));
#253135=CARTESIAN_POINT('Ctrl Pts',(128.691175116211,1.43745198996158,137.657977611568));
#253136=CARTESIAN_POINT('Ctrl Pts',(128.412727492398,6.54311999386511,133.299538941816));
#253137=CARTESIAN_POINT('Ctrl Pts',(128.134279868585,5.63598037258881,126.648153288314));
#253138=CARTESIAN_POINT('Ctrl Pts',(127.855832244772,-0.450349878148651,
123.81611912838));
#253139=CARTESIAN_POINT('Ctrl Pts',(127.577384620959,-6.12283059168226,
127.40593750243));
#253140=CARTESIAN_POINT('Ctrl Pts',(127.298936997146,-6.16872910836309,
134.118740697091));
#253141=CARTESIAN_POINT('Ctrl Pts',(127.020489373333,-0.545866933628919,
137.785790515136));
#253142=CARTESIAN_POINT('Ctrl Pts',(126.742041749521,5.57862028602806,135.037247319125));
#253143=CARTESIAN_POINT('Ctrl Pts',(126.463594125708,6.57662799357718,128.398888032392));
#253144=CARTESIAN_POINT('Ctrl Pts',(126.185146501895,1.53103586116759,123.971040537565));
#253145=CARTESIAN_POINT('Ctrl Pts',(125.906698878082,-4.92150343239493,
125.822680370014));
#253146=CARTESIAN_POINT('Ctrl Pts',(125.628251254269,-6.85142150039552,
132.252240981353));
#253147=CARTESIAN_POINT('Ctrl Pts',(125.349803630456,-2.48521792008072,
137.351270271259));
#253148=CARTESIAN_POINT('Ctrl Pts',(125.071356006643,4.16477951914341,136.434009423738));
#253149=CARTESIAN_POINT('Ctrl Pts',(124.79290838283,6.98754804106521,130.343376346978));
#253150=CARTESIAN_POINT('Ctrl Pts',(124.514460759018,3.38910127394743,124.676365294554));
#253151=CARTESIAN_POINT('Ctrl Pts',(124.236013135205,-3.32376399712637,
124.640682574762));
#253152=CARTESIAN_POINT('Ctrl Pts',(123.957565511392,-6.98225252973936,
130.269118863895));
#253153=CARTESIAN_POINT('Ctrl Pts',(123.679117887579,-4.22439208952083,
136.389416176637));
#253154=CARTESIAN_POINT('Ctrl Pts',(123.400670263766,2.41547830794073,137.377320275725));
#253155=CARTESIAN_POINT('Ctrl Pts',(123.122222639953,6.83564214308024,132.324995555895));
#253156=CARTESIAN_POINT('Ctrl Pts',(122.84377501614,4.97418478841272,125.875281614887));
#253157=CARTESIAN_POINT('Ctrl Pts',(122.565327392328,-1.45830538437,123.955150478444));
#253158=CARTESIAN_POINT('Ctrl Pts',(122.286879768514,-6.55068415109515,
128.329108857337));
#253159=CARTESIAN_POINT('Ctrl Pts',(122.008432144702,-5.62330420167569,
134.977702681109));
#253160=CARTESIAN_POINT('Ctrl Pts',(121.729984520888,0.471617595401148,
137.791199027578));
#253161=CARTESIAN_POINT('Ctrl Pts',(121.451536897076,6.13314586210485,134.184132201278));
#253162=CARTESIAN_POINT('Ctrl Pts',(121.173089273263,6.15861270236637,127.471220400567));
#253163=CARTESIAN_POINT('Ctrl Pts',(120.89464164945,0.52461533410983,123.821301626325));
#253164=CARTESIAN_POINT('Ctrl Pts',(120.616194025637,-5.5914778973097,126.588472923636));
#253165=CARTESIAN_POINT('Ctrl Pts',(120.337746401824,-6.56927609998288,
133.229839054105));
#253166=CARTESIAN_POINT('Ctrl Pts',(120.059298778011,-1.51023049375061,
137.642308992603));
#253167=CARTESIAN_POINT('Ctrl Pts',(119.780851154198,4.93664315737715,135.77103842679));
#253168=CARTESIAN_POINT('Ctrl Pts',(119.502403530385,6.84698291530094,129.33563359));
#253169=CARTESIAN_POINT('Ctrl Pts',(119.223955906573,2.46527986777437,124.249917140239));
#253170=CARTESIAN_POINT('Ctrl Pts',(118.94550828276,-4.18189494262004,125.187414043775));
#253171=CARTESIAN_POINT('Ctrl Pts',(118.667060658947,-6.98611259767199,
131.28661044553));
#253172=CARTESIAN_POINT('Ctrl Pts',(118.388613035134,-3.37043406603744,
136.942642814599));
#253173=CARTESIAN_POINT('Ctrl Pts',(118.110165411321,3.34250871742766,136.95789371635));
#253174=CARTESIAN_POINT('Ctrl Pts',(117.831717787508,6.98384928020556,131.318348317123));
#253175=CARTESIAN_POINT('Ctrl Pts',(117.553270163695,4.20737353447909,125.206473331696));
#253176=CARTESIAN_POINT('Ctrl Pts',(117.274822539882,-2.43547294780967,
124.238783289987));
#253177=CARTESIAN_POINT('Ctrl Pts',(116.99637491607,-6.84023877052931,129.304538066038));
#253178=CARTESIAN_POINT('Ctrl Pts',(116.717927292256,-4.95915932737393,
135.748556496538));
#253179=CARTESIAN_POINT('Ctrl Pts',(116.439479668444,1.47914526923655,137.649100451659));
#253180=CARTESIAN_POINT('Ctrl Pts',(116.161032044631,6.55818762368211,133.259662883379));
#253181=CARTESIAN_POINT('Ctrl Pts',(115.882584420818,5.61057593724064,126.613922481));
#253182=CARTESIAN_POINT('Ctrl Pts',(115.604136797005,-0.49288094365267,
123.818990011842));
#253183=CARTESIAN_POINT('Ctrl Pts',(115.325689173192,-6.14340431590201,
127.443271875017));
#253184=CARTESIAN_POINT('Ctrl Pts',(115.047241549379,-6.14843924382291,
134.156230094282));
#253185=CARTESIAN_POINT('Ctrl Pts',(114.768793925566,-0.5033588746261,137.78898401237));
#253186=CARTESIAN_POINT('Ctrl Pts',(114.490346301753,5.60428370990391,135.003210248456));
#253187=CARTESIAN_POINT('Ctrl Pts',(114.211898677941,6.56186334951224,128.358898798961));
#253188=CARTESIAN_POINT('Ctrl Pts',(113.933451054127,1.48941113576461,123.961847293312));
#253189=CARTESIAN_POINT('Ctrl Pts',(113.655003430315,-4.95173714997151,
125.852731257293));
#253190=CARTESIAN_POINT('Ctrl Pts',(113.376555806502,-6.84248090069202,
132.293920702821));
#253191=CARTESIAN_POINT('Ctrl Pts',(113.098108182689,-2.4453189774521,137.366277199056));
#253192=CARTESIAN_POINT('Ctrl Pts',(112.819660558876,4.19897162559319,136.408552924347));
#253193=CARTESIAN_POINT('Ctrl Pts',(112.541212935063,6.98461243588604,130.300849699721));
#253194=CARTESIAN_POINT('Ctrl Pts',(112.26276531125,3.35173563488669,124.655848410718));
#253195=CARTESIAN_POINT('Ctrl Pts',(111.984317687437,-3.3612224731848,124.661029468288));
#253196=CARTESIAN_POINT('Ctrl Pts',(111.705870063624,-6.98538133324609,
130.311631733633));
#253197=CARTESIAN_POINT('Ctrl Pts',(111.427422439812,-4.1903160029037,136.415027772168));
#253198=CARTESIAN_POINT('Ctrl Pts',(111.148974815999,2.45544502578993,137.362494791951));
#253199=CARTESIAN_POINT('Ctrl Pts',(110.870527192186,6.84477203094083,132.28335688814));
#253200=CARTESIAN_POINT('Ctrl Pts',(110.592079568373,4.94408792536061,125.845093664656));
#253201=CARTESIAN_POINT('Ctrl Pts',(110.31363194456,-1.49997145150339,123.964154497236));
#253202=CARTESIAN_POINT('Ctrl Pts',(110.035184320747,-6.56563034211481,
128.369030591753));
#253203=CARTESIAN_POINT('Ctrl Pts',(109.756736696934,-5.59779569719655,
135.011856007506));
#253204=CARTESIAN_POINT('Ctrl Pts',(109.478289073121,0.514139725922464,
137.788198707481));
#253205=CARTESIAN_POINT('Ctrl Pts',(109.199841449309,6.15360585804082,134.146735382281));
#253206=CARTESIAN_POINT('Ctrl Pts',(108.921393825496,6.13820882697821,127.433792932393));
#253207=CARTESIAN_POINT('Ctrl Pts',(108.642946201683,0.482097752094529,
123.818237523792));
#253208=CARTESIAN_POINT('Ctrl Pts',(108.36449857787,-5.61703760517944,126.622587947283));
#253209=CARTESIAN_POINT('Ctrl Pts',(108.086050954057,-6.5543898108359,133.26978316381));
#253210=CARTESIAN_POINT('Ctrl Pts',(107.807603330244,-1.46857798007734,
137.651375502926));
#253211=CARTESIAN_POINT('Ctrl Pts',(107.529155706431,4.96678527034939,135.740895657668));
#253212=CARTESIAN_POINT('Ctrl Pts',(107.250708082618,6.83791549827476,129.2939812737));
#253213=CARTESIAN_POINT('Ctrl Pts',(106.972260458805,2.42533543402888,124.23503172061));
#253214=CARTESIAN_POINT('Ctrl Pts',(106.693812834992,-4.21600940986681,
125.212974494265));
#253215=CARTESIAN_POINT('Ctrl Pts',(106.415365211179,-6.98304756960462,
131.329127960835));
#253216=CARTESIAN_POINT('Ctrl Pts',(106.136917587367,-3.33300615371489,
136.96304587525));
#253217=CARTESIAN_POINT('Ctrl Pts',(105.858469963554,3.37990509103613,136.937432906355));
#253218=CARTESIAN_POINT('Ctrl Pts',(105.580022339741,6.98684867466819,131.275826121299));
#253219=CARTESIAN_POINT('Ctrl Pts',(105.301574715928,4.1732196528133,125.180965570684));
#253220=CARTESIAN_POINT('Ctrl Pts',(105.023127092115,-2.4753943568629,124.253730350031));
#253221=CARTESIAN_POINT('Ctrl Pts',(104.744679468302,-6.84924188231931,
129.346204329164));
#253222=CARTESIAN_POINT('Ctrl Pts',(104.466231844489,-4.92897072199215,
135.778652702442));
#253223=CARTESIAN_POINT('Ctrl Pts',(104.187784220676,1.52078373823962,137.639969657397));
#253224=CARTESIAN_POINT('Ctrl Pts',(103.909336596864,6.57301223744494,133.219695842813));
#253225=CARTESIAN_POINT('Ctrl Pts',(103.63088897305,5.58496359993783,126.579846951912));
#253226=CARTESIAN_POINT('Ctrl Pts',(103.352441349238,-0.535393745272065,
123.82211974078));
#253227=CARTESIAN_POINT('Ctrl Pts',(103.073993725425,-6.1637503940156,127.480730793984));
#253228=CARTESIAN_POINT('Ctrl Pts',(102.795546101612,-6.12792154660547,
134.193595286717));
#253229=CARTESIAN_POINT('Ctrl Pts',(102.517098477799,-0.460832163475232,
137.791918691816));
#253230=CARTESIAN_POINT('Ctrl Pts',(102.238650853986,5.6297394649859,134.96901758787));
#253231=CARTESIAN_POINT('Ctrl Pts',(101.960203230173,6.54685555318778,128.319000183017));
#253232=CARTESIAN_POINT('Ctrl Pts',(101.68175560636,1.44773121968427,123.952907600908));
#253233=CARTESIAN_POINT('Ctrl Pts',(101.403307982548,-4.981787379107,125.882965629019));
#253234=CARTESIAN_POINT('Ctrl Pts',(101.124860358735,-6.83328675034245,
132.335545228093));
#253235=CARTESIAN_POINT('Ctrl Pts',(100.846412734922,-2.4053294226295,137.38104097262));
#253236=CARTESIAN_POINT('Ctrl Pts',(100.567965111109,4.23300813760519,136.382888759548));
#253237=CARTESIAN_POINT('Ctrl Pts',(100.289517487296,6.98141801332452,130.258341710245));
#253238=CARTESIAN_POINT('Ctrl Pts',(100.011069863483,3.31424579602927,124.635559362262));
#253239=CARTESIAN_POINT('Ctrl Pts',(99.7326222396699,-3.39855639790849,
124.681604005209));
#253240=CARTESIAN_POINT('Ctrl Pts',(99.4541746158571,-6.98825129087862,
130.354162861621));
#253241=CARTESIAN_POINT('Ctrl Pts',(99.1757269920442,-4.15608464258612,
136.440431462363));
#253242=CARTESIAN_POINT('Ctrl Pts',(98.8972793682313,2.49532075622072,137.347426294104));
#253243=CARTESIAN_POINT('Ctrl Pts',(98.6188317444184,6.85364828325664,132.241663415635));
#253244=CARTESIAN_POINT('Ctrl Pts',(98.3403841206056,4.91380785731226,125.815089481885));
#253245=CARTESIAN_POINT('Ctrl Pts',(98.0619364967926,-1.54158193664305,
123.97341198238));
#253246=CARTESIAN_POINT('Ctrl Pts',(97.7834888729798,-6.58033324128762,
128.409042568218));
#253247=CARTESIAN_POINT('Ctrl Pts',(97.5050412491668,-5.57207976433927,
135.045853423614));
#253248=CARTESIAN_POINT('Ctrl Pts',(97.226593625354,0.55664280480716,137.784939598694));
#253249=CARTESIAN_POINT('Ctrl Pts',(96.948146001541,6.17383782984873,134.109214710358));
#253250=CARTESIAN_POINT('Ctrl Pts',(96.6696983777281,6.11757749800464,127.396490361844));
#253251=CARTESIAN_POINT('Ctrl Pts',(96.3912507539153,0.43956230576973,123.815432294619));
#253252=CARTESIAN_POINT('Ctrl Pts',(96.1128031301024,-5.64238917165504,
126.656857928054));
#253253=CARTESIAN_POINT('Ctrl Pts',(95.8343555062895,-6.53926064636413,
133.309635916377));
#253254=CARTESIAN_POINT('Ctrl Pts',(95.5559078824767,-1.42687104770695,
137.660188294596));
#253255=CARTESIAN_POINT('Ctrl Pts',(95.2774602586637,4.99674333726689,135.710569963425));
#253256=CARTESIAN_POINT('Ctrl Pts',(94.9990126348508,6.82859469977515,129.252384925061));
#253257=CARTESIAN_POINT('Ctrl Pts',(94.720565011038,2.38530112858694,124.22038972988));
#253258=CARTESIAN_POINT('Ctrl Pts',(94.442117387225,-4.24996765133445,125.238742135624));
#253259=CARTESIAN_POINT('Ctrl Pts',(94.1636697634123,-6.97972378214161,
131.371626030693));
#253260=CARTESIAN_POINT('Ctrl Pts',(93.885222139599,-3.29545473562348,136.983220723554));
#253261=CARTESIAN_POINT('Ctrl Pts',(93.6067745157866,3.41717622101856,136.91674483311));
#253262=CARTESIAN_POINT('Ctrl Pts',(93.3283268919733,6.98958916888377,131.233286455149));
#253263=CARTESIAN_POINT('Ctrl Pts',(93.0498792681607,4.13891113095855,125.155666186642));
#253264=CARTESIAN_POINT('Ctrl Pts',(92.7714316443476,-2.51522403926791,
124.268920146089));
#253265=CARTESIAN_POINT('Ctrl Pts',(92.4929840205349,-6.85799119293255,
129.387924624807));
#253266=CARTESIAN_POINT('Ctrl Pts',(92.2145363967218,-4.89859947178764,
135.808564584124));
#253267=CARTESIAN_POINT('Ctrl Pts',(91.9360887729091,1.562365854042,137.63058556713));
#253268=CARTESIAN_POINT('Ctrl Pts',(91.6576411490961,6.58759328582208,133.179639301113));
#253269=CARTESIAN_POINT('Ctrl Pts',(91.3791935252832,5.55914430975498,126.545927963732));
#253270=CARTESIAN_POINT('Ctrl Pts',(91.1007459014705,-0.57788670767935,
123.825508199223));
#253271=CARTESIAN_POINT('Ctrl Pts',(90.8222982776573,-6.18386807209161,
127.518312871276));
#253272=CARTESIAN_POINT('Ctrl Pts',(90.5438506538447,-6.10717677700159,
134.230834889814));
#253273=CARTESIAN_POINT('Ctrl Pts',(90.2654030300316,-0.41828837601907,
137.794594444728));
#253274=CARTESIAN_POINT('Ctrl Pts',(89.9869554062187,5.65498660800168,134.934670604388));
#253275=CARTESIAN_POINT('Ctrl Pts',(89.708507782406,6.53160516072318,128.279193663018));
#253276=CARTESIAN_POINT('Ctrl Pts',(89.430060158593,1.40599765739116,123.944221791613));
#253277=CARTESIAN_POINT('Ctrl Pts',(89.1516125347801,-5.01165300627911,
125.913382364846));
#253278=CARTESIAN_POINT('Ctrl Pts',(88.8731649109673,-6.82383939003939,
132.377113014756));
#253279=CARTESIAN_POINT('Ctrl Pts',(88.5947172871542,-2.36525073744058,
137.395561044874));
#253280=CARTESIAN_POINT('Ctrl Pts',(88.3162696633415,4.26688779394398,136.357017880338));
#253281=CARTESIAN_POINT('Ctrl Pts',(88.0378220395285,6.97796489175107,130.2158539537));
#253282=CARTESIAN_POINT('Ctrl Pts',(87.7593744157156,3.2766331465752,124.615498901007));
#253283=CARTESIAN_POINT('Ctrl Pts',(87.4809267919028,-3.43576438787495,
124.702405423128));
#253284=CARTESIAN_POINT('Ctrl Pts',(87.2024791680898,-6.99086229628967,
130.396710671853));
#253285=CARTESIAN_POINT('Ctrl Pts',(86.924031544277,-4.1216992770237,136.465626305881));
#253286=CARTESIAN_POINT('Ctrl Pts',(86.6455839204641,2.53510402162323,137.332115340552));
#253287=CARTESIAN_POINT('Ctrl Pts',(86.3671362966513,6.8622705711149,132.199916683345));
#253288=CARTESIAN_POINT('Ctrl Pts',(86.0886886728382,4.88334570630671,125.785270178391));
#253289=CARTESIAN_POINT('Ctrl Pts',(85.8102410490255,-1.58313529789712,
123.982922590838));
#253290=CARTESIAN_POINT('Ctrl Pts',(85.5317934252125,-6.59479230379227,
128.449143304076));
#253291=CARTESIAN_POINT('Ctrl Pts',(85.2533458013996,-5.5461573560172,135.079693669646));
#253292=CARTESIAN_POINT('Ctrl Pts',(84.9748981775869,0.599125257088023,
137.781421821987));
#253293=CARTESIAN_POINT('Ctrl Pts',(84.6964505537737,6.19384102782544,134.071571575853));
#253294=CARTESIAN_POINT('Ctrl Pts',(84.418002929961,6.09671947994716,127.359314071181));
#253295=CARTESIAN_POINT('Ctrl Pts',(84.1395553061481,0.397010571302045,
123.812886042756));
#253296=CARTESIAN_POINT('Ctrl Pts',(83.8611076823352,-5.66753165732491,
126.691281596061));
#253297=CARTESIAN_POINT('Ctrl Pts',(83.5826600585222,-6.52388916718428,
133.349395835046));
#253298=CARTESIAN_POINT('Ctrl Pts',(83.3042124347095,-1.38511124210516,
137.66874704105));
#253299=CARTESIAN_POINT('Ctrl Pts',(83.0257648108964,5.02651624802251,135.68006246779));
#253300=CARTESIAN_POINT('Ctrl Pts',(82.7473171870836,6.81902086518772,129.210846085452));
#253301=CARTESIAN_POINT('Ctrl Pts',(82.4688695632707,2.34517843493451,124.205991710613));
#253302=CARTESIAN_POINT('Ctrl Pts',(82.1904219394578,-4.28376840868787,
125.264716013022));
#253303=CARTESIAN_POINT('Ctrl Pts',(81.9119743156449,-6.97614135844701,
131.414103080323));
#253304=CARTESIAN_POINT('Ctrl Pts',(81.6335266918322,-3.25778120324508,
137.003166611925));
#253305=CARTESIAN_POINT('Ctrl Pts',(81.355079068019,3.45432072627939,136.895830263219));
#253306=CARTESIAN_POINT('Ctrl Pts',(81.0766314442065,6.99207066130227,131.190730894994));
#253307=CARTESIAN_POINT('Ctrl Pts',(80.7981838203932,4.10444924022979,125.130576117049));
#253308=CARTESIAN_POINT('Ctrl Pts',(80.5197361965806,-2.55496051912119,
124.284352115297));
#253309=CARTESIAN_POINT('Ctrl Pts',(80.2412885727675,-6.86648637816013,
129.429697407007));
#253310=CARTESIAN_POINT('Ctrl Pts',(79.9628409489547,-4.86804670217826,
135.838291033188));
#253311=CARTESIAN_POINT('Ctrl Pts',(79.6843933251418,1.6038900758031,137.620948528586));
#253312=CARTESIAN_POINT('Ctrl Pts',(79.405945701329,6.60193022850756,133.139494742587));
#253313=CARTESIAN_POINT('Ctrl Pts',(79.1274980775159,5.53311902343524,126.512166773338));
#253314=CARTESIAN_POINT('Ctrl Pts',(78.8490504537032,-0.620358256282274,
123.829155261608));
#253315=CARTESIAN_POINT('Ctrl Pts',(78.5706028298902,-6.2037566046621,127.556016714277));
#253316=CARTESIAN_POINT('Ctrl Pts',(78.2921552060774,-6.08620570371632,
134.267947523646));
#253317=CARTESIAN_POINT('Ctrl Pts',(78.0137075822645,-0.375729088733312,
137.797011171955));
#253318=CARTESIAN_POINT('Ctrl Pts',(77.7352599584516,5.68002420340909,134.90017057075));
#253319=CARTESIAN_POINT('Ctrl Pts',(77.4568123346387,6.51611273722737,128.23948071401));
#253320=CARTESIAN_POINT('Ctrl Pts',(77.1783647108257,1.36421199533782,123.935790187287));
#253321=CARTESIAN_POINT('Ctrl Pts',(76.8999170870129,-5.04133292480603,
125.94398033767));
#253322=CARTESIAN_POINT('Ctrl Pts',(76.6214694632,-6.81413916985829,132.418622522501));
#253323=CARTESIAN_POINT('Ctrl Pts',(76.3430218393871,-2.32508440701577,
137.409836877774));
#253324=CARTESIAN_POINT('Ctrl Pts',(76.0645742155741,4.30060933918641,136.33094124537));
#253325=CARTESIAN_POINT('Ctrl Pts',(75.7861265917614,6.97425319912241,130.173388004487));
#253326=CARTESIAN_POINT('Ctrl Pts',(75.5076789679483,3.23889908027492,124.595667770297));
#253327=CARTESIAN_POINT('Ctrl Pts',(75.2292313441357,-3.47284506432852,
124.72343295124));
#253328=CARTESIAN_POINT('Ctrl Pts',(74.9507837203226,-6.99321425272744,
130.439273587703));
#253329=CARTESIAN_POINT('Ctrl Pts',(74.6723360965098,-4.08716118037883,
136.490611369118));
#253330=CARTESIAN_POINT('Ctrl Pts',(74.3938884726969,2.57479334781394,137.316562498648));
#253331=CARTESIAN_POINT('Ctrl Pts',(74.1154408488841,6.87063857501356,132.158118238212));
#253332=CARTESIAN_POINT('Ctrl Pts',(73.836993225071,4.85270260113016,125.755636859138));
#253333=CARTESIAN_POINT('Ctrl Pts',(73.5585456012583,-1.62462999549052,
123.992685970191));
#253334=CARTESIAN_POINT('Ctrl Pts',(73.2800979774453,-6.60900699384299,
128.489331313375));
#253335=CARTESIAN_POINT('Ctrl Pts',(73.0016503536324,-5.52002943279461,
135.113375491641));
#253336=CARTESIAN_POINT('Ctrl Pts',(72.7232027298196,0.641585508562261,
137.777645507711));
#253337=CARTESIAN_POINT('Ctrl Pts',(72.4447551060067,6.21361471074508,134.033807373642));
#253338=CARTESIAN_POINT('Ctrl Pts',(72.1663074821937,6.07563554570727,127.322265437984));
#253339=CARTESIAN_POINT('Ctrl Pts',(71.8878598583809,0.354444125461637,
123.810598862555));
#253340=CARTESIAN_POINT('Ctrl Pts',(71.609412234568,-5.69246413052499,126.725857675724));
#253341=CARTESIAN_POINT('Ctrl Pts',(71.330964610755,-6.5082759428922,133.3890614465));
#253342=CARTESIAN_POINT('Ctrl Pts',(71.0525169869423,-1.34330011069692,
137.677051425141));
#253343=CARTESIAN_POINT('Ctrl Pts',(70.7740693631292,5.05610289937005,135.649374301231));
#253344=CARTESIAN_POINT('Ctrl Pts',(70.4956217393166,6.80919434927445,129.16936629411));
#253345=CARTESIAN_POINT('Ctrl Pts',(70.2171741155033,2.30496883983272,124.191838196331));
#253346=CARTESIAN_POINT('Ctrl Pts',(69.9387264916908,-4.31741042942741,
125.290895163988));
#253347=CARTESIAN_POINT('Ctrl Pts',(69.6602788678776,-6.97230043126892,
131.456557535721));
#253348=CARTESIAN_POINT('Ctrl Pts',(69.3818312440649,-3.21998695258627,
137.02288280126));
#253349=CARTESIAN_POINT('Ctrl Pts',(69.1033836202519,3.49133723041524,136.874689971681));
#253350=CARTESIAN_POINT('Ctrl Pts',(68.8249359964391,6.9942930599711,131.148161017746));
#253351=CARTESIAN_POINT('Ctrl Pts',(68.5464883726262,4.0698352576252,125.105696291628));
#253352=CARTESIAN_POINT('Ctrl Pts',(68.2680407488133,-2.59460232397255,
124.300025685817));
#253353=CARTESIAN_POINT('Ctrl Pts',(67.9895931250004,-6.87472712320984,
129.471521127857));
#253354=CARTESIAN_POINT('Ctrl Pts',(67.7111455011875,-4.83731354530826,
135.867830948109));
#253355=CARTESIAN_POINT('Ctrl Pts',(67.4326978773747,1.64535486482719,137.61105889887));
#253356=CARTESIAN_POINT('Ctrl Pts',(67.1542502535617,6.61602253424027,133.099263654809));
#253357=CARTESIAN_POINT('Ctrl Pts',(66.8758026297489,5.50688870535577,126.478564631767));
#253358=CARTESIAN_POINT('Ctrl Pts',(66.5973550059358,-0.662806817281494,
123.833060792792));
#253359=CARTESIAN_POINT('Ctrl Pts',(66.3189073821232,-6.22341525475008,
127.593840925854));
#253360=CARTESIAN_POINT('Ctrl Pts',(66.0404597583101,-6.0650091038406,134.304931812993));
#253361=CARTESIAN_POINT('Ctrl Pts',(65.7620121344974,-0.333155878668442,
137.799168783944));
#253362=CARTESIAN_POINT('Ctrl Pts',(65.4835645106842,5.70485132343066,134.865518765369));
#253363=CARTESIAN_POINT('Ctrl Pts',(65.2051168868716,6.50037885677781,128.199862807569));
#253364=CARTESIAN_POINT('Ctrl Pts',(64.9266692630585,1.32237578190785,123.927613100363));
#253365=CARTESIAN_POINT('Ctrl Pts',(64.6482216392459,-5.07082603488719,
125.974758413674));
#253366=CARTESIAN_POINT('Ctrl Pts',(64.3697740154327,-6.80418644924447,
132.460072213177));
#253367=CARTESIAN_POINT('Ctrl Pts',(64.09132639162,-2.28483191973344,137.423867942321));
#253368=CARTESIAN_POINT('Ctrl Pts',(63.812878767807,4.33417152376786,136.304659820925));
#253369=CARTESIAN_POINT('Ctrl Pts',(63.5344311439942,6.97028307297671,130.130945436197));
#253370=CARTESIAN_POINT('Ctrl Pts',(63.2559835201813,3.20104499537862,124.576066704985));
#253371=CARTESIAN_POINT('Ctrl Pts',(62.9775358963684,-3.5097970532309,124.744685810362));
#253372=CARTESIAN_POINT('Ctrl Pts',(62.6990882725555,-6.9953070730393,130.481850031987));
#253373=CARTESIAN_POINT('Ctrl Pts',(62.4206406487427,-4.05247163247362,
136.51538572624));
#253374=CARTESIAN_POINT('Ctrl Pts',(62.1421930249296,2.61438726408988,137.300768344709));
#253375=CARTESIAN_POINT('Ctrl Pts',(61.8637454011169,6.87875198487314,132.116269629093));
#253376=CARTESIAN_POINT('Ctrl Pts',(61.5852977773038,4.82187967727427,125.726190622201));
#253377=CARTESIAN_POINT('Ctrl Pts',(61.3068501534911,-1.66606449182178,
124.002701758653));
#253378=CARTESIAN_POINT('Ctrl Pts',(61.0284025296781,-6.62297678470872,
128.529605106938));
#253379=CARTESIAN_POINT('Ctrl Pts',(60.7499549058653,-5.49369696285183,
135.146897641504));
#253380=CARTESIAN_POINT('Ctrl Pts',(60.4715072820523,0.684021985849089,
137.773610795799));
#253381=CARTESIAN_POINT('Ctrl Pts',(60.1930596582395,6.23315814588628,133.995923503096));
#253382=CARTESIAN_POINT('Ctrl Pts',(59.9146120344266,6.05432647655821,127.285345835106));
#253383=CARTESIAN_POINT('Ctrl Pts',(59.6361644106137,0.311864545564345,
123.808570838767));
#253384=CARTESIAN_POINT('Ctrl Pts',(59.3577167868007,-5.71718566737322,
126.760584885814));
#253385=CARTESIAN_POINT('Ctrl Pts',(59.0792691629879,-6.49242155204172,
133.428631280914));
#253386=CARTESIAN_POINT('Ctrl Pts',(58.800821539175,-1.30143920280946,137.685101139145));
#253387=CARTESIAN_POINT('Ctrl Pts',(58.5223739153621,5.08550219496502,135.618506600908));
#253388=CARTESIAN_POINT('Ctrl Pts',(58.2439262915492,6.79911551616065,129.127947088084));
#253389=CARTESIAN_POINT('Ctrl Pts',(57.9654786677363,2.26467383326308,124.1779297115));
#253390=CARTESIAN_POINT('Ctrl Pts',(57.6870310439234,-4.35089246693584,
125.317278618444));
#253391=CARTESIAN_POINT('Ctrl Pts',(57.4085834201106,-6.96820114293417,
131.498987823723));
#253392=CARTESIAN_POINT('Ctrl Pts',(57.1301357962976,-3.18207338412696,
137.042368560968));
#253393=CARTESIAN_POINT('Ctrl Pts',(56.8516881724848,3.52822436176609,136.853324741857));
#253394=CARTESIAN_POINT('Ctrl Pts',(56.5732405486719,6.9962562825383,131.105578400848));
#253395=CARTESIAN_POINT('Ctrl Pts',(56.294792924859,4.03507046577855,125.081027632309));
#253396=CARTESIAN_POINT('Ctrl Pts',(56.0163453010462,-2.63414798488075,
124.315940276861));
#253397=CARTESIAN_POINT('Ctrl Pts',(55.7378976772331,-6.8827131227178,129.513394237565));
#253398=CARTESIAN_POINT('Ctrl Pts',(55.4594500534204,-4.80640114000575,
135.897183234276));
#253399=CARTESIAN_POINT('Ctrl Pts',(55.1810024296073,1.68675868462211,137.600917044446));
#253400=CARTESIAN_POINT('Ctrl Pts',(54.9025548057946,6.62986968082513,133.058947528554));
#253401=CARTESIAN_POINT('Ctrl Pts',(54.6241071819816,5.4804543274898,126.445122784157));
#253402=CARTESIAN_POINT('Ctrl Pts',(54.3456595581689,-0.705230817730614,
123.837224648055));
#253403=CARTESIAN_POINT('Ctrl Pts',(54.0672119343557,-6.24284329389726,
127.63178410442));
#253404=CARTESIAN_POINT('Ctrl Pts',(53.7887643105431,-6.04358776282204,
134.341786387386));
#253405=CARTESIAN_POINT('Ctrl Pts',(53.51031668673,-0.290570323389535,137.801067200743));
#253406=CARTESIAN_POINT('Ctrl Pts',(53.2318690629172,5.72946704808866,134.830716472279));
#253407=CARTESIAN_POINT('Ctrl Pts',(52.9534214391043,6.48440410239917,128.160341411752));
#253408=CARTESIAN_POINT('Ctrl Pts',(52.6749738152913,1.28049056735643,123.919690833848));
#253409=CARTESIAN_POINT('Ctrl Pts',(52.3965261914786,-5.10013124364513,
126.005715452363));
#253410=CARTESIAN_POINT('Ctrl Pts',(52.1180785676656,-6.79398159699943,
132.501460550851));
#253411=CARTESIAN_POINT('Ctrl Pts',(51.8396309438527,-2.24449476716385,
137.43765371859));
#253412=CARTESIAN_POINT('Ctrl Pts',(51.5611833200399,4.36757310402998,136.278174580871));
#253413=CARTESIAN_POINT('Ctrl Pts',(51.2827356962269,6.96605466042841,130.088527821552));
#253414=CARTESIAN_POINT('Ctrl Pts',(51.0042880724141,3.16307229458231,124.556696431394));
#253415=CARTESIAN_POINT('Ctrl Pts',(50.7258404486012,-3.54661898531293,
124.766163212963));
#253416=CARTESIAN_POINT('Ctrl Pts',(50.4473928247883,-6.99714067967511,
130.52443842702));
#253417=CARTESIAN_POINT('Ctrl Pts',(50.1689452009753,-4.0176319187415,136.539948459229));
#253418=CARTESIAN_POINT('Ctrl Pts',(49.8904975771625,2.65388430328469,137.284733463992));
#253419=CARTESIAN_POINT('Ctrl Pts',(49.6120499533496,6.88661050004828,132.074372406703));
#253420=CARTESIAN_POINT('Ctrl Pts',(49.3336023295367,4.79087807689359,125.696932558722));
#253421=CARTESIAN_POINT('Ctrl Pts',(49.0551547057238,-1.7074372515208,124.012969585086));
#253422=CARTESIAN_POINT('Ctrl Pts',(48.776707081911,-6.63670115873435,128.569963192402));
#253423=CARTESIAN_POINT('Ctrl Pts',(48.498259458098,-5.46716092194746,135.180258877061));
#253424=CARTESIAN_POINT('Ctrl Pts',(48.2198118342852,0.72643311645002,137.769317835757));
#253425=CARTESIAN_POINT('Ctrl Pts',(47.9413642104722,6.25247060906043,133.957921368012));
#253426=CARTESIAN_POINT('Ctrl Pts',(47.6629165866595,6.03279306211481,127.248556630613));
#253427=CARTESIAN_POINT('Ctrl Pts',(47.3844689628464,0.269273409411107,
123.806802046542));
#253428=CARTESIAN_POINT('Ctrl Pts',(47.1060213390337,-5.74169535180415,
126.7954619395));
#253429=CARTESIAN_POINT('Ctrl Pts',(46.8275737152206,-6.47632658212296,
133.468103872012));
#253430=CARTESIAN_POINT('Ctrl Pts',(46.5491260914079,-1.25953006961336,
137.69289588478));
#253431=CARTESIAN_POINT('Ctrl Pts',(46.2706784675948,5.11471304540623,135.587460510634));
#253432=CARTESIAN_POINT('Ctrl Pts',(45.9922308437821,6.78878473932087,129.086590002178));
#253433=CARTESIAN_POINT('Ctrl Pts',(45.7137832199691,2.22429490837156,124.164266771503));
#253434=CARTESIAN_POINT('Ctrl Pts',(45.4353355961562,-4.38421328052394,
125.343865398741));
#253435=CARTESIAN_POINT('Ctrl Pts',(45.1568879723434,-6.96384364534361,
131.541392372057));
#253436=CARTESIAN_POINT('Ctrl Pts',(44.8784403485304,-3.1440419027679,137.061623168999));
#253437=CARTESIAN_POINT('Ctrl Pts',(44.5999927247176,3.56498075346585,136.831735365442));
#253438=CARTESIAN_POINT('Ctrl Pts',(44.3215451009046,6.99796025625624,131.062984622213));
#253439=CARTESIAN_POINT('Ctrl Pts',(44.0430974770918,4.00015615291162,125.056571053198));
#253440=CARTESIAN_POINT('Ctrl Pts',(43.7646498532789,-2.67359603646683,
124.332095298706));
#253441=CARTESIAN_POINT('Ctrl Pts',(43.486202229466,-6.8904440807599,129.555315184507));
#253442=CARTESIAN_POINT('Ctrl Pts',(43.2077546056531,-4.77531063174146,
135.926346804027));
#253443=CARTESIAN_POINT('Ctrl Pts',(42.9293069818402,1.72810000095366,137.590523341125));
#253444=CARTESIAN_POINT('Ctrl Pts',(42.6508593580274,6.64347115515083,133.018547857752));
#253445=CARTESIAN_POINT('Ctrl Pts',(42.3724117342144,5.4538168693733,126.411842469708));
#253446=CARTESIAN_POINT('Ctrl Pts',(42.0939641104015,-0.74762868559244,
123.841646673103));
#253447=CARTESIAN_POINT('Ctrl Pts',(41.8155164865887,-6.26204000219037,
127.669844843974));
#253448=CARTESIAN_POINT('Ctrl Pts',(41.5370688627757,-6.02194247443641,
134.378509881167));
#253449=CARTESIAN_POINT('Ctrl Pts',(41.2586212389629,-0.247974000920424,
137.802706352008));
#253450=CARTESIAN_POINT('Ctrl Pts',(40.9801736151499,5.75387046523817,134.795764981093));
#253451=CARTESIAN_POINT('Ctrl Pts',(40.7017259913371,6.46818906604193,128.120917991039));
#253452=CARTESIAN_POINT('Ctrl Pts',(40.4232783675241,1.23855790375582,123.912023681303));
#253453=CARTESIAN_POINT('Ctrl Pts',(40.1448307437113,-5.12924746516435,
126.036850306614));
#253454=CARTESIAN_POINT('Ctrl Pts',(39.8663831198984,-6.78352499126783,
132.542786001862));
#253455=CARTESIAN_POINT('Ctrl Pts',(39.5879354960856,-2.20407444401526,
137.451193695743));
#253456=CARTESIAN_POINT('Ctrl Pts',(39.3094878722726,4.40081284226458,136.251486506627));
#253457=CARTESIAN_POINT('Ctrl Pts',(39.0310402484598,6.96156811816289,130.046136732356));
#253458=CARTESIAN_POINT('Ctrl Pts',(38.7525926246468,3.12498238497894,124.537557667297));
#253459=CARTESIAN_POINT('Ctrl Pts',(38.474145000834,-3.58330949612422,124.78786436319));
#253460=CARTESIAN_POINT('Ctrl Pts',(38.195697377021,-6.9987150046898,130.567037194673));
#253461=CARTESIAN_POINT('Ctrl Pts',(37.9172497532082,-3.98264333018119,
136.564298657899));
#253462=CARTESIAN_POINT('Ctrl Pts',(37.6388021293952,2.69328300182069,137.268458450676));
#253463=CARTESIAN_POINT('Ctrl Pts',(37.3603545055824,6.89421382933879,132.032428123559));
#253464=CARTESIAN_POINT('Ctrl Pts',(37.0819068817695,4.7596989487639,125.667863752866));
#253465=CARTESIAN_POINT('Ctrl Pts',(36.8034592579566,-1.74874674150458,
124.02348906901));
#253466=CARTESIAN_POINT('Ctrl Pts',(36.5250116341437,-6.65017960735793,
128.610404074285));
#253467=CARTESIAN_POINT('Ctrl Pts',(36.2465640103308,-5.44042229338459,
135.213457962098));
#253468=CARTESIAN_POINT('Ctrl Pts',(35.968116386518,0.768817328804687,137.764766786667));
#253469=CARTESIAN_POINT('Ctrl Pts',(35.689668762705,6.27155138463682,133.919802376575));
#253470=CARTESIAN_POINT('Ctrl Pts',(35.4112211388921,6.01103610030595,127.211899187745));
#253471=CARTESIAN_POINT('Ctrl Pts',(35.1327735150793,0.226672295232647,
123.805292551423));
#253472=CARTESIAN_POINT('Ctrl Pts',(34.8543258912663,-5.76599227560232,
126.830487544402));
#253473=CARTESIAN_POINT('Ctrl Pts',(34.5758782674535,-6.45999162954105,
133.507477757125));
#253474=CARTESIAN_POINT('Ctrl Pts',(34.2974306436406,-1.21757426406734,
137.700435373207));
#253475=CARTESIAN_POINT('Ctrl Pts',(34.0189830198277,5.1437343682746,135.556237180835));
#253476=CARTESIAN_POINT('Ctrl Pts',(33.7405353960148,6.778202401566,129.045296568894));
#253477=CARTESIAN_POINT('Ctrl Pts',(33.4620877722019,2.18383356141425,124.150849882625));
#253478=CARTESIAN_POINT('Ctrl Pts',(33.1836401483891,-4.41737163547663,
125.370654519698));
#253479=CARTESIAN_POINT('Ctrl Pts',(32.9051925245761,-6.95922809996586,
131.58376960941));
#253480=CARTESIAN_POINT('Ctrl Pts',(32.6267449007632,-3.10589391777991,
137.080645911863));
#253481=CARTESIAN_POINT('Ctrl Pts',(32.3482972769504,3.60160504349277,136.80992264244));
#253482=CARTESIAN_POINT('Ctrl Pts',(32.0698496531375,6.99940491798352,131.020381260171));
#253483=CARTESIAN_POINT('Ctrl Pts',(31.7914020293246,3.96509361278713,125.032327460544));
#253484=CARTESIAN_POINT('Ctrl Pts',(31.5129544055117,-2.71294501696876,
124.348490152723));
#253485=CARTESIAN_POINT('Ctrl Pts',(31.2345067816988,-6.89791971086261,
129.597282415287));
#253486=CARTESIAN_POINT('Ctrl Pts',(30.9560591578859,-4.74404317258561,
135.955320576696));
#253487=CARTESIAN_POINT('Ctrl Pts',(30.677611534073,1.76937728190418,137.579878174048));
#253488=CARTESIAN_POINT('Ctrl Pts',(30.3991639102601,6.65682645320975,132.978066139427));
#253489=CARTESIAN_POINT('Ctrl Pts',(30.1207162864473,5.42697731806706,126.378724921634));
#253490=CARTESIAN_POINT('Ctrl Pts',(29.8422686626343,-0.789998849798377,
123.846326704078));
#253491=CARTESIAN_POINT('Ctrl Pts',(29.5638210388214,-6.28100466828836,
127.708021734164));
#253492=CARTESIAN_POINT('Ctrl Pts',(29.2853734150086,-6.00007404075783,
134.415100933532));
#253493=CARTESIAN_POINT('Ctrl Pts',(29.0069257911957,-0.205368489683527,
137.804086176998));
#253494=CARTESIAN_POINT('Ctrl Pts',(28.7284781673828,5.77806067060162,134.760665586949));
#253495=CARTESIAN_POINT('Ctrl Pts',(28.4500305435699,6.45173434856014,128.08159400628));
#253496=CARTESIAN_POINT('Ctrl Pts',(28.171582919757,1.19657934493693,123.904611926838));
#253497=CARTESIAN_POINT('Ctrl Pts',(27.8931352959441,-5.15817362053239,
126.068161822712));
#253498=CARTESIAN_POINT('Ctrl Pts',(27.6146876721312,-6.77281701952304,
132.584047034882));
#253499=CARTESIAN_POINT('Ctrl Pts',(27.3362400483183,-2.16357244807759,
137.464487372053));
#253500=CARTESIAN_POINT('Ctrl Pts',(27.0577924245054,4.4338895067609,136.22459658713));
#253501=CARTESIAN_POINT('Ctrl Pts',(26.7793448006925,6.95682361243065,130.003773739425));
#253502=CARTESIAN_POINT('Ctrl Pts',(26.5008971768797,3.08677667800406,124.518651121888));
#253503=CARTESIAN_POINT('Ctrl Pts',(26.2224495530668,-3.61986722608435,
124.809788456898));
#253504=CARTESIAN_POINT('Ctrl Pts',(25.9440019292538,-7.00002998974624,
130.609644756432));
#253505=CARTESIAN_POINT('Ctrl Pts',(25.665554305441,-3.94750716330764,136.588435419948));
#253506=CARTESIAN_POINT('Ctrl Pts',(25.3871066816281,2.7325818997646,137.251943907838));
#253507=CARTESIAN_POINT('Ctrl Pts',(25.1086590578152,6.90156169100052,131.990438333922));
#253508=CARTESIAN_POINT('Ctrl Pts',(24.8302114340022,4.72834344823931,125.638985281792));
#253509=CARTESIAN_POINT('Ctrl Pts',(24.5517638101894,-1.78999143103474,
124.034259820624));
#253510=CARTESIAN_POINT('Ctrl Pts',(24.2733161863765,-6.66341163113055,
128.650926254035));
#253511=CARTESIAN_POINT('Ctrl Pts',(23.9948685625636,-5.41348206797292,
135.246493666413));
#253512=CARTESIAN_POINT('Ctrl Pts',(23.7164209387507,0.811173052350488,
137.759957817164));
#253513=CARTESIAN_POINT('Ctrl Pts',(23.4379733149379,6.29039976557031,133.881567941299));
#253514=CARTESIAN_POINT('Ctrl Pts',(23.159525691125,5.98905639734383,127.175374864857));
#253515=CARTESIAN_POINT('Ctrl Pts',(22.8810780673121,0.184062781628937,
123.804042409345));
#253516=CARTESIAN_POINT('Ctrl Pts',(22.6026304434992,-5.79007553843628,
126.865660402631));
#253517=CARTESIAN_POINT('Ctrl Pts',(22.3241828196863,-6.44341729959363,
133.546751477239));
#253518=CARTESIAN_POINT('Ctrl Pts',(22.0457351958734,-1.17557334085921,
137.707719325048));
#253519=CARTESIAN_POINT('Ctrl Pts',(21.7672875720605,5.17256508817436,135.524837768503));
#253520=CARTESIAN_POINT('Ctrl Pts',(21.4888399482477,6.76736889502847,129.004068318375));
#253521=CARTESIAN_POINT('Ctrl Pts',(21.2103923244347,2.14329129170119,124.137679542035));
#253522=CARTESIAN_POINT('Ctrl Pts',(20.9319447006219,-4.45036630309889,
125.397644988631));
#253523=CARTESIAN_POINT('Ctrl Pts',(20.6534970768089,-6.95435467783159,
131.626117965476));
#253524=CARTESIAN_POINT('Ctrl Pts',(20.3750494529961,-3.06763084275059,
137.099436084669));
#253525=CARTESIAN_POINT('Ctrl Pts',(20.0966018291831,3.6380958747203,136.787887381128));
#253526=CARTESIAN_POINT('Ctrl Pts',(19.8181542053702,7.00059021418742,130.977769893405));
#253527=CARTESIAN_POINT('Ctrl Pts',(19.5397065815574,3.92988414466092,125.0082977527));
#253528=CARTESIAN_POINT('Ctrl Pts',(19.2612589577445,-2.75219346829522,
124.365124231394));
#253529=CARTESIAN_POINT('Ctrl Pts',(18.9828113339316,-6.90513973601376,
129.639294374793));
#253530=CARTESIAN_POINT('Ctrl Pts',(18.7043637101187,-4.71259992116536,
135.98410347865));
#253531=CARTESIAN_POINT('Ctrl Pts',(18.4259160863058,1.81058899792882,137.568981937677));
#253532=CARTESIAN_POINT('Ctrl Pts',(18.1474684624929,6.6699350801164,132.937503873645));
#253533=CARTESIAN_POINT('Ctrl Pts',(17.86902083868,5.39993666812053,126.345771367118));
#253534=CARTESIAN_POINT('Ctrl Pts',(17.5905732148672,-0.832339740306418,
123.851264567558));
#253535=CARTESIAN_POINT('Ctrl Pts',(17.3121255910542,-6.29973658944851,
127.746313360329));
#253536=CARTESIAN_POINT('Ctrl Pts',(17.0336779672413,-5.97798327212915,
134.451558188587));
#253537=CARTESIAN_POINT('Ctrl Pts',(16.7552303434285,-0.162755368441711,
137.805206624583));
#253538=CARTESIAN_POINT('Ctrl Pts',(16.4767827196156,5.80203676780203,134.72541959047));
#253539=CARTESIAN_POINT('Ctrl Pts',(16.1983350958026,6.43504055968944,128.042370914639));
#253540=CARTESIAN_POINT('Ctrl Pts',(15.9198874719898,1.15455644643036,123.897455845098));
#253541=CARTESIAN_POINT('Ctrl Pts',(15.6414398481769,-5.18690863788001,
126.0996488404));
#253542=CARTESIAN_POINT('Ctrl Pts',(15.362992224364,-6.7618580785529,132.625242120967));
#253543=CARTESIAN_POINT('Ctrl Pts',(15.0845446005511,-2.12299028016722,
137.477534254917));
#253544=CARTESIAN_POINT('Ctrl Pts',(14.8060969767383,4.466801871851,136.197505818795));
#253545=CARTESIAN_POINT('Ctrl Pts',(14.5276493529253,6.95182131904109,129.961440412534));
#253546=CARTESIAN_POINT('Ctrl Pts',(14.2492017291125,3.04845658938423,124.499977495755));
#253547=CARTESIAN_POINT('Ctrl Pts',(13.9707541052995,-3.65629082053323,
124.831934681683));
#253548=CARTESIAN_POINT('Ctrl Pts',(13.6923064814867,-7.00108558611715,
130.652259533458));
#253549=CARTESIAN_POINT('Ctrl Pts',(13.4138588576738,-3.91222472010448,
136.612357850978));
#253550=CARTESIAN_POINT('Ctrl Pts',(13.1354112338608,2.77177954088132,137.23519044743));
#253551=CARTESIAN_POINT('Ctrl Pts',(12.856963610048,6.90865381275575,131.94840459374));
#253552=CARTESIAN_POINT('Ctrl Pts',(12.5785159862351,4.6968127372094,125.6102982156));
#253553=CARTESIAN_POINT('Ctrl Pts',(12.3000683624222,-1.83116979177416,
124.045281440813));
#253554=CARTESIAN_POINT('Ctrl Pts',(12.0216207386093,-6.67639673973472,
128.691528230086));
#253555=CARTESIAN_POINT('Ctrl Pts',(11.7431731147965,-5.38634124399241,
135.279364765853));
#253556=CARTESIAN_POINT('Ctrl Pts',(11.4647254909835,0.853498717580522,
137.75489110545));
#253557=CARTESIAN_POINT('Ctrl Pts',(11.1862778671706,6.30901505342741,133.843219478972));
#253558=CARTESIAN_POINT('Ctrl Pts',(10.9078302433578,5.96685476769427,127.13898501537));
#253559=CARTESIAN_POINT('Ctrl Pts',(10.6293826195448,0.141446447510913,
123.803051666633));
#253560=CARTESIAN_POINT('Ctrl Pts',(10.350934995732,-5.81394424789186,126.900979210845));
#253561=CARTESIAN_POINT('Ctrl Pts',(10.0724873719191,-6.42660420644864,
133.585923577051));
#253562=CARTESIAN_POINT('Ctrl Pts',(9.79403974810624,-1.1335288563486,137.714747470394));
#253563=CARTESIAN_POINT('Ctrl Pts',(9.51559212429333,5.20120413677258,135.493263437154));
#253564=CARTESIAN_POINT('Ctrl Pts',(9.23714450048043,6.75628462114785,128.962906778349));
#253565=CARTESIAN_POINT('Ctrl Pts',(8.95869687666756,2.10266960154115,124.124756237763));
#253566=CARTESIAN_POINT('Ctrl Pts',(8.68024925285465,-4.48319606076117,
125.4248358054));
#253567=CARTESIAN_POINT('Ctrl Pts',(8.40180162904178,-6.94922355952728,
131.66843587102));
#253568=CARTESIAN_POINT('Ctrl Pts',(8.12335400522884,-3.0292540955323,137.117992991138));
#253569=CARTESIAN_POINT('Ctrl Pts',(7.84490638141603,3.67445189496732,136.765630398031));
#253570=CARTESIAN_POINT('Ctrl Pts',(7.56645875760307,7.00151610094645,130.935152100895));
#253571=CARTESIAN_POINT('Ctrl Pts',(7.2880111337902,3.89452905323253,124.984482820099));
#253572=CARTESIAN_POINT('Ctrl Pts',(7.00956350997733,-2.79133993608059,
124.381996918337));
#253573=CARTESIAN_POINT('Ctrl Pts',(6.73111588616443,-6.91210388867261,
129.681349506257));
#253574=CARTESIAN_POINT('Ctrl Pts',(6.45266826235151,-4.68098204262199,
136.012694443327));
#253575=CARTESIAN_POINT('Ctrl Pts',(6.17422063853866,1.85173362191231,137.557835035774));
#253576=CARTESIAN_POINT('Ctrl Pts',(5.89577301472578,6.68279655012581,132.896862563455));
#253577=CARTESIAN_POINT('Ctrl Pts',(5.61732539091285,5.37269592153495,126.312983027266));
#253578=CARTESIAN_POINT('Ctrl Pts',(5.33887776709996,-0.874649788159289,
123.856460080569));
#253579=CARTESIAN_POINT('Ctrl Pts',(5.06043014328709,-6.31823507155263,
127.784718303561));
#253580=CARTESIAN_POINT('Ctrl Pts',(4.7819825194742,-5.95567098713191,134.487880295395));
#253581=CARTESIAN_POINT('Ctrl Pts',(4.50353489566127,-0.120136216239877,
137.806067653244));
#253582=CARTESIAN_POINT('Ctrl Pts',(4.22508727184843,5.82579786839633,134.690028297709));
#253583=CARTESIAN_POINT('Ctrl Pts',(3.94663964803551,6.41810831802433,128.003250169541));
#253584=CARTESIAN_POINT('Ctrl Pts',(3.66819202422262,1.11249076541009,123.890555701254));
#253585=CARTESIAN_POINT('Ctrl Pts',(3.3897444004097,-5.21545145242058,126.131310192911));
#253586=CARTESIAN_POINT('Ctrl Pts',(3.11129677659686,-6.75064857444498,
132.666369733619));
#253587=CARTESIAN_POINT('Ctrl Pts',(2.83284915278395,-2.08232944407128,
137.490333860877));
#253588=CARTESIAN_POINT('Ctrl Pts',(2.55440152897106,4.49954871795507,136.170215205482));
#253589=CARTESIAN_POINT('Ctrl Pts',(2.27595390515816,6.94656142335602,129.919138320362));
#253590=CARTESIAN_POINT('Ctrl Pts',(1.9975062813453,3.01002353908442,124.481537480858));
#253591=CARTESIAN_POINT('Ctrl Pts',(1.71905865753238,-3.69257892978116,
124.854302216906));
#253592=CARTESIAN_POINT('Ctrl Pts',(1.44061103371947,-7.00188175468703,
130.694879946647));
#253593=CARTESIAN_POINT('Ctrl Pts',(1.16216340990662,-3.87679730797559,
136.636065064534));
#253594=CARTESIAN_POINT('Ctrl Pts',(0.883715786093727,2.81087447268782,
137.218198690258));
#253595=CARTESIAN_POINT('Ctrl Pts',(0.605268162280799,6.91548993180329,
131.906328460586));
#253596=CARTESIAN_POINT('Ctrl Pts',(0.326820538467947,4.66510798405627,
125.5818036173));
#253597=CARTESIAN_POINT('Ctrl Pts',(0.0483729146550416,-1.87228029784353,
124.056553521165));
#253598=CARTESIAN_POINT('Ctrl Pts',(-0.23007470915786,-6.68913445200245,
128.732208497919));
#253599=CARTESIAN_POINT('Ctrl Pts',(-0.508522332970751,-5.35900082715629,
135.312070042369));
#253600=CARTESIAN_POINT('Ctrl Pts',(-0.786969956783612,0.895792756101716,
137.749566839272));
#253601=CARTESIAN_POINT('Ctrl Pts',(-1.06541758059653,6.32739655841135,
133.804758410613));
#253602=CARTESIAN_POINT('Ctrl Pts',(-1.34386520440944,5.94443203404716,
127.102730987725));
#253603=CARTESIAN_POINT('Ctrl Pts',(-1.62231282822229,0.0988248720430084,
123.802320359999));
#253604=CARTESIAN_POINT('Ctrl Pts',(-1.90076045203519,-5.83759751950527,
126.936442660293));
#253605=CARTESIAN_POINT('Ctrl Pts',(-2.17920807584809,-6.40955297312139,
133.624992605024));
#253606=CARTESIAN_POINT('Ctrl Pts',(-2.45765569966099,-1.09144236850938,
137.721519548813));
#253607=CARTESIAN_POINT('Ctrl Pts',(-2.73610332347384,5.22965045283876,
135.461515356786));
#253608=CARTESIAN_POINT('Ctrl Pts',(-3.01455094728676,6.74494999065597,
128.921813474073));
#253609=CARTESIAN_POINT('Ctrl Pts',(-3.29299857109967,2.06196999618574,
124.112080448687));
#253610=CARTESIAN_POINT('Ctrl Pts',(-3.57144619491253,-4.51585969194472,
125.452225962441));
#253611=CARTESIAN_POINT('Ctrl Pts',(-3.84989381872542,-6.94383493518842,
131.710721757939));
#253612=CARTESIAN_POINT('Ctrl Pts',(-4.12834144253832,-2.99076509818949,
137.136315943637));
#253613=CARTESIAN_POINT('Ctrl Pts',(-4.40678906635123,3.71067175704807,
136.743152517891));
#253614=CARTESIAN_POINT('Ctrl Pts',(-4.68523669016409,7.00218254395157,
130.892529461858));
#253615=CARTESIAN_POINT('Ctrl Pts',(-4.963684313977,3.85902964859785,124.960883545208));
#253616=CARTESIAN_POINT('Ctrl Pts',(-5.24213193778992,-2.83038296973812,
124.399107588329));
#253617=CARTESIAN_POINT('Ctrl Pts',(-5.52057956160276,-6.91881191077996,
129.723446251312));
#253618=CARTESIAN_POINT('Ctrl Pts',(-5.79902718541567,-4.6491907085676,
136.041092411279));
#253619=CARTESIAN_POINT('Ctrl Pts',(-6.07747480922856,1.89280962922548,
137.546437881394));
#253620=CARTESIAN_POINT('Ctrl Pts',(-6.35592243304147,6.69541038665145,
132.856143714835));
#253621=CARTESIAN_POINT('Ctrl Pts',(-6.63437005685431,5.34525608772619,
126.280361117063));
#253622=CARTESIAN_POINT('Ctrl Pts',(-6.91281768066725,-0.916927425542613,
123.86191305059));
#253623=CARTESIAN_POINT('Ctrl Pts',(-7.19126530448013,-6.33649942913263,
127.823235140749));
#253624=CARTESIAN_POINT('Ctrl Pts',(-7.469712928293,-5.93313801255607,134.524065908027));
#253625=CARTESIAN_POINT('Ctrl Pts',(-7.74816055210589,-0.0775126123463511,
137.806669231077));
#253626=CARTESIAN_POINT('Ctrl Pts',(-8.02660817591882,5.84934309190818,
134.654493020103));
#253627=CARTESIAN_POINT('Ctrl Pts',(-8.3050557997317,6.40093825099524,127.964233220621));
#253628=CARTESIAN_POINT('Ctrl Pts',(-8.58350342354456,1.07038386063539,
123.883911750995));
#253629=CARTESIAN_POINT('Ctrl Pts',(-8.86195104735747,-5.2438010064896,
126.163144707024));
#253630=CARTESIAN_POINT('Ctrl Pts',(-9.14039867117038,-6.73918892257159,
132.707428348838));
#253631=CARTESIAN_POINT('Ctrl Pts',(-9.41884629498326,-2.04159144649203,
137.50288571564));
#253632=CARTESIAN_POINT('Ctrl Pts',(-9.69729391879612,4.53212883162697,
136.142725758454));
#253633=CARTESIAN_POINT('Ctrl Pts',(-9.97574154260907,6.94104412028278,
129.876869030427));
#253634=CARTESIAN_POINT('Ctrl Pts',(-10.254189166422,2.97147895125515,124.463331760497));
#253635=CARTESIAN_POINT('Ctrl Pts',(-10.5326367902348,-3.72873020915888,
124.876890233732));
#253636=CARTESIAN_POINT('Ctrl Pts',(-10.8110844140478,-7.00241846595355,
130.737504416682));
#253637=CARTESIAN_POINT('Ctrl Pts',(-11.0895320378606,-3.84122623969676,
136.659556182137));
#253638=CARTESIAN_POINT('Ctrl Pts',(-11.3679796616735,2.84986524650705,
137.200969265957));
#253639=CARTESIAN_POINT('Ctrl Pts',(-11.6464272854864,6.92206979482823,
131.864211493609));
#253640=CARTESIAN_POINT('Ctrl Pts',(-11.9248749092993,4.6332303636112,125.553502542771));
#253641=CARTESIAN_POINT('Ctrl Pts',(-12.2033225331122,-1.91332142587795,
124.068075643991));
#253642=CARTESIAN_POINT('Ctrl Pts',(-12.4817701569251,-6.70162429593314,
128.77296555011));
#253643=CARTESIAN_POINT('Ctrl Pts',(-12.760217780738,-5.33146183057377,
135.344608284054));
#253644=CARTESIAN_POINT('Ctrl Pts',(-13.0386654045509,0.938053600692905,
137.743985215925));
#253645=CARTESIAN_POINT('Ctrl Pts',(-13.3171130283637,6.34554359938892,
133.766186161411));
#253646=CARTESIAN_POINT('Ctrl Pts',(-13.5955606521767,5.92178902728497,
127.066614125326));
#253647=CARTESIAN_POINT('Ctrl Pts',(-13.8740082759896,0.0561996345831295,
123.801848516541));
#253648=CARTESIAN_POINT('Ctrl Pts',(-14.1524558998025,-5.86103447679583,
126.972049436864));
#253649=CARTESIAN_POINT('Ctrl Pts',(-14.4309035236153,-6.39226423145161,
133.663957113442));
#253650=CARTESIAN_POINT('Ctrl Pts',(-14.7093511474282,-1.04931543687181,
137.728035309365));
#253651=CARTESIAN_POINT('Ctrl Pts',(-14.9877987712411,5.25790298228423,
135.429594703837));
#253652=CARTESIAN_POINT('Ctrl Pts',(-15.266246395054,6.73336542356173,128.880789928272));
#253653=CARTESIAN_POINT('Ctrl Pts',(-15.5446940188669,2.02119398377386,
124.099652644515));
#253654=CARTESIAN_POINT('Ctrl Pts',(-15.8231416426798,-4.54835598628669,
125.479814444798));
#253655=CARTESIAN_POINT('Ctrl Pts',(-16.1015892664927,-6.93818900449243,
131.752974059312));
#253656=CARTESIAN_POINT('Ctrl Pts',(-16.3800368903055,-2.95216527694612,
137.154404263204));
#253657=CARTESIAN_POINT('Ctrl Pts',(-16.6584845141185,3.74675411882228,
136.720454573632));
#253658=CARTESIAN_POINT('Ctrl Pts',(-16.9369321379314,7.00258951850748,
130.849903555692));
#253659=CARTESIAN_POINT('Ctrl Pts',(-17.2153797617442,3.82338724620039,
124.93750080251));
#253660=CARTESIAN_POINT('Ctrl Pts',(-17.4938273855571,-2.86932112251383,
124.416455607327));
#253661=CARTESIAN_POINT('Ctrl Pts',(-17.77227500937,-6.92526355376757,129.765583050046));
#253662=CARTESIAN_POINT('Ctrl Pts',(-18.0507226331829,-4.61722709704176,
136.069296330209));
#253663=CARTESIAN_POINT('Ctrl Pts',(-18.3291702569958,1.93381549778173,
137.534790896862));
#253664=CARTESIAN_POINT('Ctrl Pts',(-18.6076178808087,6.70777612228299,
132.81534883664));
#253665=CARTESIAN_POINT('Ctrl Pts',(-18.8860655046216,5.31761818348739,
126.247906845325));
#253666=CARTESIAN_POINT('Ctrl Pts',(-19.1645131284344,-0.959171085842972,
123.867623275557));
#253667=CARTESIAN_POINT('Ctrl Pts',(-19.4429607522474,-6.35452898539608,
127.861862444637));
#253668=CARTESIAN_POINT('Ctrl Pts',(-19.7214083760603,-5.91038518336925,
134.560113685611));
#253669=CARTESIAN_POINT('Ctrl Pts',(-19.9998559998732,-0.0348861361944895,
137.807011335788));
#253670=CARTESIAN_POINT('Ctrl Pts',(-20.278303623686,5.87267156586067,134.618815074426));
#253671=CARTESIAN_POINT('Ctrl Pts',(-20.5567512474989,6.38353099484532,
127.925321513668));
#253672=CARTESIAN_POINT('Ctrl Pts',(-20.8351988713118,1.02823729239309,
123.877524240513));
#253673=CARTESIAN_POINT('Ctrl Pts',(-21.1136464951247,-5.27195624958391,
126.1951512031));
#253674=CARTESIAN_POINT('Ctrl Pts',(-21.3920941189376,-6.72747954757436,
132.748416445183));
#253675=CARTESIAN_POINT('Ctrl Pts',(-21.6705417427505,-2.00077779699093,
137.515189354092));
#253676=CARTESIAN_POINT('Ctrl Pts',(-21.9489893665634,4.56454100559805,
136.115038496344));
#253677=CARTESIAN_POINT('Ctrl Pts',(-22.2274369903762,6.93526961426714,
129.834634109035));
#253678=CARTESIAN_POINT('Ctrl Pts',(-22.5058846141892,2.93282425418085,
124.445361009293));
#253679=CARTESIAN_POINT('Ctrl Pts',(-22.784332238002,-3.76474331906749,
124.899697895151));
#253680=CARTESIAN_POINT('Ctrl Pts',(-23.062779861815,-7.0026957000287,130.780131364099));
#253681=CARTESIAN_POINT('Ctrl Pts',(-23.3412274856278,-3.80551283336702,
136.682830333316));
#253682=CARTESIAN_POINT('Ctrl Pts',(-23.6196751094408,2.88875041752152,
137.183502812971));
#253683=CARTESIAN_POINT('Ctrl Pts',(-23.8981227332536,6.92839315801137,
131.822055253468));
#253684=CARTESIAN_POINT('Ctrl Pts',(-24.1765703570665,4.60118105711114,
125.525396040718));
#253685=CARTESIAN_POINT('Ctrl Pts',(-24.4550179808794,-1.95429165508329,
124.079847382335));
#253686=CARTESIAN_POINT('Ctrl Pts',(-24.7334656046923,-6.71386580871103,
128.813797876394));
#253687=CARTESIAN_POINT('Ctrl Pts',(-25.0119132285052,-5.30372527471246,
135.376978285193));
#253688=CARTESIAN_POINT('Ctrl Pts',(-25.290360852318,0.980279685362951,
137.738146442235));
#253689=CARTESIAN_POINT('Ctrl Pts',(-25.568808476131,6.36345550391485,133.727504160674));
#253690=CARTESIAN_POINT('Ctrl Pts',(-25.8472560999438,5.89892658645264,
127.030635766497));
#253691=CARTESIAN_POINT('Ctrl Pts',(-26.1257037237567,0.0135723146251221,
123.801636153745));
#253692=CARTESIAN_POINT('Ctrl Pts',(-26.4041513475696,-5.88425425129846,
127.007798221134));
#253693=CARTESIAN_POINT('Ctrl Pts',(-26.6825989713826,-6.37473862207999,
133.70281565846));
#253694=CARTESIAN_POINT('Ctrl Pts',(-26.9610465951954,-1.00714962246484,
137.734294510605));
#253695=CARTESIAN_POINT('Ctrl Pts',(-27.2394942190083,5.28596067820108,
135.397502661138));
#253696=CARTESIAN_POINT('Ctrl Pts',(-27.5179418428212,6.72153134913555,
128.839837661092));
#253697=CARTESIAN_POINT('Ctrl Pts',(-27.7963894666341,1.98034307527561,
124.087473285763));
#253698=CARTESIAN_POINT('Ctrl Pts',(-28.0748370904469,-4.58068373962494,
125.507600230172));
#253699=CARTESIAN_POINT('Ctrl Pts',(-28.3532847142599,-6.93228597665136,
131.795191209466));
#253700=CARTESIAN_POINT('Ctrl Pts',(-28.6317323380727,-2.91345606213275,
137.172257279568));
#253701=CARTESIAN_POINT('Ctrl Pts',(-28.9101799618857,3.78269764324474,
136.697537406337));
#253702=CARTESIAN_POINT('Ctrl Pts',(-29.1886275856985,7.00273700953358,
130.807275961916));
#253703=CARTESIAN_POINT('Ctrl Pts',(-29.4670752095115,3.78760316678249,
124.914335458459));
#253704=CARTESIAN_POINT('Ctrl Pts',(-29.7455228333243,-2.90815295154017,
124.434040332496));
#253705=CARTESIAN_POINT('Ctrl Pts',(-30.0239704571372,-6.93145857856742,
129.807758341064));
#253706=CARTESIAN_POINT('Ctrl Pts',(-30.3024180809501,-4.5850923924679,
136.097305155009));
#253707=CARTESIAN_POINT('Ctrl Pts',(-30.580865704763,1.97474970809384,137.52289451376));
#253708=CARTESIAN_POINT('Ctrl Pts',(-30.8593133285759,6.71989329880362,
132.774479440534));
#253709=CARTESIAN_POINT('Ctrl Pts',(-31.1377609523888,5.28978323295099,
126.215621414657));
#253710=CARTESIAN_POINT('Ctrl Pts',(-31.4162085762017,-1.00137920370602,
123.873590543879));
#253711=CARTESIAN_POINT('Ctrl Pts',(-31.6946562000146,-6.37232307225107,
127.900598783877));
#253712=CARTESIAN_POINT('Ctrl Pts',(-31.9731038238274,-5.88741334268594,
134.596022292384));
#253713=CARTESIAN_POINT('Ctrl Pts',(-32.2515514476404,0.00774163267598956,
137.807093954702));
#253714=CARTESIAN_POINT('Ctrl Pts',(-32.5299990714533,5.89578242580862,
134.582995782735));
#253715=CARTESIAN_POINT('Ctrl Pts',(-32.8084466952661,6.36588719460685,
127.886516490566));
#253716=CARTESIAN_POINT('Ctrl Pts',(-33.086894319079,0.9860526224398,123.8713934065));
#253717=CARTESIAN_POINT('Ctrl Pts',(-33.365341942892,-5.29991613840065,
126.227328495126));
#253718=CARTESIAN_POINT('Ctrl Pts',(-33.6437895667048,-6.71552088334846,
132.789332503824));
#253719=CARTESIAN_POINT('Ctrl Pts',(-33.9222371905177,-1.95989000793276,
137.527244320318));
#253720=CARTESIAN_POINT('Ctrl Pts',(-34.2006848143306,4.59678403882356,
136.08715444511));
#253721=CARTESIAN_POINT('Ctrl Pts',(-34.4791324381435,6.9292381192855,129.792435121214));
#253722=CARTESIAN_POINT('Ctrl Pts',(-34.7575800619564,2.89406088022529,
124.427625893158));
#253723=CARTESIAN_POINT('Ctrl Pts',(-35.0360276857693,-3.80061692502793,
124.922724356021));
#253724=CARTESIAN_POINT('Ctrl Pts',(-35.3144753095821,-7.00271344663942,
130.822759209339));
#253725=CARTESIAN_POINT('Ctrl Pts',(-35.592922933395,-3.76965841235978,
136.705886655638));
#253726=CARTESIAN_POINT('Ctrl Pts',(-35.8713705572079,2.92752854482695,
137.165799978524));
#253727=CARTESIAN_POINT('Ctrl Pts',(-36.1498181810209,6.9344597870381,131.779861302279));
#253728=CARTESIAN_POINT('Ctrl Pts',(-36.4282658048337,4.56896125215494,
125.49748515264));
#253729=CARTESIAN_POINT('Ctrl Pts',(-36.7067134286466,-1.99518946729269,
124.091868299989));
#253730=CARTESIAN_POINT('Ctrl Pts',(-36.9851610524595,-6.72585853672236,
128.854703963711));
#253731=CARTESIAN_POINT('Ctrl Pts',(-37.2636086762724,-5.27579218736066,
135.409178846303));
#253732=CARTESIAN_POINT('Ctrl Pts',(-37.5420563000852,1.02246944540875,
137.732050734562));
#253733=CARTESIAN_POINT('Ctrl Pts',(-37.8205039238982,6.38113160825695,
133.688713841779));
#253734=CARTESIAN_POINT('Ctrl Pts',(-38.0989515477111,5.87584555872632,
126.994797244432));
#253735=CARTESIAN_POINT('Ctrl Pts',(-38.377399171524,-0.0290555082599903,
123.801683279478));
#253736=CARTESIAN_POINT('Ctrl Pts',(-38.6558467953367,-5.90725598259587,
127.04368768842));
#253737=CARTESIAN_POINT('Ctrl Pts',(-38.9342944191497,-6.35697679442443,
133.741566800161));
#253738=CARTESIAN_POINT('Ctrl Pts',(-39.2127420429625,-0.964946487758246,
137.740296920595));
#253739=CARTESIAN_POINT('Ctrl Pts',(-39.4911896667755,5.31382250090111,
135.365240417872));
#253740=CARTESIAN_POINT('Ctrl Pts',(-39.7696372905882,6.70944820589337,
128.798958190032));
#253741=CARTESIAN_POINT('Ctrl Pts',(-40.0480849144012,1.93941878443644,
124.07554282374));
#253742=CARTESIAN_POINT('Ctrl Pts',(-40.3265325382142,-4.61284175404266,
125.535582288951));
#253743=CARTESIAN_POINT('Ctrl Pts',(-40.604980162027,-6.9261260704041,131.837371644027));
#253744=CARTESIAN_POINT('Ctrl Pts',(-40.8834277858398,-2.87463888813357,
137.18987433118));
#253745=CARTESIAN_POINT('Ctrl Pts',(-41.1618754096529,3.81850099841496,
136.674401865208));
#253746=CARTESIAN_POINT('Ctrl Pts',(-41.4403230334656,7.00262501156454,
130.76464826011));
#253747=CARTESIAN_POINT('Ctrl Pts',(-41.7187706572786,3.75167873633635,
124.891388371457));
#253748=CARTESIAN_POINT('Ctrl Pts',(-41.9972182810916,-2.94687701788942,
124.451861112224));
#253749=CARTESIAN_POINT('Ctrl Pts',(-42.2756659049044,-6.93739675562063,
129.849970561546));
#253750=CARTESIAN_POINT('Ctrl Pts',(-42.5541135287174,-4.55278778560923,
136.125117847804));
#253751=CARTESIAN_POINT('Ctrl Pts',(-42.8325611525302,2.01561074332903,
137.510749172913));
#253752=CARTESIAN_POINT('Ctrl Pts',(-43.1110087763431,6.73176146720674,
132.733537040953));
#253753=CARTESIAN_POINT('Ctrl Pts',(-43.389456400156,5.26175226755184,126.183506021407));
#253754=CARTESIAN_POINT('Ctrl Pts',(-43.6679040239687,-1.0435502150944,
123.879814634434));
#253755=CARTESIAN_POINT('Ctrl Pts',(-43.9463516477818,-6.38988103033122,
127.93944272308));
#253756=CARTESIAN_POINT('Ctrl Pts',(-44.2247992715946,-5.86422334173611,
134.631790397739));
#253757=CARTESIAN_POINT('Ctrl Pts',(-44.5032468954075,0.050369114677416,
137.806917084757));
#253758=CARTESIAN_POINT('Ctrl Pts',(-44.7816945192204,5.91867481537061,
134.547036472328));
#253759=CARTESIAN_POINT('Ctrl Pts',(-45.0601421430334,6.34800750407734,
127.847819589252));
#253760=CARTESIAN_POINT('Ctrl Pts',(-45.3385897668461,0.943831413943965,
123.865519476137));
#253761=CARTESIAN_POINT('Ctrl Pts',(-45.6170373906592,-5.32767963687585,
126.25967539076));
#253762=CARTESIAN_POINT('Ctrl Pts',(-45.895485014472,-6.7033133730266,132.830175008601));
#253763=CARTESIAN_POINT('Ctrl Pts',(-46.1739326382849,-1.91892959442962,
137.539050167615));
#253764=CARTESIAN_POINT('Ctrl Pts',(-46.4523802620978,4.62885673652604,
136.059074638009));
#253765=CARTESIAN_POINT('Ctrl Pts',(-46.7308278859106,6.92294985883713,
129.750273630666));
#253766=CARTESIAN_POINT('Ctrl Pts',(-47.0092755097235,2.8551902657795,124.410127069272));
#253767=CARTESIAN_POINT('Ctrl Pts',(-47.2877231335364,-3.83634969773052,
124.945968763085));
#253768=CARTESIAN_POINT('Ctrl Pts',(-47.5661707573492,-7.00247170512816,
130.865386372813));
#253769=CARTESIAN_POINT('Ctrl Pts',(-47.8446183811622,-3.73366430527375,
136.728724294741));
#253770=CARTESIAN_POINT('Ctrl Pts',(-48.123066004975,2.96619819148554,137.147861418602));
#253771=CARTESIAN_POINT('Ctrl Pts',(-48.4015136287881,6.9402694571073,131.737631203552));
#253772=CARTESIAN_POINT('Ctrl Pts',(-48.6799612526008,4.53657214265928,
125.469770912784));
#253773=CARTESIAN_POINT('Ctrl Pts',(-48.9584088764139,-2.03601334702262,
124.104137951514));
#253774=CARTESIAN_POINT('Ctrl Pts',(-49.2368565002267,-6.7376020355722,
128.895682296272));
#253775=CARTESIAN_POINT('Ctrl Pts',(-49.5153041240395,-5.24766360358919,
135.441208774179));
#253776=CARTESIAN_POINT('Ctrl Pts',(-49.7937517478526,1.06462131747325,
137.725698318783));
#253777=CARTESIAN_POINT('Ctrl Pts',(-50.0721993716652,6.39857125742062,
133.649816642113));
#253778=CARTESIAN_POINT('Ctrl Pts',(-50.3506469954783,5.85254679938199,
126.959099887138));
#253779=CARTESIAN_POINT('Ctrl Pts',(-50.6290946192911,-0.0716822544825644,
123.801989891996));
#253780=CARTESIAN_POINT('Ctrl Pts',(-50.907542243104,-5.93003881835047,
127.079716508824));
#253781=CARTESIAN_POINT('Ctrl Pts',(-51.1859898669169,-6.33897940665598,
133.780209102606));
#253782=CARTESIAN_POINT('Ctrl Pts',(-51.4644374907297,-0.922707596604453,
137.746042316915));
#253783=CARTESIAN_POINT('Ctrl Pts',(-51.7428851145428,5.34148741795441,
135.332809169526));
#253784=CARTESIAN_POINT('Ctrl Pts',(-52.0213327383556,6.69711644158035,
128.758153029896));
#253785=CARTESIAN_POINT('Ctrl Pts',(-52.2997803621686,1.89842262772099,
124.063861700536));
#253786=CARTESIAN_POINT('Ctrl Pts',(-52.5782279859813,-4.64482883791282,
125.563759584248));
#253787=CARTESIAN_POINT('Ctrl Pts',(-52.8566756097944,-6.91970951400822,
131.879513799985));
#253788=CARTESIAN_POINT('Ctrl Pts',(-53.135123233607,-2.83571519333325,
137.207254765232));
#253789=CARTESIAN_POINT('Ctrl Pts',(-53.4135708574202,3.85416285762642,
136.651048807542));
#253790=CARTESIAN_POINT('Ctrl Pts',(-53.6920184812329,7.0022535287505,130.72202202986));
#253791=CARTESIAN_POINT('Ctrl Pts',(-53.9704661050458,3.71561528605495,
124.868660391816));
#253792=CARTESIAN_POINT('Ctrl Pts',(-54.2489137288587,-2.98549188662705,
124.469917286158));
#253793=CARTESIAN_POINT('Ctrl Pts',(-54.5273613526715,-6.94307786488582,
129.892218147303));
#253794=CARTESIAN_POINT('Ctrl Pts',(-54.8058089764845,-4.5203144735249,
136.152733377983));
#253795=CARTESIAN_POINT('Ctrl Pts',(-55.0842566002972,2.05639708936689,
137.498355324372));
#253796=CARTESIAN_POINT('Ctrl Pts',(-55.3627042241104,6.74338018771311,
132.69252315503));
#253797=CARTESIAN_POINT('Ctrl Pts',(-55.6411518479232,5.23352632598741,
126.151561855625));
#253798=CARTESIAN_POINT('Ctrl Pts',(-55.919599471736,-1.08568255734582,
123.886295316588));
#253799=CARTESIAN_POINT('Ctrl Pts',(-56.1980470955489,-6.40720220901991,
127.978392822871));
#253800=CARTESIAN_POINT('Ctrl Pts',(-56.4764947193619,-5.8408160398338,
134.667416676276));
#253801=CARTESIAN_POINT('Ctrl Pts',(-56.7549423431748,0.0929947302327828,
137.806480732508));
#253802=CARTESIAN_POINT('Ctrl Pts',(-57.0333899669875,5.94134788626073,
134.510938475691));
#253803=CARTESIAN_POINT('Ctrl Pts',(-57.3118375908005,6.32989258579528,
127.809232243652));
#253804=CARTESIAN_POINT('Ctrl Pts',(-57.5902852146133,0.901575231427987,
123.859902667085));
#253805=CARTESIAN_POINT('Ctrl Pts',(-57.8687328384263,-5.35524571622284,
126.292190691378));
#253806=CARTESIAN_POINT('Ctrl Pts',(-58.1471804622391,-6.69085746896258,
132.870942446081));
#253807=CARTESIAN_POINT('Ctrl Pts',(-58.4256280860521,-1.87789807428466,
137.550606458515));
#253808=CARTESIAN_POINT('Ctrl Pts',(-58.7040757098649,4.6607579102399,136.030800115547));
#253809=CARTESIAN_POINT('Ctrl Pts',(-58.9825233336777,6.91640506593584,
129.708151199698));
#253810=CARTESIAN_POINT('Ctrl Pts',(-59.2609709574908,2.81621385120844,
124.392865186062));
#253811=CARTESIAN_POINT('Ctrl Pts',(-59.5394185813036,-3.87194031308425,
124.969430255013));
#253812=CARTESIAN_POINT('Ctrl Pts',(-59.8178662051166,-7.00197048445272,
130.908011274954));
#253813=CARTESIAN_POINT('Ctrl Pts',(-60.0963138289294,-3.69753184588372,
136.751342404371));
#253814=CARTESIAN_POINT('Ctrl Pts',(-60.3747614527424,3.00475792457964,
137.129687797925));
#253815=CARTESIAN_POINT('Ctrl Pts',(-60.6532090765552,6.94582195293937,
131.695366522141));
#253816=CARTESIAN_POINT('Ctrl Pts',(-60.9316567003681,4.50401492881459,
125.442254348109));
#253817=CARTESIAN_POINT('Ctrl Pts',(-61.210104324181,-2.07676178152925,
124.116655882255));
#253818=CARTESIAN_POINT('Ctrl Pts',(-61.4885519479939,-6.74909587010084,
128.93673135561));
#253819=CARTESIAN_POINT('Ctrl Pts',(-61.7669995718066,-5.21934056571308,
135.473066881942));
#253820=CARTESIAN_POINT('Ctrl Pts',(-62.0454471956197,1.10673373960332,
137.719089430292));
#253821=CARTESIAN_POINT('Ctrl Pts',(-62.3238948194324,6.41577380517329,
133.610814003028));
#253822=CARTESIAN_POINT('Ctrl Pts',(-62.6023424432454,5.82903117176375,
126.923545017394));
#253823=CARTESIAN_POINT('Ctrl Pts',(-62.8807900670583,-0.114306344492842,
123.802555979936));
#253824=CARTESIAN_POINT('Ctrl Pts',(-63.1592376908712,-5.95260191433588,
127.115883347286));
#253825=CARTESIAN_POINT('Ctrl Pts',(-63.4376853146842,-6.32074712567447,
133.818741133891));
#253826=CARTESIAN_POINT('Ctrl Pts',(-63.716132938497,-0.880434514181572,
137.751530486667));
#253827=CARTESIAN_POINT('Ctrl Pts',(-63.99458056231,5.36895440422691,135.300210117855));
#253828=CARTESIAN_POINT('Ctrl Pts',(-64.2730281861228,6.6845365131549,128.717423692735));
#253829=CARTESIAN_POINT('Ctrl Pts',(-64.5514758099358,1.85735612425694,
124.052430348997));
#253830=CARTESIAN_POINT('Ctrl Pts',(-64.8299234337484,-4.67664380594228,
125.592131071942));
#253831=CARTESIAN_POINT('Ctrl Pts',(-65.1083710575615,-6.91303654523158,
131.921616115747));
#253832=CARTESIAN_POINT('Ctrl Pts',(-65.3868186813742,-2.79668642006362,
137.224397937687));
#253833=CARTESIAN_POINT('Ctrl Pts',(-65.6652663051872,3.88968189941585,
136.627479098696));
#253834=CARTESIAN_POINT('Ctrl Pts',(-65.9437139290001,7.00162257485687,
130.679398850698));
#253835=CARTESIAN_POINT('Ctrl Pts',(-66.2221615528129,3.67941415228271,
124.846152361731));
#253836=CARTESIAN_POINT('Ctrl Pts',(-66.500609176626,-3.02399612686491,
124.48820818522));
#253837=CARTESIAN_POINT('Ctrl Pts',(-66.7790568004388,-6.94850169584742,
129.934499532835));
#253838=CARTESIAN_POINT('Ctrl Pts',(-67.0575044242516,-4.48767365952541,
136.180150722241));
#253839=CARTESIAN_POINT('Ctrl Pts',(-67.3359520480646,2.09710723485436,
137.485713427398));
#253840=CARTESIAN_POINT('Ctrl Pts',(-67.6143996718775,6.75474902978674,
132.651439302549));
#253841=CARTESIAN_POINT('Ctrl Pts',(-67.8928472956903,5.20510645418034,
126.119790101011));
#253842=CARTESIAN_POINT('Ctrl Pts',(-68.1712949195033,-1.12777466923081,
123.893032350195));
#253843=CARTESIAN_POINT('Ctrl Pts',(-68.449742543316,-6.42428596647451,
128.017447639935));
#253844=CARTESIAN_POINT('Ctrl Pts',(-68.728190167129,-5.81719230434518,
134.702899807851));
#253845=CARTESIAN_POINT('Ctrl Pts',(-69.0066377909419,0.135616899834216,
137.805784914121));
#253846=CARTESIAN_POINT('Ctrl Pts',(-69.2850854147548,5.96380079832,134.474703130449));
#253847=CARTESIAN_POINT('Ctrl Pts',(-69.5635330385676,6.31154311101565,
127.770755883637));
#253848=CARTESIAN_POINT('Ctrl Pts',(-69.8419806623805,0.859285640710264,
123.854543187474));
#253849=CARTESIAN_POINT('Ctrl Pts',(-70.1204282861936,-5.38261335497044,
126.324873192109));
#253850=CARTESIAN_POINT('Ctrl Pts',(-70.3988759100064,-6.67815363271447,
132.911633305611));
#253851=CARTESIAN_POINT('Ctrl Pts',(-70.6773235338194,-1.83679696793597,
137.561912764793));
#253852=CARTESIAN_POINT('Ctrl Pts',(-70.9557711576322,4.69248637785542,
136.002331925448));
#253853=CARTESIAN_POINT('Ctrl Pts',(-71.2342187814451,6.90960398310133,
129.666069389173));
#253854=CARTESIAN_POINT('Ctrl Pts',(-71.5126664052579,2.77713308079745,
124.375840883174));
#253855=CARTESIAN_POINT('Ctrl Pts',(-71.7911140290708,-3.90738745226578,
124.993107962432));
#253856=CARTESIAN_POINT('Ctrl Pts',(-72.0695616528837,-7.00120980318599,
130.950632336283));
#253857=CARTESIAN_POINT('Ctrl Pts',(-72.3480092766965,-3.66126237309149,
136.773740146404));
#253858=CARTESIAN_POINT('Ctrl Pts',(-72.6264569005095,3.04320631526353,
137.111279789924));
#253859=CARTESIAN_POINT('Ctrl Pts',(-72.9049045243223,6.95111706878496,
131.653068824177));
#253860=CARTESIAN_POINT('Ctrl Pts',(-73.1833521481353,4.47129081703998,
125.414936478256));
#253861=CARTESIAN_POINT('Ctrl Pts',(-73.4617997719481,-2.11743326086482,
124.129421628353));
#253862=CARTESIAN_POINT('Ctrl Pts',(-73.7402473957612,-6.76033961440018,
128.977849620639));
#253863=CARTESIAN_POINT('Ctrl Pts',(-74.018695019574,-5.19082412325261,
135.504751989078));
#253864=CARTESIAN_POINT('Ctrl Pts',(-74.2971426433868,1.14880515130821,
137.712224313981));
#253865=CARTESIAN_POINT('Ctrl Pts',(-74.5755902671998,6.43273861406817,
133.571707369781));
#253866=CARTESIAN_POINT('Ctrl Pts',(-74.8540378910127,5.80529954725181,
126.8881339527));
#253867=CARTESIAN_POINT('Ctrl Pts',(-75.1324855148255,-0.156926198840311,
123.803381522322));
#253868=CARTESIAN_POINT('Ctrl Pts',(-75.4109331386384,-5.97494443446864,
127.15218686363));
#253869=CARTESIAN_POINT('Ctrl Pts',(-75.6893807624512,-6.30228062708332,
133.857161466198));
#253870=CARTESIAN_POINT('Ctrl Pts',(-75.9678283862644,-0.838128806933456,
137.756761226486));
#253871=CARTESIAN_POINT('Ctrl Pts',(-76.2462760100769,5.3962224419198,135.267444470826));
#253872=CARTESIAN_POINT('Ctrl Pts',(-76.52472363389,6.67170888677059,128.676771687789));
#253873=CARTESIAN_POINT('Ctrl Pts',(-76.8031712577027,1.81622079577817,
124.041249192718));
#253874=CARTESIAN_POINT('Ctrl Pts',(-77.0816188815158,-4.70828547921653,
125.620695700721));
#253875=CARTESIAN_POINT('Ctrl Pts',(-77.3600665053286,-6.90610741134329,
131.963677031195));
#253876=CARTESIAN_POINT('Ctrl Pts',(-77.6385141291417,-2.75755401454922,
137.241303213299));
#253877=CARTESIAN_POINT('Ctrl Pts',(-77.9169617529544,3.92505680761298,
136.603693612052));
#253878=CARTESIAN_POINT('Ctrl Pts',(-78.1954093767674,7.00073217326374,
130.636780302039));
#253879=CARTESIAN_POINT('Ctrl Pts',(-78.4738570005803,3.6430766764653,124.823865115242));
#253880=CARTESIAN_POINT('Ctrl Pts',(-78.7523046243931,-3.06238831181505,
124.506733131632));
#253881=CARTESIAN_POINT('Ctrl Pts',(-79.0307522482061,-6.95366804752337,
129.976813151389));
#253882=CARTESIAN_POINT('Ctrl Pts',(-79.3091998720188,-4.45486655312747,
136.207368864621));
#253883=CARTESIAN_POINT('Ctrl Pts',(-79.5876474958318,2.13773967126259,
137.472823950436));
#253884=CARTESIAN_POINT('Ctrl Pts',(-79.8660951196445,6.76586757215105,
132.610287005887));
#253885=CARTESIAN_POINT('Ctrl Pts',(-80.1445427434577,5.17649370523912,
126.08819193488));
#253886=CARTESIAN_POINT('Ctrl Pts',(-80.4229903672703,-1.16982499101125,
123.900025485612));
#253887=CARTESIAN_POINT('Ctrl Pts',(-80.7014379910835,-6.44113166965063,
128.056605727087));
#253888=CARTESIAN_POINT('Ctrl Pts',(-80.9798856148961,-5.7933530106558,
134.738238477622));
#253889=CARTESIAN_POINT('Ctrl Pts',(-81.2583332387092,0.17823404410257,
137.804829655383));
#253890=CARTESIAN_POINT('Ctrl Pts',(-81.5367808625219,5.98603271954817,
134.438331779315));
#253891=CARTESIAN_POINT('Ctrl Pts',(-81.815228486335,6.29295975968447,127.732391934959));
#253892=CARTESIAN_POINT('Ctrl Pts',(-82.0936761101477,0.816964208846405,
123.849441235906));
#253893=CARTESIAN_POINT('Ctrl Pts',(-82.3721237339607,-5.40978153900143,
126.357721681897));
#253894=CARTESIAN_POINT('Ctrl Pts',(-82.6505713577735,-6.66520233502723,
132.952246079378));
#253895=CARTESIAN_POINT('Ctrl Pts',(-82.9290189815866,-1.79562779839943,
137.572968667493));
#253896=CARTESIAN_POINT('Ctrl Pts',(-83.2074666053992,4.72404096366304,
135.97367112261));
#253897=CARTESIAN_POINT('Ctrl Pts',(-83.4859142292123,6.90254686235,129.624029758449));
#253898=CARTESIAN_POINT('Ctrl Pts',(-83.7643618530252,2.73794940269844,
124.359054791448));
#253899=CARTESIAN_POINT('Ctrl Pts',(-84.0428094768383,-3.94268980176888,
125.017001007954));
#253900=CARTESIAN_POINT('Ctrl Pts',(-84.3212571006508,-7.00018968951541,
130.99324797746));
#253901=CARTESIAN_POINT('Ctrl Pts',(-84.5997047244641,-3.62485723087481,
136.795916690882));
#253902=CARTESIAN_POINT('Ctrl Pts',(-84.8781523482765,3.08154193881888,
137.092638076712));
#253903=CARTESIAN_POINT('Ctrl Pts',(-85.1565999720898,6.95615460843127,
131.61073967702));
#253904=CARTESIAN_POINT('Ctrl Pts',(-85.4350475959023,4.4384010199398,125.387818315495));
#253905=CARTESIAN_POINT('Ctrl Pts',(-85.7134952197154,-2.1580262779319,
124.142434716771));
#253906=CARTESIAN_POINT('Ctrl Pts',(-85.9919428435283,-6.7713328518292,
129.019035567703));
#253907=CARTESIAN_POINT('Ctrl Pts',(-86.2703904673411,-5.16211533289519,
135.536262921482));
#253908=CARTESIAN_POINT('Ctrl Pts',(-86.5488380911541,1.19083399361533,
137.70510322424));
#253909=CARTESIAN_POINT('Ctrl Pts',(-86.827285714967,6.4494650554685,133.532498191482));
#253910=CARTESIAN_POINT('Ctrl Pts',(-87.1057333387799,5.78135280522977,
126.852868005224));
#253911=CARTESIAN_POINT('Ctrl Pts',(-87.3841809625928,-0.199540238229241,
123.804466488563));
#253912=CARTESIAN_POINT('Ctrl Pts',(-87.6626285864056,-5.99706555083783,
127.188625712615));
#253913=CARTESIAN_POINT('Ctrl Pts',(-87.9410762102187,-6.28358059516641,
133.895468675847));
#253914=CARTESIAN_POINT('Ctrl Pts',(-88.2195238340314,-0.795792042514341,
137.761734342542));
#253915=CARTESIAN_POINT('Ctrl Pts',(-88.4979714578443,5.42329052060546,
135.234513442586));
#253916=CARTESIAN_POINT('Ctrl Pts',(-88.7764190816572,6.65863403776028,
128.636198521433));
#253917=CARTESIAN_POINT('Ctrl Pts',(-89.0548667054699,1.77501816656995,
124.03031864602));
#253918=CARTESIAN_POINT('Ctrl Pts',(-89.3333143292831,-4.73975268523957,
125.649452412109));
#253919=CARTESIAN_POINT('Ctrl Pts',(-89.6117619530957,-6.8989223691057,
132.005694987746));
#253920=CARTESIAN_POINT('Ctrl Pts',(-89.8902095769088,-2.71831942685781,
137.257969965635));
#253921=CARTESIAN_POINT('Ctrl Pts',(-90.1686572007216,3.9602862713853,136.579693228991));
#253922=CARTESIAN_POINT('Ctrl Pts',(-90.4471048245344,6.99958235696585,
130.59416796313));
#253923=CARTESIAN_POINT('Ctrl Pts',(-90.7255524483476,3.60660420510239,
124.801799478213));
#253924=CARTESIAN_POINT('Ctrl Pts',(-91.0040000721602,-3.10066701883943,
124.525491438947));
#253925=CARTESIAN_POINT('Ctrl Pts',(-91.2824476959735,-6.95857672847263,
130.019157435019));
#253926=CARTESIAN_POINT('Ctrl Pts',(-91.560895319786,-4.4218943700117,136.234386796543));
#253927=CARTESIAN_POINT('Ctrl Pts',(-91.8393429435991,2.17829289294083,
137.459687371113));
#253928=CARTESIAN_POINT('Ctrl Pts',(-92.1177905674117,6.77673540280433,
132.56906778996));
#253929=CARTESIAN_POINT('Ctrl Pts',(-92.3962381912249,5.14768913942031,
126.056768528114));
#253930=CARTESIAN_POINT('Ctrl Pts',(-92.6746858150375,-1.21183196449619,
123.907274463707));
#253931=CARTESIAN_POINT('Ctrl Pts',(-92.9531334388505,-6.45773869432309,
128.095865633305));
#253932=CARTESIAN_POINT('Ctrl Pts',(-93.2315810626634,-5.76929904214118,
134.773431376103));
#253933=CARTESIAN_POINT('Ctrl Pts',(-93.5100286864763,0.220844583841736,
137.803614991691));
#253934=CARTESIAN_POINT('Ctrl Pts',(-93.7884763102892,6.00804282613147,
134.401825770043));
#253935=CARTESIAN_POINT('Ctrl Pts',(-94.0669239341021,6.27414322041607,
127.694141819211));
#253936=CARTESIAN_POINT('Ctrl Pts',(-94.3453715579151,0.774612504073732,
123.844597001431));
#253937=CARTESIAN_POINT('Ctrl Pts',(-94.6238191817278,-5.43674926158731,
126.390734943524));
#253938=CARTESIAN_POINT('Ctrl Pts',(-94.9022668055408,-6.65200405581671,
132.99277926246));
#253939=CARTESIAN_POINT('Ctrl Pts',(-95.1807144293538,-1.75439209121494,
137.583773756932));
#253940=CARTESIAN_POINT('Ctrl Pts',(-95.4591620531666,4.75542049839504,
135.94481876907));
#253941=CARTESIAN_POINT('Ctrl Pts',(-95.7376096769794,6.89523396518648,
129.582033865318));
#253942=CARTESIAN_POINT('Ctrl Pts',(-96.0160573007924,2.69866426887766,
124.342507532899));
#253943=CARTESIAN_POINT('Ctrl Pts',(-96.2945049246052,-3.97784605345104,
125.041108506217));
#253944=CARTESIAN_POINT('Ctrl Pts',(-96.5729525484182,-6.99891018124123,
131.035856619345));
#253945=CARTESIAN_POINT('Ctrl Pts',(-96.8514001722308,-3.58831776824163,
136.817871216047));
#253946=CARTESIAN_POINT('Ctrl Pts',(-97.129847796044,3.11976337470375,137.073763349068));
#253947=CARTESIAN_POINT('Ctrl Pts',(-97.4082954198568,6.96093438520996,
131.56838064919));
#253948=CARTESIAN_POINT('Ctrl Pts',(-97.6867430436697,4.40534675625846,
125.360900864701));
#253949=CARTESIAN_POINT('Ctrl Pts',(-97.9651906674826,-2.1985393285419,
124.155694665303));
#253950=CARTESIAN_POINT('Ctrl Pts',(-98.2436382912955,-6.78207517502872,
129.060287670645));
#253951=CARTESIAN_POINT('Ctrl Pts',(-98.5220859151084,-5.13321525845608,
135.567598511506));
#253952=CARTESIAN_POINT('Ctrl Pts',(-98.8005335389213,1.23281870913114,
137.697726424945));
#253953=CARTESIAN_POINT('Ctrl Pts',(-99.0789811627341,6.4659525095689,133.493187921042));
#253954=CARTESIAN_POINT('Ctrl Pts',(-99.3574287865471,5.7571918330539,126.817748481762));
#253955=CARTESIAN_POINT('Ctrl Pts',(-99.6358764103599,-0.242146883580649,
123.805810838454));
#253956=CARTESIAN_POINT('Ctrl Pts',(-99.9143240341728,-6.01896444373747,
127.225198543987));
#253957=CARTESIAN_POINT('Ctrl Pts',(-100.192771657986,-6.26464772285957,
133.93366134335));
#253958=CARTESIAN_POINT('Ctrl Pts',(-100.471219281798,-0.753425789729175,
137.766449650557));
#253959=CARTESIAN_POINT('Ctrl Pts',(-100.749666905611,5.45015763726631,
135.201418253402));
#253960=CARTESIAN_POINT('Ctrl Pts',(-101.028114529424,6.64531245061667,
128.595705697122));
#253961=CARTESIAN_POINT('Ctrl Pts',(-101.306562153237,1.73374976341167,
124.019639113937));
#253962=CARTESIAN_POINT('Ctrl Pts',(-101.58500977705,-4.77104425798471,
125.678400140516));
#253963=CARTESIAN_POINT('Ctrl Pts',(-101.863457400863,-6.89148168476197,
132.047668428412));
#253964=CARTESIAN_POINT('Ctrl Pts',(-102.141905024676,-2.67898411084018,
137.274397577103));
#253965=CARTESIAN_POINT('Ctrl Pts',(-102.420352648489,3.99536898529432,
136.555478838857));
#253966=CARTESIAN_POINT('Ctrl Pts',(-102.698800272302,6.99817316856906,
130.551563412989));
#253967=CARTESIAN_POINT('Ctrl Pts',(-102.977247896115,3.56999808969468,
124.779956268296));
#253968=CARTESIAN_POINT('Ctrl Pts',(-103.255695519928,-3.13883082950684,
124.544482412068));
#253969=CARTESIAN_POINT('Ctrl Pts',(-103.53414314374,-6.96322755680218,
130.061530814641));
#253970=CARTESIAN_POINT('Ctrl Pts',(-103.812590767553,-4.38875833197407,
136.261203516848));
#253971=CARTESIAN_POINT('Ctrl Pts',(-104.091038391366,2.21876539717438,
137.44630417621));
#253972=CARTESIAN_POINT('Ctrl Pts',(-104.369486015179,6.78735211903507,
132.52778318216));
#253973=CARTESIAN_POINT('Ctrl Pts',(-104.647933638992,5.11869382408742,
126.02552104512));
#253974=CARTESIAN_POINT('Ctrl Pts',(-104.926381262805,-1.25379403310144,
123.914779015865));
#253975=CARTESIAN_POINT('Ctrl Pts',(-105.204828886617,-6.47410642511416,
128.135225903801));
#253976=CARTESIAN_POINT('Ctrl Pts',(-105.483276510431,-5.74503129012806,
134.808477199207));
#253977=CARTESIAN_POINT('Ctrl Pts',(-105.761724134243,0.263446940103889,
137.802140968053));
#253978=CARTESIAN_POINT('Ctrl Pts',(-106.040171758056,6.02983030247923,
134.365186455377));
#253979=CARTESIAN_POINT('Ctrl Pts',(-106.318619381869,6.25509419046252,
127.656006953765));
#253980=CARTESIAN_POINT('Ctrl Pts',(-106.597067005682,0.732232095750508,
123.840010663559));
#253981=CARTESIAN_POINT('Ctrl Pts',(-106.875514629495,-5.46351552342998,
126.423911753675));
#253982=CARTESIAN_POINT('Ctrl Pts',(-107.153962253308,-6.63855928414971,
133.033231352883));
#253983=CARTESIAN_POINT('Ctrl Pts',(-107.432409877121,-1.71309137438684,
137.594327632723));
#253984=CARTESIAN_POINT('Ctrl Pts',(-107.710857500934,4.78662381927155,
135.915775933963));
#253985=CARTESIAN_POINT('Ctrl Pts',(-107.989305124746,6.8876655625929,129.540083265954));
#253986=CARTESIAN_POINT('Ctrl Pts',(-108.26775274856,2.65927913505975,124.326199720693));
#253987=CARTESIAN_POINT('Ctrl Pts',(-108.546200372372,-4.0128549045848,
125.065429563905));
#253988=CARTESIAN_POINT('Ctrl Pts',(-108.824647996185,-6.99737132577695,
131.078456683062));
#253989=CARTESIAN_POINT('Ctrl Pts',(-109.103095619998,-3.5516453391731,
136.839602908365));
#253990=CARTESIAN_POINT('Ctrl Pts',(-109.381543243811,3.1578692066097,137.054656306401));
#253991=CARTESIAN_POINT('Ctrl Pts',(-109.659990867624,6.96545622200577,
131.525993310316));
#253992=CARTESIAN_POINT('Ctrl Pts',(-109.938438491437,4.37212925083209,
125.334185123311));
#253993=CARTESIAN_POINT('Ctrl Pts',(-110.21688611525,-2.23897091146772,
124.169200982596));
#253994=CARTESIAN_POINT('Ctrl Pts',(-110.495333739063,-6.79256618593892,
129.10160440085));
#253995=CARTESIAN_POINT('Ctrl Pts',(-110.773781362875,-5.10412497083799,
135.598757597999));
#253996=CARTESIAN_POINT('Ctrl Pts',(-111.052228986688,1.27475774209554,
137.690094189444));
#253997=CARTESIAN_POINT('Ctrl Pts',(-111.330676610501,6.48220036542147,
133.453778015119));
#253998=CARTESIAN_POINT('Ctrl Pts',(-111.609124234314,5.73281752601749,
126.782776683677));
#253999=CARTESIAN_POINT('Ctrl Pts',(-111.887571858127,-0.284744556090853,
123.807414522182));
#254000=CARTESIAN_POINT('Ctrl Pts',(-112.16601948194,-6.04064030169634,
127.261904002525));
#254001=CARTESIAN_POINT('Ctrl Pts',(-112.444467105753,-6.24548271172772,
133.971738053464));
#254002=CARTESIAN_POINT('Ctrl Pts',(-112.722914729566,-0.71103161847358,
137.770906975801));
#254003=CARTESIAN_POINT('Ctrl Pts',(-113.001362353379,5.47682279633179,
135.16816012963));
#254004=CARTESIAN_POINT('Ctrl Pts',(-113.279809977192,6.63174461897671,
128.55529471533));
#254005=CARTESIAN_POINT('Ctrl Pts',(-113.558257601004,1.69241711551747,
124.009210992206));
#254006=CARTESIAN_POINT('Ctrl Pts',(-113.836705224817,-4.80215903792943,
125.707537813274));
#254007=CARTESIAN_POINT('Ctrl Pts',(-114.11515284863,-6.88378563403075,
132.089595797848));
#254008=CARTESIAN_POINT('Ctrl Pts',(-114.393600472443,-2.63954952408134,
137.290585438973));
#254009=CARTESIAN_POINT('Ctrl Pts',(-114.672048096256,4.03030364933543,
136.531051338922));
#254010=CARTESIAN_POINT('Ctrl Pts',(-114.950495720069,6.99650466029252,
130.508968230339));
#254011=CARTESIAN_POINT('Ctrl Pts',(-115.228943343882,3.53325968669456,
124.758336294896));
#254012=CARTESIAN_POINT('Ctrl Pts',(-115.507390967695,-3.17687832964389,
124.563705347279));
#254013=CARTESIAN_POINT('Ctrl Pts',(-115.785838591507,-6.96762036017394,
130.103931720095));
#254014=CARTESIAN_POINT('Ctrl Pts',(-116.06428621532,-4.35545966688232,
136.287818031834));
#254015=CARTESIAN_POINT('Ctrl Pts',(-116.342733839133,2.25915568424066,
137.432674861647));
#254016=CARTESIAN_POINT('Ctrl Pts',(-116.621181462946,6.79771732743703,
132.486434712303));
#254017=CARTESIAN_POINT('Ctrl Pts',(-116.899629086759,5.08950883367243,
125.994450643782));
#254018=CARTESIAN_POINT('Ctrl Pts',(-117.178076710572,-1.2957096419083,
123.922538864004));
#254019=CARTESIAN_POINT('Ctrl Pts',(-117.456524334385,-6.49023425551004,
128.174685080065));
#254020=CARTESIAN_POINT('Ctrl Pts',(-117.734971958198,-5.7205506538686,
134.843374648297));
#254021=CARTESIAN_POINT('Ctrl Pts',(-118.013419582011,0.306039534242538,
137.800407639092));
#254022=CARTESIAN_POINT('Ctrl Pts',(-118.291867205823,6.05139434124684,
134.328415193001));
#254023=CARTESIAN_POINT('Ctrl Pts',(-118.570314829636,6.23581337569426,
127.617988751722));
#254024=CARTESIAN_POINT('Ctrl Pts',(-118.848762453449,0.689824554297045,
123.835682392233));
#254025=CARTESIAN_POINT('Ctrl Pts',(-119.127210077262,-5.49007933269568,
126.457250882969));
#254026=CARTESIAN_POINT('Ctrl Pts',(-119.405657701075,-6.62486851822702,
133.073600851681));
#254027=CARTESIAN_POINT('Ctrl Pts',(-119.684105324888,-1.67172717832737,
137.60462990379));
#254028=CARTESIAN_POINT('Ctrl Pts',(-119.962552948701,4.81764977004229,
135.886543693482));
#254029=CARTESIAN_POINT('Ctrl Pts',(-120.241000572514,6.87984193501854,
129.498179514853));
#254030=CARTESIAN_POINT('Ctrl Pts',(-120.519448196327,2.61979546067638,
124.310131959122));
#254031=CARTESIAN_POINT('Ctrl Pts',(-120.79789582014,-4.04771505790416,
125.089963279793));
#254032=CARTESIAN_POINT('Ctrl Pts',(-121.076343443952,-6.9955731801444,
131.121046590047));
#254033=CARTESIAN_POINT('Ctrl Pts',(-121.354791067765,-3.51484130258126,
136.86111096256));
#254034=CARTESIAN_POINT('Ctrl Pts',(-121.633238691578,3.19585802251066,
137.035317656727));
#254035=CARTESIAN_POINT('Ctrl Pts',(-121.911686315391,6.96971995125911,
131.483579231079));
#254036=CARTESIAN_POINT('Ctrl Pts',(-122.190133939204,4.3387497345494,125.307672081285));
#254037=CARTESIAN_POINT('Ctrl Pts',(-122.468581563017,-2.2793195285039,
124.182953168171));
#254038=CARTESIAN_POINT('Ctrl Pts',(-122.74702918683,-6.80280549581075,
129.142984227312));
#254039=CARTESIAN_POINT('Ctrl Pts',(-123.025476810643,-5.07484554799192,
135.629739026348));
#254040=CARTESIAN_POINT('Ctrl Pts',(-123.303924434456,1.31664953844379,
137.682206800553));
#254041=CARTESIAN_POINT('Ctrl Pts',(-123.582372058268,6.49820802095541,
133.414269934058));
#254042=CARTESIAN_POINT('Ctrl Pts',(-123.860819682081,5.7082307873194,126.747953906865));
#254043=CARTESIAN_POINT('Ctrl Pts',(-124.139267305894,-0.327331677286216,
123.809277480321));
#254044=CARTESIAN_POINT('Ctrl Pts',(-124.417714929707,-6.06209232150722,
127.298740728095));
#254045=CARTESIAN_POINT('Ctrl Pts',(-124.69616255352,-6.22608627193705,
134.009697395242));
#254046=CARTESIAN_POINT('Ctrl Pts',(-124.974610177333,-0.668611099680587,
137.77510615311));
#254047=CARTESIAN_POINT('Ctrl Pts',(-125.253057801146,5.50328500971429,
135.134740303665));
#254048=CARTESIAN_POINT('Ctrl Pts',(-125.531505424959,6.61793104560076,
128.514967073503));
#254049=CARTESIAN_POINT('Ctrl Pts',(-125.809953048772,1.6510217544855,123.999034667242));
#254050=CARTESIAN_POINT('Ctrl Pts',(-126.088400672584,-4.8330958721059,
125.736864350674));
#254051=CARTESIAN_POINT('Ctrl Pts',(-126.366848296398,-6.87583450209069,
132.131475542423));
#254052=CARTESIAN_POINT('Ctrl Pts',(-126.64529592021,-2.60001712784396,
137.306532951397));
#254053=CARTESIAN_POINT('Ctrl Pts',(-126.923743544023,4.06508896899354,
136.506411634357));
#254054=CARTESIAN_POINT('Ctrl Pts',(-127.202191167836,6.99457689396224,
130.466383993564));
#254055=CARTESIAN_POINT('Ctrl Pts',(-127.480638791649,3.49639035745773,
124.736940359153));
#254056=CARTESIAN_POINT('Ctrl Pts',(-127.759086415462,-3.21480810938582,
124.583159532264));
#254057=CARTESIAN_POINT('Ctrl Pts',(-128.037534039275,-6.97175497581086,
130.146358580199));
#254058=CARTESIAN_POINT('Ctrl Pts',(-128.315981663087,-4.32199960863106,
136.314229355287));
#254059=CARTESIAN_POINT('Ctrl Pts',(-128.594429286901,2.29946225746178,
137.418799932461));
#254060=CARTESIAN_POINT('Ctrl Pts',(-128.872876910713,6.80783064392392,
132.44502391257));
#254061=CARTESIAN_POINT('Ctrl Pts',(-129.151324534526,5.06013524963555,
125.963558475429));
#254062=CARTESIAN_POINT('Ctrl Pts',(-129.429772158339,-1.33757723771771,
123.930553720578));
#254063=CARTESIAN_POINT('Ctrl Pts',(-129.708219782152,-6.50612158788957,
128.214241699924));
#254064=CARTESIAN_POINT('Ctrl Pts',(-129.986667405965,-5.69585804050008,
134.878122430239));
#254065=CARTESIAN_POINT('Ctrl Pts',(-130.265115029778,0.348620787973942,
137.798415069035));
#254066=CARTESIAN_POINT('Ctrl Pts',(-130.543562653591,6.07273414337257,
134.291513345486));
#254067=CARTESIAN_POINT('Ctrl Pts',(-130.822010277403,6.21630149056731,
127.58008862186));
#254068=CARTESIAN_POINT('Ctrl Pts',(-131.100457901217,0.647391451141708,
123.831612347843));
#254069=CARTESIAN_POINT('Ctrl Pts',(-131.378905525029,-5.5164397050528,
126.490751096011));
#254070=CARTESIAN_POINT('Ctrl Pts',(-131.657353148842,-6.61093226536518,
133.113886262947));
#254071=CARTESIAN_POINT('Ctrl Pts',(-131.935800772655,-1.63030103580305,
137.614680188378));
#254072=CARTESIAN_POINT('Ctrl Pts',(-132.214248396468,4.848497201029,135.857123130838));
#254073=CARTESIAN_POINT('Ctrl Pts',(-132.492696020281,6.87176337237162,
129.456324164773));
#254074=CARTESIAN_POINT('Ctrl Pts',(-132.771143644094,2.58021470880796,
124.294304843582));
#254075=CARTESIAN_POINT('Ctrl Pts',(-133.049591267907,-4.08242522165371,
125.114708744776));
#254076=CARTESIAN_POINT('Ctrl Pts',(-133.32803889172,-6.99351581097555,
131.163624762118));
#254077=CARTESIAN_POINT('Ctrl Pts',(-133.606486515532,-3.47790702225152,
136.882394581644));
#254078=CARTESIAN_POINT('Ctrl Pts',(-133.884934139345,3.23372841471757,
137.015748116649));
#254079=CARTESIAN_POINT('Ctrl Pts',(-134.163381763158,6.97372541497715,
131.441139983145));
#254080=CARTESIAN_POINT('Ctrl Pts',(-134.441829386971,4.30520944429882,
125.281362721075));
#254081=CARTESIAN_POINT('Ctrl Pts',(-134.720277010784,-2.31958368451587,
124.196950712432));
#254082=CARTESIAN_POINT('Ctrl Pts',(-134.998724634597,-6.81279272522359,
129.184425616688));
#254083=CARTESIAN_POINT('Ctrl Pts',(-135.27717225841,-5.04537807487797,
135.660541648527));
#254084=CARTESIAN_POINT('Ctrl Pts',(-135.555619882223,1.35849254585843,
137.674064550544));
#254085=CARTESIAN_POINT('Ctrl Pts',(-135.834067506036,6.51397488300169,
133.374665141848));
#254086=CARTESIAN_POINT('Ctrl Pts',(-136.112515129848,5.68343252803032,
126.713281441693));
#254087=CARTESIAN_POINT('Ctrl Pts',(-136.390962753662,-0.369906669086523,
123.811399643837));
#254088=CARTESIAN_POINT('Ctrl Pts',(-136.669410377474,-6.08331970825794,
127.335707355701));
#254089=CARTESIAN_POINT('Ctrl Pts',(-136.947858001288,-6.20645912223011,
134.047537962086));
#254090=CARTESIAN_POINT('Ctrl Pts',(-137.2263056251,-0.626165805256695,
137.779047026878));
#254091=CARTESIAN_POINT('Ctrl Pts',(-137.504753248913,5.52954329684707,
135.101160013885));
#254092=CARTESIAN_POINT('Ctrl Pts',(-137.783200872726,6.60387224235649,
128.474724265995));
#254093=CARTESIAN_POINT('Ctrl Pts',(-138.061648496539,1.60956521423443,
123.989110516135));
#254094=CARTESIAN_POINT('Ctrl Pts',(-138.340096120352,-4.86385361413656,
125.766378666012));
#254095=CARTESIAN_POINT('Ctrl Pts',(-138.618543744165,-6.86762858357524,
132.173306110266));
#254096=CARTESIAN_POINT('Ctrl Pts',(-138.896991367977,-2.56038838701599,
137.322239523433));
#254097=CARTESIAN_POINT('Ctrl Pts',(-139.17543899179,4.09972365528409,136.481560638194));
#254098=CARTESIAN_POINT('Ctrl Pts',(-139.453886615603,6.99238994101352,
130.423812280637));
#254099=CARTESIAN_POINT('Ctrl Pts',(-139.732334239416,3.45939146819007,
124.715769253897));
#254100=CARTESIAN_POINT('Ctrl Pts',(-140.010781863229,-3.25261876323132,
124.602844246145));
#254101=CARTESIAN_POINT('Ctrl Pts',(-140.289229487042,-6.97563125050334,
130.188809822811));
#254102=CARTESIAN_POINT('Ctrl Pts',(-140.567677110855,-4.28837939709471,
136.340436508528));
#254103=CARTESIAN_POINT('Ctrl Pts',(-140.846124734668,2.33968362326381,
137.404679902793));
#254104=CARTESIAN_POINT('Ctrl Pts',(-141.124572358481,6.81769169374202,
132.403552317457));
#254105=CARTESIAN_POINT('Ctrl Pts',(-141.403019982293,5.03057416042698,
125.932845684778));
#254106=CARTESIAN_POINT('Ctrl Pts',(-141.681467606106,-1.37939526911043,
123.938823288595));
#254107=CARTESIAN_POINT('Ctrl Pts',(-141.959915229919,-6.52176783354029,
128.253894297592));
#254108=CARTESIAN_POINT('Ctrl Pts',(-142.238362853732,-5.67095436501806,
134.912719257437));
#254109=CARTESIAN_POINT('Ctrl Pts',(-142.516810477545,0.39118912343359,
137.796163331718));
#254110=CARTESIAN_POINT('Ctrl Pts',(-142.795258101358,6.09384891810056,
134.254482280245));
#254111=CARTESIAN_POINT('Ctrl Pts',(-143.073705725171,6.19655925810344,
127.542307968582));
#254112=CARTESIAN_POINT('Ctrl Pts',(-143.352153348984,0.604934358657401,
123.827800681205));
#254113=CARTESIAN_POINT('Ctrl Pts',(-143.630600972796,-5.54259566370794,
126.524411151443));
#254114=CARTESIAN_POINT('Ctrl Pts',(-143.90904859661,-6.59675104197701,
133.154086093891));
#254115=CARTESIAN_POINT('Ctrl Pts',(-144.187496220422,-1.58881448187379,
137.624478114069));
#254116=CARTESIAN_POINT('Ctrl Pts',(-144.465943844235,4.87916496916901,
135.827515336221));
#254117=CARTESIAN_POINT('Ctrl Pts',(-144.744391468048,6.86343017400547,
129.41451876668));
#254118=CARTESIAN_POINT('Ctrl Pts',(-145.022839091861,2.54053834613545,
124.278718960552));
#254119=CARTESIAN_POINT('Ctrl Pts',(-145.301286715674,-4.11698410963516,
125.139665041902));
#254120=CARTESIAN_POINT('Ctrl Pts',(-145.579734339487,-6.99119929450595,
131.206189621523));
#254121=CARTESIAN_POINT('Ctrl Pts',(-145.8581819633,-3.44084386679896,136.903452976945));
#254122=CARTESIAN_POINT('Ctrl Pts',(-146.136629587113,3.27147897992919,
136.995948411323));
#254123=CARTESIAN_POINT('Ctrl Pts',(-146.415077210925,6.97747246473481,
131.398677139117));
#254124=CARTESIAN_POINT('Ctrl Pts',(-146.693524834738,4.27150962292939,
125.255258017582));
#254125=CARTESIAN_POINT('Ctrl Pts',(-146.971972458551,-2.35976188750221,
124.211193096699));
#254126=CARTESIAN_POINT('Ctrl Pts',(-147.250420082364,-6.82252750409623,
129.225927033352));
#254127=CARTESIAN_POINT('Ctrl Pts',(-147.528867706177,-5.01572364342383,
135.69116432313));
#254128=CARTESIAN_POINT('Ctrl Pts',(-147.80731532999,1.40028521383297,137.665667741127));
#254129=CARTESIAN_POINT('Ctrl Pts',(-148.085762953803,6.52950036731291,
133.334965106058));
#254130=CARTESIAN_POINT('Ctrl Pts',(-148.364210577616,5.65842366705879,
126.678760572968));
#254131=CARTESIAN_POINT('Ctrl Pts',(-148.642658201429,-0.412467953858535,
123.813780934094));
#254132=CARTESIAN_POINT('Ctrl Pts',(-148.921105825242,-6.10432167535963,
127.372802515528));
#254133=CARTESIAN_POINT('Ctrl Pts',(-149.199553449054,-6.18660198989778,
134.085258351801));
#254134=CARTESIAN_POINT('Ctrl Pts',(-149.478001072867,-0.583697308029368,
137.782729451077));
#254135=CARTESIAN_POINT('Ctrl Pts',(-149.75644869668,5.55559668471987,135.067420504625));
#254136=CARTESIAN_POINT('Ctrl Pts',(-150.034896320493,6.58956873019717,
128.434567784019));
#254137=CARTESIAN_POINT('Ctrl Pts',(-150.313343944306,1.56804903095274,
123.979438906626));
#254138=CARTESIAN_POINT('Ctrl Pts',(-150.591791568119,-4.89443112428377,
125.796079665625));
#254139=CARTESIAN_POINT('Ctrl Pts',(-150.870239191931,-6.85916818255639,
132.21508595133));
#254140=CARTESIAN_POINT('Ctrl Pts',(-151.148686815745,-2.52066477005453,
137.33770457307));
#254141=CARTESIAN_POINT('Ctrl Pts',(-151.427134439557,4.13420642480782,
136.456499271296));
#254142=CARTESIAN_POINT('Ctrl Pts',(-151.705582063371,6.98994388248347,
130.381254669068));
#254143=CARTESIAN_POINT('Ctrl Pts',(-151.984029687183,3.42226438989971,
124.694823763634));
#254144=CARTESIAN_POINT('Ctrl Pts',(-152.262477310996,-3.29030889009209,
124.622758759495));
#254145=CARTESIAN_POINT('Ctrl Pts',(-152.540924934809,-6.97924904061452,
130.231283874884));
#254146=CARTESIAN_POINT('Ctrl Pts',(-152.819372558622,-4.25460027808296,
136.366438520441));
#254147=CARTESIAN_POINT('Ctrl Pts',(-153.097820182435,2.37981829122829,
137.390315295868));
#254148=CARTESIAN_POINT('Ctrl Pts',(-153.376267806248,6.82730011148789,
132.362021463707));
#254149=CARTESIAN_POINT('Ctrl Pts',(-153.654715430061,5.00082666144207,
125.902313409905));
#254150=CARTESIAN_POINT('Ctrl Pts',(-153.933163053873,-1.42116218650446,
123.947347261623));
#254151=CARTESIAN_POINT('Ctrl Pts',(-154.211610677687,-6.53717241268631,
128.293641403726));
#254152=CARTESIAN_POINT('Ctrl Pts',(-154.490058301499,-5.64584055023574,
134.947163847896));
#254153=CARTESIAN_POINT('Ctrl Pts',(-154.768505925312,0.433742963236675,
137.79365251058));
#254154=CARTESIAN_POINT('Ctrl Pts',(-155.046953549125,6.11473788301669,
134.217323369476));
#254155=CARTESIAN_POINT('Ctrl Pts',(-155.325401172938,6.17658740985663,
127.504648191865));
#254156=CARTESIAN_POINT('Ctrl Pts',(-155.603848796751,0.562454850108638,
123.824247533559));
#254157=CARTESIAN_POINT('Ctrl Pts',(-155.882296420564,-5.5685462394425,
126.558229801974));
#254158=CARTESIAN_POINT('Ctrl Pts',(-156.160744044376,-6.5823253735531,
133.194198854895));
#254159=CARTESIAN_POINT('Ctrl Pts',(-156.43919166819,-1.54726905384013,
137.634023317798));
#254160=CARTESIAN_POINT('Ctrl Pts',(-156.717639292002,4.90965193805665,
135.79772140676));
#254161=CARTESIAN_POINT('Ctrl Pts',(-156.996086915816,6.8548426487106,129.372764869687));
#254162=CARTESIAN_POINT('Ctrl Pts',(-157.274534539628,2.50076784287941,
124.263374887574));
#254163=CARTESIAN_POINT('Ctrl Pts',(-157.552982163441,-4.15139044125659,
125.164831246407));
#254164=CARTESIAN_POINT('Ctrl Pts',(-157.831429787254,-6.98862371657603,
131.248739591007));
#254165=CARTESIAN_POINT('Ctrl Pts',(-158.109877411067,-3.40365320961064,
136.924285368134));
#254166=CARTESIAN_POINT('Ctrl Pts',(-158.38832503488,3.30910831928323,136.975919274434));
#254167=CARTESIAN_POINT('Ctrl Pts',(-158.666772658693,6.98096096168483,
131.356192272474));
#254168=CARTESIAN_POINT('Ctrl Pts',(-158.945220282506,4.23765151920024,
125.229358938127));
#254169=CARTESIAN_POINT('Ctrl Pts',(-159.223667906319,-2.39985264864321,
124.225679793212));
#254170=CARTESIAN_POINT('Ctrl Pts',(-159.502115530131,-6.8320094717036,
129.267486939452));
#254171=CARTESIAN_POINT('Ctrl Pts',(-159.780563153944,-4.98588335248574,
135.721605915426));
#254172=CARTESIAN_POINT('Ctrl Pts',(-160.059010777757,1.44202599372318,
137.657016683454));
#254173=CARTESIAN_POINT('Ctrl Pts',(-160.33745840157,6.54478389858708,133.295171297791));
#254174=CARTESIAN_POINT('Ctrl Pts',(-160.615906025383,5.63320513111742,
126.644392579866));
#254175=CARTESIAN_POINT('Ctrl Pts',(-160.894353649196,-0.455013954479453,
123.816421262852));
#254176=CARTESIAN_POINT('Ctrl Pts',(-161.172801273009,-6.12509744457689,
127.410024833003));
#254177=CARTESIAN_POINT('Ctrl Pts',(-161.451248896821,-6.16651561075379,
134.122857166646));
#254178=CARTESIAN_POINT('Ctrl Pts',(-161.729696520635,-0.541207181682879,
137.786153289251));
#254179=CARTESIAN_POINT('Ctrl Pts',(-162.008144144447,5.58144420791359,
135.033523026113));
#254180=CARTESIAN_POINT('Ctrl Pts',(-162.286591768261,6.57502103914602,
128.394499115588));
#254181=CARTESIAN_POINT('Ctrl Pts',(-162.565039392073,1.52647474303778,
123.970020197102));
#254182=CARTESIAN_POINT('Ctrl Pts',(-162.843487015886,-4.92482726948487,
125.825966248931));
#254183=CARTESIAN_POINT('Ctrl Pts',(-163.121934639699,-6.85045361253876,
132.256813517449));
#254184=CARTESIAN_POINT('Ctrl Pts',(-163.400382263512,-2.48084774893327,
137.352927527244));
#254185=CARTESIAN_POINT('Ctrl Pts',(-163.678829887325,4.16853599979124,
136.431228462323));
#254186=CARTESIAN_POINT('Ctrl Pts',(-163.957277511138,6.98723880901292,
130.338712735846));
#254187=CARTESIAN_POINT('Ctrl Pts',(-164.23572513495,3.3850104983435,124.674104664506));
#254188=CARTESIAN_POINT('Ctrl Pts',(-164.514172758764,-3.32787709334726,
124.642902334375));
#254189=CARTESIAN_POINT('Ctrl Pts',(-164.792620382576,-6.98260821208591,
130.273779162525));
#254190=CARTESIAN_POINT('Ctrl Pts',(-165.07106800639,-4.22066350329308,
136.392234427513));
#254191=CARTESIAN_POINT('Ctrl Pts',(-165.349515630202,2.4198647741513,137.37570664397));
#254192=CARTESIAN_POINT('Ctrl Pts',(-165.627963254015,6.83665554111671,
132.320432890263));
#254193=CARTESIAN_POINT('Ctrl Pts',(-165.906410877828,4.97089385498702,
125.871962782194));
#254194=CARTESIAN_POINT('Ctrl Pts',(-166.184858501641,-1.46287644221077,
123.956125323802));
#254195=CARTESIAN_POINT('Ctrl Pts',(-166.463306125454,-6.55233475450377,
128.333481545486));
#254196=CARTESIAN_POINT('Ctrl Pts',(-166.741753749267,-5.62051752675643,
134.981454925258));
#254197=CARTESIAN_POINT('Ctrl Pts',(-167.020201373079,0.476280730534997,
137.790882698662));
#254198=CARTESIAN_POINT('Ctrl Pts',(-167.298648996893,6.13540026407138,
134.180037990117));
#254199=CARTESIAN_POINT('Ctrl Pts',(-167.577096620705,6.15638668589229,
127.467110687205));
#254200=CARTESIAN_POINT('Ctrl Pts',(-167.855544244518,0.519954499587912,
123.820953036571));
#254201=CARTESIAN_POINT('Ctrl Pts',(-168.133991868331,-5.5942904706483,
126.592205794446));
#254202=CARTESIAN_POINT('Ctrl Pts',(-168.412439492144,-6.56765579464175,
133.234223059563));
#254203=CARTESIAN_POINT('Ctrl Pts',(-168.690887115956,-1.50566629118217,
137.643315445865));
#254204=CARTESIAN_POINT('Ctrl Pts',(-168.96933473977,4.93995697798634,135.767742446477));
#254205=CARTESIAN_POINT('Ctrl Pts',(-169.247782363582,6.84600111470013,
129.331064021001));
#254206=CARTESIAN_POINT('Ctrl Pts',(-169.526229987396,2.46090467275213,
124.248273193229));
#254207=CARTESIAN_POINT('Ctrl Pts',(-169.804677611208,-4.18564294157836,
125.190206425745));
#254208=CARTESIAN_POINT('Ctrl Pts',(-170.083125235021,-6.98578917262369,
131.291273093865));
#254209=CARTESIAN_POINT('Ctrl Pts',(-170.361572858834,-3.36633642880185,
136.944890983262));
#254210=CARTESIAN_POINT('Ctrl Pts',(-170.640020482647,3.34661503841248,
136.955661448171));
#254211=CARTESIAN_POINT('Ctrl Pts',(-170.91846810646,6.98419077655865,131.313686957504));
#254212=CARTESIAN_POINT('Ctrl Pts',(-171.196915730273,4.20363638773547,
125.203666442409));
#254213=CARTESIAN_POINT('Ctrl Pts',(-171.475363354086,-2.43985448236259,
124.240410265162));
#254214=CARTESIAN_POINT('Ctrl Pts',(-171.753810977898,-6.84123827668714,
129.309103794972));
#254215=CARTESIAN_POINT('Ctrl Pts',(-172.032258601712,-4.9558583078063,
135.751865297389));
#254216=CARTESIAN_POINT('Ctrl Pts',(-172.310706225524,1.48371333881067,
137.648111698089));
#254217=CARTESIAN_POINT('Ctrl Pts',(-172.589153849337,6.55982491048677,
133.255285191615));
#254218=CARTESIAN_POINT('Ctrl Pts',(-172.86760147315,5.60777785468832,126.610178735912));
#254219=CARTESIAN_POINT('Ctrl Pts',(-173.146049096963,-0.497543094390354,
123.819320532272));
#254220=CARTESIAN_POINT('Ctrl Pts',(-173.424496720776,-6.14564624605571,
127.447372928838));
#254221=CARTESIAN_POINT('Ctrl Pts',(-173.702944344589,-6.14620072910595,
134.160333013378));
#254222=CARTESIAN_POINT('Ctrl Pts',(-173.981391968402,-0.498697000705985,
137.789318414533));
#254223=CARTESIAN_POINT('Ctrl Pts',(-174.259839592215,5.60708490864046,
134.999468834432));
#254224=CARTESIAN_POINT('Ctrl Pts',(-174.538287216028,6.56022970827155,
128.354519745462));
#254225=CARTESIAN_POINT('Ctrl Pts',(-174.81673483984,1.48484389103961,123.960854736574));
#254226=CARTESIAN_POINT('Ctrl Pts',(-175.095182463654,-4.95504092340126,
125.85603730847));
#254227=CARTESIAN_POINT('Ctrl Pts',(-175.373630087466,-6.8414851964426,
132.298487262391));
#254228=CARTESIAN_POINT('Ctrl Pts',(-175.652077711279,-2.44093879908611,
137.367907821863));
#254229=CARTESIAN_POINT('Ctrl Pts',(-175.930525335092,4.20271110814107,
136.405749147692));
#254230=CARTESIAN_POINT('Ctrl Pts',(-176.208972958905,6.98427482083815,
130.296188057377));
#254231=CARTESIAN_POINT('Ctrl Pts',(-176.487420582718,3.3476311739788,124.653612724266));
#254232=CARTESIAN_POINT('Ctrl Pts',(-176.765868206531,-3.36532198089259,
124.663274224357));
#254233=CARTESIAN_POINT('Ctrl Pts',(-177.044315830343,-6.98570864044213,
130.316294111058));
#254234=CARTESIAN_POINT('Ctrl Pts',(-177.322763454156,-4.18657033026512,
136.417823273865));
#254235=CARTESIAN_POINT('Ctrl Pts',(-177.601211077969,2.4598215880947,137.360854488428));
#254236=CARTESIAN_POINT('Ctrl Pts',(-177.879658701782,6.84575763596098,
132.278788138201));
#254237=CARTESIAN_POINT('Ctrl Pts',(-178.158106325595,4.94077685023126,
125.841794926299));
#254238=CARTESIAN_POINT('Ctrl Pts',(-178.436553949408,-1.50453649049278,
123.965157149858));
#254239=CARTESIAN_POINT('Ctrl Pts',(-178.715001573221,-6.56725429714808,
128.373413246577));
#254240=CARTESIAN_POINT('Ctrl Pts',(-178.993449197033,-5.59498623293233,
135.015591218853));
#254241=CARTESIAN_POINT('Ctrl Pts',(-179.271896820847,0.518800849074927,
137.787853998597));
#254242=CARTESIAN_POINT('Ctrl Pts',(-179.550344444659,6.15583529561319,
134.142627523792));
#254243=CARTESIAN_POINT('Ctrl Pts',(-179.828792068472,6.13595783475539,
127.429696845569));
#254244=CARTESIAN_POINT('Ctrl Pts',(-180.107239692285,0.477434881962636,
123.81791731232));
#254245=CARTESIAN_POINT('Ctrl Pts',(-180.385687316098,-5.61982740336347,
126.626337869861));
#254246=CARTESIAN_POINT('Ctrl Pts',(-180.664134939911,-6.55274284882976,
133.274157224785));
#254247=CARTESIAN_POINT('Ctrl Pts',(-180.942582563724,-1.4640077355066,
137.652354153945));
#254248=CARTESIAN_POINT('Ctrl Pts',(-181.221030187537,4.97007896599344,
135.737579566256));
#254249=CARTESIAN_POINT('Ctrl Pts',(-181.499477811349,6.83690589960112,
129.289417765863));
#254250=CARTESIAN_POINT('Ctrl Pts',(-181.777925435163,2.42095031289641,
124.233414437113));
#254251=CARTESIAN_POINT('Ctrl Pts',(-182.056373058975,-4.21974034136189,
125.215789639631));
#254252=CARTESIAN_POINT('Ctrl Pts',(-182.334820682789,-6.98269576768506,
131.333788554001));
#254253=CARTESIAN_POINT('Ctrl Pts',(-182.613268306601,-3.32889490715784,
136.965269058779));
#254254=CARTESIAN_POINT('Ctrl Pts',(-182.891715930414,3.38399774748988,
136.935175683191));
#254255=CARTESIAN_POINT('Ctrl Pts',(-183.170163554227,6.98716178967534,
131.27116276926));
#254256=CARTESIAN_POINT('Ctrl Pts',(-183.44861117804,4.16946548897866,125.178181482475));
#254257=CARTESIAN_POINT('Ctrl Pts',(-183.727058801853,-2.47976590637605,
124.255383966707));
#254258=CARTESIAN_POINT('Ctrl Pts',(-184.005506425666,-6.85021357707087,
129.350776057783));
#254259=CARTESIAN_POINT('Ctrl Pts',(-184.283954049479,-4.92564962197493,
135.781941347746));
#254260=CARTESIAN_POINT('Ctrl Pts',(-184.562401673291,1.52534570435398,
137.63895311501));
#254261=CARTESIAN_POINT('Ctrl Pts',(-184.840849297105,6.5746228456623,133.215308265529));
#254262=CARTESIAN_POINT('Ctrl Pts',(-185.119296920917,5.58214277998856,
126.576120308909));
#254263=CARTESIAN_POINT('Ctrl Pts',(-185.39774454473,-0.540053797659538,
123.822478634922));
#254264=CARTESIAN_POINT('Ctrl Pts',(-185.676192168543,-6.16596731835295,
127.484845419088));
#254265=CARTESIAN_POINT('Ctrl Pts',(-185.954639792356,-6.12565809773001,
134.197684503321));
#254266=CARTESIAN_POINT('Ctrl Pts',(-186.233087416169,-0.456168340327589,
137.792224709632));
#254267=CARTESIAN_POINT('Ctrl Pts',(-186.511535039982,5.63251783677319,
134.965259191474));
#254268=CARTESIAN_POINT('Ctrl Pts',(-186.789982663795,6.54519528567348,
128.314631155089));
#254269=CARTESIAN_POINT('Ctrl Pts',(-187.068430287608,1.44315801760525,
123.951942864674));
#254270=CARTESIAN_POINT('Ctrl Pts',(-187.346877911421,-4.98507096645316,
125.886291729948));
#254271=CARTESIAN_POINT('Ctrl Pts',(-187.625325535233,-6.83226326659722,
132.340105641921));
#254272=CARTESIAN_POINT('Ctrl Pts',(-187.903773159046,-2.40093939935397,
137.382644901827));
#254273=CARTESIAN_POINT('Ctrl Pts',(-188.182220782859,4.23673048348491,
136.380062271549));
#254274=CARTESIAN_POINT('Ctrl Pts',(-188.460668406672,6.98105202779173,
130.25368220943));
#254275=CARTESIAN_POINT('Ctrl Pts',(-188.739116030485,3.31012780190951,
124.633348702251));
#254276=CARTESIAN_POINT('Ctrl Pts',(-189.017563654298,-3.40264216519462,
124.683873674555));
#254277=CARTESIAN_POINT('Ctrl Pts',(-189.296011278111,-6.98855021079573,
130.358827145076));
#254278=CARTESIAN_POINT('Ctrl Pts',(-189.574458901924,-4.15232202233378,
136.443204111294));
#254279=CARTESIAN_POINT('Ctrl Pts',(-189.852906525736,2.49968725244504,
137.345759379595));
#254280=CARTESIAN_POINT('Ctrl Pts',(-190.13135414955,6.85460605873784,132.237088750687));
#254281=CARTESIAN_POINT('Ctrl Pts',(-190.409801773362,4.91047676317321,
125.8118109601));
#254282=CARTESIAN_POINT('Ctrl Pts',(-190.688249397175,-1.5461407876216,
123.974442405114));
#254283=CARTESIAN_POINT('Ctrl Pts',(-190.966697020988,-6.58193048776853,
128.413435027317));
#254284=CARTESIAN_POINT('Ctrl Pts',(-191.245144644801,-5.56924761483672,
135.049571463749));
#254285=CARTESIAN_POINT('Ctrl Pts',(-191.523592268614,0.561301743259386,
137.784566522618));
#254286=CARTESIAN_POINT('Ctrl Pts',(-191.802039892427,6.17604222041412,
134.105093356759));
#254287=CARTESIAN_POINT('Ctrl Pts',(-192.08048751624,6.11530161344434,127.39240805334));
#254288=CARTESIAN_POINT('Ctrl Pts',(-192.358935140053,0.43489757281158,
123.815140473294));
#254289=CARTESIAN_POINT('Ctrl Pts',(-192.637382763865,-5.64515609130746,
126.660624763449));
#254290=CARTESIAN_POINT('Ctrl Pts',(-192.915830387678,-6.53758708872167,
133.313999870785));
#254291=CARTESIAN_POINT('Ctrl Pts',(-193.194278011491,-1.42229493048546,
137.661139107108));
#254292=CARTESIAN_POINT('Ctrl Pts',(-193.472725635304,5.00001678589681,
135.707233883791));
#254293=CARTESIAN_POINT('Ctrl Pts',(-193.751173259117,6.82755734043935,
129.247827647489));
#254294=CARTESIAN_POINT('Ctrl Pts',(-194.02962088293,2.38090624383734,124.218799169824));
#254295=CARTESIAN_POINT('Ctrl Pts',(-194.308068506743,-4.25368137711504,
125.241579940071));
#254296=CARTESIAN_POINT('Ctrl Pts',(-194.586516130556,-6.97934361638637,
131.376284395991));
#254297=CARTESIAN_POINT('Ctrl Pts',(-194.864963754369,-3.29133003208973,
136.985418839569));
#254298=CARTESIAN_POINT('Ctrl Pts',(-195.143411378181,3.42125506128717,
136.914462738605));
#254299=CARTESIAN_POINT('Ctrl Pts',(-195.421859001994,6.98987389094189,
131.22862128349));
#254300=CARTESIAN_POINT('Ctrl Pts',(-195.700306625807,4.13514008914463,
125.152905002676));
#254301=CARTESIAN_POINT('Ctrl Pts',(-195.97875424962,-2.51958544175274,
124.270600342989));
#254302=CARTESIAN_POINT('Ctrl Pts',(-196.257201873433,-6.85893504027095,
129.392502183704));
#254303=CARTESIAN_POINT('Ctrl Pts',(-196.535649497246,-4.89525841438522,
135.811832952018));
#254304=CARTESIAN_POINT('Ctrl Pts',(-196.814097121059,1.56692154765205,
137.629541273595));
#254305=CARTESIAN_POINT('Ctrl Pts',(-197.092544744872,6.58917715577019,
133.175242000891));
#254306=CARTESIAN_POINT('Ctrl Pts',(-197.370992368684,5.55630085693524,
126.542218560906));
#254307=CARTESIAN_POINT('Ctrl Pts',(-197.649439992498,-0.582544489036021,
123.825895453776));
#254308=CARTESIAN_POINT('Ctrl Pts',(-197.92788761631,-6.18605990846357,
127.522440915193));
#254309=CARTESIAN_POINT('Ctrl Pts',(-198.206335240123,-6.10488847784037,
134.234910252398));
#254310=CARTESIAN_POINT('Ctrl Pts',(-198.484782863936,-0.413622776464342,
137.79487206686));
#254311=CARTESIAN_POINT('Ctrl Pts',(-198.763230487749,5.657742049887,134.930895364888));
#254312=CARTESIAN_POINT('Ctrl Pts',(-199.041678111562,6.52991832845634,
128.274834822558));
#254313=CARTESIAN_POINT('Ctrl Pts',(-199.320125735375,1.40141866741961,
123.943284911633));
#254314=CARTESIAN_POINT('Ctrl Pts',(-199.598573359188,-5.01491628586802,
125.916728392279));
#254315=CARTESIAN_POINT('Ctrl Pts',(-199.877020983,-6.82278816472322,132.381667113854));
#254316=CARTESIAN_POINT('Ctrl Pts',(-200.155468606814,-2.36085103192995,
137.397138221046));
#254317=CARTESIAN_POINT('Ctrl Pts',(-200.433916230626,4.27059286522247,
136.354168785731));
#254318=CARTESIAN_POINT('Ctrl Pts',(-200.712363854439,6.97757054929515,
130.211196767073));
#254319=CARTESIAN_POINT('Ctrl Pts',(-200.990811478252,3.27250177183757,
124.613313349352));
#254320=CARTESIAN_POINT('Ctrl Pts',(-201.269259102065,-3.43983626333961,
124.704699921646));
#254321=CARTESIAN_POINT('Ctrl Pts',(-201.547706725878,-6.9911328178512,
130.401376688499));
#254322=CARTESIAN_POINT('Ctrl Pts',(-201.826154349691,-4.1179198485831,
136.468375999304));
#254323=CARTESIAN_POINT('Ctrl Pts',(-202.104601973504,2.53946028996452,
137.330421876826));
#254324=CARTESIAN_POINT('Ctrl Pts',(-202.383049597317,6.86320048156709,
132.195336272904));
#254325=CARTESIAN_POINT('Ctrl Pts',(-202.66149722113,4.87999471659204,125.782011994664));
#254326=CARTESIAN_POINT('Ctrl Pts',(-202.939944844942,-1.5876877919352,
123.983980745501));
#254327=CARTESIAN_POINT('Ctrl Pts',(-203.218392468755,-6.59636278253501,
128.453545404684));
#254328=CARTESIAN_POINT('Ctrl Pts',(-203.496840092568,-5.54330262622176,
135.083394400798));
#254329=CARTESIAN_POINT('Ctrl Pts',(-203.775287716381,0.603781838200554,
137.781020392543));
#254330=CARTESIAN_POINT('Ctrl Pts',(-204.053735340194,6.19602028969954,
134.067436879861));
#254331=CARTESIAN_POINT('Ctrl Pts',(-204.332182964007,6.09441878738321,
127.355245692268));
#254332=CARTESIAN_POINT('Ctrl Pts',(-204.61063058782,0.392344148371673,
123.812622622391));
#254333=CARTESIAN_POINT('Ctrl Pts',(-204.889078211633,-5.67027559591653,
126.69506520469));
#254334=CARTESIAN_POINT('Ctrl Pts',(-205.167525835445,-6.5221890759199,
133.353749521179));
#254335=CARTESIAN_POINT('Ctrl Pts',(-205.445973459259,-1.38052942180316,
137.66966997982));
#254336=CARTESIAN_POINT('Ctrl Pts',(-205.724421083071,5.02976932833932,
135.676706523556));
#254337=CARTESIAN_POINT('Ctrl Pts',(-206.002868706884,6.8179557836299,129.206295207017));
#254338=CARTESIAN_POINT('Ctrl Pts',(-206.281316330697,2.340773949421,124.204427932937));
#254339=CARTESIAN_POINT('Ctrl Pts',(-206.55976395451,-4.28746479114066,
125.267576371395));
#254340=CARTESIAN_POINT('Ctrl Pts',(-206.838211578323,-6.97573284294384,
131.418759045136));
#254341=CARTESIAN_POINT('Ctrl Pts',(-207.116659202136,-3.253643195576,137.005339578972));
#254342=CARTESIAN_POINT('Ctrl Pts',(-207.395106825949,3.4583855992191,136.893523381939));
#254343=CARTESIAN_POINT('Ctrl Pts',(-207.673554449762,6.99232697986142,
131.186064076586));
#254344=CARTESIAN_POINT('Ctrl Pts',(-207.952002073574,4.10066146017411,
125.127837939644));
#254345=CARTESIAN_POINT('Ctrl Pts',(-208.230449697387,-2.55931161296347,
124.286058830161));
#254346=CARTESIAN_POINT('Ctrl Pts',(-208.5088973212,-6.86740234311116,129.434280626559));
#254347=CARTESIAN_POINT('Ctrl Pts',(-208.787344945013,-4.86468581119477,
135.841539002563));
#254348=CARTESIAN_POINT('Ctrl Pts',(-209.065792568826,1.60843932809579,
137.619876522599));
#254349=CARTESIAN_POINT('Ctrl Pts',(-209.344240192639,6.60348730149562,
133.135087882371));
#254350=CARTESIAN_POINT('Ctrl Pts',(-209.622687816452,5.53025304311036,
126.508474748144));
#254351=CARTESIAN_POINT('Ctrl Pts',(-209.901135440264,-0.625013594012848,
123.829570862223));
#254352=CARTESIAN_POINT('Ctrl Pts',(-210.179583064078,-6.20592327184948,
127.56015802404));
#254353=CARTESIAN_POINT('Ctrl Pts',(-210.45803068789,-6.08389263906328,
134.272008881199));
#254354=CARTESIAN_POINT('Ctrl Pts',(-210.736478311703,-0.371061885656257,
137.797260388114));
#254355=CARTESIAN_POINT('Ctrl Pts',(-211.014925935516,5.68275661328764,
134.896378628042));
#254356=CARTESIAN_POINT('Ctrl Pts',(-211.293373559329,6.51439940271492,
128.235132222534));
#254357=CARTESIAN_POINT('Ctrl Pts',(-211.571821183142,1.35962738715011,
123.934881198276));
#254358=CARTESIAN_POINT('Ctrl Pts',(-211.850268806955,-5.04457577571481,
125.947346167619));
#254359=CARTESIAN_POINT('Ctrl Pts',(-212.128716430768,-6.81306024192543,
132.423170138115));
#254360=CARTESIAN_POINT('Ctrl Pts',(-212.40716405458,-2.32067518230222,
137.411387242468));
#254361=CARTESIAN_POINT('Ctrl Pts',(-212.685611678394,4.30429699857105,
136.32806964973));
#254362=CARTESIAN_POINT('Ctrl Pts',(-212.964059302206,6.97383051435588,
130.168733304621));
#254363=CARTESIAN_POINT('Ctrl Pts',(-213.24250692602,3.23475447800865,124.593507407987));
#254364=CARTESIAN_POINT('Ctrl Pts',(-213.520954549832,-3.47690289708716,
124.725752193909));
#254365=CARTESIAN_POINT('Ctrl Pts',(-213.799402173646,-6.99345636590915,
130.443941164641));
#254366=CARTESIAN_POINT('Ctrl Pts',(-214.077849797458,-4.08336508379785,
136.49333800514));
#254367=CARTESIAN_POINT('Ctrl Pts',(-214.356297421271,2.57913922684953,
137.314842548456));
#254368=CARTESIAN_POINT('Ctrl Pts',(-214.634745045084,6.87154058597789,
132.153532252007));
#254369=CARTESIAN_POINT('Ctrl Pts',(-214.913192668897,4.84933184001288,
125.752399134204));
#254370=CARTESIAN_POINT('Ctrl Pts',(-215.19164029271,-1.62917596389355,
123.993771817573));
#254371=CARTESIAN_POINT('Ctrl Pts',(-215.470087916522,-6.61055064665203,
128.493742892374));
#254372=CARTESIAN_POINT('Ctrl Pts',(-215.748535540335,-5.51715222849034,
135.117058776675));
#254373=CARTESIAN_POINT('Ctrl Pts',(-216.026983164148,0.646239559784443,
137.777215739773));
#254374=CARTESIAN_POINT('Ctrl Pts',(-216.305430787961,6.21576876317433,
134.029659488472));
#254375=CARTESIAN_POINT('Ctrl Pts',(-216.583878411774,6.0733101303926,127.318211139417));
#254376=CARTESIAN_POINT('Ctrl Pts',(-216.862326035587,0.349776185474419,
123.810363852911));
#254377=CARTESIAN_POINT('Ctrl Pts',(-217.1407736594,-5.69518498637811,126.729657917385));
#254378=CARTESIAN_POINT('Ctrl Pts',(-217.419221283213,-6.50654938100331,
133.393404703032));
#254379=CARTESIAN_POINT('Ctrl Pts',(-217.697668907026,-1.33871275709491,
137.67794645597));
#254380=CARTESIAN_POINT('Ctrl Pts',(-217.976116530838,5.05933549082977,
135.64599861675));
#254381=CARTESIAN_POINT('Ctrl Pts',(-218.254564154652,6.80810158496121,
129.164821983446));
#254382=CARTESIAN_POINT('Ctrl Pts',(-218.533011778464,2.30055491676597,
124.190301258982));
#254383=CARTESIAN_POINT('Ctrl Pts',(-218.811459402277,-4.32108933158155,
125.293777970294));
#254384=CARTESIAN_POINT('Ctrl Pts',(-219.08990702609,-6.97186358115499,
131.461210927519));
#254385=CARTESIAN_POINT('Ctrl Pts',(-219.368354649903,-3.21583579411804,
137.02503053882));
#254386=CARTESIAN_POINT('Ctrl Pts',(-219.646802273716,3.49538798540175,
136.872358389107));
#254387=CARTESIAN_POINT('Ctrl Pts',(-219.925249897529,6.99452096553273,
131.143492725519));
#254388=CARTESIAN_POINT('Ctrl Pts',(-220.203697521342,4.06603087968498,
125.102981222246));
#254389=CARTESIAN_POINT('Ctrl Pts',(-220.482145145155,-2.59894294794204,
124.301758855404));
#254390=CARTESIAN_POINT('Ctrl Pts',(-220.760592768967,-6.87561517183164,
129.476109838232));
#254391=CARTESIAN_POINT('Ctrl Pts',(-221.03904039278,-4.83393294528274,
135.87105839861));
#254392=CARTESIAN_POINT('Ctrl Pts',(-221.317488016593,1.64989750722823,
137.609959220154));
#254393=CARTESIAN_POINT('Ctrl Pts',(-221.595935640406,6.61755275257056,
133.094847397895));
#254394=CARTESIAN_POINT('Ctrl Pts',(-221.874383264219,5.5040003037252,126.474890121013));
#254395=CARTESIAN_POINT('Ctrl Pts',(-222.152830888031,-0.667459538880483,
123.83350472407));
#254396=CARTESIAN_POINT('Ctrl Pts',(-222.431278511845,-6.22555667246622,
127.597995348007));
#254397=CARTESIAN_POINT('Ctrl Pts',(-222.709726135657,-6.06267135940695,
134.308979015016));
#254398=CARTESIAN_POINT('Ctrl Pts',(-222.988173759471,-0.328487245014279,
137.799389584896));
#254399=CARTESIAN_POINT('Ctrl Pts',(-223.266621383283,5.70756060005303,
134.861710259961));
#254400=CARTESIAN_POINT('Ctrl Pts',(-223.545069007096,6.49863908350723,
128.195524826214));
#254401=CARTESIAN_POINT('Ctrl Pts',(-223.823516630909,1.31778572538753,
123.926732036005));
#254402=CARTESIAN_POINT('Ctrl Pts',(-224.101964254722,-5.07404833695195,
125.978143921416));
#254403=CARTESIAN_POINT('Ctrl Pts',(-224.380411878535,-6.80307985867417,
132.464613176793));
#254404=CARTESIAN_POINT('Ctrl Pts',(-224.658859502348,-2.28041333920269,
137.425391438088));
#254405=CARTESIAN_POINT('Ctrl Pts',(-224.937307126161,4.33784163461131,
136.30176583066));
#254406=CARTESIAN_POINT('Ctrl Pts',(-225.215754749974,6.96983206156226,
130.126293395573));
#254407=CARTESIAN_POINT('Ctrl Pts',(-225.494202373786,3.19688731916334,
124.573931612073));
#254408=CARTESIAN_POINT('Ctrl Pts',(-225.7726499976,-3.51384069291894,124.747029711241));
#254409=CARTESIAN_POINT('Ctrl Pts',(-226.051097621412,-6.9955207688696,
130.486518996257));
#254410=CARTESIAN_POINT('Ctrl Pts',(-226.329545245225,-4.04865900841799,
136.518089203828));
#254411=CARTESIAN_POINT('Ctrl Pts',(-226.607992869038,2.61872259278156,
137.299021971784));
#254412=CARTESIAN_POINT('Ctrl Pts',(-226.886440492851,6.87962606292594,
132.111678237058));
#254413=CARTESIAN_POINT('Ctrl Pts',(-227.164888116664,4.81848926965818,
125.722973476035));
#254414=CARTESIAN_POINT('Ctrl Pts',(-227.443335740477,-1.67060376613766,
124.003815258517));
#254415=CARTESIAN_POINT('Ctrl Pts',(-227.72178336429,-6.62449355438458,
128.534026000853));
#254416=CARTESIAN_POINT('Ctrl Pts',(-228.000230988102,-5.49079739065326,
135.150563343936));
#254417=CARTESIAN_POINT('Ctrl Pts',(-228.278678611916,0.688673334723007,
137.773152705292));
#254418=CARTESIAN_POINT('Ctrl Pts',(-228.557126235728,6.23528690905198,
133.991762582447));
#254419=CARTESIAN_POINT('Ctrl Pts',(-228.835573859542,6.05197642466173,
127.281305767118));
#254420=CARTESIAN_POINT('Ctrl Pts',(-229.114021483354,0.307195261492642,
123.808364248553));
#254421=CARTESIAN_POINT('Ctrl Pts',(-229.392469107167,-5.7198833396657,
126.764401619687));
#254422=CARTESIAN_POINT('Ctrl Pts',(-229.670916730979,-6.49066858350677,
133.432963946903));
#254423=CARTESIAN_POINT('Ctrl Pts',(-229.949364354793,-1.29684648589306,
137.685968228869));
#254424=CARTESIAN_POINT('Ctrl Pts',(-230.227811978605,5.0887141777831,135.615111301269));
#254425=CARTESIAN_POINT('Ctrl Pts',(-230.506259602419,6.79799510958498,
129.123409513582));
#254426=CARTESIAN_POINT('Ctrl Pts',(-230.784707226231,2.26025063620168,
124.176419671429));
#254427=CARTESIAN_POINT('Ctrl Pts',(-231.063154850045,-4.35455375246839,
125.32018376586));
#254428=CARTESIAN_POINT('Ctrl Pts',(-231.341602473857,-6.96773597439774,
131.503638470075));
#254429=CARTESIAN_POINT('Ctrl Pts',(-231.62005009767,-3.17790922868121,
137.044490989456));
#254430=CARTESIAN_POINT('Ctrl Pts',(-231.898497721483,3.53226084869627,
136.850968544386));
#254431=CARTESIAN_POINT('Ctrl Pts',(-232.176945345296,6.99645576665798,
131.100908807788));
#254432=CARTESIAN_POINT('Ctrl Pts',(-232.455392969109,4.03124963092651,
125.078335771559));
#254433=CARTESIAN_POINT('Ctrl Pts',(-232.733840592922,-2.63847797813309,
124.317699836946));
#254434=CARTESIAN_POINT('Ctrl Pts',(-233.012288216734,-6.88357322210384,
129.517988268725));
#254435=CARTESIAN_POINT('Ctrl Pts',(-233.290735840548,-4.80300095620762,
135.900390046307));
#254436=CARTESIAN_POINT('Ctrl Pts',(-233.56918346436,1.6912945488023,137.599789733751));
#254437=CARTESIAN_POINT('Ctrl Pts',(-233.847631088173,6.63137298779474,
133.05452203859));
#254438=CARTESIAN_POINT('Ctrl Pts',(-234.126078711986,5.47754361158473,
126.441465924004));
#254439=CARTESIAN_POINT('Ctrl Pts',(-234.404526335799,-0.709880750790079,
123.837696893545));
#254440=CARTESIAN_POINT('Ctrl Pts',(-234.682973959612,-6.24495938279112,
127.635951485018));
#254441=CARTESIAN_POINT('Ctrl Pts',(-234.961421583425,-6.04122542523402,
134.345819283911));
#254442=CARTESIAN_POINT('Ctrl Pts',(-235.239869207238,-0.285900432155891,
137.801259578306));
#254443=CARTESIAN_POINT('Ctrl Pts',(-235.518316831051,5.73215309106056,
134.826891545298));
#254444=CARTESIAN_POINT('Ctrl Pts',(-235.796764454864,6.48263795483918,
128.156014101264));
#254445=CARTESIAN_POINT('Ctrl Pts',(-236.075212078676,1.27589523259052,
123.918837726791));
#254446=CARTESIAN_POINT('Ctrl Pts',(-236.353659702489,-5.10333287746112,
126.009120512446));
#254447=CARTESIAN_POINT('Ctrl Pts',(-236.632107326302,-6.79284738479763,
132.505994694203));
#254448=CARTESIAN_POINT('Ctrl Pts',(-236.910554950115,-2.24006699454776,
137.439150288976));
#254449=CARTESIAN_POINT('Ctrl Pts',(-237.189002573928,4.3712255303347,136.275258303218));
#254450=CARTESIAN_POINT('Ctrl Pts',(-237.467450197741,6.96557533907847,
130.083878612554));
#254451=CARTESIAN_POINT('Ctrl Pts',(-237.745897821554,3.15890169848239,
124.554586686994));
#254452=CARTESIAN_POINT('Ctrl Pts',(-238.024345445366,-3.55064828209192,
124.768531685198));
#254453=CARTESIAN_POINT('Ctrl Pts',(-238.30279306918,-6.99732595023538,
130.529108605612));
#254454=CARTESIAN_POINT('Ctrl Pts',(-238.581240692992,-4.01380290848946,
136.542628678202));
#254455=CARTESIAN_POINT('Ctrl Pts',(-238.859688316805,2.65820892098533,
137.282960733047));
#254456=CARTESIAN_POINT('Ctrl Pts',(-239.138135940618,6.88745661279959,
132.069775778975));
#254457=CARTESIAN_POINT('Ctrl Pts',(-239.416583564431,4.78746814841248,
125.693736110535));
#254458=CARTESIAN_POINT('Ctrl Pts',(-239.695031188244,-1.71196966354462,
124.014110696169));
#254459=CARTESIAN_POINT('Ctrl Pts',(-239.973478812057,-6.63819098907155,
128.574393237416));
#254460=CARTESIAN_POINT('Ctrl Pts',(-240.25192643587,-5.46423908930053,
135.183906861057));
#254461=CARTESIAN_POINT('Ctrl Pts',(-240.530374059683,0.731081590618679,
137.768831439659));
#254462=CARTESIAN_POINT('Ctrl Pts',(-240.808821683496,6.25457400407998,
133.95374756607));
#254463=CARTESIAN_POINT('Ctrl Pts',(-241.087269307308,6.03041846071876,
127.244530942912));
#254464=CARTESIAN_POINT('Ctrl Pts',(-241.365716931122,0.264602954276818,
123.806623883412));
#254465=CARTESIAN_POINT('Ctrl Pts',(-241.644164554934,-5.74436974057257,
126.799295024156));
#254466=CARTESIAN_POINT('Ctrl Pts',(-241.922612178747,-6.47454727189872,
133.472425786911));
#254467=CARTESIAN_POINT('Ctrl Pts',(-242.20105980256,-1.25493215956847,
137.693735001267));
#254468=CARTESIAN_POINT('Ctrl Pts',(-242.479507426373,5.11790430056101,
135.584045721651));
#254469=CARTESIAN_POINT('Ctrl Pts',(-242.757955050186,6.78763673199965,
129.082059331979));
#254470=CARTESIAN_POINT('Ctrl Pts',(-243.036402673998,2.21986260121965,
124.162783684665));
#254471=CARTESIAN_POINT('Ctrl Pts',(-243.314850297812,-4.38785681376436,
125.346792779616));
#254472=CARTESIAN_POINT('Ctrl Pts',(-243.593297921624,-6.96335017562108,
131.54604010063));
#254473=CARTESIAN_POINT('Ctrl Pts',(-243.871745545438,-3.13986490465013,
137.063720209766));
#254474=CARTESIAN_POINT('Ctrl Pts',(-244.15019316925,3.56900282276695,136.829354640385));
#254475=CARTESIAN_POINT('Ctrl Pts',(-244.428640793064,6.99813131154132,
131.058313901354));
#254476=CARTESIAN_POINT('Ctrl Pts',(-244.707088416876,3.99631900273028,
125.053902500829));
#254477=CARTESIAN_POINT('Ctrl Pts',(-244.985536040689,-2.67791523855318,
124.333881184089));
#254478=CARTESIAN_POINT('Ctrl Pts',(-245.263983664501,-6.89127619903846,
129.559914366219));
#254479=CARTESIAN_POINT('Ctrl Pts',(-245.542431288315,-4.7718909901659,
135.929532858758));
#254480=CARTESIAN_POINT('Ctrl Pts',(-245.820878912128,1.73262891883438,
137.589368440225));
#254481=CARTESIAN_POINT('Ctrl Pts',(-246.09932653594,6.6449474950541,133.014113298726));
#254482=CARTESIAN_POINT('Ctrl Pts',(-246.377774159753,5.45088394705135,
126.408203395661));
#254483=CARTESIAN_POINT('Ctrl Pts',(-246.656221783566,-0.752275657806765,
123.842147215306));
#254484=CARTESIAN_POINT('Ctrl Pts',(-246.934669407379,-6.26413068384941,
127.674025028594));
#254485=CARTESIAN_POINT('Ctrl Pts',(-247.213117031192,-6.01955563123113,
134.382528322752));
#254486=CARTESIAN_POINT('Ctrl Pts',(-247.491564655005,-0.243303025152602,
137.802870299053));
#254487=CARTESIAN_POINT('Ctrl Pts',(-247.770012278818,5.75653317502817,
134.791923774272));
#254488=CARTESIAN_POINT('Ctrl Pts',(-248.048459902631,6.46639660963695,
128.116601511768));
#254489=CARTESIAN_POINT('Ctrl Pts',(-248.326907526444,1.23395746102625,
123.91119856316));
#254490=CARTESIAN_POINT('Ctrl Pts',(-248.605355150257,-5.13242831209467,
126.040274792862));
#254491=CARTESIAN_POINT('Ctrl Pts',(-248.883802774069,-6.78236319946242,
132.547313156937));
#254492=CARTESIAN_POINT('Ctrl Pts',(-249.162250397883,-2.19963764338714,
137.452663285294));
#254493=CARTESIAN_POINT('Ctrl Pts',(-249.440698021695,4.40444744868852,
136.24854804965));
#254494=CARTESIAN_POINT('Ctrl Pts',(-249.719145645508,6.96106050463867,
130.041490527264));
#254495=CARTESIAN_POINT('Ctrl Pts',(-249.997593269321,3.12079902353814,
124.535473349588));
#254496=CARTESIAN_POINT('Ctrl Pts',(-250.276040893134,-3.58732430068758,
124.790257319018));
#254497=CARTESIAN_POINT('Ctrl Pts',(-250.554488516946,-6.99887184311352,
130.571708414529));
#254498=CARTESIAN_POINT('Ctrl Pts',(-250.83293614076,-3.97879807562073,
136.566955518948));
#254499=CARTESIAN_POINT('Ctrl Pts',(-251.111383764572,2.69759674828547,
137.26665942739));
#254500=CARTESIAN_POINT('Ctrl Pts',(-251.389831388386,6.89503194542569,
132.027826430486));
#254501=CARTESIAN_POINT('Ctrl Pts',(-251.668279012198,4.75626962579305,
125.66468812107));
#254502=CARTESIAN_POINT('Ctrl Pts',(-251.946726636011,-1.75327212332407,
124.024657749096));
#254503=CARTESIAN_POINT('Ctrl Pts',(-252.225174259824,-6.65164244307981,
128.614843106116));
#254504=CARTESIAN_POINT('Ctrl Pts',(-252.503621883637,-5.43747830869239,
135.217088092717));
#254505=CARTESIAN_POINT('Ctrl Pts',(-252.78206950745,0.773462756270139,
137.764252102553));
#254506=CARTESIAN_POINT('Ctrl Pts',(-253.060517131263,6.2736293330892,133.91561584884));
#254507=CARTESIAN_POINT('Ctrl Pts',(-253.338964755075,6.00863703830687,
127.207888027921));
#254508=CARTESIAN_POINT('Ctrl Pts',(-253.617412378889,0.222000840393564,
123.805142824969));
#254509=CARTESIAN_POINT('Ctrl Pts',(-253.895860002702,-5.76864327852066,
126.83433683216));
#254510=CARTESIAN_POINT('Ctrl Pts',(-254.174307626514,-6.45818604965135,
133.511788771436));
#254511=CARTESIAN_POINT('Ctrl Pts',(-254.452755250327,-1.21297131977014,
137.701246465247));
#254512=CARTESIAN_POINT('Ctrl Pts',(-254.73120287414,5.14690475579816,135.55280306703));
#254513=CARTESIAN_POINT('Ctrl Pts',(-255.009650497953,6.7770268770417,129.040772899161));
#254514=CARTESIAN_POINT('Ctrl Pts',(-255.288098121766,2.17939223099114,
124.149393939406));
#254515=CARTESIAN_POINT('Ctrl Pts',(-255.566545745579,-4.42099713522674,
125.37360376984));
#254516=CARTESIAN_POINT('Ctrl Pts',(-255.844993369392,-6.95870662337211,
131.588414730824));
#254517=CARTESIAN_POINT('Ctrl Pts',(-256.123440993205,-3.10170371057109,
137.082716575498));
#254518=CARTESIAN_POINT('Ctrl Pts',(-256.401888617018,3.60561156199617,
136.807519199501));
#254519=CARTESIAN_POINT('Ctrl Pts',(-256.68033624083,6.99954939633056,131.01570633407));
#254520=CARTESIAN_POINT('Ctrl Pts',(-256.958783864643,3.96123678073902,
125.029688453078));
#254521=CARTESIAN_POINT('Ctrl Pts',(-257.237231488456,-2.71724664265218,
124.350290708114));
#254522=CARTESIAN_POINT('Ctrl Pts',(-257.515679112269,-6.89873632689917,
129.601908459729));
#254523=CARTESIAN_POINT('Ctrl Pts',(-257.794126736082,-4.74058057908887,
135.958444437253));
#254524=CARTESIAN_POINT('Ctrl Pts',(-258.072574359895,1.77385448465437,
137.578773744179));
#254525=CARTESIAN_POINT('Ctrl Pts',(-258.351021983707,6.6583599873155,132.973475360041));
#254526=CARTESIAN_POINT('Ctrl Pts',(-258.629469607521,5.42386327951784,
126.375381938049));
#254527=CARTESIAN_POINT('Ctrl Pts',(-258.907917231333,-0.794342416617398,
123.846330221273));
#254528=CARTESIAN_POINT('Ctrl Pts',(-259.186364855146,-6.28363694765996,
127.713206958712));
#254529=CARTESIAN_POINT('Ctrl Pts',(-259.464812478959,-5.99659113747434,
134.41722675292));
#254530=CARTESIAN_POINT('Ctrl Pts',(-259.743260102772,-0.202727240537578,
137.807801967267));
#254531=CARTESIAN_POINT('Ctrl Pts',(-260.021707726585,5.7845923739281,134.749768174183));
#254532=CARTESIAN_POINT('Ctrl Pts',(-260.253747413096,6.33253704604016,
129.202365411857));
#254533=CARTESIAN_POINT('Ctrl Pts',(-260.439389088604,3.82430165355141,
125.973250269562));
#254534=CARTESIAN_POINT('Ctrl Pts',(-260.532214889509,1.97943258085903,
125.138073123498));
#254535=CARTESIAN_POINT('Ctrl Pts',(-260.578632753112,1.00712299976162,
124.970230583726));
#254536=CARTESIAN_POINT('',(-177.785171091631,5.06474445112881,133.863166627639));
#254537=CARTESIAN_POINT('',(-177.476367722506,5.12014273339247,130.804360617566));
#254538=CARTESIAN_POINT('Ctrl Pts',(-177.786046227816,5.06143466734273,
133.861215740604));
#254539=CARTESIAN_POINT('Ctrl Pts',(-177.742821434039,5.08507708225877,
133.650067943741));
#254540=CARTESIAN_POINT('Ctrl Pts',(-177.704041383372,5.10684921384841,
133.437850811182));
#254541=CARTESIAN_POINT('Ctrl Pts',(-177.627101194856,5.14805987156466,
132.959434264776));
#254542=CARTESIAN_POINT('Ctrl Pts',(-177.591430156013,5.16562332921322,
132.692970957434));
#254543=CARTESIAN_POINT('Ctrl Pts',(-177.51826800244,5.18983313181224,132.008875337098));
#254544=CARTESIAN_POINT('Ctrl Pts',(-177.491889782598,5.18373170393937,
131.607069645772));
#254545=CARTESIAN_POINT('Ctrl Pts',(-177.478015568181,5.14508328177199,
131.063381533424));
#254546=CARTESIAN_POINT('Ctrl Pts',(-177.476367722506,5.13366996699167,
130.933750143363));
#254547=CARTESIAN_POINT('Ctrl Pts',(-177.476367722506,5.1201427333925,130.804360617566));
#254548=CARTESIAN_POINT('',(-178.183936147798,3.7463393230346,126.224944438273));
#254549=CARTESIAN_POINT('Ctrl Pts',(-177.785171091631,5.06474445112881,
133.863166627639));
#254550=CARTESIAN_POINT('Ctrl Pts',(-177.792868498275,5.14945412057303,
133.722905091974));
#254551=CARTESIAN_POINT('Ctrl Pts',(-177.800565904919,5.228288425839,133.579195727341));
#254552=CARTESIAN_POINT('Ctrl Pts',(-177.808263311562,5.30097891580062,
133.43258303904));
#254553=CARTESIAN_POINT('Ctrl Pts',(-177.815673272437,5.37095491050639,
133.291445337178));
#254554=CARTESIAN_POINT('Ctrl Pts',(-177.823083233312,5.43523756743315,
133.147617601296));
#254555=CARTESIAN_POINT('Ctrl Pts',(-177.830493194186,5.49363698048319,
133.001605093988));
#254556=CARTESIAN_POINT('Ctrl Pts',(-177.837908263093,5.552076650981,132.855491933428));
#254557=CARTESIAN_POINT('Ctrl Pts',(-177.845323332,5.60462487314325,132.707191351285));
#254558=CARTESIAN_POINT('Ctrl Pts',(-177.852738400907,5.65114171470356,
132.557223385394));
#254559=CARTESIAN_POINT('Ctrl Pts',(-177.86016325716,5.69771995507294,132.407057472819));
#254560=CARTESIAN_POINT('Ctrl Pts',(-177.867588113413,5.73825082931068,
132.255220142398));
#254561=CARTESIAN_POINT('Ctrl Pts',(-177.875012969665,5.77264542002059,
132.102241743562));
#254562=CARTESIAN_POINT('Ctrl Pts',(-177.875855303563,5.77654741201243,
132.084886674789));
#254563=CARTESIAN_POINT('Ctrl Pts',(-177.87669763746,5.78037048244532,132.067516925213));
#254564=CARTESIAN_POINT('Ctrl Pts',(-177.877539971357,5.78411454368991,
132.050133272578));
#254565=CARTESIAN_POINT('Ctrl Pts',(-177.884963237763,5.8171099676497,131.8969357282));
#254566=CARTESIAN_POINT('Ctrl Pts',(-177.892386504168,5.8440647157557,131.742194755227));
#254567=CARTESIAN_POINT('Ctrl Pts',(-177.899809770574,5.8648359806621,131.586428058668));
#254568=CARTESIAN_POINT('Ctrl Pts',(-177.907224263295,5.88558269565839,
131.430845465408));
#254569=CARTESIAN_POINT('Ctrl Pts',(-177.914638756016,5.90016042593303,
131.2742399281));
#254570=CARTESIAN_POINT('Ctrl Pts',(-177.922053248737,5.9084768456705,131.117141573948));
#254571=CARTESIAN_POINT('Ctrl Pts',(-177.929460595091,5.91678524972953,
130.960194637105));
#254572=CARTESIAN_POINT('Ctrl Pts',(-177.936867941444,5.91884433792154,
130.802756199313));
#254573=CARTESIAN_POINT('Ctrl Pts',(-177.944275287798,5.91461330392028,
130.645363675491));
#254574=CARTESIAN_POINT('Ctrl Pts',(-177.951677109474,5.91038542558379,
130.488088540951));
#254575=CARTESIAN_POINT('Ctrl Pts',(-177.959078931149,5.89987677627349,
130.330859623753));
#254576=CARTESIAN_POINT('Ctrl Pts',(-177.966480752825,5.88309857495091,
130.174216411919));
#254577=CARTESIAN_POINT('Ctrl Pts',(-177.973878667136,5.86632923071016,
130.017655890817));
#254578=CARTESIAN_POINT('Ctrl Pts',(-177.981276581447,5.84329696543529,
129.861680829548));
#254579=CARTESIAN_POINT('Ctrl Pts',(-177.988674495759,5.81406499171618,
129.706827549909));
#254580=CARTESIAN_POINT('Ctrl Pts',(-177.996071180671,5.78483787582098,
129.552000004077));
#254581=CARTESIAN_POINT('Ctrl Pts',(-178.003467865583,5.74941316545811,
129.398294236346));
#254582=CARTESIAN_POINT('Ctrl Pts',(-178.010864550496,5.7079055513191,129.246238420907));
#254583=CARTESIAN_POINT('Ctrl Pts',(-178.018260907431,5.66639977767119,
129.094189347783));
#254584=CARTESIAN_POINT('Ctrl Pts',(-178.025657264366,5.61881173485076,
128.943790441604));
#254585=CARTESIAN_POINT('Ctrl Pts',(-178.033053621302,5.56530649258155,
128.7955564444));
#254586=CARTESIAN_POINT('Ctrl Pts',(-178.040451110638,5.51179305852316,
128.647299752193));
#254587=CARTESIAN_POINT('Ctrl Pts',(-178.047848599975,5.45236074791929,
128.501208980075));
#254588=CARTESIAN_POINT('Ctrl Pts',(-178.055246089312,5.38722339221779,
128.357780415561));
#254589=CARTESIAN_POINT('Ctrl Pts',(-178.062646171827,5.3220632027175,128.214301572387));
#254590=CARTESIAN_POINT('Ctrl Pts',(-178.070046254342,5.25119414060659,
128.073487134552));
#254591=CARTESIAN_POINT('Ctrl Pts',(-178.077446336857,5.1748766688598,127.935810108234));
#254592=CARTESIAN_POINT('Ctrl Pts',(-178.084854556523,5.0984752782071,127.797981691871));
#254593=CARTESIAN_POINT('Ctrl Pts',(-178.09226277619,5.01661369441823,127.663297903407));
#254594=CARTESIAN_POINT('Ctrl Pts',(-178.099670995856,4.92959690775233,
127.532204617376));
#254595=CARTESIAN_POINT('Ctrl Pts',(-178.107083775158,4.84252656370595,
127.401030645615));
#254596=CARTESIAN_POINT('Ctrl Pts',(-178.11449655446,4.75029491249686,127.273451881598));
#254597=CARTESIAN_POINT('Ctrl Pts',(-178.121909333762,4.65324782702301,
127.14988182808));
#254598=CARTESIAN_POINT('Ctrl Pts',(-178.129332704791,4.55606207612225,
127.026135211873));
#254599=CARTESIAN_POINT('Ctrl Pts',(-178.13675607582,4.45404739048349,126.906409029321));
#254600=CARTESIAN_POINT('Ctrl Pts',(-178.144179446849,4.34758769447436,
126.791081185312));
#254601=CARTESIAN_POINT('Ctrl Pts',(-178.148115496289,4.29114020918847,
126.729931595168));
#254602=CARTESIAN_POINT('Ctrl Pts',(-178.15205154573,4.23344365617117,126.670017889433));
#254603=CARTESIAN_POINT('Ctrl Pts',(-178.15598759517,4.17455901249308,126.611391787046));
#254604=CARTESIAN_POINT('Ctrl Pts',(-178.163412098033,4.0634859144098,126.500806370986));
#254605=CARTESIAN_POINT('Ctrl Pts',(-178.170836600896,3.94784763173947,
126.394470301888));
#254606=CARTESIAN_POINT('Ctrl Pts',(-178.178261103759,3.82800271599344,
126.292783756994));
#254607=CARTESIAN_POINT('Ctrl Pts',(-178.1797891116,3.80333790351263,126.271856047662));
#254608=CARTESIAN_POINT('Ctrl Pts',(-178.18131711944,3.77849505168981,126.251125163909));
#254609=CARTESIAN_POINT('Ctrl Pts',(-178.18284512728,3.75347749648132,126.230594418261));
#254610=CARTESIAN_POINT('Ctrl Pts',(-177.476367722506,5.1201427333925,130.804360617566));
#254611=CARTESIAN_POINT('Ctrl Pts',(-177.476367722506,5.0948783866862,130.5627042718));
#254612=CARTESIAN_POINT('Ctrl Pts',(-177.48211809202,5.06224363656916,130.321891244269));
#254613=CARTESIAN_POINT('Ctrl Pts',(-177.495355899915,5.01616195097393,
130.042752414703));
#254614=CARTESIAN_POINT('Ctrl Pts',(-177.497386085719,5.00943885560551,
130.003205734465));
#254615=CARTESIAN_POINT('Ctrl Pts',(-177.499617454833,5.00237413411682,
129.962810309717));
#254616=CARTESIAN_POINT('Ctrl Pts',(-177.499666670813,5.00221846150168,
129.961920748202));
#254617=CARTESIAN_POINT('Ctrl Pts',(-177.499730694524,5.00201614547379,
129.960765378705));
#254618=CARTESIAN_POINT('Ctrl Pts',(-177.499745432065,5.00196958791774,
129.960499551648));
#254619=CARTESIAN_POINT('Ctrl Pts',(-177.499769029077,5.00189506362177,
129.960074124391));
#254620=CARTESIAN_POINT('Ctrl Pts',(-177.499777884095,5.00186710242369,
129.959914523897));
#254621=CARTESIAN_POINT('Ctrl Pts',(-177.499794570173,5.00181442238816,
129.95961386397));
#254622=CARTESIAN_POINT('Ctrl Pts',(-177.499802400734,5.00178970407401,
129.959472803585));
#254623=CARTESIAN_POINT('Ctrl Pts',(-177.499820020531,5.00173409303354,
129.959155478821));
#254624=CARTESIAN_POINT('Ctrl Pts',(-177.499829810846,5.00170319900482,
129.958979214899));
#254625=CARTESIAN_POINT('Ctrl Pts',(-177.49985857684,5.00161244305434,129.958461477023));
#254626=CARTESIAN_POINT('Ctrl Pts',(-177.499877560812,5.00155257106515,
129.958120006032));
#254627=CARTESIAN_POINT('Ctrl Pts',(-177.500018881264,5.00110703522932,
129.955579570966));
#254628=CARTESIAN_POINT('Ctrl Pts',(-177.500141677395,5.00072080907722,
129.953380730883));
#254629=CARTESIAN_POINT('Ctrl Pts',(-177.500536626073,4.99948149158206,
129.94633603335));
#254630=CARTESIAN_POINT('Ctrl Pts',(-177.500810594968,4.99862617902564,
129.941490668575));
#254631=CARTESIAN_POINT('Ctrl Pts',(-177.505780023924,4.98319006347085,
129.854340602474));
#254632=CARTESIAN_POINT('Ctrl Pts',(-177.511132903343,4.96780601042822,
129.772215719214));
#254633=CARTESIAN_POINT('Ctrl Pts',(-177.529349382818,4.91874040928095,
129.523654579321));
#254634=CARTESIAN_POINT('Ctrl Pts',(-177.544257370828,4.88258806682499,
129.357846583682));
#254635=CARTESIAN_POINT('Ctrl Pts',(-177.614171330561,4.72588974921601,
128.700200073337));
#254636=CARTESIAN_POINT('Ctrl Pts',(-177.690013732162,4.58067706950535,
128.216337619616));
#254637=CARTESIAN_POINT('Ctrl Pts',(-177.84225534922,4.31179323860895,127.473090897716));
#254638=CARTESIAN_POINT('Ctrl Pts',(-177.904956701624,4.2047636979896,127.204993718243));
#254639=CARTESIAN_POINT('Ctrl Pts',(-178.037928907979,3.98269005161135,
126.69739203434));
#254640=CARTESIAN_POINT('Ctrl Pts',(-178.106102869168,3.87028467230515,
126.461623567896));
#254641=CARTESIAN_POINT('Ctrl Pts',(-178.179024752208,3.75385310384345,
126.229852392558));
#254642=CARTESIAN_POINT('Ctrl Pts',(210.579426101437,-2.14555810197798,
126.384433368448));
#254643=CARTESIAN_POINT('Ctrl Pts',(210.533016425084,-2.88204635455982,
126.741945114569));
#254644=CARTESIAN_POINT('Ctrl Pts',(210.440198811428,-4.16073755837059,
127.832228156677));
#254645=CARTESIAN_POINT('Ctrl Pts',(210.254565323169,-5.41774734084591,
130.983824311839));
#254646=CARTESIAN_POINT('Ctrl Pts',(210.022525636658,-3.70466367662459,
135.280954889074));
#254647=CARTESIAN_POINT('Ctrl Pts',(209.744078012845,1.77278938863763,136.341871604603));
#254648=CARTESIAN_POINT('Ctrl Pts',(209.465630389032,5.61248518735455,132.305536381355));
#254649=CARTESIAN_POINT('Ctrl Pts',(209.187182765219,4.2990952821384,126.894094626803));
#254650=CARTESIAN_POINT('Ctrl Pts',(208.908735141406,-0.967335548355457,
125.073681250508));
#254651=CARTESIAN_POINT('Ctrl Pts',(208.630287517594,-5.34357155608916,
128.520706403956));
#254652=CARTESIAN_POINT('Ctrl Pts',(208.351839893781,-4.80999390579215,
134.065650134797));
#254653=CARTESIAN_POINT('Ctrl Pts',(208.073392269968,0.144086686833323,
136.613971320579));
#254654=CARTESIAN_POINT('Ctrl Pts',(207.794944646155,4.96557142732685,133.823362329787));
#254655=CARTESIAN_POINT('Ctrl Pts',(207.516497022342,5.22403776314189,128.258534510045));
#254656=CARTESIAN_POINT('Ctrl Pts',(207.238049398529,0.681816090004523,
125.033145533949));
#254657=CARTESIAN_POINT('Ctrl Pts',(206.959601774716,-4.48693345015888,
127.111248278652));
#254658=CARTESIAN_POINT('Ctrl Pts',(206.681154150904,-5.53242507739068,
132.583126545744));
#254659=CARTESIAN_POINT('Ctrl Pts',(206.40270652709,-1.49388053201802,136.420413394932));
#254660=CARTESIAN_POINT('Ctrl Pts',(206.124258903278,3.91746311099657,135.0968180907));
#254661=CARTESIAN_POINT('Ctrl Pts',(205.845811279465,5.72885172159717,129.828666190814));
#254662=CARTESIAN_POINT('Ctrl Pts',(205.567363655652,2.27570431130586,125.457128678938));
#254663=CARTESIAN_POINT('Ctrl Pts',(205.288916031839,-3.26870357308214,
125.999436687584));
#254664=CARTESIAN_POINT('Ctrl Pts',(205.010468408026,-5.80933288384994,
130.9572347388));
#254665=CARTESIAN_POINT('Ctrl Pts',(204.732020784213,-3.01146890392974,
135.774549108008));
#254666=CARTESIAN_POINT('Ctrl Pts',(204.4535731604,2.5537877891123,136.024502973214));
#254667=CARTESIAN_POINT('Ctrl Pts',(204.175125536587,5.77223831170541,131.477401078575));
#254668=CARTESIAN_POINT('Ctrl Pts',(203.896677912775,3.6862837897924,126.311807855303));
#254669=CARTESIAN_POINT('Ctrl Pts',(203.618230288961,-1.78718543642468,
125.274651160291));
#254670=CARTESIAN_POINT('Ctrl Pts',(203.339782665149,-5.61831856260093,
129.319027308227));
#254671=CARTESIAN_POINT('Ctrl Pts',(203.061335041336,-4.28649139606962,
134.728352208566));
#254672=CARTESIAN_POINT('Ctrl Pts',(202.782887417523,0.984411954691954,
136.531720532469));
#254673=CARTESIAN_POINT('Ctrl Pts',(202.50443979371,5.3506888113544,133.071924892697));
#254674=CARTESIAN_POINT('Ctrl Pts',(202.225992169897,4.79994404549834,127.528348460205));
#254675=CARTESIAN_POINT('Ctrl Pts',(201.947544546084,-0.161714807569177,
124.995267158526));
#254676=CARTESIAN_POINT('Ctrl Pts',(201.669096922271,-4.97476565284641,
127.800458955558));
#254677=CARTESIAN_POINT('Ctrl Pts',(201.390649298458,-5.21624989388704,
133.366089631302));
#254678=CARTESIAN_POINT('Ctrl Pts',(201.112201674645,-0.664255310463968,
136.577616490799));
#254679=CARTESIAN_POINT('Ctrl Pts',(200.833754050833,4.49815745262305,134.483803242045));
#254680=CARTESIAN_POINT('Ctrl Pts',(200.55530642702,5.52698326394509,129.008761972148));
#254681=CARTESIAN_POINT('Ctrl Pts',(200.276858803207,1.47678146385132,125.183788137525));
#254682=CARTESIAN_POINT('Ctrl Pts',(199.998411179394,-3.93051035674001,
126.523845831826));
#254683=CARTESIAN_POINT('Ctrl Pts',(199.719963555581,-5.7258551755912,131.79748749945));
#254684=CARTESIAN_POINT('Ctrl Pts',(199.441515931768,-2.25941881165118,
136.158494079568));
#254685=CARTESIAN_POINT('Ctrl Pts',(199.163068307955,3.28331306145151,135.599313572066));
#254686=CARTESIAN_POINT('Ctrl Pts',(198.884620684142,5.80884062984016,130.633805545853));
#254687=CARTESIAN_POINT('Ctrl Pts',(198.606173060329,2.99632743704681,125.825029298466));
#254688=CARTESIAN_POINT('Ctrl Pts',(198.327725436517,-2.56966429165962,
125.592015279473));
#254689=CARTESIAN_POINT('Ctrl Pts',(198.049277812704,-5.77426007141042,
130.148891988961));
#254690=CARTESIAN_POINT('Ctrl Pts',(197.770830188891,-3.6725929338218,135.308112346714));
#254691=CARTESIAN_POINT('Ctrl Pts',(197.492382565078,1.80400769380988,136.328604885883));
#254692=CARTESIAN_POINT('Ctrl Pts',(197.213934941265,5.62281338150559,132.272586816804));
#254693=CARTESIAN_POINT('Ctrl Pts',(196.935487317452,4.27452826130232,126.867340597462));
#254694=CARTESIAN_POINT('Ctrl Pts',(196.657039693639,-1.00183950872307,
125.080023442474));
#254695=CARTESIAN_POINT('Ctrl Pts',(196.378592069827,-5.35756571281285,
128.553092501978));
#254696=CARTESIAN_POINT('Ctrl Pts',(196.100144446013,-4.78995075846325,
134.094966979145));
#254697=CARTESIAN_POINT('Ctrl Pts',(195.821696822201,0.179394940810534,
136.612934965078));
#254698=CARTESIAN_POINT('Ctrl Pts',(195.543249198387,4.98388545340951,133.79310689028));
#254699=CARTESIAN_POINT('Ctrl Pts',(195.264801574575,5.20842871066526,128.22676699923));
#254700=CARTESIAN_POINT('Ctrl Pts',(194.986353950762,0.64668042870769,125.029109720981));
#254701=CARTESIAN_POINT('Ctrl Pts',(194.70790632695,-4.50933557513701,127.138625880003));
#254702=CARTESIAN_POINT('Ctrl Pts',(194.429458703136,-5.52149247872048,
132.616773181746));
#254703=CARTESIAN_POINT('Ctrl Pts',(194.151011079324,-1.4596675342632,136.429401878284));
#254704=CARTESIAN_POINT('Ctrl Pts',(193.87256345551,3.9435205654586,135.072892454764));
#254705=CARTESIAN_POINT('Ctrl Pts',(193.594115831698,5.72280591721378,129.793810802232));
#254706=CARTESIAN_POINT('Ctrl Pts',(193.315668207884,2.24311220566103,125.443375061888));
#254707=CARTESIAN_POINT('Ctrl Pts',(193.037220584072,-3.29789204077089,
126.019423148508));
#254708=CARTESIAN_POINT('Ctrl Pts',(192.758772960259,-5.80829461271728,
130.992595012001));
#254709=CARTESIAN_POINT('Ctrl Pts',(192.480325336446,-2.98115818654302,
135.792788662769));
#254710=CARTESIAN_POINT('Ctrl Pts',(192.201877712633,2.58551697539033,136.008860638253));
#254711=CARTESIAN_POINT('Ctrl Pts',(191.92343008882,5.77622834646622,131.442251348686));
#254712=CARTESIAN_POINT('Ctrl Pts',(191.644982465007,3.658868051582,126.289451639914));
#254713=CARTESIAN_POINT('Ctrl Pts',(191.366534841194,-1.82081323706467,
125.285632716038));
#254714=CARTESIAN_POINT('Ctrl Pts',(191.088087217381,-5.6272561125207,129.35325512882));
#254715=CARTESIAN_POINT('Ctrl Pts',(190.809639593569,-4.26252552731426,
134.754372595315));
#254716=CARTESIAN_POINT('Ctrl Pts',(190.531191969755,1.01925778154541,136.525622023071));
#254717=CARTESIAN_POINT('Ctrl Pts',(190.252744345943,5.36439298267566,133.039311718326));
#254718=CARTESIAN_POINT('Ctrl Pts',(189.974296722129,4.77991309789331,127.499190535413));
#254719=CARTESIAN_POINT('Ctrl Pts',(189.695849098317,-0.197073412116412,
124.996359191464));
#254720=CARTESIAN_POINT('Ctrl Pts',(189.417401474504,-4.99295908396257,
127.830797421458));
#254721=CARTESIAN_POINT('Ctrl Pts',(189.138953850692,-5.20055927725872,
133.397794962038));
#254722=CARTESIAN_POINT('Ctrl Pts',(188.860506226878,-0.629099556198964,
136.581553036358));
#254723=CARTESIAN_POINT('Ctrl Pts',(188.582058603065,4.52047192378579,134.456353509349));
#254724=CARTESIAN_POINT('Ctrl Pts',(188.303610979253,5.51595054314194,128.975150924561));
#254725=CARTESIAN_POINT('Ctrl Pts',(188.02516335544,1.44254008251539,125.174902685784));
#254726=CARTESIAN_POINT('Ctrl Pts',(187.746715731627,-3.95649424194195,
126.547851272005));
#254727=CARTESIAN_POINT('Ctrl Pts',(187.468268107814,-5.71970364354381,
131.832324004755));
#254728=CARTESIAN_POINT('Ctrl Pts',(187.189820484001,-2.22678481978599,
136.172148603481));
#254729=CARTESIAN_POINT('Ctrl Pts',(186.911372860188,3.312440468869,135.579238274173));
#254730=CARTESIAN_POINT('Ctrl Pts',(186.632925236375,5.80769478834652,130.598448644184));
#254731=CARTESIAN_POINT('Ctrl Pts',(186.354477612562,2.96596131899707,125.806882058373));
#254732=CARTESIAN_POINT('Ctrl Pts',(186.076029988749,-2.60134570724499,
125.607754128061));
#254733=CARTESIAN_POINT('Ctrl Pts',(185.797582364937,-5.7781431113317,130.184053693262));
#254734=CARTESIAN_POINT('Ctrl Pts',(185.519134741124,-3.64510927408837,
135.33038501822));
#254735=CARTESIAN_POINT('Ctrl Pts',(185.240687117311,1.83760191255446,136.317521027561));
#254736=CARTESIAN_POINT('Ctrl Pts',(184.962239493498,5.63164671340385,132.238331952975));
#254737=CARTESIAN_POINT('Ctrl Pts',(184.683791869685,4.25048330587202,126.841393274542));
#254738=CARTESIAN_POINT('Ctrl Pts',(184.405344245872,-1.03666661210287,
125.086227982629));
#254739=CARTESIAN_POINT('Ctrl Pts',(184.126896622059,-5.37117055753467,
128.585747235914));
#254740=CARTESIAN_POINT('Ctrl Pts',(183.848448998247,-4.7698311568614,134.124063801647));
#254741=CARTESIAN_POINT('Ctrl Pts',(183.570001374433,0.214750057761129,
136.611735317726));
#254742=CARTESIAN_POINT('Ctrl Pts',(183.291553750621,5.00198646042476,133.762713190383));
#254743=CARTESIAN_POINT('Ctrl Pts',(183.013106126807,5.19264166658148,128.195109572179));
#254744=CARTESIAN_POINT('Ctrl Pts',(182.734658502995,0.611512855797894,
125.025280195685));
#254745=CARTESIAN_POINT('Ctrl Pts',(182.456210879182,-4.53156639540017,
127.166143403126));
#254746=CARTESIAN_POINT('Ctrl Pts',(182.177763255369,-5.5103575085511,132.650350493844));
#254747=CARTESIAN_POINT('Ctrl Pts',(181.899315631556,-1.42539926727337,
136.438183069882));
#254748=CARTESIAN_POINT('Ctrl Pts',(181.620868007743,3.96943126600311,135.048808039769));
#254749=CARTESIAN_POINT('Ctrl Pts',(181.34242038393,5.71654838332065,129.758993181434));
#254750=CARTESIAN_POINT('Ctrl Pts',(181.063972760118,2.21043680528058,125.429819927867));
#254751=CARTESIAN_POINT('Ctrl Pts',(180.785525136304,-3.32695821097111,
126.039587007222));
#254752=CARTESIAN_POINT('Ctrl Pts',(180.507077512492,-5.80704116228462,
131.027948262352));
#254753=CARTESIAN_POINT('Ctrl Pts',(180.228629888679,-2.95073697519064,
135.810843394787));
#254754=CARTESIAN_POINT('Ctrl Pts',(179.950182264866,2.61715034058839,135.993025435236));
#254755=CARTESIAN_POINT('Ctrl Pts',(179.671734641053,5.78000434826875,131.407077988614));
#254756=CARTESIAN_POINT('Ctrl Pts',(179.39328701724,3.63131672880039,126.26726272238));
#254757=CARTESIAN_POINT('Ctrl Pts',(179.114839393428,-1.8543735647511,125.296818772266));
#254758=CARTESIAN_POINT('Ctrl Pts',(178.836391769614,-5.63598514348121,
129.387536719606));
#254759=CARTESIAN_POINT('Ctrl Pts',(178.557944145802,-4.23840170853308,
134.780246613475));
#254760=CARTESIAN_POINT('Ctrl Pts',(178.279496521988,1.05406583912245,136.519311509933));
#254761=CARTESIAN_POINT('Ctrl Pts',(178.001048898175,5.3778983746034,133.006615727177));
#254762=CARTESIAN_POINT('Ctrl Pts',(177.722601274363,4.75970502876524,127.470155084831));
#254763=CARTESIAN_POINT('Ctrl Pts',(177.44415365055,-0.232424713990654,
124.997666442073));
#254764=CARTESIAN_POINT('Ctrl Pts',(177.165706026737,-5.01096749916768,
127.861246073811));
#254765=CARTESIAN_POINT('Ctrl Pts',(176.887258402924,-5.18467595198119,
133.429404192122));
#254766=CARTESIAN_POINT('Ctrl Pts',(176.608810779111,-0.593920490425269,
136.585275505922));
#254767=CARTESIAN_POINT('Ctrl Pts',(176.330363155298,4.54261888720253,134.428768450716));
#254768=CARTESIAN_POINT('Ctrl Pts',(176.051915531486,5.50471342676105,128.941607659011));
#254769=CARTESIAN_POINT('Ctrl Pts',(175.773467907672,1.40824524732727,125.166225835676));
#254770=CARTESIAN_POINT('Ctrl Pts',(175.49502028386,-3.98233151779528,126.572014438702));
#254771=CARTESIAN_POINT('Ctrl Pts',(175.216572660047,-5.7133401657742,131.867122418498));
#254772=CARTESIAN_POINT('Ctrl Pts',(174.938125036234,-2.19406831359054,
136.185604222037));
#254773=CARTESIAN_POINT('Ctrl Pts',(174.659677412421,3.34144513258691,135.558986041432));
#254774=CARTESIAN_POINT('Ctrl Pts',(174.381229788608,5.80633374058666,130.563099372659));
#254775=CARTESIAN_POINT('Ctrl Pts',(174.102782164795,2.93548529615992,125.788920001687));
#254776=CARTESIAN_POINT('Ctrl Pts',(173.824334540982,-2.63293072900865,
125.623685538813));
#254777=CARTESIAN_POINT('Ctrl Pts',(173.54588691717,-5.7818120400351,130.219238383264));
#254778=CARTESIAN_POINT('Ctrl Pts',(173.267439293356,-3.61749054349026,
135.352489976228));
#254779=CARTESIAN_POINT('Ctrl Pts',(172.988991669544,1.87112803828436,136.306232877052));
#254780=CARTESIAN_POINT('Ctrl Pts',(172.71054404573,5.64027136256211,132.204023952811));
#254781=CARTESIAN_POINT('Ctrl Pts',(172.432096421918,4.22628084721974,126.815592800833));
#254782=CARTESIAN_POINT('Ctrl Pts',(172.153648798105,-1.07145530142008,
125.092644410292));
#254783=CARTESIAN_POINT('Ctrl Pts',(171.875201174292,-5.38457637155629,
128.618484181386));
#254784=CARTESIAN_POINT('Ctrl Pts',(171.596753550479,-4.74953480741189,
134.153037611328));
#254785=CARTESIAN_POINT('Ctrl Pts',(171.318305926666,0.25009721706947,136.610320475968));
#254786=CARTESIAN_POINT('Ctrl Pts',(171.039858302853,5.01990211699227,133.732209867644));
#254787=CARTESIAN_POINT('Ctrl Pts',(170.76141067904,5.1766622072511,128.163548831885));
#254788=CARTESIAN_POINT('Ctrl Pts',(170.482963055228,0.576322623054293,
125.021664816339));
#254789=CARTESIAN_POINT('Ctrl Pts',(170.204515431414,-4.55362929680409,
127.193795741725));
#254790=CARTESIAN_POINT('Ctrl Pts',(169.926067807602,-5.4990183500578,132.683859402108));
#254791=CARTESIAN_POINT('Ctrl Pts',(169.647620183788,-1.39107818158956,
136.446755498118));
#254792=CARTESIAN_POINT('Ctrl Pts',(169.369172559976,3.99519487781229,135.024566345214));
#254793=CARTESIAN_POINT('Ctrl Pts',(169.090724936163,5.71007902062496,129.724214297113));
#254794=CARTESIAN_POINT('Ctrl Pts',(168.81227731235,2.17767949635139,125.416463949427));
#254795=CARTESIAN_POINT('Ctrl Pts',(168.533829688537,-3.35590109951139,
126.059927426375));
#254796=CARTESIAN_POINT('Ctrl Pts',(168.255382064725,-5.80557252980615,
131.063293227581));
#254797=CARTESIAN_POINT('Ctrl Pts',(167.976934440911,-2.92020642319446,
135.828712609743));
#254798=CARTESIAN_POINT('Ctrl Pts',(167.698486817099,2.64868672631821,135.976997964335));
#254799=CARTESIAN_POINT('Ctrl Pts',(167.420039193286,5.78356616988455,131.371882294628));
#254800=CARTESIAN_POINT('Ctrl Pts',(167.141591569473,3.60363084624196,126.245241928676));
#254801=CARTESIAN_POINT('Ctrl Pts',(166.86314394566,-1.88786517794308,125.308208912483));
#254802=CARTESIAN_POINT('Ctrl Pts',(166.584696321847,-5.64450533093961,
129.421870811324));
#254803=CARTESIAN_POINT('Ctrl Pts',(166.306248698034,-4.21412083421794,
134.805973303719));
#254804=CARTESIAN_POINT('Ctrl Pts',(166.027801074221,1.08883483790225,136.512789227187));
#254805=CARTESIAN_POINT('Ctrl Pts',(165.749353450409,5.3912044865292,132.973838130654));
#254806=CARTESIAN_POINT('Ctrl Pts',(165.470905826595,4.73932058701693,127.441243184462));
#254807=CARTESIAN_POINT('Ctrl Pts',(165.192458202783,-0.267767403281747,
124.999188861871));
#254808=CARTESIAN_POINT('Ctrl Pts',(164.914010578969,-5.02879023112935,
127.891803784357));
#254809=CARTESIAN_POINT('Ctrl Pts',(164.635562955157,-5.16860050662956,
133.46091615025));
#254810=CARTESIAN_POINT('Ctrl Pts',(164.357115331344,-0.55871941670932,
136.588783761558));
#254811=CARTESIAN_POINT('Ctrl Pts',(164.078667707531,4.56459752220588,134.401049088318));
#254812=CARTESIAN_POINT('Ctrl Pts',(163.800220083718,5.49327233119978,128.908133418456));
#254813=CARTESIAN_POINT('Ctrl Pts',(163.521772459905,1.37389822909362,125.157757908727));
#254814=CARTESIAN_POINT('Ctrl Pts',(163.243324836092,-4.00802122688977,
126.596334436543));
#254815=CARTESIAN_POINT('Ctrl Pts',(162.964877212279,-5.70676497808368,
131.901881451211));
#254816=CARTESIAN_POINT('Ctrl Pts',(162.686429588467,-2.16127050538683,
136.198860436632));
#254817=CARTESIAN_POINT('Ctrl Pts',(162.407981964654,3.37032597782655,135.538557624299));
#254818=CARTESIAN_POINT('Ctrl Pts',(162.129534340841,5.80475753699479,130.527759041158));
#254819=CARTESIAN_POINT('Ctrl Pts',(161.851086717028,2.90490049783562,125.771143793998));
#254820=CARTESIAN_POINT('Ctrl Pts',(161.572639093215,-2.66441818655578,
125.639808921385));
#254821=CARTESIAN_POINT('Ctrl Pts',(161.294191469402,-5.7852667215671,130.254444755185));
#254822=CARTESIAN_POINT('Ctrl Pts',(161.015743845589,-3.58973776544978,
135.37442640163));
#254823=CARTESIAN_POINT('Ctrl Pts',(160.737296221776,1.90458482867669,136.294740852644));
#254824=CARTESIAN_POINT('Ctrl Pts',(160.458848597964,5.64868700939082,132.169664087608));
#254825=CARTESIAN_POINT('Ctrl Pts',(160.18040097415,4.20192178217643,126.789940132385));
#254826=CARTESIAN_POINT('Ctrl Pts',(159.901953350338,-1.10620428756715,
125.099272487699));
#254827=CARTESIAN_POINT('Ctrl Pts',(159.623505726525,-5.39778265812024,
128.651302125312));
#254828=CARTESIAN_POINT('Ctrl Pts',(159.345058102712,-4.72906246220349,
134.18188733455));
#254829=CARTESIAN_POINT('Ctrl Pts',(159.066610478899,0.285435108933367,
136.608690492233));
#254830=CARTESIAN_POINT('Ctrl Pts',(158.788162855086,5.03763175924073,133.701598052375));
#254831=CARTESIAN_POINT('Ctrl Pts',(158.509715231273,5.16049092479898,128.132085947844));
#254832=CARTESIAN_POINT('Ctrl Pts',(158.23126760746,0.541111034464008,125.018263716911));
#254833=CARTESIAN_POINT('Ctrl Pts',(157.952819983648,-4.57552346179978,
127.221581871133));
#254834=CARTESIAN_POINT('Ctrl Pts',(157.674372359834,-5.48747542341729,
132.717298664853));
#254835=CARTESIAN_POINT('Ctrl Pts',(157.395924736022,-1.35670554899215,
136.455118845335));
#254836=CARTESIAN_POINT('Ctrl Pts',(157.117477112209,4.02081044620608,135.000168269382));
#254837=CARTESIAN_POINT('Ctrl Pts',(156.839029488396,5.70339806885126,129.68947543801));
#254838=CARTESIAN_POINT('Ctrl Pts',(156.560581864583,2.1448414927076,125.403307621479));
#254839=CARTESIAN_POINT('Ctrl Pts',(156.28213424077,-3.38471963390224,126.080443652244));
#254840=CARTESIAN_POINT('Ctrl Pts',(156.003686616957,-5.8038887697026,131.098628597966));
#254841=CARTESIAN_POINT('Ctrl Pts',(155.725238993144,-2.88956766187541,
135.846395645489));
#254842=CARTESIAN_POINT('Ctrl Pts',(155.446791369331,2.68012496398725,135.960778819456));
#254843=CARTESIAN_POINT('Ctrl Pts',(155.168343745519,5.78691367932904,131.336665570917));
#254844=CARTESIAN_POINT('Ctrl Pts',(154.889896121706,3.57581142981733,126.223390074792));
#254845=CARTESIAN_POINT('Ctrl Pts',(154.611448497893,-1.92128683559663,
125.319802714623));
#254846=CARTESIAN_POINT('Ctrl Pts',(154.33300087408,-5.65281635917722,129.456256131708));
#254847=CARTESIAN_POINT('Ctrl Pts',(154.054553250267,-4.18968380410554,
134.831551712731));
#254848=CARTESIAN_POINT('Ctrl Pts',(153.776105626454,1.12356348950664,136.50605541652));
#254849=CARTESIAN_POINT('Ctrl Pts',(153.497658002641,5.40431082539012,132.940980143345));
#254850=CARTESIAN_POINT('Ctrl Pts',(153.219210378828,4.71876052800142,127.412455905645));
#254851=CARTESIAN_POINT('Ctrl Pts',(152.940762755016,-0.303100170353132,
125.000926394444));
#254852=CARTESIAN_POINT('Ctrl Pts',(152.662315131202,-5.04642661941966,
127.922469420767));
#254853=CARTESIAN_POINT('Ctrl Pts',(152.38386750739,-5.15233353688545,133.492329668737));
#254854=CARTESIAN_POINT('Ctrl Pts',(152.105419883576,-0.523497639439988,
136.592077673268));
#254855=CARTESIAN_POINT('Ctrl Pts',(151.826972259764,4.58640701436939,134.373196449306));
#254856=CARTESIAN_POINT('Ctrl Pts',(151.548524635951,5.48162768041213,128.874729443297));
#254857=CARTESIAN_POINT('Ctrl Pts',(151.270077012138,1.33950030055583,125.149499218718));
#254858=CARTESIAN_POINT('Ctrl Pts',(150.991629388325,-4.03356241728369,
126.620810364342));
#254859=CARTESIAN_POINT('Ctrl Pts',(150.713181764512,-5.69997832411825,
131.936599814887));
#254860=CARTESIAN_POINT('Ctrl Pts',(150.434734140699,-2.1283926105098,136.211916756054));
#254861=CARTESIAN_POINT('Ctrl Pts',(150.156286516886,3.39908193439765,135.517953779753));
#254862=CARTESIAN_POINT('Ctrl Pts',(149.877838893074,5.8029662359777,130.49242895923));
#254863=CARTESIAN_POINT('Ctrl Pts',(149.599391269261,2.87420805735513,125.753554094008));
#254864=CARTESIAN_POINT('Ctrl Pts',(149.320943645448,-2.69580691310719,
125.65612367832));
#254865=CARTESIAN_POINT('Ctrl Pts',(149.042496021635,-5.7885070279132,130.289671504441));
#254866=CARTESIAN_POINT('Ctrl Pts',(148.764048397822,-3.56185196835627,
135.396193481562));
#254867=CARTESIAN_POINT('Ctrl Pts',(148.485600774009,1.93797104397778,136.283045380177));
#254868=CARTESIAN_POINT('Ctrl Pts',(148.207153150196,5.6568933420451,132.135253630582));
#254869=CARTESIAN_POINT('Ctrl Pts',(147.928705526383,4.17740701337624,126.764436219762));
#254870=CARTESIAN_POINT('Ctrl Pts',(147.65025790257,-1.14091228290746,125.106111969245));
#254871=CARTESIAN_POINT('Ctrl Pts',(147.371810278758,-5.41078892786276,
128.684199851613));
#254872=CARTESIAN_POINT('Ctrl Pts',(147.093362654945,-4.70841487984645,
134.210611902278));
#254873=CARTESIAN_POINT('Ctrl Pts',(146.814915031132,0.320762423894332,
136.60684542692));
#254874=CARTESIAN_POINT('Ctrl Pts',(146.536467407319,5.05517473019176,133.670878878906));
#254875=CARTESIAN_POINT('Ctrl Pts',(146.258019783506,5.14412841845787,128.100722085923));
#254876=CARTESIAN_POINT('Ctrl Pts',(145.979572159693,0.505879394805349,
125.015077023433));
#254877=CARTESIAN_POINT('Ctrl Pts',(145.70112453588,-4.59724807909095,127.249500761725));
#254878=CARTESIAN_POINT('Ctrl Pts',(145.422676912067,-5.47572915635697,
132.750667042976));
#254879=CARTESIAN_POINT('Ctrl Pts',(145.144229288255,-1.32228264317164,
136.463272801628));
#254880=CARTESIAN_POINT('Ctrl Pts',(144.865781664442,4.0462770219901,134.975614716357));
#254881=CARTESIAN_POINT('Ctrl Pts',(144.587334040629,5.69650577556471,129.654777891387));
#254882=CARTESIAN_POINT('Ctrl Pts',(144.308886416816,2.11192401117359,125.390351431538));
#254883=CARTESIAN_POINT('Ctrl Pts',(144.030438793003,-3.41341274626234,
126.101134924595));
#254884=CARTESIAN_POINT('Ctrl Pts',(143.75199116919,-5.80198994436631,131.133953064144));
#254885=CARTESIAN_POINT('Ctrl Pts',(143.473543545377,-2.85882182656403,
135.863891846773));
#254886=CARTESIAN_POINT('Ctrl Pts',(143.195095921564,2.71146388864014,135.944368601604));
#254887=CARTESIAN_POINT('Ctrl Pts',(142.916648297751,5.790046752559,131.301429122451));
#254888=CARTESIAN_POINT('Ctrl Pts',(142.638200673938,3.54785951038517,126.201707970457));
#254889=CARTESIAN_POINT('Ctrl Pts',(142.359753050125,-1.95463729925998,
125.331599749072));
#254890=CARTESIAN_POINT('Ctrl Pts',(142.081305426313,-5.66091792022584,
129.490691406602));
#254891=CARTESIAN_POINT('Ctrl Pts',(141.8028578025,-4.16509152371897,134.856980892698));
#254892=CARTESIAN_POINT('Ctrl Pts',(141.524410178687,1.15825050705268,136.499110327454));
#254893=CARTESIAN_POINT('Ctrl Pts',(141.245962554874,5.41721690552589,132.908042982814));
#254894=CARTESIAN_POINT('Ctrl Pts',(140.967514931061,4.69802561357932,127.383794315106));
#254895=CARTESIAN_POINT('Ctrl Pts',(140.689067307248,-0.338421705936203,
125.002878975406));
#254896=CARTESIAN_POINT('Ctrl Pts',(140.410619683435,-5.06387601051571,
127.953241846716));
#254897=CARTESIAN_POINT('Ctrl Pts',(140.132172059623,-5.13587564552739,
133.523643583541));
#254898=CARTESIAN_POINT('Ctrl Pts',(139.85372443581,-0.48825646377323,136.595157118993));
#254899=CARTESIAN_POINT('Ctrl Pts',(139.575276811997,4.60804655553434,134.34521156577));
#254900=CARTESIAN_POINT('Ctrl Pts',(139.296829188184,5.46977990589493,128.841396971331));
#254901=CARTESIAN_POINT('Ctrl Pts',(139.018381564371,1.30505273634171,125.141450071677));
#254902=CARTESIAN_POINT('Ctrl Pts',(138.739933940558,-4.05895414253892,
126.645441315135));
#254903=CARTESIAN_POINT('Ctrl Pts',(138.461486316745,-5.69298045535984,
131.971276223022));
#254904=CARTESIAN_POINT('Ctrl Pts',(138.183038692932,-2.09543584726193,
136.224772696493));
#254905=CARTESIAN_POINT('Ctrl Pts',(137.904591069119,3.42771193673771,135.49717527128));
#254906=CARTESIAN_POINT('Ctrl Pts',(137.626143445306,5.80095990391266,130.457110436044));
#254907=CARTESIAN_POINT('Ctrl Pts',(137.347695821494,2.84340911203807,125.736151553513));
#254908=CARTESIAN_POINT('Ctrl Pts',(137.069248197681,-2.727095745542,125.672629205068));
#254909=CARTESIAN_POINT('Ctrl Pts',(136.790800573868,-5.7915328390027,130.324917325691));
#254910=CARTESIAN_POINT('Ctrl Pts',(136.512352950055,-3.53383418552815,
135.417790409441));
#254911=CARTESIAN_POINT('Ctrl Pts',(136.233905326242,1.97128544704926,136.271146893031));
#254912=CARTESIAN_POINT('Ctrl Pts',(135.955457702429,5.66489005643625,132.100793856825));
#254913=CARTESIAN_POINT('Ctrl Pts',(135.677010078616,4.15273744922295,126.739082008025));
#254914=CARTESIAN_POINT('Ctrl Pts',(135.398562454803,-1.17557800132362,
125.113162601491));
#254915=CARTESIAN_POINT('Ctrl Pts',(135.12011483099,-5.42359469883174,128.717176141249));
#254916=CARTESIAN_POINT('Ctrl Pts',(134.841667207177,-4.68759282544451,
134.239210250113));
#254917=CARTESIAN_POINT('Ctrl Pts',(134.563219583365,0.356077852885664,
136.604785348398));
#254918=CARTESIAN_POINT('Ctrl Pts',(134.284771959552,5.0725303797842,133.640053485549));
#254919=CARTESIAN_POINT('Ctrl Pts',(134.006324335739,5.12757529454644,128.069458408322));
#254920=CARTESIAN_POINT('Ctrl Pts',(133.727876711926,0.470629009599695,
125.012104853988));
#254921=CARTESIAN_POINT('Ctrl Pts',(133.449429088113,-4.61880234366392,
127.277551378957));
#254922=CARTESIAN_POINT('Ctrl Pts',(133.1709814643,-5.46377998413907,132.783963299997));
#254923=CARTESIAN_POINT('Ctrl Pts',(132.892533840487,-1.28781073968153,
136.47121706485));
#254924=CARTESIAN_POINT('Ctrl Pts',(132.614086216674,4.07159366149105,134.950906595976));
#254925=CARTESIAN_POINT('Ctrl Pts',(132.335638592862,5.68940239616175,129.620122942976));
#254926=CARTESIAN_POINT('Ctrl Pts',(132.057190969048,2.07892827151876,125.377595859696));
#254927=CARTESIAN_POINT('Ctrl Pts',(131.778743345236,-3.44197937335791,
126.122000476702));
#254928=CARTESIAN_POINT('Ctrl Pts',(131.500295721423,-5.79987612415893,
131.169265317152));
#254929=CARTESIAN_POINT('Ctrl Pts',(131.22184809761,-2.82797005655853,135.881200565267));
#254930=CARTESIAN_POINT('Ctrl Pts',(130.943400473797,2.74270233900145,135.927767918864));
#254931=CARTESIAN_POINT('Ctrl Pts',(130.664952849984,5.79296527347731,131.26617425493));
#254932=CARTESIAN_POINT('Ctrl Pts',(130.386505226171,3.51977612371406,126.180196419108));
#254933=CARTESIAN_POINT('Ctrl Pts',(130.108057602358,-1.98791533311939,
125.343599578688));
#254934=CARTESIAN_POINT('Ctrl Pts',(129.829609978546,-5.66880971387908,
129.52517535999));
#254935=CARTESIAN_POINT('Ctrl Pts',(129.551162354732,-4.14034490433441,
134.882259901329));
#254936=CARTESIAN_POINT('Ctrl Pts',(129.27271473092,1.19289460520041,136.491954217345));
#254937=CARTESIAN_POINT('Ctrl Pts',(128.994267107107,5.42992224869717,132.875027869557));
#254938=CARTESIAN_POINT('Ctrl Pts',(128.715819483294,4.67711661209022,127.355259474909));
#254939=CARTESIAN_POINT('Ctrl Pts',(128.437371859481,-0.373730701178542,
125.005046532403));
#254940=CARTESIAN_POINT('Ctrl Pts',(128.158924235668,-5.0811377578241,127.984119921918));
#254941=CARTESIAN_POINT('Ctrl Pts',(127.880476611855,-5.11922744240848,
133.554856734316));
#254942=CARTESIAN_POINT('Ctrl Pts',(127.602028988042,-0.452997195583419,
136.598021984625));
#254943=CARTESIAN_POINT('Ctrl Pts',(127.323581364229,4.62951534383955,134.3170954747));
#254944=CARTESIAN_POINT('Ctrl Pts',(127.045133740417,5.45772944667181,128.808137237705));
#254945=CARTESIAN_POINT('Ctrl Pts',(126.766686116604,1.2705568129186,125.133610765869));
#254946=CARTESIAN_POINT('Ctrl Pts',(126.488238492791,-4.08419546175569,
126.67022637621));
#254947=CARTESIAN_POINT('Ctrl Pts',(126.209790868978,-5.68577163111709,
132.005909390672));
#254948=CARTESIAN_POINT('Ctrl Pts',(125.931343245165,-2.06240143686808,
136.237427781569));
#254949=CARTESIAN_POINT('Ctrl Pts',(125.652895621352,3.45621492395137,135.476222868834));
#254950=CARTESIAN_POINT('Ctrl Pts',(125.374447997539,5.79873861514512,130.421804780342));
#254951=CARTESIAN_POINT('Ctrl Pts',(125.096000373726,2.8125048031507,125.718936817367));
#254952=CARTESIAN_POINT('Ctrl Pts',(124.817552749914,-2.75828352444112,
125.68932489001));
#254953=CARTESIAN_POINT('Ctrl Pts',(124.5391051261,-5.79434404271298,130.36018091289));
#254954=CARTESIAN_POINT('Ctrl Pts',(124.260657502288,-3.50568545517477,
135.439216384981));
#254955=CARTESIAN_POINT('Ctrl Pts',(123.982209878475,2.00452680341345,136.25904583211));
#254956=CARTESIAN_POINT('Ctrl Pts',(123.703762254662,5.67267685624313,132.066286043259));
#254957=CARTESIAN_POINT('Ctrl Pts',(123.425314630849,4.12791400385628,126.71387843668));
#254958=CARTESIAN_POINT('Ctrl Pts',(123.146867007036,-1.21020015826455,
125.120424123171));
#254959=CARTESIAN_POINT('Ctrl Pts',(122.868419383223,-5.43619949650465,
128.750229772276));
#254960=CARTESIAN_POINT('Ctrl Pts',(122.58997175941,-4.66659707056658,134.267681318331));
#254961=CARTESIAN_POINT('Ctrl Pts',(122.311524135597,0.391380087281262,
136.602510333005));
#254962=CARTESIAN_POINT('Ctrl Pts',(122.033076511785,5.08969806489794,133.609123014551));
#254963=CARTESIAN_POINT('Ctrl Pts',(121.754628887972,5.11083216644683,128.038296073528));
#254964=CARTESIAN_POINT('Ctrl Pts',(121.476181264159,0.435361185062875,
125.00934731871));
#254965=CARTESIAN_POINT('Ctrl Pts',(121.197733640346,-4.64018545681751,
127.305732683402));
#254966=CARTESIAN_POINT('Ctrl Pts',(120.919286016533,-5.45162834954452,
132.817186202114));
#254967=CARTESIAN_POINT('Ctrl Pts',(120.64083839272,-1.25329111589093,136.478951340622));
#254968=CARTESIAN_POINT('Ctrl Pts',(120.362390768907,4.09675942659154,134.92604482381));
#254969=CARTESIAN_POINT('Ctrl Pts',(120.083943145094,5.68208819386074,129.585511876926));
#254970=CARTESIAN_POINT('Ctrl Pts',(119.805495521281,2.04585549641223,125.36504137862));
#254971=CARTESIAN_POINT('Ctrl Pts',(119.527047897469,-3.47041845664194,
126.143039535386));
#254972=CARTESIAN_POINT('Ctrl Pts',(119.248600273655,-5.79754738740892,
131.204564048482));
#254973=CARTESIAN_POINT('Ctrl Pts',(118.970152649843,-2.7970134950826,135.898321159589));
#254974=CARTESIAN_POINT('Ctrl Pts',(118.69170502603,2.77383915751901,135.910977386384));
#254975=CARTESIAN_POINT('Ctrl Pts',(118.413257402217,5.795669133937,131.230902274733));
#254976=CARTESIAN_POINT('Ctrl Pts',(118.134809778404,3.49156231044436,126.158856217863));
#254977=CARTESIAN_POINT('Ctrl Pts',(117.856362154591,-2.02111970404504,
125.355801758813));
#254978=CARTESIAN_POINT('Ctrl Pts',(117.577914530778,-5.67649144770371,
129.559706714059));
#254979=CARTESIAN_POINT('Ctrl Pts',(117.299466906965,-4.11544486294674,
134.907387801903));
#254980=CARTESIAN_POINT('Ctrl Pts',(117.021019283153,1.22749450019975,136.484587351363));
#254981=CARTESIAN_POINT('Ctrl Pts',(116.74257165934,5.44242638410263,132.841936026965));
#254982=CARTESIAN_POINT('Ctrl Pts',(116.464124035527,4.65603429832517,127.326852442422));
#254983=CARTESIAN_POINT('Ctrl Pts',(116.185676411714,-0.409025847692317,
125.007428985116));
#254984=CARTESIAN_POINT('Ctrl Pts',(115.907228787901,-5.09821122170419,
128.015102502178));
#254985=CARTESIAN_POINT('Ctrl Pts',(115.628781164088,-5.10238954443416,
133.585967964446));
#254986=CARTESIAN_POINT('Ctrl Pts',(115.350333540275,-0.417721141415912,
136.600672164005));
#254987=CARTESIAN_POINT('Ctrl Pts',(115.071885916462,4.65081258375125,134.288849217947));
#254988=CARTESIAN_POINT('Ctrl Pts',(114.793438292649,5.44547674927697,128.77495147487));
#254989=CARTESIAN_POINT('Ctrl Pts',(114.514990668836,1.23601380854556,125.125981591782));
#254990=CARTESIAN_POINT('Ctrl Pts',(114.236543045024,-4.10928543960769,
126.695164629152));
#254991=CARTESIAN_POINT('Ctrl Pts',(113.958095421211,-5.67835211851559,
132.040498034489));
#254992=CARTESIAN_POINT('Ctrl Pts',(113.679647797398,-2.02929060343055,
136.249881542344));
#254993=CARTESIAN_POINT('Ctrl Pts',(113.401200173585,3.48458983985001,135.455097348814));
#254994=CARTESIAN_POINT('Ctrl Pts',(113.122752549772,5.79630245198571,130.386513300387));
#254995=CARTESIAN_POINT('Ctrl Pts',(112.844304925959,2.78149627586357,125.701910523471));
#254996=CARTESIAN_POINT('Ctrl Pts',(112.565857302146,-2.78936909412988,
125.706210114483));
#254997=CARTESIAN_POINT('Ctrl Pts',(112.287409678333,-5.7969405348739,130.395460959329));
#254998=CARTESIAN_POINT('Ctrl Pts',(112.008962054521,-3.47740682035766,
135.460470614237));
#254999=CARTESIAN_POINT('Ctrl Pts',(111.730514430707,2.03769388129978,136.246742645822));
#255000=CARTESIAN_POINT('Ctrl Pts',(111.452066806895,5.68025345292297,132.031731468582));
#255001=CARTESIAN_POINT('Ctrl Pts',(111.173619183082,4.10293759711819,126.688826439658));
#255002=CARTESIAN_POINT('Ctrl Pts',(110.895171559269,-1.24477747079359,
125.127896265209));
#255003=CARTESIAN_POINT('Ctrl Pts',(110.616723935456,-5.44860285380605,
128.783359519875));
#255004=CARTESIAN_POINT('Ctrl Pts',(110.338276311643,-4.64542839321807,
134.296024051927));
#255005=CARTESIAN_POINT('Ctrl Pts',(110.05982868783,0.426667818943798,136.600020465042));
#255006=CARTESIAN_POINT('Ctrl Pts',(109.781381064017,5.10667714937814,133.57808861205));
#255007=CARTESIAN_POINT('Ctrl Pts',(109.502933440204,5.0938996545818,128.007236236273));
#255008=CARTESIAN_POINT('Ctrl Pts',(109.224485816392,0.400077228057368,
125.006804519781));
#255009=CARTESIAN_POINT('Ctrl Pts',(108.946038192578,-4.66139662619255,
127.334043630792));
#255010=CARTESIAN_POINT('Ctrl Pts',(108.667590568766,-5.43927470285667,
132.850334518237));
#255011=CARTESIAN_POINT('Ctrl Pts',(108.389142944953,-1.21872505093712,
136.486475342347));
#255012=CARTESIAN_POINT('Ctrl Pts',(108.11069532114,4.1217733847649,134.901030321119));
#255013=CARTESIAN_POINT('Ctrl Pts',(107.832247697327,5.67456343969215,129.550945975765));
#255014=CARTESIAN_POINT('Ctrl Pts',(107.553800073514,2.01270691137792,125.352688453517));
#255015=CARTESIAN_POINT('Ctrl Pts',(107.275352449701,-3.49872894229381,
126.164251321038));
#255016=CARTESIAN_POINT('Ctrl Pts',(106.996904825888,-5.7950038204084,131.239847950126));
#255017=CARTESIAN_POINT('Ctrl Pts',(106.718457202076,-2.76595328924301,
135.91525299533));
#255018=CARTESIAN_POINT('Ctrl Pts',(106.440009578262,2.80487319040651,135.893997626342));
#255019=CARTESIAN_POINT('Ctrl Pts',(106.16156195445,5.7981582337456,131.195614488879));
#255020=CARTESIAN_POINT('Ctrl Pts',(105.883114330637,3.46321911604922,126.137688157493));
#255021=CARTESIAN_POINT('Ctrl Pts',(105.604666706824,-2.05424918163679,
125.36820583729));
#255022=CARTESIAN_POINT('Ctrl Pts',(105.326219083011,-5.68396283705021,
129.594284189235));
#255023=CARTESIAN_POINT('Ctrl Pts',(105.047771459198,-4.09039232223623,
134.932363663296));
#255024=CARTESIAN_POINT('Ctrl Pts',(104.769323835385,1.26204890993897,136.47701000249));
#255025=CARTESIAN_POINT('Ctrl Pts',(104.490876211572,5.45472884839698,132.808768681268));
#255026=CARTESIAN_POINT('Ctrl Pts',(104.21242858776,4.63477945349693,127.29857427028));
#255027=CARTESIAN_POINT('Ctrl Pts',(103.933980963947,-0.444305837602887,
125.010026245263));
#255028=CARTESIAN_POINT('Ctrl Pts',(103.655533340134,-5.1150957694926,128.046188439421));
#255029=CARTESIAN_POINT('Ctrl Pts',(103.377085716321,-5.08536257553889,
133.616976121092));
#255030=CARTESIAN_POINT('Ctrl Pts',(103.098638092508,-0.38242960843803,
136.603107558928));
#255031=CARTESIAN_POINT('Ctrl Pts',(102.820190468695,4.6719374860923,134.260473842188));
#255032=CARTESIAN_POINT('Ctrl Pts',(102.541742844882,5.4330222677386,128.741840912539));
#255033=CARTESIAN_POINT('Ctrl Pts',(102.263295221069,1.2014250032263,125.118562832119));
#255034=CARTESIAN_POINT('Ctrl Pts',(101.984847597256,-4.13422314637653,
126.720255149861));
#255035=CARTESIAN_POINT('Ctrl Pts',(101.706399973443,-5.67072219248816,
132.07504087278));
#255036=CARTESIAN_POINT('Ctrl Pts',(101.427952349631,-1.99610457388343,
136.262133517338));
#255037=CARTESIAN_POINT('Ctrl Pts',(101.149504725818,3.51283563299066,135.433799494034));
#255038=CARTESIAN_POINT('Ctrl Pts',(100.871057102005,5.7936515047074,130.351237303918));
#255039=CARTESIAN_POINT('Ctrl Pts',(100.592609478192,2.75038467920892,125.685073302739));
#255040=CARTESIAN_POINT('Ctrl Pts',(100.314161854379,-2.82035130272114,
125.723284252797));
#255041=CARTESIAN_POINT('Ctrl Pts',(100.035714230566,-5.79932221927147,
130.430756157697));
#255042=CARTESIAN_POINT('Ctrl Pts',(99.7572666067534,-3.44899932895201,
135.481552309624));
#255043=CARTESIAN_POINT('Ctrl Pts',(99.4788189829407,2.07078545168999,136.234237790066));
#255044=CARTESIAN_POINT('Ctrl Pts',(99.2003713591278,5.6876195657222,131.997131413226));
#255045=CARTESIAN_POINT('Ctrl Pts',(98.9219237353147,4.07780915451857,126.663926945268));
#255046=CARTESIAN_POINT('Ctrl Pts',(98.6434761115021,-1.27930865763567,
125.13557875072));
#255047=CARTESIAN_POINT('Ctrl Pts',(98.3650284876889,-5.460804311125,128.816564156414));
#255048=CARTESIAN_POINT('Ctrl Pts',(98.0865808638763,-4.62408757781209,
134.324237400649));
#255049=CARTESIAN_POINT('Ctrl Pts',(97.8081332400632,0.461939740273397,
136.597315836771));
#255050=CARTESIAN_POINT('Ctrl Pts',(97.5296856162504,5.12346700405862,133.546951428038));
#255051=CARTESIAN_POINT('Ctrl Pts',(97.2512379924375,5.07677838639178,127.97628004749));
#255052=CARTESIAN_POINT('Ctrl Pts',(96.9727903686245,0.364778446043045,
125.004476551425));
#255053=CARTESIAN_POINT('Ctrl Pts',(96.6943427448119,-4.68243506580139,
127.362483172053));
#255054=CARTESIAN_POINT('Ctrl Pts',(96.4158951209985,-5.42671950184442,
132.883407020047));
#255055=CARTESIAN_POINT('Ctrl Pts',(96.1374474971861,-1.18411382567837,
136.493788791223));
#255056=CARTESIAN_POINT('Ctrl Pts',(95.8589998733729,4.14663460910971,134.875864014826));
#255057=CARTESIAN_POINT('Ctrl Pts',(95.5805522495601,5.66682841248846,129.516426520346));
#255058=CARTESIAN_POINT('Ctrl Pts',(95.3021046257473,1.97948374474885,125.340537542131));
#255059=CARTESIAN_POINT('Ctrl Pts',(95.0236570019342,-3.52690978125809,
126.185635047646));
#255060=CARTESIAN_POINT('Ctrl Pts',(94.7452093781216,-5.79224551741027,
131.275115714627));
#255061=CARTESIAN_POINT('Ctrl Pts',(94.4667617543085,-2.73479058998699,
135.931995445075));
#255062=CARTESIAN_POINT('Ctrl Pts',(94.1883141304955,2.8358032876865,135.876829267928));
#255063=CARTESIAN_POINT('Ctrl Pts',(93.909866506683,5.80043248066857,131.160312204968));
#255064=CARTESIAN_POINT('Ctrl Pts',(93.6314188828698,3.43474759079615,126.116693022386));
#255065=CARTESIAN_POINT('Ctrl Pts',(93.352971259057,-2.08730253826965,125.380811354481));
#255066=CARTESIAN_POINT('Ctrl Pts',(93.0745236352441,-5.69122360506351,
129.628906504239));
#255067=CARTESIAN_POINT('Ctrl Pts',(92.7960760114314,-4.06518821053398,
134.957186560018));
#255068=CARTESIAN_POINT('Ctrl Pts',(92.5176283876181,1.29655655399172,136.469222451509));
#255069=CARTESIAN_POINT('Ctrl Pts',(92.2391807638055,5.46682918570788,132.775527061492));
#255070=CARTESIAN_POINT('Ctrl Pts',(91.9607331399925,4.61335286521161,127.270426006341));
#255071=CARTESIAN_POINT('Ctrl Pts',(91.6822855161797,-0.479569363597252,
125.012838216602));
#255072=CARTESIAN_POINT('Ctrl Pts',(91.4038378923669,-5.13179077552621,
128.077376581749));
#255073=CARTESIAN_POINT('Ctrl Pts',(91.1253902685539,-5.06814716666323,
133.647880055237));
#255074=CARTESIAN_POINT('Ctrl Pts',(90.846942644741,-0.347123904390365,
136.605328079151));
#255075=CARTESIAN_POINT('Ctrl Pts',(90.5684950209282,4.69288926807169,134.231970398883));
#255076=CARTESIAN_POINT('Ctrl Pts',(90.2900473971151,5.42036646356212,128.708806777632));
#255077=CARTESIAN_POINT('Ctrl Pts',(90.0115997733025,1.16679167866171,125.111354761782));
#255078=CARTESIAN_POINT('Ctrl Pts',(89.7331521494893,-4.15900765798632,
126.7454970086));
#255079=CARTESIAN_POINT('Ctrl Pts',(89.4547045256766,-5.66288213576447,
132.109536625546));
#255080=CARTESIAN_POINT('Ctrl Pts',(89.1762569018636,-1.96284457794726,
136.274183252551));
#255081=CARTESIAN_POINT('Ctrl Pts',(88.8978092780507,3.5409512567151,135.412330093694));
#255082=CARTESIAN_POINT('Ctrl Pts',(88.619361654238,5.79078587154194,130.3159780981));
#255083=CARTESIAN_POINT('Ctrl Pts',(88.3409140304249,2.71917116603865,125.668425779081));
#255084=CARTESIAN_POINT('Ctrl Pts',(88.0624664066122,-2.85122900215762,
125.740546672265));
#255085=CARTESIAN_POINT('Ctrl Pts',(87.7840187827991,-5.80148900765152,
130.466065200115));
#255086=CARTESIAN_POINT('Ctrl Pts',(87.5055711589863,-3.42046403360785,
135.502460689953));
#255087=CARTESIAN_POINT('Ctrl Pts',(87.2271235351733,2.10380028836375,136.221531728214));
#255088=CARTESIAN_POINT('Ctrl Pts',(86.9486759113605,5.69477492168681,131.962487159311));
#255089=CARTESIAN_POINT('Ctrl Pts',(86.6702282875477,4.05252960720113,126.63918087617));
#255090=CARTESIAN_POINT('Ctrl Pts',(86.3917806637346,-1.31379243922498,
125.14347129503));
#255091=CARTESIAN_POINT('Ctrl Pts',(86.113333039922,-5.47280341633199,128.849842451481));
#255092=CARTESIAN_POINT('Ctrl Pts',(85.8348854161089,-4.6025754151404,134.352320319043));
#255093=CARTESIAN_POINT('Ctrl Pts',(85.5564377922961,0.497194544256039,
136.594396548415));
#255094=CARTESIAN_POINT('Ctrl Pts',(85.2779901684829,5.1400670067851,133.515712616316));
#255095=CARTESIAN_POINT('Ctrl Pts',(84.9995425446705,5.05946899631168,127.945428654274));
#255096=CARTESIAN_POINT('Ctrl Pts',(84.7210949208572,0.329466147029263,
125.002363499906));
#255097=CARTESIAN_POINT('Ctrl Pts',(84.4426472970446,-4.70329999605691,
127.391050253351));
#255098=CARTESIAN_POINT('Ctrl Pts',(84.1641996732315,-5.41396321174535,
132.916402482027));
#255099=CARTESIAN_POINT('Ctrl Pts',(83.8857520494189,-1.14945872264635,
136.500891416245));
#255100=CARTESIAN_POINT('Ctrl Pts',(83.6073044256056,4.17134217838416,134.850546837477));
#255101=CARTESIAN_POINT('Ctrl Pts',(83.328856801793,5.65888339887398,129.481954789796));
#255102=CARTESIAN_POINT('Ctrl Pts',(83.05040917798,1.94618722762166,125.328589094719));
#255103=CARTESIAN_POINT('Ctrl Pts',(82.7719615541671,-3.5549599292834,126.207189922827));
#255104=CARTESIAN_POINT('Ctrl Pts',(82.4935139303543,-5.78927258062435,
131.310366035126));
#255105=CARTESIAN_POINT('Ctrl Pts',(82.2150663065413,-2.70352655206008,
135.948547888425));
#255106=CARTESIAN_POINT('Ctrl Pts',(81.9366186827285,2.86662830323276,135.859472947324));
#255107=CARTESIAN_POINT('Ctrl Pts',(81.6581710589156,5.80249179043285,131.124996731141));
#255108=CARTESIAN_POINT('Ctrl Pts',(81.3797234351026,3.40614878970799,126.095871590527));
#255109=CARTESIAN_POINT('Ctrl Pts',(81.1012758112897,-2.12027854913937,
125.393617843285));
#255110=CARTESIAN_POINT('Ctrl Pts',(80.822828187477,-5.6982734826932,129.663572376127));
#255111=CARTESIAN_POINT('Ctrl Pts',(80.5443805636639,-4.03983346178761,
134.981855572247));
#255112=CARTESIAN_POINT('Ctrl Pts',(80.2659329398512,1.33101615366455,136.461224986989));
#255113=CARTESIAN_POINT('Ctrl Pts',(79.9874853160382,5.47872694765296,132.742212399419));
#255114=CARTESIAN_POINT('Ctrl Pts',(79.7090376922254,4.59175532743923,127.242408693648));
#255115=CARTESIAN_POINT('Ctrl Pts',(79.4305900684125,-0.514815118972584,
125.015864794932));
#255116=CARTESIAN_POINT('Ctrl Pts',(79.1521424445996,-5.1482956211654,128.108665773475));
#255117=CARTESIAN_POINT('Ctrl Pts',(78.8736948207867,-5.05074395573051,
133.678678621723));
#255118=CARTESIAN_POINT('Ctrl Pts',(78.5952471969738,-0.31180533753877,
136.607333642391));
#255119=CARTESIAN_POINT('Ctrl Pts',(78.3167995731609,4.71366715331346,134.203339944237));
#255120=CARTESIAN_POINT('Ctrl Pts',(78.0383519493481,5.407509805713,128.675850294243));
#255121=CARTESIAN_POINT('Ctrl Pts',(77.7599043255351,1.1321151182024,125.104357647873));
#255122=CARTESIAN_POINT('Ctrl Pts',(77.4814567017223,-4.18363805603787,
126.770889270024));
#255123=CARTESIAN_POINT('Ctrl Pts',(77.2030090779094,-5.65483223886072,
132.143984014535));
#255124=CARTESIAN_POINT('Ctrl Pts',(76.9245614540965,-1.92951184808342,
136.286030301474));
#255125=CARTESIAN_POINT('Ctrl Pts',(76.6461138302835,3.56893566918854,135.390689943351));
#255126=CARTESIAN_POINT('Ctrl Pts',(76.3676662064707,5.78770565867644,130.280736989476));
#255127=CARTESIAN_POINT('Ctrl Pts',(76.0892185826578,2.68785689298084,125.651968569378));
#255128=CARTESIAN_POINT('Ctrl Pts',(75.8107709588449,-2.8820010482549,125.75799673322));
#255129=CARTESIAN_POINT('Ctrl Pts',(75.532323335032,-5.8034408197229,130.501386778194));
#255130=CARTESIAN_POINT('Ctrl Pts',(75.2538757112192,-3.39180199171105,
135.523194980456));
#255131=CARTESIAN_POINT('Ctrl Pts',(74.9754280874062,2.13673716794415,136.208624931095));
#255132=CARTESIAN_POINT('Ctrl Pts',(74.6969804635933,5.70171925567246,131.92779999059));
#255133=CARTESIAN_POINT('Ctrl Pts',(74.4185328397805,4.02709989190878,126.61458914934));
#255134=CARTESIAN_POINT('Ctrl Pts',(74.1400852159675,-1.34822753775231,
125.151573605674));
#255135=CARTESIAN_POINT('Ctrl Pts',(73.8616375921548,-5.48459972479585,
128.883193171938));
#255136=CARTESIAN_POINT('Ctrl Pts',(73.5831899683417,-4.58089270234404,
134.380271766487));
#255137=CARTESIAN_POINT('Ctrl Pts',(73.3047423445289,0.532430924512096,
136.591262708148));
#255138=CARTESIAN_POINT('Ctrl Pts',(73.026294720716,5.15647654243839,133.484373334449));
#255139=CARTESIAN_POINT('Ctrl Pts',(72.7478470969032,5.04197212574731,127.914683199832));
#255140=CARTESIAN_POINT('Ctrl Pts',(72.46939947309,0.294141639526237,125.000465443524));
#255141=CARTESIAN_POINT('Ctrl Pts',(72.1909518492774,-4.72399064380143,
127.419743816117));
#255142=CARTESIAN_POINT('Ctrl Pts',(71.9125042254643,-5.40100630524849,
132.949319681519));
#255143=CARTESIAN_POINT('Ctrl Pts',(71.6340566016516,-1.11476102599866,
136.507782954223));
#255144=CARTESIAN_POINT('Ctrl Pts',(71.3556089778387,4.19589517704018,134.82507972721));
#255145=CARTESIAN_POINT('Ctrl Pts',(71.0771613540258,5.65072869325411,129.447532061481));
#255146=CARTESIAN_POINT('Ctrl Pts',(70.7987137302128,1.91281859381102,125.316843554035));
#255147=CARTESIAN_POINT('Ctrl Pts',(70.5202661064001,-3.58287834696108,
126.22891514786));
#255148=CARTESIAN_POINT('Ctrl Pts',(70.241818482587,-5.78608512021397,131.345597605407));
#255149=CARTESIAN_POINT('Ctrl Pts',(69.9633708587742,-2.67216233396265,
135.964909712024));
#255150=CARTESIAN_POINT('Ctrl Pts',(69.6849232349613,2.89734709481291,135.841929307673));
#255151=CARTESIAN_POINT('Ctrl Pts',(69.4064756111484,5.80433608672999,131.089669376025));
#255152=CARTESIAN_POINT('Ctrl Pts',(69.1280279873355,3.37742377252397,126.07522463346));
#255153=CARTESIAN_POINT('Ctrl Pts',(68.8495803635227,-2.15317599230747,
125.406624829152));
#255154=CARTESIAN_POINT('Ctrl Pts',(68.5711327397097,-5.70511220870344,
129.698280520343));
#255155=CARTESIAN_POINT('Ctrl Pts',(68.2926851158969,-4.01432901552682,
135.006369785865));
#255156=CARTESIAN_POINT('Ctrl Pts',(68.014237492084,1.36542643204398,136.45301790528));
#255157=CARTESIAN_POINT('Ctrl Pts',(67.735789868271,5.49042169335597,132.708825929535));
#255158=CARTESIAN_POINT('Ctrl Pts',(67.4573422444582,4.56998764048497,127.214523370394));
#255159=CARTESIAN_POINT('Ctrl Pts',(67.1788946206453,-0.550041797684044,
125.019105868103));
#255160=CARTESIAN_POINT('Ctrl Pts',(66.9004469968323,-5.164609694817,128.140054855163));
#255161=CARTESIAN_POINT('Ctrl Pts',(66.6219993730196,-5.03315358762317,
133.709370679297));
#255162=CARTESIAN_POINT('Ctrl Pts',(66.3435517492066,-0.2764752166261,136.609124174332));
#255163=CARTESIAN_POINT('Ctrl Pts',(66.0651041253938,4.73427037188528,134.174583539162));
#255164=CARTESIAN_POINT('Ctrl Pts',(65.7866565015808,5.39445277059944,128.642972683589));
#255165=CARTESIAN_POINT('Ctrl Pts',(65.508208877768,1.0973966068015,125.097571749668));
#255166=CARTESIAN_POINT('Ctrl Pts',(65.2297612539551,-4.20811342784249,
126.796430993211));
#255167=CARTESIAN_POINT('Ctrl Pts',(64.9513136301422,-5.64657280006891,
132.178381763287));
#255168=CARTESIAN_POINT('Ctrl Pts',(64.6728660063292,-1.89610761944867,
136.297674225111));
#255169=CARTESIAN_POINT('Ctrl Pts',(64.3944183825164,3.59678783343796,135.368879844889));
#255170=CARTESIAN_POINT('Ctrl Pts',(64.1159707587035,5.78441098024938,130.245515283918));
#255171=CARTESIAN_POINT('Ctrl Pts',(63.8375231348906,2.65644302039782,125.635702283457));
#255172=CARTESIAN_POINT('Ctrl Pts',(63.5590755110777,-2.91266630074331,
125.775633789045));
#255173=CARTESIAN_POINT('Ctrl Pts',(63.2806278872649,-5.80517758316048,
130.53671958308));
#255174=CARTESIAN_POINT('Ctrl Pts',(63.0021802634519,-3.36301426534433,
135.543754412816));
#255175=CARTESIAN_POINT('Ctrl Pts',(62.723732639639,2.16959486994269,136.195517876976));
#255176=CARTESIAN_POINT('Ctrl Pts',(62.4452850158262,5.70845231035428,131.893071192411));
#255177=CARTESIAN_POINT('Ctrl Pts',(62.1668373920132,4.00152095094907,126.590152676031));
#255178=CARTESIAN_POINT('Ctrl Pts',(61.8883897682004,-1.38261267721222,
125.159885382419));
#255179=CARTESIAN_POINT('Ctrl Pts',(61.6099421443874,-5.49619279939966,
128.916615081961));
#255180=CARTESIAN_POINT('Ctrl Pts',(61.3314945205747,-4.55904024288434,
134.408090707227));
#255181=CARTESIAN_POINT('Ctrl Pts',(61.0530468967616,0.567647575344072,
136.587914432096));
#255182=CARTESIAN_POINT('Ctrl Pts',(60.7745992729488,5.17269500295686,133.452934743723));
#255183=CARTESIAN_POINT('Ctrl Pts',(60.496151649136,5.02428842305186,127.884044823451));
#255184=CARTESIAN_POINT('Ctrl Pts',(60.2177040253229,0.258806232497024,
124.998782452612));
#255185=CARTESIAN_POINT('Ctrl Pts',(59.9392564015102,-4.74450624233532,
127.448562797104));
#255186=CARTESIAN_POINT('Ctrl Pts',(59.6608087776971,-5.38784926247686,
132.982157398764));
#255187=CARTESIAN_POINT('Ctrl Pts',(59.3823611538844,-1.08002202147149,
136.514463149789));
#255188=CARTESIAN_POINT('Ctrl Pts',(59.1039135300714,4.22029269525717,134.799463627718));
#255189=CARTESIAN_POINT('Ctrl Pts',(58.8254659062585,5.64236459780459,129.413159610949));
#255190=CARTESIAN_POINT('Ctrl Pts',(58.5470182824457,1.8793790798041,125.305301355313));
#255191=CARTESIAN_POINT('Ctrl Pts',(58.2685706586328,-3.61066399976409,
126.250809917708));
#255192=CARTESIAN_POINT('Ctrl Pts',(57.9901230348199,-5.78268325429153,
131.380809119953));
#255193=CARTESIAN_POINT('Ctrl Pts',(57.711675411007,-2.64069909790739,135.981080309579));
#255194=CARTESIAN_POINT('Ctrl Pts',(57.4332277871941,2.92795852413098,135.824198999061));
#255195=CARTESIAN_POINT('Ctrl Pts',(57.1547801633813,5.80596530121877,131.054331448687));
#255196=CARTESIAN_POINT('Ctrl Pts',(56.8763325395683,3.34857360366007,126.054752916266));
#255197=CARTESIAN_POINT('Ctrl Pts',(56.5978849157555,-2.18599364874745,
125.419831830104));
#255198=CARTESIAN_POINT('Ctrl Pts',(56.3194372919424,-5.71173952968275,
129.733029650764));
#255199=CARTESIAN_POINT('Ctrl Pts',(56.0409896681298,-3.98867581682796,
135.030728292487));
#255200=CARTESIAN_POINT('Ctrl Pts',(55.7625420443167,1.39978611404518,136.444601510497));
#255201=CARTESIAN_POINT('Ctrl Pts',(55.4840944205039,5.50191298946419,132.675368888989));
#255202=CARTESIAN_POINT('Ctrl Pts',(55.2056467966909,4.54805061095778,127.186771069878));
#255203=CARTESIAN_POINT('Ctrl Pts',(54.9271991728781,-0.585248094394635,
125.022561316018));
#255204=CARTESIAN_POINT('Ctrl Pts',(54.6487515490652,-5.18073239195715,
128.171542663682));
#255205=CARTESIAN_POINT('Ctrl Pts',(54.3703039252523,-5.01537671415865,
133.739955090657));
#255206=CARTESIAN_POINT('Ctrl Pts',(54.0918563014394,-0.241134850822232,
136.610699608625));
#255207=CARTESIAN_POINT('Ctrl Pts',(53.8134086776265,4.75469816032759,134.145702249237));
#255208=CARTESIAN_POINT('Ctrl Pts',(53.5349610538137,5.38119584205463,128.610175163959));
#255209=CARTESIAN_POINT('Ctrl Pts',(53.2565134300007,1.06263743096531,125.090997318624));
#255210=CARTESIAN_POINT('Ctrl Pts',(52.9780658061879,-4.23243286645675,
126.822121231705));
#255211=CARTESIAN_POINT('Ctrl Pts',(52.6996181823749,-5.63810412544538,
132.21272859718));
#255212=CARTESIAN_POINT('Ctrl Pts',(52.4211705585621,-1.86263312984859,
136.309114591992));
#255213=CARTESIAN_POINT('Ctrl Pts',(52.1427229347491,3.62450671739182,135.346900606486));
#255214=CARTESIAN_POINT('Ctrl Pts',(51.8642753109363,5.7809019583462,130.210314286579));
#255215=CARTESIAN_POINT('Ctrl Pts',(51.5858276871234,2.62493071234137,125.619627524071));
#255216=CARTESIAN_POINT('Ctrl Pts',(51.3073800633105,-2.94322362331098,
125.793457186192));
#255217=CARTESIAN_POINT('Ctrl Pts',(51.0289324394976,-5.80669923360788,
130.572062305503));
#255218=CARTESIAN_POINT('Ctrl Pts',(50.7504848156848,-3.33410192124705,
135.564138225197));
#255219=CARTESIAN_POINT('Ctrl Pts',(50.4720371918718,2.20237217680579,136.182211051539));
#255220=CARTESIAN_POINT('Ctrl Pts',(50.193589568059,5.71497383623647,131.858302051661));
#255221=CARTESIAN_POINT('Ctrl Pts',(49.915141944246,3.97579373215887,126.565872361749));
#255222=CARTESIAN_POINT('Ctrl Pts',(49.6366943204332,-1.41694658345112,
125.168406317271));
#255223=CARTESIAN_POINT('Ctrl Pts',(49.3582466966203,-5.50758221055828,
128.950106943089));
#255224=CARTESIAN_POINT('Ctrl Pts',(49.0797990728074,-4.53701884651156,
134.435776110423));
#255225=CARTESIAN_POINT('Ctrl Pts',(48.8013514489945,0.602843191786665,
136.584351844331));
#255226=CARTESIAN_POINT('Ctrl Pts',(48.5229038251815,5.18872178735999,133.421398009111));
#255227=CARTESIAN_POINT('Ctrl Pts',(48.2444562013688,5.006418543501,127.853514660444));
#255228=CARTESIAN_POINT('Ctrl Pts',(47.9660085775558,0.223461235307256,
124.997314589534));
#255229=CARTESIAN_POINT('Ctrl Pts',(47.6875609537429,-4.7648460314457,127.477506128414));
#255230=CARTESIAN_POINT('Ctrl Pts',(47.40911332993,-5.37449257096935,133.014914416948));
#255231=CARTESIAN_POINT('Ctrl Pts',(47.1306657061172,-1.04524299633083,
136.520931755405));
#255232=CARTESIAN_POINT('Ctrl Pts',(46.8522180823042,4.24453382897653,134.773699488214));
#255233=CARTESIAN_POINT('Ctrl Pts',(46.5737704584914,5.6337914224598,129.378838711881));
#255234=CARTESIAN_POINT('Ctrl Pts',(46.2953228346785,1.84586992471411,125.293962926255));
#255235=CARTESIAN_POINT('Ctrl Pts',(46.0168752108656,-3.63831585808481,
126.272873421051));
#255236=CARTESIAN_POINT('Ctrl Pts',(45.7384275870526,-5.77906710891461,
131.415999273987));
#255237=CARTESIAN_POINT('Ctrl Pts',(45.4599799632399,-2.60913800977569,
135.997059081882));
#255238=CARTESIAN_POINT('Ctrl Pts',(45.1815323394269,2.95846145686929,135.806282678493));
#255239=CARTESIAN_POINT('Ctrl Pts',(44.903084715614,5.80737937352832,131.018984258588));
#255240=CARTESIAN_POINT('Ctrl Pts',(44.6246370918012,3.31959935216964,126.034457197533));
#255241=CARTESIAN_POINT('Ctrl Pts',(44.3461894679882,-2.21873030238901,
125.43323835675));
#255242=CARTESIAN_POINT('Ctrl Pts',(44.0677418441753,-5.7181552000533,129.767818479747));
#255243=CARTESIAN_POINT('Ctrl Pts',(43.7892942203624,-3.96287481627985,
135.054930189501));
#255244=CARTESIAN_POINT('Ctrl Pts',(43.5108465965496,1.43409392645716,136.435976114513));
#255245=CARTESIAN_POINT('Ctrl Pts',(43.2323989727367,5.51320041016325,132.641842517543));
#255246=CARTESIAN_POINT('Ctrl Pts',(42.9539513489238,4.52594505174265,127.159152820475));
#255247=CARTESIAN_POINT('Ctrl Pts',(42.6755037251109,-0.620432704521861,
125.026231010632));
#255248=CARTESIAN_POINT('Ctrl Pts',(42.397056101298,-5.19666311515333,128.203128032237));
#255249=CARTESIAN_POINT('Ctrl Pts',(42.1186084774851,-4.99741399406557,
133.770430722483));
#255250=CARTESIAN_POINT('Ctrl Pts',(41.8401608536722,-0.205785549677785,
136.612059886891));
#255251=CARTESIAN_POINT('Ctrl Pts',(41.5617132298594,4.77494976168102,134.11669714467));
#255252=CARTESIAN_POINT('Ctrl Pts',(41.2832656060464,5.36773951131901,128.577458950676));
#255253=CARTESIAN_POINT('Ctrl Pts',(41.0048179822336,1.02783887870806,125.084634598359));
#255254=CARTESIAN_POINT('Ctrl Pts',(40.7263703584206,-4.25659547071474,
126.847959033542));
#255255=CARTESIAN_POINT('Ctrl Pts',(40.4479227346078,-5.62942652880005,
132.24702324348));
#255256=CARTESIAN_POINT('Ctrl Pts',(40.1694751107948,-1.82908961969292,
136.320350978189));
#255257=CARTESIAN_POINT('Ctrl Pts',(39.891027486982,3.65209129391637,135.324753042595));
#255258=CARTESIAN_POINT('Ctrl Pts',(39.6125798631691,5.77717872299504,130.175135301845));
#255259=CARTESIAN_POINT('Ctrl Pts',(39.3341322393562,2.59332113651206,125.603744886877));
#255260=CARTESIAN_POINT('Ctrl Pts',(39.0556846155433,-2.97367188364494,
125.811466264208));
#255261=CARTESIAN_POINT('Ctrl Pts',(38.7772369917304,-5.80800571467979,
130.607413635826));
#255262=CARTESIAN_POINT('Ctrl Pts',(38.4987893679175,-3.30506603077697,
135.584345662267));
#255263=CARTESIAN_POINT('Ctrl Pts',(38.2203417441046,2.23506787395795,136.16870494788));
#255264=CARTESIAN_POINT('Ctrl Pts',(37.9418941202917,5.72128359166147,131.823493856722));
#255265=CARTESIAN_POINT('Ctrl Pts',(37.6634464964789,3.94991918886983,126.541749106207));
#255266=CARTESIAN_POINT('Ctrl Pts',(37.3849988726659,-1.45122798421329,
125.177136094481));
#255267=CARTESIAN_POINT('Ctrl Pts',(37.1065512488531,-5.51876753623267,
128.983667514269));
#255268=CARTESIAN_POINT('Ctrl Pts',(36.8281036250402,-4.51482932923697,
134.463326950183));
#255269=CARTESIAN_POINT('Ctrl Pts',(36.5496560012273,0.6380164696531,136.580575076865));
#255270=CARTESIAN_POINT('Ctrl Pts',(36.2712083774144,5.20455630176915,133.389764299214));
#255271=CARTESIAN_POINT('Ctrl Pts',(35.9927607536015,4.9883631492699,127.82309384212));
#255272=CARTESIAN_POINT('Ctrl Pts',(35.7143131297886,0.188107957679239,
124.996061908681));
#255273=CARTESIAN_POINT('Ctrl Pts',(35.4358655059757,-4.78500925743413,
127.50657273754));
#255274=CARTESIAN_POINT('Ctrl Pts',(35.1574178821628,-5.36093672566315,
133.047589522248));
#255275=CARTESIAN_POINT('Ctrl Pts',(34.87897025835,-1.01042523932657,136.527188531377));
#255276=CARTESIAN_POINT('Ctrl Pts',(34.6005226345371,4.26861767993396,134.747788263399));
#255277=CARTESIAN_POINT('Ctrl Pts',(34.3220750107242,5.62500948490202,129.34457063605));
#255278=CARTESIAN_POINT('Ctrl Pts',(34.0436273869112,1.81229237023524,125.282828687009));
#255279=CARTESIAN_POINT('Ctrl Pts',(33.7651797630984,-3.66583289727342,
126.295104840318));
#255280=CARTESIAN_POINT('Ctrl Pts',(33.4867321392855,-5.77523681808073,
131.451166763527));
#255281=CARTESIAN_POINT('Ctrl Pts',(33.2082845154725,-2.57748023907555,
136.012845436834));
#255282=CARTESIAN_POINT('Ctrl Pts',(32.9298368916598,2.98885476273036,135.788181009863));
#255283=CARTESIAN_POINT('Ctrl Pts',(32.6513892678468,5.80857825125962,130.983629115531));
#255284=CARTESIAN_POINT('Ctrl Pts',(32.3729416440339,3.29050209170421,126.014338229324));
#255285=CARTESIAN_POINT('Ctrl Pts',(32.094494020221,-2.25138474016344,125.446843912307));
#255286=CARTESIAN_POINT('Ctrl Pts',(31.8160463964081,-5.72435898208005,
129.802645718181));
#255287=CARTESIAN_POINT('Ctrl Pts',(31.5375987725953,-3.93692696994811,
135.078974580096));
#255288=CARTESIAN_POINT('Ctrl Pts',(31.2591511487823,1.46834859799131,136.427142036947));
#255289=CARTESIAN_POINT('Ctrl Pts',(30.9807035249695,5.52428353719365,132.608248057529));
#255290=CARTESIAN_POINT('Ctrl Pts',(30.7022559011566,4.50367178196922,127.131669645585));
#255291=CARTESIAN_POINT('Ctrl Pts',(30.4238082773436,-0.655594324287056,
125.030114815962));
#255292=CARTESIAN_POINT('Ctrl Pts',(30.1453606535308,-5.21240127408669,
128.234809790423));
#255293=CARTESIAN_POINT('Ctrl Pts',(29.8669130297179,-4.97926609295916,
133.80079644549));
#255294=CARTESIAN_POINT('Ctrl Pts',(29.588465405905,-0.170428623074124,
136.613204958723));
#255295=CARTESIAN_POINT('Ctrl Pts',(29.3100177820921,4.79502442551506,134.087569300254));
#255296=CARTESIAN_POINT('Ctrl Pts',(29.0315701582792,5.35408427702179,128.544825256054));
#255297=CARTESIAN_POINT('Ctrl Pts',(28.7531225344664,0.99300223950345,125.078483824645));
#255298=CARTESIAN_POINT('Ctrl Pts',(28.4746749106534,-4.28060034526213,
126.873943441297));
#255299=CARTESIAN_POINT('Ctrl Pts',(28.1962272868406,-5.6205403316845,132.281264431386));
#255300=CARTESIAN_POINT('Ctrl Pts',(27.9177796630277,-1.79547833194873,
136.331382967337));
#255301=CARTESIAN_POINT('Ctrl Pts',(27.6393320392148,3.67954054085496,135.3024379739));
#255302=CARTESIAN_POINT('Ctrl Pts',(27.3608844154018,5.77324141216173,130.139979633288));
#255303=CARTESIAN_POINT('Ctrl Pts',(27.082436791589,2.56161546421434,125.58805496041));
#255304=CARTESIAN_POINT('Ctrl Pts',(26.8039891677761,-3.00400995347367,
125.82966035576));
#255305=CARTESIAN_POINT('Ctrl Pts',(26.5255415439632,-5.80909697796402,
130.642772264091));
#255306=CARTESIAN_POINT('Ctrl Pts',(26.2470939201503,-3.27590766986969,
135.604375975235));
#255307=CARTESIAN_POINT('Ctrl Pts',(25.9686462963375,2.2676807498481,136.155000066467));
#255308=CARTESIAN_POINT('Ctrl Pts',(25.6901986725246,5.727381342819,131.788647897428));
#255309=CARTESIAN_POINT('Ctrl Pts',(25.4117510487116,3.92389827987267,126.517783803302));
#255310=CARTESIAN_POINT('Ctrl Pts',(25.1333034248988,-1.48545560918882,
125.186074390566));
#255311=CARTESIAN_POINT('Ctrl Pts',(24.8548558010858,-5.5297483619465,129.017295551901));
#255312=CARTESIAN_POINT('Ctrl Pts',(24.576408177273,-4.49247251330123,134.490742205601));
#255313=CARTESIAN_POINT('Ctrl Pts',(24.2979605534601,0.673166105584617,
136.576584269648));
#255314=CARTESIAN_POINT('Ctrl Pts',(24.0195129296472,5.22019795943058,133.358034786234));
#255315=CARTESIAN_POINT('Ctrl Pts',(23.7410653058343,4.97012290940784,127.792783495733));
#255316=CARTESIAN_POINT('Ctrl Pts',(23.4626176820214,0.152747709641667,
124.995024456474));
#255317=CARTESIAN_POINT('Ctrl Pts',(23.1841700582085,-4.80499517314482,
127.53576154741));
#255318=CARTESIAN_POINT('Ctrl Pts',(22.9057224343956,-5.34718222887511,
133.080181503877));
#255319=CARTESIAN_POINT('Ctrl Pts',(22.6272748105827,-0.975570040643468,
136.533233245855));
#255320=CARTESIAN_POINT('Ctrl Pts',(22.3488271867698,4.29254335569345,134.721730913422));
#255321=CARTESIAN_POINT('Ctrl Pts',(22.070379562957,5.61601911054919,129.310356653276));
#255322=CARTESIAN_POINT('Ctrl Pts',(21.791931939144,1.77864766059611,125.27189905016));
#255323=CARTESIAN_POINT('Ctrl Pts',(21.5134843153312,-3.69321409767591,
126.317503351717));
#255324=CARTESIAN_POINT('Ctrl Pts',(21.2350366915183,-5.77119252372273,
131.486310285425));
#255325=CARTESIAN_POINT('Ctrl Pts',(20.9565890677054,-2.54572695889727,
136.028438789465));
#255326=CARTESIAN_POINT('Ctrl Pts',(20.6781414438925,3.01913731547902,135.769894663934));
#255327=CARTESIAN_POINT('Ctrl Pts',(20.3996938200796,5.80956188998761,130.948267329615));
#255328=CARTESIAN_POINT('Ctrl Pts',(20.1212461962667,3.26128290047392,125.994396757156));
#255329=CARTESIAN_POINT('Ctrl Pts',(19.8427985724538,-2.28395575204823,
125.460647992615));
#255330=CARTESIAN_POINT('Ctrl Pts',(19.5643509486409,-5.7303506458796,129.837510075529));
#255331=CARTESIAN_POINT('Ctrl Pts',(19.285903324828,-3.91083323933969,135.102860573299));
#255332=CARTESIAN_POINT('Ctrl Pts',(19.0074557010152,1.50254885932817,136.418099605148));
#255333=CARTESIAN_POINT('Ctrl Pts',(18.7290080772022,5.53516195986603,132.574586753804));
#255334=CARTESIAN_POINT('Ctrl Pts',(18.4505604533894,4.48123162698169,127.104322563612));
#255335=CARTESIAN_POINT('Ctrl Pts',(18.1721128295765,-0.690731650763477,
125.034212588094));
#255336=CARTESIAN_POINT('Ctrl Pts',(17.8936652057636,-5.22794628557398,
128.26658676426));
#255337=CARTESIAN_POINT('Ctrl Pts',(17.6152175819507,-4.96093368331654,
133.831051134467));
#255338=CARTESIAN_POINT('Ctrl Pts',(17.3367699581378,-0.135065381175154,
136.614134781694));
#255339=CARTESIAN_POINT('Ctrl Pts',(17.0583223343249,4.81492140795562,134.058319795333));
#255340=CARTESIAN_POINT('Ctrl Pts',(16.779874710512,5.34023064516271,128.512275289347));
#255341=CARTESIAN_POINT('Ctrl Pts',(16.5014270866992,0.958128804235671,
125.0725452254));
#255342=CARTESIAN_POINT('Ctrl Pts',(16.2229794628862,-4.30444660058956,
126.900073492105));
#255343=CARTESIAN_POINT('Ctrl Pts',(15.9445318390734,-5.61144586338,132.315450892077));
#255344=CARTESIAN_POINT('Ctrl Pts',(15.6660842152604,-1.76180051209467,
136.342210150638));
#255345=CARTESIAN_POINT('Ctrl Pts',(15.3876365914476,3.70685344106567,135.279956227294));
#255346=CARTESIAN_POINT('Ctrl Pts',(15.1091889676347,5.76909017174479,130.104848583611));
#255347=CARTESIAN_POINT('Ctrl Pts',(14.8307413438218,2.52981487031356,125.572558326068));
#255348=CARTESIAN_POINT('Ctrl Pts',(14.5522937200089,-3.03423670860886,
125.848038786661));
#255349=CARTESIAN_POINT('Ctrl Pts',(14.273846096196,-5.80997298302346,130.678136880072));
#255350=CARTESIAN_POINT('Ctrl Pts',(13.9953984723831,-3.24662791899898,
135.624228421867));
#255351=CARTESIAN_POINT('Ctrl Pts',(13.7169508485702,2.30020959599411,136.141096915141));
#255352=CARTESIAN_POINT('Ctrl Pts',(13.4385032247574,5.73326686375462,131.753765465006));
#255353=CARTESIAN_POINT('Ctrl Pts',(13.1600556009444,3.89773196938174,126.493977341077));
#255354=CARTESIAN_POINT('Ctrl Pts',(12.8816079771316,-1.51962819006047,
125.195220874312));
#255355=CARTESIAN_POINT('Ctrl Pts',(12.6031603533186,-5.54052428080121,
129.050989809886));
#255356=CARTESIAN_POINT('Ctrl Pts',(12.3247127295058,-4.46994922714442,
134.518020860792));
#255357=CARTESIAN_POINT('Ctrl Pts',(12.0462651056929,0.708290797098533,
136.572379570561));
#255358=CARTESIAN_POINT('Ctrl Pts',(11.76781748188,5.23564618073708,133.326210645918));
#255359=CARTESIAN_POINT('Ctrl Pts',(11.4893698580671,4.95169849981347,127.762584744442));
#255360=CARTESIAN_POINT('Ctrl Pts',(11.2109222342542,0.117381801481337,
124.994202271355));
#255361=CARTESIAN_POINT('Ctrl Pts',(10.9324746104413,-4.82480303799234,
127.565071476419));
#255362=CARTESIAN_POINT('Ctrl Pts',(10.6540269866284,-5.33322959028317,
133.112689154126));
#255363=CARTESIAN_POINT('Ctrl Pts',(10.3755793628155,-0.940678691853753,
136.539065674851));
#255364=CARTESIAN_POINT('Ctrl Pts',(10.0971317390026,4.31630996968034,134.695528403849));
#255365=CARTESIAN_POINT('Ctrl Pts',(9.81868411518972,5.60682063254294,129.276198031366));
#255366=CARTESIAN_POINT('Ctrl Pts',(9.54023649137686,1.74493704251384,125.261174420708));
#255367=CARTESIAN_POINT('Ctrl Pts',(9.26178886756394,-3.72045844467185,
126.340068125262));
#255368=CARTESIAN_POINT('Ctrl Pts',(8.98334124375105,-5.76693437570339,
131.52142853743));
#255369=CARTESIAN_POINT('Ctrl Pts',(8.70489361993813,-2.51387934587036,
136.043838561958));
#255370=CARTESIAN_POINT('Ctrl Pts',(8.42644599612531,3.0493079929842,135.751424318317));
#255371=CARTESIAN_POINT('Ctrl Pts',(8.14799837231237,5.81033025326331,130.912900211183));
#255372=CARTESIAN_POINT('Ctrl Pts',(7.86955074849947,3.23194286120641,125.974633519968));
#255373=CARTESIAN_POINT('Ctrl Pts',(7.59110312468663,-2.3164421311127,125.47465008616));
#255374=CARTESIAN_POINT('Ctrl Pts',(7.31265550087371,-5.73612996942864,
129.872410259879));
#255375=CARTESIAN_POINT('Ctrl Pts',(7.0342078770608,-3.88459459136738,135.126587284006));
#255376=CARTESIAN_POINT('Ctrl Pts',(6.75576025324794,1.53669344316449,136.408849154185));
#255377=CARTESIAN_POINT('Ctrl Pts',(6.47731262943506,5.54583527507644,132.540859853697));
#255378=CARTESIAN_POINT('Ctrl Pts',(6.19886500562214,4.45862541830825,127.077112587908));
#255379=CARTESIAN_POINT('Ctrl Pts',(5.92041738180924,-0.725843381924555,
125.038524175185));
#255380=CARTESIAN_POINT('Ctrl Pts',(5.64196975799638,-5.24329757358911,
128.29845777624));
#255381=CARTESIAN_POINT('Ctrl Pts',(5.36352213418349,-4.94241744445191,
133.861193668313));
#255382=CARTESIAN_POINT('Ctrl Pts',(5.08507451037056,-0.0996971343788212,
136.614849321347));
#255383=CARTESIAN_POINT('Ctrl Pts',(4.80662688655771,4.83463997171276,134.028949713759));
#255384=CARTESIAN_POINT('Ctrl Pts',(4.5281792627448,5.32617912909322,128.479810256704));
#255385=CARTESIAN_POINT('Ctrl Pts',(4.24973163893191,0.923219865152705,
125.066819020683));
#255386=CARTESIAN_POINT('Ctrl Pts',(3.97128401511898,-4.32813335306523,
126.926348217707));
#255387=CARTESIAN_POINT('Ctrl Pts',(3.69283639130614,-5.60214346088543,
132.349581358763));
#255388=CARTESIAN_POINT('Ctrl Pts',(3.41438876749324,-1.72805740807474,
136.352832126888));
#255389=CARTESIAN_POINT('Ctrl Pts',(3.13594114368033,3.73402898245891,135.257308635848));
#255390=CARTESIAN_POINT('Ctrl Pts',(2.85749351986744,5.76472515556999,130.06974345461));
#255391=CARTESIAN_POINT('Ctrl Pts',(2.5790458960546,2.49792053319242,125.557255558086));
#255392=CARTESIAN_POINT('Ctrl Pts',(2.30059827224166,-3.06435102898697,
125.866600875889));
#255393=CARTESIAN_POINT('Ctrl Pts',(2.02215064842876,-5.81063369739741,
130.713506173321));
#255394=CARTESIAN_POINT('Ctrl Pts',(1.74370302461591,-3.21722786313679,
135.643902266527));
#255395=CARTESIAN_POINT('Ctrl Pts',(1.46525540080302,2.33265320702766,136.12699600909));
#255396=CARTESIAN_POINT('Ctrl Pts',(1.18680777699008,5.73893993637821,131.718847852038));
#255397=CARTESIAN_POINT('Ctrl Pts',(0.908360153177235,3.87142122699929,
126.47033060169));
#255398=CARTESIAN_POINT('Ctrl Pts',(0.629912529364331,-1.55374446055069,
125.204575206795));
#255399=CARTESIAN_POINT('Ctrl Pts',(0.351464905551429,-5.55109489349118,
129.084749039672));
#255400=CARTESIAN_POINT('Ctrl Pts',(0.0730172817385382,-4.44726030537518,
134.545161904937));
#255401=CARTESIAN_POINT('Ctrl Pts',(-0.205430342074321,0.743389242636492,
136.56796113541));
#255402=CARTESIAN_POINT('Ctrl Pts',(-0.48387796588724,5.25090039324876,
133.294293057522));
#255403=CARTESIAN_POINT('Ctrl Pts',(-0.762325589700153,4.93309060321035,
127.732498707276));
#255404=CARTESIAN_POINT('Ctrl Pts',(-1.040773213513,0.0820115436953976,
124.993595383789));
#255405=CARTESIAN_POINT('Ctrl Pts',(-1.3192208373259,-4.84443211798899,
127.594501438479));
#255406=CARTESIAN_POINT('Ctrl Pts',(-1.5976684611388,-5.31907932690746,
133.145111268411));
#255407=CARTESIAN_POINT('Ctrl Pts',(-1.8761160849517,-0.905752485869179,
136.544685602242));
#255408=CARTESIAN_POINT('Ctrl Pts',(-2.15456370876455,4.33991664121397,
134.669181705622));
#255409=CARTESIAN_POINT('Ctrl Pts',(-2.43301133257747,5.59741439173625,
129.242096036083));
#255410=CARTESIAN_POINT('Ctrl Pts',(-2.71145895639038,1.71116176514775,
125.250655196059));
#255411=CARTESIAN_POINT('Ctrl Pts',(-2.98990658020324,-3.74756492871192,
126.362798324807));
#255412=CARTESIAN_POINT('Ctrl Pts',(-3.26835420401613,-5.76246253181,131.556520218218));
#255413=CARTESIAN_POINT('Ctrl Pts',(-3.54680182782904,-2.48193858011979,
136.059044183669));
#255414=CARTESIAN_POINT('Ctrl Pts',(-3.82524945164193,3.0793656772603,135.732770657435));
#255415=CARTESIAN_POINT('Ctrl Pts',(-4.1036970754548,5.81088331261472,130.877529070775));
#255416=CARTESIAN_POINT('Ctrl Pts',(-4.38214469926771,3.20248306110764,
125.955049250094));
#255417=CARTESIAN_POINT('Ctrl Pts',(-4.66059232308062,-2.34884267356213,
125.488849674089));
#255418=CARTESIAN_POINT('Ctrl Pts',(-4.93903994689347,-5.7416967385722,
129.907344977992));
#255419=CARTESIAN_POINT('Ctrl Pts',(-5.21748757070636,-3.85821199831392,
135.150153833014));
#255420=CARTESIAN_POINT('Ctrl Pts',(-5.49593519451928,1.57078108426016,
136.399391026839));
#255421=CARTESIAN_POINT('Ctrl Pts',(-5.77438281833216,5.55630308732125,
132.507068606974));
#255422=CARTESIAN_POINT('Ctrl Pts',(-6.05283044214503,4.43585399363028,
127.050040726751));
#255423=CARTESIAN_POINT('Ctrl Pts',(-6.33127806595794,-0.76092821669219,
125.043049417465));
#255424=CARTESIAN_POINT('Ctrl Pts',(-6.60972568977086,-5.25845456928442,
128.330421645371));
#255425=CARTESIAN_POINT('Ctrl Pts',(-6.88817331358369,-4.92371806249131,
133.891222930087));
#255426=CARTESIAN_POINT('Ctrl Pts',(-7.16662093739661,-0.0643251932685087,
136.615348551203));
#255427=CARTESIAN_POINT('Ctrl Pts',(-7.44506856120951,4.8541793861078,133.999460143849));
#255428=CARTESIAN_POINT('Ctrl Pts',(-7.72351618502242,5.3119302494974,128.44743136113));
#255429=CARTESIAN_POINT('Ctrl Pts',(-8.00196380883526,0.888276715818123,
125.06130542268));
#255430=CARTESIAN_POINT('Ctrl Pts',(-8.28041143264819,-4.35165972496785,
126.952766644486));
#255431=CARTESIAN_POINT('Ctrl Pts',(-8.55885905646108,-5.59263346890473,
132.383654566726));
#255432=CARTESIAN_POINT('Ctrl Pts',(-8.83730668027396,-1.69425027025207,
136.363248502487));
#255433=CARTESIAN_POINT('Ctrl Pts',(-9.11575430408684,3.76106615803527,
135.234496038775));
#255434=CARTESIAN_POINT('Ctrl Pts',(-9.39420192789976,5.7601465253845,130.034665547118));
#255435=CARTESIAN_POINT('Ctrl Pts',(-9.67264955171265,2.4659336347071,125.542147223509));
#255436=CARTESIAN_POINT('Ctrl Pts',(-9.95109717552551,-3.09435179871079,
125.885345935621));
#255437=CARTESIAN_POINT('Ctrl Pts',(-10.2295447993384,-5.81107909660284,
130.748878833214));
#255438=CARTESIAN_POINT('Ctrl Pts',(-10.5079924231513,-3.18770859171301,
135.663396780189));
#255439=CARTESIAN_POINT('Ctrl Pts',(-10.7864400469642,2.36501038073878,
136.112697870828));
#255440=CARTESIAN_POINT('Ctrl Pts',(-11.0648876707771,5.74440035047196,
131.683896352409));
#255441=CARTESIAN_POINT('Ctrl Pts',(-11.34333529459,3.84496702767957,126.446844461378));
#255442=CARTESIAN_POINT('Ctrl Pts',(-11.6217829184029,-1.58780315646856,
125.214137041385));
#255443=CARTESIAN_POINT('Ctrl Pts',(-11.9002305422157,-5.56145980831845,
129.118571990297));
#255444=CARTESIAN_POINT('Ctrl Pts',(-12.1786781660286,-4.42440658873985,
134.572164332316));
#255445=CARTESIAN_POINT('Ctrl Pts',(-12.4571257898416,0.778460141612691,
136.563329127923));
#255446=CARTESIAN_POINT('Ctrl Pts',(-12.7355734136544,5.26596003171537,
133.262283203764));
#255447=CARTESIAN_POINT('Ctrl Pts',(-13.0140210374673,4.91429990912079,
127.702526499083));
#255448=CARTESIAN_POINT('Ctrl Pts',(-13.2924686612802,0.0466382469415425,
124.993203816266));
#255449=CARTESIAN_POINT('Ctrl Pts',(-13.5709162850931,-4.86388168577195,
127.624050343051));
#255450=CARTESIAN_POINT('Ctrl Pts',(-13.849363908906,-5.30473196309121,
133.177446645321));
#255451=CARTESIAN_POINT('Ctrl Pts',(-14.1278115327188,-0.87079271689315,
136.550092819781));
#255452=CARTESIAN_POINT('Ctrl Pts',(-14.4062591565318,4.36336249554048,
134.642691795028));
#255453=CARTESIAN_POINT('Ctrl Pts',(-14.6847067803446,5.58780073668082,
129.20805193109));
#255454=CARTESIAN_POINT('Ctrl Pts',(-14.9631544041576,1.67732308005318,
125.240341766008));
#255455=CARTESIAN_POINT('Ctrl Pts',(-15.2416020279704,-3.77453254535539,
126.385693108075));
#255456=CARTESIAN_POINT('Ctrl Pts',(-15.5200496517834,-5.75777715774833,
131.591584027456));
#255457=CARTESIAN_POINT('Ctrl Pts',(-15.7984972755962,-2.44990584522241,
136.074055091149));
#255458=CARTESIAN_POINT('Ctrl Pts',(-16.0769448994091,3.1093092545088,135.713934372506));
#255459=CARTESIAN_POINT('Ctrl Pts',(-16.355392523222,5.81122104754806,130.842155219084));
#255460=CARTESIAN_POINT('Ctrl Pts',(-16.6338401470349,3.17290459182133,
125.935644673236));
#255461=CARTESIAN_POINT('Ctrl Pts',(-16.9122877708478,-2.38115617878252,
125.50324623023));
#255462=CARTESIAN_POINT('Ctrl Pts',(-17.1907353946607,-5.74705074703162,
129.94231293535));
#255463=CARTESIAN_POINT('Ctrl Pts',(-17.4691830184736,-3.83168643779603,
135.173559347056));
#255464=CARTESIAN_POINT('Ctrl Pts',(-17.7476306422864,1.6048105194851,136.389725573584));
#255465=CARTESIAN_POINT('Ctrl Pts',(-18.0260782660994,5.56656500871184,
132.473214265779));
#255466=CARTESIAN_POINT('Ctrl Pts',(-18.3045258899123,4.4129181967513,127.023107983299));
#255467=CARTESIAN_POINT('Ctrl Pts',(-18.5829735137251,-0.795984854984928,
125.047788147249));
#255468=CARTESIAN_POINT('Ctrl Pts',(-18.861421137538,-5.27341671101187,
128.362477187221));
#255469=CARTESIAN_POINT('Ctrl Pts',(-19.1398687613509,-4.90483623034722,
133.921137807042));
#255470=CARTESIAN_POINT('Ctrl Pts',(-19.4183163851638,-0.0289508685644962,
136.615632452765));
#255471=CARTESIAN_POINT('Ctrl Pts',(-19.6967640089767,4.87353892710056,
133.969852178351));
#255472=CARTESIAN_POINT('Ctrl Pts',(-19.9752116327896,5.29748453437273,
128.415139802436));
#255473=CARTESIAN_POINT('Ctrl Pts',(-20.2536592566025,0.853300651063172,
125.056004635698));
#255474=CARTESIAN_POINT('Ctrl Pts',(-20.5321068804154,-4.37502484451904,
126.979327793496));
#255475=CARTESIAN_POINT('Ctrl Pts',(-20.8105545042282,-5.58291623983416,
132.417669253371));
#255476=CARTESIAN_POINT('Ctrl Pts',(-21.0890021280412,-1.66038035136256,
136.37345889145));
#255477=CARTESIAN_POINT('Ctrl Pts',(-21.367449751854,3.78796396592178,135.211519281404));
#255478=CARTESIAN_POINT('Ctrl Pts',(-21.6458973756669,5.75535445085128,
129.999616160961));
#255479=CARTESIAN_POINT('Ctrl Pts',(-21.9243449994798,2.43385536014432,
125.527233882186));
#255480=CARTESIAN_POINT('Ctrl Pts',(-22.2027926232928,-3.12423790609075,
125.904273271251));
#255481=CARTESIAN_POINT('Ctrl Pts',(-22.4812402471056,-5.81130916413533,
130.784253549004));
#255482=CARTESIAN_POINT('Ctrl Pts',(-22.7596878709185,-3.15807119857507,
135.682711240481));
#255483=CARTESIAN_POINT('Ctrl Pts',(-23.0381354947314,2.39727991812053,
136.098203030175));
#255484=CARTESIAN_POINT('Ctrl Pts',(-23.3165831185443,5.74964790369824,
131.648912261261));
#255485=CARTESIAN_POINT('Ctrl Pts',(-23.5950307423572,3.81837035169266,
126.423519790431));
#255486=CARTESIAN_POINT('Ctrl Pts',(-23.8734783661701,-1.62180301575654,
125.223906023766));
#255487=CARTESIAN_POINT('Ctrl Pts',(-24.151925989983,-5.57161864120731,
129.15245740844));
#255488=CARTESIAN_POINT('Ctrl Pts',(-24.4303736137958,-4.4013889240913,
134.599027142342));
#255489=CARTESIAN_POINT('Ctrl Pts',(-24.7088212376087,0.813502194462058,
136.558483719739));
#255490=CARTESIAN_POINT('Ctrl Pts',(-24.9872688614217,5.28082453809644,
133.230182270781));
#255491=CARTESIAN_POINT('Ctrl Pts',(-25.2657164852345,4.89532711384086,
127.672669230493));
#255492=CARTESIAN_POINT('Ctrl Pts',(-25.5441641090475,0.0112632219902977,
124.993027583295));
#255493=CARTESIAN_POINT('Ctrl Pts',(-25.8226117328602,-4.88315102063038,
127.65371709519));
#255494=CARTESIAN_POINT('Ctrl Pts',(-26.1010593566733,-5.29018803048126,
133.209694086655));
#255495=CARTESIAN_POINT('Ctrl Pts',(-26.3795069804861,-0.835800680372761,
136.555287127099));
#255496=CARTESIAN_POINT('Ctrl Pts',(-26.6579546042989,4.38664666386508,
134.616059653661));
#255497=CARTESIAN_POINT('Ctrl Pts',(-26.9364022281119,5.57798002361419,
129.174066977901));
#255498=CARTESIAN_POINT('Ctrl Pts',(-27.2148498519247,1.64342224113504,
125.23023451272));
#255499=CARTESIAN_POINT('Ctrl Pts',(-27.4932974757377,-3.80136029530733,
126.408751626694));
#255500=CARTESIAN_POINT('Ctrl Pts',(-27.7717450995505,-5.75287842713667,
131.626618665841));
#255501=CARTESIAN_POINT('Ctrl Pts',(-28.0501927233634,-2.41778232816299,
136.088870728161));
#255502=CARTESIAN_POINT('Ctrl Pts',(-28.3286403471763,3.13913761515943,
135.694916161515));
#255503=CARTESIAN_POINT('Ctrl Pts',(-28.6070879709892,5.8113434455484,130.8067799669));
#255504=CARTESIAN_POINT('Ctrl Pts',(-28.8855355948021,3.14320854938853,
125.916420508438));
#255505=CARTESIAN_POINT('Ctrl Pts',(-29.163983218615,-2.41338144938502,
125.517839221114));
#255506=CARTESIAN_POINT('Ctrl Pts',(-29.4424308424279,-5.75219179641212,
129.977312836202));
#255507=CARTESIAN_POINT('Ctrl Pts',(-29.7208784662408,-3.80501889272807,
135.196802958832));
#255508=CARTESIAN_POINT('Ctrl Pts',(-29.9993260900537,1.6387804878663,136.379853152576));
#255509=CARTESIAN_POINT('Ctrl Pts',(-30.2777737138665,5.576620658989,132.439298084597));
#255510=CARTESIAN_POINT('Ctrl Pts',(-30.5562213376795,4.38981887756547,
126.996315355552));
#255511=CARTESIAN_POINT('Ctrl Pts',(-30.8346689614924,-0.831011997766135,
125.052740188944));
#255512=CARTESIAN_POINT('Ctrl Pts',(-31.1131165853052,-5.2881834443438,
128.394623213959));
#255513=CARTESIAN_POINT('Ctrl Pts',(-31.3915642091181,-4.88577264769286,
133.950937190672));
#255514=CARTESIAN_POINT('Ctrl Pts',(-31.670011832931,0.00642452892459172,
136.615701015511));
#255515=CARTESIAN_POINT('Ctrl Pts',(-31.9484594567439,4.89271787731614,
133.940126914399));
#255516=CARTESIAN_POINT('Ctrl Pts',(-32.2269070805568,5.28284251901049,
128.382936777197));
#255517=CARTESIAN_POINT('Ctrl Pts',(-32.5053547043697,0.818292966938792,
125.050916856162));
#255518=CARTESIAN_POINT('Ctrl Pts',(-32.7838023281826,-4.3982278459157,
127.006030680504));
#255519=CARTESIAN_POINT('Ctrl Pts',(-33.0622499519955,-5.57299213374921,
132.451624158271));
#255520=CARTESIAN_POINT('Ctrl Pts',(-33.3406975758084,-1.62644890646854,
136.383462915428));
#255521=CARTESIAN_POINT('Ctrl Pts',(-33.6191451996212,3.81472140941051,
135.188379215148));
#255522=CARTESIAN_POINT('Ctrl Pts',(-33.8975928234342,5.75034910954236,
129.964596594906));
#255523=CARTESIAN_POINT('Ctrl Pts',(-34.176040447247,2.40168689817613,125.512516086734));
#255524=CARTESIAN_POINT('Ctrl Pts',(-34.4544880710599,-3.15400824368619,
125.923382181419));
#255525=CARTESIAN_POINT('Ctrl Pts',(-34.7329356948729,-5.81132389146964,
130.81962900987));
#255526=CARTESIAN_POINT('Ctrl Pts',(-35.0113833186857,-3.1283167819475,
135.701844931696));
#255527=CARTESIAN_POINT('Ctrl Pts',(-35.2898309424986,2.42946062341331,
136.083512024245));
#255528=CARTESIAN_POINT('Ctrl Pts',(-35.5682785663115,5.75468240160701,
131.613896874941));
#255529=CARTESIAN_POINT('Ctrl Pts',(-35.8467261901244,3.79163218458816,
126.400357453152));
#255530=CARTESIAN_POINT('Ctrl Pts',(-36.1251738139373,-1.65574277853735,
125.233881791944));
#255531=CARTESIAN_POINT('Ctrl Pts',(-36.4036214377501,-5.58157101571846,
129.186404038463));
#255532=CARTESIAN_POINT('Ctrl Pts',(-36.6820690615631,-4.37820816435757,
134.625749339604));
#255533=CARTESIAN_POINT('Ctrl Pts',(-36.960516685376,0.848514102688449,
136.553425090409));
#255534=CARTESIAN_POINT('Ctrl Pts',(-37.2389643091888,5.29549336158222,
133.197991448084));
#255535=CARTESIAN_POINT('Ctrl Pts',(-37.5174119330018,4.87617292041449,
127.64292800788));
#255536=CARTESIAN_POINT('Ctrl Pts',(-37.7958595568146,-0.0241122203237842,
124.993066691407));
#255537=CARTESIAN_POINT('Ctrl Pts',(-38.0743071806275,-4.90223940853195,
127.683500595584));
#255538=CARTESIAN_POINT('Ctrl Pts',(-38.3527548044404,-5.27544806800837,
133.241852397473));
#255539=CARTESIAN_POINT('Ctrl Pts',(-38.6312024282533,-0.800777672950798,
136.560268331721));
#255540=CARTESIAN_POINT('Ctrl Pts',(-38.9096500520661,4.40976828338437,
134.589286268384));
#255541=CARTESIAN_POINT('Ctrl Pts',(-39.1880976758791,5.56795261644649,
129.140142435842));
#255542=CARTESIAN_POINT('Ctrl Pts',(-39.4665452996919,1.6094605046014,125.220333810727));
#255543=CARTESIAN_POINT('Ctrl Pts',(-39.7449929235049,-3.82804718445556,
126.43197302622));
#255544=CARTESIAN_POINT('Ctrl Pts',(-40.0234405473177,-5.74776652149929,
131.661622835152));
#255545=CARTESIAN_POINT('Ctrl Pts',(-40.3018881711306,-2.38556921929025,
136.103490545709));
#255546=CARTESIAN_POINT('Ctrl Pts',(-40.5803357949436,3.16884965391132,
135.675716729192));
#255547=CARTESIAN_POINT('Ctrl Pts',(-40.8587834187564,5.81125050208024,
130.771404625066));
#255548=CARTESIAN_POINT('Ctrl Pts',(-41.1372310425694,3.11339603420704,
125.897377468058));
#255549=CARTESIAN_POINT('Ctrl Pts',(-41.4156786663821,-2.4455172912504,
125.532628105994));
#255550=CARTESIAN_POINT('Ctrl Pts',(-41.6941262901951,-5.75711969621025,
130.012343383614));
#255551=CARTESIAN_POINT('Ctrl Pts',(-41.9725739140079,-3.77821035128576,
135.219883807042));
#255552=CARTESIAN_POINT('Ctrl Pts',(-42.2510215378209,1.67268973063362,
136.369774129642));
#255553=CARTESIAN_POINT('Ctrl Pts',(-42.5294691616338,5.58646966553678,
132.405321320208));
#255554=CARTESIAN_POINT('Ctrl Pts',(-42.8079167854466,4.366556892027,126.969663836325));
#255555=CARTESIAN_POINT('Ctrl Pts',(-43.0863644092596,-0.866008347092154,
125.057905359049));
#255556=CARTESIAN_POINT('Ctrl Pts',(-43.3648120330724,-5.3027542220935,
128.426858534403));
#255557=CARTESIAN_POINT('Ctrl Pts',(-43.6432596568854,-4.86652802093628,
133.98061997675));
#255558=CARTESIAN_POINT('Ctrl Pts',(-43.9217072806982,0.0417996883503892,
136.615554236903));
#255559=CARTESIAN_POINT('Ctrl Pts',(-44.2001549045111,4.9117155260715,133.910285453475));
#255560=CARTESIAN_POINT('Ctrl Pts',(-44.478602528324,5.26800474597596,128.350823478709));
#255561=CARTESIAN_POINT('Ctrl Pts',(-44.7570501521369,0.783254960667603,
125.046042272601));
#255562=CARTESIAN_POINT('Ctrl Pts',(-45.0354977759497,-4.42126786936209,
127.032874316024));
#255563=CARTESIAN_POINT('Ctrl Pts',(-45.3139453997627,-5.56286151839129,
132.485518023215));
#255564=CARTESIAN_POINT('Ctrl Pts',(-45.5923930235756,-1.59245719291215,
136.393260203719));
#255565=CARTESIAN_POINT('Ctrl Pts',(-45.8708406473885,3.84133749699455,
135.165076697471));
#255566=CARTESIAN_POINT('Ctrl Pts',(-46.1492882712014,5.74513068693249,
129.929608146614));
#255567=CARTESIAN_POINT('Ctrl Pts',(-46.4277358950142,2.3694294408167,125.497994382526));
#255568=CARTESIAN_POINT('Ctrl Pts',(-46.7061835188271,-3.18366170834627,
125.942671958037));
#255569=CARTESIAN_POINT('Ctrl Pts',(-46.98463114264,-5.81112327806003,130.85500390496));
#255570=CARTESIAN_POINT('Ctrl Pts',(-47.263078766453,-3.09844644439114,
135.720797144829));
#255571=CARTESIAN_POINT('Ctrl Pts',(-47.5415263902657,2.46155130414924,
136.068625397419));
#255572=CARTESIAN_POINT('Ctrl Pts',(-47.8199740140787,5.75950365764311,
131.578851490957));
#255573=CARTESIAN_POINT('Ctrl Pts',(-48.0984216378915,3.76475351715869,
126.377358307829));
#255574=CARTESIAN_POINT('Ctrl Pts',(-48.3768692617045,-1.6896211871606,
125.244063976264));
#255575=CARTESIAN_POINT('Ctrl Pts',(-48.6553168855173,-5.59131656306301,
129.220410622463));
#255576=CARTESIAN_POINT('Ctrl Pts',(-48.9337645093303,-4.35486516851022,
134.652329933902));
#255577=CARTESIAN_POINT('Ctrl Pts',(-49.2122121331431,0.883494568912716,
136.548153427379));
#255578=CARTESIAN_POINT('Ctrl Pts',(-49.4906597569561,5.3099659586141,133.165711928516));
#255579=CARTESIAN_POINT('Ctrl Pts',(-49.7691073807689,4.85683803860733,
127.613303933314));
#255580=CARTESIAN_POINT('Ctrl Pts',(-50.0475550045819,-0.0594867691506708,
124.993321139153));
#255581=CARTESIAN_POINT('Ctrl Pts',(-50.3260026283946,-4.92114614214944,
127.713399740592));
#255582=CARTESIAN_POINT('Ctrl Pts',(-50.6044502522077,-5.26051262186729,
133.273920386136));
#255583=CARTESIAN_POINT('Ctrl Pts',(-50.8828978760204,-0.765724992417492,
136.565036249065));
#255584=CARTESIAN_POINT('Ctrl Pts',(-51.1613454998334,4.4327264973184,134.562372631296));
#255585=CARTESIAN_POINT('Ctrl Pts',(-51.4397931236463,5.55771888674681,
129.106279562002));
#255586=CARTESIAN_POINT('Ctrl Pts',(-51.7182407474591,1.57543912891688,
125.210640026899));
#255587=CARTESIAN_POINT('Ctrl Pts',(-51.9966883712721,-3.85459222390762,
126.455356446176));
#255588=CARTESIAN_POINT('Ctrl Pts',(-52.2751359950849,-5.7424416302597,
131.696595238295));
#255589=CARTESIAN_POINT('Ctrl Pts',(-52.5535836188979,-2.35326771227282,
136.117914002047));
#255590=CARTESIAN_POINT('Ctrl Pts',(-52.8320312427106,3.19844426977395,
135.656336786975));
#255591=CARTESIAN_POINT('Ctrl Pts',(-53.1104788665238,5.81094222058764,
130.736030504428));
#255592=CARTESIAN_POINT('Ctrl Pts',(-53.3889264903363,3.08346815099054,
125.878516257743));
#255593=CARTESIAN_POINT('Ctrl Pts',(-53.6673741141495,-2.47756251357323,
125.547612336859));
#255594=CARTESIAN_POINT('Ctrl Pts',(-53.9458217379622,-5.76183426382087,
130.047403279515));
#255595=CARTESIAN_POINT('Ctrl Pts',(-54.2242693617753,-3.75126180686946,
135.242801036416));
#255596=CARTESIAN_POINT('Ctrl Pts',(-54.502716985588,1.70653699126786,136.359488878264));
#255597=CARTESIAN_POINT('Ctrl Pts',(-54.7811646094011,5.59611166339667,
132.371285231631));
#255598=CARTESIAN_POINT('Ctrl Pts',(-55.0596122332138,4.3431331021171,126.943154413196));
#255599=CARTESIAN_POINT('Ctrl Pts',(-55.3380598570268,-0.900972606160421,
125.063283466166));
#255600=CARTESIAN_POINT('Ctrl Pts',(-55.6165074808396,-5.31712850433539,
128.459181954061));
#255601=CARTESIAN_POINT('Ctrl Pts',(-55.8949551046525,-4.84710306319425,
134.01018506537));
#255602=CARTESIAN_POINT('Ctrl Pts',(-56.1734027284654,0.0771732988733811,
136.615192122377));
#255603=CARTESIAN_POINT('Ctrl Pts',(-56.4518503522783,4.93053116940174,
133.880328901363));
#255604=CARTESIAN_POINT('Ctrl Pts',(-56.7302979760911,5.25297176508825,
128.318801096944));
#255605=CARTESIAN_POINT('Ctrl Pts',(-57.0087455999042,0.748187930595796,
125.041381065643));
#255606=CARTESIAN_POINT('Ctrl Pts',(-57.2871932237169,-4.44414406110167,
127.059857705357));
#255607=CARTESIAN_POINT('Ctrl Pts',(-57.5656408475299,-5.55252476915405,
132.519349592253));
#255608=CARTESIAN_POINT('Ctrl Pts',(-57.8440884713427,-1.55840647026886,
136.402850393281));
#255609=CARTESIAN_POINT('Ctrl Pts',(-58.1225360951557,3.867811242405,135.141612591857));
#255610=CARTESIAN_POINT('Ctrl Pts',(-58.4009837189685,5.73969937639226,
129.894652112598));
#255611=CARTESIAN_POINT('Ctrl Pts',(-58.6794313427815,2.33708418337799,
125.483669307672));
#255612=CARTESIAN_POINT('Ctrl Pts',(-58.9578789665944,-3.21319720125095,
125.962141886319));
#255613=CARTESIAN_POINT('Ctrl Pts',(-59.2363265904072,-5.81070733134035,
130.890376923444));
#255614=CARTESIAN_POINT('Ctrl Pts',(-59.5147742142201,-3.06846129276222,
135.739567177598));
#255615=CARTESIAN_POINT('Ctrl Pts',(-59.793221838033,2.49355077119662,136.053543701326));
#255616=CARTESIAN_POINT('Ctrl Pts',(-60.071669461846,5.76411149315304,131.543777407928));
#255617=CARTESIAN_POINT('Ctrl Pts',(-60.3501170856587,3.73773534540316,
126.354523206705));
#255618=CARTESIAN_POINT('Ctrl Pts',(-60.6285647094717,-1.72343698624942,
125.254452199421));
#255619=CARTESIAN_POINT('Ctrl Pts',(-60.9070123332846,-5.6008549221161,
129.254475900312));
#255620=CARTESIAN_POINT('Ctrl Pts',(-61.1854599570975,-4.33136080153256,
134.678767940282));
#255621=CARTESIAN_POINT('Ctrl Pts',(-61.4639075809103,0.918442296920838,
136.542668925995));
#255622=CARTESIAN_POINT('Ctrl Pts',(-61.7423552047232,5.32424179290464,
133.133344908207));
#255623=CARTESIAN_POINT('Ctrl Pts',(-62.0208028285362,4.83732318488056,
127.583798104527));
#255624=CARTESIAN_POINT('Ctrl Pts',(-62.299250452349,-0.0948591136734494,
124.993790917104));
#255625=CARTESIAN_POINT('Ctrl Pts',(-62.5776980761619,-4.93987052088691,
127.743413422294));
#255626=CARTESIAN_POINT('Ctrl Pts',(-62.8561456999749,-5.24538224549645,
133.305896864355));
#255627=CARTESIAN_POINT('Ctrl Pts',(-63.1345933237877,-0.730643937663188,
136.569590702456));
#255628=CARTESIAN_POINT('Ctrl Pts',(-63.4130409476006,4.45552045494177,
134.53531973969));
#255629=CARTESIAN_POINT('Ctrl Pts',(-63.6914885714135,5.5472792137301,129.072479611178));
#255630=CARTESIAN_POINT('Ctrl Pts',(-63.9699361952264,1.54135937475606,
125.201153520444));
#255631=CARTESIAN_POINT('Ctrl Pts',(-64.2483838190392,-3.88099443002729,
126.478901020081));
#255632=CARTESIAN_POINT('Ctrl Pts',(-64.5268314428522,-5.73690395073373,
131.731534579357));
#255633=CARTESIAN_POINT('Ctrl Pts',(-64.805279066665,-2.32087900405488,
136.132140562712));
#255634=CARTESIAN_POINT('Ctrl Pts',(-65.083726690478,3.22792036610792,135.636777052998));
#255635=CARTESIAN_POINT('Ctrl Pts',(-65.3621743142908,5.81041861249411,
130.700658915789));
#255636=CARTESIAN_POINT('Ctrl Pts',(-65.6406219381037,3.05342600872776,
125.859837576403));
#255637=CARTESIAN_POINT('Ctrl Pts',(-65.9190695619166,-2.50951592890599,
125.562791358466));
#255638=CARTESIAN_POINT('Ctrl Pts',(-66.1975171857295,-5.76633532454392,
130.082491224748));
#255639=CARTESIAN_POINT('Ctrl Pts',(-66.4759648095424,-3.72417425806736,
135.26555379775));
#255640=CARTESIAN_POINT('Ctrl Pts',(-66.7544124333553,1.74032101554631,
136.348997779564));
#255641=CARTESIAN_POINT('Ctrl Pts',(-67.0328600571681,5.60554629528092,
132.337191080086));
#255642=CARTESIAN_POINT('Ctrl Pts',(-67.3113076809811,4.31954837581292,
126.916788068483));
#255643=CARTESIAN_POINT('Ctrl Pts',(-67.5897553047939,-0.935903479357421,
125.068874311009));
#255644=CARTESIAN_POINT('Ctrl Pts',(-67.8682029286069,-5.33130575842519,
128.491592275178));
#255645=CARTESIAN_POINT('Ctrl Pts',(-68.1466505524197,-4.82749849426569,
134.039631360986));
#255646=CARTESIAN_POINT('Ctrl Pts',(-68.4250981762326,0.112544049711387,
136.614614685353));
#255647=CARTESIAN_POINT('Ctrl Pts',(-68.7035458000455,4.94916411008632,
133.850258368115));
#255648=CARTESIAN_POINT('Ctrl Pts',(-68.9819934238584,5.23774413340002,
128.286870818499));
#255649=CARTESIAN_POINT('Ctrl Pts',(-69.2604410476712,0.713093176145084,
125.036933408012));
#255650=CARTESIAN_POINT('Ctrl Pts',(-69.5388886714842,-4.46685557344872,
127.086979848621));
#255651=CARTESIAN_POINT('Ctrl Pts',(-69.8173362952971,-5.54198226906957,
132.553117611744));
#255652=CARTESIAN_POINT('Ctrl Pts',(-70.09578391911,-1.52429800030071,136.412233128746));
#255653=CARTESIAN_POINT('Ctrl Pts',(-70.3742315429229,3.89414166464747,
135.117987767775));
#255654=CARTESIAN_POINT('Ctrl Pts',(-70.6526791667357,5.73405537918087,
129.859729788164));
#255655=CARTESIAN_POINT('Ctrl Pts',(-70.9311267905487,2.3046523244254,125.469541392991));
#255656=CARTESIAN_POINT('Ctrl Pts',(-71.2095744143614,-3.24261362795168,
125.981791244794));
#255657=CARTESIAN_POINT('Ctrl Pts',(-71.4880220381746,-5.81007606672361,
130.925746754563));
#255658=CARTESIAN_POINT('Ctrl Pts',(-71.7664696619872,-3.03836243817177,
135.758154334473));
#255659=CARTESIAN_POINT('Ctrl Pts',(-72.0449172858002,2.52545783880292,
136.038267494822));
#255660=CARTESIAN_POINT('Ctrl Pts',(-72.3233649096131,5.76850573739207,
131.508675925537));
#255661=CARTESIAN_POINT('Ctrl Pts',(-72.601812533426,3.71057867048956,126.331852995942));
#255662=CARTESIAN_POINT('Ctrl Pts',(-72.8802601572389,-1.75718892274731,
125.265046076474));
#255663=CARTESIAN_POINT('Ctrl Pts',(-73.1587077810518,-5.61018573943046,
129.28859860971));
#255664=CARTESIAN_POINT('Ctrl Pts',(-73.4371554048648,-4.30769593438731,
134.705062379074));
#255665=CARTESIAN_POINT('Ctrl Pts',(-73.7156030286775,0.953355991712339,
136.536971789486));
#255666=CARTESIAN_POINT('Ctrl Pts',(-73.9940506524905,5.33832033545752,
133.100891586529));
#255667=CARTESIAN_POINT('Ctrl Pts',(-74.2724982763033,4.81762908236426,
127.554411614868));
#255668=CARTESIAN_POINT('Ctrl Pts',(-74.5509459001162,-0.130227943157576,
124.994476007852));
#255669=CARTESIAN_POINT('Ctrl Pts',(-74.8293935239292,-4.95841185090586,
127.77354052852));
#255670=CARTESIAN_POINT('Ctrl Pts',(-75.107841147742,-5.23005749955717,
133.337780647228));
#255671=CARTESIAN_POINT('Ctrl Pts',(-75.3862887715549,-0.695535808628632,
136.573931523126));
#255672=CARTESIAN_POINT('Ctrl Pts',(-75.6647363953679,4.4781493116164,134.508128596022));
#255673=CARTESIAN_POINT('Ctrl Pts',(-75.9431840191806,5.53663398424198,
129.038743835842));
#255674=CARTESIAN_POINT('Ctrl Pts',(-76.2216316429937,1.50722250495638,
125.191874642891));
#255675=CARTESIAN_POINT('Ctrl Pts',(-76.5000792668064,-3.90725282447187,
126.502605875483));
#255676=CARTESIAN_POINT('Ctrl Pts',(-76.7785268906195,-5.73115368812196,
131.766439563647));
#255677=CARTESIAN_POINT('Ctrl Pts',(-77.0569745144322,-2.28840429481114,
136.146169700531));
#255678=CARTESIAN_POINT('Ctrl Pts',(-77.3354221382452,3.25727685066645,
135.617038252052));
#255679=CARTESIAN_POINT('Ctrl Pts',(-77.613869762058,5.80967969720196,130.665291169852));
#255680=CARTESIAN_POINT('Ctrl Pts',(-77.8923173858709,3.0232707206408,125.841342116181));
#255681=CARTESIAN_POINT('Ctrl Pts',(-78.1707650096839,-2.54137635320382,
125.57816460835));
#255682=CARTESIAN_POINT('Ctrl Pts',(-78.4492126334967,-5.77062271159095,
130.117605919119));
#255683=CARTESIAN_POINT('Ctrl Pts',(-78.7276602573096,-3.69694870861804,
135.288141247929));
#255684=CARTESIAN_POINT('Ctrl Pts',(-79.0061078811224,1.77404055158998,
136.338301222296));
#255685=CARTESIAN_POINT('Ctrl Pts',(-79.2845555049354,5.61477321158579,
132.303040128944));
#255686=CARTESIAN_POINT('Ctrl Pts',(-79.5630031287483,4.29580358705489,
126.8905657792));
#255687=CARTESIAN_POINT('Ctrl Pts',(-79.8414507525611,-0.970799672307275,
125.074677686406));
#255688=CARTESIAN_POINT('Ctrl Pts',(-80.1198983763742,-5.34528545901998,
128.524088296775));
#255689=CARTESIAN_POINT('Ctrl Pts',(-80.3983460001869,-4.80771504060458,
134.068957772455));
#255690=CARTESIAN_POINT('Ctrl Pts',(-80.6767936239998,0.147910630189091,
136.613821947228));
#255691=CARTESIAN_POINT('Ctrl Pts',(-80.9552412478128,4.96761365767528,
133.820074968005));
#255692=CARTESIAN_POINT('Ctrl Pts',(-81.2336888716256,5.22232241517632,
128.255033826564));
#255693=CARTESIAN_POINT('Ctrl Pts',(-81.5121364954386,0.6779719977639,125.032699464516));
#255694=CARTESIAN_POINT('Ctrl Pts',(-81.7905841192513,-4.48940156482041,
127.114239740797));
#255695=CARTESIAN_POINT('Ctrl Pts',(-82.0690317430644,-5.53123440879372,
132.586820830401));
#255696=CARTESIAN_POINT('Ctrl Pts',(-82.3474793668772,-1.490133046909,136.421408062431));
#255697=CARTESIAN_POINT('Ctrl Pts',(-82.62592699069,3.92032778803891,135.094203100652));
#255698=CARTESIAN_POINT('Ctrl Pts',(-82.9043746145031,5.72819890443852,
129.824842467372));
#255699=CARTESIAN_POINT('Ctrl Pts',(-83.1828222383158,2.27213506573304,
125.455611161998));
#255700=CARTESIAN_POINT('Ctrl Pts',(-83.4612698621288,-3.27190989841242,
126.001619305352));
#255701=CARTESIAN_POINT('Ctrl Pts',(-83.7397174859417,-5.80922950760163,
130.961112087674));
#255702=CARTESIAN_POINT('Ctrl Pts',(-84.0181651097544,-3.00815099594316,
135.776557926701));
#255703=CARTESIAN_POINT('Ctrl Pts',(-84.2966127335676,2.55727132464077,
136.022797343974));
#255704=CARTESIAN_POINT('Ctrl Pts',(-84.5750603573801,5.77268622752965,
131.473548344486));
#255705=CARTESIAN_POINT('Ctrl Pts',(-84.8535079811934,3.68328449871872,
126.309348515594));
#255706=CARTESIAN_POINT('Ctrl Pts',(-85.131955605006,-1.79087574596318,
125.275845214866));
#255707=CARTESIAN_POINT('Ctrl Pts',(-85.4104032288191,-5.61930866924928,
129.322777486226));
#255708=CARTESIAN_POINT('Ctrl Pts',(-85.6888508526319,-4.28387144398495,
134.731212275928));
#255709=CARTESIAN_POINT('Ctrl Pts',(-85.9672984764448,0.98823435954663,
136.531062228962));
#255710=CARTESIAN_POINT('Ctrl Pts',(-86.2457461002577,5.35220106458756,
133.068353166051));
#255711=CARTESIAN_POINT('Ctrl Pts',(-86.5241937240705,4.79775646083024,
127.525145553266));
#255712=CARTESIAN_POINT('Ctrl Pts',(-86.8026413478836,-0.165591946996939,
124.995376386011));
#255713=CARTESIAN_POINT('Ctrl Pts',(-87.0810889716963,-4.97676944515001,
127.803779942897));
#255714=CARTESIAN_POINT('Ctrl Pts',(-87.3595365955093,-5.21453895191432,
133.36957055329));
#255715=CARTESIAN_POINT('Ctrl Pts',(-87.6379842193221,-0.660401906259044,
136.578058550223));
#255716=CARTESIAN_POINT('Ctrl Pts',(-87.916431843135,4.50061222882128,134.480800207869));
#255717=CARTESIAN_POINT('Ctrl Pts',(-88.1948794669479,5.52578359274576,
129.005073486085));
#255718=CARTESIAN_POINT('Ctrl Pts',(-88.4733270907608,1.47302978447255,
125.182803738068));
#255719=CARTESIAN_POINT('Ctrl Pts',(-88.7517747145737,-3.93336643422502,
126.526470133988));
#255720=CARTESIAN_POINT('Ctrl Pts',(-89.0302223383866,-5.7251910555031,
131.801308897747));
#255721=CARTESIAN_POINT('Ctrl Pts',(-89.3086699621995,-2.25584478790559,
136.16000089565));
#255722=CARTESIAN_POINT('Ctrl Pts',(-89.5871175860123,3.28651263563227,
135.597121115567));
#255723=CARTESIAN_POINT('Ctrl Pts',(-89.8655652098253,5.80872550209253,
130.629928577187));
#255724=CARTESIAN_POINT('Ctrl Pts',(-90.1440128336381,2.99300340414587,
125.823030562435));
#255725=CARTESIAN_POINT('Ctrl Pts',(-90.4224604574511,-2.57314260586573,
125.593731516848));
#255726=CARTESIAN_POINT('Ctrl Pts',(-90.7009080812639,-5.77469626609129,
130.152746061436));
#255727=CARTESIAN_POINT('Ctrl Pts',(-90.9793557050769,-3.66958616737523,
135.310562549967));
#255728=CARTESIAN_POINT('Ctrl Pts',(-91.2578033288896,1.80769434990835,
136.327399602824));
#255729=CARTESIAN_POINT('Ctrl Pts',(-91.5362509527026,5.62379207040447,
132.268833643682));
#255730=CARTESIAN_POINT('Ctrl Pts',(-91.8146985765155,4.27189961571542,
126.864488517025));
#255731=CARTESIAN_POINT('Ctrl Pts',(-92.0931462003284,-1.00565989191805,
125.080693377311));
#255732=CARTESIAN_POINT('Ctrl Pts',(-92.3715938241412,-5.3590670880956,
128.556668814702));
#255733=CARTESIAN_POINT('Ctrl Pts',(-92.6500414479542,-4.78775343529548,
134.098163213075));
#255734=CARTESIAN_POINT('Ctrl Pts',(-92.928489071767,0.183271729783054,
136.612813937377));
#255735=CARTESIAN_POINT('Ctrl Pts',(-93.2069366955801,4.98587912851244,
133.789779819492));
#255736=CARTESIAN_POINT('Ctrl Pts',(-93.4853843193926,5.2067071818758,128.223291300872));
#255737=CARTESIAN_POINT('Ctrl Pts',(-93.7638319432059,0.642825696881324,
125.028679392048));
#255738=CARTESIAN_POINT('Ctrl Pts',(-94.0422795670186,-4.51178119976554,
127.14163637176));
#255739=CARTESIAN_POINT('Ctrl Pts',(-94.3207271908314,-5.52028158659305,
132.62045799934));
#255740=CARTESIAN_POINT('Ctrl Pts',(-94.5991748146444,-1.45591287608963,
136.430374854359));
#255741=CARTESIAN_POINT('Ctrl Pts',(-94.8776224384574,3.94636864224209,
135.07025947184));
#255742=CARTESIAN_POINT('Ctrl Pts',(-95.1560700622702,5.7221301691794,129.789991442987));
#255743=CARTESIAN_POINT('Ctrl Pts',(-95.4345176860831,2.23953361224044,
125.441879130882));
#255744=CARTESIAN_POINT('Ctrl Pts',(-95.7129653098959,-3.30108492704829,
126.021625333256));
#255745=CARTESIAN_POINT('Ctrl Pts',(-95.9914129337089,-5.80816768534362,
130.996471612301));
#255746=CARTESIAN_POINT('Ctrl Pts',(-96.2698605575217,-2.97782808557417,
135.794777272329));
#255747=CARTESIAN_POINT('Ctrl Pts',(-96.5483081813347,2.58899004984866,
136.007133822036));
#255748=CARTESIAN_POINT('Ctrl Pts',(-96.8267558051475,5.77665280865574,
131.438395966436));
#255749=CARTESIAN_POINT('Ctrl Pts',(-97.1052034289604,3.65585384148698,
126.287010599573));
#255750=CARTESIAN_POINT('Ctrl Pts',(-97.3836510527732,-1.82449620761995,
125.286849214428));
#255751=CARTESIAN_POINT('Ctrl Pts',(-97.6620986765863,-5.62822337351841,
129.35701126335));
#255752=CARTESIAN_POINT('Ctrl Pts',(-97.9405463003989,-4.25988821315111,
134.757216661848));
#255753=CARTESIAN_POINT('Ctrl Pts',(-98.2189939242121,1.02307610799351,
136.524940463405));
#255754=CARTESIAN_POINT('Ctrl Pts',(-98.4974415480248,5.36588346593846,
133.035730852497));
#255755=CARTESIAN_POINT('Ctrl Pts',(-98.7758891718378,4.77770605666655,
127.496001004183));
#255756=CARTESIAN_POINT('Ctrl Pts',(-99.0543367956506,-0.200949814765295,
124.996492018215));
#255757=CARTESIAN_POINT('Ctrl Pts',(-99.3327844194636,-4.99494262337204,
127.834130544897));
#255758=CARTESIAN_POINT('Ctrl Pts',(-99.6112320432764,-5.19882717761281,
133.401265404553));
#255759=CARTESIAN_POINT('Ctrl Pts',(-99.8896796670892,-0.625243532454567,
136.581971630822));
#255760=CARTESIAN_POINT('Ctrl Pts',(-100.168127290903,4.5229083741848,134.453335587896));
#255761=CARTESIAN_POINT('Ctrl Pts',(-100.446574914715,5.51472844130613,
128.971469809575));
#255762=CARTESIAN_POINT('Ctrl Pts',(-100.725022538528,1.43878248032906,
125.173941142103));
#255763=CARTESIAN_POINT('Ctrl Pts',(-101.003470162341,-3.95933429163924,
126.550492911299));
#255764=CARTESIAN_POINT('Ctrl Pts',(-101.281917786154,-5.71901627382367,
131.836141289563));
#255765=CARTESIAN_POINT('Ctrl Pts',(-101.560365409967,-2.22320168984167,
136.17363363555));
#255766=CARTESIAN_POINT('Ctrl Pts',(-101.83881303378,3.31562663766449,135.577026381578));
#255767=CARTESIAN_POINT('Ctrl Pts',(-102.117260657593,5.80755606252295,
130.594572448163));
#255768=CARTESIAN_POINT('Ctrl Pts',(-102.395708281405,2.96262518080941,
125.804903593708));
#255769=CARTESIAN_POINT('Ctrl Pts',(-102.674155905219,-2.60481350978186,
125.609491507123));
#255770=CARTESIAN_POINT('Ctrl Pts',(-102.952603529031,-5.77855583709781,
130.187910349571));
#255771=CARTESIAN_POINT('Ctrl Pts',(-103.231051152844,-3.64208764826766,
135.332816873036));
#255772=CARTESIAN_POINT('Ctrl Pts',(-103.509498776657,1.84128116344741,
136.316293325111));
#255773=CARTESIAN_POINT('Ctrl Pts',(-103.78794640047,5.63260253753978,132.234572891835));
#255774=CARTESIAN_POINT('Ctrl Pts',(-104.066394024283,4.24783734756473,
126.838557248259));
#255775=CARTESIAN_POINT('Ctrl Pts',(-104.344841648096,-1.04048284643121,
125.086921160811));
#255776=CARTESIAN_POINT('Ctrl Pts',(-104.623289271909,-5.3726501349701,
128.589332621676));
#255777=CARTESIAN_POINT('Ctrl Pts',(-104.901736895722,-4.76761441802147,
134.12724660063));
#255778=CARTESIAN_POINT('Ctrl Pts',(-105.180184519534,0.218626038175886,
136.611590693152));
#255779=CARTESIAN_POINT('Ctrl Pts',(-105.458632143348,5.00395984576562,
133.759374045173));
#255780=CARTESIAN_POINT('Ctrl Pts',(-105.73707976716,5.1908990121252,128.191644417652));
#255781=CARTESIAN_POINT('Ctrl Pts',(-106.015527390973,0.607655575856702,
125.024873339572));
#255782=CARTESIAN_POINT('Ctrl Pts',(-106.293975014786,-4.53399364899913,
127.169168726316));
#255783=CARTESIAN_POINT('Ctrl Pts',(-106.572422638599,-5.50912420832816,
132.654027872123));
#255784=CARTESIAN_POINT('Ctrl Pts',(-106.850870262412,-1.42163875588365,
136.43913317226));
#255785=CARTESIAN_POINT('Ctrl Pts',(-107.129317886225,3.97226326230387,
135.046157768576));
#255786=CARTESIAN_POINT('Ctrl Pts',(-107.407765510038,5.71584939828273,
129.755178006424));
#255787=CARTESIAN_POINT('Ctrl Pts',(-107.686213133851,2.20684917200607,
125.428345808491));
#255788=CARTESIAN_POINT('Ctrl Pts',(-107.964660757664,-3.3301376327682,
126.041808587174));
#255789=CARTESIAN_POINT('Ctrl Pts',(-108.243108381476,-5.80689063929651,
131.031824018185));
#255790=CARTESIAN_POINT('Ctrl Pts',(-108.521556005289,-2.94739483068967,
135.812811696231));
#255791=CARTESIAN_POINT('Ctrl Pts',(-108.800003629102,2.62061283907833,
135.991277509423));
#255792=CARTESIAN_POINT('Ctrl Pts',(-109.078451252915,5.7804053337882,131.403220093974));
#255793=CARTESIAN_POINT('Ctrl Pts',(-109.356898876728,3.62828771524594,
126.264840075618));
#255794=CARTESIAN_POINT('Ctrl Pts',(-109.635346500541,-1.85804906189805,
125.298057667405));
#255795=CARTESIAN_POINT('Ctrl Pts',(-109.913794124354,-5.636929521901,129.391298672536));
#255796=CARTESIAN_POINT('Ctrl Pts',(-110.192241748167,-4.2357471305931,
134.783074573235));
#255797=CARTESIAN_POINT('Ctrl Pts',(-110.470689371979,1.05787994597834,
136.518606719657));
#255798=CARTESIAN_POINT('Ctrl Pts',(-110.749136995792,5.37936703250445,
133.003025854698));
#255799=CARTESIAN_POINT('Ctrl Pts',(-111.027584619605,4.75747861284798,
127.466979047582));
#255800=CARTESIAN_POINT('Ctrl Pts',(-111.306032243418,-0.23630023626489,
124.997822863128));
#255801=CARTESIAN_POINT('Ctrl Pts',(-111.584479867231,-5.01293071215839,
127.864591209862));
#255802=CARTESIAN_POINT('Ctrl Pts',(-111.862927491044,-5.18292275885852,
133.432864026556));
#255803=CARTESIAN_POINT('Ctrl Pts',(-112.141375114857,-0.590061990020461,
136.585670619917));
#255804=CARTESIAN_POINT('Ctrl Pts',(-112.41982273867,4.54503692151536,134.425735753813));
#255805=CARTESIAN_POINT('Ctrl Pts',(-112.698270362483,5.50346893957634,
128.937934051507));
#255806=CARTESIAN_POINT('Ctrl Pts',(-112.976717986295,1.40448186157095,
125.165287183403));
#255807=CARTESIAN_POINT('Ctrl Pts',(-113.255165610108,-3.98515543446448,
126.574673317241));
#255808=CARTESIAN_POINT('Ctrl Pts',(-113.533613233921,-5.71262957189362,
131.870935448366));
#255809=CARTESIAN_POINT('Ctrl Pts',(-113.812060857734,-2.19047621022174,
136.187067415062));
#255810=CARTESIAN_POINT('Ctrl Pts',(-114.090508481547,3.34461777793161,
135.556754794705));
#255811=CARTESIAN_POINT('Ctrl Pts',(-114.36895610536,5.80617142182825,130.559224092919));
#255812=CARTESIAN_POINT('Ctrl Pts',(-114.647403729173,2.9321371763071,125.786961881698));
#255813=CARTESIAN_POINT('Ctrl Pts',(-114.925851352986,-2.63638789137572,
125.625443995184));
#255814=CARTESIAN_POINT('Ctrl Pts',(-115.204298976799,-5.78220128159277,
130.223097480497));
#255815=CARTESIAN_POINT('Ctrl Pts',(-115.482746600612,-3.61445417026275,
135.354903392492));
#255816=CARTESIAN_POINT('Ctrl Pts',(-115.761194224424,1.87479974763623,
136.304982800703));
#255817=CARTESIAN_POINT('Ctrl Pts',(-116.039641848237,5.64120428651674,
132.200259142944));
#255818=CARTESIAN_POINT('Ctrl Pts',(-116.31808947205,4.22361767423897,126.812772933795));
#255819=CARTESIAN_POINT('Ctrl Pts',(-116.596537095863,-1.07526724547036,
125.093360806132));
#255820=CARTESIAN_POINT('Ctrl Pts',(-116.874984719676,-5.38603409631742,
128.622078507325));
#255821=CARTESIAN_POINT('Ctrl Pts',(-117.153432343489,-4.7472987350426,
134.156206857421));
#255822=CARTESIAN_POINT('Ctrl Pts',(-117.431879967302,0.253972245300257,
136.610152259881));
#255823=CARTESIAN_POINT('Ctrl Pts',(-117.710327591115,5.02185513944583,
133.728858771743));
#255824=CARTESIAN_POINT('Ctrl Pts',(-117.988775214928,5.17489849170343,
128.160094349593));
#255825=CARTESIAN_POINT('Ctrl Pts',(-118.26722283874,0.572462937930709,
125.021281448121));
#255826=CARTESIAN_POINT('Ctrl Pts',(-118.545670462553,-4.55603808943068,
127.196835784245));
#255827=CARTESIAN_POINT('Ctrl Pts',(-118.824118086366,-5.49776268743969,
132.687529204804));
#255828=CARTESIAN_POINT('Ctrl Pts',(-119.102565710179,-1.38731195633035,
136.447682691592));
#255829=CARTESIAN_POINT('Ctrl Pts',(-119.381013333992,3.99801068868978,
135.021898883958));
#255830=CARTESIAN_POINT('Ctrl Pts',(-119.659460957805,5.70935682448427,
129.720403447709));
#255831=CARTESIAN_POINT('Ctrl Pts',(-119.937908581618,2.17408295616475,
125.415011696306));
#255832=CARTESIAN_POINT('Ctrl Pts',(-120.216356205431,-3.3590669390133,
126.062168319208));
#255833=CARTESIAN_POINT('Ctrl Pts',(-120.494803829244,-5.80539841678086,
131.067167995328));
#255834=CARTESIAN_POINT('Ctrl Pts',(-120.773251453056,-2.91685235900652,
135.830660530138));
#255835=CARTESIAN_POINT('Ctrl Pts',(-121.051699076869,2.65213852053535,
135.975228993696));
#255836=CARTESIAN_POINT('Ctrl Pts',(-121.330146700682,5.78394366387473,
131.368022030553));
#255837=CARTESIAN_POINT('Ctrl Pts',(-121.608594324495,3.60058714147007,
126.242837765265));
#255838=CARTESIAN_POINT('Ctrl Pts',(-121.887041948308,-1.89153306548558,
125.309470158462));
#255839=CARTESIAN_POINT('Ctrl Pts',(-122.165489572121,-5.64542679178685,
129.425638443252));
#255840=CARTESIAN_POINT('Ctrl Pts',(-122.443937195934,-4.21144909086733,
134.808785051914));
#255841=CARTESIAN_POINT('Ctrl Pts',(-122.722384819747,1.09264458383337,
136.512061232418));
#255842=CARTESIAN_POINT('Ctrl Pts',(-123.00083244356,5.39265126464657,132.97023938455));
#255843=CARTESIAN_POINT('Ctrl Pts',(-123.279280067372,4.73707487890982,
127.438080758883));
#255844=CARTESIAN_POINT('Ctrl Pts',(-123.557727691185,-0.27164190157181,
124.999368871432));
#255845=CARTESIAN_POINT('Ctrl Pts',(-123.836175314998,-5.03073304495359,
127.895160809065));
#255846=CARTESIAN_POINT('Ctrl Pts',(-124.114622938811,-5.16682628499523,
133.464365248398));
#255847=CARTESIAN_POINT('Ctrl Pts',(-124.393070562624,-0.554858582622917,
136.589155380447));
#255848=CARTESIAN_POINT('Ctrl Pts',(-124.671518186437,4.56699705083122,
134.398001728342));
#255849=CARTESIAN_POINT('Ctrl Pts',(-124.94996581025,5.49200550478084,128.904467454562));
#255850=CARTESIAN_POINT('Ctrl Pts',(-125.228413434063,1.37012919922165,
125.156842182641));
#255851=CARTESIAN_POINT('Ctrl Pts',(-125.506861057876,-4.0108289058903,
126.599010455801));
#255852=CARTESIAN_POINT('Ctrl Pts',(-125.785308681688,-5.70603118637341,
131.905690084846));
#255853=CARTESIAN_POINT('Ctrl Pts',(-126.063756305501,-2.1576695617001,
136.200301736396));
#255854=CARTESIAN_POINT('Ctrl Pts',(-126.342203929314,3.37348498215772,
135.536307106118));
#255855=CARTESIAN_POINT('Ctrl Pts',(-126.620651553127,5.8045716313158,130.523884821299));
#255856=CARTESIAN_POINT('Ctrl Pts',(-126.89909917694,2.90154052038371,125.769206091244));
#255857=CARTESIAN_POINT('Ctrl Pts',(-127.177546800753,-2.66786458064647,
125.641588389905));
#255858=CARTESIAN_POINT('Ctrl Pts',(-127.455994424566,-5.7856324644928,
130.258306150342));
#255859=CARTESIAN_POINT('Ctrl Pts',(-127.734442048379,-3.5866867573295,
135.376821289913));
#255860=CARTESIAN_POINT('Ctrl Pts',(-128.012889672192,1.90824886043053,
136.293468448719));
#255861=CARTESIAN_POINT('Ctrl Pts',(-128.291337296005,5.64959699859458,
132.16589366852));
#255862=CARTESIAN_POINT('Ctrl Pts',(-128.569784919818,4.19924149320669,
126.787136529081));
#255863=CARTESIAN_POINT('Ctrl Pts',(-128.84823254363,-1.11001180008614,
125.100012074652));
#255864=CARTESIAN_POINT('Ctrl Pts',(-129.126680167443,-5.39921847619124,
128.654905258242));
#255865=CARTESIAN_POINT('Ctrl Pts',(-129.405127791256,-4.72680713916258,
134.185042910317));
#255866=CARTESIAN_POINT('Ctrl Pts',(-129.683575415069,0.289309041389885,
136.608498690867));
#255867=CARTESIAN_POINT('Ctrl Pts',(-129.962023038882,5.03956434643776,
133.69823512996));
#255868=CARTESIAN_POINT('Ctrl Pts',(-130.240470662695,5.15870621351431,
128.128642265792));
#255869=CARTESIAN_POINT('Ctrl Pts',(-130.518918286508,0.537249087180579,
125.017903850796));
#255870=CARTESIAN_POINT('Ctrl Pts',(-130.79736591032,-4.57791370419536,
127.224636520332));
#255871=CARTESIAN_POINT('Ctrl Pts',(-131.075813534134,-5.4861974449331,
132.720960755981));
#255872=CARTESIAN_POINT('Ctrl Pts',(-131.354261157946,-1.35293374942274,
136.456023095549));
#255873=CARTESIAN_POINT('Ctrl Pts',(-131.632708781759,4.02360996731925,
134.99748371691));
#255874=CARTESIAN_POINT('Ctrl Pts',(-131.911156405572,5.7026526883694,129.685669055425));
#255875=CARTESIAN_POINT('Ctrl Pts',(-132.189604029385,2.1412361788793,125.401877288427));
#255876=CARTESIAN_POINT('Ctrl Pts',(-132.468051653198,-3.38787177379785,
126.082703774923));
#255877=CARTESIAN_POINT('Ctrl Pts',(-132.746499277011,-5.80369107309236,
131.102502234048));
#255878=CARTESIAN_POINT('Ctrl Pts',(-133.024946900823,-2.88620180228584,
135.848323112653));
#255879=CARTESIAN_POINT('Ctrl Pts',(-133.303394524637,2.68356592602436,
135.95898886954));
#255880=CARTESIAN_POINT('Ctrl Pts',(-133.581842148449,5.78726766780228,
131.332803080451));
#255881=CARTESIAN_POINT('Ctrl Pts',(-133.860289772262,3.57275314661281,
126.221004483821));
#255882=CARTESIAN_POINT('Ctrl Pts',(-134.138737396075,-1.92494697761906,
125.321086264707));
#255883=CARTESIAN_POINT('Ctrl Pts',(-134.417185019888,-5.65371486830715,
129.460029303025));
#255884=CARTESIAN_POINT('Ctrl Pts',(-134.695632643701,-4.1869949943469,
134.834347145171));
#255885=CARTESIAN_POINT('Ctrl Pts',(-134.974080267514,1.1273687333409,136.505304244234));
#255886=CARTESIAN_POINT('Ctrl Pts',(-135.252527891327,5.40573567011315,
132.937372656969));
#255887=CARTESIAN_POINT('Ctrl Pts',(-135.53097551514,4.71649561092,127.409307208922));
#255888=CARTESIAN_POINT('Ctrl Pts',(-135.809423138953,-0.306973501088704,
125.001129985841));
#255889=CARTESIAN_POINT('Ctrl Pts',(-136.087870762765,-5.04834896208586,
127.925838209736));
#255890=CARTESIAN_POINT('Ctrl Pts',(-136.366318386578,-5.15053835248403,
133.49576790279));
#255891=CARTESIAN_POINT('Ctrl Pts',(-136.644766010391,-0.519634614735935,
136.592425783278));
#255892=CARTESIAN_POINT('Ctrl Pts',(-136.923213634204,4.58878794839197,
134.37013453918));
#255893=CARTESIAN_POINT('Ctrl Pts',(-137.201661258017,5.48033856170195,
128.871071258858));
#255894=CARTESIAN_POINT('Ctrl Pts',(-137.48010888183,1.33572576623031,125.148606452753));
#255895=CARTESIAN_POINT('Ctrl Pts',(-137.758556505643,-4.03635375457527,
126.623503425159));
#255896=CARTESIAN_POINT('Ctrl Pts',(-138.037004129456,-5.69922136176977,
131.940403911158));
#255897=CARTESIAN_POINT('Ctrl Pts',(-138.315451753269,-2.12478295993955,
136.213336109146));
#255898=CARTESIAN_POINT('Ctrl Pts',(-138.593899377082,3.40222718065648,
135.515684073514));
#255899=CARTESIAN_POINT('Ctrl Pts',(-138.872347000894,5.80275675026745,
130.488555942812));
#255900=CARTESIAN_POINT('Ctrl Pts',(-139.150794624707,2.870836346809,125.751636880291));
#255901=CARTESIAN_POINT('Ctrl Pts',(-139.42924224852,-2.69924241121433,
125.65792409305));
#255902=CARTESIAN_POINT('Ctrl Pts',(-139.707689872333,-5.78884925865424,
130.293535054436));
#255903=CARTESIAN_POINT('Ctrl Pts',(-139.986137496146,-3.55878643839929,
135.398569753122));
#255904=CARTESIAN_POINT('Ctrl Pts',(-140.264585119959,1.94162726236197,
136.281750695826));
#255905=CARTESIAN_POINT('Ctrl Pts',(-140.543032743772,5.65778036277742,
132.131477741989));
#255906=CARTESIAN_POINT('Ctrl Pts',(-140.821480367585,4.17470970773734,
126.761648984083));
#255907=CARTESIAN_POINT('Ctrl Pts',(-141.099927991397,-1.14471522280625,
125.106874719905));
#255908=CARTESIAN_POINT('Ctrl Pts',(-141.37837561521,-5.41220278603824,
128.687811658017));
#255909=CARTESIAN_POINT('Ctrl Pts',(-141.656823239023,-4.70614038970644,
134.213753690789));
#255910=CARTESIAN_POINT('Ctrl Pts',(-141.935270862836,0.324635117026387,
136.60663004738));
#255911=CARTESIAN_POINT('Ctrl Pts',(-142.213718486649,5.05708681051884,
133.667504254592));
#255912=CARTESIAN_POINT('Ctrl Pts',(-142.492166110462,5.14232277757003,
128.097289331719));
#255913=CARTESIAN_POINT('Ctrl Pts',(-142.770613734275,0.502015328467386,
125.014740672754));
#255914=CARTESIAN_POINT('Ctrl Pts',(-143.049061358088,-4.59961968268416,
127.252569904414));
#255915=CARTESIAN_POINT('Ctrl Pts',(-143.327508981901,-5.4744289093626,
132.754321286837));
#255916=CARTESIAN_POINT('Ctrl Pts',(-143.605956605714,-1.31850540905707,
136.464154075075));
#255917=CARTESIAN_POINT('Ctrl Pts',(-143.884404229526,4.04906014960179,
134.972913172143));
#255918=CARTESIAN_POINT('Ctrl Pts',(-144.162851853339,5.69573723836169,
129.650976116669));
#255919=CARTESIAN_POINT('Ctrl Pts',(-144.441299477152,2.10831005730047,
125.388943071553));
#255920=CARTESIAN_POINT('Ctrl Pts',(-144.719747100965,-3.41655106974776,
126.103414193369));
#255921=CARTESIAN_POINT('Ctrl Pts',(-144.998194724778,-5.80176867149642,
131.13782542502));
#255922=CARTESIAN_POINT('Ctrl Pts',(-145.276642348591,-2.85544429629671,
135.865798789283));
#255923=CARTESIAN_POINT('Ctrl Pts',(-145.555089972404,2.71489389099137,
135.942557738738));
#255924=CARTESIAN_POINT('Ctrl Pts',(-145.833537596217,5.79037722239768,
131.29756454872));
#255925=CARTESIAN_POINT('Ctrl Pts',(-146.111985220029,3.54478676207412,
126.199341040322));
#255926=CARTESIAN_POINT('Ctrl Pts',(-146.390432843843,-1.95828956013508,
125.332905555698));
#255927=CARTESIAN_POINT('Ctrl Pts',(-146.668880467655,-5.66179344434354,
129.49446997749));
#255928=CARTESIAN_POINT('Ctrl Pts',(-146.947328091469,-4.16238574718705,
134.859759905796));
#255929=CARTESIAN_POINT('Ctrl Pts',(-147.225775715281,1.16205110778606,
136.498336005488));
#255930=CARTESIAN_POINT('Ctrl Pts',(-147.504223339094,5.41861976405632,
132.904426889841));
#255931=CARTESIAN_POINT('Ctrl Pts',(-147.782670962907,4.6957415714508,127.380659463914));
#255932=CARTESIAN_POINT('Ctrl Pts',(-148.06111858672,-0.342293725589094,
125.003106141093));
#255933=CARTESIAN_POINT('Ctrl Pts',(-148.339566210533,-5.06577781079073,
127.956622275114));
#255934=CARTESIAN_POINT('Ctrl Pts',(-148.618013834346,-5.1340595648799,
133.527070826096));
#255935=CARTESIAN_POINT('Ctrl Pts',(-148.896461458158,-0.48439139159784,
136.595481707227));
#255936=CARTESIAN_POINT('Ctrl Pts',(-149.174909081971,4.61040880672808,
134.342135218952));
#255937=CARTESIAN_POINT('Ctrl Pts',(-149.453356705784,5.4684685426618,128.837746701901));
#255938=CARTESIAN_POINT('Ctrl Pts',(-149.731804329597,1.30127283742975,
125.140580298914));
#255939=CARTESIAN_POINT('Ctrl Pts',(-150.01025195341,-4.06172903468827,
126.648151317718));
#255940=CARTESIAN_POINT('Ctrl Pts',(-150.288699577223,-5.69220035042211,
131.975075640969));
#255941=CARTESIAN_POINT('Ctrl Pts',(-150.567147201036,-2.09181762356486,
136.226170050321));
#255942=CARTESIAN_POINT('Ctrl Pts',(-150.845594824849,3.43084330837664,
135.494886461086));
#255943=CARTESIAN_POINT('Ctrl Pts',(-151.124042448661,5.80072684593324,
130.453238766583));
#255944=CARTESIAN_POINT('Ctrl Pts',(-151.402490072475,2.84002579333802,
125.734254899877));
#255945=CARTESIAN_POINT('Ctrl Pts',(-151.680937696287,-2.73052022036177,
125.674450499292));
#255946=CARTESIAN_POINT('Ctrl Pts',(-151.9593853201,-5.79185154487752,130.32878288736));
#255947=CARTESIAN_POINT('Ctrl Pts',(-152.237832943913,-3.53075424732904,
135.420147976222));
#255948=CARTESIAN_POINT('Ctrl Pts',(-152.516280567726,1.97493371658077,
136.269829976228));
#255949=CARTESIAN_POINT('Ctrl Pts',(-152.794728191539,5.66575407582884,
132.097012638644));
#255950=CARTESIAN_POINT('Ctrl Pts',(-153.073175815352,4.15002322686382,
126.736311243251));
#255951=CARTESIAN_POINT('Ctrl Pts',(-153.351623439165,-1.17937622768304,
125.113948487592));
#255952=CARTESIAN_POINT('Ctrl Pts',(-153.630071062978,-5.42498654472129,
128.720796487292));
#255953=CARTESIAN_POINT('Ctrl Pts',(-153.90851868679,-4.6852992524868,134.242338134946));
#255954=CARTESIAN_POINT('Ctrl Pts',(-154.186966310604,0.359949163189457,
136.604546398667));
#255955=CARTESIAN_POINT('Ctrl Pts',(-154.465413934416,5.0744218823891,133.636667284384));
#255956=CARTESIAN_POINT('Ctrl Pts',(-154.743861558229,5.12574879096345,
128.066036709167));
#255957=CARTESIAN_POINT('Ctrl Pts',(-155.022309182042,0.466762967392146,
125.011792031209));
#255958=CARTESIAN_POINT('Ctrl Pts',(-155.300756805855,-4.62115522057418,
127.280634901405));
#255959=CARTESIAN_POINT('Ctrl Pts',(-155.579204429668,-5.46245751681569,
132.787609561181));
#255960=CARTESIAN_POINT('Ctrl Pts',(-155.857652053481,-1.28402821098903,
136.472075328871));
#255961=CARTESIAN_POINT('Ctrl Pts',(-156.136099677293,4.07436029247137,
134.948188160129));
#255962=CARTESIAN_POINT('Ctrl Pts',(-156.414547301107,5.68861073071636,
129.616325916999));
#255963=CARTESIAN_POINT('Ctrl Pts',(-156.692994924919,2.07530581151645,
125.376209524969));
#255964=CARTESIAN_POINT('Ctrl Pts',(-156.971442548732,-3.44510376414151,
126.124298807112));
#255965=CARTESIAN_POINT('Ctrl Pts',(-157.249890172545,-5.79963128322921,
131.173136259331));
#255966=CARTESIAN_POINT('Ctrl Pts',(-157.528337796358,-2.82458098076833,
135.883086912459));
#255967=CARTESIAN_POINT('Ctrl Pts',(-157.806785420171,2.74612125456611,
135.925936210153));
#255968=CARTESIAN_POINT('Ctrl Pts',(-158.085233043984,5.79327221243612,
131.262307741136));
#255969=CARTESIAN_POINT('Ctrl Pts',(-158.363680667797,3.51668902415852,
126.177848237519));
#255970=CARTESIAN_POINT('Ctrl Pts',(-158.64212829161,-1.9915595775106,125.344927593469));
#255971=CARTESIAN_POINT('Ctrl Pts',(-158.920575915422,-5.66966222054205,
129.528959190434));
#255972=CARTESIAN_POINT('Ctrl Pts',(-159.199023539236,-4.13762226129274,
134.885022392109));
#255973=CARTESIAN_POINT('Ctrl Pts',(-159.477471163048,1.19669042199943,
136.491156774389));
#255974=CARTESIAN_POINT('Ctrl Pts',(-159.755918786861,5.43130306905165,
132.871403303985));
#255975=CARTESIAN_POINT('Ctrl Pts',(-160.034366410674,4.67481352955083,
127.352138585409));
#255976=CARTESIAN_POINT('Ctrl Pts',(-160.312814034487,-0.377601266270116,
125.005297263965));
#255977=CARTESIAN_POINT('Ctrl Pts',(-160.5912616583,-5.08301894523598,127.987511864483));
#255978=CARTESIAN_POINT('Ctrl Pts',(-160.869709282113,-5.1173905328107,
133.558272858373));
#255979=CARTESIAN_POINT('Ctrl Pts',(-161.148156905926,-0.449130219157962,
136.598323039052));
#255980=CARTESIAN_POINT('Ctrl Pts',(-161.426604529739,4.63185882466967,
134.314004805186));
#255981=CARTESIAN_POINT('Ctrl Pts',(-161.705052153551,5.45639588750942,
128.804495018547));
#255982=CARTESIAN_POINT('Ctrl Pts',(-161.983499777364,1.26677168948586,
125.13276401854));
#255983=CARTESIAN_POINT('Ctrl Pts',(-162.261947401177,-4.08695380593746,
126.67295322014));
#255984=CARTESIAN_POINT('Ctrl Pts',(-162.54039502499,-5.68496841249774,
132.009703989503));
#255985=CARTESIAN_POINT('Ctrl Pts',(-162.818842648803,-2.05877477411906,
136.238803084352));
#255986=CARTESIAN_POINT('Ctrl Pts',(-163.097290272616,3.45933230493559,
135.473915039499));
#255987=CARTESIAN_POINT('Ctrl Pts',(-163.375737896429,5.79848199353304,
130.417934601304));
#255988=CARTESIAN_POINT('Ctrl Pts',(-163.654185520242,2.80911000166655,
125.717060794092));
#255989=CARTESIAN_POINT('Ctrl Pts',(-163.932633144055,-2.76169684907854,
125.691166996241));
#255990=CARTESIAN_POINT('Ctrl Pts',(-164.211080767867,-5.79463921191188,
130.36404834299));
#255991=CARTESIAN_POINT('Ctrl Pts',(-164.489528391681,-3.50259122286156,
135.441555159625));
#255992=CARTESIAN_POINT('Ctrl Pts',(-164.767976015493,2.00816698890481,
136.257706731653));
#255993=CARTESIAN_POINT('Ctrl Pts',(-165.046423639306,5.67351784227885,
132.062499635604));
#255994=CARTESIAN_POINT('Ctrl Pts',(-165.324871263119,4.12518296535417,
126.711124245485));
#255995=CARTESIAN_POINT('Ctrl Pts',(-165.603318886932,-1.21399353033979,
125.121233115594));
#255996=CARTESIAN_POINT('Ctrl Pts',(-165.881766510745,-5.43756927853226,
128.753858523801));
#255997=CARTESIAN_POINT('Ctrl Pts',(-166.160214134558,-4.66428449978105,
134.270795183582));
#255998=CARTESIAN_POINT('Ctrl Pts',(-166.438661758371,0.395249871304121,
136.602247821935));
#255999=CARTESIAN_POINT('Ctrl Pts',(-166.717109382183,5.09156891968999,
133.60572536201));
#256000=CARTESIAN_POINT('Ctrl Pts',(-166.995557005996,5.10898486785074,
128.034885556215));
#256001=CARTESIAN_POINT('Ctrl Pts',(-167.274004629809,0.431493310242956,
125.009058035423));
#256002=CARTESIAN_POINT('Ctrl Pts',(-167.552452253622,-4.64251951985801,
127.30883047135));
#256003=CARTESIAN_POINT('Ctrl Pts',(-167.830899877435,-5.45028371089662,
132.820824345507));
#256004=CARTESIAN_POINT('Ctrl Pts',(-168.109347501248,-1.24950343278299,
136.479786563416));
#256005=CARTESIAN_POINT('Ctrl Pts',(-168.387795125061,4.09950945842204,
134.923309597059));
#256006=CARTESIAN_POINT('Ctrl Pts',(-168.666242748874,5.68127342950807,
129.581719740392));
#256007=CARTESIAN_POINT('Ctrl Pts',(-168.944690372687,2.04222466451309,
125.36367712052));
#256008=CARTESIAN_POINT('Ctrl Pts',(-169.223137996499,-3.47352879894819,
126.145356842267));
#256009=CARTESIAN_POINT('Ctrl Pts',(-169.501585620313,-5.79727898749155,
131.208433428525));
#256010=CARTESIAN_POINT('Ctrl Pts',(-169.780033244125,-2.79361299935373,
135.900186841566));
#256011=CARTESIAN_POINT('Ctrl Pts',(-170.058480867939,2.77724685960862,
135.909124899701));
#256012=CARTESIAN_POINT('Ctrl Pts',(-170.336928491751,5.79595253064181,
131.227033964152));
#256013=CARTESIAN_POINT('Ctrl Pts',(-170.615376115564,3.48846097403773,
126.156526871832));
#256014=CARTESIAN_POINT('Ctrl Pts',(-170.893823739377,-2.02475579691427,
125.357151932539));
#256015=CARTESIAN_POINT('Ctrl Pts',(-171.17227136319,-5.67732090532164,
129.563495663847));
#256016=CARTESIAN_POINT('Ctrl Pts',(-171.450718987003,-4.11270545428381,
134.910133667999));
#256017=CARTESIAN_POINT('Ctrl Pts',(-171.729166610815,1.23128539240979,
136.483766816968));
#256018=CARTESIAN_POINT('Ctrl Pts',(-172.007614234629,5.44378511511418,
132.838303123102));
#256019=CARTESIAN_POINT('Ctrl Pts',(-172.286061858441,4.65371226071637,
127.323745630264));
#256020=CARTESIAN_POINT('Ctrl Pts',(-172.564509482254,-0.412894814796852,
125.00770327326));
#256021=CARTESIAN_POINT('Ctrl Pts',(-172.842957106067,-5.10007172654484,
128.018505833219));
#256022=CARTESIAN_POINT('Ctrl Pts',(-173.12140472988,-5.10053187395325,
133.589372843419));
#256023=CARTESIAN_POINT('Ctrl Pts',(-173.399852353693,-0.413852404033268,
136.600949673471));
#256024=CARTESIAN_POINT('Ctrl Pts',(-173.678299977506,4.65313720737985,
134.285744340263));
#256025=CARTESIAN_POINT('Ctrl Pts',(-173.956747601319,5.44412104360021,
128.771317440947));
#256026=CARTESIAN_POINT('Ctrl Pts',(-174.235195225131,1.23222360085094,
125.125157901261));
#256027=CARTESIAN_POINT('Ctrl Pts',(-174.513642848945,-4.11202713361109,
126.697908213384));
#256028=CARTESIAN_POINT('Ctrl Pts',(-174.792090472757,-5.67752581597763,
132.044287673595));
#256029=CARTESIAN_POINT('Ctrl Pts',(-175.070538096571,-2.02565563601667,
136.251234743121));
#256030=CARTESIAN_POINT('Ctrl Pts',(-175.348985720383,3.48769311466452,
135.452770585855));
#256031=CARTESIAN_POINT('Ctrl Pts',(-175.627433344196,5.79602227624969,
130.382644755183));
#256032=CARTESIAN_POINT('Ctrl Pts',(-175.905880968009,2.77809011739122,
125.700055200075));
#256033=CARTESIAN_POINT('Ctrl Pts',(-176.184328591822,-2.79277114210269,
125.708072964459));
#256034=CARTESIAN_POINT('Ctrl Pts',(-176.462776215635,-5.79721215645926,
130.399330114555));
#256035=CARTESIAN_POINT('Ctrl Pts',(-176.741223839448,-3.47429840858841,
135.462790510077));
#256036=CARTESIAN_POINT('Ctrl Pts',(-177.019671463261,2.04132584786218,
136.245381411334));
#256037=CARTESIAN_POINT('Ctrl Pts',(-177.298119087073,5.68107137443935,
132.02794001176));
#256038=CARTESIAN_POINT('Ctrl Pts',(-177.576566710886,4.10018984367198,
126.686088924097));
#256039=CARTESIAN_POINT('Ctrl Pts',(-177.855014334699,-1.24856584802001,
125.128728333976));
#256040=CARTESIAN_POINT('Ctrl Pts',(-178.133461958512,-5.4499505212146,
128.786996542421));
#256041=CARTESIAN_POINT('Ctrl Pts',(-178.411909582325,-4.64309691029714,
134.29912378221));
#256042=CARTESIAN_POINT('Ctrl Pts',(-178.690357206138,0.430535933288815,
136.599734402363));
#256043=CARTESIAN_POINT('Ctrl Pts',(-178.968804829951,5.10852728703229,
133.574679634036));
#256044=CARTESIAN_POINT('Ctrl Pts',(-179.247252453763,5.09203162942501,
128.00383702718));
#256045=CARTESIAN_POINT('Ctrl Pts',(-179.525700077576,0.396207663951002,
125.006538786706));
#256046=CARTESIAN_POINT('Ctrl Pts',(-179.80414770139,-4.66371178887382,
127.337155569449));
#256047=CARTESIAN_POINT('Ctrl Pts',(-180.082595325202,-5.43790794271038,
132.853964409027));
#256048=CARTESIAN_POINT('Ctrl Pts',(-180.361042949015,-1.2149323537682,
136.487287492965));
#256049=CARTESIAN_POINT('Ctrl Pts',(-180.639490572828,4.12450671554208,
134.898278404822));
#256050=CARTESIAN_POINT('Ctrl Pts',(-180.917938196641,5.67372560662389,
129.547158869193));
#256051=CARTESIAN_POINT('Ctrl Pts',(-181.196385820454,2.00906784212309,
125.351346322599));
#256052=CARTESIAN_POINT('Ctrl Pts',(-181.474833444267,-3.50182512086801,
126.166587518521));
#256053=CARTESIAN_POINT('Ctrl Pts',(-181.75328106808,-5.79471187144949,
131.243715624654));
#256054=CARTESIAN_POINT('Ctrl Pts',(-182.031728691892,-2.76254149958135,
135.917097942958));
#256055=CARTESIAN_POINT('Ctrl Pts',(-182.310176315705,2.80826955274668,
135.892124430331));
#256056=CARTESIAN_POINT('Ctrl Pts',(-182.588623939518,5.79841807769547,
131.191744524852));
#256057=CARTESIAN_POINT('Ctrl Pts',(-182.867071563331,3.46010365771282,
126.135377733334));
#256058=CARTESIAN_POINT('Ctrl Pts',(-183.145519187144,-2.05787698824661,
125.369578119929));
#256059=CARTESIAN_POINT('Ctrl Pts',(-183.423966810957,-5.68476921488759,
129.598078117967));
#256060=CARTESIAN_POINT('Ctrl Pts',(-183.70241443477,-4.08763624946197,
134.93509280296));
#256061=CARTESIAN_POINT('Ctrl Pts',(-183.980862058583,1.26583473708647,
136.476166407061));
#256062=CARTESIAN_POINT('Ctrl Pts',(-184.259309682396,5.45606543971754,
132.805127573733));
#256063=CARTESIAN_POINT('Ctrl Pts',(-184.537757306209,4.63243854686269,
127.295481650585));
#256064=CARTESIAN_POINT('Ctrl Pts',(-184.816204930021,-0.448173063354899,
125.010324079826));
#256065=CARTESIAN_POINT('Ctrl Pts',(-185.094652553834,-5.11693552282041,
128.049603032828));
#256066=CARTESIAN_POINT('Ctrl Pts',(-185.373100177647,-5.08348421301165,
133.620369628814));
#256067=CARTESIAN_POINT('Ctrl Pts',(-185.65154780146,-0.378559253454916,
136.60336151315));
#256068=CARTESIAN_POINT('Ctrl Pts',(-185.929995425273,4.67424316637891,
134.257354871388));
#256069=CARTESIAN_POINT('Ctrl Pts',(-186.208443049086,5.4316444657843,128.73821519851));
#256070=CARTESIAN_POINT('Ctrl Pts',(-186.486890672899,1.19762985171755,
125.117762228929));
#256071=CARTESIAN_POINT('Ctrl Pts',(-186.765338296712,-4.13694808860639,
126.72301537273));
#256072=CARTESIAN_POINT('Ctrl Pts',(-187.043785920525,-5.66987283665109,
132.078825411735));
#256073=CARTESIAN_POINT('Ctrl Pts',(-187.322233544337,-1.99246143649967,
136.263464565965));
#256074=CARTESIAN_POINT('Ctrl Pts',(-187.600681168151,3.51592468664221,
135.43145388367));
#256075=CARTESIAN_POINT('Ctrl Pts',(-187.879128791963,5.79334778522967,
130.347370535898));
#256076=CARTESIAN_POINT('Ctrl Pts',(-188.157576415776,2.74696728996466,
125.683238747971));
#256077=CARTESIAN_POINT('Ctrl Pts',(-188.436024039589,-2.82374194796541,
125.72516777749));
#256078=CARTESIAN_POINT('Ctrl Pts',(-188.714471663402,-5.79957028317828,
130.434626894674));
#256079=CARTESIAN_POINT('Ctrl Pts',(-188.992919287215,-3.44587685290989,
135.483853240698));
#256080=CARTESIAN_POINT('Ctrl Pts',(-189.271366911028,2.07440906473995,
136.232854471987));
#256081=CARTESIAN_POINT('Ctrl Pts',(-189.54981453484,5.68841439241029,131.993335047731));
#256082=CARTESIAN_POINT('Ctrl Pts',(-189.828262158654,4.07504478794802,
126.661206206783));
#256083=CARTESIAN_POINT('Ctrl Pts',(-190.106709782466,-1.28309189963338,
125.136433864998));
#256084=CARTESIAN_POINT('Ctrl Pts',(-190.385157406279,-5.46212981397553,
128.820209315208));
#256085=CARTESIAN_POINT('Ctrl Pts',(-190.663605030092,-4.62173726915045,
134.327322881104));
#256086=CARTESIAN_POINT('Ctrl Pts',(-190.942052653905,0.465806041606811,
136.597006233083));
#256087=CARTESIAN_POINT('Ctrl Pts',(-191.220500277718,5.12529635601715,
133.543531250871));
#256088=CARTESIAN_POINT('Ctrl Pts',(-191.49894790153,5.07488970389458,127.972892272577));
#256089=CARTESIAN_POINT('Ctrl Pts',(-191.777395525344,0.360907336037817,
125.004234378408));
#256090=CARTESIAN_POINT('Ctrl Pts',(-192.055843149156,-4.68473124233415,
127.365609146106));
#256091=CARTESIAN_POINT('Ctrl Pts',(-192.33429077297,-5.42533067084548,
132.887028523726));
#256092=CARTESIAN_POINT('Ctrl Pts',(-192.612738396782,-1.1803162549878,
136.494577839569));
#256093=CARTESIAN_POINT('Ctrl Pts',(-192.891186020595,4.14935113754904,
134.873095510955));
#256094=CARTESIAN_POINT('Ctrl Pts',(-193.169633644408,5.66596754175055,
129.512644584067));
#256095=CARTESIAN_POINT('Ctrl Pts',(-193.448081268221,1.97583657298603,
125.339217588127));
#256096=CARTESIAN_POINT('Ctrl Pts',(-193.726528892034,-3.52999168137001,
126.187990049162));
#256097=CARTESIAN_POINT('Ctrl Pts',(-194.004976515847,-5.79193003022761,
131.27898154032));
#256098=CARTESIAN_POINT('Ctrl Pts',(-194.28342413966,-2.73136763281852,
135.933819589987));
#256099=CARTESIAN_POINT('Ctrl Pts',(-194.561871763472,2.83918818442447,
135.874935432001));
#256100=CARTESIAN_POINT('Ctrl Pts',(-194.840319387286,5.80066876223446,
131.156440730899));
#256101=CARTESIAN_POINT('Ctrl Pts',(-195.118767011098,3.43161812597426,
126.114401605713));
#256102=CARTESIAN_POINT('Ctrl Pts',(-195.397214634911,-2.09092192419104,
125.382205695184));
#256103=CARTESIAN_POINT('Ctrl Pts',(-195.675662258724,-5.69200687323938,
129.63270527133));
#256104=CARTESIAN_POINT('Ctrl Pts',(-195.954109882537,-4.06241557577554,
134.95989887212));
#256105=CARTESIAN_POINT('Ctrl Pts',(-196.23255750635,1.30033717579212,136.468355826305));
#256106=CARTESIAN_POINT('Ctrl Pts',(-196.511005130163,5.46814358780935,
132.771877885207));
#256107=CARTESIAN_POINT('Ctrl Pts',(-196.789452753976,4.61099317629508,
127.267347693709));
#256108=CARTESIAN_POINT('Ctrl Pts',(-197.067900377789,-0.483434704694746,
125.013159586548));
#256109=CARTESIAN_POINT('Ctrl Pts',(-197.346348001602,-5.13360970916836,
128.080802310993));
#256110=CARTESIAN_POINT('Ctrl Pts',(-197.624795625414,-5.06624818169292,
133.651262065958));
#256111=CARTESIAN_POINT('Ctrl Pts',(-197.903243249227,-0.343252075224855,
136.605558468718));
#256112=CARTESIAN_POINT('Ctrl Pts',(-198.18169087304,4.69517591957924,134.228837450539));
#256113=CARTESIAN_POINT('Ctrl Pts',(-198.460138496853,5.41896661638458,
128.705189517851));
#256114=CARTESIAN_POINT('Ctrl Pts',(-198.738586120666,1.1629917239694,125.110577275591));
#256115=CARTESIAN_POINT('Ctrl Pts',(-199.017033744479,-4.16171574746965,
126.748273767825));
#256116=CARTESIAN_POINT('Ctrl Pts',(-199.295481368292,-5.6620097581009,
132.113315924113));
#256117=CARTESIAN_POINT('Ctrl Pts',(-199.573928992105,-1.95919340559182,
136.275492099704));
#256118=CARTESIAN_POINT('Ctrl Pts',(-199.852376615917,3.54402597473752,
135.409965722843));
#256119=CARTESIAN_POINT('Ctrl Pts',(-200.13082423973,5.79045861957696,130.312113250549));
#256120=CARTESIAN_POINT('Ctrl Pts',(-200.409271863544,2.71574267265526,
125.666612060922));
#256121=CARTESIAN_POINT('Ctrl Pts',(-200.687719487356,-2.85460811903155,
125.742450801881));
#256122=CARTESIAN_POINT('Ctrl Pts',(-200.966167111169,-5.80171350468764,
130.469937375411));
#256123=CARTESIAN_POINT('Ctrl Pts',(-201.244614734982,-3.41732760899753,
135.504742570997));
#256124=CARTESIAN_POINT('Ctrl Pts',(-201.523062358795,2.10741541362659,
136.220126377805));
#256125=CARTESIAN_POINT('Ctrl Pts',(-201.801509982608,5.69554662409457,
131.958686025817));
#256126=CARTESIAN_POINT('Ctrl Pts',(-202.079957606421,4.04974872994014,
126.636477015578));
#256127=CARTESIAN_POINT('Ctrl Pts',(-202.358405230234,-1.31757040580477,
125.144349423131));
#256128=CARTESIAN_POINT('Ctrl Pts',(-202.636852854047,-5.47410670550813,
128.853495611451));
#256129=CARTESIAN_POINT('Ctrl Pts',(-202.915300477859,-4.6002063678289,
134.355391435336));
#256130=CARTESIAN_POINT('Ctrl Pts',(-203.193748101672,0.501058889310003,
136.594063415189));
#256131=CARTESIAN_POINT('Ctrl Pts',(-203.472195725485,5.14187550526088,
133.512281366733));
#256132=CARTESIAN_POINT('Ctrl Pts',(-203.750643349298,5.05755972645996,
127.942052439074));
#256133=CARTESIAN_POINT('Ctrl Pts',(-204.029090973111,0.325593634571106,
125.002144895921));
#256134=CARTESIAN_POINT('Ctrl Pts',(-204.307538596924,-4.70557710135553,
127.394190146963));
#256135=CARTESIAN_POINT('Ctrl Pts',(-204.585986220737,-5.41255236135747,
132.920015464399));
#256136=CARTESIAN_POINT('Ctrl Pts',(-204.864433844549,-1.14565641915494,
136.50165733308));
#256137=CARTESIAN_POINT('Ctrl Pts',(-205.142881468362,4.17404180382362,
134.847761848621));
#256138=CARTESIAN_POINT('Ctrl Pts',(-205.421329092175,5.6579995223666,129.478178163952));
#256139=CARTESIAN_POINT('Ctrl Pts',(-205.699776715988,1.94253208849746,
125.327291366541));
#256140=CARTESIAN_POINT('Ctrl Pts',(-205.978224339801,-3.55802743673226,
126.209563641112));
#256141=CARTESIAN_POINT('Ctrl Pts',(-206.256671963614,-5.78893356690891,
131.314229868733));
#256142=CARTESIAN_POINT('Ctrl Pts',(-206.535119587427,-2.70009255422283,
135.950351163029));
#256143=CARTESIAN_POINT('Ctrl Pts',(-206.81356721124,2.87000160893922,135.857558541658));
#256144=CARTESIAN_POINT('Ctrl Pts',(-207.092014835053,5.80270450085972,
131.121123890489));
#256145=CARTESIAN_POINT('Ctrl Pts',(-207.370462458865,3.40300543436423,
126.09359926625));
#256146=CARTESIAN_POINT('Ctrl Pts',(-207.648910082679,-2.12388938025395,
125.395034190384));
#256147=CARTESIAN_POINT('Ctrl Pts',(-207.927357706491,-5.69903361218359,
129.667375840811));
#256148=CARTESIAN_POINT('Ctrl Pts',(-208.205805330304,-4.03704436778601,
134.984550956282));
#256149=CARTESIAN_POINT('Ctrl Pts',(-208.484252954117,1.33479143002538,
136.460335364123));
#256150=CARTESIAN_POINT('Ctrl Pts',(-208.76270057793,5.48001911182977,132.738555289606));
#256151=CARTESIAN_POINT('Ctrl Pts',(-209.041148201743,4.58937694367963,
127.239344802146));
#256152=CARTESIAN_POINT('Ctrl Pts',(-209.319595825556,-0.518678432184342,
125.016209688352));
#256153=CARTESIAN_POINT('Ctrl Pts',(-209.598043449369,-5.15009366772074,
128.112102511612));
#256154=CARTESIAN_POINT('Ctrl Pts',(-209.876491073182,-5.04882441868487,
133.682049010123));
#256155=CARTESIAN_POINT('Ctrl Pts',(-210.154938696994,-0.307932177662294,
136.607540458767));
#256156=CARTESIAN_POINT('Ctrl Pts',(-210.433386320807,4.71593469130848,
134.200193134443));
#256157=CARTESIAN_POINT('Ctrl Pts',(-210.71183394462,5.40608796518471,128.672241622749));
#256158=CARTESIAN_POINT('Ctrl Pts',(-210.990281568433,1.12831050113542,
125.103603307488));
#256159=CARTESIAN_POINT('Ctrl Pts',(-211.268729192246,-4.18632919242468,
126.773682462711));
#256160=CARTESIAN_POINT('Ctrl Pts',(-211.547176816059,-5.65393687169752,
132.14775793267));
#256161=CARTESIAN_POINT('Ctrl Pts',(-211.825624439872,-1.92585277605142,
136.287316898656));
#256162=CARTESIAN_POINT('Ctrl Pts',(-212.104072063685,3.57199593764717,
135.388306899624));
#256163=CARTESIAN_POINT('Ctrl Pts',(-212.382519687498,5.78735488635066,
130.276874205606));
#256164=CARTESIAN_POINT('Ctrl Pts',(-212.660967311311,2.68441742250212,
125.650175755035));
#256165=CARTESIAN_POINT('Ctrl Pts',(-212.939414935123,-2.88536851154432,
125.759921397201));
#256166=CARTESIAN_POINT('Ctrl Pts',(-213.217862558936,-5.80364174156953,
130.505260248325));
#256167=CARTESIAN_POINT('Ctrl Pts',(-213.496310182749,-3.38865173475374,
135.525457726916));
#256168=CARTESIAN_POINT('Ctrl Pts',(-213.774757806562,2.14034367146046,
136.20719760043));
#256169=CARTESIAN_POINT('Ctrl Pts',(-214.053205430375,5.7024678052036,131.923994229952));
#256170=CARTESIAN_POINT('Ctrl Pts',(-214.331653054188,4.02430260700449,
126.611902266833));
#256171=CARTESIAN_POINT('Ctrl Pts',(-214.610100678001,-1.35200008892003,
125.152474715061));
#256172=CARTESIAN_POINT('Ctrl Pts',(-214.888548301814,-5.48588075200302,
128.886854197714));
#256173=CARTESIAN_POINT('Ctrl Pts',(-215.166995925626,-4.5785050041694,
134.383328404815));
#256174=CARTESIAN_POINT('Ctrl Pts',(-215.445443549439,0.536293170092427,
136.59090605773));
#256175=CARTESIAN_POINT('Ctrl Pts',(-215.723891173253,5.15826412041666,
133.480931139593));
#256176=CARTESIAN_POINT('Ctrl Pts',(-216.002338797065,5.04004233928969,
127.911318669453));
#256177=CARTESIAN_POINT('Ctrl Pts',(-216.280786420879,0.290267868112,125.000270416672));
#256178=CARTESIAN_POINT('Ctrl Pts',(-216.559234044691,-4.72624859348692,
127.422897512942));
#256179=CARTESIAN_POINT('Ctrl Pts',(-216.837681668504,-5.39957348775117,
132.952924008705));
#256180=CARTESIAN_POINT('Ctrl Pts',(-217.116129292317,-1.11095413060172,
136.508525711168));
#256181=CARTESIAN_POINT('Ctrl Pts',(-217.39457691613,4.19857779944424,134.822278356567));
#256182=CARTESIAN_POINT('Ctrl Pts',(-217.673024539943,5.64982184372931,
129.443760886018));
#256183=CARTESIAN_POINT('Ctrl Pts',(-217.951472163756,1.90915562276867,
125.315568099769));
#256184=CARTESIAN_POINT('Ctrl Pts',(-218.229919787568,-3.58593134807924,
126.231307494954));
#256185=CARTESIAN_POINT('Ctrl Pts',(-218.508367411381,-5.78572259252759,
131.349459303753));
#256186=CARTESIAN_POINT('Ctrl Pts',(-218.786815035194,-2.66871742270537,
135.966692049498));
#256187=CARTESIAN_POINT('Ctrl Pts',(-219.065262659007,2.90070868448967,
135.839994403207));
#256188=CARTESIAN_POINT('Ctrl Pts',(-219.34371028282,5.80452521813531,131.085795312298));
#256189=CARTESIAN_POINT('Ctrl Pts',(-219.622157906633,3.37426664313623,
126.07297148578));
#256190=CARTESIAN_POINT('Ctrl Pts',(-219.900605530446,-2.15677813481551,
125.408063130162));
#256191=CARTESIAN_POINT('Ctrl Pts',(-220.179053154259,-5.70584917134113,
129.702088541682));
#256192=CARTESIAN_POINT('Ctrl Pts',(-220.457500778071,-4.01152356563293,
135.009048141953));
#256193=CARTESIAN_POINT('Ctrl Pts',(-220.735948401884,1.36919622307095,
136.452105317718));
#256194=CARTESIAN_POINT('Ctrl Pts',(-221.014396025697,5.49169157172664,
132.705161021709));
#256195=CARTESIAN_POINT('Ctrl Pts',(-221.29284364951,4.56759065001379,127.211474013555));
#256196=CARTESIAN_POINT('Ctrl Pts',(-221.571291273323,-0.553902939853376,
125.019474272218));
#256197=CARTESIAN_POINT('Ctrl Pts',(-221.849738897136,-5.16638678765824,
128.143502474846));
#256198=CARTESIAN_POINT('Ctrl Pts',(-222.128186520948,-5.03121356963114,
133.712729320486));
#256199=CARTESIAN_POINT('Ctrl Pts',(-222.406634144762,-0.272600869560251,
136.609307409853));
#256200=CARTESIAN_POINT('Ctrl Pts',(-222.685081768574,4.73651871234416,
134.171422984523));
#256201=CARTESIAN_POINT('Ctrl Pts',(-222.963529392388,5.39300898940659,
128.639372734101));
#256202=CARTESIAN_POINT('Ctrl Pts',(-223.2419770162,1.09358746834067,125.096840583045));
#256203=CARTESIAN_POINT('Ctrl Pts',(-223.520424640014,-4.21078751141269,
126.799240515859));
#256204=CARTESIAN_POINT('Ctrl Pts',(-223.798872263826,-5.64565447658353,
132.182150161146));
#256205=CARTESIAN_POINT('Ctrl Pts',(-224.077319887639,-1.89244078332859,
136.298938524645));
#256206=CARTESIAN_POINT('Ctrl Pts',(-224.355767511452,3.59983353893359,
135.366478216591));
#256207=CARTESIAN_POINT('Ctrl Pts',(-224.634215135265,5.78403670056078,
130.241654706868));
#256208=CARTESIAN_POINT('Ctrl Pts',(-224.912662759078,2.65299270027449,
125.633930439363));
#256209=CARTESIAN_POINT('Ctrl Pts',(-225.191110382891,-2.91602198566553,
125.77757891607));
#256210=CARTESIAN_POINT('Ctrl Pts',(-225.469558006704,-5.8053549223724,
130.540594204513));
#256211=CARTESIAN_POINT('Ctrl Pts',(-225.748005630516,-3.35985029277391,
135.545997940844));
#256212=CARTESIAN_POINT('Ctrl Pts',(-226.026453254329,2.17319261807209,
136.194068618944));
#256213=CARTESIAN_POINT('Ctrl Pts',(-226.304900878142,5.7091776792716,131.88926094565));
#256214=CARTESIAN_POINT('Ctrl Pts',(-226.583348501955,3.99870736205508,
126.587482871174));
#256215=CARTESIAN_POINT('Ctrl Pts',(-226.861796125768,-1.38637967317499,
125.160809439701));
#256216=CARTESIAN_POINT('Ctrl Pts',(-227.140243749581,-5.49745151716988,
128.920283837883));
#256217=CARTESIAN_POINT('Ctrl Pts',(-227.418691373394,-4.55663398232247,
134.411132754326));
#256218=CARTESIAN_POINT('Ctrl Pts',(-227.697138997207,0.571507578333558,
136.5875342777));
#256219=CARTESIAN_POINT('Ctrl Pts',(-227.97558662102,5.17446159419872,133.44948173115));
#256220=CARTESIAN_POINT('Ctrl Pts',(-228.254034244832,5.02233819149715,
127.880692102567));
#256221=CARTESIAN_POINT('Ctrl Pts',(-228.532481868645,0.254931345670833,
124.998611010119));
#256222=CARTESIAN_POINT('Ctrl Pts',(-228.810929492458,-4.74674495273865,
127.451730180279));
#256223=CARTESIAN_POINT('Ctrl Pts',(-229.089377116271,-5.38639453096373,
132.985752937203));
#256224=CARTESIAN_POINT('Ctrl Pts',(-229.367824740084,-1.07621067523457,
136.515182719319));
#256225=CARTESIAN_POINT('Ctrl Pts',(-229.646272363897,4.22295821522052,
134.796645979094));
#256226=CARTESIAN_POINT('Ctrl Pts',(-229.92471998771,5.64143480886619,129.409394025606));
#256227=CARTESIAN_POINT('Ctrl Pts',(-230.203167611523,1.87570841257552,
125.304048222223));
#256228=CARTESIAN_POINT('Ctrl Pts',(-230.481615235336,-3.61370238142155,
126.25322080496));
#256229=CARTESIAN_POINT('Ctrl Pts',(-230.760062859148,-5.78229722606833,
131.384668539942));
#256230=CARTESIAN_POINT('Ctrl Pts',(-231.038510482961,-2.63724340088164,
135.982841643878));
#256231=CARTESIAN_POINT('Ctrl Pts',(-231.316958106774,2.93130827321233,
135.822243667495));
#256232=CARTESIAN_POINT('Ctrl Pts',(-231.595405730587,5.80613084659478,
131.050456305442));
#256233=CARTESIAN_POINT('Ctrl Pts',(-231.8738533544,3.34540281721704,126.052519028673));
#256234=CARTESIAN_POINT('Ctrl Pts',(-232.152300978213,-2.18958696916944,
125.42129203173));
#256235=CARTESIAN_POINT('Ctrl Pts',(-232.430748602025,-5.71245329815966,
129.736842087648));
#256236=CARTESIAN_POINT('Ctrl Pts',(-232.709196225839,-3.98585411499877,
135.033389521383));
#256237=CARTESIAN_POINT('Ctrl Pts',(-232.987643849651,1.40355028004735,
136.443665992055));
#256238=CARTESIAN_POINT('Ctrl Pts',(-233.266091473464,5.50316053497282,
132.671696318956));
#256239=CARTESIAN_POINT('Ctrl Pts',(-233.544539097277,4.5456351025967,127.183736360699));
#256240=CARTESIAN_POINT('Ctrl Pts',(-233.82298672109,-0.589106922445798,
125.022953217175));
#256241=CARTESIAN_POINT('Ctrl Pts',(-234.101434344904,-5.18248846523346,
128.175001037157));
#256242=CARTESIAN_POINT('Ctrl Pts',(-234.379881968716,-5.01341628710851,
133.743301860178));
#256243=CARTESIAN_POINT('Ctrl Pts',(-234.658329592529,-0.237259460132118,
136.610859256499));
#256244=CARTESIAN_POINT('Ctrl Pts',(-234.936777216342,4.75692721993639,
134.14252806687));
#256245=CARTESIAN_POINT('Ctrl Pts',(-235.215224840155,5.37973017369771,
128.606584069875));
#256246=CARTESIAN_POINT('Ctrl Pts',(-235.493672463967,1.05882391226032,
125.090289352854));
#256247=CARTESIAN_POINT('Ctrl Pts',(-235.772120087781,-4.23508979812022,
126.824946980203));
#256248=CARTESIAN_POINT('Ctrl Pts',(-236.050567711593,-5.63716287966734,
132.216491335124));
#256249=CARTESIAN_POINT('Ctrl Pts',(-236.329015335406,-1.85895866551617,
136.310356547029));
#256250=CARTESIAN_POINT('Ctrl Pts',(-236.607462959219,3.62753774706455,
135.344480482612));
#256251=CARTESIAN_POINT('Ctrl Pts',(-236.885910583032,5.78050418516386,
130.206456059403));
#256252=CARTESIAN_POINT('Ctrl Pts',(-237.164358206845,2.62146967042642,
125.617876715884));
#256253=CARTESIAN_POINT('Ctrl Pts',(-237.442805830658,-2.94656740551997,
125.795422704185));
#256254=CARTESIAN_POINT('Ctrl Pts',(-237.72125345447,-5.80685298361372,
130.575937934662));
#256255=CARTESIAN_POINT('Ctrl Pts',(-237.999701078284,-3.33092435030571,
135.566362451659));
#256256=CARTESIAN_POINT('Ctrl Pts',(-238.278148702096,2.20596103623244,
136.180739919846));
#256257=CARTESIAN_POINT('Ctrl Pts',(-238.55659632591,5.7156759976606,131.854487459968));
#256258=CARTESIAN_POINT('Ctrl Pts',(-238.835043949722,3.97296394353457,
126.56321973347));
#256259=CARTESIAN_POINT('Ctrl Pts',(-239.113491573535,-1.42070788462113,
125.169353288205));
#256260=CARTESIAN_POINT('Ctrl Pts',(-239.391939197348,-5.50881857224844,
128.95378329321));
#256261=CARTESIAN_POINT('Ctrl Pts',(-239.670386821161,-4.53459411272838,
134.438803453569));
#256262=CARTESIAN_POINT('Ctrl Pts',(-239.948834444974,0.606700809151854,
136.583948200045));
#256263=CARTESIAN_POINT('Ctrl Pts',(-240.227282068787,5.1904673264033,133.417934306771));
#256264=CARTESIAN_POINT('Ctrl Pts',(-240.5057296926,5.00444793911587,127.850173873291));
#256265=CARTESIAN_POINT('Ctrl Pts',(-240.784177316413,0.21958537665436,
124.997166737753));
#256266=CARTESIAN_POINT('Ctrl Pts',(-241.062624940225,-4.76706541961049,
127.48068708057));
#256267=CARTESIAN_POINT('Ctrl Pts',(-241.341072564039,-5.37301597934592,
133.018501033406));
#256268=CARTESIAN_POINT('Ctrl Pts',(-241.619520187851,-1.04142734048567,
136.521628110858));
#256269=CARTESIAN_POINT('Ctrl Pts',(-241.897967811664,4.24718214772698,
134.770865666018));
#256270=CARTESIAN_POINT('Ctrl Pts',(-242.176415435477,5.63283872856131,
129.375078856195));
#256271=CARTESIAN_POINT('Ctrl Pts',(-242.45486305929,1.84219169731802,125.292732160775));
#256272=CARTESIAN_POINT('Ctrl Pts',(-242.733310683103,-3.64133950769301,
126.275302759127));
#256273=CARTESIAN_POINT('Ctrl Pts',(-243.011758306915,-5.77865759445851,
131.419856272607));
#256274=CARTESIAN_POINT('Ctrl Pts',(-243.290205930729,-2.60567165503458,
135.998799347738));
#256275=CARTESIAN_POINT('Ctrl Pts',(-243.568653554541,2.96179924122969,
135.80430699228));
#256276=CARTESIAN_POINT('Ctrl Pts',(-243.847101178355,5.80752132674009,
131.015108179419));
#256277=CARTESIAN_POINT('Ctrl Pts',(-244.125548802166,3.31641502616601,
126.032242652805));
#256278=CARTESIAN_POINT('Ctrl Pts',(-244.403996425981,-2.22231466757369,
125.434720404883));
#256279=CARTESIAN_POINT('Ctrl Pts',(-244.682444049792,-5.71884574792013,
129.771635190908));
#256280=CARTESIAN_POINT('Ctrl Pts',(-244.960891673606,-3.96003696707471,
135.05757419259));
#256281=CARTESIAN_POINT('Ctrl Pts',(-245.239339297418,1.43785232795156,
136.435017699859));
#256282=CARTESIAN_POINT('Ctrl Pts',(-245.517786921232,5.51442557658153,
132.638162421391));
#256283=CARTESIAN_POINT('Ctrl Pts',(-245.796234545044,4.52351111499922,
127.156132871406));
#256284=CARTESIAN_POINT('Ctrl Pts',(-246.074682168857,-0.624289075464052,
125.026646394309));
#256285=CARTESIAN_POINT('Ctrl Pts',(-246.353129792671,-5.19839810379266,
128.206597031353));
#256286=CARTESIAN_POINT('Ctrl Pts',(-246.631577416483,-4.99543323060155,
133.773765496319));
#256287=CARTESIAN_POINT('Ctrl Pts',(-246.910025040296,-0.201909258968066,
136.612195941205));
#256288=CARTESIAN_POINT('Ctrl Pts',(-247.188472664109,4.77715945784187,
134.113509452194));
#256289=CARTESIAN_POINT('Ctrl Pts',(-247.466920287922,5.36625201010822,
128.573876845067));
#256290=CARTESIAN_POINT('Ctrl Pts',(-247.745367911734,1.02402112107033,
125.083949859676));
#256291=CARTESIAN_POINT('Ctrl Pts',(-248.023815535548,-4.25923515201858,
126.850800903184));
#256292=CARTESIAN_POINT('Ctrl Pts',(-248.30226315936,-5.62846239560694,
132.250780182078));
#256293=CARTESIAN_POINT('Ctrl Pts',(-248.580710783174,-1.82540766330725,
136.32157054271));
#256294=CARTESIAN_POINT('Ctrl Pts',(-248.859158406986,3.65510753545023,
135.322314512822));
#256295=CARTESIAN_POINT('Ctrl Pts',(-249.137606030799,5.7767574710584,130.171279567513));
#256296=CARTESIAN_POINT('Ctrl Pts',(-249.416053654612,2.58984950105633,
125.602015179472));
#256297=CARTESIAN_POINT('Ctrl Pts',(-249.694501278425,-2.97700363923603,
125.813452100338));
#256298=CARTESIAN_POINT('Ctrl Pts',(-249.972948902238,-5.80813586978118,
130.611290129096));
#256299=CARTESIAN_POINT('Ctrl Pts',(-250.251396526051,-3.30187497921299,
135.586550504748));
#256300=CARTESIAN_POINT('Ctrl Pts',(-250.529844149864,2.23864771169993,
136.167211997028));
#256301=CARTESIAN_POINT('Ctrl Pts',(-250.808291773676,5.72196251956533,
131.819675061465));
#256302=CARTESIAN_POINT('Ctrl Pts',(-251.08673939749,3.94707330538994,126.539113752772));
#256303=CARTESIAN_POINT('Ctrl Pts',(-251.365187021302,-1.45498345124562,
125.178105944033));
#256304=CARTESIAN_POINT('Ctrl Pts',(-251.643634645115,-5.5199814959705,
128.987351322257));
#256305=CARTESIAN_POINT('Ctrl Pts',(-251.922082268928,-4.51238621219265,
134.466339477392));
#256306=CARTESIAN_POINT('Ctrl Pts',(-252.200529892741,0.641871558658502,
136.580147957277));
#256307=CARTESIAN_POINT('Ctrl Pts',(-252.478977516554,5.20628072353487,
133.386290036154));
#256308=CARTESIAN_POINT('Ctrl Pts',(-252.757425140367,4.98637224582674,
127.819765111179));
#256309=CARTESIAN_POINT('Ctrl Pts',(-253.035872764179,0.184231269403876,
124.995937655572));
#256310=CARTESIAN_POINT('Ctrl Pts',(-253.314320387993,-4.78720923844335,
127.509767136124));
#256311=CARTESIAN_POINT('Ctrl Pts',(-253.592768011806,-5.35943833369967,
133.051167092665));
#256312=CARTESIAN_POINT('Ctrl Pts',(-253.871215635618,-1.00660540571931,
136.527861630253));
#256313=CARTESIAN_POINT('Ctrl Pts',(-254.149663259431,4.27124868131666,
134.744938404161));
#256314=CARTESIAN_POINT('Ctrl Pts',(-254.428110883244,5.62403395537261,
129.340816589823));
#256315=CARTESIAN_POINT('Ctrl Pts',(-254.706558507057,1.80860665472018,
125.281620447135));
#256316=CARTESIAN_POINT('Ctrl Pts',(-254.98500613087,-3.66884158147516,
126.297552326988));
#256317=CARTESIAN_POINT('Ctrl Pts',(-255.263453754682,-5.77480406163408,
131.45502159855));
#256318=CARTESIAN_POINT('Ctrl Pts',(-255.541901378496,-2.57400292253984,
136.014563813166));
#256319=CARTESIAN_POINT('Ctrl Pts',(-255.820349002309,2.99217964199006,
135.78618647082));
#256320=CARTESIAN_POINT('Ctrl Pts',(-256.098796626121,5.80869814913581,
130.979749546569));
#256321=CARTESIAN_POINT('Ctrl Pts',(-256.377244249934,3.28730143236016,
126.01214820295));
#256322=CARTESIAN_POINT('Ctrl Pts',(-256.655691873747,-2.25495451926359,
125.448338134603));
#256323=CARTESIAN_POINT('Ctrl Pts',(-256.93413949756,-5.72503666514098,
129.806484721847));
#256324=CARTESIAN_POINT('Ctrl Pts',(-257.212587121373,-3.93405347634203,
135.081566970265));
#256325=CARTESIAN_POINT('Ctrl Pts',(-257.491034745186,1.47206408278265,
136.426225506557));
#256326=CARTESIAN_POINT('Ctrl Pts',(-257.769482368999,5.52555616721843,
132.604438319186));
#256327=CARTESIAN_POINT('Ctrl Pts',(-258.047929992812,4.50108754276566,
127.128895412351));
#256328=CARTESIAN_POINT('Ctrl Pts',(-258.326377616624,-0.659198908970111,
125.030117734768));
#256329=CARTESIAN_POINT('Ctrl Pts',(-258.604825240438,-5.21458571703409,
128.239112839452));
#256330=CARTESIAN_POINT('Ctrl Pts',(-258.883272864251,-4.97637574492231,
133.802560593787));
#256331=CARTESIAN_POINT('Ctrl Pts',(-259.161720488063,-0.168236736403017,
136.616288572087));
#256332=CARTESIAN_POINT('Ctrl Pts',(-259.440168111876,4.80044487344316,
134.078525892203));
#256333=CARTESIAN_POINT('Ctrl Pts',(-259.672207798387,5.25516631655033,
129.4749169549));
#256334=CARTESIAN_POINT('Ctrl Pts',(-259.857849473896,3.17366342871357,
126.795179433485));
#256335=CARTESIAN_POINT('Ctrl Pts',(-259.9506752748,1.64266665146648,126.102093112095));
#256336=CARTESIAN_POINT('Ctrl Pts',(-259.997093138402,0.835778587061721,
125.962806053044));
#256337=CARTESIAN_POINT('Ctrl Pts',(210.385579563201,-2.29217962691353,
126.082387726892));
#256338=CARTESIAN_POINT('Ctrl Pts',(210.339169886847,-3.0789974560272,126.464330840008));
#256339=CARTESIAN_POINT('Ctrl Pts',(210.246352273192,-4.44507089109247,
127.629120819077));
#256340=CARTESIAN_POINT('Ctrl Pts',(210.060718784933,-5.78798125627161,
130.996088365878));
#256341=CARTESIAN_POINT('Ctrl Pts',(209.828679098422,-3.95783017776954,
135.586872998689));
#256342=CARTESIAN_POINT('Ctrl Pts',(209.550231474609,1.89393692750204,136.720289837399));
#256343=CARTESIAN_POINT('Ctrl Pts',(209.271783850796,5.99602695027556,132.40812259401));
#256344=CARTESIAN_POINT('Ctrl Pts',(208.993336226983,4.59288360023261,126.626877830413));
#256345=CARTESIAN_POINT('Ctrl Pts',(208.71488860317,-1.03344059257722,124.682062423228));
#256346=CARTESIAN_POINT('Ctrl Pts',(208.436440979357,-5.70873650289865,
128.364647771496));
#256347=CARTESIAN_POINT('Ctrl Pts',(208.157993355544,-5.13869562717284,
134.288517668348));
#256348=CARTESIAN_POINT('Ctrl Pts',(207.879545731732,0.153933173725622,
137.010984097728));
#256349=CARTESIAN_POINT('Ctrl Pts',(207.601098107919,5.30490488755997,134.029672582798));
#256350=CARTESIAN_POINT('Ctrl Pts',(207.322650484106,5.58103410012833,128.084559773234));
#256351=CARTESIAN_POINT('Ctrl Pts',(207.044202860293,0.728409521696789,
124.638756607567));
#256352=CARTESIAN_POINT('Ctrl Pts',(206.76575523648,-4.79355811073501,126.858871164077));
#256353=CARTESIAN_POINT('Ctrl Pts',(206.487307612667,-5.91049575314416,
132.704682504842));
#256354=CARTESIAN_POINT('Ctrl Pts',(206.208859988854,-1.59596820864792,
136.804198957117));
#256355=CARTESIAN_POINT('Ctrl Pts',(205.930412365042,4.1851717387407,135.390152799229));
#256356=CARTESIAN_POINT('Ctrl Pts',(205.651964741228,6.12034565262566,129.76198992389));
#256357=CARTESIAN_POINT('Ctrl Pts',(205.373517117416,2.43121966936229,125.091713591677));
#256358=CARTESIAN_POINT('Ctrl Pts',(205.095069493603,-3.49207776276838,
125.671081434371));
#256359=CARTESIAN_POINT('Ctrl Pts',(204.81662186979,-6.20632667560231,130.96768173473));
#256360=CARTESIAN_POINT('Ctrl Pts',(204.538174245977,-3.21726438559061,
136.114198085604));
#256361=CARTESIAN_POINT('Ctrl Pts',(204.259726622164,2.72830660529182,136.381233108793));
#256362=CARTESIAN_POINT('Ctrl Pts',(203.981278998351,6.16669716267351,131.523394807979));
#256363=CARTESIAN_POINT('Ctrl Pts',(203.702831374538,3.9381942601484,126.004799186432));
#256364=CARTESIAN_POINT('Ctrl Pts',(203.424383750725,-1.909316761502,124.896766062528));
#256365=CARTESIAN_POINT('Ctrl Pts',(203.145936126912,-6.00225896230248,
129.217523725228));
#256366=CARTESIAN_POINT('Ctrl Pts',(202.867488503099,-4.57941839934143,
134.996506974633));
#256367=CARTESIAN_POINT('Ctrl Pts',(202.589040879287,1.05168395343957,136.923112517541));
#256368=CARTESIAN_POINT('Ctrl Pts',(202.310593255474,5.71634013176502,133.226883983125));
#256369=CARTESIAN_POINT('Ctrl Pts',(202.032145631661,5.12795898713612,127.30447482202));
#256370=CARTESIAN_POINT('Ctrl Pts',(201.753698007848,-0.172765951628197,
124.598289728405));
#256371=CARTESIAN_POINT('Ctrl Pts',(201.475250384035,-5.31472742110118,
127.595180598346));
#256372=CARTESIAN_POINT('Ctrl Pts',(201.196802760222,-5.57271402936141,
133.541151128878));
#256373=CARTESIAN_POINT('Ctrl Pts',(200.918355136409,-0.709648686901125,
136.972144879116));
#256374=CARTESIAN_POINT('Ctrl Pts',(200.639907512596,4.80554913058071,134.735246206027));
#256375=CARTESIAN_POINT('Ctrl Pts',(200.361459888783,5.90468206117194,128.886055711564));
#256376=CARTESIAN_POINT('Ctrl Pts',(200.083012264971,1.57770063730838,124.799693711321));
#256377=CARTESIAN_POINT('Ctrl Pts',(199.804564641158,-4.19911059728431,
126.231327253625));
#256378=CARTESIAN_POINT('Ctrl Pts',(199.526117017345,-6.11714433092778,
131.865355052293));
#256379=CARTESIAN_POINT('Ctrl Pts',(199.247669393532,-2.4138212635637,136.524380797905));
#256380=CARTESIAN_POINT('Ctrl Pts',(198.969221769719,3.50768562329156,135.926987436306));
#256381=CARTESIAN_POINT('Ctrl Pts',(198.690774145906,6.20580078231077,130.622150282517));
#256382=CARTESIAN_POINT('Ctrl Pts',(198.412326522093,3.20108819260905,125.484755525167));
#256383=CARTESIAN_POINT('Ctrl Pts',(198.13387889828,-2.74526806424844,125.235817970576));
#256384=CARTESIAN_POINT('Ctrl Pts',(197.855431274468,-6.16885708386238,
130.104099070135));
#256385=CARTESIAN_POINT('Ctrl Pts',(197.576983650655,-3.92356780882929,
135.615886322105));
#256386=CARTESIAN_POINT('Ctrl Pts',(197.298536026841,1.92728860557448,136.706116507701));
#256387=CARTESIAN_POINT('Ctrl Pts',(197.020088403029,6.00706094473797,132.372921347066));
#256388=CARTESIAN_POINT('Ctrl Pts',(196.741640779216,4.56663773692898,126.598295504472));
#256389=CARTESIAN_POINT('Ctrl Pts',(196.463193155403,-1.07030245846182,
124.688838023107));
#256390=CARTESIAN_POINT('Ctrl Pts',(196.184745531591,-5.72368698170812,
128.399247046161));
#256391=CARTESIAN_POINT('Ctrl Pts',(195.906297907777,-5.11728278641862,
134.319837945007));
#256392=CARTESIAN_POINT('Ctrl Pts',(195.627850283965,0.191654296427489,
137.009876920548));
#256393=CARTESIAN_POINT('Ctrl Pts',(195.349402660151,5.32447044368961,133.997349569974));
#256394=CARTESIAN_POINT('Ctrl Pts',(195.070955036339,5.56435836804288,128.050621358318));
#256395=CARTESIAN_POINT('Ctrl Pts',(194.792507412526,0.690872786183208,
124.634444998269));
#256396=CARTESIAN_POINT('Ctrl Pts',(194.514059788713,-4.81749113516689,
126.888119675218));
#256397=CARTESIAN_POINT('Ctrl Pts',(194.2356121649,-5.89881605082435,132.740628459178));
#256398=CARTESIAN_POINT('Ctrl Pts',(193.957164541087,-1.55941718895885,
136.81380168864));
#256399=CARTESIAN_POINT('Ctrl Pts',(193.678716917274,4.21300988779493,135.364592151301));
#256400=CARTESIAN_POINT('Ctrl Pts',(193.400269293461,6.11388669464029,129.724752614155));
#256401=CARTESIAN_POINT('Ctrl Pts',(193.121821669648,2.39640030908087,125.077020090361));
#256402=CARTESIAN_POINT('Ctrl Pts',(192.843374045836,-3.52326088986039,
125.692433714928));
#256403=CARTESIAN_POINT('Ctrl Pts',(192.564926422022,-6.20521745188322,
131.005458431507));
#256404=CARTESIAN_POINT('Ctrl Pts',(192.28647879821,-3.1848823173506,136.133684081248));
#256405=CARTESIAN_POINT('Ctrl Pts',(192.008031174397,2.76220407667619,136.36452181979));
#256406=CARTESIAN_POINT('Ctrl Pts',(191.729583550584,6.17095986540858,131.485843042463));
#256407=CARTESIAN_POINT('Ctrl Pts',(191.451135926771,3.90890500597959,125.980915208923));
#256408=CARTESIAN_POINT('Ctrl Pts',(191.172688302958,-1.94524259331895,
124.908498067517));
#256409=CARTESIAN_POINT('Ctrl Pts',(190.894240679145,-6.01180727974115,
129.254090580708));
#256410=CARTESIAN_POINT('Ctrl Pts',(190.615793055332,-4.5538147691942,135.024305522869));
#256411=CARTESIAN_POINT('Ctrl Pts',(190.337345431519,1.08891104802307,136.916597252826));
#256412=CARTESIAN_POINT('Ctrl Pts',(190.058897807707,5.73098080836918,133.192042114338));
#256413=CARTESIAN_POINT('Ctrl Pts',(189.780450183893,5.10655917980125,127.273324325042));
#256414=CARTESIAN_POINT('Ctrl Pts',(189.502002560081,-0.210540865719208,
124.599456387862));
#256415=CARTESIAN_POINT('Ctrl Pts',(189.223554936268,-5.33416414113684,
127.627592311355));
#256416=CARTESIAN_POINT('Ctrl Pts',(188.945107312455,-5.55595115925501,
133.575023114497));
#256417=CARTESIAN_POINT('Ctrl Pts',(188.666659688642,-0.672090485321342,
136.976350437346));
#256418=CARTESIAN_POINT('Ctrl Pts',(188.388212064829,4.82938851117716,134.705920634282));
#256419=CARTESIAN_POINT('Ctrl Pts',(188.109764441016,5.89289539464864,128.850147777659));
#256420=CARTESIAN_POINT('Ctrl Pts',(187.831316817203,1.54111929438253,124.790201052305));
#256421=CARTESIAN_POINT('Ctrl Pts',(187.552869193391,-4.22687014955807,
126.256973159398));
#256422=CARTESIAN_POINT('Ctrl Pts',(187.274421569578,-6.11057242014135,
131.902572188318));
#256423=CARTESIAN_POINT('Ctrl Pts',(186.995973945765,-2.37895715467313,
136.538968434335));
#256424=CARTESIAN_POINT('Ctrl Pts',(186.717526321952,3.53880351742172,135.905540247907));
#256425=CARTESIAN_POINT('Ctrl Pts',(186.439078698139,6.20457663716883,130.584377187674));
#256426=CARTESIAN_POINT('Ctrl Pts',(186.160631074326,3.16864693777749,125.465368152723));
#256427=CARTESIAN_POINT('Ctrl Pts',(185.882183450513,-2.77911450042273,
125.25263236868));
#256428=CARTESIAN_POINT('Ctrl Pts',(185.6037358267,-6.17300548002561,130.14166362836));
#256429=CARTESIAN_POINT('Ctrl Pts',(185.325288202887,-3.89420599156785,
135.639681046572));
#256430=CARTESIAN_POINT('Ctrl Pts',(185.046840579075,1.96317856060187,136.694275209062));
#256431=CARTESIAN_POINT('Ctrl Pts',(184.768392955261,6.0164979221829,132.336325600291));
#256432=CARTESIAN_POINT('Ctrl Pts',(184.489945331449,4.54094961554151,126.570575013045));
#256433=CARTESIAN_POINT('Ctrl Pts',(184.211497707636,-1.10750955006109,
124.695466564429));
#256434=CARTESIAN_POINT('Ctrl Pts',(183.933050083823,-5.73822154400692,
128.434133314579));
#256435=CARTESIAN_POINT('Ctrl Pts',(183.65460246001,-5.09578826671723,134.350923164133));
#256436=CARTESIAN_POINT('Ctrl Pts',(183.376154836197,0.229425484589131,
137.008595292604));
#256437=CARTESIAN_POINT('Ctrl Pts',(183.097707212384,5.34380842361613,133.964878848429));
#256438=CARTESIAN_POINT('Ctrl Pts',(182.819259588571,5.54749248089459,128.016800549989));
#256439=CARTESIAN_POINT('Ctrl Pts',(182.540811964758,0.653301958305029,
124.630353773773));
#256440=CARTESIAN_POINT('Ctrl Pts',(182.262364340946,-4.84124114839195,
126.917517669999));
#256441=CARTESIAN_POINT('Ctrl Pts',(181.983916717133,-5.88692014749505,
132.776500352206));
#256442=CARTESIAN_POINT('Ctrl Pts',(181.70546909332,-1.52280712308763,136.82318296266));
#256443=CARTESIAN_POINT('Ctrl Pts',(181.427021469507,4.24069125417353,135.33886187379));
#256444=CARTESIAN_POINT('Ctrl Pts',(181.148573845694,6.10720153813428,129.687555653153));
#256445=CARTESIAN_POINT('Ctrl Pts',(180.870126221881,2.36149196193127,125.062538635854));
#256446=CARTESIAN_POINT('Ctrl Pts',(180.591678598068,-3.55431336199069,
125.713975516152));
#256447=CARTESIAN_POINT('Ctrl Pts',(180.313230974255,-6.20387834410407,
131.04322762551));
#256448=CARTESIAN_POINT('Ctrl Pts',(180.034783350442,-3.15238220429199,
136.15297262387));
#256449=CARTESIAN_POINT('Ctrl Pts',(179.75633572663,2.79599917883219,136.347604482659));
#256450=CARTESIAN_POINT('Ctrl Pts',(179.477888102817,6.17499390876314,131.448266031944));
#256451=CARTESIAN_POINT('Ctrl Pts',(179.199440479004,3.8794709017638,125.957209961944));
#256452=CARTESIAN_POINT('Ctrl Pts',(178.920992855191,-1.98109634126673,
124.920448547985));
#256453=CARTESIAN_POINT('Ctrl Pts',(178.642545231378,-6.02113282860982,
129.290714880887));
#256454=CARTESIAN_POINT('Ctrl Pts',(178.364097607565,-4.52804239515191,
135.051947700091));
#256455=CARTESIAN_POINT('Ctrl Pts',(178.085649983752,1.12609779228193,136.909855496619));
#256456=CARTESIAN_POINT('Ctrl Pts',(177.807202359939,5.74540912154417,133.157111769304));
#256457=CARTESIAN_POINT('Ctrl Pts',(177.528754736127,5.08497014694685,127.242304671825));
#256458=CARTESIAN_POINT('Ctrl Pts',(177.250307112313,-0.248307978092709,
124.600852972375));
#256459=CARTESIAN_POINT('Ctrl Pts',(176.971859488501,-5.35340320178418,
127.660121740658));
#256460=CARTESIAN_POINT('Ctrl Pts',(176.693411864688,-5.53898241132168,
133.608792432211));
#256461=CARTESIAN_POINT('Ctrl Pts',(176.414964240875,-0.634507379188621,
136.980327290216));
#256462=CARTESIAN_POINT('Ctrl Pts',(176.136516617062,4.85304893701009,134.676450488799));
#256463=CARTESIAN_POINT('Ctrl Pts',(175.858068993249,5.88089036471739,128.814312257825));
#256464=CARTESIAN_POINT('Ctrl Pts',(175.579621369436,1.50448084471559,124.780931250186));
#256465=CARTESIAN_POINT('Ctrl Pts',(175.301173745623,-4.25447307360455,
126.282787570284));
#256466=CARTESIAN_POINT('Ctrl Pts',(175.02272612181,-6.10377407984646,131.939748629711));
#256467=CARTESIAN_POINT('Ctrl Pts',(174.744278497998,-2.34400489265046,
136.553343572764));
#256468=CARTESIAN_POINT('Ctrl Pts',(174.465830874185,3.56979027988629,135.883904033421));
#256469=CARTESIAN_POINT('Ctrl Pts',(174.187383250372,6.20312257915782,130.546612244398));
#256470=CARTESIAN_POINT('Ctrl Pts',(173.908935626559,3.13608826756835,125.446178618609));
#256471=CARTESIAN_POINT('Ctrl Pts',(173.630488002746,-2.81285795548731,
125.269652488117));
#256472=CARTESIAN_POINT('Ctrl Pts',(173.352040378933,-6.17692513320066,
130.179252743065));
#256473=CARTESIAN_POINT('Ctrl Pts',(173.07359275512,-3.86469987307124,135.663296596462));
#256474=CARTESIAN_POINT('Ctrl Pts',(172.795145131307,1.99899576932572,136.682215657471));
#256475=CARTESIAN_POINT('Ctrl Pts',(172.516697507494,6.02571195608475,132.29967308599));
#256476=CARTESIAN_POINT('Ctrl Pts',(172.238249883681,4.51509322759614,126.543011406101));
#256477=CARTESIAN_POINT('Ctrl Pts',(171.959802259869,-1.14467560248665,
124.702321473066));
#256478=CARTESIAN_POINT('Ctrl Pts',(171.681354636056,-5.75254347439624,
128.469107412642));
#256479=CARTESIAN_POINT('Ctrl Pts',(171.402907012243,-5.07410492070761,
134.38187696408));
#256480=CARTESIAN_POINT('Ctrl Pts',(171.12445938843,0.267188171305193,137.007083764462));
#256481=CARTESIAN_POINT('Ctrl Pts',(170.846011764617,5.36294838675633,133.932291012718));
#256482=CARTESIAN_POINT('Ctrl Pts',(170.567564140804,5.53042102937231,127.983083035723));
#256483=CARTESIAN_POINT('Ctrl Pts',(170.289116516991,0.615706922082464,
124.62649132937));
#256484=CARTESIAN_POINT('Ctrl Pts',(170.010668893178,-4.86481176764585,
126.947059693175));
#256485=CARTESIAN_POINT('Ctrl Pts',(169.732221269365,-5.87480610217478,
132.812299166869));
#256486=CARTESIAN_POINT('Ctrl Pts',(169.453773645553,-1.48614062903852,
136.832341207004));
#256487=CARTESIAN_POINT('Ctrl Pts',(169.17532602174,4.26821548017818,135.312963568669));
#256488=CARTESIAN_POINT('Ctrl Pts',(168.896878397927,6.10029007702938,129.650400075769));
#256489=CARTESIAN_POINT('Ctrl Pts',(168.618430774114,2.32649610882855,125.048269946673));
#256490=CARTESIAN_POINT('Ctrl Pts',(168.339983150301,-3.58523412773234,
125.735705943466));
#256491=CARTESIAN_POINT('Ctrl Pts',(168.061535526488,-6.2023093493314,131.08098796821));
#256492=CARTESIAN_POINT('Ctrl Pts',(167.783087902675,-3.11976527855146,
136.172062971709));
#256493=CARTESIAN_POINT('Ctrl Pts',(167.504640278862,2.82969067421049,136.330481738588));
#256494=CARTESIAN_POINT('Ctrl Pts',(167.22619265505,6.17879913544756,131.410665161273));
#256495=CARTESIAN_POINT('Ctrl Pts',(166.947745031236,3.84989304232704,125.933684327914));
#256496=CARTESIAN_POINT('Ctrl Pts',(166.669297407424,-2.01687667896098,
124.93261705898));
#256497=CARTESIAN_POINT('Ctrl Pts',(166.39084978361,-6.03023526218728,129.327395269766));
#256498=CARTESIAN_POINT('Ctrl Pts',(166.112402159798,-4.50210223283349,
135.079432481411));
#256499=CARTESIAN_POINT('Ctrl Pts',(165.833954535985,1.16324280857304,136.902887499053));
#256500=CARTESIAN_POINT('Ctrl Pts',(165.555506912173,5.75962453647134,133.122094242209));
#256501=CARTESIAN_POINT('Ctrl Pts',(165.277059288359,5.06319268865361,127.2114170119));
#256502=CARTESIAN_POINT('Ctrl Pts',(164.998611664547,-0.286065889322858,
124.602479430144));
#256503=CARTESIAN_POINT('Ctrl Pts',(164.720164040733,-5.37244389010723,
127.692767680889));
#256504=CARTESIAN_POINT('Ctrl Pts',(164.441716416921,-5.52180841435808,
133.642457830674));
#256505=CARTESIAN_POINT('Ctrl Pts',(164.163268793108,-0.596900761151562,
136.984075290369));
#256506=CARTESIAN_POINT('Ctrl Pts',(163.884821169295,4.87652953132996,134.646836861603));
#256507=CARTESIAN_POINT('Ctrl Pts',(163.606373545482,5.86866741623098,128.778550479967));
#256508=CARTESIAN_POINT('Ctrl Pts',(163.327925921669,1.46778664595768,124.771884648456));
#256509=CARTESIAN_POINT('Ctrl Pts',(163.049478297856,-4.28191834658676,
126.308769529723));
#256510=CARTESIAN_POINT('Ctrl Pts',(162.771030674043,-6.09674956195837,
131.976882998882));
#256511=CARTESIAN_POINT('Ctrl Pts',(162.49258305023,-2.30896577266445,136.567505680515));
#256512=CARTESIAN_POINT('Ctrl Pts',(162.214135426418,3.60064476245918,135.862079594585));
#256513=CARTESIAN_POINT('Ctrl Pts',(161.935687802605,6.20143866215845,130.508856852083));
#256514=CARTESIAN_POINT('Ctrl Pts',(161.657240178792,3.10341338845521,125.427187633898));
#256515=CARTESIAN_POINT('Ctrl Pts',(161.378792554979,-2.84649717906582,
125.2868776982));
#256516=CARTESIAN_POINT('Ctrl Pts',(161.100344931166,-6.18061589814333,
130.216865021372));
#256517=CARTESIAN_POINT('Ctrl Pts',(160.821897307353,-3.83505054669964,
135.686732096692));
#256518=CARTESIAN_POINT('Ctrl Pts',(160.54344968354,2.0347389045262,136.6699382998));
#256519=CARTESIAN_POINT('Ctrl Pts',(160.265002059727,6.03470270501411,132.262965162335));
#256520=CARTESIAN_POINT('Ctrl Pts',(159.986554435914,4.48906953121078,126.51560570502));
#256521=CARTESIAN_POINT('Ctrl Pts',(159.708106812101,-1.18179923853688,
124.709402495009));
#256522=CARTESIAN_POINT('Ctrl Pts',(159.429659188289,-5.76665224217155,
128.50416804437));
#256523=CARTESIAN_POINT('Ctrl Pts',(159.151211564475,-5.05223355187421,
134.412698197843));
#256524=CARTESIAN_POINT('Ctrl Pts',(158.872763940663,0.304940957265202,
137.005342392132));
#256525=CARTESIAN_POINT('Ctrl Pts',(158.59431631685,5.38188962387183,133.899587270395));
#256526=CARTESIAN_POINT('Ctrl Pts',(158.315868693037,5.51314464606502,127.949470064936));
#256527=CARTESIAN_POINT('Ctrl Pts',(158.037421069224,0.57808907061355,124.622857808186));
#256528=CARTESIAN_POINT('Ctrl Pts',(157.758973445411,-4.88820211951067,
126.976744650055));
#256529=CARTESIAN_POINT('Ctrl Pts',(157.480525821598,-5.86247436375394,
132.848023576631));
#256530=CARTESIAN_POINT('Ctrl Pts',(157.202078197785,-1.44941906550188,
136.841276082311));
#256531=CARTESIAN_POINT('Ctrl Pts',(156.923630573973,4.29558154588865,135.286898195607));
#256532=CARTESIAN_POINT('Ctrl Pts',(156.645182950159,6.09315256743229,129.613287258817));
#256533=CARTESIAN_POINT('Ctrl Pts',(156.366735326347,2.29141404655692,125.034214551549));
#256534=CARTESIAN_POINT('Ctrl Pts',(156.088287702534,-3.61602204130483,
125.757624191644));
#256535=CARTESIAN_POINT('Ctrl Pts',(155.809840078721,-6.2005105257049,131.11873806038));
#256536=CARTESIAN_POINT('Ctrl Pts',(155.531392454908,-3.08703274876129,
136.190954417361));
#256537=CARTESIAN_POINT('Ctrl Pts',(155.252944831095,2.86327731436015,136.313154222067));
#256538=CARTESIAN_POINT('Ctrl Pts',(154.974497207282,6.18237540445775,131.373041823765));
#256539=CARTESIAN_POINT('Ctrl Pts',(154.696049583469,3.82017252368788,125.910339178587));
#256540=CARTESIAN_POINT('Ctrl Pts',(154.417601959656,-2.05258228054818,
124.945003149591));
#256541=CARTESIAN_POINT('Ctrl Pts',(154.139154335844,-6.03911424317947,
129.364130388138));
#256542=CARTESIAN_POINT('Ctrl Pts',(153.860706712031,-4.47599524346119,
135.106758848372));
#256543=CARTESIAN_POINT('Ctrl Pts',(153.582259088218,1.20034472047403,136.895693518332));
#256544=CARTESIAN_POINT('Ctrl Pts',(153.303811464405,5.77362652639317,133.086990830643));
#256545=CARTESIAN_POINT('Ctrl Pts',(153.025363840592,5.04122761189337,127.180662489822));
#256546=CARTESIAN_POINT('Ctrl Pts',(152.746916216779,-0.323813200276178,
124.604335700902));
#256547=CARTESIAN_POINT('Ctrl Pts',(152.468468592966,-5.39128550054617,
127.725528922339));
#256548=CARTESIAN_POINT('Ctrl Pts',(152.190020969154,-5.5044298047531,133.6760180624));
#256549=CARTESIAN_POINT('Ctrl Pts',(151.91157334534,-0.55927202473736,136.987594298923));
#256550=CARTESIAN_POINT('Ctrl Pts',(151.633125721528,4.89982942405471,134.617080850036));
#256551=CARTESIAN_POINT('Ctrl Pts',(151.354678097715,5.85622700211526,128.742863769248));
#256552=CARTESIAN_POINT('Ctrl Pts',(151.076230473902,1.43103805782584,124.763061582343));
#256553=CARTESIAN_POINT('Ctrl Pts',(150.797782850089,-4.3092049515099,126.334918074943));
#256554=CARTESIAN_POINT('Ctrl Pts',(150.519335226276,-6.0894991267732,132.013973919806));
#256555=CARTESIAN_POINT('Ctrl Pts',(150.240887602463,-2.27384109310269,
136.581454232806));
#256556=CARTESIAN_POINT('Ctrl Pts',(149.96243997865,3.63136582181627,135.840067740113));
#256557=CARTESIAN_POINT('Ctrl Pts',(149.683992354837,6.19952494856889,130.471112409769));
#256558=CARTESIAN_POINT('Ctrl Pts',(149.405544731024,3.0706235112177,125.40839590231));
#256559=CARTESIAN_POINT('Ctrl Pts',(149.127097107212,-2.88003092464457,
125.30430736064));
#256560=CARTESIAN_POINT('Ctrl Pts',(148.848649483398,-6.18407763809098,
130.254499069545));
#256561=CARTESIAN_POINT('Ctrl Pts',(148.570201859586,-3.80525911111971,
135.709986678852));
#256562=CARTESIAN_POINT('Ctrl Pts',(148.291754235773,2.07040664172831,136.657443590992));
#256563=CARTESIAN_POINT('Ctrl Pts',(148.01330661196,6.04346983581547,132.226203189553));
#256564=CARTESIAN_POINT('Ctrl Pts',(147.734858988147,4.46287949070312,126.488358925329));
#256565=CARTESIAN_POINT('Ctrl Pts',(147.456411364334,-1.21887908258166,
124.716709367866));
#256566=CARTESIAN_POINT('Ctrl Pts',(147.177963740522,-5.78054732452736,
128.53931391058));
#256567=CARTESIAN_POINT('Ctrl Pts',(146.899516116708,-5.03017497066859,
134.44338572333));
#256568=CARTESIAN_POINT('Ctrl Pts',(146.621068492896,0.342682443525903,
137.003371240143));
#256569=CARTESIAN_POINT('Ctrl Pts',(146.342620869082,5.40063143308812,133.866768833311));
#256570=CARTESIAN_POINT('Ctrl Pts',(146.06417324527,5.49566397115542,127.915962883168));
#256571=CARTESIAN_POINT('Ctrl Pts',(145.785725621457,0.540449797841529,
124.619453344862));
#256572=CARTESIAN_POINT('Ctrl Pts',(145.507277997644,-4.91141133724831,
127.006571440652));
#256573=CARTESIAN_POINT('Ctrl Pts',(145.228830373831,-5.84992538918966,
132.883672257711));
#256574=CARTESIAN_POINT('Ctrl Pts',(144.950382750018,-1.41264379320865,
136.849987257496));
#256575=CARTESIAN_POINT('Ctrl Pts',(144.671935126205,4.32278843724517,135.260666720466));
#256576=CARTESIAN_POINT('Ctrl Pts',(144.393487502392,6.08578927382608,129.576218577526));
#256577=CARTESIAN_POINT('Ctrl Pts',(144.11503987858,2.25624707509518,125.020372971309));
#256578=CARTESIAN_POINT('Ctrl Pts',(143.836592254767,-3.64667596185081,
125.779729448496));
#256579=CARTESIAN_POINT('Ctrl Pts',(143.558144630954,-6.19848193988065,
131.156476503179));
#256580=CARTESIAN_POINT('Ctrl Pts',(143.279697007141,-3.05418582783736,
136.209646260801));
#256581=CARTESIAN_POINT('Ctrl Pts',(143.001249383328,2.89675785471595,136.295622575173));
#256582=CARTESIAN_POINT('Ctrl Pts',(142.722801759515,6.18572258327378,131.335397413564));
#256583=CARTESIAN_POINT('Ctrl Pts',(142.444354135702,3.79031044715096,125.887175379022));
#256584=CARTESIAN_POINT('Ctrl Pts',(142.165906511889,-2.0882118229442,124.957606360848));
#256585=CARTESIAN_POINT('Ctrl Pts',(141.887458888076,-6.04776944257254,
129.400918874772));
#256586=CARTESIAN_POINT('Ctrl Pts',(141.609011264264,-4.44972239443904,
135.133925788383));
#256587=CARTESIAN_POINT('Ctrl Pts',(141.33056364045,1.2374021531599,136.888273821029));
#256588=CARTESIAN_POINT('Ctrl Pts',(141.052116016638,5.78741457246075,133.051802835376));
#256589=CARTESIAN_POINT('Ctrl Pts',(140.773668392825,5.01907573059014,127.15004224521));
#256590=CARTESIAN_POINT('Ctrl Pts',(140.495220769012,-0.361548512212229,
124.606421715863));
#256591=CARTESIAN_POINT('Ctrl Pts',(140.216773145199,-5.4099273349182,127.758404251031));
#256592=CARTESIAN_POINT('Ctrl Pts',(139.938325521386,-5.48684722647749,
133.709471883804));
#256593=CARTESIAN_POINT('Ctrl Pts',(139.659877897573,-0.521622564292735,
136.990884185479));
#256594=CARTESIAN_POINT('Ctrl Pts',(139.38143027376,4.92294775179823,134.58718355672));
#256595=CARTESIAN_POINT('Ctrl Pts',(139.102982649947,5.84356958335437,128.707253448052));
#256596=CARTESIAN_POINT('Ctrl Pts',(138.824535026135,1.39423644205237,124.754462378786));
#256597=CARTESIAN_POINT('Ctrl Pts',(138.546087402322,-4.33633187725888,
126.361232236999));
#256598=CARTESIAN_POINT('Ctrl Pts',(138.267639778509,-6.08202304295846,
132.051020018064));
#256599=CARTESIAN_POINT('Ctrl Pts',(137.989192154696,-2.23863215552307,
136.595188712768));
#256600=CARTESIAN_POINT('Ctrl Pts',(137.710744530883,3.66195231957746,135.817869285661));
#256601=CARTESIAN_POINT('Ctrl Pts',(137.43229690707,6.19738150930245,130.433380316089));
#256602=CARTESIAN_POINT('Ctrl Pts',(137.153849283257,3.03771985089675,125.389804120178));
#256603=CARTESIAN_POINT('Ctrl Pts',(136.875401659444,-2.91345794961824,
125.321940829576));
#256604=CARTESIAN_POINT('Ctrl Pts',(136.596954035631,-6.1873102247676,130.29215349304));
#256605=CARTESIAN_POINT('Ctrl Pts',(136.318506411819,-3.77532667026395,
135.733059481234));
#256606=CARTESIAN_POINT('Ctrl Pts',(136.040058788006,2.10599765925102,136.644731994041));
#256607=CARTESIAN_POINT('Ctrl Pts',(135.761611164193,6.05201302361958,132.189388529871));
#256608=CARTESIAN_POINT('Ctrl Pts',(135.48316354038,4.4365240765547,126.461272076668));
#256609=CARTESIAN_POINT('Ctrl Pts',(135.204715916567,-1.25591376061384,
124.724241820878));
#256610=CARTESIAN_POINT('Ctrl Pts',(134.926268292754,-5.79422820657625,
128.574543708929));
#256611=CARTESIAN_POINT('Ctrl Pts',(134.647820668941,-5.00792999447956,
134.473938403405));
#256612=CARTESIAN_POINT('Ctrl Pts',(134.369373045128,0.380411231562576,
137.001170381535));
#256613=CARTESIAN_POINT('Ctrl Pts',(134.090925421316,5.41917311992063,133.833836917565));
#256614=CARTESIAN_POINT('Ctrl Pts',(133.812477797503,5.4779796523963,127.88256273204));
#256615=CARTESIAN_POINT('Ctrl Pts',(133.53403017369,0.502790498503515,124.616278065551));
#256616=CARTESIAN_POINT('Ctrl Pts',(133.255582549877,-4.93443856083268,
127.036538959725));
#256617=CARTESIAN_POINT('Ctrl Pts',(132.977134926064,-5.83715964348875,
132.919243889133));
#256618=CARTESIAN_POINT('Ctrl Pts',(132.698687302251,-1.37581617488021,
136.858474409763));
#256619=CARTESIAN_POINT('Ctrl Pts',(132.420239678438,4.34983514608645,135.234270115264));
#256620=CARTESIAN_POINT('Ctrl Pts',(132.141792054625,6.07820046906025,129.539195405491));
#256621=CARTESIAN_POINT('Ctrl Pts',(131.863344430812,2.22099649756843,125.006745718858));
#256622=CARTESIAN_POINT('Ctrl Pts',(131.584896806999,-3.67719475347803,
125.802020894903));
#256623=CARTESIAN_POINT('Ctrl Pts',(131.306449183186,-6.1962236670286,131.194201898194));
#256624=CARTESIAN_POINT('Ctrl Pts',(131.028001559374,-3.02122573293442,
136.228137809392));
#256625=CARTESIAN_POINT('Ctrl Pts',(130.749553935561,2.93013105464412,136.277887447547));
#256626=CARTESIAN_POINT('Ctrl Pts',(130.471106311748,6.18884054786473,131.2977333256));
#256627=CARTESIAN_POINT('Ctrl Pts',(130.192658687935,3.76030791926647,125.864193787566));
#256628=CARTESIAN_POINT('Ctrl Pts',(129.914211064122,-2.12376398588317,
124.970426225734));
#256629=CARTESIAN_POINT('Ctrl Pts',(129.635763440309,-6.05620053964477,
129.437759366456));
#256630=CARTESIAN_POINT('Ctrl Pts',(129.357315816496,-4.42328465931731,
135.160932294765));
#256631=CARTESIAN_POINT('Ctrl Pts',(129.078868192683,1.27441373345414,136.880628682086));
#256632=CARTESIAN_POINT('Ctrl Pts',(128.800420568871,5.80098816375315,133.01653156031));
#256633=CARTESIAN_POINT('Ctrl Pts',(128.521972945058,4.99673786558976,127.11955741271));
#256634=CARTESIAN_POINT('Ctrl Pts',(128.243525321245,-0.399270426835251,
124.608737397728));
#256635=CARTESIAN_POINT('Ctrl Pts',(127.965077697432,-5.42836870244348,
127.791392448756));
#256636=CARTESIAN_POINT('Ctrl Pts',(127.686630073619,-5.46906133106002,
133.742818055242));
#256637=CARTESIAN_POINT('Ctrl Pts',(127.408182449806,-0.483953774931917,
136.993944828129));
#256638=CARTESIAN_POINT('Ctrl Pts',(127.129734825993,4.9458836579024,134.557146089508));
#256639=CARTESIAN_POINT('Ctrl Pts',(126.85128720218,5.8306956289736,128.671720835934));
#256640=CARTESIAN_POINT('Ctrl Pts',(126.572839578367,1.35738316233494,124.746087356435));
#256641=CARTESIAN_POINT('Ctrl Pts',(126.294391954555,-4.36329811863544,
126.387711040812));
#256642=CARTESIAN_POINT('Ctrl Pts',(126.015944330741,-6.07432158754323,
132.088019920899));
#256643=CARTESIAN_POINT('Ctrl Pts',(125.737496706929,-2.20334026460562,
136.608708611466));
#256644=CARTESIAN_POINT('Ctrl Pts',(125.459049083116,3.69240312234872,135.795485053802));
#256645=CARTESIAN_POINT('Ctrl Pts',(125.180601459303,6.19500842378515,130.39566196922));
#256646=CARTESIAN_POINT('Ctrl Pts',(124.90215383549,3.00470362674961,125.371412976429));
#256647=CARTESIAN_POINT('Ctrl Pts',(124.623706211677,-2.9467770153362,125.339777451594));
#256648=CARTESIAN_POINT('Ctrl Pts',(124.345258587864,-6.19031353838844,
130.329826896558));
#256649=CARTESIAN_POINT('Ctrl Pts',(124.066810964051,-3.74525433329013,
135.755949648866));
#256650=CARTESIAN_POINT('Ctrl Pts',(123.788363340238,2.14151063825588,136.631803979981));
#256651=CARTESIAN_POINT('Ctrl Pts',(123.509915716426,6.0603319518555,132.152522547471));
#256652=CARTESIAN_POINT('Ctrl Pts',(123.231468092613,4.4100042653751,126.43434616275));
#256653=CARTESIAN_POINT('Ctrl Pts',(122.9530204688,-1.29290190029971,124.731999574929));
#256654=CARTESIAN_POINT('Ctrl Pts',(122.674572844987,-5.80769438136815,
128.609856133963));
#256655=CARTESIAN_POINT('Ctrl Pts',(122.396125221174,-4.98549944760296,
134.504355105923));
#256656=CARTESIAN_POINT('Ctrl Pts',(122.117677597361,0.418125923321227,
136.998739897863));
#256657=CARTESIAN_POINT('Ctrl Pts',(121.839229973548,5.43751399730024,133.80079274346));
#256658=CARTESIAN_POINT('Ctrl Pts',(121.560782349735,5.46009234508668,127.849270849208));
#256659=CARTESIAN_POINT('Ctrl Pts',(121.282334725922,0.465112568078527,
124.613332087916));
#256660=CARTESIAN_POINT('Ctrl Pts',(121.00388710211,-4.95728293698158,127.066646096814));
#256661=CARTESIAN_POINT('Ctrl Pts',(120.725439478297,-5.82417759969065,
132.954737152777));
#256662=CARTESIAN_POINT('Ctrl Pts',(120.446991854484,-1.33893757517749,
136.866737224615));
#256663=CARTESIAN_POINT('Ctrl Pts',(120.168544230671,4.37672067018674,135.207709358136));
#256664=CARTESIAN_POINT('Ctrl Pts',(119.890096606858,6.07038643434081,129.502219114618));
#256665=CARTESIAN_POINT('Ctrl Pts',(119.611648983045,2.18566362019961,124.993333299159));
#256666=CARTESIAN_POINT('Ctrl Pts',(119.333201359232,-3.7075772853013,125.82449770485));
#256667=CARTESIAN_POINT('Ctrl Pts',(119.054753735419,-6.19373579082994,
131.231912847497));
#256668=CARTESIAN_POINT('Ctrl Pts',(118.776306111606,-2.98815368540088,
136.246428377926));
#256669=CARTESIAN_POINT('Ctrl Pts',(118.497858487794,2.96339567748857,136.259949496373));
#256670=CARTESIAN_POINT('Ctrl Pts',(118.219410863981,6.1917291826932,131.26005095553));
#256671=CARTESIAN_POINT('Ctrl Pts',(117.940963240168,3.73016605178927,125.841395255808));
#256672=CARTESIAN_POINT('Ctrl Pts',(117.662515616355,-2.15923745196658,
124.983462269205));
#256673=CARTESIAN_POINT('Ctrl Pts',(117.384067992542,-6.06440722197891,
129.474650498052));
#256674=CARTESIAN_POINT('Ctrl Pts',(117.105620368729,-4.39668301775581,
135.187777366781));
#256675=CARTESIAN_POINT('Ctrl Pts',(116.827172744916,1.31137808987868,136.872758384795));
#256676=CARTESIAN_POINT('Ctrl Pts',(116.548725121103,5.81434679729579,132.981178312436));
#256677=CARTESIAN_POINT('Ctrl Pts',(116.27027749729,4.97421484463032,127.089209121948));
#256678=CARTESIAN_POINT('Ctrl Pts',(115.991829873478,-0.436977546345769,
124.611282660692));
#256679=CARTESIAN_POINT('Ctrl Pts',(115.713382249665,-5.44660891977013,
127.824492293124));
#256680=CARTESIAN_POINT('Ctrl Pts',(115.434934625852,-5.45107277756375,
133.776055341058));
#256681=CARTESIAN_POINT('Ctrl Pts',(115.156487002039,-0.446267052485976,
136.99677611346));
#256682=CARTESIAN_POINT('Ctrl Pts',(114.878039378226,4.9686362924688,134.526969561451));
#256683=CARTESIAN_POINT('Ctrl Pts',(114.599591754413,5.81760561602206,128.636267249567));
#256684=CARTESIAN_POINT('Ctrl Pts',(114.3211441306,1.32047958428524,124.737936825626));
#256685=CARTESIAN_POINT('Ctrl Pts',(114.042696506787,-4.39010267639563,
126.414353505198));
#256686=CARTESIAN_POINT('Ctrl Pts',(113.764248882975,-6.06639504590774,
132.124972257267));
#256687=CARTESIAN_POINT('Ctrl Pts',(113.485801259161,-2.16796672810439,
136.622013427915));
#256688=CARTESIAN_POINT('Ctrl Pts',(113.207353635349,3.72271710176439,135.772915873991));
#256689=CARTESIAN_POINT('Ctrl Pts',(112.928906011536,6.19240577995249,130.357958766832));
#256690=CARTESIAN_POINT('Ctrl Pts',(112.650458387723,2.97157606220462,125.353223152553));
#256691=CARTESIAN_POINT('Ctrl Pts',(112.37201076391,-2.9799868871482,125.357816565752));
#256692=CARTESIAN_POINT('Ctrl Pts',(112.093563140097,-6.19308746766462,
130.367517884098));
#256693=CARTESIAN_POINT('Ctrl Pts',(111.815115516284,-3.71504321453968,
135.778656333547));
#256694=CARTESIAN_POINT('Ctrl Pts',(111.536667892471,2.1769442627965,136.618660027865));
#256695=CARTESIAN_POINT('Ctrl Pts',(111.258220268658,6.06842631226225,132.115606608435));
#256696=CARTESIAN_POINT('Ctrl Pts',(110.979772644846,4.38332103986566,126.407582181323));
#256697=CARTESIAN_POINT('Ctrl Pts',(110.701325021032,-1.32984213103019,
124.739982342551));
#256698=CARTESIAN_POINT('Ctrl Pts',(110.42287739722,-5.82094534990898,128.645249877167));
#256699=CARTESIAN_POINT('Ctrl Pts',(110.144429773407,-4.96288416121089,
134.534634703787));
#256700=CARTESIAN_POINT('Ctrl Pts',(109.865982149594,0.455825121270016,
136.996079879188));
#256701=CARTESIAN_POINT('Ctrl Pts',(109.587534525781,5.45565338559904,133.767637535461));
#256702=CARTESIAN_POINT('Ctrl Pts',(109.309086901968,5.44200271204727,127.816088468313));
#256703=CARTESIAN_POINT('Ctrl Pts',(109.030639278155,0.427417402736423,
124.610615521118));
#256704=CARTESIAN_POINT('Ctrl Pts',(108.752191654342,-4.97994361918818,
127.096891736289));
#256705=CARTESIAN_POINT('Ctrl Pts',(108.473744030529,-5.81097973884976,
132.990150733429));
#256706=CARTESIAN_POINT('Ctrl Pts',(108.195296406717,-1.30200936065053,
136.874775395874));
#256707=CARTESIAN_POINT('Ctrl Pts',(107.916848782904,4.40344401329306,135.180985433302));
#256708=CARTESIAN_POINT('Ctrl Pts',(107.638401159091,6.06234745921968,129.465291075077));
#256709=CARTESIAN_POINT('Ctrl Pts',(107.359953535278,2.15024975226158,124.980136209215));
#256710=CARTESIAN_POINT('Ctrl Pts',(107.081505911465,-3.73782243148481,
125.847159045447));
#256711=CARTESIAN_POINT('Ctrl Pts',(106.803058287652,-6.19101840347381,
131.269607953695));
#256712=CARTESIAN_POINT('Ctrl Pts',(106.524610663839,-2.95497091073364,
136.264517288637));
#256713=CARTESIAN_POINT('Ctrl Pts',(106.246163040026,2.99655049061638,136.241809386346));
#256714=CARTESIAN_POINT('Ctrl Pts',(105.967715416213,6.1943883807198,131.222351699685));
#256715=CARTESIAN_POINT('Ctrl Pts',(105.689267792401,3.69988596163724,125.818780628557));
#256716=CARTESIAN_POINT('Ctrl Pts',(105.410820168588,-2.19463090671215,
124.996714008204));
#256717=CARTESIAN_POINT('Ctrl Pts',(105.132372544775,-6.07238918547325,
129.511590902545));
#256718=CARTESIAN_POINT('Ctrl Pts',(104.853924920962,-4.36991845548819,
135.214460009678));
#256719=CARTESIAN_POINT('Ctrl Pts',(104.575477297149,1.34829385270585,136.864663220793));
#256720=CARTESIAN_POINT('Ctrl Pts',(104.297029673336,5.82748997807964,132.945744401783));
#256721=CARTESIAN_POINT('Ctrl Pts',(104.018582049523,4.95150750231056,127.058998497491));
#256722=CARTESIAN_POINT('Ctrl Pts',(103.74013442571,-0.474668473492613,
124.614057410436));
#256723=CARTESIAN_POINT('Ctrl Pts',(103.461686801897,-5.46464731100027,
127.857702557609));
#256724=CARTESIAN_POINT('Ctrl Pts',(103.183239178085,-5.43288223256107,
133.809182509633));
#256725=CARTESIAN_POINT('Ctrl Pts',(102.904791554272,-0.408563793450433,
136.999377936557));
#256726=CARTESIAN_POINT('Ctrl Pts',(102.626343930459,4.99120481239017,134.496655090749));
#256727=CARTESIAN_POINT('Ctrl Pts',(102.347896306646,5.80430002955499,128.600894002697));
#256728=CARTESIAN_POINT('Ctrl Pts',(102.069448682833,1.28352707537895,124.730011088381));
#256729=CARTESIAN_POINT('Ctrl Pts',(101.79100105902,-4.41674455728669,126.441158642913));
#256730=CARTESIAN_POINT('Ctrl Pts',(101.512553435207,-6.05824371177293,
132.161875657885));
#256731=CARTESIAN_POINT('Ctrl Pts',(101.234105811394,-2.13251285679878,
136.635102669099));
#256732=CARTESIAN_POINT('Ctrl Pts',(100.955658187581,3.75289313452884,135.750162582539));
#256733=CARTESIAN_POINT('Ctrl Pts',(100.677210563769,6.18957367424645,130.320272106026));
#256734=CARTESIAN_POINT('Ctrl Pts',(100.398762939956,2.93833838481571,125.33523532258));
#256735=CARTESIAN_POINT('Ctrl Pts',(100.120315316143,-3.01308633445025,
125.376057503601));
#256736=CARTESIAN_POINT('Ctrl Pts',(99.8418676923298,-6.19563190980719,
130.405225059005));
#256737=CARTESIAN_POINT('Ctrl Pts',(99.5634200685172,-3.68469443349671,
135.801178693871));
#256738=CARTESIAN_POINT('Ctrl Pts',(99.2849724447041,2.2122972198669,136.605300624745));
#256739=CARTESIAN_POINT('Ctrl Pts',(99.0065248208913,6.07629580490035,132.078642080696));
#256740=CARTESIAN_POINT('Ctrl Pts',(98.7280771970783,4.35647538878314,126.380981124141));
#256741=CARTESIAN_POINT('Ctrl Pts',(98.4496295732656,-1.36673308397146,
124.748189827941));
#256742=CARTESIAN_POINT('Ctrl Pts',(98.1711819494526,-5.8339806211792,128.680723627015));
#256743=CARTESIAN_POINT('Ctrl Pts',(97.8927343256397,-4.94008497332115,
134.564776074971));
#256744=CARTESIAN_POINT('Ctrl Pts',(97.6142867018267,0.493507428451318,
136.993190424079));
#256745=CARTESIAN_POINT('Ctrl Pts',(97.3358390780141,5.47359061265531,133.734372522146));
#256746=CARTESIAN_POINT('Ctrl Pts',(97.0573914542009,5.42371142359607,127.783016818942));
#256747=CARTESIAN_POINT('Ctrl Pts',(96.7789438303882,0.389706399285272,
124.608128465823));
#256748=CARTESIAN_POINT('Ctrl Pts',(96.5004962065753,-5.0024197677526,127.127274757387));
#256749=CARTESIAN_POINT('Ctrl Pts',(96.2220485827623,-5.79756655001767,
133.025483318824));
#256750=CARTESIAN_POINT('Ctrl Pts',(95.9436009589496,-1.26503289968789,
136.882588625681));
#256751=CARTESIAN_POINT('Ctrl Pts',(95.6651533351365,4.4300041851621,135.154099331026));
#256752=CARTESIAN_POINT('Ctrl Pts',(95.3867057113237,6.05408384158403,129.428412655251));
#256753=CARTESIAN_POINT('Ctrl Pts',(95.1082580875108,2.11475620602821,124.967154938047));
#256754=CARTESIAN_POINT('Ctrl Pts',(94.8298104636979,-3.76792907128354,
125.870004076972));
#256755=CARTESIAN_POINT('Ctrl Pts',(94.5513628398851,-6.18807160565406,
131.307285819983));
#256756=CARTESIAN_POINT('Ctrl Pts',(94.2729152160721,-2.92167863853249,
136.282403871234));
#256757=CARTESIAN_POINT('Ctrl Pts',(93.9944675922592,3.02959426546386,136.223467789656));
#256758=CARTESIAN_POINT('Ctrl Pts',(93.7160199684464,6.19681804340696,131.184636955029));
#256759=CARTESIAN_POINT('Ctrl Pts',(93.4375723446334,3.66946877085029,125.796350743805));
#256760=CARTESIAN_POINT('Ctrl Pts',(93.1591247208205,-2.22994303860241,
125.010180951684));
#256761=CARTESIAN_POINT('Ctrl Pts',(92.8806770970077,-6.08014613435319,
129.548579211095));
#256762=CARTESIAN_POINT('Ctrl Pts',(92.6022294731947,-4.3429919642852,135.24097923472));
#256763=CARTESIAN_POINT('Ctrl Pts',(92.323781849382,1.38515965400848,136.856343490049));
#256764=CARTESIAN_POINT('Ctrl Pts',(92.045334225569,5.84041721907928,132.910231141365));
#256765=CARTESIAN_POINT('Ctrl Pts',(91.7668866017561,4.9286166800594,127.028926658805));
#256766=CARTESIAN_POINT('Ctrl Pts',(91.4884389779432,-0.512341811624615,
124.617061544141));
#256767=CARTESIAN_POINT('Ctrl Pts',(91.2099913541303,-5.48248320771468,
127.891022011592));
#256768=CARTESIAN_POINT('Ctrl Pts',(90.9315437303175,-5.41449037010934,
133.842198333429));
#256769=CARTESIAN_POINT('Ctrl Pts',(90.6530961065044,-0.370845394933272,
137.00175020101));
#256770=CARTESIAN_POINT('Ctrl Pts',(90.3746484826917,5.01358838138169,134.466203800718));
#256771=CARTESIAN_POINT('Ctrl Pts',(90.0962008588786,5.79077936261581,128.565602406094));
#256772=CARTESIAN_POINT('Ctrl Pts',(89.817753235066,1.24652700490487,124.722310438393));
#256773=CARTESIAN_POINT('Ctrl Pts',(89.5393056112528,-4.44322277408392,
126.468125460682));
#256774=CARTESIAN_POINT('Ctrl Pts',(89.2608579874402,-6.04986788718945,
132.198728755283));
#256775=CARTESIAN_POINT('Ctrl Pts',(88.9824103636271,-2.09697996444503,
136.647975849991));
#256776=CARTESIAN_POINT('Ctrl Pts',(88.7039627398144,3.78293010245805,135.727226022576));
#256777=CARTESIAN_POINT('Ctrl Pts',(88.4255151160013,6.18651221161165,130.282603383299));
#256778=CARTESIAN_POINT('Ctrl Pts',(88.1470674921886,2.9049918262175,125.317450153056));
#256779=CARTESIAN_POINT('Ctrl Pts',(87.8686198683756,-3.04607413073006,
125.394499589218));
#256780=CARTESIAN_POINT('Ctrl Pts',(87.5901722445627,-6.19794677053091,
130.442947024027));
#256781=CARTESIAN_POINT('Ctrl Pts',(87.3117246207499,-3.65420911474647,
135.823515895262));
#256782=CARTESIAN_POINT('Ctrl Pts',(87.033276996937,2.24756819945024,136.59172626566));
#256783=CARTESIAN_POINT('Ctrl Pts',(86.754829373124,6.08394013816284,132.041630333989));
#256784=CARTESIAN_POINT('Ctrl Pts',(86.4763817493112,4.32946830690299,126.35454397691));
#256785=CARTESIAN_POINT('Ctrl Pts',(86.1979341254982,-1.40357339211569,
124.756621726966));
#256786=CARTESIAN_POINT('Ctrl Pts',(85.9194865016854,-5.84679971215209,
128.716276069012));
#256787=CARTESIAN_POINT('Ctrl Pts',(85.6410388778725,-4.91710272876601,
134.594778102578));
#256788=CARTESIAN_POINT('Ctrl Pts',(85.3625912540596,0.531171448533366,
136.990071639606));
#256789=CARTESIAN_POINT('Ctrl Pts',(85.0841436302467,5.49132501379855,133.700998936161));
#256790=CARTESIAN_POINT('Ctrl Pts',(84.8056960064338,5.4052191575235,127.750057126576));
#256791=CARTESIAN_POINT('Ctrl Pts',(84.527248382621,0.351980955120191,124.60587101419));
#256792=CARTESIAN_POINT('Ctrl Pts',(84.2488007588079,-5.02471054981291,
127.157794034254));
#256793=CARTESIAN_POINT('Ctrl Pts',(83.9703531349953,-5.78393853022499,
133.0607335997));
#256794=CARTESIAN_POINT('Ctrl Pts',(83.6919055111822,-1.22800956246596,
136.890176624513));
#256795=CARTESIAN_POINT('Ctrl Pts',(83.4134578873695,4.45640020159694,135.127052047582));
#256796=CARTESIAN_POINT('Ctrl Pts',(83.1350102635564,6.04559588764522,129.391585221682));
#256797=CARTESIAN_POINT('Ctrl Pts',(82.8565626397436,2.07918429672594,124.954389966684));
#256798=CARTESIAN_POINT('Ctrl Pts',(82.5781150159307,-3.79789608908488,
125.893031952893));
#256799=CARTESIAN_POINT('Ctrl Pts',(82.2996673921181,-6.18489550656524,
131.344945050191));
#256800=CARTESIAN_POINT('Ctrl Pts',(82.0212197683047,-2.88827810245507,
136.300087462925));
#256801=CARTESIAN_POINT('Ctrl Pts',(81.7427721444922,3.06252577758164,136.204925385956));
#256802=CARTESIAN_POINT('Ctrl Pts',(81.464324520679,6.19901808072266,131.146908119091));
#256803=CARTESIAN_POINT('Ctrl Pts',(81.1858768968663,3.6389156065486,125.774106432701));
#256804=CARTESIAN_POINT('Ctrl Pts',(80.9074292730533,-2.26517253913331,
125.023862600622));
#256805=CARTESIAN_POINT('Ctrl Pts',(80.6289816492404,-6.08767778118217,
129.585614053086));
#256806=CARTESIAN_POINT('Ctrl Pts',(80.3505340254275,-4.31590454191782,
135.267334059228));
#256807=CARTESIAN_POINT('Ctrl Pts',(80.0720864016147,1.42197412771073,136.847799500855));
#256808=CARTESIAN_POINT('Ctrl Pts',(79.7936387778018,5.85312804127117,132.874639847142));
#256809=CARTESIAN_POINT('Ctrl Pts',(79.5151911539889,4.90554322610457,126.998994720211));
#256810=CARTESIAN_POINT('Ctrl Pts',(79.236743530176,-0.54999616474248,124.62029495049));
#256811=CARTESIAN_POINT('Ctrl Pts',(78.9582959063631,-5.50011594899764,
127.924449420408));
#256812=CARTESIAN_POINT('Ctrl Pts',(78.6798482825503,-5.39589787172579,
133.87510158903));
#256813=CARTESIAN_POINT('Ctrl Pts',(78.4014006587372,-0.333113254603616,
137.003892818912));
#256814=CARTESIAN_POINT('Ctrl Pts',(78.1229530349246,5.035786170012,134.435616819741));
#256815=CARTESIAN_POINT('Ctrl Pts',(77.8445054111114,5.77704411621779,128.530393767498));
#256816=CARTESIAN_POINT('Ctrl Pts',(77.5660577872988,1.20948074391421,124.71483516101));
#256817=CARTESIAN_POINT('Ctrl Pts',(77.2876101634857,-4.46953634562727,
126.49525295924));
#256818=CARTESIAN_POINT('Ctrl Pts',(77.009162539673,-6.04126788252658,132.235530183857));
#256819=CARTESIAN_POINT('Ctrl Pts',(76.73071491586,-2.06136936772754,136.660632493573));
#256820=CARTESIAN_POINT('Ctrl Pts',(76.4522672920471,3.81282689252116,135.704107044024));
#256821=CARTESIAN_POINT('Ctrl Pts',(76.1738196682342,6.18322150549176,130.244953994479));
#256822=CARTESIAN_POINT('Ctrl Pts',(75.8953720444213,2.87153762207887,125.299868303017));
#256823=CARTESIAN_POINT('Ctrl Pts',(75.6169244206085,-3.07894905361277,
125.413142139227));
#256824=CARTESIAN_POINT('Ctrl Pts',(75.3384767967955,-6.20003196405775,
130.480682381363));
#256825=CARTESIAN_POINT('Ctrl Pts',(75.0600291729826,-3.62358838793365,
135.84566711001));
#256826=CARTESIAN_POINT('Ctrl Pts',(74.7815815491698,2.28275589456742,136.577937453613));
#256827=CARTESIAN_POINT('Ctrl Pts',(74.5031339253568,6.09135902878616,132.004572739798));
#256828=CARTESIAN_POINT('Ctrl Pts',(74.224686301544,4.30230079498258,126.328271719272));
#256829=CARTESIAN_POINT('Ctrl Pts',(73.946238677731,-1.44036169033171,124.76527772718));
#256830=CARTESIAN_POINT('Ctrl Pts',(73.6677910539182,-5.85940214781156,
128.75190588575));
#256831=CARTESIAN_POINT('Ctrl Pts',(73.3893434301052,-4.89393827916089,
134.624639674871));
#256832=CARTESIAN_POINT('Ctrl Pts',(73.1108958062924,0.56881578586215,136.986723641335));
#256833=CARTESIAN_POINT('Ctrl Pts',(72.8324481824796,5.50885593187395,133.66751801418));
#256834=CARTESIAN_POINT('Ctrl Pts',(72.5540005586665,5.38652659906729,127.717210612549));
#256835=CARTESIAN_POINT('Ctrl Pts',(72.2755529348538,0.314242468171368,
124.603843249867));
#256836=CARTESIAN_POINT('Ctrl Pts',(71.9971053110409,-5.04681513937595,
127.188448435987));
#256837=CARTESIAN_POINT('Ctrl Pts',(71.7186576872279,-5.77009618446306,
133.095900269846));
#256838=CARTESIAN_POINT('Ctrl Pts',(71.4402100634152,-1.19094072089807,
136.897539111196));
#256839=CARTESIAN_POINT('Ctrl Pts',(71.1617624396021,4.48263108448347,135.099844585217));
#256840=CARTESIAN_POINT('Ctrl Pts',(70.8833148157894,6.03688391192757,129.354810139024));
#256841=CARTESIAN_POINT('Ctrl Pts',(70.6048671919763,2.04353534248492,124.941841768133));
#256842=CARTESIAN_POINT('Ctrl Pts',(70.3264195681636,-3.82772237444985,
125.916241819903));
#256843=CARTESIAN_POINT('Ctrl Pts',(70.0479719443506,-6.18149022389895,
131.382584248845));
#256844=CARTESIAN_POINT('Ctrl Pts',(69.7695243205378,-2.85477054017052,
136.317567408437));
#256845=CARTESIAN_POINT('Ctrl Pts',(69.4910766967249,3.09534380668036,136.186182862342));
#256846=CARTESIAN_POINT('Ctrl Pts',(69.2126290729119,6.20098841114368,131.109166589932));
#256847=CARTESIAN_POINT('Ctrl Pts',(68.934181449099,3.60822760089105,125.752048519516));
#256848=CARTESIAN_POINT('Ctrl Pts',(68.6557338252862,-2.30031810286251,
125.037758448041));
#256849=CARTESIAN_POINT('Ctrl Pts',(68.3772862014732,-6.09498384687224,
129.622694056181));
#256850=CARTESIAN_POINT('Ctrl Pts',(68.0988385776604,-4.28865719212064,
135.293523506613));
#256851=CARTESIAN_POINT('Ctrl Pts',(67.8203909538475,1.45873590963839,136.83903156981));
#256852=CARTESIAN_POINT('Ctrl Pts',(67.5419433300346,5.86562197365073,132.83897183796));
#256853=CARTESIAN_POINT('Ctrl Pts',(67.2634957062218,4.88228799544191,126.969203790852));
#256854=CARTESIAN_POINT('Ctrl Pts',(66.9850480824087,-0.587630137549865,
124.623757509667));
#256855=CARTESIAN_POINT('Ctrl Pts',(66.706600458596,-5.51754488146136,127.957983545393));
#256856=CARTESIAN_POINT('Ctrl Pts',(66.428152834783,-5.37710542636232,133.907891057196));
#256857=CARTESIAN_POINT('Ctrl Pts',(66.1497052109702,-0.295368770640213,
137.00580571087));
#256858=CARTESIAN_POINT('Ctrl Pts',(65.8712575871573,5.05779735573374,134.404895281231));
#256859=CARTESIAN_POINT('Ctrl Pts',(65.5928099633443,5.76309479932555,128.495269391582));
#256860=CARTESIAN_POINT('Ctrl Pts',(65.3143623395316,1.17238966517029,124.707585533234));
#256861=CARTESIAN_POINT('Ctrl Pts',(65.0359147157185,-4.49568429685739,
126.522540133366));
#256862=CARTESIAN_POINT('Ctrl Pts',(64.7574670919057,-6.03244401646077,
132.272278579917));
#256863=CARTESIAN_POINT('Ctrl Pts',(64.4790194680927,-2.02568238621027,
136.673072130848));
#256864=CARTESIAN_POINT('Ctrl Pts',(64.20057184428,3.84258239688126,135.680806503568));
#256865=CARTESIAN_POINT('Ctrl Pts',(63.922124220467,6.17970167782515,130.207325334677));
#256866=CARTESIAN_POINT('Ctrl Pts',(63.6436765966542,2.8379770120581,125.282490423967));
#256867=CARTESIAN_POINT('Ctrl Pts',(63.3652289728412,-3.11170988490585,
125.431984462817));
#256868=CARTESIAN_POINT('Ctrl Pts',(63.0867813490283,-6.20188741312008,
130.518429732716));
#256869=CARTESIAN_POINT('Ctrl Pts',(62.8083337252156,-3.59283338772076,
135.86763151729));
#256870=CARTESIAN_POINT('Ctrl Pts',(62.5298861014024,2.31785900132509,136.563934699553));
#256871=CARTESIAN_POINT('Ctrl Pts',(62.2514384775899,6.09855220186056,131.967470671305));
#256872=CARTESIAN_POINT('Ctrl Pts',(61.9729908537767,4.27497385972414,126.302165324755));
#256873=CARTESIAN_POINT('Ctrl Pts',(61.6945432299639,-1.47709661541541,
124.774157507831));
#256874=CARTESIAN_POINT('Ctrl Pts',(61.416095606151,-5.87178746116934,128.787611756953));
#256875=CARTESIAN_POINT('Ctrl Pts',(61.1376479823382,-4.8705924828735,134.65435968532));
#256876=CARTESIAN_POINT('Ctrl Pts',(60.8592003585251,0.606439045512412,
136.983146553331));
#256877=CARTESIAN_POINT('Ctrl Pts',(60.5807527347125,5.52618271726667,133.633930996847));
#256878=CARTESIAN_POINT('Ctrl Pts',(60.3023051108993,5.36763444088732,127.684478494003));
#256879=CARTESIAN_POINT('Ctrl Pts',(60.0238574870866,0.276492336852797,
124.602045247997));
#256880=CARTESIAN_POINT('Ctrl Pts',(59.7454098632736,-5.06873271734795,
127.219236826675));
#256881=CARTESIAN_POINT('Ctrl Pts',(59.4669622394608,-5.75604002566515,
133.130982026147));
#256882=CARTESIAN_POINT('Ctrl Pts',(59.1885146156479,-1.15382774858414,
136.904675812908));
#256883=CARTESIAN_POINT('Ctrl Pts',(58.9100669918351,4.50869586182645,135.072477952114));
#256884=CARTESIAN_POINT('Ctrl Pts',(58.6316193680221,6.02794823725661,129.318088769994));
#256885=CARTESIAN_POINT('Ctrl Pts',(58.3531717442092,2.00781066429043,124.929510807376));
#256886=CARTESIAN_POINT('Ctrl Pts',(58.0747241203963,-3.85740682215468,
125.939632817953));
#256887=CARTESIAN_POINT('Ctrl Pts',(57.7962764965834,-6.17785588383907,
131.42020202121));
#256888=CARTESIAN_POINT('Ctrl Pts',(57.5178288727705,-2.82115719331391,
136.334843060042));
#256889=CARTESIAN_POINT('Ctrl Pts',(57.2393812489577,3.12804713667602,136.167240913326));
#256890=CARTESIAN_POINT('Ctrl Pts',(56.9609336251447,6.20272896165862,131.071413766074));
#256891=CARTESIAN_POINT('Ctrl Pts',(56.6824860013319,3.57740589103289,125.730177821614));
#256892=CARTESIAN_POINT('Ctrl Pts',(56.404038377519,-2.33537842745856,125.051867979023));
#256893=CARTESIAN_POINT('Ctrl Pts',(56.125590753706,-6.10206406069443,129.659817846364));
#256894=CARTESIAN_POINT('Ctrl Pts',(55.8471431298932,-4.26125092455389,
135.319546606417));
#256895=CARTESIAN_POINT('Ctrl Pts',(55.5686955060803,1.49544363757083,136.830040021814));
#256896=CARTESIAN_POINT('Ctrl Pts',(55.2902478822675,5.87789855325116,132.80322843551));
#256897=CARTESIAN_POINT('Ctrl Pts',(55.0118002584545,4.85885184980179,126.939554974638));
#256898=CARTESIAN_POINT('Ctrl Pts',(54.7333526346416,-0.625242335506623,
124.627449093364));
#256899=CARTESIAN_POINT('Ctrl Pts',(54.4549050108287,-5.53476935927053,
127.991623143927));
#256900=CARTESIAN_POINT('Ctrl Pts',(54.1764573870159,-5.35811373037978,
133.9405655229));
#256901=CARTESIAN_POINT('Ctrl Pts',(53.8980097632029,-0.257613341678002,
137.007488805997));
#256902=CARTESIAN_POINT('Ctrl Pts',(53.61956213939,5.07962112291461,134.374040323585));
#256903=CARTESIAN_POINT('Ctrl Pts',(53.3411145155772,5.74893192883615,128.460230579889));
#256904=CARTESIAN_POINT('Ctrl Pts',(53.0626668917642,1.13525514309568,124.7005618237));
#256905=CARTESIAN_POINT('Ctrl Pts',(52.7842192679514,-4.52166565885288,
126.549985971924));
#256906=CARTESIAN_POINT('Ctrl Pts',(52.5057716441385,-6.0233966159634,132.308972581737));
#256907=CARTESIAN_POINT('Ctrl Pts',(52.2273240203255,-1.98992034228702,
136.685294300858));
#256908=CARTESIAN_POINT('Ctrl Pts',(51.9488763965128,3.87219551293788,135.657325264614));
#256909=CARTESIAN_POINT('Ctrl Pts',(51.6704287726998,6.17595285904027,130.169718798237));
#256910=CARTESIAN_POINT('Ctrl Pts',(51.391981148887,2.80431123975502,125.265317159845));
#256911=CARTESIAN_POINT('Ctrl Pts',(51.113533525074,-3.14435541064497,125.451025861782));
#256912=CARTESIAN_POINT('Ctrl Pts',(50.8350859012611,-6.20351304896362,
130.556187679343));
#256913=CARTESIAN_POINT('Ctrl Pts',(50.5566382774483,-3.5619452537452,135.889408303207));
#256914=CARTESIAN_POINT('Ctrl Pts',(50.2781906536353,2.35287621896542,136.549718522358));
#256915=CARTESIAN_POINT('Ctrl Pts',(49.9997430298226,6.10551939084041,131.930325503341));
#256916=CARTESIAN_POINT('Ctrl Pts',(49.7212954060095,4.2474885137371,126.27622576074));
#256917=CARTESIAN_POINT('Ctrl Pts',(49.4428477821967,-1.51377680614101,
124.783260739875));
#256918=CARTESIAN_POINT('Ctrl Pts',(49.1644001583838,-5.88395519328364,
128.823392359526));
#256919=CARTESIAN_POINT('Ctrl Pts',(48.8859525345709,-4.84706620499019,
134.683937032636));
#256920=CARTESIAN_POINT('Ctrl Pts',(48.607504910758,0.644039833341117,136.97934050814));
#256921=CARTESIAN_POINT('Ctrl Pts',(48.3290572869451,5.54330472792681,133.600239128744));
#256922=CARTESIAN_POINT('Ctrl Pts',(48.0506096631323,5.34854338303893,127.651861983834));
#256923=CARTESIAN_POINT('Ctrl Pts',(47.7721620393193,0.23873196000854,124.600477075203));
#256924=CARTESIAN_POINT('Ctrl Pts',(47.4937144155065,-5.09046247156518,
127.250158065443));
#256925=CARTESIAN_POINT('Ctrl Pts',(47.2152667916935,-5.74177057468722,
133.165977568637));
#256926=CARTESIAN_POINT('Ctrl Pts',(46.9368191678807,-1.11667202075834,
136.911586465198));
#256927=CARTESIAN_POINT('Ctrl Pts',(46.6583715440677,4.53459356778643,135.044953162355));
#256928=CARTESIAN_POINT('Ctrl Pts',(46.379923920255,6.01878919474683,129.281422475313));
#256929=CARTESIAN_POINT('Ctrl Pts',(46.101476296442,1.97201158593325,124.917397541337));
#256930=CARTESIAN_POINT('Ctrl Pts',(45.8230286726291,-3.88694833223118,
125.963204080281));
#256931=CARTESIAN_POINT('Ctrl Pts',(45.5445810488162,-6.17399262105761,
131.457796973343));
#256932=CARTESIAN_POINT('Ctrl Pts',(45.2661334250033,-2.78743930743976,
136.351913777587));
#256933=CARTESIAN_POINT('Ctrl Pts',(44.9876858011905,3.16063455573481,136.148100240809));
#256934=CARTESIAN_POINT('Ctrl Pts',(44.7092381773775,6.20423966777097,131.033651046464));
#256935=CARTESIAN_POINT('Ctrl Pts',(44.4307905535647,3.54645161908363,125.708495149421));
#256936=CARTESIAN_POINT('Ctrl Pts',(44.1523429297517,-2.37035221374829,
125.066190670735));
#256937=CARTESIAN_POINT('Ctrl Pts',(43.8738953059389,-6.10891816028884,
129.696984048001));
#256938=CARTESIAN_POINT('Ctrl Pts',(43.5954476821259,-4.23368675476706,
135.345402394343));
#256939=CARTESIAN_POINT('Ctrl Pts',(43.3170000583131,1.53209595128933,136.820825190051));
#256940=CARTESIAN_POINT('Ctrl Pts',(43.0385524345002,5.88995732515911,132.767410964279));
#256941=CARTESIAN_POINT('Ctrl Pts',(42.7601048106873,4.83523565761953,126.910049370218));
#256942=CARTESIAN_POINT('Ctrl Pts',(42.4816571868744,-0.662831364878718,
124.631369564788));
#256943=CARTESIAN_POINT('Ctrl Pts',(42.2032095630615,-5.55178874416567,
128.025366969483));
#256944=CARTESIAN_POINT('Ctrl Pts',(41.9247619392486,-5.33892348752252,
133.973123775378));
#256945=CARTESIAN_POINT('Ctrl Pts',(41.6463143154357,-0.219848366758665,
137.008942041929));
#256946=CARTESIAN_POINT('Ctrl Pts',(41.3678666916229,5.10125666286673,134.343053090145));
#256947=CARTESIAN_POINT('Ctrl Pts',(41.0894190678099,5.73455602955998,128.425278630796));
#256948=CARTESIAN_POINT('Ctrl Pts',(40.8109714439971,1.09807855372398,124.693764292674));
#256949=CARTESIAN_POINT('Ctrl Pts',(40.5325238201841,-4.5474794688646,126.5775894579));
#256950=CARTESIAN_POINT('Ctrl Pts',(40.2540761963713,-6.01412601628932,
132.345610829607));
#256951=CARTESIAN_POINT('Ctrl Pts',(39.9756285725584,-1.95408456113369,
136.697298550707));
#256952=CARTESIAN_POINT('Ctrl Pts',(39.6971809487455,3.90166514336576,135.633664197272));
#256953=CARTESIAN_POINT('Ctrl Pts',(39.4187333249326,6.171975188051,130.132135778682));
#256954=CARTESIAN_POINT('Ctrl Pts',(39.1402857011198,2.77054155266769,125.248349147017));
#256955=CARTESIAN_POINT('Ctrl Pts',(38.8618380773068,-3.17688442113803,
125.470265630536));
#256956=CARTESIAN_POINT('Ctrl Pts',(38.583390453494,-6.20490881134979,130.593954822108));
#256957=CARTESIAN_POINT('Ctrl Pts',(38.304942829681,-3.53092513057837,135.910996660811));
#256958=CARTESIAN_POINT('Ctrl Pts',(38.0264952058682,2.38780624991219,136.535289448812));
#256959=CARTESIAN_POINT('Ctrl Pts',(37.7480475820552,6.11226033755391,131.893138612335));
#256960=CARTESIAN_POINT('Ctrl Pts',(37.4695999582424,4.21984577550119,126.250453988427));
#256961=CARTESIAN_POINT('Ctrl Pts',(37.1911523344295,-1.55040090331038,
124.792587085991));
#256962=CARTESIAN_POINT('Ctrl Pts',(36.9127047106166,-5.89590489327443,
128.859246367608));
#256963=CARTESIAN_POINT('Ctrl Pts',(36.6342570868037,-4.82336031728617,
134.713370620821));
#256964=CARTESIAN_POINT('Ctrl Pts',(36.3558094629908,0.681616756036961,
136.975305646799));
#256965=CARTESIAN_POINT('Ctrl Pts',(36.0773618391779,5.56022132939171,133.566443658335));
#256966=CARTESIAN_POINT('Ctrl Pts',(35.798914215365,5.32925413294858,127.619362290662));
#256967=CARTESIAN_POINT('Ctrl Pts',(35.5204665915522,0.200962736863706,
124.599138789596));
#256968=CARTESIAN_POINT('Ctrl Pts',(35.2420189677392,-5.11200359682353,
127.281211006494));
#256969=CARTESIAN_POINT('Ctrl Pts',(34.9635713439263,-5.72728836028912,
133.200885600541));
#256970=CARTESIAN_POINT('Ctrl Pts',(34.6851237201134,-1.07947491424015,
136.918270811987));
#256971=CARTESIAN_POINT('Ctrl Pts',(34.4066760963006,4.56032324271418,135.017271235878));
#256972=CARTESIAN_POINT('Ctrl Pts',(34.1282284724876,6.00940712379002,129.244812613665));
#256973=CARTESIAN_POINT('Ctrl Pts',(33.8497808486748,1.93613943396156,124.905502418881));
#256974=CARTESIAN_POINT('Ctrl Pts',(33.5713332248619,-3.91634581000783,
125.986954733445));
#256975=CARTESIAN_POINT('Ctrl Pts',(33.292885601049,-6.16990057870911,131.495367712155));
#256976=CARTESIAN_POINT('Ctrl Pts',(33.0144379772361,-2.753618131977,136.368778928511));
#256977=CARTESIAN_POINT('Ctrl Pts',(32.7359903534233,3.19310485631782,136.128761554055));
#256978=CARTESIAN_POINT('Ctrl Pts',(32.4575427296103,6.20552047350092,130.995879830412));
#256979=CARTESIAN_POINT('Ctrl Pts',(32.1790951057975,3.51536593206519,125.687001306397));
#256980=CARTESIAN_POINT('Ctrl Pts',(31.9006474819845,-2.40523816576522,
125.080725992446));
#256981=CARTESIAN_POINT('Ctrl Pts',(31.6221998581717,-6.11554589167424,
129.734191283883));
#256982=CARTESIAN_POINT('Ctrl Pts',(31.3437522343588,-4.20596570416061,
135.371089912296));
#256983=CARTESIAN_POINT('Ctrl Pts',(31.0653046105458,1.56869149262894,136.811387415981));
#256984=CARTESIAN_POINT('Ctrl Pts',(30.786856986733,5.90179784253235,132.731520751495));
#256985=CARTESIAN_POINT('Ctrl Pts',(30.5084093629201,4.81144029400183,126.880688070935));
#256986=CARTESIAN_POINT('Ctrl Pts',(30.2299617391072,-0.700395832790832,
124.635518778667));
#256987=CARTESIAN_POINT('Ctrl Pts',(29.9515141152943,-5.56860240548724,
128.05921377167));
#256988=CARTESIAN_POINT('Ctrl Pts',(29.6730664914815,-5.31953540889204,
134.005564608172));
#256989=CARTESIAN_POINT('Ctrl Pts',(29.3946188676685,-0.182075245277261,
137.010165364815));
#256990=CARTESIAN_POINT('Ctrl Pts',(29.1161712438556,5.12270317387725,134.311934729152));
#256991=CARTESIAN_POINT('Ctrl Pts',(28.8377236200427,5.71996763420123,128.390414839463));
#256992=CARTESIAN_POINT('Ctrl Pts',(28.5592759962298,1.06086127464794,124.687193192043));
#256993=CARTESIAN_POINT('Ctrl Pts',(28.280828372417,-4.57312477035222,126.605349568435));
#256994=CARTESIAN_POINT('Ctrl Pts',(28.0023807486041,-6.00463256096402,
132.382191965885));
#256995=CARTESIAN_POINT('Ctrl Pts',(27.7239331247912,-1.91817637065835,
136.709084435575));
#256996=CARTESIAN_POINT('Ctrl Pts',(27.4454855009783,3.93099019615694,135.60982417831));
#256997=CARTESIAN_POINT('Ctrl Pts',(27.1670378771654,6.16776881225138,130.094577668667));
#256998=CARTESIAN_POINT('Ctrl Pts',(26.8885902533525,2.73666920214424,125.231587014236));
#256999=CARTESIAN_POINT('Ctrl Pts',(26.6101426295396,-3.20929571101057,
125.48970305614));
#257000=CARTESIAN_POINT('Ctrl Pts',(26.3316950057267,-6.2060746485581,130.631729761538));
#257001=CARTESIAN_POINT('Ctrl Pts',(26.0532473819138,-3.49977416768234,
135.932395790139));
#257002=CARTESIAN_POINT('Ctrl Pts',(25.774799758101,2.42264779982026,136.52064801359));
#257003=CARTESIAN_POINT('Ctrl Pts',(25.4963521342881,6.11877479221284,131.85591137626));
#257004=CARTESIAN_POINT('Ctrl Pts',(25.2179045104751,4.19204666932822,126.224850962798));
#257005=CARTESIAN_POINT('Ctrl Pts',(24.9394568866623,-1.58696754980412,
124.802136200585));
#257006=CARTESIAN_POINT('Ctrl Pts',(24.6610092628494,-5.90763611834117,
128.895172452612));
#257007=CARTESIAN_POINT('Ctrl Pts',(24.3825616390365,-4.79947569819179,
134.742659359205));
#257008=CARTESIAN_POINT('Ctrl Pts',(24.1041140152236,0.719168421173241,
136.97104211882));
#257009=CARTESIAN_POINT('Ctrl Pts',(23.8256663914108,5.57693189481048,133.532545837923));
#257010=CARTESIAN_POINT('Ctrl Pts',(23.5472187675978,5.3097674053865,127.586980618775));
#257011=CARTESIAN_POINT('Ctrl Pts',(23.2687711437849,0.163186066970757,
124.598030440764));
#257012=CARTESIAN_POINT('Ctrl Pts',(22.990323519972,-5.13335529490864,127.312394499151));
#257013=CARTESIAN_POINT('Ctrl Pts',(22.7118758961592,-5.71259391911463,
133.235704828331));
#257014=CARTESIAN_POINT('Ctrl Pts',(22.4334282723462,-1.04223780738205,
136.924728605587));
#257015=CARTESIAN_POINT('Ctrl Pts',(22.1549806485334,4.58588393318709,134.98943319845));
#257016=CARTESIAN_POINT('Ctrl Pts',(21.8765330247205,5.9998023720423,129.208260541641));
#257017=CARTESIAN_POINT('Ctrl Pts',(21.5980854009075,1.90019553763114,124.893825880784));
#257018=CARTESIAN_POINT('Ctrl Pts',(21.3196377770947,-3.94559816615024,
126.010883897355));
#257019=CARTESIAN_POINT('Ctrl Pts',(21.0411901532818,-6.16557990842568,
131.532912845442));
#257020=CARTESIAN_POINT('Ctrl Pts',(20.7627425294689,-2.71969492018171,
136.385437887866));
#257021=CARTESIAN_POINT('Ctrl Pts',(20.484294905656,3.22545683522612,136.109225569666));
#257022=CARTESIAN_POINT('Ctrl Pts',(20.2058472818431,6.20657133138755,130.958101517545));
#257023=CARTESIAN_POINT('Ctrl Pts',(19.9273996580302,3.48414998186958,125.665697089004));
#257024=CARTESIAN_POINT('Ctrl Pts',(19.6489520342174,-2.44003499079723,
125.095473405541));
#257025=CARTESIAN_POINT('Ctrl Pts',(19.3705044104044,-6.12194700925765,
129.771438175283));
#257026=CARTESIAN_POINT('Ctrl Pts',(19.0920567865916,-4.17808879994825,
135.396608208416));
#257027=CARTESIAN_POINT('Ctrl Pts',(18.8136091627787,1.60522890552839,136.801727049323));
#257028=CARTESIAN_POINT('Ctrl Pts',(18.5351615389658,5.91341966661616,132.695559127084));
#257029=CARTESIAN_POINT('Ctrl Pts',(18.2567139151529,4.78746664069464,126.85147216478));
#257030=CARTESIAN_POINT('Ctrl Pts',(17.97826629134,-0.737934347277788,124.63989658125));
#257031=CARTESIAN_POINT('Ctrl Pts',(17.6998186675271,-5.58520972019883,
128.093162296283));
#257032=CARTESIAN_POINT('Ctrl Pts',(17.4213710437142,-5.29995021292075,
134.037886819174));
#257033=CARTESIAN_POINT('Ctrl Pts',(17.1429234199013,-0.144295376930669,
137.011158729324));
#257034=CARTESIAN_POINT('Ctrl Pts',(16.8644757960885,5.14395986123776,134.280686393713));
#257035=CARTESIAN_POINT('Ctrl Pts',(16.5860281722755,5.70516728333829,128.355640497777));
#257036=CARTESIAN_POINT('Ctrl Pts',(16.3075805484627,1.02360468496723,124.6808487653));
#257037=CARTESIAN_POINT('Ctrl Pts',(16.0291329246498,-4.5986006130197,126.633265274869));
#257038=CARTESIAN_POINT('Ctrl Pts',(15.7506853008369,-5.99491660177097,
132.418714635041));
#257039=CARTESIAN_POINT('Ctrl Pts',(15.472237677024,-1.88219710145218,136.720651518731));
#257040=CARTESIAN_POINT('Ctrl Pts',(15.1937900532111,3.96016958466077,135.585806091128));
#257041=CARTESIAN_POINT('Ctrl Pts',(14.9153424293982,6.16333388751023,130.057045859918));
#257042=CARTESIAN_POINT('Ctrl Pts',(14.6368948055853,2.70269544333712,125.215031382631));
#257043=CARTESIAN_POINT('Ctrl Pts',(14.3584471817724,-3.24158807925031,
125.509337418335));
#257044=CARTESIAN_POINT('Ctrl Pts',(14.0799995579596,-6.20701051738803,
130.669511097867));
#257045=CARTESIAN_POINT('Ctrl Pts',(13.8015519341466,-3.46849351936748,
135.953604898237));
#257046=CARTESIAN_POINT('Ctrl Pts',(13.5231043103337,2.45739957762318,136.505794759238));
#257047=CARTESIAN_POINT('Ctrl Pts',(13.2446566865208,6.12506251342167,131.818645174584));
#257048=CARTESIAN_POINT('Ctrl Pts',(12.966209062708,4.16409222532429,126.199417632585));
#257049=CARTESIAN_POINT('Ctrl Pts',(12.687761438895,-1.62347539063169,124.811907729812));
#257050=CARTESIAN_POINT('Ctrl Pts',(12.4093138150822,-5.91914843377905,
128.931169283287));
#257051=CARTESIAN_POINT('Ctrl Pts',(12.1308661912693,-4.77541323276041,
134.771802162479));
#257052=CARTESIAN_POINT('Ctrl Pts',(11.8524185674564,0.756693437259193,
136.96655008219));
#257053=CARTESIAN_POINT('Ctrl Pts',(11.5739709436435,5.59343580496719,133.498546923603));
#257054=CARTESIAN_POINT('Ctrl Pts',(11.2955233198306,5.2900839224404,127.554718168085));
#257055=CARTESIAN_POINT('Ctrl Pts',(11.0170756960177,0.125403350157864,
124.597152069781));
#257056=CARTESIAN_POINT('Ctrl Pts',(10.7386280722048,-5.15451677462551,
127.343707387895));
#257057=CARTESIAN_POINT('Ctrl Pts',(10.460180448392,-5.69768779567166,133.270433961767));
#257058=CARTESIAN_POINT('Ctrl Pts',(10.1817328245791,-1.0049620800187,136.930959606699));
#257059=CARTESIAN_POINT('Ctrl Pts',(9.90328520076621,4.61127469204443,134.961440081617));
#257060=CARTESIAN_POINT('Ctrl Pts',(9.62483757695328,5.98997529541125,129.171767613693));
#257061=CARTESIAN_POINT('Ctrl Pts',(9.34638995314043,1.86418122885626,124.882368359726));
#257062=CARTESIAN_POINT('Ctrl Pts',(9.0679423293275,-3.97470431670162,126.034990685308));
#257063=CARTESIAN_POINT('Ctrl Pts',(8.78949470551463,-6.16103077031137,
131.57043098196));
#257064=CARTESIAN_POINT('Ctrl Pts',(8.5110470817017,-2.68567092909101,136.401890038352));
#257065=CARTESIAN_POINT('Ctrl Pts',(8.2325994578889,3.25768929364524,136.089493011555));
#257066=CARTESIAN_POINT('Ctrl Pts',(7.95415183407592,6.20739220249103,130.920317507753));
#257067=CARTESIAN_POINT('Ctrl Pts',(7.67570421026306,3.45280492521512,125.644583286679));
#257068=CARTESIAN_POINT('Ctrl Pts',(7.39725658645018,-2.47474139943534,
125.110432363552));
#257069=CARTESIAN_POINT('Ctrl Pts',(7.11880896263729,-6.1281212758433,129.808723342005));
#257070=CARTESIAN_POINT('Ctrl Pts',(6.84036133882437,-4.15005707511893,
135.421956337113));
#257071=CARTESIAN_POINT('Ctrl Pts',(6.56191371501151,1.64170683608044,136.791844448048));
#257072=CARTESIAN_POINT('Ctrl Pts',(6.28346609119863,5.92482236675955,132.659527423617));
#257073=CARTESIAN_POINT('Ctrl Pts',(6.00501846738572,4.76331558605049,126.822402734361));
#257074=CARTESIAN_POINT('Ctrl Pts',(5.72657084357281,-0.775445517336138,
124.644502810313));
#257075=CARTESIAN_POINT('Ctrl Pts',(5.44812321975995,-5.60161007291028,
128.127211285347));
#257076=CARTESIAN_POINT('Ctrl Pts',(5.16967559594705,-5.28016862534525,
134.070089210674));
#257077=CARTESIAN_POINT('Ctrl Pts',(4.89122797213414,-0.106510161665837,
137.011922098645));
#257078=CARTESIAN_POINT('Ctrl Pts',(4.6127803483213,5.16502593727395,134.249309241742));
#257079=CARTESIAN_POINT('Ctrl Pts',(4.33433272450837,5.69015552540359,128.320956894316));
#257080=CARTESIAN_POINT('Ctrl Pts',(4.05588510069549,0.986310165238503,
124.674731247541));
#257081=CARTESIAN_POINT('Ctrl Pts',(3.77743747688256,-4.62390605285035,
126.661335542776));
#257082=CARTESIAN_POINT('Ctrl Pts',(3.49898985306972,-5.98497849873861,
132.455177483715));
#257083=CARTESIAN_POINT('Ctrl Pts',(3.22054222925682,-1.84614808674025,
136.731999371551));
#257084=CARTESIAN_POINT('Ctrl Pts',(2.94209460544391,3.9892022276243,135.561610825727));
#257085=CARTESIAN_POINT('Ctrl Pts',(2.66364698163102,6.15867057816533,130.019541743194));
#257086=CARTESIAN_POINT('Ctrl Pts',(2.38519935781816,2.66862153515642,125.198682865676));
#257087=CARTESIAN_POINT('Ctrl Pts',(2.10675173400524,-3.27376032925169,
125.529167989562));
#257088=CARTESIAN_POINT('Ctrl Pts',(1.82830411019233,-6.20771638316062,
130.707297431096));
#257089=CARTESIAN_POINT('Ctrl Pts',(1.54985648637947,-3.43708434474973,
135.974623199195));
#257090=CARTESIAN_POINT('Ctrl Pts',(1.27140886256659,2.49206029558105,136.490730236146));
#257091=CARTESIAN_POINT('Ctrl Pts',(0.992961238753657,6.13112326818657,
131.78134138822));
#257092=CARTESIAN_POINT('Ctrl Pts',(0.714513614940807,4.13598347935162,
126.174154940227));
#257093=CARTESIAN_POINT('Ctrl Pts',(0.436065991127901,-1.65992307298164,
124.821901311585));
#257094=CARTESIAN_POINT('Ctrl Pts',(0.157618367314999,-5.93044141299494,
128.967235525755));
#257095=CARTESIAN_POINT('Ctrl Pts',(-0.120829256497892,-4.75117381263555,
134.800797950748));
#257096=CARTESIAN_POINT('Ctrl Pts',(-0.399276880310752,0.794190413791566,
136.961829703365));
#257097=CARTESIAN_POINT('Ctrl Pts',(-0.67772450412367,5.60973244830296,
133.464448175219));
#257098=CARTESIAN_POINT('Ctrl Pts',(-0.956172127936585,5.27020441348929,
127.522576134092));
#257099=CARTESIAN_POINT('Ctrl Pts',(-1.23461975174943,0.0876159864779326,
124.596503709192));
#257100=CARTESIAN_POINT('Ctrl Pts',(-1.51306737556233,-5.17548725182775,
127.375148512417));
#257101=CARTESIAN_POINT('Ctrl Pts',(-1.79151499937523,-5.6825705423121,
133.305071713949));
#257102=CARTESIAN_POINT('Ctrl Pts',(-2.06996262318813,-0.967649113415911,
136.936963584433));
#257103=CARTESIAN_POINT('Ctrl Pts',(-2.34841024700098,4.63649457842225,
134.933292922676));
#257104=CARTESIAN_POINT('Ctrl Pts',(-2.62685787081389,5.97992625804282,
129.13533518208));
#257105=CARTESIAN_POINT('Ctrl Pts',(-2.90530549462681,1.82809784216042,
124.871130280269));
#257106=CARTESIAN_POINT('Ctrl Pts',(-3.18375311843967,-4.00366318312286,
126.059274204017));
#257107=CARTESIAN_POINT('Ctrl Pts',(-3.46220074225256,-6.15625333293613,
131.607920731459));
#257108=CARTESIAN_POINT('Ctrl Pts',(-3.74064836606547,-2.65154741947636,
136.418134770325));
#257109=CARTESIAN_POINT('Ctrl Pts',(-4.01909598987837,3.28980103718956,
136.06956461092));
#257110=CARTESIAN_POINT('Ctrl Pts',(-4.29754361369122,6.20798305639367,
130.882529201136));
#257111=CARTESIAN_POINT('Ctrl Pts',(-4.57599123750414,3.42133192360438,
125.623660681799));
#257112=CARTESIAN_POINT('Ctrl Pts',(-4.85443886131705,-2.5093561056208,
125.125602312169));
#257113=CARTESIAN_POINT('Ctrl Pts',(-5.13288648512991,-6.13406846264146,
129.846045402432));
#257114=CARTESIAN_POINT('Ctrl Pts',(-5.41133410894279,-4.12187156839848,
135.447133359102));
#257115=CARTESIAN_POINT('Ctrl Pts',(-5.68978173275571,1.67812393258193,
136.781739978358));
#257116=CARTESIAN_POINT('Ctrl Pts',(-5.9682293565686,5.93600552043131,132.623426976261));
#257117=CARTESIAN_POINT('Ctrl Pts',(-6.24667698038146,4.73898802499559,
126.793480856855));
#257118=CARTESIAN_POINT('Ctrl Pts',(-6.52512460419438,-0.812927952975666,
124.649337295173));
#257119=CARTESIAN_POINT('Ctrl Pts',(-6.80357222800728,-5.61780285590049,
128.161359477164));
#257120=CARTESIAN_POINT('Ctrl Pts',(-7.08201985182013,-5.26019137917956,
134.1021705894));
#257121=CARTESIAN_POINT('Ctrl Pts',(-7.36046747563304,-0.0687209996277829,
137.012455444495));
#257122=CARTESIAN_POINT('Ctrl Pts',(-7.63891509944595,5.18590062137458,
134.217804435933));
#257123=CARTESIAN_POINT('Ctrl Pts',(-7.91736272325884,5.67493291666336,
128.286365314294));
#257124=CARTESIAN_POINT('Ctrl Pts',(-8.1958103470717,0.948979097423875,
124.668840865451));
#257125=CARTESIAN_POINT('Ctrl Pts',(-8.47425797088461,-4.64904015214177,
126.689559331999));
#257126=CARTESIAN_POINT('Ctrl Pts',(-8.75270559469752,-5.97481862012702,
132.491579160764));
#257127=CARTESIAN_POINT('Ctrl Pts',(-9.03115321851038,-1.81003066233205,
136.743127573537));
#257128=CARTESIAN_POINT('Ctrl Pts',(-9.30960084232328,4.0180870492325,135.537239278668));
#257129=CARTESIAN_POINT('Ctrl Pts',(-9.58804846613619,6.15377905701727,
129.982066708221));
#257130=CARTESIAN_POINT('Ctrl Pts',(-9.86649608994908,2.63444874022312,
125.182542069172));
#257131=CARTESIAN_POINT('Ctrl Pts',(-10.144943713762,-3.30581126886015,
125.549194034992));
#257132=CARTESIAN_POINT('Ctrl Pts',(-10.4233913375749,-6.20819221971975,
130.745087361036));
#257133=CARTESIAN_POINT('Ctrl Pts',(-10.7018389613878,-3.40554780770759,
135.995449914173));
#257134=CARTESIAN_POINT('Ctrl Pts',(-10.9802865852006,2.52662866932821,
136.475455002538));
#257135=CARTESIAN_POINT('Ctrl Pts',(-11.2587342090136,6.13695683192405,
131.744001399476));
#257136=CARTESIAN_POINT('Ctrl Pts',(-11.5371818328265,4.10772147299012,
126.149063821843));
#257137=CARTESIAN_POINT('Ctrl Pts',(-11.8156294566394,-1.69630924627168,
124.832116575588));
#257138=CARTESIAN_POINT('Ctrl Pts',(-12.0940770804522,-5.94151463752335,
129.003369843568));
#257139=CARTESIAN_POINT('Ctrl Pts',(-12.3725247042651,-4.72675833601782,
134.829645649562));
#257140=CARTESIAN_POINT('Ctrl Pts',(-12.6509723280781,0.83165796130609,
136.956881157257));
#257141=CARTESIAN_POINT('Ctrl Pts',(-12.9294199518909,5.62582122093989,
133.430250856313));
#257142=CARTESIAN_POINT('Ctrl Pts',(-13.2078675757038,5.25012961517551,
127.490555707831));
#257143=CARTESIAN_POINT('Ctrl Pts',(-13.4863151995167,0.0498253761554086,
124.596085383024));
#257144=CARTESIAN_POINT('Ctrl Pts',(-13.7647628233296,-5.19626594944658,
127.406716707655));
#257145=CARTESIAN_POINT('Ctrl Pts',(-14.0432104471424,-5.66724271921134,
133.339616801361));
#257146=CARTESIAN_POINT('Ctrl Pts',(-14.3216580709554,-0.930300290219375,
136.942740316309));
#257147=CARTESIAN_POINT('Ctrl Pts',(-14.6001056947683,4.6615426577884,134.904992764631));
#257148=CARTESIAN_POINT('Ctrl Pts',(-14.8785533185811,5.96965563230779,
129.098964596818));
#257149=CARTESIAN_POINT('Ctrl Pts',(-15.157000942394,1.79194671462675,124.860112058844));
#257150=CARTESIAN_POINT('Ctrl Pts',(-15.4354485662069,-4.03247369233249,
126.08373355365));
#257151=CARTESIAN_POINT('Ctrl Pts',(-15.7138961900198,-6.15124777332969,
131.645380704742));
#257152=CARTESIAN_POINT('Ctrl Pts',(-15.9923438138327,-2.61732565579698,
136.434171481834));
#257153=CARTESIAN_POINT('Ctrl Pts',(-16.2707914376456,3.32179087594663,
136.049441106215));
#257154=CARTESIAN_POINT('Ctrl Pts',(-16.5492390614585,6.2083438712012,130.844737997954));
#257155=CARTESIAN_POINT('Ctrl Pts',(-16.8276866852714,3.38973214328102,
125.602930049661));
#257156=CARTESIAN_POINT('Ctrl Pts',(-17.1061343090842,-2.54387782669295,
125.140982689263));
#257157=CARTESIAN_POINT('Ctrl Pts',(-17.3845819328972,-6.13978834927694,
129.883402973582));
#257158=CARTESIAN_POINT('Ctrl Pts',(-17.66302955671,-4.09353332421128,135.47213834144));
#257159=CARTESIAN_POINT('Ctrl Pts',(-17.9414771805229,1.71447884558397,
136.771414014676));
#257160=CARTESIAN_POINT('Ctrl Pts',(-18.2199248043358,5.94696871323555,
132.587259122732));
#257161=CARTESIAN_POINT('Ctrl Pts',(-18.4983724281487,4.71448485899666,
126.764707603974));
#257162=CARTESIAN_POINT('Ctrl Pts',(-18.7768200519616,-0.850380265270943,
124.654399856686));
#257163=CARTESIAN_POINT('Ctrl Pts',(-19.0552676757745,-5.63378746913994,
128.19560560636));
#257164=CARTESIAN_POINT('Ctrl Pts',(-19.3337152995874,-5.24001921468789,
134.134129766565));
#257165=CARTESIAN_POINT('Ctrl Pts',(-19.6121629234003,-0.0309292911078312,
137.012758747106));
#257166=CARTESIAN_POINT('Ctrl Pts',(-19.8906105472132,5.2065831400206,134.18617314371));
#257167=CARTESIAN_POINT('Ctrl Pts',(-20.1690581710261,5.65950002119693,
128.251867039513));
#257168=CARTESIAN_POINT('Ctrl Pts',(-20.447505794839,0.911612864839816,
124.663177837304));
#257169=CARTESIAN_POINT('Ctrl Pts',(-20.7259534186518,-4.67400197954067,
126.717935596697));
#257170=CARTESIAN_POINT('Ctrl Pts',(-21.0044010424647,-5.96443734241423,
132.527918317308));
#257171=CARTESIAN_POINT('Ctrl Pts',(-21.2828486662776,-1.77384616657202,
136.754035712331));
#257172=CARTESIAN_POINT('Ctrl Pts',(-21.5612962900905,4.0468229791472,135.512692353051));
#257173=CARTESIAN_POINT('Ctrl Pts',(-21.8397439139034,6.14865950532324,
129.944622143653));
#257174=CARTESIAN_POINT('Ctrl Pts',(-22.1181915377163,2.60017832482316,
125.166609591221));
#257175=CARTESIAN_POINT('Ctrl Pts',(-22.3966391615293,-3.33773971041633,
125.569414812551));
#257176=CARTESIAN_POINT('Ctrl Pts',(-22.6750867853421,-6.20843800943312,
130.782879487369));
#257177=CARTESIAN_POINT('Ctrl Pts',(-22.953534409155,-3.37388507683905,
136.016084271426));
#257178=CARTESIAN_POINT('Ctrl Pts',(-23.2319820329679,2.56110341792085,
136.45996962444));
#257179=CARTESIAN_POINT('Ctrl Pts',(-23.5104296567807,6.14256298846929,
131.706626591997));
#257180=CARTESIAN_POINT('Ctrl Pts',(-23.7888772805937,4.07930725349882,
126.124145207193));
#257181=CARTESIAN_POINT('Ctrl Pts',(-24.0673249044065,-1.73263256219878,
124.842553143289));
#257182=CARTESIAN_POINT('Ctrl Pts',(-24.3457725282195,-5.95236769704188,
129.039570897758));
#257183=CARTESIAN_POINT('Ctrl Pts',(-24.6242201520323,-4.70216770763169,
134.858344189959));
#257184=CARTESIAN_POINT('Ctrl Pts',(-24.9026677758452,0.86909469142902,
136.951704627238));
#257185=CARTESIAN_POINT('Ctrl Pts',(-25.1811153996581,5.64170152670257,
133.395956234079));
#257186=CARTESIAN_POINT('Ctrl Pts',(-25.459563023471,5.22986027137813,127.458658075828));
#257187=CARTESIAN_POINT('Ctrl Pts',(-25.7380106472839,0.0120329195352371,
124.595897106778));
#257188=CARTESIAN_POINT('Ctrl Pts',(-26.0164582710968,-5.21685209751974,
127.438410803838));
#257189=CARTESIAN_POINT('Ctrl Pts',(-26.2949058949097,-5.6517048943475,
133.374067943923));
#257190=CARTESIAN_POINT('Ctrl Pts',(-26.5733535187226,-0.892916994403456,
136.948289588268));
#257191=CARTESIAN_POINT('Ctrl Pts',(-26.8518011425354,4.68641800197708,
134.876540656153));
#257192=CARTESIAN_POINT('Ctrl Pts',(-27.1302487663484,5.95916379878798,
129.062657205632));
#257193=CARTESIAN_POINT('Ctrl Pts',(-27.4086963901612,1.75572918584856,
124.849314103734));
#257194=CARTESIAN_POINT('Ctrl Pts',(-27.6871440139742,-4.06113477674652,
126.108367827853));
#257195=CARTESIAN_POINT('Ctrl Pts',(-27.965591637787,-6.1460142769749,131.682809513716));
#257196=CARTESIAN_POINT('Ctrl Pts',(-28.2440392616,-2.5830069061529,136.449999578631));
#257197=CARTESIAN_POINT('Ctrl Pts',(-28.5224868854127,3.3536576245212,136.029123243122));
#257198=CARTESIAN_POINT('Ctrl Pts',(-28.8009345092257,6.20847463354345,
130.806945298572));
#257199=CARTESIAN_POINT('Ctrl Pts',(-29.0793821330386,3.35800675518651,
125.582392158445));
#257200=CARTESIAN_POINT('Ctrl Pts',(-29.3578297568515,-2.57830528343674,
125.156572924908));
#257201=CARTESIAN_POINT('Ctrl Pts',(-29.6362773806644,-6.14528072379723,
129.920794671155));
#257202=CARTESIAN_POINT('Ctrl Pts',(-29.9147250044772,-4.06504339264135,
135.496970357558));
#257203=CARTESIAN_POINT('Ctrl Pts',(-30.1931726282902,1.75077022794215,
136.760866939637));
#257204=CARTESIAN_POINT('Ctrl Pts',(-30.471620252103,5.95771153892721,132.551025203244));
#257205=CARTESIAN_POINT('Ctrl Pts',(-30.750067875916,4.68980699602731,126.736084041921));
#257206=CARTESIAN_POINT('Ctrl Pts',(-31.0285154997288,-0.887801066412759,
124.659690307256));
#257207=CARTESIAN_POINT('Ctrl Pts',(-31.3069631235417,-5.6495633203129,
128.229948403933));
#257208=CARTESIAN_POINT('Ctrl Pts',(-31.5854107473546,-5.21965287935721,
134.16596555791));
#257209=CARTESIAN_POINT('Ctrl Pts',(-31.8638583711675,0.00686356350839004,
137.012831995241));
#257210=CARTESIAN_POINT('Ctrl Pts',(-32.1423059949804,5.22707272681363,
134.154416537178));
#257211=CARTESIAN_POINT('Ctrl Pts',(-32.4207536187933,5.64385741087595,
128.217463348321));
#257212=CARTESIAN_POINT('Ctrl Pts',(-32.6992012426062,0.874212852105795,
124.657742372942));
#257213=CARTESIAN_POINT('Ctrl Pts',(-32.9776488664191,-4.69879061007736,
126.746463285377));
#257214=CARTESIAN_POINT('Ctrl Pts',(-33.2560964902319,-5.9538350502823,
132.564193606789));
#257215=CARTESIAN_POINT('Ctrl Pts',(-33.5345441140448,-1.73759594028995,
136.764723383724));
#257216=CARTESIAN_POINT('Ctrl Pts',(-33.8129917378578,4.07540895254819,
135.487970958469));
#257217=CARTESIAN_POINT('Ctrl Pts',(-34.0914393616706,6.14331211279008,
129.907209437008));
#257218=CARTESIAN_POINT('Ctrl Pts',(-34.3698869854835,2.56581155885918,
125.150886022208));
#257219=CARTESIAN_POINT('Ctrl Pts',(-34.6483346092964,-3.3695444708001,
125.589829572953));
#257220=CARTESIAN_POINT('Ctrl Pts',(-34.9267822331094,-6.2084537431929,
130.820672409693));
#257221=CARTESIAN_POINT('Ctrl Pts',(-35.2052298569221,-3.34209732541825,
136.036525506343));
#257222=CARTESIAN_POINT('Ctrl Pts',(-35.4836774807351,2.59548326388451,
136.444274675672));
#257223=CARTESIAN_POINT('Ctrl Pts',(-35.7621251045479,6.14794153008404,
131.66921835072));
#257224=CARTESIAN_POINT('Ctrl Pts',(-36.0405727283609,4.05074187377708,
126.099400019648));
#257225=CARTESIAN_POINT('Ctrl Pts',(-36.3190203521737,-1.76889167478912,
124.85321062796));
#257226=CARTESIAN_POINT('Ctrl Pts',(-36.5974679759867,-5.96300018938643,
129.075837346879));
#257227=CARTESIAN_POINT('Ctrl Pts',(-36.8759155997995,-4.67740283869194,
134.886892508504));
#257228=CARTESIAN_POINT('Ctrl Pts',(-37.1543632236125,0.906499216928551,
136.946300305126));
#257229=CARTESIAN_POINT('Ctrl Pts',(-37.4328108474252,5.65737277714046,
133.361565579315));
#257230=CARTESIAN_POINT('Ctrl Pts',(-37.7112584712383,5.2093971331851,127.426884420063));
#257231=CARTESIAN_POINT('Ctrl Pts',(-37.9897060950511,-0.0257599829691867,
124.595938887431));
#257232=CARTESIAN_POINT('Ctrl Pts',(-38.268153718864,-5.23724493321992,
127.470229626529));
#257233=CARTESIAN_POINT('Ctrl Pts',(-38.5466013426768,-5.63595764348039,
133.408423865036));
#257234=CARTESIAN_POINT('Ctrl Pts',(-38.8250489664898,-0.855500611219946,
136.953611194679));
#257235=CARTESIAN_POINT('Ctrl Pts',(-39.1034965903026,4.71111968922328,
134.847937651547));
#257236=CARTESIAN_POINT('Ctrl Pts',(-39.3819442141156,5.94845114626212,
129.026414353905));
#257237=CARTESIAN_POINT('Ctrl Pts',(-39.6603918379284,1.71944659787975,
124.838736815064));
#257238=CARTESIAN_POINT('Ctrl Pts',(-39.9388394617414,-4.08964537431793,
126.133176113797));
#257239=CARTESIAN_POINT('Ctrl Pts',(-40.2172870855541,-6.14055303780089,
131.720205771443));
#257240=CARTESIAN_POINT('Ctrl Pts',(-40.495734709367,-2.54859244223803,
136.465618474199));
#257241=CARTESIAN_POINT('Ctrl Pts',(-40.7741823331801,3.3854001020792,136.008611774531));
#257242=CARTESIAN_POINT('Ctrl Pts',(-41.0526299569928,6.20837533857501,
130.769152503414));
#257243=CARTESIAN_POINT('Ctrl Pts',(-41.3310775808058,3.3261569349168,125.562047769191));
#257244=CARTESIAN_POINT('Ctrl Pts',(-41.6095252046187,-2.61263720013008,
125.172372441404));
#257245=CARTESIAN_POINT('Ctrl Pts',(-41.8879728284316,-6.15054538268038,
129.958219109591));
#257246=CARTESIAN_POINT('Ctrl Pts',(-42.1664204522444,-4.03640282939359,
135.521628487296));
#257247=CARTESIAN_POINT('Ctrl Pts',(-42.4448680760573,1.78699673486542,
136.750099144066));
#257248=CARTESIAN_POINT('Ctrl Pts',(-42.7233156998703,5.96823359942677,
132.514726560457));
#257249=CARTESIAN_POINT('Ctrl Pts',(-43.0017633236831,4.66495535053527,
126.707611231352));
#257250=CARTESIAN_POINT('Ctrl Pts',(-43.2802109474961,-0.925188969759574,
124.665208450844));
#257251=CARTESIAN_POINT('Ctrl Pts',(-43.5586585713089,-5.6651298248394,
128.264386597296));
#257252=CARTESIAN_POINT('Ctrl Pts',(-43.8371061951219,-5.19909312786956,
134.197676783747));
#257253=CARTESIAN_POINT('Ctrl Pts',(-44.1155538189346,0.0446561637927345,
137.012675186187));
#257254=CARTESIAN_POINT('Ctrl Pts',(-44.3940014427476,5.24736862250453,
134.122535793092));
#257255=CARTESIAN_POINT('Ctrl Pts',(-44.6724490665605,5.62800566534308,
128.183155515557));
#257256=CARTESIAN_POINT('Ctrl Pts',(-44.9508966903734,0.836780445093053,
124.65253467378));
#257257=CARTESIAN_POINT('Ctrl Pts',(-45.2293443141862,-4.72340512520001,
126.775141340936));
#257258=CARTESIAN_POINT('Ctrl Pts',(-45.5077919379991,-5.94301213660306,
132.600403685011));
#257259=CARTESIAN_POINT('Ctrl Pts',(-45.7862395618121,-1.7012813267513,
136.775190191685));
#257260=CARTESIAN_POINT('Ctrl Pts',(-46.0646871856249,4.10384391017172,
135.463076010984));
#257261=CARTESIAN_POINT('Ctrl Pts',(-46.3431348094379,6.13773707756737,
129.869829974632));
#257262=CARTESIAN_POINT('Ctrl Pts',(-46.6215824332507,2.5313497158043,125.135371944775));
#257263=CARTESIAN_POINT('Ctrl Pts',(-46.9000300570636,-3.40122437147435,
125.610437559721));
#257264=CARTESIAN_POINT('Ctrl Pts',(-47.1784776808764,-6.20823942041608,
130.858464727578));
#257265=CARTESIAN_POINT('Ctrl Pts',(-47.4569253046894,-3.31018573135201,
136.056772861467));
#257266=CARTESIAN_POINT('Ctrl Pts',(-47.7353729285023,2.62976693326135,
136.428370737814));
#257267=CARTESIAN_POINT('Ctrl Pts',(-48.0138205523151,6.15309225746451,
131.631778061822));
#257268=CARTESIAN_POINT('Ctrl Pts',(-48.2922681761281,4.02202639232555,
126.074829176147));
#257269=CARTESIAN_POINT('Ctrl Pts',(-48.570715799941,-1.80508524044794,
124.864088634681));
#257270=CARTESIAN_POINT('Ctrl Pts',(-48.8491634237538,-5.97341172056607,
129.112167847066));
#257271=CARTESIAN_POINT('Ctrl Pts',(-49.1276110475668,-4.65246464686987,
134.915289547327));
#257272=CARTESIAN_POINT('Ctrl Pts',(-49.4060586713796,0.943870151766231,
136.940668391181));
#257273=CARTESIAN_POINT('Ctrl Pts',(-49.6845062951925,5.6728343915496,133.327080166382));
#257274=CARTESIAN_POINT('Ctrl Pts',(-49.9629539190054,5.18874095886556,
127.395235917922));
#257275=CARTESIAN_POINT('Ctrl Pts',(-50.2414015428183,-0.0635519309279763,
124.596210723434));
#257276=CARTESIAN_POINT('Ctrl Pts',(-50.5198491666312,-5.25744370088312,
127.50217199667));
#257277=CARTESIAN_POINT('Ctrl Pts',(-50.798296790444,-5.6200015501302,133.442683291627));
#257278=CARTESIAN_POINT('Ctrl Pts',(-51.076744414257,-0.818052527146474,
136.958704938348));
#257279=CARTESIAN_POINT('Ctrl Pts',(-51.3551920380699,4.73564680419706,
134.819184810706));
#257280=CARTESIAN_POINT('Ctrl Pts',(-51.6336396618827,5.93751807169133,
128.990237384633));
#257281=CARTESIAN_POINT('Ctrl Pts',(-51.9120872856956,1.68310029518491,
124.828380584778));
#257282=CARTESIAN_POINT('Ctrl Pts',(-52.1905349095086,-4.11800442857602,
126.1581574922));
#257283=CARTESIAN_POINT('Ctrl Pts',(-52.4689825333214,-6.13486425817587,
131.757568092191));
#257284=CARTESIAN_POINT('Ctrl Pts',(-52.7474301571343,-2.51408353929296,
136.481027589776));
#257285=CARTESIAN_POINT('Ctrl Pts',(-53.0258777809472,3.41701713239144,
135.987907460498));
#257286=CARTESIAN_POINT('Ctrl Pts',(-53.3043254047601,6.20804598997526,
130.731361012906));
#257287=CARTESIAN_POINT('Ctrl Pts',(-53.5827730285729,3.29418386267868,
125.541897635768));
#257288=CARTESIAN_POINT('Ctrl Pts',(-53.8612206523859,-2.64687230459117,
125.188380653292));
#257289=CARTESIAN_POINT('Ctrl Pts',(-54.1396682761987,-6.15558213084251,
129.995674902111));
#257290=CARTESIAN_POINT('Ctrl Pts',(-54.4181159000117,-4.0076126957546,
135.546111816938));
#257291=CARTESIAN_POINT('Ctrl Pts',(-54.6965635238244,1.82315702396754,
136.739111026966));
#257292=CARTESIAN_POINT('Ctrl Pts',(-54.9750111476374,5.97853450483549,
132.478364539431));
#257293=CARTESIAN_POINT('Ctrl Pts',(-55.2534587714502,4.63993084340721,
126.679290227339));
#257294=CARTESIAN_POINT('Ctrl Pts',(-55.5319063952633,-0.962542589888887,
124.670954082973));
#257295=CARTESIAN_POINT('Ctrl Pts',(-55.810354019076,-5.68048640589689,
128.298918910331));
#257296=CARTESIAN_POINT('Ctrl Pts',(-56.088801642889,-5.1783407220741,134.229262269005));
#257297=CARTESIAN_POINT('Ctrl Pts',(-56.3672492667019,0.0824471093265141,
137.012288325754));
#257298=CARTESIAN_POINT('Ctrl Pts',(-56.6456968905149,5.26747007502141,
134.090532092806));
#257299=CARTESIAN_POINT('Ctrl Pts',(-56.9241445143275,5.6119453719906,128.148944812513));
#257300=CARTESIAN_POINT('Ctrl Pts',(-57.2025921381407,0.799317030873196,
124.64755493279));
#257301=CARTESIAN_POINT('Ctrl Pts',(-57.4810397619534,-4.74784461280872,
126.803968700697));
#257302=CARTESIAN_POINT('Ctrl Pts',(-57.7594873857663,-5.93196900242356,
132.636547210196));
#257303=CARTESIAN_POINT('Ctrl Pts',(-58.0379350095792,-1.66490367160747,
136.785435748359));
#257304=CARTESIAN_POINT('Ctrl Pts',(-58.3163826333922,4.13212679834998,
135.438008433087));
#257305=CARTESIAN_POINT('Ctrl Pts',(-58.5948302572049,6.13193460624012,
129.832485141631));
#257306=CARTESIAN_POINT('Ctrl Pts',(-58.873277881018,2.49679407265481,125.120067933803));
#257307=CARTESIAN_POINT('Ctrl Pts',(-59.1517255048308,-3.43277823852872,
125.631238009216));
#257308=CARTESIAN_POINT('Ctrl Pts',(-59.4301731286437,-6.20779504904446,
130.896255040614));
#257309=CARTESIAN_POINT('Ctrl Pts',(-59.7086207524566,-3.27815147713605,
136.076825586523));
#257310=CARTESIAN_POINT('Ctrl Pts',(-59.9870683762695,2.66395315565763,
136.412258400192));
#257311=CARTESIAN_POINT('Ctrl Pts',(-60.2655160000824,6.15801497974849,
131.594307112665));
#257312=CARTESIAN_POINT('Ctrl Pts',(-60.5439636238952,3.99316187320697,
126.050433587173));
#257313=CARTESIAN_POINT('Ctrl Pts',(-60.8224112477081,-1.84121191800936,
124.875186760365));
#257314=CARTESIAN_POINT('Ctrl Pts',(-61.1008588715211,-5.98360190477769,
129.148561052078));
#257315=CARTESIAN_POINT('Ctrl Pts',(-61.3793064953339,-4.62735405625939,
134.943534254169));
#257316=CARTESIAN_POINT('Ctrl Pts',(-61.6577541191468,0.981206111148332,
136.934809094094));
#257317=CARTESIAN_POINT('Ctrl Pts',(-61.9362017429597,5.68808579699418,
133.292501273148));
#257318=CARTESIAN_POINT('Ctrl Pts',(-62.2146493667725,5.16789251384163,
127.36371374215));
#257319=CARTESIAN_POINT('Ctrl Pts',(-62.4930969905855,-0.10134152394658,
124.596712604715));
#257320=CARTESIAN_POINT('Ctrl Pts',(-62.7715446143984,-5.27744765203657,
127.534236730624));
#257321=CARTESIAN_POINT('Ctrl Pts',(-63.0499922382113,-5.60383720555579,
133.476844954201));
#257322=CARTESIAN_POINT('Ctrl Pts',(-63.3284398620242,-0.780574129835986,
136.963570630527));
#257323=CARTESIAN_POINT('Ctrl Pts',(-63.606887485837,4.75999843803683,134.790283199078));
#257324=CARTESIAN_POINT('Ctrl Pts',(-63.88533510965,5.92636498020503,128.954127638363));
#257325=CARTESIAN_POINT('Ctrl Pts',(-64.1637827334628,1.64669162458969,
124.818245796629));
#257326=CARTESIAN_POINT('Ctrl Pts',(-64.4422303572757,-4.14621088866563,
126.183311037368));
#257327=CARTESIAN_POINT('Ctrl Pts',(-64.7206779810887,-6.12894814889968,
131.794895091487));
#257328=CARTESIAN_POINT('Ctrl Pts',(-64.9991256049015,-2.47948147605779,
136.49622635437));
#257329=CARTESIAN_POINT('Ctrl Pts',(-65.2775732287142,3.44850754387722,
135.967011068231));
#257330=CARTESIAN_POINT('Ctrl Pts',(-65.5560208525274,6.20748659994837,
130.693572227424));
#257331=CARTESIAN_POINT('Ctrl Pts',(-65.83446847634,3.26208872324607,125.521942504845));
#257332=CARTESIAN_POINT('Ctrl Pts',(-66.1129161001531,-2.68100932822562,
125.204596967384));
#257333=CARTESIAN_POINT('Ctrl Pts',(-66.3913637239659,-6.1603907816451,
130.033160660777));
#257334=CARTESIAN_POINT('Ctrl Pts',(-66.6698113477789,-3.97867405855336,
135.570419439246));
#257335=CARTESIAN_POINT('Ctrl Pts',(-66.9482589715917,1.85924975531565,
136.727902995508));
#257336=CARTESIAN_POINT('Ctrl Pts',(-67.2267065954047,5.98861387344954,
132.441940487574));
#257337=CARTESIAN_POINT('Ctrl Pts',(-67.5051542192175,4.61473440193538,
126.651122079325));
#257338=CARTESIAN_POINT('Ctrl Pts',(-67.7836018430304,-0.999860542648545,
124.676926990737));
#257339=CARTESIAN_POINT('Ctrl Pts',(-68.0620494668433,-5.69563249444164,
128.33354406343));
#257340=CARTESIAN_POINT('Ctrl Pts',(-68.3404970906562,-5.15739643095884,
134.260720843274));
#257341=CARTESIAN_POINT('Ctrl Pts',(-68.618944714469,0.120234999752325,
137.011671428276));
#257342=CARTESIAN_POINT('Ctrl Pts',(-68.8973923382821,5.28737633949755,
134.058406622227));
#257343=CARTESIAN_POINT('Ctrl Pts',(-69.1758399620947,5.59567712593856,
128.114832506878));
#257344=CARTESIAN_POINT('Ctrl Pts',(-69.4542875859078,0.761823997666808,
124.642803334499));
#257345=CARTESIAN_POINT('Ctrl Pts',(-69.7327352097205,-4.77210816728929,
126.832944296451));
#257346=CARTESIAN_POINT('Ctrl Pts',(-70.0111828335336,-5.92070605695121,
132.672622843033));
#257347=CARTESIAN_POINT('Ctrl Pts',(-70.2896304573463,-1.62846432284579,
136.795459674095));
#257348=CARTESIAN_POINT('Ctrl Pts',(-70.5680780811594,4.16025656905012,
135.412769153666));
#257349=CARTESIAN_POINT('Ctrl Pts',(-70.8465257049722,6.12590491382102,
129.795176321834));
#257350=CARTESIAN_POINT('Ctrl Pts',(-71.1249733287852,2.46214590988275,
125.104974556385));
#257351=CARTESIAN_POINT('Ctrl Pts',(-71.4034209525978,-3.46420490272305,
125.652230150673));
#257352=CARTESIAN_POINT('Ctrl Pts',(-71.681868576411,-6.20712064554441,
130.93404194847));
#257353=CARTESIAN_POINT('Ctrl Pts',(-71.9603162002238,-3.24599574981168,
136.09668293845));
#257354=CARTESIAN_POINT('Ctrl Pts',(-72.2387638240367,2.69804066428979,
136.395938259856));
#257355=CARTESIAN_POINT('Ctrl Pts',(-72.5172114478495,6.16270951452303,
131.556806891751));
#257356=CARTESIAN_POINT('Ctrl Pts',(-72.7956590716624,3.96414938600637,
126.026214156713));
#257357=CARTESIAN_POINT('Ctrl Pts',(-73.0741066954753,-1.87727036878649,
124.886504593767));
#257358=CARTESIAN_POINT('Ctrl Pts',(-73.3525543192881,-5.99357036442037,
129.185015613353));
#257359=CARTESIAN_POINT('Ctrl Pts',(-73.6310019431012,-4.60207199734241,
134.971625582408));
#257360=CARTESIAN_POINT('Ctrl Pts',(-73.909449566914,1.01850571157763,136.928722630985));
#257361=CARTESIAN_POINT('Ctrl Pts',(-74.187897190727,5.70312642832773,133.257830180947));
#257362=CARTESIAN_POINT('Ctrl Pts',(-74.4663448145398,5.14685257066011,
127.332319060812));
#257363=CARTESIAN_POINT('Ctrl Pts',(-74.7447924383527,-0.139127361718492,
124.597444512675));
#257364=CARTESIAN_POINT('Ctrl Pts',(-75.0232400621657,-5.29725604542678,
127.566422640223));
#257365=CARTESIAN_POINT('Ctrl Pts',(-75.3016876859784,-5.58746520873256,
133.510907586884));
#257366=CARTESIAN_POINT('Ctrl Pts',(-75.5801353097915,-0.743066808063574,
136.968208090913));
#257367=CARTESIAN_POINT('Ctrl Pts',(-75.8585829336042,4.7841736883842,134.761233887624));
#257368=CARTESIAN_POINT('Ctrl Pts',(-76.1370305574171,5.91499228508486,
128.918086453158));
#257369=CARTESIAN_POINT('Ctrl Pts',(-76.41547818123,1.61022193523031,124.808332826166));
#257370=CARTESIAN_POINT('Ctrl Pts',(-76.693925805043,-4.17426370938676,
126.208635817229));
#257371=CARTESIAN_POINT('Ctrl Pts',(-76.9723734288558,-6.12280492919574,
131.832185386163));
#257372=CARTESIAN_POINT('Ctrl Pts',(-77.2508210526686,-2.44478753472383,
136.511214204787));
#257373=CARTESIAN_POINT('Ctrl Pts',(-77.5292686764817,3.47987016964863,
135.945923372052));
#257374=CARTESIAN_POINT('Ctrl Pts',(-77.8077163002943,6.20669718922256,
130.655787547247));
#257375=CARTESIAN_POINT('Ctrl Pts',(-78.0861639241075,3.22987270591563,
125.502183115868));
#257376=CARTESIAN_POINT('Ctrl Pts',(-78.3646115479203,-2.71504700607423,
125.221020782777));
#257377=CARTESIAN_POINT('Ctrl Pts',(-78.6430591717333,-6.16497115690175,
130.070674996542));
#257378=CARTESIAN_POINT('Ctrl Pts',(-78.921506795546,-3.94958799012119,
135.594550453492));
#257379=CARTESIAN_POINT('Ctrl Pts',(-79.199954419359,1.89527359148086,136.71647546501));
#257380=CARTESIAN_POINT('Ctrl Pts',(-79.4784020431719,5.9984713317742,132.405455754592));
#257381=CARTESIAN_POINT('Ctrl Pts',(-79.7568496669848,4.58936695978296,
126.623107831093));
#257382=CARTESIAN_POINT('Ctrl Pts',(-80.0352972907976,-1.0371414452086,
124.683126952807));
#257383=CARTESIAN_POINT('Ctrl Pts',(-80.3137449146107,-5.71056752923021,
128.368260773546));
#257384=CARTESIAN_POINT('Ctrl Pts',(-80.5921925384234,-5.13626103062165,
134.292051340844));
#257385=CARTESIAN_POINT('Ctrl Pts',(-80.8706401622364,0.158018434826916,
137.010824516613));
#257386=CARTESIAN_POINT('Ctrl Pts',(-81.1490877860493,5.30708667829958,
134.026160571776));
#257387=CARTESIAN_POINT('Ctrl Pts',(-81.4275354098621,5.57920153001237,
128.080819862696));
#257388=CARTESIAN_POINT('Ctrl Pts',(-81.705983033675,0.724302734791404,
124.63828005498));
#257389=CARTESIAN_POINT('Ctrl Pts',(-81.984430657488,-4.79619488954742,
126.862067054498));
#257390=CARTESIAN_POINT('Ctrl Pts',(-82.2628782813007,-5.90922371753823,
132.708629246728));
#257391=CARTESIAN_POINT('Ctrl Pts',(-82.5413259051138,-1.59196463073914,
136.805261597452));
#257392=CARTESIAN_POINT('Ctrl Pts',(-82.8197735289264,4.18823217991362,
135.387359107972));
#257393=CARTESIAN_POINT('Ctrl Pts',(-83.0982211527395,6.11964822374235,
129.757904897731));
#257394=CARTESIAN_POINT('Ctrl Pts',(-83.3766687765523,2.42740651138818,
125.090092371815));
#257395=CARTESIAN_POINT('Ctrl Pts',(-83.6551164003652,-3.49550319953123,
125.67341320622));
#257396=CARTESIAN_POINT('Ctrl Pts',(-83.9335640241781,-6.20621623490623,
130.971824050937));
#257397=CARTESIAN_POINT('Ctrl Pts',(-84.2120116479911,-3.21371974092037,
136.116344181428));
#257398=CARTESIAN_POINT('Ctrl Pts',(-84.4904592718038,2.73202819603347,
136.379410921554));
#257399=CARTESIAN_POINT('Ctrl Pts',(-84.7689068956169,6.16717568783019,
131.519278788663));
#257400=CARTESIAN_POINT('Ctrl Pts',(-85.0473545194296,3.9349900057924,126.002171782228));
#257401=CARTESIAN_POINT('Ctrl Pts',(-85.3258021432425,-1.91325925661942,
124.898041715501));
#257402=CARTESIAN_POINT('Ctrl Pts',(-85.6042497670555,-6.00331673010926,
129.221530180052));
#257403=CARTESIAN_POINT('Ctrl Pts',(-85.8826973908683,-4.57661940695503,
134.999562491112));
#257404=CARTESIAN_POINT('Ctrl Pts',(-86.1611450146813,1.05576757090286,
136.922409227389));
#257405=CARTESIAN_POINT('Ctrl Pts',(-86.4395926384942,5.71795572821454,
133.223068174528));
#257406=CARTESIAN_POINT('Ctrl Pts',(-86.718040262307,5.12562190896342,127.301053037252));
#257407=CARTESIAN_POINT('Ctrl Pts',(-86.9964878861199,-0.176908044074368,
124.598406420195));
#257408=CARTESIAN_POINT('Ctrl Pts',(-87.2749355099329,-5.31686814704595,
127.598728532803));
#257409=CARTESIAN_POINT('Ctrl Pts',(-87.5533831337457,-5.57088616633168,
133.544869927476));
#257410=CARTESIAN_POINT('Ctrl Pts',(-87.8318307575586,-0.70553195167748,
136.972617147663));
#257411=CARTESIAN_POINT('Ctrl Pts',(-88.1102783813713,4.80817165941601,
134.732037952774));
#257412=CARTESIAN_POINT('Ctrl Pts',(-88.3887260051845,5.90340040775061,
128.882115164534));
#257413=CARTESIAN_POINT('Ctrl Pts',(-88.6671736289971,1.57369257850503,
124.798642040718));
#257414=CARTESIAN_POINT('Ctrl Pts',(-88.9456212528103,-4.20216185122988,
126.234130893362));
#257415=CARTESIAN_POINT('Ctrl Pts',(-89.2240688766231,-6.11643482670397,
131.869437594414));
#257416=CARTESIAN_POINT('Ctrl Pts',(-89.5025165004358,-2.41000300088966,
136.525990585645));
#257417=CARTESIAN_POINT('Ctrl Pts',(-89.7809641242489,3.51110384754994,
135.924645153375));
#257418=CARTESIAN_POINT('Ctrl Pts',(-90.0594117480617,6.20567778705031,
130.618008372501));
#257419=CARTESIAN_POINT('Ctrl Pts',(-90.3378593718745,3.19753700446471,
125.482620201028));
#257420=CARTESIAN_POINT('Ctrl Pts',(-90.6163069956876,-2.74898407685696,
125.237651490881));
#257421=CARTESIAN_POINT('Ctrl Pts',(-90.8947546195002,-6.16932308688508,
130.108216519297));
#257422=CARTESIAN_POINT('Ctrl Pts',(-91.1732022433134,-3.92035556825405,
135.618503965492));
#257423=CARTESIAN_POINT('Ctrl Pts',(-91.4516498671261,1.93122719758584,
136.70482885892));
#257424=CARTESIAN_POINT('Ctrl Pts',(-91.7300974909391,6.00810651453776,
132.368911692441));
#257425=CARTESIAN_POINT('Ctrl Pts',(-92.0085451147519,4.56382945695037,
126.595248520721));
#257426=CARTESIAN_POINT('Ctrl Pts',(-92.2869927385648,-1.07438391611076,
124.689553739443));
#257427=CARTESIAN_POINT('Ctrl Pts',(-92.5654403623776,-5.72529095683809,
128.403067754236));
#257428=CARTESIAN_POINT('Ctrl Pts',(-92.8438879861907,-5.11493530424405,
134.323252600751));
#257429=CARTESIAN_POINT('Ctrl Pts',(-93.1223356100035,0.195796014469281,
137.009747622148));
#257430=CARTESIAN_POINT('Ctrl Pts',(-93.4007832338166,5.32660036105212,
133.993795136343));
#257431=CARTESIAN_POINT('Ctrl Pts',(-93.6792308576291,5.56251919472255,
128.046908140318));
#257432=CARTESIAN_POINT('Ctrl Pts',(-93.9576784814422,0.686754632612129,
124.633985261843));
#257433=CARTESIAN_POINT('Ctrl Pts',(-94.2361261052551,-4.82010388703947,
126.891335895681));
#257434=CARTESIAN_POINT('Ctrl Pts',(-94.5145737290679,-5.8975224096676,
132.744565087048));
#257435=CARTESIAN_POINT('Ctrl Pts',(-94.7930213528811,-1.55540594779807,
136.814841155217));
#257436=CARTESIAN_POINT('Ctrl Pts',(-95.0714689766937,4.21605259429308,
135.361779237583));
#257437=CARTESIAN_POINT('Ctrl Pts',(-95.3499166005066,6.11316476784841,
129.720672250431));
#257438=CARTESIAN_POINT('Ctrl Pts',(-95.6283642243196,2.39257716445285,
125.075421931555));
#257439=CARTESIAN_POINT('Ctrl Pts',(-95.9068118481323,-3.52667196918255,
125.694786390909));
#257440=CARTESIAN_POINT('Ctrl Pts',(-96.1852594719453,-6.20508185064282,
131.009599947983));
#257441=CARTESIAN_POINT('Ctrl Pts',(-96.4637070957582,-3.18132464646333,
136.135808586901));
#257442=CARTESIAN_POINT('Ctrl Pts',(-96.742154719571,2.76591449146702,136.362676997713));
#257443=CARTESIAN_POINT('Ctrl Pts',(-97.020602343384,6.17141333417382,131.481724194021));
#257444=CARTESIAN_POINT('Ctrl Pts',(-97.299049967197,3.90568481307747,125.978307354616));
#257445=CARTESIAN_POINT('Ctrl Pts',(-97.5774975910097,-1.94917724792726,
124.909797698053));
#257446=CARTESIAN_POINT('Ctrl Pts',(-97.8559452148228,-6.01284064068852,
129.258103399115));
#257447=CARTESIAN_POINT('Ctrl Pts',(-98.1343928386354,-4.55099722825276,
135.027343945068));
#257448=CARTESIAN_POINT('Ctrl Pts',(-98.4128404624484,1.09299030837272,
136.915869117251));
#257449=CARTESIAN_POINT('Ctrl Pts',(-98.6912880862614,5.73257314714861,
133.188216542011));
#257450=CARTESIAN_POINT('Ctrl Pts',(-98.9697357100741,5.10420131546234,
127.269916830042));
#257451=CARTESIAN_POINT('Ctrl Pts',(-99.2481833338871,-0.214682171037078,
124.599598291628));
#257452=CARTESIAN_POINT('Ctrl Pts',(-99.5266309576999,-5.33628323016052,
127.631153211259));
#257453=CARTESIAN_POINT('Ctrl Pts',(-99.8050785815131,-5.55410069269506,
133.578730717485));
#257454=CARTESIAN_POINT('Ctrl Pts',(-100.083526205326,-0.667970951546107,
136.976797637399));
#257455=CARTESIAN_POINT('Ctrl Pts',(-100.361973829139,4.83199146187865,
134.702696476397));
#257456=CARTESIAN_POINT('Ctrl Pts',(-100.640421452952,5.89158977774298,
128.846215105423));
#257457=CARTESIAN_POINT('Ctrl Pts',(-100.918869076765,1.53710490802326,
124.789173799381));
#257458=CARTESIAN_POINT('Ctrl Pts',(-101.197316700577,-4.22990428042106,
126.259795321038));
#257459=CARTESIAN_POINT('Ctrl Pts',(-101.47576432439,-6.10983807746976,
131.906650335846));
#257460=CARTESIAN_POINT('Ctrl Pts',(-101.754211948203,-2.37512916350784,
136.540554949401));
#257461=CARTESIAN_POINT('Ctrl Pts',(-102.032659572016,3.54220742020778,
135.903177200671));
#257462=CARTESIAN_POINT('Ctrl Pts',(-102.311107195829,6.20442843120499,
130.580236103105));
#257463=CARTESIAN_POINT('Ctrl Pts',(-102.589554819642,3.16508281710451,
125.463254485237));
#257464=CARTESIAN_POINT('Ctrl Pts',(-102.868002443455,-2.78281928302352,
125.254488475437));
#257465=CARTESIAN_POINT('Ctrl Pts',(-103.146450067268,-6.1734464103326,
130.145783837928));
#257466=CARTESIAN_POINT('Ctrl Pts',(-103.424897691081,-3.8909778761698,
135.642279087639));
#257467=CARTESIAN_POINT('Ctrl Pts',(-103.703345314893,1.96710924135641,
136.69296360881));
#257468=CARTESIAN_POINT('Ctrl Pts',(-103.981792938706,6.01751906470488,
132.332309655276));
#257469=CARTESIAN_POINT('Ctrl Pts',(-104.260240562519,4.53812283973896,
126.567545180546));
#257470=CARTESIAN_POINT('Ctrl Pts',(-104.538688186332,-1.11158657532129,
124.696207112496));
#257471=CARTESIAN_POINT('Ctrl Pts',(-104.817135810145,-5.73980223168479,
128.437963715717));
#257472=CARTESIAN_POINT('Ctrl Pts',(-105.095583433958,-5.093420042057,134.354323466822));
#257473=CARTESIAN_POINT('Ctrl Pts',(-105.374031057771,0.233566338818549,
137.008440784786));
#257474=CARTESIAN_POINT('Ctrl Pts',(-105.652478681584,5.34591666467016,
133.961311515241));
#257475=CARTESIAN_POINT('Ctrl Pts',(-105.930926305397,5.54563073823764,
128.013098596357));
#257476=CARTESIAN_POINT('Ctrl Pts',(-106.20937392921,0.649181082487974,
124.629919114234));
#257477=CARTESIAN_POINT('Ctrl Pts',(-106.487821553022,-4.84383427380942,
126.920749735436));
#257478=CARTESIAN_POINT('Ctrl Pts',(-106.766269176835,-5.88560256693534,
132.780429032376));
#257479=CARTESIAN_POINT('Ctrl Pts',(-107.044716800648,-1.51878962871805,
136.824197992414));
#257480=CARTESIAN_POINT('Ctrl Pts',(-107.323164424461,4.2437167812931,135.336030490371));
#257481=CARTESIAN_POINT('Ctrl Pts',(-107.601612048274,6.10645478638612,
129.683479759601));
#257482=CARTESIAN_POINT('Ctrl Pts',(-107.880059672087,2.35765915969063,
125.060963779225));
#257483=CARTESIAN_POINT('Ctrl Pts',(-108.1585072959,-3.55771005670707,125.716348912751));
#257484=CARTESIAN_POINT('Ctrl Pts',(-108.436954919713,-6.20371753478999,
131.04736823981));
#257485=CARTESIAN_POINT('Ctrl Pts',(-108.715402543526,-3.14881166685081,
136.155075433609));
#257486=CARTESIAN_POINT('Ctrl Pts',(-108.993850167338,2.79969829492213,
136.345737108415));
#257487=CARTESIAN_POINT('Ctrl Pts',(-109.272297791151,6.17542229652738,
131.444144499421));
#257488=CARTESIAN_POINT('Ctrl Pts',(-109.550745414964,3.87623489377466,
125.954621758183));
#257489=CARTESIAN_POINT('Ctrl Pts',(-109.829193038777,-1.98502301175461,
124.921772105802));
#257490=CARTESIAN_POINT('Ctrl Pts',(-110.10764066259,-6.02214174324697,
129.294733915307));
#257491=CARTESIAN_POINT('Ctrl Pts',(-110.386088286403,-4.52520641067474,
135.054968914823));
#257492=CARTESIAN_POINT('Ctrl Pts',(-110.664535910216,1.13017254468408,
136.909102542919));
#257493=CARTESIAN_POINT('Ctrl Pts',(-110.942983534029,5.74697814347679,
133.153276574838));
#257494=CARTESIAN_POINT('Ctrl Pts',(-111.221431157841,5.08259158390449,
127.238911592946));
#257495=CARTESIAN_POINT('Ctrl Pts',(-111.499878781655,-0.252448342873548,
124.601020082813));
#257496=CARTESIAN_POINT('Ctrl Pts',(-111.778326405467,-5.3555005753377,
127.663695474083));
#257497=CARTESIAN_POINT('Ctrl Pts',(-112.05677402928,-5.53710940981492,
133.612488702192));
#257498=CARTESIAN_POINT('Ctrl Pts',(-112.335221653093,-0.630385199504834,
136.980749405212));
#257499=CARTESIAN_POINT('Ctrl Pts',(-112.613669276906,4.85563221312083,
134.673210545752));
#257500=CARTESIAN_POINT('Ctrl Pts',(-112.892116900719,5.8795608327098,128.810387606114));
#257501=CARTESIAN_POINT('Ctrl Pts',(-113.170564524532,1.50046027955312,
124.779928453004));
#257502=CARTESIAN_POINT('Ctrl Pts',(-113.449012148345,-4.25748996895278,
126.285628149252));
#257503=CARTESIAN_POINT('Ctrl Pts',(-113.727459772158,-6.10301492593933,
131.943822231527));
#257504=CARTESIAN_POINT('Ctrl Pts',(-114.00590739597,-2.3401673148416,136.554906756366));
#257505=CARTESIAN_POINT('Ctrl Pts',(-114.284355019783,3.57317973506622,
135.881520309444));
#257506=CARTESIAN_POINT('Ctrl Pts',(-114.562802643596,6.202949167983,130.542472138726));
#257507=CARTESIAN_POINT('Ctrl Pts',(-114.841250267409,3.13251134643626,
125.444086686097));
#257508=CARTESIAN_POINT('Ctrl Pts',(-115.119697891222,-2.81655137079845,
125.271531112549));
#257509=CARTESIAN_POINT('Ctrl Pts',(-115.398145515035,-6.17734097445314,
130.183375560363));
#257510=CARTESIAN_POINT('Ctrl Pts',(-115.676593138848,-3.86145600246928,
135.665874938939));
#257511=CARTESIAN_POINT('Ctrl Pts',(-115.955040762661,2.00291839317105,
136.680880154352));
#257512=CARTESIAN_POINT('Ctrl Pts',(-116.233488386474,6.02670863349017,
132.295650999397));
#257513=CARTESIAN_POINT('Ctrl Pts',(-116.511936010287,4.51224806071678,
126.539998837124));
#257514=CARTESIAN_POINT('Ctrl Pts',(-116.790383634099,-1.14874804428301,
124.703086825424));
#257515=CARTESIAN_POINT('Ctrl Pts',(-117.068831257912,-5.75410081604829,
128.472947364906));
#257516=CARTESIAN_POINT('Ctrl Pts',(-117.347278881725,-5.07171604131793,
134.385262787713));
#257517=CARTESIAN_POINT('Ctrl Pts',(-117.625726505538,0.271328008281021,
137.006904052952));
#257518=CARTESIAN_POINT('Ctrl Pts',(-117.904174129351,5.3650348733795,133.928710912162));
#257519=CARTESIAN_POINT('Ctrl Pts',(-118.182621753164,5.52853678636705,
127.979392483636));
#257520=CARTESIAN_POINT('Ctrl Pts',(-118.461069376977,0.611583476719488,
124.626081762825));
#257521=CARTESIAN_POINT('Ctrl Pts',(-118.73951700079,-4.86738517051901,
126.95030748382));
#257522=CARTESIAN_POINT('Ctrl Pts',(-119.017964624603,-5.87346463103546,
132.816219753764));
#257523=CARTESIAN_POINT('Ctrl Pts',(-119.296412248415,-1.48211703032935,
136.833331762325));
#257524=CARTESIAN_POINT('Ctrl Pts',(-119.574859872228,4.27122371580729,
135.310113820466));
#257525=CARTESIAN_POINT('Ctrl Pts',(-119.853307496041,6.09951852799569,
129.646328803424));
#257526=CARTESIAN_POINT('Ctrl Pts',(-120.131755119854,2.32265379100196,
125.046718450578));
#257527=CARTESIAN_POINT('Ctrl Pts',(-120.410202743667,-3.58861631197691,
125.738099972737));
#257528=CARTESIAN_POINT('Ctrl Pts',(-120.68865036748,-6.20212333790203,
131.085127526901));
#257529=CARTESIAN_POINT('Ctrl Pts',(-120.967097991293,-3.11618200686478,
136.174144007612));
#257530=CARTESIAN_POINT('Ctrl Pts',(-121.245545615105,2.83337835452712,
136.328591881372));
#257531=CARTESIAN_POINT('Ctrl Pts',(-121.523993238919,6.17920242633619,
131.406541097396));
#257532=CARTESIAN_POINT('Ctrl Pts',(-121.802440862731,3.84664133916317,
125.931115870606));
#257533=CARTESIAN_POINT('Ctrl Pts',(-122.080888486544,-2.02079521982502,
124.933964495032));
#257534=CARTESIAN_POINT('Ctrl Pts',(-122.359336110357,-6.03121969312815,
129.331420371272));
#257535=CARTESIAN_POINT('Ctrl Pts',(-122.63778373417,-4.49924790990888,
135.082436376724));
#257536=CARTESIAN_POINT('Ctrl Pts',(-122.916231357983,1.16731290203685,
136.90210975513));
#257537=CARTESIAN_POINT('Ctrl Pts',(-123.194678981796,5.76117018341619,
133.118249567719));
#257538=CARTESIAN_POINT('Ctrl Pts',(-123.473126605609,5.06079351504635,
127.208038474877));
#257539=CARTESIAN_POINT('Ctrl Pts',(-123.751574229422,-0.290205160143283,
124.602671741062));
#257540=CARTESIAN_POINT('Ctrl Pts',(-124.030021853235,-5.37451947047147,
127.696354115408));
#257541=CARTESIAN_POINT('Ctrl Pts',(-124.308469477047,-5.51991294730918,
133.646142630679));
#257542=CARTESIAN_POINT('Ctrl Pts',(-124.58691710086,-0.592776088308802,
136.984472304668));
#257543=CARTESIAN_POINT('Ctrl Pts',(-124.865364724673,4.87909303712557,
134.64358125345));
#257544=CARTESIAN_POINT('Ctrl Pts',(-125.143812348486,5.86731401838748,
128.774633994209));
#257545=CARTESIAN_POINT('Ctrl Pts',(-125.422259972299,1.46376005097626,
124.770906344175));
#257546=CARTESIAN_POINT('Ctrl Pts',(-125.700707596112,-4.28491789462882,
126.311628420759));
#257547=CARTESIAN_POINT('Ctrl Pts',(-125.979155219925,-6.09596562494584,
131.980951904039));
#257548=CARTESIAN_POINT('Ctrl Pts',(-126.257602843738,-2.30511875041471,
136.569045474729));
#257549=CARTESIAN_POINT('Ctrl Pts',(-126.536050467551,3.60401964443632,
135.859675282198));
#257550=CARTESIAN_POINT('Ctrl Pts',(-126.814498091363,6.20124005219796,
130.50471787872));
#257551=CARTESIAN_POINT('Ctrl Pts',(-127.092945715177,3.09982379940838,
125.42511751388));
#257552=CARTESIAN_POINT('Ctrl Pts',(-127.371393338989,-2.85017909022625,
125.288778770691));
#257553=CARTESIAN_POINT('Ctrl Pts',(-127.649840962802,-6.18100663493216,
130.220990293627));
#257554=CARTESIAN_POINT('Ctrl Pts',(-127.928288586615,-3.83179104109667,
135.689290645038));
#257555=CARTESIAN_POINT('Ctrl Pts',(-128.206736210428,2.03865332610762,
136.6685789433));
#257556=CARTESIAN_POINT('Ctrl Pts',(-128.485183834241,6.03567488037103,
132.258937083203));
#257557=CARTESIAN_POINT('Ctrl Pts',(-128.763631458054,4.48620607868298,
126.512610511197));
#257558=CARTESIAN_POINT('Ctrl Pts',(-129.042079081867,-1.18586694596332,
124.710192623294));
#257559=CARTESIAN_POINT('Ctrl Pts',(-129.32052670568,-5.76818618009069,
128.508017405469));
#257560=CARTESIAN_POINT('Ctrl Pts',(-129.598974329492,-5.04982410627509,
134.416069416958));
#257561=CARTESIAN_POINT('Ctrl Pts',(-129.877421953305,0.30907962358457,
137.005137483589));
#257562=CARTESIAN_POINT('Ctrl Pts',(-130.155869577118,5.38395427874936,
133.895994535135));
#257563=CARTESIAN_POINT('Ctrl Pts',(-130.434317200931,5.51123797253198,
127.945791051148));
#257564=CARTESIAN_POINT('Ctrl Pts',(-130.712764824744,0.573963208500954,
124.622473349811));
#257565=CARTESIAN_POINT('Ctrl Pts',(-130.991212448557,-4.89075570448117,
126.980008045559));
#257566=CARTESIAN_POINT('Ctrl Pts',(-131.26966007237,-5.8611090517438,132.851935924971));
#257567=CARTESIAN_POINT('Ctrl Pts',(-131.548107696183,-1.44538951154951,
136.842242126491));
#257568=CARTESIAN_POINT('Ctrl Pts',(-131.826555319995,4.29857237855583,
135.28403018822));
#257569=CARTESIAN_POINT('Ctrl Pts',(-132.105002943808,6.09235624970348,
129.609220758541));
#257570=CARTESIAN_POINT('Ctrl Pts',(-132.383450567622,2.28756235552218,
125.032686473479));
#257571=CARTESIAN_POINT('Ctrl Pts',(-132.661898191434,-3.6193895897498,
125.760038764874));
#257572=CARTESIAN_POINT('Ctrl Pts',(-132.940345815247,-6.20029931905343,
131.122876410071));
#257573=CARTESIAN_POINT('Ctrl Pts',(-133.21879343906,-3.08343687560774,
136.193013602317));
#257574=CARTESIAN_POINT('Ctrl Pts',(-133.497241062873,2.86695342225543,
136.311241951909));
#257575=CARTESIAN_POINT('Ctrl Pts',(-133.775688686686,6.18275358352724,
131.368915381349));
#257576=CARTESIAN_POINT('Ctrl Pts',(-134.054136310499,3.81690524584148,
125.907790562906));
#257577=CARTESIAN_POINT('Ctrl Pts',(-134.332583934311,-2.05649254658467,
124.946374413949));
#257578=CARTESIAN_POINT('Ctrl Pts',(-134.611031558124,-6.04007415394596,
129.36816140758));
#257579=CARTESIAN_POINT('Ctrl Pts',(-134.889479181937,-4.47312268785726,
135.109745312956));
#257580=CARTESIAN_POINT('Ctrl Pts',(-135.16792680575,1.20441000418008,136.894891013003));
#257581=CARTESIAN_POINT('Ctrl Pts',(-135.446374429563,5.775148741076,133.083136818595));
#257582=CARTESIAN_POINT('Ctrl Pts',(-135.724822053376,5.03880791662344,
127.177298619846));
#257583=CARTESIAN_POINT('Ctrl Pts',(-136.003269677189,-0.327951223754644,
124.604553205172));
#257584=CARTESIAN_POINT('Ctrl Pts',(-136.281717301002,-5.39333921080989,
127.729127925058));
#257585=CARTESIAN_POINT('Ctrl Pts',(-136.560164924815,-5.50251194239939,
133.679691255889));
#257586=CARTESIAN_POINT('Ctrl Pts',(-136.838612548628,-0.555145011576188,
136.987966197812));
#257587=CARTESIAN_POINT('Ctrl Pts',(-137.117060172441,4.90237306454367,
134.613809697415));
#257588=CARTESIAN_POINT('Ctrl Pts',(-137.395507796253,5.8548497885868,128.73895559457));
#257589=CARTESIAN_POINT('Ctrl Pts',(-137.673955420066,1.42700558223168,
124.762107807213));
#257590=CARTESIAN_POINT('Ctrl Pts',(-137.952403043879,-4.3121870410957,
126.33779517211));
#257591=CARTESIAN_POINT('Ctrl Pts',(-138.230850667692,-6.08869043570493,
132.018037977528));
#257592=CARTESIAN_POINT('Ctrl Pts',(-138.509298291505,-2.26998476896503,
136.582970580575));
#257593=CARTESIAN_POINT('Ctrl Pts',(-138.787745915318,3.63472600553235,
135.837642928407));
#257594=CARTESIAN_POINT('Ctrl Pts',(-139.066193539131,6.1993011471828,130.466974722087));
#257595=CARTESIAN_POINT('Ctrl Pts',(-139.344641162943,3.06702138726935,
125.406347671494));
#257596=CARTESIAN_POINT('Ctrl Pts',(-139.623088786757,-2.88370119522,125.306230810748));
#257597=CARTESIAN_POINT('Ctrl Pts',(-139.901536410569,-6.18444325593727,
130.258626643894));
#257598=CARTESIAN_POINT('Ctrl Pts',(-140.179984034382,-3.80198409129777,
135.712525338258));
#257599=CARTESIAN_POINT('Ctrl Pts',(-140.458431658195,2.07431271599591,
136.656060431482));
#257600=CARTESIAN_POINT('Ctrl Pts',(-140.736879282008,6.04441747309895,
132.222169267145));
#257601=CARTESIAN_POINT('Ctrl Pts',(-141.015326905821,4.45999785863389,
126.485381217648));
#257602=CARTESIAN_POINT('Ctrl Pts',(-141.293774529634,-1.22294190490765,
124.717524242802));
#257603=CARTESIAN_POINT('Ctrl Pts',(-141.572222153447,-5.78205780187226,
128.543172537875));
#257604=CARTESIAN_POINT('Ctrl Pts',(-141.85066977726,-5.02774504814366,
134.446742213005));
#257605=CARTESIAN_POINT('Ctrl Pts',(-142.129117401072,0.346819785828787,
137.003141142159));
#257606=CARTESIAN_POINT('Ctrl Pts',(-142.407565024885,5.40267417971275,
133.863163596476));
#257607=CARTESIAN_POINT('Ctrl Pts',(-142.686012648698,5.49373493774783,
127.912295544006));
#257608=CARTESIAN_POINT('Ctrl Pts',(-142.964460272511,0.536321671864061,
124.619094008905));
#257609=CARTESIAN_POINT('Ctrl Pts',(-143.242907896324,-4.91394500969209,
127.00985032009));
#257610=CARTESIAN_POINT('Ctrl Pts',(-143.521355520137,-5.84853628690073,
132.887576222521));
#257611=CARTESIAN_POINT('Ctrl Pts',(-143.79980314395,-1.40860843332932,
136.850928754739));
#257612=CARTESIAN_POINT('Ctrl Pts',(-144.078250767763,4.32576175612421,
135.257780560169));
#257613=CARTESIAN_POINT('Ctrl Pts',(-144.356698391576,6.08496821690962,
129.572157000006));
#257614=CARTESIAN_POINT('Ctrl Pts',(-144.635146015388,2.2523861535788,125.018868367886));
#257615=CARTESIAN_POINT('Ctrl Pts',(-144.913593639201,-3.65002874971022,
125.782164476213));
#257616=CARTESIAN_POINT('Ctrl Pts',(-145.192041263014,-6.19824554583293,
131.160613490521));
#257617=CARTESIAN_POINT('Ctrl Pts',(-145.470488886827,-3.05057748646412,
136.211683518503));
#257618=CARTESIAN_POINT('Ctrl Pts',(-145.74893651064,2.90042225397064,136.293687962933));
#257619=CARTESIAN_POINT('Ctrl Pts',(-146.027384134453,6.18607563651005,
131.33126874552));
#257620=CARTESIAN_POINT('Ctrl Pts',(-146.305831758266,3.78702771569254,
125.884646699409));
#257621=CARTESIAN_POINT('Ctrl Pts',(-146.584279382079,-2.09211366925746,
124.959001402698));
#257622=CARTESIAN_POINT('Ctrl Pts',(-146.862727005891,-6.04870479759444,
129.404955662777));
#257623=CARTESIAN_POINT('Ctrl Pts',(-147.141174629705,-4.4468317125993,
135.136894711575));
#257624=CARTESIAN_POINT('Ctrl Pts',(-147.419622253517,1.24146247646836,
136.887446584034));
#257625=CARTESIAN_POINT('Ctrl Pts',(-147.69806987733,5.78891329847519,133.04793962858));
#257626=CARTESIAN_POINT('Ctrl Pts',(-147.976517501143,5.01663560332014,
127.146693166932));
#257627=CARTESIAN_POINT('Ctrl Pts',(-148.254965124956,-0.365685135012239,
124.606664405427));
#257628=CARTESIAN_POINT('Ctrl Pts',(-148.533412748769,-5.41195909898036,
127.762015688586));
#257629=CARTESIAN_POINT('Ctrl Pts',(-148.811860372582,-5.48490703988586,
133.713133334664));
#257630=CARTESIAN_POINT('Ctrl Pts',(-149.090307996395,-0.517493363741682,
136.991230955176));
#257631=CARTESIAN_POINT('Ctrl Pts',(-149.368755620208,4.92547143272535,
134.583896980843));
#257632=CARTESIAN_POINT('Ctrl Pts',(-149.647203244021,5.84216860517359,
128.703353729273));
#257633=CARTESIAN_POINT('Ctrl Pts',(-149.925650867833,1.39019823527075,
124.753533168151));
#257634=CARTESIAN_POINT('Ctrl Pts',(-150.204098491647,-4.33929639788676,
126.364127433687));
#257635=CARTESIAN_POINT('Ctrl Pts',(-150.482546115459,-6.08118962780021,
132.055079077756));
#257636=CARTESIAN_POINT('Ctrl Pts',(-150.760993739272,-2.23476667239474,
136.596681557904));
#257637=CARTESIAN_POINT('Ctrl Pts',(-151.039441363085,3.66529768052036,
135.81542406449));
#257638=CARTESIAN_POINT('Ctrl Pts',(-151.317888986898,6.19713252478332,
130.429244067412));
#257639=CARTESIAN_POINT('Ctrl Pts',(-151.596336610711,3.03410532552526,
125.387777854462));
#257640=CARTESIAN_POINT('Ctrl Pts',(-151.874784234524,-2.91711644360522,
125.323886586026));
#257641=CARTESIAN_POINT('Ctrl Pts',(-152.153231858337,-6.18765071012318,
130.296283216534));
#257642=CARTESIAN_POINT('Ctrl Pts',(-152.431679482149,-3.77203625758034,
135.735578157629));
#257643=CARTESIAN_POINT('Ctrl Pts',(-152.710127105962,2.10989524146327,
136.643325082775));
#257644=CARTESIAN_POINT('Ctrl Pts',(-152.988574729775,6.0529360877152,132.185348913665));
#257645=CARTESIAN_POINT('Ctrl Pts',(-153.267022353588,4.43362437172323,
126.458311965469));
#257646=CARTESIAN_POINT('Ctrl Pts',(-153.545469977401,-1.25997154729018,
124.725081412269));
#257647=CARTESIAN_POINT('Ctrl Pts',(-153.823917601214,-5.79571516737629,
128.578411459437));
#257648=CARTESIAN_POINT('Ctrl Pts',(-154.102365225027,-5.00547968506979,
134.477280039263));
#257649=CARTESIAN_POINT('Ctrl Pts',(-154.38081284884,0.38454709653853,137.000915102638));
#257650=CARTESIAN_POINT('Ctrl Pts',(-154.659260472653,5.4211938825983,133.830219312748));
#257651=CARTESIAN_POINT('Ctrl Pts',(-154.937708096465,5.47602833059452,
127.8789072034));
#257652=CARTESIAN_POINT('Ctrl Pts',(-155.216155720278,0.498660261630971,
124.615943865326));
#257653=CARTESIAN_POINT('Ctrl Pts',(-155.494603344091,-4.93695222686361,
127.039833201595));
#257654=CARTESIAN_POINT('Ctrl Pts',(-155.773050967904,-5.83574680239484,
132.923139325752));
#257655=CARTESIAN_POINT('Ctrl Pts',(-156.051498591717,-1.37177515860606,
136.85939132518));
#257656=CARTESIAN_POINT('Ctrl Pts',(-156.32994621553,4.3527908409998,135.231365909006));
#257657=CARTESIAN_POINT('Ctrl Pts',(-156.608393839343,6.0773547033811,129.535138901228));
#257658=CARTESIAN_POINT('Ctrl Pts',(-156.886841463156,2.21712648863745,
125.005264645838));
#257659=CARTESIAN_POINT('Ctrl Pts',(-157.165289086968,-3.68053265651321,
125.804476286877));
#257660=CARTESIAN_POINT('Ctrl Pts',(-157.443736710782,-6.19596209434481,
131.19833736989));
#257661=CARTESIAN_POINT('Ctrl Pts',(-157.722184334594,-3.0176050570491,
136.230153064351));
#257662=CARTESIAN_POINT('Ctrl Pts',(-158.000631958407,2.93378360947182,
136.275930564914));
#257663=CARTESIAN_POINT('Ctrl Pts',(-158.27907958222,6.18916846218569,131.293602584915));
#257664=CARTESIAN_POINT('Ctrl Pts',(-158.557527206033,3.7570098558391,125.861685137721));
#257665=CARTESIAN_POINT('Ctrl Pts',(-158.835974829846,-2.12765726788813,
124.971844993383));
#257666=CARTESIAN_POINT('Ctrl Pts',(-159.114422453659,-6.05711130426257,
129.44180177344));
#257667=CARTESIAN_POINT('Ctrl Pts',(-159.392870077472,-4.42037595835707,
135.163883566548));
#257668=CARTESIAN_POINT('Ctrl Pts',(-159.671317701285,1.27846894590735,
136.879776744077));
#257669=CARTESIAN_POINT('Ctrl Pts',(-159.949765325097,5.80246334556346,
133.01265930192));
#257670=CARTESIAN_POINT('Ctrl Pts',(-160.22821294891,4.9942773967397,127.116223250229));
#257671=CARTESIAN_POINT('Ctrl Pts',(-160.506660572723,-0.403405495673234,
124.609005263594));
#257672=CARTESIAN_POINT('Ctrl Pts',(-160.785108196536,-5.43037844501628,
127.795016187323));
#257673=CARTESIAN_POINT('Ctrl Pts',(-161.063555820349,-5.46709889212507,
133.746467627798));
#257674=CARTESIAN_POINT('Ctrl Pts',(-161.342003444162,-0.479822539999598,
136.994266455786));
#257675=CARTESIAN_POINT('Ctrl Pts',(-161.620451067975,4.94838728575097,
134.553844212161));
#257676=CARTESIAN_POINT('Ctrl Pts',(-161.898898691787,5.82927093805496,
128.66782971756));
#257677=CARTESIAN_POINT('Ctrl Pts',(-162.177346315601,1.35333937400316,
124.745182744726));
#257678=CARTESIAN_POINT('Ctrl Pts',(-162.455793939413,-4.36624496045326,
126.390624229737));
#257679=CARTESIAN_POINT('Ctrl Pts',(-162.734241563226,-6.07346347917808,
132.092073832152));
#257680=CARTESIAN_POINT('Ctrl Pts',(-163.012689187039,-2.19946576572379,
136.61017789865));
#257681=CARTESIAN_POINT('Ctrl Pts',(-163.291136810852,3.69573353655413,
135.793019513774));
#257682=CARTESIAN_POINT('Ctrl Pts',(-163.569584434665,6.19473426535967,
130.391527312818));
#257683=CARTESIAN_POINT('Ctrl Pts',(-163.848032058478,3.0010768338922,125.369408750896));
#257684=CARTESIAN_POINT('Ctrl Pts',(-164.126479682291,-2.95042359716811,
125.341745442286));
#257685=CARTESIAN_POINT('Ctrl Pts',(-164.404927306104,-6.19062887863655,
130.333958616169));
#257686=CARTESIAN_POINT('Ctrl Pts',(-164.683374929917,-3.74194864967208,
135.758448248921));
#257687=CARTESIAN_POINT('Ctrl Pts',(-164.961822553729,2.14539958398697,
136.630373369092));
#257688=CARTESIAN_POINT('Ctrl Pts',(-165.240270177542,6.06123040855813,
132.148477387157));
#257689=CARTESIAN_POINT('Ctrl Pts',(-165.518717801355,4.40708659523179,
126.431403757722));
#257690=CARTESIAN_POINT('Ctrl Pts',(-165.797165425168,-1.29695450096345,
124.732863851664));
#257691=CARTESIAN_POINT('Ctrl Pts',(-166.075613048981,-5.80915777052276,
128.613732864363));
#257692=CARTESIAN_POINT('Ctrl Pts',(-166.354060672794,-4.98302884210618,
134.50768176414));
#257693=CARTESIAN_POINT('Ctrl Pts',(-166.632508296607,0.422260157714416,
136.998459447511));
#257694=CARTESIAN_POINT('Ctrl Pts',(-166.91095592042,5.43951270115045,133.797162904712));
#257695=CARTESIAN_POINT('Ctrl Pts',(-167.189403544233,5.45811880719792,
127.845627266545));
#257696=CARTESIAN_POINT('Ctrl Pts',(-167.467851168046,0.460980373357943,
124.613023035806));
#257697=CARTESIAN_POINT('Ctrl Pts',(-167.746298791858,-4.95977650345479,
127.069955579048));
#257698=CARTESIAN_POINT('Ctrl Pts',(-168.024746415672,-5.822741072145,132.958623916859));
#257699=CARTESIAN_POINT('Ctrl Pts',(-168.303194039484,-1.33489105224939,
136.867629524233));
#257700=CARTESIAN_POINT('Ctrl Pts',(-168.581641663297,4.37965863161014,
135.204787213532));
#257701=CARTESIAN_POINT('Ctrl Pts',(-168.86008928711,6.06951599123876,129.498167833929));
#257702=CARTESIAN_POINT('Ctrl Pts',(-169.138536910923,2.18178466725943,
124.991875811423));
#257703=CARTESIAN_POINT('Ctrl Pts',(-169.416984534736,-3.71090017982492,
125.826973370093));
#257704=CARTESIAN_POINT('Ctrl Pts',(-169.695432158549,-6.19344904920226,
131.236046650305));
#257705=CARTESIAN_POINT('Ctrl Pts',(-169.973879782361,-2.98452080916978,
136.248421555465));
#257706=CARTESIAN_POINT('Ctrl Pts',(-170.252327406175,2.96703625254325,
136.257970415857));
#257707=CARTESIAN_POINT('Ctrl Pts',(-170.530775029987,6.19203194594742,
131.25591829527));
#257708=CARTESIAN_POINT('Ctrl Pts',(-170.8092226538,3.72685277860365,125.838906728691));
#257709=CARTESIAN_POINT('Ctrl Pts',(-171.087670277614,-2.16312202539704,
124.984904710079));
#257710=CARTESIAN_POINT('Ctrl Pts',(-171.366117901426,-6.06529336244348,
129.478698374222));
#257711=CARTESIAN_POINT('Ctrl Pts',(-171.644565525239,-4.39375640545797,
135.190710877796));
#257712=CARTESIAN_POINT('Ctrl Pts',(-171.923013149052,1.31542804121008,
136.871881777341));
#257713=CARTESIAN_POINT('Ctrl Pts',(-172.201460772865,5.81579838023838,
132.977297145939));
#257714=CARTESIAN_POINT('Ctrl Pts',(-172.479908396678,4.97173412537368,
127.085889998814));
#257715=CARTESIAN_POINT('Ctrl Pts',(-172.75835602049,-0.441110907994683,
124.611575692932));
#257716=CARTESIAN_POINT('Ctrl Pts',(-173.036803644304,-5.4485965663818,
127.828128198426));
#257717=CARTESIAN_POINT('Ctrl Pts',(-173.315251268116,-5.44908815900415,
133.779692900072));
#257718=CARTESIAN_POINT('Ctrl Pts',(-173.593698891929,-0.442133936257506,
136.997072587158));
#257719=CARTESIAN_POINT('Ctrl Pts',(-173.872146515742,4.97111977446672,
134.523652504987));
#257720=CARTESIAN_POINT('Ctrl Pts',(-174.150594139555,5.81615726515733,
128.632384875785));
#257721=CARTESIAN_POINT('Ctrl Pts',(-174.429041763368,1.31643036424716,
124.737056846366));
#257722=CARTESIAN_POINT('Ctrl Pts',(-174.707489387181,-4.39303173020782,
126.417284578411));
#257723=CARTESIAN_POINT('Ctrl Pts',(-174.985937010994,-6.06551227613263,
132.129020869861));
#257724=CARTESIAN_POINT('Ctrl Pts',(-175.264384634806,-2.16408335703982,
136.623459102702));
#257725=CARTESIAN_POINT('Ctrl Pts',(-175.542832258619,3.72603244582337,
135.770430106468));
#257726=CARTESIAN_POINT('Ctrl Pts',(-175.821279882432,6.19210645777918,
130.353825855915));
#257727=CARTESIAN_POINT('Ctrl Pts',(-176.099727506245,2.96793713625374,
125.351241041473));
#257728=CARTESIAN_POINT('Ctrl Pts',(-176.378175130058,-2.98362142169932,
125.359806717758));
#257729=CARTESIAN_POINT('Ctrl Pts',(-176.656622753871,-6.19337765112022,
130.371651446723));
#257730=CARTESIAN_POINT('Ctrl Pts',(-176.935070377684,-3.71172238248064,
135.781134764673));
#257731=CARTESIAN_POINT('Ctrl Pts',(-177.213518001496,2.18082442793968,
136.617205770365));
#257732=CARTESIAN_POINT('Ctrl Pts',(-177.49196562531,6.06930012827989,132.111556053907));
#257733=CARTESIAN_POINT('Ctrl Pts',(-177.770413249122,4.38038551252508,
126.404657591498));
#257734=CARTESIAN_POINT('Ctrl Pts',(-178.048860872936,-1.33388939551094,
124.740871272604));
#257735=CARTESIAN_POINT('Ctrl Pts',(-178.327308496748,-5.82238511319243,
128.649135443807));
#257736=CARTESIAN_POINT('Ctrl Pts',(-178.605756120561,-4.96039335117553,
134.537946261091));
#257737=CARTESIAN_POINT('Ctrl Pts',(-178.884203744374,0.459957571884186,
136.995774267775));
#257738=CARTESIAN_POINT('Ctrl Pts',(-179.162651368187,5.45762995655925,
133.763995597288));
#257739=CARTESIAN_POINT('Ctrl Pts',(-179.441098991999,5.44000703120181,
127.812456966643));
#257740=CARTESIAN_POINT('Ctrl Pts',(-179.719546615813,0.423283403288203,
124.610331628578));
#257741=CARTESIAN_POINT('Ctrl Pts',(-179.997994239625,-4.98241699370369,
127.100216336253));
#257742=CARTESIAN_POINT('Ctrl Pts',(-180.276441863438,-5.80951957808352,
132.994028680947));
#257743=CARTESIAN_POINT('Ctrl Pts',(-180.554889487251,-1.29795748101432,
136.875643046625));
#257744=CARTESIAN_POINT('Ctrl Pts',(-180.833337111064,4.40636413235919,
135.178045458633));
#257745=CARTESIAN_POINT('Ctrl Pts',(-181.111784734877,6.06145237094964,
129.461245168083));
#257746=CARTESIAN_POINT('Ctrl Pts',(-181.39023235869,2.14636199904753,124.97870236077));
#257747=CARTESIAN_POINT('Ctrl Pts',(-181.668679982503,-3.74113019436597,
125.849654892224));
#257748=CARTESIAN_POINT('Ctrl Pts',(-181.947127606316,-6.19070650352801,
131.273739934436));
#257749=CARTESIAN_POINT('Ctrl Pts',(-182.225575230128,-2.95132596877351,
136.266488314898));
#257750=CARTESIAN_POINT('Ctrl Pts',(-182.504022853942,3.00017895099442,
136.239808181284));
#257751=CARTESIAN_POINT('Ctrl Pts',(-182.782470477755,6.19466598168877,
131.218217272988));
#257752=CARTESIAN_POINT('Ctrl Pts',(-183.060918101567,3.6965576014681,125.81631231638));
#257753=CARTESIAN_POINT('Ctrl Pts',(-183.33936572538,-2.19850662762309,
124.998180068855));
#257754=CARTESIAN_POINT('Ctrl Pts',(-183.617813349193,-6.07325066894868,
129.515644097905));
#257755=CARTESIAN_POINT('Ctrl Pts',(-183.896260973006,-4.36697404029963,
135.217375651221));
#257756=CARTESIAN_POINT('Ctrl Pts',(-184.174708596819,1.35233839284232,
136.863761976378));
#257757=CARTESIAN_POINT('Ctrl Pts',(-184.453156220632,5.8289179083658,132.941854470998));
#257758=CARTESIAN_POINT('Ctrl Pts',(-184.731603844444,4.94900662457131,
127.055694536694));
#257759=CARTESIAN_POINT('Ctrl Pts',(-185.010051468258,-0.478799974789776,
124.614375598192));
#257760=CARTESIAN_POINT('Ctrl Pts',(-185.28849909207,-5.46661278799793,
127.861350494915));
#257761=CARTESIAN_POINT('Ctrl Pts',(-185.566946715884,-5.43087550791776,
133.812807920317));
#257762=CARTESIAN_POINT('Ctrl Pts',(-185.845394339696,-0.404428949079144,
136.999649245311));
#257763=CARTESIAN_POINT('Ctrl Pts',(-186.123841963509,4.99366805651034,
134.493322978084));
#257764=CARTESIAN_POINT('Ctrl Pts',(-186.402289587322,5.80282807241402,
128.59702051737));
#257765=CARTESIAN_POINT('Ctrl Pts',(-186.680737211135,1.27947257368013,
124.729155774178));
#257766=CARTESIAN_POINT('Ctrl Pts',(-186.959184834948,-4.41965571455532,
126.444107491802));
#257767=CARTESIAN_POINT('Ctrl Pts',(-187.237632458761,-6.0573363132998,
132.165918821797));
#257768=CARTESIAN_POINT('Ctrl Pts',(-187.516080082574,-2.12862075745111,
136.636524677919));
#257769=CARTESIAN_POINT('Ctrl Pts',(-187.794527706387,3.75619328558978,
135.74765667963));
#257770=CARTESIAN_POINT('Ctrl Pts',(-188.072975330199,6.18924919941703,
130.316141093742));
#257771=CARTESIAN_POINT('Ctrl Pts',(-188.351422954013,2.93468746061294,
125.333275399398));
#257772=CARTESIAN_POINT('Ctrl Pts',(-188.629870577825,-3.01670868704181,
125.378069743179));
#257773=CARTESIAN_POINT('Ctrl Pts',(-188.908318201638,-6.19589692571743,
130.409360311474));
#257774=CARTESIAN_POINT('Ctrl Pts',(-189.186765825451,-3.68135857605119,
135.80363686423));
#257775=CARTESIAN_POINT('Ctrl Pts',(-189.465213449264,2.21616846064164,
136.603822774524));
#257776=CARTESIAN_POINT('Ctrl Pts',(-189.743661073077,6.07714494785282,
132.07458628205));
#257777=CARTESIAN_POINT('Ctrl Pts',(-190.02210869689,4.35352211302309,126.378074457888));
#257778=CARTESIAN_POINT('Ctrl Pts',(-190.300556320702,-1.37077486229612,
124.749103378371));
#257779=CARTESIAN_POINT('Ctrl Pts',(-190.579003944516,-5.83539670523986,
128.684617885911));
#257780=CARTESIAN_POINT('Ctrl Pts',(-190.857451568328,-4.93757405104588,
134.568072408653));
#257781=CARTESIAN_POINT('Ctrl Pts',(-191.135899192141,0.497637942157669,
136.992859662928));
#257782=CARTESIAN_POINT('Ctrl Pts',(-191.414346815954,5.47554497748281,
133.730718619501));
#257783=CARTESIAN_POINT('Ctrl Pts',(-191.692794439767,5.42169367374449,
127.779397532831));
#257784=CARTESIAN_POINT('Ctrl Pts',(-191.97124206358,0.385570748295746,
124.60786974337));
#257785=CARTESIAN_POINT('Ctrl Pts',(-192.249689687393,-5.00487285865859,
127.130614351886));
#257786=CARTESIAN_POINT('Ctrl Pts',(-192.528137311206,-5.79608281013753,
133.029352306079));
#257787=CARTESIAN_POINT('Ctrl Pts',(-192.806584935019,-1.26097581348702,
136.883431595415));
#257788=CARTESIAN_POINT('Ctrl Pts',(-193.085032558831,4.43290635366497,
135.151141635234));
#257789=CARTESIAN_POINT('Ctrl Pts',(-193.363480182644,6.05316414131348,
129.424372271875));
#257790=CARTESIAN_POINT('Ctrl Pts',(-193.641927806457,2.11085979660312,
124.965744782026));
#257791=CARTESIAN_POINT('Ctrl Pts',(-193.92037543027,-3.77122157995168,
125.872520012798));
#257792=CARTESIAN_POINT('Ctrl Pts',(-194.198823054083,-6.1877345589472,
131.311415825543));
#257793=CARTESIAN_POINT('Ctrl Pts',(-194.477270677896,-2.91802176590892,
136.284352673182));
#257794=CARTESIAN_POINT('Ctrl Pts',(-194.755718301709,3.03321047671203,
136.221444534203));
#257795=CARTESIAN_POINT('Ctrl Pts',(-195.034165925522,6.19707047180361,
131.180500915096));
#257796=CARTESIAN_POINT('Ctrl Pts',(-195.312613549334,3.66612544703105,
125.793902738034));
#257797=CARTESIAN_POINT('Ctrl Pts',(-195.591061173148,-2.23380976337827,
125.011670577786));
#257798=CARTESIAN_POINT('Ctrl Pts',(-195.86950879696,-6.08098292891658,
129.552637575454));
#257799=CARTESIAN_POINT('Ctrl Pts',(-196.147956420774,-4.3400298553121,
135.243876898752));
#257800=CARTESIAN_POINT('Ctrl Pts',(-196.426404044586,1.38919863307876,
136.855417642068));
#257801=CARTESIAN_POINT('Ctrl Pts',(-196.704851668399,5.84182144379631,
132.906332590435));
#257802=CARTESIAN_POINT('Ctrl Pts',(-196.983299292212,4.92609573650846,
127.025637982775));
#257803=CARTESIAN_POINT('Ctrl Pts',(-197.261746916025,-0.516471299475173,
124.617404875624));
#257804=CARTESIAN_POINT('Ctrl Pts',(-197.540194539838,-5.48442644226676,
127.894681845726));
#257805=CARTESIAN_POINT('Ctrl Pts',(-197.81864216365,-5.41246161374207,
133.845811461438));
#257806=CARTESIAN_POINT('Ctrl Pts',(-198.097089787464,-0.36670897563802,
137.001996334766));
#257807=CARTESIAN_POINT('Ctrl Pts',(-198.375537411276,5.01603129634849,
134.462856755322));
#257808=CARTESIAN_POINT('Ctrl Pts',(-198.65398503509,5.78928385374183,128.561737952753));
#257809=CARTESIAN_POINT('Ctrl Pts',(-198.932432658902,1.24246737178614,
124.721479820939));
#257810=CARTESIAN_POINT('Ctrl Pts',(-199.210880282716,-4.44611592693577,
126.471091975977));
#257811=CARTESIAN_POINT('Ctrl Pts',(-199.489327906528,-6.04893589364168,
132.202766320694));
#257812=CARTESIAN_POINT('Ctrl Pts',(-199.767775530341,-2.09307928103787,
136.649374140152));
#257813=CARTESIAN_POINT('Ctrl Pts',(-200.046223154153,3.7862149382325,135.724700077139));
#257814=CARTESIAN_POINT('Ctrl Pts',(-200.324670777967,6.18616259614969,
130.278474422724));
#257815=CARTESIAN_POINT('Ctrl Pts',(-200.603118401779,2.90132903904936,
125.315512490399));
#257816=CARTESIAN_POINT('Ctrl Pts',(-200.881566025592,-3.04968416713424,
125.396533841802));
#257817=CARTESIAN_POINT('Ctrl Pts',(-201.160013649405,-6.1981866090755,
130.447083813107));
#257818=CARTESIAN_POINT('Ctrl Pts',(-201.438461273218,-3.65085835552605,
135.825953713766));
#257819=CARTESIAN_POINT('Ctrl Pts',(-201.716908897031,2.2514303724059,136.590224877478));
#257820=CARTESIAN_POINT('Ctrl Pts',(-201.995356520844,6.08476457658541,
132.037569441512));
#257821=CARTESIAN_POINT('Ctrl Pts',(-202.273804144657,4.32649739215744,
126.35165534194));
#257822=CARTESIAN_POINT('Ctrl Pts',(-202.55225176847,-1.40760953451491,
124.757559863922));
#257823=CARTESIAN_POINT('Ctrl Pts',(-202.830699392283,-5.84819206451709,
128.720178875862));
#257824=CARTESIAN_POINT('Ctrl Pts',(-203.109147016096,-4.91457178729319,
134.59805909049));
#257825=CARTESIAN_POINT('Ctrl Pts',(-203.387594639908,0.535299872273523,
136.989715740974));
#257826=CARTESIAN_POINT('Ctrl Pts',(-203.666042263721,5.49325710007376,
133.697333204442));
#257827=CARTESIAN_POINT('Ctrl Pts',(-203.944489887534,5.40317941343439,
127.746450190138));
#257828=CARTESIAN_POINT('Ctrl Pts',(-204.222937511347,0.347843805837959,
124.605637471411));
#257829=CARTESIAN_POINT('Ctrl Pts',(-204.50138513516,-5.0271432662092,127.161148499539));
#257830=CARTESIAN_POINT('Ctrl Pts',(-204.779832758973,-5.78243126621161,
133.064593483327));
#257831=CARTESIAN_POINT('Ctrl Pts',(-205.058280382786,-1.22394742003769,
136.890994881994));
#257832=CARTESIAN_POINT('Ctrl Pts',(-205.336728006599,4.45928431199552,
135.124076740266));
#257833=CARTESIAN_POINT('Ctrl Pts',(-205.615175630412,6.04465160945437,
129.387550511641));
#257834=CARTESIAN_POINT('Ctrl Pts',(-205.893623254225,2.07527937547198,
124.953003555339));
#257835=CARTESIAN_POINT('Ctrl Pts',(-206.172070878037,-3.80117322153507,
125.89556788454));
#257836=CARTESIAN_POINT('Ctrl Pts',(-206.45051850185,-6.18453332558722,
131.349072927534));
#257837=CARTESIAN_POINT('Ctrl Pts',(-206.728966125663,-2.8846094346739,
136.302013968343));
#257838=CARTESIAN_POINT('Ctrl Pts',(-207.007413749476,3.06612960569919,
136.202880155086));
#257839=CARTESIAN_POINT('Ctrl Pts',(-207.285861373289,6.19924532719362,
131.142770619188));
#257840=CARTESIAN_POINT('Ctrl Pts',(-207.564308997102,3.63555744296752,
125.771678824048));
#257841=CARTESIAN_POINT('Ctrl Pts',(-207.842756620915,-2.26903012449045,
125.025375736976));
#257842=CARTESIAN_POINT('Ctrl Pts',(-208.121204244728,-6.08848985582611,
129.58967743606));
#257843=CARTESIAN_POINT('Ctrl Pts',(-208.399651868541,-4.31292484892225,
135.270213638376));
#257844=CARTESIAN_POINT('Ctrl Pts',(-208.678099492353,1.42600739604885,
136.846849083615));
#257845=CARTESIAN_POINT('Ctrl Pts',(-208.956547116166,5.85450850838505,
132.870732820528));
#257846=CARTESIAN_POINT('Ctrl Pts',(-209.234994739979,4.90300231015654,
126.995721450812));
#257847=CARTESIAN_POINT('Ctrl Pts',(-209.513442363792,-0.554123486127181,
124.620663412976));
#257848=CARTESIAN_POINT('Ctrl Pts',(-209.791889987605,-5.50203686909699,
127.928121015754));
#257849=CARTESIAN_POINT('Ctrl Pts',(-210.070337611418,-5.393847158811,133.878702300482));
#257850=CARTESIAN_POINT('Ctrl Pts',(-210.348785235231,-0.328975413660277,
137.004113768549));
#257851=CARTESIAN_POINT('Ctrl Pts',(-210.627232859043,5.03820866530154,
134.432254965643));
#257852=CARTESIAN_POINT('Ctrl Pts',(-210.905680482857,5.77552511102812,
128.526538489345));
#257853=CARTESIAN_POINT('Ctrl Pts',(-211.184128106669,1.20541612980698,
124.714029271085));
#257854=CARTESIAN_POINT('Ctrl Pts',(-211.462575730482,-4.47241138685473,
126.498237031013));
#257855=CARTESIAN_POINT('Ctrl Pts',(-211.741023354295,-6.04031132844015,
132.239562001151));
#257856=CARTESIAN_POINT('Ctrl Pts',(-212.019470978108,-2.05746024480169,
136.66200701326));
#257857=CARTESIAN_POINT('Ctrl Pts',(-212.297918601921,3.81609629128846,
135.701561149659));
#257858=CARTESIAN_POINT('Ctrl Pts',(-212.576366225734,6.1828467623524,130.240827238612));
#257859=CARTESIAN_POINT('Ctrl Pts',(-212.854813849547,2.86786310767097,
125.297952972686));
#257860=CARTESIAN_POINT('Ctrl Pts',(-213.133261473359,-3.0825466400586,
125.415198329437));
#257861=CARTESIAN_POINT('Ctrl Pts',(-213.411709097173,-6.20024661634941,
130.484820553763));
#257862=CARTESIAN_POINT('Ctrl Pts',(-213.690156720985,-3.62022285110177,
135.848084486325));
#257863=CARTESIAN_POINT('Ctrl Pts',(-213.968604344798,2.28660885659016,
136.576412583105));
#257864=CARTESIAN_POINT('Ctrl Pts',(-214.247051968611,6.09215873212836,
132.00050690397));
#257865=CARTESIAN_POINT('Ctrl Pts',(-214.525499592424,4.29931235134063,
126.325401222624));
#257866=CARTESIAN_POINT('Ctrl Pts',(-214.803947216237,-1.44439204724454,
124.766240415898));
#257867=CARTESIAN_POINT('Ctrl Pts',(-215.08239484005,-5.86077071688603,
128.755817095934));
#257868=CARTESIAN_POINT('Ctrl Pts',(-215.360842463863,-4.89138741227638,
134.627905195436));
#257869=CARTESIAN_POINT('Ctrl Pts',(-215.639290087675,0.572941966656434,
136.986342618411));
#257870=CARTESIAN_POINT('Ctrl Pts',(-215.917737711489,5.51076566800256,
133.66384058922));
#257871=CARTESIAN_POINT('Ctrl Pts',(-216.196185335301,5.38446493632399,
127.713616159441));
#257872=CARTESIAN_POINT('Ctrl Pts',(-216.474632959115,0.310103973899474,
124.603634895418));
#257873=CARTESIAN_POINT('Ctrl Pts',(-216.753080582927,-5.04922739111732,
127.191817647757));
#257874=CARTESIAN_POINT('Ctrl Pts',(-217.031528206741,-5.76856545216855,
133.099750906814));
#257875=CARTESIAN_POINT('Ctrl Pts',(-217.309975830553,-1.18687367276612,
136.898332626102));
#257876=CARTESIAN_POINT('Ctrl Pts',(-217.588423454366,4.48549702990607,
135.096851776628));
#257877=CARTESIAN_POINT('Ctrl Pts',(-217.866871078179,6.03591509080661,
129.350781251827));
#257878=CARTESIAN_POINT('Ctrl Pts',(-218.145318701992,2.03962205410111,
124.94047915284));
#257879=CARTESIAN_POINT('Ctrl Pts',(-218.423766325804,-3.83098400924668,
125.9187976534));
#257880=CARTESIAN_POINT('Ctrl Pts',(-218.702213949618,-6.18110292207006,
131.386709845009));
#257881=CARTESIAN_POINT('Ctrl Pts',(-218.98066157343,-2.85109021317626,
136.319471545938));
#257882=CARTESIAN_POINT('Ctrl Pts',(-219.259109197243,3.09893511812703,
136.18411573184));
#257883=CARTESIAN_POINT('Ctrl Pts',(-219.537556821056,6.20119046726778,
131.105027783371));
#257884=CARTESIAN_POINT('Ctrl Pts',(-219.816004444869,3.6048547219858,125.749641397935));
#257885=CARTESIAN_POINT('Ctrl Pts',(-220.094452068682,-2.30416640585769,
125.039295038577));
#257886=CARTESIAN_POINT('Ctrl Pts',(-220.372899692494,-6.09577117150464,
129.626762307198));
#257887=CARTESIAN_POINT('Ctrl Pts',(-220.651347316308,-4.28566002551621,
135.296384894171));
#257888=CARTESIAN_POINT('Ctrl Pts',(-220.929794940121,1.46276331779004,
136.83805661853));
#257889=CARTESIAN_POINT('Ctrl Pts',(-221.208242563933,5.86697863200795,
132.835056480438));
#257890=CARTESIAN_POINT('Ctrl Pts',(-221.486690187747,4.87972720125093,
126.965946049375));
#257891=CARTESIAN_POINT('Ctrl Pts',(-221.765137811559,-0.591755139529082,
124.624151089502));
#257892=CARTESIAN_POINT('Ctrl Pts',(-222.043585435373,-5.51944341592756,
127.961666765899));
#257893=CARTESIAN_POINT('Ctrl Pts',(-222.322033059185,-5.37503283288975,
133.911479218663));
#257894=CARTESIAN_POINT('Ctrl Pts',(-222.600480682998,-0.29122966137826,
137.006001468201));
#257895=CARTESIAN_POINT('Ctrl Pts',(-222.878928306811,5.06019934158045,
134.401518743003));
#257896=CARTESIAN_POINT('Ctrl Pts',(-223.157375930624,5.7615523541068,128.491423431472));
#257897=CARTESIAN_POINT('Ctrl Pts',(-223.435823554437,1.16832022068962,
124.706804400699));
#257898=CARTESIAN_POINT('Ctrl Pts',(-223.71427117825,-4.49854111992577,
126.525541651043));
#257899=CARTESIAN_POINT('Ctrl Pts',(-223.992718802062,-6.03146293728042,
132.276304499695));
#257900=CARTESIAN_POINT('Ctrl Pts',(-224.271166425875,-2.02176496861996,
136.674422829126));
#257901=CARTESIAN_POINT('Ctrl Pts',(-224.549614049688,3.84583623749284,
135.678240754614));
#257902=CARTESIAN_POINT('Ctrl Pts',(-224.828061673501,6.1793018208946,130.203200936436));
#257903=CARTESIAN_POINT('Ctrl Pts',(-225.106509297314,2.83429090657077,
125.280597496933));
#257904=CARTESIAN_POINT('Ctrl Pts',(-225.384956921127,-3.11529488808334,
125.434062514461));
#257905=CARTESIAN_POINT('Ctrl Pts',(-225.66340454494,-6.20207687120481,
130.522569135094));
#257906=CARTESIAN_POINT('Ctrl Pts',(-225.941852168753,-3.5894531979886,
135.87002836184));
#257907=CARTESIAN_POINT('Ctrl Pts',(-226.220299792565,2.32170260964191,
136.562386403224));
#257908=CARTESIAN_POINT('Ctrl Pts',(-226.498747416378,6.09932714048972,
131.963400042786));
#257909=CARTESIAN_POINT('Ctrl Pts',(-226.777195040191,4.27196799792278,
126.299313072794));
#257910=CARTESIAN_POINT('Ctrl Pts',(-227.055642664004,-1.48112103749588,
124.775144712639));
#257911=CARTESIAN_POINT('Ctrl Pts',(-227.334090287817,-5.87313219624144,
128.79153122554));
#257912=CARTESIAN_POINT('Ctrl Pts',(-227.61253791163,-4.8680217850994,134.65760961753));
#257913=CARTESIAN_POINT('Ctrl Pts',(-227.890985535443,0.610562830463375,
136.982740420231));
#257914=CARTESIAN_POINT('Ctrl Pts',(-228.169433159256,5.52807003248314,
133.630242014917));
#257915=CARTESIAN_POINT('Ctrl Pts',(-228.447880783069,5.36555093588535,
127.680896657417));
#257916=CARTESIAN_POINT('Ctrl Pts',(-228.726328406882,0.272352650944771,
124.601862089598));
#257917=CARTESIAN_POINT('Ctrl Pts',(-229.004776030695,-5.07112441504767,
127.222620660081));
#257918=CARTESIAN_POINT('Ctrl Pts',(-229.283223654507,-5.75448588181141,
133.134823273769));
#257919=CARTESIAN_POINT('Ctrl Pts',(-229.561671278321,-1.14975594545406,
136.905444555836));
#257920=CARTESIAN_POINT('Ctrl Pts',(-229.840118902133,4.51154353607471,
135.069467753152));
#257921=CARTESIAN_POINT('Ctrl Pts',(-230.118566525947,6.0269549091058,129.314065854931));
#257922=CARTESIAN_POINT('Ctrl Pts',(-230.397014149759,2.00388915378425,
124.928172038625));
#257923=CARTESIAN_POINT('Ctrl Pts',(-230.675461773572,-3.86065283843716,
125.942208458593));
#257924=CARTESIAN_POINT('Ctrl Pts',(-230.953909397385,-6.17744347551146,
131.424325183319));
#257925=CARTESIAN_POINT('Ctrl Pts',(-231.232357021197,-2.81746534348149,
136.33672475907));
#257926=CARTESIAN_POINT('Ctrl Pts',(-231.510804645011,3.13162579837364,
136.165151959792));
#257927=CARTESIAN_POINT('Ctrl Pts',(-231.789252268823,6.20290581994918,
131.067273806224));
#257928=CARTESIAN_POINT('Ctrl Pts',(-232.067699892636,3.57401842178686,
125.727791276302));
#257929=CARTESIAN_POINT('Ctrl Pts',(-232.346147516449,-2.33921730549066,
125.053427966802));
#257930=CARTESIAN_POINT('Ctrl Pts',(-232.624595140262,-6.10282660614105,
129.663890814674));
#257931=CARTESIAN_POINT('Ctrl Pts',(-232.903042764075,-4.25823639540172,
135.322389696357));
#257932=CARTESIAN_POINT('Ctrl Pts',(-233.181490387888,1.499465036299,136.829040572621));
#257933=CARTESIAN_POINT('Ctrl Pts',(-233.459938011701,5.87923135258013,
132.799304892167));
#257934=CARTESIAN_POINT('Ctrl Pts',(-233.738385635514,4.85627127225937,
126.9363128818));
#257935=CARTESIAN_POINT('Ctrl Pts',(-234.016833259326,-0.629364865227224,
124.627867775965));
#257936=CARTESIAN_POINT('Ctrl Pts',(-234.29528088314,-5.53664543775268,
127.99531785311));
#257937=CARTESIAN_POINT('Ctrl Pts',(-234.573728506952,-5.35601933315035,
133.944141001422));
#257938=CARTESIAN_POINT('Ctrl Pts',(-234.852176130765,-0.253473117473377,
137.007659363768));
#257939=CARTESIAN_POINT('Ctrl Pts',(-235.130623754578,5.08200251031112,
134.370649226346));
#257940=CARTESIAN_POINT('Ctrl Pts',(-235.409071378391,5.74736610074488,
128.456394080338));
#257941=CARTESIAN_POINT('Ctrl Pts',(-235.687519002204,1.13118101903705,
124.699805477501));
#257942=CARTESIAN_POINT('Ctrl Pts',(-235.965966626017,-4.52450415790052,
126.553004824284));
#257943=CARTESIAN_POINT('Ctrl Pts',(-236.24441424983,-6.0223910480441,132.312992454817));
#257944=CARTESIAN_POINT('Ctrl Pts',(-236.522861873642,-1.98599477519336,
136.686621127679));
#257945=CARTESIAN_POINT('Ctrl Pts',(-236.801309497456,3.87543367482126,
135.654739756147));
#257946=CARTESIAN_POINT('Ctrl Pts',(-237.079757121268,6.1755279031354,130.165596910454));
#257947=CARTESIAN_POINT('Ctrl Pts',(-237.358204745081,2.80061367977841,
125.263446706254));
#257948=CARTESIAN_POINT('Ctrl Pts',(-237.636652368894,-3.14792769771062,
125.453125697856));
#257949=CARTESIAN_POINT('Ctrl Pts',(-237.915099992707,-6.20367730582095,
130.560328158313));
#257950=CARTESIAN_POINT('Ctrl Pts',(-238.19354761652,-3.55855053636696,
135.891784527174));
#257951=CARTESIAN_POINT('Ctrl Pts',(-238.471995240333,2.35671033115007,
136.54814685758));
#257952=CARTESIAN_POINT('Ctrl Pts',(-238.750442864146,6.10626953604027,
131.92625023297));
#257953=CARTESIAN_POINT('Ctrl Pts',(-239.028890487959,4.24446534516054,
126.273391859158));
#257954=CARTESIAN_POINT('Ctrl Pts',(-239.307338111771,-1.51779514426229,
124.784272424193));
#257955=CARTESIAN_POINT('Ctrl Pts',(-239.585785735585,-5.88527604452282,
128.827319941278));
#257956=CARTESIAN_POINT('Ctrl Pts',(-239.864233359397,-4.84447577158576,
134.687171256065));
#257957=CARTESIAN_POINT('Ctrl Pts',(-240.14268098321,0.648161069640796,
136.978909279916));
#257958=CARTESIAN_POINT('Ctrl Pts',(-240.421128607023,5.54516955229552,
133.596538726537));
#257959=CARTESIAN_POINT('Ctrl Pts',(-240.699576230836,5.34643811298351,
127.648292896498));
#257960=CARTESIAN_POINT('Ctrl Pts',(-240.978023854649,0.234591235861842,
124.600319119639));
#257961=CARTESIAN_POINT('Ctrl Pts',(-241.256471478461,-5.09283352659785,
127.253556395099));
#257962=CARTESIAN_POINT('Ctrl Pts',(-241.534919102275,-5.74019307686353,
133.169809284574));
#257963=CARTESIAN_POINT('Ctrl Pts',(-241.813366726087,-1.11259561351327,
136.912330407661));
#257964=CARTESIAN_POINT('Ctrl Pts',(-242.0918143499,4.53742286533832,135.041925684563));
#257965=CARTESIAN_POINT('Ctrl Pts',(-242.370261973713,6.01777139637409,
129.277405681456));
#257966=CARTESIAN_POINT('Ctrl Pts',(-242.648709597526,1.96808199861856,
124.916082668738));
#257967=CARTESIAN_POINT('Ctrl Pts',(-242.927157221339,-3.89017860971679,
125.965799432623));
#257968=CARTESIAN_POINT('Ctrl Pts',(-243.205604845152,-6.1735551215127,
131.461917548614));
#257969=CARTESIAN_POINT('Ctrl Pts',(-243.484052468965,-2.78373607157309,
136.353772968415));
#257970=CARTESIAN_POINT('Ctrl Pts',(-243.762500092778,3.16420043507544,
136.145989541648));
#257971=CARTESIAN_POINT('Ctrl Pts',(-244.040947716591,6.20439132167383,
131.029510086731));
#257972=CARTESIAN_POINT('Ctrl Pts',(-244.319395340403,3.54304968502077,
125.706129268813));
#257973=CARTESIAN_POINT('Ctrl Pts',(-244.597842964216,-2.37418152456686,
125.067773997952));
#257974=CARTESIAN_POINT('Ctrl Pts',(-244.876290588029,-6.10965589829292,
129.701061582678));
#257975=CARTESIAN_POINT('Ctrl Pts',(-245.154738211842,-4.23065497477177,
135.348227081313));
#257976=CARTESIAN_POINT('Ctrl Pts',(-245.433185835655,1.53611119157916,
136.819801279981));
#257977=CARTESIAN_POINT('Ctrl Pts',(-245.711633459468,5.89126621607239,
132.763479380503));
#257978=CARTESIAN_POINT('Ctrl Pts',(-245.990081083281,4.83263539234992,
126.906823046158));
#257979=CARTESIAN_POINT('Ctrl Pts',(-246.268528707094,-0.666951269578287,
124.631813334641));
#257980=CARTESIAN_POINT('Ctrl Pts',(-246.546976330906,-5.55364229714491,
128.029073030433));
#257981=CARTESIAN_POINT('Ctrl Pts',(-246.825423954719,-5.33680736414475,
133.976686438464));
#257982=CARTESIAN_POINT('Ctrl Pts',(-247.103871578532,-0.215707181029578,
137.009087393821));
#257983=CARTESIAN_POINT('Ctrl Pts',(-247.382319202345,5.10361736357064,
134.339647559554));
#257984=CARTESIAN_POINT('Ctrl Pts',(-247.660766826158,5.73296687661779,
128.421451733968));
#257985=CARTESIAN_POINT('Ctrl Pts',(-247.939214449971,1.09399990105564,
124.693032760838));
#257986=CARTESIAN_POINT('Ctrl Pts',(-248.217662073784,-4.55029953871062,
126.580625533077));
#257987=CARTESIAN_POINT('Ctrl Pts',(-248.496109697597,-6.01309599689209,
132.349624507031));
#257988=CARTESIAN_POINT('Ctrl Pts',(-248.77455732141,-1.95015099000055,
136.698601456905));
#257989=CARTESIAN_POINT('Ctrl Pts',(-249.053004945222,3.90488750652966,
135.631059025098));
#257990=CARTESIAN_POINT('Ctrl Pts',(-249.331452569036,6.17152514891849,
130.128016554096));
#257991=CARTESIAN_POINT('Ctrl Pts',(-249.609900192848,2.76683267521693,
125.246501236177));
#257992=CARTESIAN_POINT('Ctrl Pts',(-249.888347816661,-3.18044385971988,
125.472387173231));
#257993=CARTESIAN_POINT('Ctrl Pts',(-250.166795440474,-6.20504786089197,
130.598096224241));
#257994=CARTESIAN_POINT('Ctrl Pts',(-250.445243064287,-3.5275160113489,
135.913352176149));
#257995=CARTESIAN_POINT('Ctrl Pts',(-250.7236906881,2.39163072389511,136.533694473816));
#257996=CARTESIAN_POINT('Ctrl Pts',(-251.002138311913,6.11298566151878,
131.889058851139));
#257997=CARTESIAN_POINT('Ctrl Pts',(-251.280585935725,4.21680541219097,
126.247638542206));
#257998=CARTESIAN_POINT('Ctrl Pts',(-251.559033559539,-1.5544130086051,
124.793623212388));
#257999=CARTESIAN_POINT('Ctrl Pts',(-251.837481183351,-5.89720181167361,
128.863181916876));
#258000=CARTESIAN_POINT('Ctrl Pts',(-252.115928807165,-4.82075024435922,
134.716589015834));
#258001=CARTESIAN_POINT('Ctrl Pts',(-252.394376430977,0.685735291195708,
136.974849339035));
#258002=CARTESIAN_POINT('Ctrl Pts',(-252.67282405479,5.56206359338632,133.562731973716));
#258003=CARTESIAN_POINT('Ctrl Pts',(-252.951271678603,5.32712717665345,
127.615806083426));
#258004=CARTESIAN_POINT('Ctrl Pts',(-253.229719302416,0.196821126400439,
124.599006045371));
#258005=CARTESIAN_POINT('Ctrl Pts',(-253.508166926229,-5.11435391846912,
127.284623701469));
#258006=CARTESIAN_POINT('Ctrl Pts',(-253.786614550041,-5.72568757235024,
133.204707652256));
#258007=CARTESIAN_POINT('Ctrl Pts',(-254.065062173855,-1.07539404373626,
136.918989908584));
#258008=CARTESIAN_POINT('Ctrl Pts',(-254.343509797667,4.56313403947717,
135.014226625117));
#258009=CARTESIAN_POINT('Ctrl Pts',(-254.621957421481,6.00836492926231,
129.240802026269));
#258010=CARTESIAN_POINT('Ctrl Pts',(-254.900405045293,1.9322018468105,124.904211611225));
#258011=CARTESIAN_POINT('Ctrl Pts',(-255.178852669106,-3.91956009939235,
125.989569474605));
#258012=CARTESIAN_POINT('Ctrl Pts',(-255.457300292919,-6.16943824888009,
131.499485975975));
#258013=CARTESIAN_POINT('Ctrl Pts',(-255.735747916732,-2.74990318521692,
136.370614733943));
#258014=CARTESIAN_POINT('Ctrl Pts',(-256.014195540545,3.19665694865877,
136.126630713714));
#258015=CARTESIAN_POINT('Ctrl Pts',(-256.292643164358,6.20564856486739,
130.991735142402));
#258016=CARTESIAN_POINT('Ctrl Pts',(-256.571090788171,3.51194654848645,
125.68466161966));
#258017=CARTESIAN_POINT('Ctrl Pts',(-256.849538411983,-2.40905189372645,
125.082322325773));
#258018=CARTESIAN_POINT('Ctrl Pts',(-257.127986035797,-6.11626988572704,
129.738292634474));
#258019=CARTESIAN_POINT('Ctrl Pts',(-257.406433659609,-4.20289584392431,
135.373859459261));
#258020=CARTESIAN_POINT('Ctrl Pts',(-257.684881283423,1.57266088340656,
136.810408252432));
#258021=CARTESIAN_POINT('Ctrl Pts',(-257.963328907235,5.90315744058412,
132.727450666138));
#258022=CARTESIAN_POINT('Ctrl Pts',(-258.241776531048,4.80867945501638,
126.87772425425));
#258023=CARTESIAN_POINT('Ctrl Pts',(-258.520224154861,-0.704246744852541,
124.635521896935));
#258024=CARTESIAN_POINT('Ctrl Pts',(-258.798671778674,-5.5709361272427,
128.063810879205));
#258025=CARTESIAN_POINT('Ctrl Pts',(-259.077119402487,-5.31644754243966,
134.007449313497));
#258026=CARTESIAN_POINT('Ctrl Pts',(-259.355567026299,-0.179733571114533,
137.013459703814));
#258027=CARTESIAN_POINT('Ctrl Pts',(-259.634014650113,5.12849404027147,
134.30227331953));
#258028=CARTESIAN_POINT('Ctrl Pts',(-259.866054336623,5.61428989304695,
129.384066440553));
#258029=CARTESIAN_POINT('Ctrl Pts',(-260.051696012132,3.39054283699284,
126.521203045511));
#258030=CARTESIAN_POINT('Ctrl Pts',(-260.144521813036,1.754921961264,125.780753115897));
#258031=CARTESIAN_POINT('Ctrl Pts',(-260.190939676638,0.892893391295023,
125.631947563271));
#258032=CARTESIAN_POINT('Ctrl Pts',(210.191733024964,-2.43880115184907,
125.780342085335));
#258033=CARTESIAN_POINT('Ctrl Pts',(210.145323348611,-3.27594855749458,
126.186716565447));
#258034=CARTESIAN_POINT('Ctrl Pts',(210.052505734956,-4.72940422381435,
127.426013481475));
#258035=CARTESIAN_POINT('Ctrl Pts',(209.866872246696,-6.15821517169733,
131.008352419918));
#258036=CARTESIAN_POINT('Ctrl Pts',(209.634832560185,-4.21099667891447,
135.892791108304));
#258037=CARTESIAN_POINT('Ctrl Pts',(209.356384936373,2.01508446636645,137.098708070195));
#258038=CARTESIAN_POINT('Ctrl Pts',(209.07793731256,6.37956871319657,132.510708806665));
#258039=CARTESIAN_POINT('Ctrl Pts',(208.799489688747,4.8866719183268,126.359661034021));
#258040=CARTESIAN_POINT('Ctrl Pts',(208.521042064934,-1.09954563679898,
124.290443595948));
#258041=CARTESIAN_POINT('Ctrl Pts',(208.242594441121,-6.07390144970816,
128.208589139036));
#258042=CARTESIAN_POINT('Ctrl Pts',(207.964146817309,-5.46739734855352,
134.511385201899));
#258043=CARTESIAN_POINT('Ctrl Pts',(207.685699193495,0.163779660617915,
137.407996874876));
#258044=CARTESIAN_POINT('Ctrl Pts',(207.407251569682,5.6442383477931,134.235982835808));
#258045=CARTESIAN_POINT('Ctrl Pts',(207.128803945869,5.93803043711477,127.910585036422));
#258046=CARTESIAN_POINT('Ctrl Pts',(206.850356322057,0.775002953389061,
124.244367681185));
#258047=CARTESIAN_POINT('Ctrl Pts',(206.571908698243,-5.10018277131114,
126.606494049502));
#258048=CARTESIAN_POINT('Ctrl Pts',(206.293461074431,-6.28856642889766,
132.82623846394));
#258049=CARTESIAN_POINT('Ctrl Pts',(206.015013450618,-1.69805588527783,
137.187984519302));
#258050=CARTESIAN_POINT('Ctrl Pts',(205.736565826805,4.45288036648484,135.683487507757));
#258051=CARTESIAN_POINT('Ctrl Pts',(205.458118202992,6.51183958365415,129.695313656966));
#258052=CARTESIAN_POINT('Ctrl Pts',(205.179670579179,2.58673502741873,124.726298504418));
#258053=CARTESIAN_POINT('Ctrl Pts',(204.901222955366,-3.71545195245463,
125.342726181157));
#258054=CARTESIAN_POINT('Ctrl Pts',(204.622775331554,-6.60332046735468,
130.978128730661));
#258055=CARTESIAN_POINT('Ctrl Pts',(204.344327707741,-3.42305986725146,
136.4538470632));
#258056=CARTESIAN_POINT('Ctrl Pts',(204.065880083927,2.90282542147133,136.737963244372));
#258057=CARTESIAN_POINT('Ctrl Pts',(203.787432460115,6.56115601364161,131.569388537382));
#258058=CARTESIAN_POINT('Ctrl Pts',(203.508984836302,4.1901047305044,125.69779051756));
#258059=CARTESIAN_POINT('Ctrl Pts',(203.230537212489,-2.03144808657932,
124.518880964767));
#258060=CARTESIAN_POINT('Ctrl Pts',(202.952089588676,-6.38619936200403,
129.116020142231));
#258061=CARTESIAN_POINT('Ctrl Pts',(202.673641964863,-4.87234540261322,
135.2646617407));
#258062=CARTESIAN_POINT('Ctrl Pts',(202.39519434105,1.1189559521872,137.314504502614));
#258063=CARTESIAN_POINT('Ctrl Pts',(202.116746717238,6.08199145217563,133.381843073553));
#258064=CARTESIAN_POINT('Ctrl Pts',(201.838299093424,5.45597392877388,127.080601183836));
#258065=CARTESIAN_POINT('Ctrl Pts',(201.559851469612,-0.183817095687214,
124.201312298284));
#258066=CARTESIAN_POINT('Ctrl Pts',(201.281403845799,-5.65468918935595,
127.389902241135));
#258067=CARTESIAN_POINT('Ctrl Pts',(201.002956221986,-5.92917816483575,
133.716212626452));
#258068=CARTESIAN_POINT('Ctrl Pts',(200.724508598173,-0.755042063338292,
137.366673267433));
#258069=CARTESIAN_POINT('Ctrl Pts',(200.44606097436,5.11294080853837,134.986689170007));
#258070=CARTESIAN_POINT('Ctrl Pts',(200.167613350547,6.2823808583988,128.763349450982));
#258071=CARTESIAN_POINT('Ctrl Pts',(199.889165726734,1.67861981076543,124.415599285115));
#258072=CARTESIAN_POINT('Ctrl Pts',(199.610718102921,-4.46771083782862,
125.938808675424));
#258073=CARTESIAN_POINT('Ctrl Pts',(199.332270479108,-6.50843348626435,
131.933222605136));
#258074=CARTESIAN_POINT('Ctrl Pts',(199.053822855296,-2.56822371547623,
136.890267516244));
#258075=CARTESIAN_POINT('Ctrl Pts',(198.775375231483,3.73205818513161,136.254661300547));
#258076=CARTESIAN_POINT('Ctrl Pts',(198.49692760767,6.60276093478139,130.610495019181));
#258077=CARTESIAN_POINT('Ctrl Pts',(198.218479983857,3.4058489481713,125.14448175187));
#258078=CARTESIAN_POINT('Ctrl Pts',(197.940032360044,-2.92087183683725,
124.879620661678));
#258079=CARTESIAN_POINT('Ctrl Pts',(197.661584736231,-6.56345409631434,
130.05930615131));
#258080=CARTESIAN_POINT('Ctrl Pts',(197.383137112418,-4.1745426838368,135.923660297497));
#258081=CARTESIAN_POINT('Ctrl Pts',(197.104689488605,2.05056951733907,137.083628129519));
#258082=CARTESIAN_POINT('Ctrl Pts',(196.826241864792,6.39130850797037,132.473255877329));
#258083=CARTESIAN_POINT('Ctrl Pts',(196.54779424098,4.85874721255563,126.329250411482));
#258084=CARTESIAN_POINT('Ctrl Pts',(196.269346617166,-1.13876540820057,
124.297652603739));
#258085=CARTESIAN_POINT('Ctrl Pts',(195.990898993354,-6.0898082506034,128.245401590344));
#258086=CARTESIAN_POINT('Ctrl Pts',(195.712451369541,-5.44461481437399,
134.544708910868));
#258087=CARTESIAN_POINT('Ctrl Pts',(195.434003745728,0.203913652044436,
137.406818876019));
#258088=CARTESIAN_POINT('Ctrl Pts',(195.155556121915,5.66505543396973,134.201592249669));
#258089=CARTESIAN_POINT('Ctrl Pts',(194.877108498102,5.92028802542049,127.874475717408));
#258090=CARTESIAN_POINT('Ctrl Pts',(194.59866087429,0.735065143658737,124.239780275557));
#258091=CARTESIAN_POINT('Ctrl Pts',(194.320213250476,-5.1256466951968,126.637613470433));
#258092=CARTESIAN_POINT('Ctrl Pts',(194.041765626664,-6.2761396229282,132.86448373661));
#258093=CARTESIAN_POINT('Ctrl Pts',(193.763318002851,-1.6591668436545,137.198201498994));
#258094=CARTESIAN_POINT('Ctrl Pts',(193.484870379038,4.48249921013125,135.656291847837));
#258095=CARTESIAN_POINT('Ctrl Pts',(193.206422755225,6.50496747206681,129.655694426079));
#258096=CARTESIAN_POINT('Ctrl Pts',(192.927975131412,2.54968841250072,124.710665118833));
#258097=CARTESIAN_POINT('Ctrl Pts',(192.649527507599,-3.74862973894988,
125.365444281348));
#258098=CARTESIAN_POINT('Ctrl Pts',(192.371079883787,-6.60214029104917,
131.018321851013));
#258099=CARTESIAN_POINT('Ctrl Pts',(192.092632259973,-3.38860644815819,
136.474579499726));
#258100=CARTESIAN_POINT('Ctrl Pts',(191.814184636161,2.93889117796205,136.720183001327));
#258101=CARTESIAN_POINT('Ctrl Pts',(191.535737012347,6.56569138435095,131.529434736241));
#258102=CARTESIAN_POINT('Ctrl Pts',(191.257289388535,4.15894196037717,125.672378777932));
#258103=CARTESIAN_POINT('Ctrl Pts',(190.978841764722,-2.06967194957323,
124.531363418996));
#258104=CARTESIAN_POINT('Ctrl Pts',(190.700394140909,-6.3963584469616,129.154926032595));
#258105=CARTESIAN_POINT('Ctrl Pts',(190.421946517096,-4.84510401107414,
135.294238450423));
#258106=CARTESIAN_POINT('Ctrl Pts',(190.143498893283,1.15856431450073,137.307572482581));
#258107=CARTESIAN_POINT('Ctrl Pts',(189.86505126947,6.09756863406271,133.344772510351));
#258108=CARTESIAN_POINT('Ctrl Pts',(189.586603645657,5.4332052617092,127.047458114672));
#258109=CARTESIAN_POINT('Ctrl Pts',(189.308156021844,-0.224008319322015,
124.202553584261));
#258110=CARTESIAN_POINT('Ctrl Pts',(189.029708398032,-5.67536919831109,
127.424387201254));
#258111=CARTESIAN_POINT('Ctrl Pts',(188.751260774218,-5.91134304125131,
133.752251266956));
#258112=CARTESIAN_POINT('Ctrl Pts',(188.472813150406,-0.71508141444371,
137.371147838333));
#258113=CARTESIAN_POINT('Ctrl Pts',(188.194365526593,5.13830509856852,134.955487759214));
#258114=CARTESIAN_POINT('Ctrl Pts',(187.91591790278,6.26984024615536,128.725144630756));
#258115=CARTESIAN_POINT('Ctrl Pts',(187.637470278967,1.63969850624965,124.405499418827));
#258116=CARTESIAN_POINT('Ctrl Pts',(187.359022655154,-4.49724605717418,
125.966095046791));
#258117=CARTESIAN_POINT('Ctrl Pts',(187.080575031341,-6.5014411967389,131.972820371883));
#258118=CARTESIAN_POINT('Ctrl Pts',(186.802127407528,-2.53112948956026,
136.905788265189));
#258119=CARTESIAN_POINT('Ctrl Pts',(186.523679783716,3.76516656597443,136.231842221641));
#258120=CARTESIAN_POINT('Ctrl Pts',(186.245232159903,6.60145848599114,130.570305731164));
#258121=CARTESIAN_POINT('Ctrl Pts',(185.96678453609,3.3713325565579,125.123854247073));
#258122=CARTESIAN_POINT('Ctrl Pts',(185.688336912277,-2.95688329360047,
124.897510609301));
#258123=CARTESIAN_POINT('Ctrl Pts',(185.409889288464,-6.5678678487195,130.099273563458));
#258124=CARTESIAN_POINT('Ctrl Pts',(185.131441664651,-4.14330270904733,
135.948977074923));
#258125=CARTESIAN_POINT('Ctrl Pts',(184.852994040838,2.08875520864929,137.071029390563));
#258126=CARTESIAN_POINT('Ctrl Pts',(184.574546417025,6.40134913096194,132.434319247607));
#258127=CARTESIAN_POINT('Ctrl Pts',(184.296098793212,4.831415925211,126.299756751549));
#258128=CARTESIAN_POINT('Ctrl Pts',(184.017651169399,-1.17835248801931,
124.304705146227));
#258129=CARTESIAN_POINT('Ctrl Pts',(183.739203545587,-6.10527253047917,
128.282519393244));
#258130=CARTESIAN_POINT('Ctrl Pts',(183.460755921774,-5.42174537657308,
134.577782526619));
#258131=CARTESIAN_POINT('Ctrl Pts',(183.182308297961,0.244100911417136,
137.405455267482));
#258132=CARTESIAN_POINT('Ctrl Pts',(182.903860674148,5.68563038680749,134.167044506474));
#258133=CARTESIAN_POINT('Ctrl Pts',(182.625413050335,5.90234329520773,127.838491527799));
#258134=CARTESIAN_POINT('Ctrl Pts',(182.346965426522,0.695091060812155,
124.23542735186));
#258135=CARTESIAN_POINT('Ctrl Pts',(182.068517802709,-5.15091590138369,
126.668891936874));
#258136=CARTESIAN_POINT('Ctrl Pts',(181.790070178896,-6.263482786439,132.902650210566));
#258137=CARTESIAN_POINT('Ctrl Pts',(181.511622555083,-1.62021497890189,
137.208182855437));
#258138=CARTESIAN_POINT('Ctrl Pts',(181.233174931271,4.51195124234396,135.628915707812));
#258139=CARTESIAN_POINT('Ctrl Pts',(180.954727307458,6.49785469294791,129.61611812487));
#258140=CARTESIAN_POINT('Ctrl Pts',(180.676279683645,2.51254711858197,124.695257343842));
#258141=CARTESIAN_POINT('Ctrl Pts',(180.397832059832,-3.78166851301026,
125.388364025079));
#258142=CARTESIAN_POINT('Ctrl Pts',(180.119384436019,-6.60071552592353,
131.058506988669));
#258143=CARTESIAN_POINT('Ctrl Pts',(179.840936812206,-3.35402743339335,
136.495101852955));
#258144=CARTESIAN_POINT('Ctrl Pts',(179.562489188393,2.97484801707599,136.702183530083));
#258145=CARTESIAN_POINT('Ctrl Pts',(179.28404156458,6.56998346925752,131.489454075275));
#258146=CARTESIAN_POINT('Ctrl Pts',(179.005593940767,4.12762507472721,125.647157201507));
#258147=CARTESIAN_POINT('Ctrl Pts',(178.727146316955,-2.10781911778238,
124.544078323705));
#258148=CARTESIAN_POINT('Ctrl Pts',(178.448698693142,-6.40628051373842,
129.193893042167));
#258149=CARTESIAN_POINT('Ctrl Pts',(178.170251069329,-4.81768308177075,
135.323648786705));
#258150=CARTESIAN_POINT('Ctrl Pts',(177.891803445516,1.19812974544141,137.300399483306));
#258151=CARTESIAN_POINT('Ctrl Pts',(177.613355821703,6.11291986848493,133.307607811431));
#258152=CARTESIAN_POINT('Ctrl Pts',(177.33490819789,5.41023526512845,127.014454258818));
#258153=CARTESIAN_POINT('Ctrl Pts',(177.056460574078,-0.264191242194762,
124.204039502676));
#258154=CARTESIAN_POINT('Ctrl Pts',(176.778012950264,-5.69583890440069,
127.458997407505));
#258155=CARTESIAN_POINT('Ctrl Pts',(176.499565326452,-5.89328887066216,
133.788180672302));
#258156=CARTESIAN_POINT('Ctrl Pts',(176.221117702638,-0.675094267951971,
137.375379074508));
#258157=CARTESIAN_POINT('Ctrl Pts',(175.942670078826,5.16347898681764,134.924132526884));
#258158=CARTESIAN_POINT('Ctrl Pts',(175.664222455013,6.25706730267374,128.687016856641));
#258159=CARTESIAN_POINT('Ctrl Pts',(175.3857748312,1.60071644210391,124.395636664696));
#258160=CARTESIAN_POINT('Ctrl Pts',(175.107327207387,-4.5266146294138,125.993560701866));
#258161=CARTESIAN_POINT('Ctrl Pts',(174.828879583574,-6.49420799391872,
132.012374840923));
#258162=CARTESIAN_POINT('Ctrl Pts',(174.550431959762,-2.49394147171037,
136.92108292349));
#258163=CARTESIAN_POINT('Ctrl Pts',(174.271984335948,3.79813542718566,136.208822025409));
#258164=CARTESIAN_POINT('Ctrl Pts',(173.993536712136,6.59991141772898,130.530125116137));
#258165=CARTESIAN_POINT('Ctrl Pts',(173.715089088322,3.33669123897678,125.103437235529));
#258166=CARTESIAN_POINT('Ctrl Pts',(173.43664146451,-2.99278518196597,124.915619437422));
#258167=CARTESIAN_POINT('Ctrl Pts',(173.158193840697,-6.5720382263662,130.139267102866));
#258168=CARTESIAN_POINT('Ctrl Pts',(172.879746216884,-4.11190920265221,
135.974103216695));
#258169=CARTESIAN_POINT('Ctrl Pts',(172.601298593071,2.12686350036709,137.058198437889));
#258170=CARTESIAN_POINT('Ctrl Pts',(172.322850969258,6.41115254960738,132.395322219168));
#258171=CARTESIAN_POINT('Ctrl Pts',(172.044403345445,4.80390560797255,126.270430011369));
#258172=CARTESIAN_POINT('Ctrl Pts',(171.765955721632,-1.21789590355323,
124.31199853584));
#258173=CARTESIAN_POINT('Ctrl Pts',(171.487508097819,-6.12051057723618,
128.319730643897));
#258174=CARTESIAN_POINT('Ctrl Pts',(171.209060474007,-5.39867503400336,
134.610716316833));
#258175=CARTESIAN_POINT('Ctrl Pts',(170.930612850193,0.284279125540913,
137.403847052956));
#258176=CARTESIAN_POINT('Ctrl Pts',(170.652165226381,5.70599465652041,134.13237215779));
#258177=CARTESIAN_POINT('Ctrl Pts',(170.373717602568,5.88417985149351,127.802617239562));
#258178=CARTESIAN_POINT('Ctrl Pts',(170.095269978755,0.655091221110643,
124.231317842401));
#258179=CARTESIAN_POINT('Ctrl Pts',(169.816822354942,-5.17599423848763,
126.700323644626));
#258180=CARTESIAN_POINT('Ctrl Pts',(169.538374731129,-6.25059385429175,
132.940738931629));
#258181=CARTESIAN_POINT('Ctrl Pts',(169.259927107316,-1.58120307648749,
137.217926915891));
#258182=CARTESIAN_POINT('Ctrl Pts',(168.981479483503,4.54123608254409,135.601360792124));
#258183=CARTESIAN_POINT('Ctrl Pts',(168.703031859691,6.49050113343381,129.576585854424));
#258184=CARTESIAN_POINT('Ctrl Pts',(168.424584235878,2.47531272130571,124.680075943919));
#258185=CARTESIAN_POINT('Ctrl Pts',(168.146136612065,-3.81456715595326,
125.411484460556));
#258186=CARTESIAN_POINT('Ctrl Pts',(167.867688988252,-6.59904616885666,
131.098682708838));
#258187=CARTESIAN_POINT('Ctrl Pts',(167.589241364439,-3.31932413390846,
136.515413333674));
#258188=CARTESIAN_POINT('Ctrl Pts',(167.310793740626,3.01069462210276,136.683965512842));
#258189=CARTESIAN_POINT('Ctrl Pts',(167.032346116813,6.57403210101054,131.449448027918));
#258190=CARTESIAN_POINT('Ctrl Pts',(166.753898493,4.09615523841214,125.622126727152));
#258191=CARTESIAN_POINT('Ctrl Pts',(166.475450869187,-2.14588817997888,
124.557025205477));
#258192=CARTESIAN_POINT('Ctrl Pts',(166.197003245374,-6.41596519343492,
129.232919728208));
#258193=CARTESIAN_POINT('Ctrl Pts',(165.918555621562,-4.79008363144905,
135.352891659104));
#258194=CARTESIAN_POINT('Ctrl Pts',(165.640107997748,1.23765077924384,137.292985770921));
#258195=CARTESIAN_POINT('Ctrl Pts',(165.361660373936,6.12804458641347,133.270350353765));
#258196=CARTESIAN_POINT('Ctrl Pts',(165.083212750123,5.38706479029029,126.981590839339));
#258197=CARTESIAN_POINT('Ctrl Pts',(164.80476512631,-0.304364375363971,
124.205769998417));
#258198=CARTESIAN_POINT('Ctrl Pts',(164.526317502497,-5.71609754908509,
127.493731577419));
#258199=CARTESIAN_POINT('Ctrl Pts',(164.247869878684,-5.8750163220866,133.823999511097));
#258200=CARTESIAN_POINT('Ctrl Pts',(163.969422254871,-0.635082105593798,
137.37936681918));
#258201=CARTESIAN_POINT('Ctrl Pts',(163.690974631059,5.18846154045405,134.892624634889));
#258202=CARTESIAN_POINT('Ctrl Pts',(163.412527007245,6.24406250126218,128.648967541478));
#258203=CARTESIAN_POINT('Ctrl Pts',(163.134079383433,1.56167506282176,124.386011388187));
#258204=CARTESIAN_POINT('Ctrl Pts',(162.85563175962,-4.55581546628373,126.021204622902));
#258205=CARTESIAN_POINT('Ctrl Pts',(162.577184135807,-6.48673414583306,
132.051884546553));
#258206=CARTESIAN_POINT('Ctrl Pts',(162.298736511994,-2.45666103994207,
136.936150924396));
#258207=CARTESIAN_POINT('Ctrl Pts',(162.020288888181,3.83096354709181,136.185601564872));
#258208=CARTESIAN_POINT('Ctrl Pts',(161.741841264368,6.59811978732212,130.489954663008));
#258209=CARTESIAN_POINT('Ctrl Pts',(161.463393640556,3.30192627907479,125.083231473798));
#258210=CARTESIAN_POINT('Ctrl Pts',(161.184946016742,-3.02857617157586,
124.933946475014));
#258211=CARTESIAN_POINT('Ctrl Pts',(160.90649839293,-6.57596507471956,130.179285287561));
#258212=CARTESIAN_POINT('Ctrl Pts',(160.628050769116,-4.08036332794952,
135.999037791754));
#258213=CARTESIAN_POINT('Ctrl Pts',(160.349603145304,2.16489298037573,137.045135746957));
#258214=CARTESIAN_POINT('Ctrl Pts',(160.07115552149,6.42071840063739,132.356266237063));
#258215=CARTESIAN_POINT('Ctrl Pts',(159.792707897678,4.77621728024515,126.241271277656));
#258216=CARTESIAN_POINT('Ctrl Pts',(159.514260273865,-1.25739418950663,
124.319532502318));
#258217=CARTESIAN_POINT('Ctrl Pts',(159.235812650052,-6.13552182622286,
128.357033963427));
#258218=CARTESIAN_POINT('Ctrl Pts',(158.957365026239,-5.37540464154493,
134.643509061136));
#258219=CARTESIAN_POINT('Ctrl Pts',(158.678917402427,0.324446805597038,
137.401994292032));
#258220=CARTESIAN_POINT('Ctrl Pts',(158.400469778613,5.72614748850293,134.097576488416));
#258221=CARTESIAN_POINT('Ctrl Pts',(158.122022154801,5.86579836733105,127.766854182028));
#258222=CARTESIAN_POINT('Ctrl Pts',(157.843574530988,0.615067106763091,
124.22745189946));
#258223=CARTESIAN_POINT('Ctrl Pts',(157.565126907175,-5.20088077722156,
126.731907428977));
#258224=CARTESIAN_POINT('Ctrl Pts',(157.286679283362,-6.23747330409059,
132.978748488409));
#258225=CARTESIAN_POINT('Ctrl Pts',(157.008231659549,-1.54213258201158,
137.227433319288));
#258226=CARTESIAN_POINT('Ctrl Pts',(156.729784035736,4.5703526455712,135.57362812183));
#258227=CARTESIAN_POINT('Ctrl Pts',(156.451336411923,6.48290706601333,129.537099079623));
#258228=CARTESIAN_POINT('Ctrl Pts',(156.172888788111,2.43798660040623,124.665121481617));
#258229=CARTESIAN_POINT('Ctrl Pts',(155.894441164297,-3.84732444870741,
125.434804731043));
#258230=CARTESIAN_POINT('Ctrl Pts',(155.615993540485,-6.59713228170722,
131.138847522794));
#258231=CARTESIAN_POINT('Ctrl Pts',(155.337545916672,-3.28449783564716,
136.535513189234));
#258232=CARTESIAN_POINT('Ctrl Pts',(155.059098292859,3.04642966473303,136.665529624679));
#258233=CARTESIAN_POINT('Ctrl Pts',(154.780650669046,6.57783712958646,131.409418076611));
#258234=CARTESIAN_POINT('Ctrl Pts',(154.502203045233,4.06453361755842,125.597288282381));
#258235=CARTESIAN_POINT('Ctrl Pts',(154.22375542142,-2.18387772549973,124.57020358456));
#258236=CARTESIAN_POINT('Ctrl Pts',(153.945307797607,-6.42541212718171,
129.272004644569));
#258237=CARTESIAN_POINT('Ctrl Pts',(153.666860173794,-4.76230668281685,
135.381965984011));
#258238=CARTESIAN_POINT('Ctrl Pts',(153.388412549982,1.27712595144142,137.285331620145));
#258239=CARTESIAN_POINT('Ctrl Pts',(153.109964926169,6.14294222739622,133.233001517943));
#258240=CARTESIAN_POINT('Ctrl Pts',(152.831517302356,5.36369469578529,126.948869073999));
#258241=CARTESIAN_POINT('Ctrl Pts',(152.553069678543,-0.344526230199219,
124.207745007359));
#258242=CARTESIAN_POINT('Ctrl Pts',(152.27462205473,-5.73614438167267,127.528588423912));
#258243=CARTESIAN_POINT('Ctrl Pts',(151.996174430917,-5.85652607262075,
133.859706456064));
#258244=CARTESIAN_POINT('Ctrl Pts',(151.717726807104,-0.595046410034728,
137.383110924578));
#258245=CARTESIAN_POINT('Ctrl Pts',(151.439279183291,5.21325183374003,134.860965250768));
#258246=CARTESIAN_POINT('Ctrl Pts',(151.160831559478,6.23082632381839,128.610998095198));
#258247=CARTESIAN_POINT('Ctrl Pts',(150.882383935665,1.52257581509584,124.376623945969));
#258248=CARTESIAN_POINT('Ctrl Pts',(150.603936311853,-4.58484748573611,
126.049025785542));
#258249=CARTESIAN_POINT('Ctrl Pts',(150.32548868804,-6.47901992942814,132.091348024725));
#258250=CARTESIAN_POINT('Ctrl Pts',(150.047041064227,-2.41928957569559,
136.950991709558));
#258251=CARTESIAN_POINT('Ctrl Pts',(149.768593440414,3.8636497092349,136.162181700472));
#258252=CARTESIAN_POINT('Ctrl Pts',(149.490145816601,6.59608366116008,130.449795860306));
#258253=CARTESIAN_POINT('Ctrl Pts',(149.211698192788,3.26703896508027,125.06323771061));
#258254=CARTESIAN_POINT('Ctrl Pts',(148.933250568975,-3.06425493618196,
124.95249104296));
#258255=CARTESIAN_POINT('Ctrl Pts',(148.654802945162,-6.57964824826877,
130.219326634649));
#258256=CARTESIAN_POINT('Ctrl Pts',(148.376355321349,-4.04866625388314,
136.02377987614));
#258257=CARTESIAN_POINT('Ctrl Pts',(148.097907697537,2.20284223947883,137.031841801807));
#258258=CARTESIAN_POINT('Ctrl Pts',(147.819460073724,6.43004632958585,132.317152748525));
#258259=CARTESIAN_POINT('Ctrl Pts',(147.541012449911,4.74835196802999,126.212281630895));
#258260=CARTESIAN_POINT('Ctrl Pts',(147.262564826098,-1.29684588225586,
124.327306766486));
#258261=CARTESIAN_POINT('Ctrl Pts',(146.984117202285,-6.15030572119196,
128.394427969547));
#258262=CARTESIAN_POINT('Ctrl Pts',(146.705669578472,-5.35193506149072,
134.676159544383));
#258263=CARTESIAN_POINT('Ctrl Pts',(146.427221954659,0.364602463157475,
137.399897053366));
#258264=CARTESIAN_POINT('Ctrl Pts',(146.148774330846,5.74608813598446,134.062658787717));
#258265=CARTESIAN_POINT('Ctrl Pts',(145.870326707034,5.84719952385297,127.731203680413));
#258266=CARTESIAN_POINT('Ctrl Pts',(145.59187908322,0.575020200877703,124.22382966629));
#258267=CARTESIAN_POINT('Ctrl Pts',(145.313431459408,-5.22557459540567,
126.76364211958));
#258268=CARTESIAN_POINT('Ctrl Pts',(145.034983835595,-6.22412162202233,
133.016677472446));
#258269=CARTESIAN_POINT('Ctrl Pts',(144.756536211782,-1.50300494324566,
137.236701713364));
#258270=CARTESIAN_POINT('Ctrl Pts',(144.478088587969,4.59929985250025,135.545718724575));
#258271=CARTESIAN_POINT('Ctrl Pts',(144.199640964156,6.47507277208744,129.497659263665));
#258272=CARTESIAN_POINT('Ctrl Pts',(143.921193340343,2.40057013901678,124.65039451108));
#258273=CARTESIAN_POINT('Ctrl Pts',(143.64274571653,-3.87993917743928,125.458323972397));
#258274=CARTESIAN_POINT('Ctrl Pts',(143.364298092718,-6.594973935395,131.178999942215));
#258275=CARTESIAN_POINT('Ctrl Pts',(143.085850468904,-3.2495498291107,136.555400674828));
#258276=CARTESIAN_POINT('Ctrl Pts',(142.807402845092,3.08205182079176,136.646876548744));
#258277=CARTESIAN_POINT('Ctrl Pts',(142.528955221279,6.58139841398854,131.369365704677));
#258278=CARTESIAN_POINT('Ctrl Pts',(142.250507597466,4.03276138391676,125.572642787588));
#258279=CARTESIAN_POINT('Ctrl Pts',(141.972059973653,-2.2217863466284,124.583612972623));
#258280=CARTESIAN_POINT('Ctrl Pts',(141.69361234984,-6.43462096491922,129.311146342943));
#258281=CARTESIAN_POINT('Ctrl Pts',(141.415164726027,-4.7343532651591,135.410870684068));
#258282=CARTESIAN_POINT('Ctrl Pts',(141.136717102214,1.31655379926713,137.277437314604));
#258283=CARTESIAN_POINT('Ctrl Pts',(140.858269478402,6.15761223939561,133.195562687939));
#258284=CARTESIAN_POINT('Ctrl Pts',(140.579821854588,5.34012584760095,126.916290175316));
#258285=CARTESIAN_POINT('Ctrl Pts',(140.301374230776,-0.384675318488256,
124.20996445632));
#258286=CARTESIAN_POINT('Ctrl Pts',(140.022926606963,-5.75597865932068,
127.563566655346));
#258287=CARTESIAN_POINT('Ctrl Pts',(139.74447898315,-5.83781880742758,133.895300184066));
#258288=CARTESIAN_POINT('Ctrl Pts',(139.466031359337,-0.554988664812238,
137.386611251964));
#258289=CARTESIAN_POINT('Ctrl Pts',(139.187583735524,5.23784894806212,134.829155547671));
#258290=CARTESIAN_POINT('Ctrl Pts',(138.909136111711,6.21735926081381,128.573109924773));
#258291=CARTESIAN_POINT('Ctrl Pts',(138.630688487898,1.48342014776303,124.367474685896));
#258292=CARTESIAN_POINT('Ctrl Pts',(138.352240864086,-4.61370961197883,
126.077023158863));
#258293=CARTESIAN_POINT('Ctrl Pts',(138.073793240272,-6.47106563055709,
132.130763813104));
#258294=CARTESIAN_POINT('Ctrl Pts',(137.79534561646,-2.38182846378423,136.965604729043));
#258295=CARTESIAN_POINT('Ctrl Pts',(137.516897992647,3.89619270241722,136.138563300043));
#258296=CARTESIAN_POINT('Ctrl Pts',(137.238450368834,6.59380311469226,130.409650196134));
#258297=CARTESIAN_POINT('Ctrl Pts',(136.960002745021,3.23203058975544,125.043456686844));
#258298=CARTESIAN_POINT('Ctrl Pts',(136.681555121208,-3.09982015369448,
124.971252454085));
#258299=CARTESIAN_POINT('Ctrl Pts',(136.403107497395,-6.58308761053252,
130.259389660389));
#258300=CARTESIAN_POINT('Ctrl Pts',(136.124659873582,-4.01681915499975,
136.048328553027));
#258301=CARTESIAN_POINT('Ctrl Pts',(135.846212249769,2.24070987145278,137.018317095051));
#258302=CARTESIAN_POINT('Ctrl Pts',(135.567764625956,6.43913599080291,132.277983202917));
#258303=CARTESIAN_POINT('Ctrl Pts',(135.289317002144,4.72031070388647,126.183462145311));
#258304=CARTESIAN_POINT('Ctrl Pts',(135.010869378331,-1.33624951990408,
124.335321040266));
#258305=CARTESIAN_POINT('Ctrl Pts',(134.732421754518,-6.16486171432077,
128.431911276607));
#258306=CARTESIAN_POINT('Ctrl Pts',(134.453974130705,-5.32826716351462,
134.708666556695));
#258307=CARTESIAN_POINT('Ctrl Pts',(134.175526506892,0.404744610239488,
137.397555414672));
#258308=CARTESIAN_POINT('Ctrl Pts',(133.897078883079,5.76581586005707,134.027620349581));
#258309=CARTESIAN_POINT('Ctrl Pts',(133.618631259266,5.82838401024617,127.695667055759));
#258310=CARTESIAN_POINT('Ctrl Pts',(133.340183635453,0.534951987407334,
124.220451277114));
#258311=CARTESIAN_POINT('Ctrl Pts',(133.06173601164,-5.25007477800144,126.795526540492));
#258312=CARTESIAN_POINT('Ctrl Pts',(132.783288387828,-6.21053930283845,
133.054524478268));
#258313=CARTESIAN_POINT('Ctrl Pts',(132.504840764015,-1.46382161007886,
137.245731754674));
#258314=CARTESIAN_POINT('Ctrl Pts',(132.226393140202,4.62807663068185,135.517633634551));
#258315=CARTESIAN_POINT('Ctrl Pts',(131.947945516389,6.46699854195874,129.458267868007));
#258316=CARTESIAN_POINT('Ctrl Pts',(131.669497892576,2.3630647236181,124.635895578019));
#258317=CARTESIAN_POINT('Ctrl Pts',(131.391050268763,-3.91241013359816,
125.482041313105));
#258318=CARTESIAN_POINT('Ctrl Pts',(131.11260264495,-6.59257120989826,131.219138479237));
#258319=CARTESIAN_POINT('Ctrl Pts',(130.834155021138,-3.2144814093103,136.575075053519));
#258320=CARTESIAN_POINT('Ctrl Pts',(130.555707397324,3.1175597702868,136.628006976231));
#258321=CARTESIAN_POINT('Ctrl Pts',(130.277259773512,6.58471582225214,131.329292396271));
#258322=CARTESIAN_POINT('Ctrl Pts',(129.998812149698,4.0008397148189,125.548191156024));
#258323=CARTESIAN_POINT('Ctrl Pts',(129.720364525886,-2.25961263864694,
124.59725287278));
#258324=CARTESIAN_POINT('Ctrl Pts',(129.441916902073,-6.44359136541048,
129.350343372922));
#258325=CARTESIAN_POINT('Ctrl Pts',(129.16346927826,-4.70622441430021,135.439604688201));
#258326=CARTESIAN_POINT('Ctrl Pts',(128.885021654447,1.35593286170785,137.269303146827));
#258327=CARTESIAN_POINT('Ctrl Pts',(128.606574030634,6.17205407880915,133.158035251063));
#258328=CARTESIAN_POINT('Ctrl Pts',(128.328126406821,5.31635911908928,126.883855350513));
#258329=CARTESIAN_POINT('Ctrl Pts',(128.049678783009,-0.424810152491945,
124.212428263054));
#258330=CARTESIAN_POINT('Ctrl Pts',(127.771231159195,-5.77559964706288,
127.598664975593));
#258331=CARTESIAN_POINT('Ctrl Pts',(127.492783535383,-5.81889521971155,
133.930779376167));
#258332=CARTESIAN_POINT('Ctrl Pts',(127.21433591157,-0.514910354280421,
137.389867671632));
#258333=CARTESIAN_POINT('Ctrl Pts',(126.935888287757,5.26225197196523,134.797196704317));
#258334=CARTESIAN_POINT('Ctrl Pts',(126.657440663944,6.20366181127538,128.535304434163));
#258335=CARTESIAN_POINT('Ctrl Pts',(126.378993040131,1.44420951175126,124.358563947));
#258336=CARTESIAN_POINT('Ctrl Pts',(126.100545416318,-4.64240077551519,
126.105195705413));
#258337=CARTESIAN_POINT('Ctrl Pts',(125.822097792505,-6.46287154396936,
132.170130451126));
#258338=CARTESIAN_POINT('Ctrl Pts',(125.543650168692,-2.34427909234318,
136.979989441362));
#258339=CARTESIAN_POINT('Ctrl Pts',(125.26520254488,3.92859132074607,136.114747238771));
#258340=CARTESIAN_POINT('Ctrl Pts',(124.986754921067,6.59127823242518,130.369519158099));
#258341=CARTESIAN_POINT('Ctrl Pts',(124.708307297254,3.19690245034852,125.023889135492));
#258342=CARTESIAN_POINT('Ctrl Pts',(124.429859673441,-3.13527050623128,
124.990230013179));
#258343=CARTESIAN_POINT('Ctrl Pts',(124.151412049628,-6.58628303406391,
130.299472880227));
#258344=CARTESIAN_POINT('Ctrl Pts',(123.872964425815,-3.98482321140548,
136.072682912751));
#258345=CARTESIAN_POINT('Ctrl Pts',(123.594516802002,2.2784944730983,137.004562127853));
#258346=CARTESIAN_POINT('Ctrl Pts',(123.316069178189,6.44798704746787,132.238759051683));
#258347=CARTESIAN_POINT('Ctrl Pts',(123.037621554376,4.6920945268939,126.154813888819));
#258348=CARTESIAN_POINT('Ctrl Pts',(122.759173930564,-1.37560364233486,
124.343575026687));
#258349=CARTESIAN_POINT('Ctrl Pts',(122.480726306751,-6.17918926623166,
128.46948249565));
#258350=CARTESIAN_POINT('Ctrl Pts',(122.202278682938,-5.30440182463932,
134.741028893516));
#258351=CARTESIAN_POINT('Ctrl Pts',(121.923831059125,0.444871759361186,
137.394969462721));
#258352=CARTESIAN_POINT('Ctrl Pts',(121.645383435312,5.78532992970255,133.992462472369));
#258353=CARTESIAN_POINT('Ctrl Pts',(121.366935811499,5.80935252372653,127.660245624887));
#258354=CARTESIAN_POINT('Ctrl Pts',(121.088488187686,0.494863951094175,
124.21731685712));
#258355=CARTESIAN_POINT('Ctrl Pts',(120.810040563873,-5.27438041714564,
126.827559510225));
#258356=CARTESIAN_POINT('Ctrl Pts',(120.53159294006,-6.19672684983677,133.092288103441));
#258357=CARTESIAN_POINT('Ctrl Pts',(120.253145316248,-1.42458403446405,
137.254523108609));
#258358=CARTESIAN_POINT('Ctrl Pts',(119.974697692435,4.65668191378195,135.489373892464));
#258359=CARTESIAN_POINT('Ctrl Pts',(119.696250068622,6.45868467482089,129.418926352309));
#258360=CARTESIAN_POINT('Ctrl Pts',(119.417802444809,2.32547174398699,124.621625219699));
#258361=CARTESIAN_POINT('Ctrl Pts',(119.139354820996,-3.94473611396066,
125.505955874312));
#258362=CARTESIAN_POINT('Ctrl Pts',(118.860907197183,-6.58992419425096,
131.259261646514));
#258363=CARTESIAN_POINT('Ctrl Pts',(118.58245957337,-3.17929387571916,136.594535596262));
#258364=CARTESIAN_POINT('Ctrl Pts',(118.304011949557,3.15295219745811,136.608921606362));
#258365=CARTESIAN_POINT('Ctrl Pts',(118.025564325744,6.58778923144938,131.289199636326));
#258366=CARTESIAN_POINT('Ctrl Pts',(117.747116701932,3.96876979313418,125.523934293753));
#258367=CARTESIAN_POINT('Ctrl Pts',(117.468669078118,-2.29735519988813,
124.611122779595));
#258368=CARTESIAN_POINT('Ctrl Pts',(117.190221454306,-6.45232299625411,
129.389594282045));
#258369=CARTESIAN_POINT('Ctrl Pts',(116.911773830493,-4.67792117256487,
135.468166931659));
#258370=CARTESIAN_POINT('Ctrl Pts',(116.63332620668,1.39526167955762,137.260929418227));
#258371=CARTESIAN_POINT('Ctrl Pts',(116.354878582867,6.18626721048894,133.120420597908));
#258372=CARTESIAN_POINT('Ctrl Pts',(116.076430959054,5.29239539093549,126.851565801475));
#258373=CARTESIAN_POINT('Ctrl Pts',(115.797983335241,-0.464929244999223,
124.215136336267));
#258374=CARTESIAN_POINT('Ctrl Pts',(115.519535711428,-5.79500661783607,
127.633882084071));
#258375=CARTESIAN_POINT('Ctrl Pts',(115.241088087616,-5.79975601069334,
133.96614271767));
#258376=CARTESIAN_POINT('Ctrl Pts',(114.962640463802,-0.474812963556037,
137.392880062915));
#258377=CARTESIAN_POINT('Ctrl Pts',(114.68419283999,5.28646000118636,134.765089904953));
#258378=CARTESIAN_POINT('Ctrl Pts',(114.405745216177,6.18973448276714,128.497583024264));
#258379=CARTESIAN_POINT('Ctrl Pts',(114.127297592364,1.40494536002493,124.349892059469));
#258380=CARTESIAN_POINT('Ctrl Pts',(113.848849968551,-4.67091991318358,
126.133542381245));
#258381=CARTESIAN_POINT('Ctrl Pts',(113.570402344738,-6.45443797329988,
132.209446480045));
#258382=CARTESIAN_POINT('Ctrl Pts',(113.291954720925,-2.30664285277824,
136.994145313484));
#258383=CARTESIAN_POINT('Ctrl Pts',(113.013507097112,3.96084436367879,136.09073439917));
#258384=CARTESIAN_POINT('Ctrl Pts',(112.735059473299,6.58850910791926,130.329404233275));
#258385=CARTESIAN_POINT('Ctrl Pts',(112.456611849487,3.16165584854565,125.004535781636));
#258386=CARTESIAN_POINT('Ctrl Pts',(112.178164225674,-3.1706046801665,125.00942301702));
#258387=CARTESIAN_POINT('Ctrl Pts',(111.899716601861,-6.58923440045535,
130.339574808866));
#258388=CARTESIAN_POINT('Ctrl Pts',(111.621268978048,-3.9526796087217,136.096842052857));
#258389=CARTESIAN_POINT('Ctrl Pts',(111.342821354235,2.31619464429322,136.990577409908));
#258390=CARTESIAN_POINT('Ctrl Pts',(111.064373730422,6.45659917160154,132.199481748287));
#258391=CARTESIAN_POINT('Ctrl Pts',(110.785926106609,4.66370448261314,126.12633792299));
#258392=CARTESIAN_POINT('Ctrl Pts',(110.507478482796,-1.41490679126679,
124.352068419894));
#258393=CARTESIAN_POINT('Ctrl Pts',(110.229030858983,-6.19328784601188,
128.50714023446));
#258394=CARTESIAN_POINT('Ctrl Pts',(109.950583235171,-5.28033992920373,
134.773245355646));
#258395=CARTESIAN_POINT('Ctrl Pts',(109.672135611358,0.484982423596243,
137.392139293334));
#258396=CARTESIAN_POINT('Ctrl Pts',(109.393687987545,5.80462962181993,133.957186458871));
#258397=CARTESIAN_POINT('Ctrl Pts',(109.115240363732,5.79010576951274,127.624940700352));
#258398=CARTESIAN_POINT('Ctrl Pts',(108.836792739919,0.454757577415474,
124.214426522456));
#258399=CARTESIAN_POINT('Ctrl Pts',(108.558345116106,-5.29849061218381,
126.859739841786));
#258400=CARTESIAN_POINT('Ctrl Pts',(108.279897492293,-6.18268477484283,
133.12996694862));
#258401=CARTESIAN_POINT('Ctrl Pts',(108.00144986848,-1.38529367036394,137.2630754494));
#258402=CARTESIAN_POINT('Ctrl Pts',(107.723002244667,4.68511464182123,135.460940545486));
#258403=CARTESIAN_POINT('Ctrl Pts',(107.444554620855,6.45013147874722,129.379636174388));
#258404=CARTESIAN_POINT('Ctrl Pts',(107.166106997042,2.28779259314522,124.607583964913));
#258405=CARTESIAN_POINT('Ctrl Pts',(106.887659373229,-3.97691592067581,
125.530066769856));
#258406=CARTESIAN_POINT('Ctrl Pts',(106.609211749416,-6.58703298653922,
131.299367957265));
#258407=CARTESIAN_POINT('Ctrl Pts',(106.330764125603,-3.14398853222427,
136.613781581943));
#258408=CARTESIAN_POINT('Ctrl Pts',(106.05231650179,3.18822779082625,136.589621146351));
#258409=CARTESIAN_POINT('Ctrl Pts',(105.773868877977,6.59061852769399,131.249088910493));
#258410=CARTESIAN_POINT('Ctrl Pts',(105.495421254164,3.93655280722527,125.49987309962));
#258411=CARTESIAN_POINT('Ctrl Pts',(105.216973630351,-2.33501263178752,
124.625222179118));
#258412=CARTESIAN_POINT('Ctrl Pts',(104.938526006539,-6.46081553389627,
129.428897615854));
#258413=CARTESIAN_POINT('Ctrl Pts',(104.660078382726,-4.64944458874018,
135.49655635606));
#258414=CARTESIAN_POINT('Ctrl Pts',(104.381630758913,1.43453879547275,137.252316439095));
#258415=CARTESIAN_POINT('Ctrl Pts',(104.1031831351,6.20025110776228,133.082720122298));
#258416=CARTESIAN_POINT('Ctrl Pts',(103.824735511287,5.26823555112421,126.819422724701));
#258417=CARTESIAN_POINT('Ctrl Pts',(103.546287887474,-0.505031109382345,
124.218088575609));
#258418=CARTESIAN_POINT('Ctrl Pts',(103.267840263661,-5.81419885250792,
127.669216675797));
#258419=CARTESIAN_POINT('Ctrl Pts',(102.989392639848,-5.78040188958328,
134.001388898174));
#258420=CARTESIAN_POINT('Ctrl Pts',(102.710945016035,-0.434697978462825,
137.395648314187));
#258421=CARTESIAN_POINT('Ctrl Pts',(102.432497392222,5.31047213868803,134.732836339309));
#258422=CARTESIAN_POINT('Ctrl Pts',(102.15404976841,6.17557779137139,128.459947092858));
#258423=CARTESIAN_POINT('Ctrl Pts',(101.875602144597,1.3656291475316,124.341459344644));
#258424=CARTESIAN_POINT('Ctrl Pts',(101.597154520784,-4.69926596819684,
126.162062135967));
#258425=CARTESIAN_POINT('Ctrl Pts',(101.318706896971,-6.44576523105769,
132.248710442988));
#258426=CARTESIAN_POINT('Ctrl Pts',(101.040259273158,-2.26892113971413,
137.008071820859));
#258427=CARTESIAN_POINT('Ctrl Pts',(100.761811649345,3.99295063606701,136.066525671043));
#258428=CARTESIAN_POINT('Ctrl Pts',(100.483364025532,6.58549584378548,130.289306908136));
#258429=CARTESIAN_POINT('Ctrl Pts',(100.204916401719,3.12629209042249,124.985397342422));
#258430=CARTESIAN_POINT('Ctrl Pts',(99.9264687779064,-3.20582136617937,
125.028830754405));
#258431=CARTESIAN_POINT('Ctrl Pts',(99.6480211540935,-6.5919416003429,130.379693960313));
#258432=CARTESIAN_POINT('Ctrl Pts',(99.3695735302808,-3.92038953804142,
136.120805078117));
#258433=CARTESIAN_POINT('Ctrl Pts',(99.0911259064677,2.35380898804382,136.976363459425));
#258434=CARTESIAN_POINT('Ctrl Pts',(98.812678282655,6.46497204407849,132.160152748165));
#258435=CARTESIAN_POINT('Ctrl Pts',(98.5342306588419,4.63514162304771,126.098035303012));
#258436=CARTESIAN_POINT('Ctrl Pts',(98.2557830350292,-1.45415751030726,
124.36080090516));
#258437=CARTESIAN_POINT('Ctrl Pts',(97.9773354112161,-6.20715693123341,
128.544883097616));
#258438=CARTESIAN_POINT('Ctrl Pts',(97.6988877874034,-5.25608236883021,
134.805314749293));
#258439=CARTESIAN_POINT('Ctrl Pts',(97.4204401635904,0.525075116629235,
137.389065011387));
#258440=CARTESIAN_POINT('Ctrl Pts',(97.1419925397775,5.82371422125203,133.921793616252));
#258441=CARTESIAN_POINT('Ctrl Pts',(96.8635449159648,5.77064446080036,127.589753590393));
#258442=CARTESIAN_POINT('Ctrl Pts',(96.5850972921516,0.414634352527504,
124.211780380221));
#258443=CARTESIAN_POINT('Ctrl Pts',(96.306649668339,-5.32240446970382,126.89206634272));
#258444=CARTESIAN_POINT('Ctrl Pts',(96.0282020445258,-6.16841359819089,
133.1675596176));
#258445=CARTESIAN_POINT('Ctrl Pts',(95.7497544207132,-1.34595197369742,
137.271388460138));
#258446=CARTESIAN_POINT('Ctrl Pts',(95.4713067969001,4.7133737612145,135.432334647225));
#258447=CARTESIAN_POINT('Ctrl Pts',(95.1928591730874,6.44133927067958,129.340398790155));
#258448=CARTESIAN_POINT('Ctrl Pts',(94.9144115492744,2.25002866730758,124.593772333964));
#258449=CARTESIAN_POINT('Ctrl Pts',(94.6359639254615,-4.008948361309,125.554373106298));
#258450=CARTESIAN_POINT('Ctrl Pts',(94.3575163016487,-6.58389769389783,
131.339455925338));
#258451=CARTESIAN_POINT('Ctrl Pts',(94.0790686778357,-3.10856668707799,
136.632812297395));
#258452=CARTESIAN_POINT('Ctrl Pts',(93.8006210540229,3.22338524324122,136.570106311383));
#258453=CARTESIAN_POINT('Ctrl Pts',(93.52217343021,6.59320360614536,131.208961705089));
#258454=CARTESIAN_POINT('Ctrl Pts',(93.2437258063971,3.90418995090443,125.476008465224));
#258455=CARTESIAN_POINT('Ctrl Pts',(92.9652781825842,-2.37258353893516,
124.639550548886));
#258456=CARTESIAN_POINT('Ctrl Pts',(92.6868305587713,-6.46906866364288,
129.468251917951));
#258457=CARTESIAN_POINT('Ctrl Pts',(92.4083829349583,-4.62079571803641,
135.524771909422));
#258458=CARTESIAN_POINT('Ctrl Pts',(92.1299353111456,1.47376275402524,137.24346452859));
#258459=CARTESIAN_POINT('Ctrl Pts',(91.8514876873325,6.21400525245068,133.04493522124));
#258460=CARTESIAN_POINT('Ctrl Pts',(91.5730400635199,5.24388049490719,126.787427311268));
#258461=CARTESIAN_POINT('Ctrl Pts',(91.2945924397067,-0.545114259651984,
124.221284871682));
#258462=CARTESIAN_POINT('Ctrl Pts',(91.016144815894,-5.83317563990314,127.704667441434));
#258463=CARTESIAN_POINT('Ctrl Pts',(90.7376971920811,-5.76083357355547,
134.036516611621));
#258464=CARTESIAN_POINT('Ctrl Pts',(90.4592495682681,-0.394566885476172,
137.398172322869));
#258465=CARTESIAN_POINT('Ctrl Pts',(90.1808019444553,5.33428749469169,134.700437202553));
#258466=CARTESIAN_POINT('Ctrl Pts',(89.9023543206424,6.16119226166949,128.422398034556));
#258467=CARTESIAN_POINT('Ctrl Pts',(89.6239066968295,1.32626233114802,124.333266115003));
#258468=CARTESIAN_POINT('Ctrl Pts',(89.3454590730166,-4.72743789018152,
126.190753912764));
#258469=CARTESIAN_POINT('Ctrl Pts',(89.0670114492037,-6.43685363861442,
132.28792088502));
#258470=CARTESIAN_POINT('Ctrl Pts',(88.7885638253908,-2.23111535094281,
137.021768447433));
#258471=CARTESIAN_POINT('Ctrl Pts',(88.5101162015778,4.02490894820102,136.042121951457));
#258472=CARTESIAN_POINT('Ctrl Pts',(88.2316685777651,6.58223855168135,130.2492286685));
#258473=CARTESIAN_POINT('Ctrl Pts',(87.9532209539521,3.09081248639635,124.966474527032));
#258474=CARTESIAN_POINT('Ctrl Pts',(87.6747733301392,-3.2409192593025,125.048452506173));
#258475=CARTESIAN_POINT('Ctrl Pts',(87.3963257063264,-6.59440453341028,
130.41982884794));
#258476=CARTESIAN_POINT('Ctrl Pts',(87.1178780825135,-3.88795419588509,
136.144571100572));
#258477=CARTESIAN_POINT('Ctrl Pts',(86.8394304587006,2.39133611053674,136.961920803106));
#258478=CARTESIAN_POINT('Ctrl Pts',(86.5609828348878,6.47310535463887,132.120773508667));
#258479=CARTESIAN_POINT('Ctrl Pts',(86.2825352110747,4.60640700660486,126.06990707765));
#258480=CARTESIAN_POINT('Ctrl Pts',(86.004087587262,-1.49335434500641,124.369772158902));
#258481=CARTESIAN_POINT('Ctrl Pts',(85.725639963449,-6.22079600797217,128.582709686544));
#258482=CARTESIAN_POINT('Ctrl Pts',(85.4471923396362,-5.23163004239161,
134.837235886113));
#258483=CARTESIAN_POINT('Ctrl Pts',(85.1687447158232,0.565148352810691,
137.385746730796));
#258484=CARTESIAN_POINT('Ctrl Pts',(84.8902970920103,5.842583020812,133.886285256006));
#258485=CARTESIAN_POINT('Ctrl Pts',(84.6118494681974,5.75096931873532,127.554685598878));
#258486=CARTESIAN_POINT('Ctrl Pts',(84.3334018443846,0.374495763211118,
124.209378528473));
#258487=CARTESIAN_POINT('Ctrl Pts',(84.0549542205716,-5.34612110356891,
126.924537815158));
#258488=CARTESIAN_POINT('Ctrl Pts',(83.7765065967588,-6.15391384870464,
133.205064717373));
#258489=CARTESIAN_POINT('Ctrl Pts',(83.498058972946,-1.30656040228555,137.279461832782));
#258490=CARTESIAN_POINT('Ctrl Pts',(83.2196113491328,4.74145822480973,135.403557257686));
#258491=CARTESIAN_POINT('Ctrl Pts',(82.9411637253203,6.43230837641647,129.301215653567));
#258492=CARTESIAN_POINT('Ctrl Pts',(82.6627161015071,2.21218136583022,124.580190838648));
#258493=CARTESIAN_POINT('Ctrl Pts',(82.3842684776944,-4.04083224888638,
125.578873982957));
#258494=CARTESIAN_POINT('Ctrl Pts',(82.1058208538814,-6.58051843250612,
131.379524065257));
#258495=CARTESIAN_POINT('Ctrl Pts',(81.8273732300686,-3.07302965285007,
136.651627037425));
#258496=CARTESIAN_POINT('Ctrl Pts',(81.5489256062556,3.25842325193051,136.550377824588));
#258497=CARTESIAN_POINT('Ctrl Pts',(81.270477982443,6.59554437101248,131.168819507043));
#258498=CARTESIAN_POINT('Ctrl Pts',(80.9920303586297,3.87168242338918,125.452341274876));
#258499=CARTESIAN_POINT('Ctrl Pts',(80.713582734817,-2.41006652912724,124.654107357959));
#258500=CARTESIAN_POINT('Ctrl Pts',(80.435135111004,-6.47708207967116,129.507655730047));
#258501=CARTESIAN_POINT('Ctrl Pts',(80.1566874871913,-4.59197562204804,
135.552812546207));
#258502=CARTESIAN_POINT('Ctrl Pts',(79.8782398633782,1.51293210175691,137.234374014721));
#258503=CARTESIAN_POINT('Ctrl Pts',(79.5997922395654,6.22752913488936,133.007067294864));
#258504=CARTESIAN_POINT('Ctrl Pts',(79.3213446157525,5.2193311247699,126.755580746775));
#258505=CARTESIAN_POINT('Ctrl Pts',(79.0428969919396,-0.585177210512381,
124.224725106049));
#258506=CARTESIAN_POINT('Ctrl Pts',(78.7644493681267,-5.85193627682986,
127.740233067343));
#258507=CARTESIAN_POINT('Ctrl Pts',(78.4860017443139,-5.74105178772106,
134.071524556339));
#258508=CARTESIAN_POINT('Ctrl Pts',(78.2075541205009,-0.354421171668466,
137.400451995434));
#258509=CARTESIAN_POINT('Ctrl Pts',(77.9291064966881,5.35790518671055,134.667893695246));
#258510=CARTESIAN_POINT('Ctrl Pts',(77.6506588728751,6.14657842672258,128.384937240753));
#258511=CARTESIAN_POINT('Ctrl Pts',(77.3722112490624,1.28684636962602,124.325312674148));
#258512=CARTESIAN_POINT('Ctrl Pts',(77.0937636252493,-4.75543463521666,
126.219616648455));
#258513=CARTESIAN_POINT('Ctrl Pts',(76.8153160014366,-6.42770352619243,
132.327076353179));
#258514=CARTESIAN_POINT('Ctrl Pts',(76.5368683776235,-2.19322688737167,
137.035234685673));
#258515=CARTESIAN_POINT('Ctrl Pts',(76.2584207538107,4.05671811585379,136.017524144697));
#258516=CARTESIAN_POINT('Ctrl Pts',(75.9799731299978,6.57873735230709,130.209170999483));
#258517=CARTESIAN_POINT('Ctrl Pts',(75.7015255061849,3.05521835117689,124.947768036657));
#258518=CARTESIAN_POINT('Ctrl Pts',(75.423077882372,-3.27589705897064,125.068287545233));
#258519=CARTESIAN_POINT('Ctrl Pts',(75.1446302585591,-6.5966231083926,130.459977984534));
#258520=CARTESIAN_POINT('Ctrl Pts',(74.8661826347462,-3.85537478415624,
136.168139239563));
#258521=CARTESIAN_POINT('Ctrl Pts',(74.5877350109334,2.42877462119068,136.94724997613));
#258522=CARTESIAN_POINT('Ctrl Pts',(74.3092873871204,6.48099880189986,132.081345489005));
#258523=CARTESIAN_POINT('Ctrl Pts',(74.0308397633076,4.57750169805637,126.041954289206));
#258524=CARTESIAN_POINT('Ctrl Pts',(73.7523921394947,-1.53249584291112,
124.378981848686));
#258525=CARTESIAN_POINT('Ctrl Pts',(73.4739445156818,-6.23420457082727,
128.620618599563));
#258526=CARTESIAN_POINT('Ctrl Pts',(73.1954968918689,-5.20698385597775,
134.869007583256));
#258527=CARTESIAN_POINT('Ctrl Pts',(72.917049268056,0.605200647212208,137.382184574524));
#258528=CARTESIAN_POINT('Ctrl Pts',(72.6386016442432,5.86123532130951,133.850662693911));
#258529=CARTESIAN_POINT('Ctrl Pts',(72.3601540204302,5.73108107238729,127.519738025268));
#258530=CARTESIAN_POINT('Ctrl Pts',(72.0817063966174,0.334343296816498,
124.207221056211));
#258531=CARTESIAN_POINT('Ctrl Pts',(71.8032587728044,-5.36963963495047,
126.957153055855));
#258532=CARTESIAN_POINT('Ctrl Pts',(71.5248111489915,-6.13918606367764,
133.242480858172));
#258533=CARTESIAN_POINT('Ctrl Pts',(71.2463635251787,-1.26712041579749,
137.287295268168));
#258534=CARTESIAN_POINT('Ctrl Pts',(70.9679159013657,4.76936699192676,135.374609443224));
#258535=CARTESIAN_POINT('Ctrl Pts',(70.689468277553,6.423039130601,129.262088216567));
#258536=CARTESIAN_POINT('Ctrl Pts',(70.4110206537399,2.17425209115883,124.566839982233));
#258537=CARTESIAN_POINT('Ctrl Pts',(70.1325730299272,-4.07256640193864,
125.603568491945));
#258538=CARTESIAN_POINT('Ctrl Pts',(69.8541254061142,-6.57689532758393,
131.419570892283));
#258539=CARTESIAN_POINT('Ctrl Pts',(69.5756777823013,-3.03737874637841,
136.670225104848));
#258540=CARTESIAN_POINT('Ctrl Pts',(69.2972301584884,3.2933405185478,136.530436417012));
#258541=CARTESIAN_POINT('Ctrl Pts',(69.0187825346755,6.5976407355574,131.128663803839));
#258542=CARTESIAN_POINT('Ctrl Pts',(68.7403349108627,3.83903142925813,125.428872405572));
#258543=CARTESIAN_POINT('Ctrl Pts',(68.4618872870498,-2.44746021341752,
124.668892066929));
#258544=CARTESIAN_POINT('Ctrl Pts',(68.1834396632368,-6.48485548504104,
129.547107592018));
#258545=CARTESIAN_POINT('Ctrl Pts',(67.904992039424,-4.56298536871445,135.580677227361));
#258546=CARTESIAN_POINT('Ctrl Pts',(67.6265444156111,1.55204538723279,137.225045234339));
#258547=CARTESIAN_POINT('Ctrl Pts',(67.3480967917982,6.2408222539455,132.969117746385));
#258548=CARTESIAN_POINT('Ctrl Pts',(67.0696491679854,5.19458835039884,126.723884211309));
#258549=CARTESIAN_POINT('Ctrl Pts',(66.7912015441724,-0.625218477415679,
124.228409151229));
#258550=CARTESIAN_POINT('Ctrl Pts',(66.5127539203596,-5.87048006810572,
127.775912235624));
#258551=CARTESIAN_POINT('Ctrl Pts',(66.2343062965465,-5.72105726510147,
134.106411435094));
#258552=CARTESIAN_POINT('Ctrl Pts',(65.9558586727338,-0.314262324654327,
137.402487247406));
#258553=CARTESIAN_POINT('Ctrl Pts',(65.6774110489208,5.3813243395822,134.6352070233));
#258554=CARTESIAN_POINT('Ctrl Pts',(65.398963425108,6.13173682805169,128.347566099575));
#258555=CARTESIAN_POINT('Ctrl Pts',(65.120515801295,1.24738272353907,124.317599316798));
#258556=CARTESIAN_POINT('Ctrl Pts',(64.8420681774823,-4.78325516587229,
126.248649273519));
#258557=CARTESIAN_POINT('Ctrl Pts',(64.5636205536692,-6.41831523285262,
132.366175396547));
#258558=CARTESIAN_POINT('Ctrl Pts',(64.2851729298565,-2.15525715297185,
137.048470036584));
#258559=CARTESIAN_POINT('Ctrl Pts',(64.0067253060435,4.08837696032456,135.992733162246));
#258560=CARTESIAN_POINT('Ctrl Pts',(63.7282776822307,6.57499237540094,130.169135385437));
#258561=CARTESIAN_POINT('Ctrl Pts',(63.4498300584178,3.01951100371835,124.929278564476));
#258562=CARTESIAN_POINT('Ctrl Pts',(63.1713824346048,-3.31075346906837,
125.088335136589));
#258563=CARTESIAN_POINT('Ctrl Pts',(62.892934810792,-6.59859724307971,130.500139882352));
#258564=CARTESIAN_POINT('Ctrl Pts',(62.614487186979,-3.82265251009718,136.191508621766));
#258565=CARTESIAN_POINT('Ctrl Pts',(62.3360395631662,2.46612313270748,136.932351522132));
#258566=CARTESIAN_POINT('Ctrl Pts',(62.0575919393533,6.48865209336687,132.041870150199));
#258567=CARTESIAN_POINT('Ctrl Pts',(61.7791443155403,4.5484267684992,126.014177973478));
#258568=CARTESIAN_POINT('Ctrl Pts',(61.5006966917276,-1.57158055361859,
124.388429633243));
#258569=CARTESIAN_POINT('Ctrl Pts',(61.2222490679146,-6.24738212293903,
128.658608431946));
#258570=CARTESIAN_POINT('Ctrl Pts',(60.9438014441017,-5.18214472286266,
134.900628663412));
#258571=CARTESIAN_POINT('Ctrl Pts',(60.6653538202889,0.645230515680748,
137.378378674564));
#258572=CARTESIAN_POINT('Ctrl Pts',(60.3869061964759,5.87967043157647,133.814927249971));
#258573=CARTESIAN_POINT('Ctrl Pts',(60.108458572663,5.71098045872276,127.484912164554));
#258574=CARTESIAN_POINT('Ctrl Pts',(59.8300109488502,0.294178441208572,
124.205308043382));
#258575=CARTESIAN_POINT('Ctrl Pts',(59.5515633250373,-5.39295919236059,
126.989910856244));
#258576=CARTESIAN_POINT('Ctrl Pts',(59.2731157012244,-6.12423078885343,
133.27980665353));
#258577=CARTESIAN_POINT('Ctrl Pts',(58.9946680774115,-1.2276334756968,137.294888476026));
#258578=CARTESIAN_POINT('Ctrl Pts',(58.7162204535986,4.79709902839574,135.345492276511));
#258579=CARTESIAN_POINT('Ctrl Pts',(58.4377728297857,6.41353187670863,129.223017929039));
#258580=CARTESIAN_POINT('Ctrl Pts',(58.1593252059728,2.13624224877676,124.553720259438));
#258581=CARTESIAN_POINT('Ctrl Pts',(57.8808775821599,-4.10414964454526,
125.628455718198));
#258582=CARTESIAN_POINT('Ctrl Pts',(57.602429958347,-6.57302851338661,131.459594922466));
#258583=CARTESIAN_POINT('Ctrl Pts',(57.3239823345341,-3.00161528872044,
136.688605810505));
#258584=CARTESIAN_POINT('Ctrl Pts',(57.0455347107212,3.32813574922106,136.510282827592));
#258585=CARTESIAN_POINT('Ctrl Pts',(56.7670870869083,6.59949262209846,131.088496083461));
#258586=CARTESIAN_POINT('Ctrl Pts',(56.4886394630955,3.80623817840574,125.405602726962));
#258587=CARTESIAN_POINT('Ctrl Pts',(56.2101918392826,-2.48476320616966,
124.683904127941));
#258588=CARTESIAN_POINT('Ctrl Pts',(55.9317442154696,-6.49238859170611,
129.586606041964));
#258589=CARTESIAN_POINT('Ctrl Pts',(55.6532965916568,-4.53382603227983,
135.608364920346));
#258590=CARTESIAN_POINT('Ctrl Pts',(55.3748489678439,1.59110116109648,137.215478533129));
#258591=CARTESIAN_POINT('Ctrl Pts',(55.096401344031,6.25388411703813,132.931087982032));
#258592=CARTESIAN_POINT('Ctrl Pts',(54.8179537202181,5.1696530886458,126.692338879397));
#258593=CARTESIAN_POINT('Ctrl Pts',(54.5395060964052,-0.665236576618623,
124.23233687071));
#258594=CARTESIAN_POINT('Ctrl Pts',(54.2610584725923,-5.88880632658389,
127.811703624173));
#258595=CARTESIAN_POINT('Ctrl Pts',(53.9826108487795,-5.70085074660091,
134.141175955143));
#258596=CARTESIAN_POINT('Ctrl Pts',(53.7041632249665,-0.274091832533765,
137.40427800337));
#258597=CARTESIAN_POINT('Ctrl Pts',(53.4257156011537,5.40454408550164,134.602378397932));
#258598=CARTESIAN_POINT('Ctrl Pts',(53.1472679773408,6.11666801561766,128.310285995821));
#258599=CARTESIAN_POINT('Ctrl Pts',(52.8688203535278,1.20787285522606,124.310126328773));
#258600=CARTESIAN_POINT('Ctrl Pts',(52.590372729715,-4.81089845124901,126.277850712144));
#258601=CARTESIAN_POINT('Ctrl Pts',(52.3119251059021,-6.40868910648141,
132.405216566294));
#258602=CARTESIAN_POINT('Ctrl Pts',(52.0334774820892,-2.11720755472543,
137.061474009724));
#258603=CARTESIAN_POINT('Ctrl Pts',(51.7550298582764,4.11988430848393,135.967749922743));
#258604=CARTESIAN_POINT('Ctrl Pts',(51.4765822344634,6.57100375973434,130.129123309894));
#258605=CARTESIAN_POINT('Ctrl Pts',(51.1981346106506,2.98369176716867,124.91100679562));
#258606=CARTESIAN_POINT('Ctrl Pts',(50.9196869868376,-3.34548719797895,
125.108594537373));
#258607=CARTESIAN_POINT('Ctrl Pts',(50.6412393630248,-6.60032686431936,
130.540313053181));
#258608=CARTESIAN_POINT('Ctrl Pts',(50.3627917392119,-3.78978858624336,
136.214678381218));
#258609=CARTESIAN_POINT('Ctrl Pts',(50.0843441153989,2.50338026112505,136.917225993175));
#258610=CARTESIAN_POINT('Ctrl Pts',(49.8058964915862,6.49606494544435,132.002348955022));
#258611=CARTESIAN_POINT('Ctrl Pts',(49.5274488677731,4.51918329531533,125.986579159731));
#258612=CARTESIAN_POINT('Ctrl Pts',(49.2490012439603,-1.6106070288309,124.39811516248));
#258613=CARTESIAN_POINT('Ctrl Pts',(48.9705536201474,-6.26032817600901,
128.696677775965));
#258614=CARTESIAN_POINT('Ctrl Pts',(48.6921059963345,-5.15711356346882,
134.932097954848));
#258615=CARTESIAN_POINT('Ctrl Pts',(48.4136583725217,0.685236474895564,
137.374329171949));
#258616=CARTESIAN_POINT('Ctrl Pts',(48.1352107487087,5.89788766849362,133.779080248378));
#258617=CARTESIAN_POINT('Ctrl Pts',(47.8567631248959,5.69066822257687,127.450209307224));
#258618=CARTESIAN_POINT('Ctrl Pts',(47.578315501083,0.254002684709825,124.203639560873));
#258619=CARTESIAN_POINT('Ctrl Pts',(47.29986787727,-5.41607891168467,127.022810002472));
#258620=CARTESIAN_POINT('Ctrl Pts',(47.0214202534572,-6.10904857840509,
133.317040720324));
#258621=CARTESIAN_POINT('Ctrl Pts',(46.7429726296443,-1.18810104518584,
137.302241174989));
#258622=CARTESIAN_POINT('Ctrl Pts',(46.4645250058313,4.82465330659632,135.316206836494));
#258623=CARTESIAN_POINT('Ctrl Pts',(46.1860773820186,6.40378696703385,129.184006238746));
#258624=CARTESIAN_POINT('Ctrl Pts',(45.9076297582056,2.09815324715241,124.54083215642));
#258625=CARTESIAN_POINT('Ctrl Pts',(45.6291821343927,-4.13558080637756,
125.653534739511));
#258626=CARTESIAN_POINT('Ctrl Pts',(45.3507345105798,-6.56891813320061,
131.499594672701));
#258627=CARTESIAN_POINT('Ctrl Pts',(45.072286886767,-2.96574060510383,136.706768473292));
#258628=CARTESIAN_POINT('Ctrl Pts',(44.793839262954,3.36280765460034,136.489917803126));
#258629=CARTESIAN_POINT('Ctrl Pts',(44.5153916391412,6.60109996201359,131.048317834339));
#258630=CARTESIAN_POINT('Ctrl Pts',(44.2369440153282,3.77330388599763,125.38253310131));
#258631=CARTESIAN_POINT('Ctrl Pts',(43.9584963915154,-2.52197412510756,
124.699142984721));
#258632=CARTESIAN_POINT('Ctrl Pts',(43.6800487677024,-6.49968112052436,
129.626149616253));
#258633=CARTESIAN_POINT('Ctrl Pts',(43.4016011438896,-4.50449869325427,
135.635874599185));
#258634=CARTESIAN_POINT('Ctrl Pts',(43.1231535200766,1.6300979761215,137.205674265588));
#258635=CARTESIAN_POINT('Ctrl Pts',(42.8447058962639,6.26671424015497,132.892979411015));
#258636=CARTESIAN_POINT('Ctrl Pts',(42.5662582724509,5.14452626349642,126.660945919963));
#258637=CARTESIAN_POINT('Ctrl Pts',(42.287810648638,-0.705230025235587,
124.236508118946));
#258638=CARTESIAN_POINT('Ctrl Pts',(42.0093630248251,-5.90691437317801,
127.847605906729));
#258639=CARTESIAN_POINT('Ctrl Pts',(41.7309154010123,-5.68043298097947,
134.175816828272));
#258640=CARTESIAN_POINT('Ctrl Pts',(41.4524677771993,-0.233911183839542,
137.405824196969));
#258641=CARTESIAN_POINT('Ctrl Pts',(41.1740201533865,5.42756356405245,134.569409035618));
#258642=CARTESIAN_POINT('Ctrl Pts',(40.8955725295735,6.10137254780096,128.273098310918));
#258643=CARTESIAN_POINT('Ctrl Pts',(40.6171249057607,1.1683182287399,124.302893986988));
#258644=CARTESIAN_POINT('Ctrl Pts',(40.3386772819477,-4.83836346701448,
126.307219882257));
#258645=CARTESIAN_POINT('Ctrl Pts',(40.060229658135,-6.39882550377857,132.444198415735));
#258646=CARTESIAN_POINT('Ctrl Pts',(39.781782034322,-2.07907950257448,137.074246123225));
#258647=CARTESIAN_POINT('Ctrl Pts',(39.5033344105091,4.15123899281517,135.94257535195));
#258648=CARTESIAN_POINT('Ctrl Pts',(39.2248867866962,6.56677165310695,130.089136255519));
#258649=CARTESIAN_POINT('Ctrl Pts',(38.9464391628834,2.94776196882331,124.892953407157));
#258650=CARTESIAN_POINT('Ctrl Pts',(38.6679915390704,-3.38009695863112,
125.129064996863));
#258651=CARTESIAN_POINT('Ctrl Pts',(38.3895439152575,-6.6018119080198,130.58049600839));
#258652=CARTESIAN_POINT('Ctrl Pts',(38.1110962914447,-3.75678423037978,
136.237647659355));
#258653=CARTESIAN_POINT('Ctrl Pts',(37.8326486676317,2.54054462586645,136.901873949744));
#258654=CARTESIAN_POINT('Ctrl Pts',(37.5542010438189,6.50323708344635,131.962783367948));
#258655=CARTESIAN_POINT('Ctrl Pts',(37.275753420006,4.48977236213255,125.959158870647));
#258656=CARTESIAN_POINT('Ctrl Pts',(36.9973057961931,-1.64957382240749,
124.4080380775));
#258657=CARTESIAN_POINT('Ctrl Pts',(36.7188581723802,-6.27304225031618,
128.734825220947));
#258658=CARTESIAN_POINT('Ctrl Pts',(36.4404105485673,-5.13189130533538,
134.96341429146));
#258659=CARTESIAN_POINT('Ctrl Pts',(36.1619629247544,0.725217042420823,
137.370036216732));
#258660=CARTESIAN_POINT('Ctrl Pts',(35.8835153009416,5.91588635701427,133.743123017455));
#258661=CARTESIAN_POINT('Ctrl Pts',(35.6050676771286,5.67014511662727,127.415630739204));
#258662=CARTESIAN_POINT('Ctrl Pts',(35.3266200533158,0.213817516048174,
124.202215670509));
#258663=CARTESIAN_POINT('Ctrl Pts',(35.0481724295028,-5.43899793621292,
127.055849275448));
#258664=CARTESIAN_POINT('Ctrl Pts',(34.76972480569,-6.09363999491508,133.354181678833));
#258665=CARTESIAN_POINT('Ctrl Pts',(34.4912771818771,-1.14852458915375,
137.309353092597));
#258666=CARTESIAN_POINT('Ctrl Pts',(34.2128295580642,4.85202880549439,135.286754208357));
#258667=CARTESIAN_POINT('Ctrl Pts',(33.9343819342512,6.393804762678,129.145054591279));
#258668=CARTESIAN_POINT('Ctrl Pts',(33.6559343104384,2.05998649768791,124.528176150753));
#258669=CARTESIAN_POINT('Ctrl Pts',(33.3774866866255,-4.16685872274224,
125.678804626571));
#258670=CARTESIAN_POINT('Ctrl Pts',(33.0990390628127,-6.56456433933747,
131.539568660782));
#258671=CARTESIAN_POINT('Ctrl Pts',(32.8205914389997,-2.92975602487846,
136.724712420187));
#258672=CARTESIAN_POINT('Ctrl Pts',(32.5421438151868,3.39735494990529,136.469342098247));
#258673=CARTESIAN_POINT('Ctrl Pts',(32.263696191374,6.60246269574222,131.008130545292));
#258674=CARTESIAN_POINT('Ctrl Pts',(31.985248567561,3.74022977242616,125.359664383471));
#258675=CARTESIAN_POINT('Ctrl Pts',(31.7068009437482,-2.55909159136699,
124.714608072585));
#258676=CARTESIAN_POINT('Ctrl Pts',(31.4283533199352,-6.50673280126843,
129.665736849585));
#258677=CARTESIAN_POINT('Ctrl Pts',(31.1499056961224,-4.47500443837311,
135.663205244496));
#258678=CARTESIAN_POINT('Ctrl Pts',(30.8714580723094,1.66903438726656,137.195632795014));
#258679=CARTESIAN_POINT('Ctrl Pts',(30.5930104484966,6.27931214787105,132.854793445461));
#258680=CARTESIAN_POINT('Ctrl Pts',(30.3145628246837,5.11920880603445,126.629706496284));
#258681=CARTESIAN_POINT('Ctrl Pts',(30.0361152008708,-0.745197341294603,
124.240922741373));
#258682=CARTESIAN_POINT('Ctrl Pts',(29.7576675770579,-5.9248035368878,127.883617752917));
#258683=CARTESIAN_POINT('Ctrl Pts',(29.4792199532451,-5.65980472482494,
134.210332770852));
#258684=CARTESIAN_POINT('Ctrl Pts',(29.2007723294321,-0.193721867480399,
137.407125770907));
#258685=CARTESIAN_POINT('Ctrl Pts',(28.9223247056193,5.45038192223944,134.536300158051));
#258686=CARTESIAN_POINT('Ctrl Pts',(28.6438770818064,6.08585099138068,128.236004422871));
#258687=CARTESIAN_POINT('Ctrl Pts',(28.3654294579935,1.12872030979243,124.29590255944));
#258688=CARTESIAN_POINT('Ctrl Pts',(28.0869818341806,-4.86564919544231,
126.336755695574));
#258689=CARTESIAN_POINT('Ctrl Pts',(27.8085342103677,-6.38872479024353,
132.483119500384));
#258690=CARTESIAN_POINT('Ctrl Pts',(27.5300865865548,-2.04087440936798,
137.086785903815));
#258691=CARTESIAN_POINT('Ctrl Pts',(27.2516389627419,4.18243985145892,135.91721038272));
#258692=CARTESIAN_POINT('Ctrl Pts',(26.973191338929,6.56229621234102,130.049175704046));
#258693=CARTESIAN_POINT('Ctrl Pts',(26.6947437151162,2.91172294007416,124.875119068062));
#258694=CARTESIAN_POINT('Ctrl Pts',(26.4162960913032,-3.41458146854746,
125.149745756519));
#258695=CARTESIAN_POINT('Ctrl Pts',(26.1378484674903,-6.60305231915217,
130.620687258984));
#258696=CARTESIAN_POINT('Ctrl Pts',(25.8594008436774,-3.72364066549499,
136.260415605043));
#258697=CARTESIAN_POINT('Ctrl Pts',(25.5809532198646,2.57761484979243,136.886295960714));
#258698=CARTESIAN_POINT('Ctrl Pts',(25.3025055960517,6.51016824160669,131.92317485509));
#258699=CARTESIAN_POINT('Ctrl Pts',(25.0240579722387,4.46019505878377,125.931918122295));
#258700=CARTESIAN_POINT('Ctrl Pts',(24.7456103484259,-1.68847949041943,
124.418198010604));
#258701=CARTESIAN_POINT('Ctrl Pts',(24.467162724613,-6.28552387473587,128.773049353324));
#258702=CARTESIAN_POINT('Ctrl Pts',(24.1887151008001,-5.10647888308236,
134.994576512808));
#258703=CARTESIAN_POINT('Ctrl Pts',(23.9102674769872,0.765170736761864,
137.365499967992));
#258704=CARTESIAN_POINT('Ctrl Pts',(23.6318198531744,5.93366583019039,133.707056889611));
#258705=CARTESIAN_POINT('Ctrl Pts',(23.3533722293614,5.64941190136517,127.381177741815));
#258706=CARTESIAN_POINT('Ctrl Pts',(23.0749246055485,0.173624424299845,
124.201036425055));
#258707=CARTESIAN_POINT('Ctrl Pts',(22.7964769817356,-5.46171541667246,
127.08902745089));
#258708=CARTESIAN_POINT('Ctrl Pts',(22.5180293579228,-6.07800560935413,
133.391228152785));
#258709=CARTESIAN_POINT('Ctrl Pts',(22.2395817341099,-1.10890557412062,
137.316223965318));
#258710=CARTESIAN_POINT('Ctrl Pts',(21.9611341102969,4.87922451068073,135.257135483476));
#258711=CARTESIAN_POINT('Ctrl Pts',(21.6826864864842,6.38358563353538,129.106164430008));
#258712=CARTESIAN_POINT('Ctrl Pts',(21.4042388626712,2.02174341466617,124.515752711409));
#258713=CARTESIAN_POINT('Ctrl Pts',(21.1257912388583,-4.19798223462457,
125.704264442993));
#258714=CARTESIAN_POINT('Ctrl Pts',(20.8473436150454,-6.55996729312864,
131.579515405459));
#258715=CARTESIAN_POINT('Ctrl Pts',(20.5688959912325,-2.89366288146616,
136.742436986267));
#258716=CARTESIAN_POINT('Ctrl Pts',(20.2904483674196,3.43177635497322,136.448556475397));
#258717=CARTESIAN_POINT('Ctrl Pts',(20.0120007436067,6.60358077278748,130.967935705476));
#258718=CARTESIAN_POINT('Ctrl Pts',(19.7335531197938,3.70701706326526,125.336997420853));
#258719=CARTESIAN_POINT('Ctrl Pts',(19.455105495981,-2.59611422954622,124.730298818468));
#258720=CARTESIAN_POINT('Ctrl Pts',(19.176657872168,-6.51354337263571,129.705366275038));
#258721=CARTESIAN_POINT('Ctrl Pts',(18.8982102483552,-4.4453443605568,135.690355843533));
#258722=CARTESIAN_POINT('Ctrl Pts',(18.6197626245423,1.70790895172861,137.1853544935));
#258723=CARTESIAN_POINT('Ctrl Pts',(18.3413150007294,6.29167737336628,132.816531500364));
#258724=CARTESIAN_POINT('Ctrl Pts',(18.0628673769165,5.09370165440758,126.598621765949));
#258725=CARTESIAN_POINT('Ctrl Pts',(17.7844197531036,-0.785137043792105,
124.245580574404));
#258726=CARTESIAN_POINT('Ctrl Pts',(17.5059721292907,-5.94247315482366,
127.919737828307));
#258727=CARTESIAN_POINT('Ctrl Pts',(17.2275245054778,-5.63896674252494,
134.244722503881));
#258728=CARTESIAN_POINT('Ctrl Pts',(16.949076881665,-0.15352537268619,137.408182676953));
#258729=CARTESIAN_POINT('Ctrl Pts',(16.6706292578521,5.47299831451989,134.503052992091));
#258730=CARTESIAN_POINT('Ctrl Pts',(16.3921816340391,6.07010392151387,128.199005706208));
#258731=CARTESIAN_POINT('Ctrl Pts',(16.1137340102263,1.08908056569879,124.289152305198));
#258732=CARTESIAN_POINT('Ctrl Pts',(15.8352863864134,-4.89275462544986,
126.366457057635));
#258733=CARTESIAN_POINT('Ctrl Pts',(15.5568387626005,-6.37838734016194,
132.521978378005));
#258734=CARTESIAN_POINT('Ctrl Pts',(15.2783911387876,-2.00259369080969,
137.099092886824));
#258735=CARTESIAN_POINT('Ctrl Pts',(14.9999435149747,4.21348572825588,135.891655954962));
#258736=CARTESIAN_POINT('Ctrl Pts',(14.7214958911618,6.55757760327567,130.009243136227));
#258737=CARTESIAN_POINT('Ctrl Pts',(14.4430482673489,2.87557601636067,124.857504439193));
#258738=CARTESIAN_POINT('Ctrl Pts',(14.164600643536,-3.44893944989177,125.170636050008));
#258739=CARTESIAN_POINT('Ctrl Pts',(13.8861530197231,-6.60404805175259,
130.660885315664));
#258740=CARTESIAN_POINT('Ctrl Pts',(13.6077053959103,-3.69035911973598,
136.282981374608));
#258741=CARTESIAN_POINT('Ctrl Pts',(13.3292577720973,2.61458955925225,136.870492603333));
#258742=CARTESIAN_POINT('Ctrl Pts',(13.0508101482845,6.5168581630887,131.883524884162));
#258743=CARTESIAN_POINT('Ctrl Pts',(12.7723625244716,4.43045248126686,125.904857924092));
#258744=CARTESIAN_POINT('Ctrl Pts',(12.4939149006587,-1.72732259120293,
124.428594585312));
#258745=CARTESIAN_POINT('Ctrl Pts',(12.2154672768458,-6.29777258675688,
128.811348756686));
#258746=CARTESIAN_POINT('Ctrl Pts',(11.9370196530329,-5.08087723837641,
135.025583464166));
#258747=CARTESIAN_POINT('Ctrl Pts',(11.65857202922,0.805096077419857,137.36072059382));
#258748=CARTESIAN_POINT('Ctrl Pts',(11.3801244054071,5.95122542919731,133.670883201288));
#258749=CARTESIAN_POINT('Ctrl Pts',(11.1016767815943,5.62846934506734,127.346851591727));
#258750=CARTESIAN_POINT('Ctrl Pts',(10.8232291577813,0.13342489883439,124.200101868207));
#258751=CARTESIAN_POINT('Ctrl Pts',(10.5447815339684,-5.4842305112587,127.12234329937));
#258752=CARTESIAN_POINT('Ctrl Pts',(10.2663339101556,-6.06214600106014,
133.428178769409));
#258753=CARTESIAN_POINT('Ctrl Pts',(9.98788628634267,-1.06924546818365,
137.322853538546));
#258754=CARTESIAN_POINT('Ctrl Pts',(9.70943866252976,4.90623941440849,135.227351759386));
#258755=CARTESIAN_POINT('Ctrl Pts',(9.43099103871685,6.37312995827954,129.067337196021));
#258756=CARTESIAN_POINT('Ctrl Pts',(9.15254341490403,1.98342541519871,124.503562298745));
#258757=CARTESIAN_POINT('Ctrl Pts',(8.87409579109107,-4.22895018873139,
125.729913245354));
#258758=CARTESIAN_POINT('Ctrl Pts',(8.59564816727821,-6.55512716491932,
131.61943342649));
#258759=CARTESIAN_POINT('Ctrl Pts',(8.31720054346528,-2.85746251231165,
136.759941514744));
#258760=CARTESIAN_POINT('Ctrl Pts',(8.03875291965246,3.46607059430627,136.427561704794));
#258761=CARTESIAN_POINT('Ctrl Pts',(7.76030529583951,6.60445415171875,130.927734804324));
#258762=CARTESIAN_POINT('Ctrl Pts',(7.48185767202662,3.67366698922382,125.314533053388));
#258763=CARTESIAN_POINT('Ctrl Pts',(7.20341004821377,-2.63304066775796,
124.746214640945));
#258764=CARTESIAN_POINT('Ctrl Pts',(6.92496242440086,-6.52011258225796,
129.745036424131));
#258765=CARTESIAN_POINT('Ctrl Pts',(6.64651480058794,-4.41551955887045,
135.71732539022));
#258766=CARTESIAN_POINT('Ctrl Pts',(6.36806717677509,1.74672022899638,137.174839741911));
#258767=CARTESIAN_POINT('Ctrl Pts',(6.08961955296221,6.30380945844269,132.778194993536));
#258768=CARTESIAN_POINT('Ctrl Pts',(5.81117192914928,5.06800575379271,126.567692880813));
#258769=CARTESIAN_POINT('Ctrl Pts',(5.53272430533639,-0.825047652747706,
124.250481445441));
#258770=CARTESIAN_POINT('Ctrl Pts',(5.25427668152353,-5.95992257223146,
127.955964794454));
#258771=CARTESIAN_POINT('Ctrl Pts',(4.97582905771062,-5.61791980623858,
134.278984753035));
#258772=CARTESIAN_POINT('Ctrl Pts',(4.69738143389771,-0.113323188952861,
137.408994875945));
#258773=CARTESIAN_POINT('Ctrl Pts',(4.41893381008486,5.49541190283514,134.469668769726));
#258774=CARTESIAN_POINT('Ctrl Pts',(4.14048618627195,6.05413192171396,128.162103531929));
#258775=CARTESIAN_POINT('Ctrl Pts',(3.86203856245905,1.0494004653243,124.282643474398));
#258776=CARTESIAN_POINT('Ctrl Pts',(3.58359093864613,-4.91967875263547,
126.396322867843));
#258777=CARTESIAN_POINT('Ctrl Pts',(3.30514331483329,-6.36781353659179,
132.560773608667));
#258778=CARTESIAN_POINT('Ctrl Pts',(3.02669569102039,-1.96423876540577,
137.111166616214));
#258779=CARTESIAN_POINT('Ctrl Pts',(2.74824806720748,4.24437547278969,135.865913015604));
#258780=CARTESIAN_POINT('Ctrl Pts',(2.46980044339459,6.55261600076067,129.969340031779));
#258781=CARTESIAN_POINT('Ctrl Pts',(2.19135281958173,2.83932253712042,124.840110173268));
#258782=CARTESIAN_POINT('Ctrl Pts',(1.91290519576881,-3.48316962951642,
125.191735103234));
#258783=CARTESIAN_POINT('Ctrl Pts',(1.6344575719559,-6.60479906892382,130.701088688872));
#258784=CARTESIAN_POINT('Ctrl Pts',(1.35600994814304,-3.65694082636265,
136.305344131865));
#258785=CARTESIAN_POINT('Ctrl Pts',(1.07756232433016,2.65146738413444,136.854464463202));
#258786=CARTESIAN_POINT('Ctrl Pts',(0.799114700517227,6.52330659999492,
131.843834924404));
#258787=CARTESIAN_POINT('Ctrl Pts',(0.520667076704378,4.40054573170394,
125.877979278764));
#258788=CARTESIAN_POINT('Ctrl Pts',(0.242219452891471,-1.76610168541259,
124.439227416375));
#258789=CARTESIAN_POINT('Ctrl Pts',(-0.03622817092143,-6.30978793249869,
128.849722011837));
#258790=CARTESIAN_POINT('Ctrl Pts',(-0.314675794734322,-5.05508731989592,
135.056433996558));
#258791=CARTESIAN_POINT('Ctrl Pts',(-0.593123418547181,0.844991584946641,
137.355698271319));
#258792=CARTESIAN_POINT('Ctrl Pts',(-0.871571042360099,5.96856450335716,
133.634603292916));
#258793=CARTESIAN_POINT('Ctrl Pts',(-1.15001866617301,5.60731822376822,
127.312653560908));
#258794=CARTESIAN_POINT('Ctrl Pts',(-1.42846628998586,0.0932204292604712,
124.199412034595));
#258795=CARTESIAN_POINT('Ctrl Pts',(-1.70691391379876,-5.50654238566651,
127.155795586355));
#258796=CARTESIAN_POINT('Ctrl Pts',(-1.98536153761166,-6.04606175771675,
133.465032159487));
#258797=CARTESIAN_POINT('Ctrl Pts',(-2.26380916142456,-1.02954574096264,
137.329241566624));
#258798=CARTESIAN_POINT('Ctrl Pts',(-2.5422567852374,4.9330725156305,135.197404139731));
#258799=CARTESIAN_POINT('Ctrl Pts',(-2.82070440905033,6.36243812434939,
129.028574328076));
#258800=CARTESIAN_POINT('Ctrl Pts',(-3.09915203286324,1.94503391917308,
124.491605364478));
#258801=CARTESIAN_POINT('Ctrl Pts',(-3.3775996566761,-4.25976143753379,
125.755750083229));
#258802=CARTESIAN_POINT('Ctrl Pts',(-3.65604728048899,-6.55004413406227,
131.659321244699));
#258803=CARTESIAN_POINT('Ctrl Pts',(-3.9344949043019,-2.82115625883292,
136.777225356981));
#258804=CARTESIAN_POINT('Ctrl Pts',(-4.2129425281148,3.50023639711881,136.406358564405));
#258805=CARTESIAN_POINT('Ctrl Pts',(-4.49139015192765,6.60508280017262,
130.887529331496));
#258806=CARTESIAN_POINT('Ctrl Pts',(-4.76983777574057,3.64018078610111,
125.292272113504));
#258807=CARTESIAN_POINT('Ctrl Pts',(-5.04828539955349,-2.66986953767946,
124.762354950249));
#258808=CARTESIAN_POINT('Ctrl Pts',(-5.32673302336633,-6.52644018671072,
129.784745826872));
#258809=CARTESIAN_POINT('Ctrl Pts',(-5.60518064717923,-4.38553113848304,
135.74411288519));
#258810=CARTESIAN_POINT('Ctrl Pts',(-5.88362827099213,1.7854667809037,137.164088929876));
#258811=CARTESIAN_POINT('Ctrl Pts',(-6.16207589480503,6.31570795354138,
132.739785345549));
#258812=CARTESIAN_POINT('Ctrl Pts',(-6.44052351861788,5.04212205636089,
126.536920986959));
#258813=CARTESIAN_POINT('Ctrl Pts',(-6.71897114243081,-0.864927689259141,
124.255625172881));
#258814=CARTESIAN_POINT('Ctrl Pts',(-6.99741876624371,-5.97715114251656,
127.992297308957));
#258815=CARTESIAN_POINT('Ctrl Pts',(-7.27586639005655,-5.59666469586782,
134.313118248714));
#258816=CARTESIAN_POINT('Ctrl Pts',(-7.55431401386947,-0.0731168059870705,
137.409562337785));
#258817=CARTESIAN_POINT('Ctrl Pts',(-7.83276163768236,5.51762185664139,
134.436148728019));
#258818=CARTESIAN_POINT('Ctrl Pts',(-8.11120926149529,6.03793558382929,
128.125299267457));
#258819=CARTESIAN_POINT('Ctrl Pts',(-8.38965688530811,1.00968147902963,
124.276376308223));
#258820=CARTESIAN_POINT('Ctrl Pts',(-8.66810450912106,-4.94642057931569,
126.426352019512));
#258821=CARTESIAN_POINT('Ctrl Pts',(-8.94655213293394,-6.3570037713493,
132.599503754801));
#258822=CARTESIAN_POINT('Ctrl Pts',(-9.22499975674682,-1.92581105441205,
137.123006644589));
#258823=CARTESIAN_POINT('Ctrl Pts',(-9.50344738055969,4.27510794042973,
135.839982518561));
#258824=CARTESIAN_POINT('Ctrl Pts',(-9.78189500437264,6.54741158865002,
129.929467869325));
#258825=CARTESIAN_POINT('Ctrl Pts',(-10.0603426281855,2.80296384573913,
124.822936914835));
#258826=CARTESIAN_POINT('Ctrl Pts',(-10.3387902519984,-3.51727073900952,
125.213042134361));
#258827=CARTESIAN_POINT('Ctrl Pts',(-10.6172378758113,-6.60530534283666,
130.74129588886));
#258828=CARTESIAN_POINT('Ctrl Pts',(-10.8956854996242,-3.62338702370218,
136.327503048155));
#258829=CARTESIAN_POINT('Ctrl Pts',(-11.174133123437,2.68824695791763,136.838212134247));
#258830=CARTESIAN_POINT('Ctrl Pts',(-11.4525807472499,6.52951331337615,
131.804106446543));
#258831=CARTESIAN_POINT('Ctrl Pts',(-11.7310283710628,4.37047591830066,
125.851283182307));
#258832=CARTESIAN_POINT('Ctrl Pts',(-12.0094759948757,-1.80481533607482,
124.450096109789));
#258833=CARTESIAN_POINT('Ctrl Pts',(-12.2879236186886,-6.32156946672825,
128.88816769684));
#258834=CARTESIAN_POINT('Ctrl Pts',(-12.5663712425015,-5.02911008329581,
135.087126966809));
#258835=CARTESIAN_POINT('Ctrl Pts',(-12.8448188663144,0.884855780999501,
137.350433186591));
#258836=CARTESIAN_POINT('Ctrl Pts',(-13.1232664901273,5.98568241016441,
133.598218508862));
#258837=CARTESIAN_POINT('Ctrl Pts',(-13.4017141139402,5.58595932123025,
127.278584916578));
#258838=CARTESIAN_POINT('Ctrl Pts',(-13.6801617377531,0.0530125053692662,
124.198966949783));
#258839=CARTESIAN_POINT('Ctrl Pts',(-13.958609361566,-5.5286502131212,127.189383072259));
#258840=CARTESIAN_POINT('Ctrl Pts',(-14.2370569853788,-6.02975347533148,
133.501786957402));
#258841=CARTESIAN_POINT('Ctrl Pts',(-14.5155046091917,-0.989807863545592,
137.335387812837));
#258842=CARTESIAN_POINT('Ctrl Pts',(-14.7939522330047,4.95972282003631,
135.167293734234));
#258843=CARTESIAN_POINT('Ctrl Pts',(-15.0723998568175,6.35151052793477,
128.989877262545));
#258844=CARTESIAN_POINT('Ctrl Pts',(-15.3508474806304,1.9065703492003,124.479882351679));
#258845=CARTESIAN_POINT('Ctrl Pts',(-15.6292951044433,-4.29041483930959,
125.781773999224));
#258846=CARTESIAN_POINT('Ctrl Pts',(-15.9077427282562,-6.54471838891106,
131.699177382027));
#258847=CARTESIAN_POINT('Ctrl Pts',(-16.186190352069,-2.78474546637155,
136.794287872519));
#258848=CARTESIAN_POINT('Ctrl Pts',(-16.464637975882,3.53427249738445,136.384947839923));
#258849=CARTESIAN_POINT('Ctrl Pts',(-16.7430855996949,6.60546669485434,
130.847320776822));
#258850=CARTESIAN_POINT('Ctrl Pts',(-17.0215332235078,3.6065596947407,125.270215426085));
#258851=CARTESIAN_POINT('Ctrl Pts',(-17.2999808473206,-2.7065994746034,
124.778719148295));
#258852=CARTESIAN_POINT('Ctrl Pts',(-17.5784284711336,-6.53252595152224,
129.824493011814));
#258853=CARTESIAN_POINT('Ctrl Pts',(-17.8568760949464,-4.35538021062653,
135.770717335825));
#258854=CARTESIAN_POINT('Ctrl Pts',(-18.1353237187593,1.82414717168286,
137.153102455769));
#258855=CARTESIAN_POINT('Ctrl Pts',(-18.4137713425722,6.32737241775927,
132.701303979686));
#258856=CARTESIAN_POINT('Ctrl Pts',(-18.6922189663851,5.01605152124203,
126.506307224649));
#258857=CARTESIAN_POINT('Ctrl Pts',(-18.9706665901979,-0.904775675556959,
124.261011566121));
#258858=CARTESIAN_POINT('Ctrl Pts',(-19.2491142140109,-5.99415822726801,
128.028734025499));
#258859=CARTESIAN_POINT('Ctrl Pts',(-19.5275618378238,-5.57520219902858,
134.347121726088));
#258860=CARTESIAN_POINT('Ctrl Pts',(-19.8060094616367,-0.0329077136511566,
137.409885041447));
#258861=CARTESIAN_POINT('Ctrl Pts',(-20.0844570854496,5.53962735294063,
134.402494109067));
#258862=CARTESIAN_POINT('Ctrl Pts',(-20.3629047092624,6.02151550802112,
128.08859427659));
#258863=CARTESIAN_POINT('Ctrl Pts',(-20.6413523330754,0.969925078616457,
124.270351038909));
#258864=CARTESIAN_POINT('Ctrl Pts',(-20.9197999568882,-4.9729791145623,
126.456543399899));
#258865=CARTESIAN_POINT('Ctrl Pts',(-21.1982475807011,-6.34595844499429,
132.638167381246));
#258866=CARTESIAN_POINT('Ctrl Pts',(-21.476695204514,-1.88731198178147,
137.134612533211));
#258867=CARTESIAN_POINT('Ctrl Pts',(-21.7551428283269,4.30568199237261,
135.813865424697));
#258868=CARTESIAN_POINT('Ctrl Pts',(-22.0335904521398,6.54196455979519,
129.889628126344));
#258869=CARTESIAN_POINT('Ctrl Pts',(-22.3120380759527,2.766501289502,124.805985300257));
#258870=CARTESIAN_POINT('Ctrl Pts',(-22.5904856997656,-3.5512415147419,
125.234556353852));
#258871=CARTESIAN_POINT('Ctrl Pts',(-22.8689333235784,-6.60556685473091,
130.781505425734));
#258872=CARTESIAN_POINT('Ctrl Pts',(-23.1473809473914,-3.58969895510304,
136.349457302372));
#258873=CARTESIAN_POINT('Ctrl Pts',(-23.4258285712042,2.7249269177212,136.821736218705));
#258874=CARTESIAN_POINT('Ctrl Pts',(-23.7042761950172,6.53547807324032,
131.764340922733));
#258875=CARTESIAN_POINT('Ctrl Pts',(-23.98272381883,4.34024415530499,125.824770623956));
#258876=CARTESIAN_POINT('Ctrl Pts',(-24.2611714426429,-1.84346210864104,
124.461200262812));
#258877=CARTESIAN_POINT('Ctrl Pts',(-24.5396190664558,-6.33311675287646,
128.926684387076));
#258878=CARTESIAN_POINT('Ctrl Pts',(-24.8180666902687,-5.00294649117208,
135.117661237576));
#258879=CARTESIAN_POINT('Ctrl Pts',(-25.0965143140816,0.924687188395989,
137.344925534737));
#258880=CARTESIAN_POINT('Ctrl Pts',(-25.3749619378945,6.00257851530871,
133.561730197376));
#258881=CARTESIAN_POINT('Ctrl Pts',(-25.6534095617074,5.56439342891538,
127.244646921163));
#258882=CARTESIAN_POINT('Ctrl Pts',(-25.9318571855203,0.0128026170801758,
124.198766630261));
#258883=CARTESIAN_POINT('Ctrl Pts',(-26.2103048093331,-5.5505531744091,
127.223104512485));
#258884=CARTESIAN_POINT('Ctrl Pts',(-26.4887524331461,-6.01322175821376,
133.538441801192));
#258885=CARTESIAN_POINT('Ctrl Pts',(-26.7672000569589,-0.950033308434149,
137.341292049436));
#258886=CARTESIAN_POINT('Ctrl Pts',(-27.0456476807718,4.98618934008908,
135.137021658645));
#258887=CARTESIAN_POINT('Ctrl Pts',(-27.3240953045847,6.34034757396176,
128.951247433362));
#258888=CARTESIAN_POINT('Ctrl Pts',(-27.6025429283976,1.86803613056208,
124.468393694749));
#258889=CARTESIAN_POINT('Ctrl Pts',(-27.8809905522105,-4.32090925818572,
125.807984029013));
#258890=CARTESIAN_POINT('Ctrl Pts',(-28.1594381760234,-6.53915012681315,
131.739000361591));
#258891=CARTESIAN_POINT('Ctrl Pts',(-28.4378857998363,-2.74823148414282,
136.811128429099));
#258892=CARTESIAN_POINT('Ctrl Pts',(-28.7163334236492,3.56817763388296,
136.36333032473));
#258893=CARTESIAN_POINT('Ctrl Pts',(-28.994781047462,6.60560582153853,130.807110630244));
#258894=CARTESIAN_POINT('Ctrl Pts',(-29.273228671275,3.5728049609845,125.248363808452));
#258895=CARTESIAN_POINT('Ctrl Pts',(-29.5516762950878,-2.74322911748845,
124.795306628702));
#258896=CARTESIAN_POINT('Ctrl Pts',(-29.8301239189007,-6.53836965118233,
129.86427650611));
#258897=CARTESIAN_POINT('Ctrl Pts',(-30.1085715427137,-4.32506789255462,
135.797137756284));
#258898=CARTESIAN_POINT('Ctrl Pts',(-30.3870191665265,1.862759968018,137.141880726698));
#258899=CARTESIAN_POINT('Ctrl Pts',(-30.6654667903394,6.33880241886542,
132.662752321889));
#258900=CARTESIAN_POINT('Ctrl Pts',(-30.9439144141524,4.98979511448915,
126.475852728289));
#258901=CARTESIAN_POINT('Ctrl Pts',(-31.2223620379652,-0.944590135059391,
124.266640425567));
#258902=CARTESIAN_POINT('Ctrl Pts',(-31.5008096617781,-6.01094319628198,
128.065273593905));
#258903=CARTESIAN_POINT('Ctrl Pts',(-31.7792572855909,-5.55353311102158,
134.380993925146));
#258904=CARTESIAN_POINT('Ctrl Pts',(-32.0577049094039,0.00730259809219468,
137.409962974972));
#258905=CARTESIAN_POINT('Ctrl Pts',(-32.3361525332168,5.56142757631112,
134.368706159956));
#258906=CARTESIAN_POINT('Ctrl Pts',(-32.6146001570296,6.0048723027414,128.051989919443));
#258907=CARTESIAN_POINT('Ctrl Pts',(-32.8930477808425,0.930132737272799,
124.264567889721));
#258908=CARTESIAN_POINT('Ctrl Pts',(-33.1714954046555,-4.99935337423901,
126.486895890252));
#258909=CARTESIAN_POINT('Ctrl Pts',(-33.4499430284683,-6.33467796681538,
132.676763055306));
#258910=CARTESIAN_POINT('Ctrl Pts',(-33.7283906522812,-1.84874297411136,
137.145983852021));
#258911=CARTESIAN_POINT('Ctrl Pts',(-34.0068382760941,4.33609649568588,
135.787562701789));
#258912=CARTESIAN_POINT('Ctrl Pts',(-34.285285899907,6.53627511603778,129.849822279112));
#258913=CARTESIAN_POINT('Ctrl Pts',(-34.5637335237199,2.72993621954223,
124.789255957683));
#258914=CARTESIAN_POINT('Ctrl Pts',(-34.8421811475328,-3.58508069791401,
125.256276964487));
#258915=CARTESIAN_POINT('Ctrl Pts',(-35.1206287713457,-6.60558359491616,
130.821715809516));
#258916=CARTESIAN_POINT('Ctrl Pts',(-35.3990763951586,-3.55587786888901,
136.37120608099));
#258917=CARTESIAN_POINT('Ctrl Pts',(-35.6775240189714,2.76150590435573,
136.805037327097));
#258918=CARTESIAN_POINT('Ctrl Pts',(-35.9559716427844,6.54120065856107,
131.724539826499));
#258919=CARTESIAN_POINT('Ctrl Pts',(-36.2344192665972,4.30985156296601,
125.798442586144));
#258920=CARTESIAN_POINT('Ctrl Pts',(-36.5128668904101,-1.8820405710409,
124.472539463974));
#258921=CARTESIAN_POINT('Ctrl Pts',(-36.791314514223,-6.3444293630544,128.965270655295));
#258922=CARTESIAN_POINT('Ctrl Pts',(-37.0697621380359,-4.9765975130263,
135.148035677403));
#258923=CARTESIAN_POINT('Ctrl Pts',(-37.3482097618488,0.964484331168655,
137.339175519844));
#258924=CARTESIAN_POINT('Ctrl Pts',(-37.6266573856617,6.0192521926987,133.525139710547));
#258925=CARTESIAN_POINT('Ctrl Pts',(-37.9051050094746,5.54262134595571,
127.210840832248));
#258926=CARTESIAN_POINT('Ctrl Pts',(-38.1835526332875,-0.0274077456145885,
124.198811083455));
#258927=CARTESIAN_POINT('Ctrl Pts',(-38.4620002571004,-5.5722504579079,
127.256958657474));
#258928=CARTESIAN_POINT('Ctrl Pts',(-38.7404478809132,-5.99646721895241,
133.574995332598));
#258929=CARTESIAN_POINT('Ctrl Pts',(-39.0188955047262,-0.910223549489097,
137.346954057637));
#258930=CARTESIAN_POINT('Ctrl Pts',(-39.297343128539,5.0124710950622,135.106589034709));
#258931=CARTESIAN_POINT('Ctrl Pts',(-39.5757907523519,6.32894967607775,
128.912686271968));
#258932=CARTESIAN_POINT('Ctrl Pts',(-39.8542383761648,1.82943269115809,
124.457139819403));
#258933=CARTESIAN_POINT('Ctrl Pts',(-40.1326859999777,-4.35124356418029,
125.834379201373));
#258934=CARTESIAN_POINT('Ctrl Pts',(-40.4111336237906,-6.53333955410249,
131.778788707735));
#258935=CARTESIAN_POINT('Ctrl Pts',(-40.6895812476035,-2.7116156651858,
136.827746402689));
#258936=CARTESIAN_POINT('Ctrl Pts',(-40.9680288714165,3.60195055024708,
136.34150681987));
#258937=CARTESIAN_POINT('Ctrl Pts',(-41.2464764952292,6.60550017506977,
130.766900381762));
#258938=CARTESIAN_POINT('Ctrl Pts',(-41.5249241190422,3.53891783562657,
125.226718070324));
#258939=CARTESIAN_POINT('Ctrl Pts',(-41.803371742855,-2.77975710900975,
124.812116776814));
#258940=CARTESIAN_POINT('Ctrl Pts',(-42.081819366668,-6.5439710691505,129.904094835568));
#258941=CARTESIAN_POINT('Ctrl Pts',(-42.3602669904808,-4.2945953075014,
135.82337316755));
#258942=CARTESIAN_POINT('Ctrl Pts',(-42.6387146142937,1.90130373909722,
137.130424158489));
#258943=CARTESIAN_POINT('Ctrl Pts',(-42.9171622381066,6.34999753331677,
132.624131800705));
#258944=CARTESIAN_POINT('Ctrl Pts',(-43.1956098619195,4.96335380904355,
126.44555862638));
#258945=CARTESIAN_POINT('Ctrl Pts',(-43.4740574857324,-0.984369592426984,
124.272511542639));
#258946=CARTESIAN_POINT('Ctrl Pts',(-43.7525051095453,-6.02750542758532,
128.101914660188));
#258947=CARTESIAN_POINT('Ctrl Pts',(-44.0309527333582,-5.53165823480283,
134.414733590743));
#258948=CARTESIAN_POINT('Ctrl Pts',(-44.3094003571711,0.0475126392350714,
137.409796135472));
#258949=CARTESIAN_POINT('Ctrl Pts',(-44.5878479809839,5.58302171893757,
134.334786132711));
#258950=CARTESIAN_POINT('Ctrl Pts',(-44.8662956047969,5.98800658471021,
128.015487552405));
#258951=CARTESIAN_POINT('Ctrl Pts',(-45.1447432286098,0.890305929518511,
124.259027074959));
#258952=CARTESIAN_POINT('Ctrl Pts',(-45.4231908524226,-5.02554238103793,
126.517408365848));
#258953=CARTESIAN_POINT('Ctrl Pts',(-45.7016384762356,-6.32316275481482,
132.715289346806));
#258954=CARTESIAN_POINT('Ctrl Pts',(-45.9800861000484,-1.81010546059046,
137.15712017965));
#258955=CARTESIAN_POINT('Ctrl Pts',(-46.2585337238614,4.36635032334889,
135.761075324496));
#258956=CARTESIAN_POINT('Ctrl Pts',(-46.5369813476741,6.53034346820225,
129.810051802649));
#258957=CARTESIAN_POINT('Ctrl Pts',(-46.8154289714873,2.6932699907919,124.772749507024));
#258958=CARTESIAN_POINT('Ctrl Pts',(-47.0938765952999,-3.61878703460243,
125.278203161403));
#258959=CARTESIAN_POINT('Ctrl Pts',(-47.3723242191129,-6.60535556277213,
130.861925550195));
#258960=CARTESIAN_POINT('Ctrl Pts',(-47.6507718429257,-3.52192501831287,
136.392748578105));
#258961=CARTESIAN_POINT('Ctrl Pts',(-47.9292194667387,2.79798256237344,
136.788116078208));
#258962=CARTESIAN_POINT('Ctrl Pts',(-48.2076670905515,6.54668085728591,
131.684704632686));
#258963=CARTESIAN_POINT('Ctrl Pts',(-48.4861147143645,4.27929926749242,
125.772300044465));
#258964=CARTESIAN_POINT('Ctrl Pts',(-48.7645623381774,-1.92054929373528,
124.484113293097));
#258965=CARTESIAN_POINT('Ctrl Pts',(-49.0430099619902,-6.35550687806913,
129.003925071669));
#258966=CARTESIAN_POINT('Ctrl Pts',(-49.3214575858032,-4.95006412522954,
135.178249160753));
#258967=CARTESIAN_POINT('Ctrl Pts',(-49.5999052096159,1.00424573461974,
137.333183354982));
#258968=CARTESIAN_POINT('Ctrl Pts',(-49.878352833429,6.03570282448511,133.488448404247));
#258969=CARTESIAN_POINT('Ctrl Pts',(-50.1568004572417,5.52064387912377,
127.17716790253));
#258970=CARTESIAN_POINT('Ctrl Pts',(-50.4352480810547,-0.0676170927052693,
124.199100307716));
#258971=CARTESIAN_POINT('Ctrl Pts',(-50.7136957048675,-5.5937412596168,
127.290944252747));
#258972=CARTESIAN_POINT('Ctrl Pts',(-50.9921433286805,-5.97949047839309,
133.611446197116));
#258973=CARTESIAN_POINT('Ctrl Pts',(-51.2705909524933,-0.870380061875472,
137.352373627632));
#258974=CARTESIAN_POINT('Ctrl Pts',(-51.5490385763063,5.03856711107574,
135.075996990117));
#258975=CARTESIAN_POINT('Ctrl Pts',(-51.8274862001192,6.31731725663583,
128.874195207264));
#258976=CARTESIAN_POINT('Ctrl Pts',(-52.105933823932,1.79076146145295,124.446121142656));
#258977=CARTESIAN_POINT('Ctrl Pts',(-52.3843814477449,-4.38141663324442,
125.860958538224));
#258978=CARTESIAN_POINT('Ctrl Pts',(-52.6628290715579,-6.52728688609205,
131.818540946088));
#258979=CARTESIAN_POINT('Ctrl Pts',(-52.9412766953706,-2.67489936631311,
136.844141177504));
#258980=CARTESIAN_POINT('Ctrl Pts',(-53.2197243191836,3.63558999500893,
136.319478134021));
#258981=CARTESIAN_POINT('Ctrl Pts',(-53.4981719429964,6.60514975936288,
130.726691521383));
#258982=CARTESIAN_POINT('Ctrl Pts',(-53.7766195668094,3.50489957436681,
125.205279013792));
#258983=CARTESIAN_POINT('Ctrl Pts',(-54.0550671906223,-2.8161820956091,
124.829148969725));
#258984=CARTESIAN_POINT('Ctrl Pts',(-54.3335148144351,-6.54932999786417,
129.943946524707));
#258985=CARTESIAN_POINT('Ctrl Pts',(-54.6119624382481,-4.26396358463975,
135.849422597461));
#258986=CARTESIAN_POINT('Ctrl Pts',(-54.890410062061,1.93977705666721,137.11873317567));
#258987=CARTESIAN_POINT('Ctrl Pts',(-55.1688576858738,6.3609573462743,132.58544384723));
#258988=CARTESIAN_POINT('Ctrl Pts',(-55.4473053096868,4.93672858469731,
126.415426041482));
#258989=CARTESIAN_POINT('Ctrl Pts',(-55.7257529334997,-1.02411257361735,
124.278624699781));
#258990=CARTESIAN_POINT('Ctrl Pts',(-56.0042005573125,-6.0438443074584,
128.138655866601));
#258991=CARTESIAN_POINT('Ctrl Pts',(-56.2826481811254,-5.50957838095395,
134.448339472641));
#258992=CARTESIAN_POINT('Ctrl Pts',(-56.5610958049383,0.0877209197796484,
137.40938452913));
#258993=CARTESIAN_POINT('Ctrl Pts',(-56.8395434287512,5.60440898064107,
134.300735284249));
#258994=CARTESIAN_POINT('Ctrl Pts',(-57.117991052564,5.97091897889293,127.979088528083));
#258995=CARTESIAN_POINT('Ctrl Pts',(-57.396438676377,0.850446131150592,
124.253728799937));
#258996=CARTESIAN_POINT('Ctrl Pts',(-57.6748863001899,-5.05154516451579,
126.548079696037));
#258997=CARTESIAN_POINT('Ctrl Pts',(-57.9533339240027,-6.31141323569307,
132.753744828139));
#258998=CARTESIAN_POINT('Ctrl Pts',(-58.2317815478157,-1.77140087294607,
137.168021103437));
#258999=CARTESIAN_POINT('Ctrl Pts',(-58.5102291716285,4.39644235429495,
135.734404274317));
#259000=CARTESIAN_POINT('Ctrl Pts',(-58.7886767954414,6.52416983608798,
129.770318170665));
#259001=CARTESIAN_POINT('Ctrl Pts',(-59.0671244192543,2.65650396193163,
124.756466559932));
#259002=CARTESIAN_POINT('Ctrl Pts',(-59.3455720430672,-3.6523592758065,
125.300334132115));
#259003=CARTESIAN_POINT('Ctrl Pts',(-59.62401966688,-6.60488276674858,130.902133157784));
#259004=CARTESIAN_POINT('Ctrl Pts',(-59.902467290693,-3.48784166150989,
136.414083995446));
#259005=CARTESIAN_POINT('Ctrl Pts',(-60.1809149145059,2.83435554011865,
136.770973099059));
#259006=CARTESIAN_POINT('Ctrl Pts',(-60.4593625383188,6.55191846634393,
131.644836817403));
#259007=CARTESIAN_POINT('Ctrl Pts',(-60.7378101621316,4.24858840101079,
125.746343967642));
#259008=CARTESIAN_POINT('Ctrl Pts',(-61.0162577859445,-1.95898684976931,
124.49592132131));
#259009=CARTESIAN_POINT('Ctrl Pts',(-61.2947054097575,-6.36634888743926,
129.042646203845));
#259010=CARTESIAN_POINT('Ctrl Pts',(-61.5731530335703,-4.92334731098624,
135.208300568055));
#259011=CARTESIAN_POINT('Ctrl Pts',(-61.8516006573832,1.04396992537583,
137.326949262193));
#259012=CARTESIAN_POINT('Ctrl Pts',(-62.1300482811962,6.05192980108374,
133.451657638088));
#259013=CARTESIAN_POINT('Ctrl Pts',(-62.408495905009,5.49846184280268,127.143629379772));
#259014=CARTESIAN_POINT('Ctrl Pts',(-62.6869435288219,-0.107823934219708,
124.199634292325));
#259015=CARTESIAN_POINT('Ctrl Pts',(-62.9653911526347,-5.61502478318622,
127.325060038955));
#259016=CARTESIAN_POINT('Ctrl Pts',(-63.2438387764477,-5.96229216561512,
133.647793044045));
#259017=CARTESIAN_POINT('Ctrl Pts',(-63.5222864002605,-0.830504322008783,
137.357550558596));
#259018=CARTESIAN_POINT('Ctrl Pts',(-63.8007340240734,5.06447642113188,
135.045246658467));
#259019=CARTESIAN_POINT('Ctrl Pts',(-64.0791816478864,6.30545074667997,
128.835775665549));
#259020=CARTESIAN_POINT('Ctrl Pts',(-64.3576292716992,1.75202387442331,
124.435338072814));
#259021=CARTESIAN_POINT('Ctrl Pts',(-64.6360768955121,-4.41142734730395,
125.887721054655));
#259022=CARTESIAN_POINT('Ctrl Pts',(-64.914524519325,-6.52099234706562,
131.858255603616));
#259023=CARTESIAN_POINT('Ctrl Pts',(-65.1929721431379,-2.63808394806071,
136.860312146029));
#259024=CARTESIAN_POINT('Ctrl Pts',(-65.4714197669508,3.66909472164654,
136.297245083462));
#259025=CARTESIAN_POINT('Ctrl Pts',(-65.7498673907637,6.60455458740261,
130.686485539062));
#259026=CARTESIAN_POINT('Ctrl Pts',(-66.0283150145766,3.4707514377644,125.184047433287));
#259027=CARTESIAN_POINT('Ctrl Pts',(-66.3067626383895,-2.85250272754526,
124.846402576302));
#259028=CARTESIAN_POINT('Ctrl Pts',(-66.5852102622024,-6.55444623874626,
129.983830096806));
#259029=CARTESIAN_POINT('Ctrl Pts',(-66.8636578860152,-4.23317385903938,
135.875285080744));
#259030=CARTESIAN_POINT('Ctrl Pts',(-67.1421055098281,1.978178495085,137.106808211453));
#259031=CARTESIAN_POINT('Ctrl Pts',(-67.4205531336411,6.37168145161813,
132.546689895061));
#259032=CARTESIAN_POINT('Ctrl Pts',(-67.6990007574539,4.90992042805787,
126.385456090168));
#259033=CARTESIAN_POINT('Ctrl Pts',(-67.9774483812669,-1.06381760593968,
124.284979670466));
#259034=CARTESIAN_POINT('Ctrl Pts',(-68.2558960050797,-6.05995923045808,
128.175495851683));
#259035=CARTESIAN_POINT('Ctrl Pts',(-68.5343436288926,-5.48729436765201,
134.481810325563));
#259036=CARTESIAN_POINT('Ctrl Pts',(-68.8127912527054,0.12792594979327,
137.408728171199));
#259037=CARTESIAN_POINT('Ctrl Pts',(-69.0912388765185,5.62558856890878,
134.266554876337));
#259038=CARTESIAN_POINT('Ctrl Pts',(-69.3696865003312,5.9536101184771,127.942794195258));
#259039=CARTESIAN_POINT('Ctrl Pts',(-69.6481341241442,0.810554819188534,
124.248673260987));
#259040=CARTESIAN_POINT('Ctrl Pts',(-69.9265817479571,-5.07736076112986,
126.578908744281));
#259041=CARTESIAN_POINT('Ctrl Pts',(-70.2050293717699,-6.29942984483285,
132.792128074323));
#259042=CARTESIAN_POINT('Ctrl Pts',(-70.4834769955829,-1.73263064539088,
137.178686219444));
#259043=CARTESIAN_POINT('Ctrl Pts',(-70.7619246193956,4.42637147345276,
135.707550539556));
#259044=CARTESIAN_POINT('Ctrl Pts',(-71.0403722432087,6.51775444846118,
129.730622855503));
#259045=CARTESIAN_POINT('Ctrl Pts',(-71.3188198670216,2.6196394953401,124.740407719779));
#259046=CARTESIAN_POINT('Ctrl Pts',(-71.5972674908343,-3.68579617749442,
125.322669056552));
#259047=CARTESIAN_POINT('Ctrl Pts',(-71.8757151146474,-6.6041652243652,
130.942337142376));
#259048=CARTESIAN_POINT('Ctrl Pts',(-72.1541627384602,-3.45362906145158,
136.435211542427));
#259049=CARTESIAN_POINT('Ctrl Pts',(-72.4326103622731,2.87062348977667,
136.753609024891));
#259050=CARTESIAN_POINT('Ctrl Pts',(-72.711057986086,6.55691329165398,131.604937857965));
#259051=CARTESIAN_POINT('Ctrl Pts',(-72.9895056098989,4.21772010152317,
125.720575317484));
#259052=CARTESIAN_POINT('Ctrl Pts',(-73.2679532337117,-1.99735181482566,
124.50796311106));
#259053=CARTESIAN_POINT('Ctrl Pts',(-73.5464008575247,-6.37695498941029,
129.081432616995));
#259054=CARTESIAN_POINT('Ctrl Pts',(-73.8248484813376,-4.89644806029751,
135.238188785743));
#259055=CARTESIAN_POINT('Ctrl Pts',(-74.1032961051504,1.08365543144292,
137.320473472483));
#259056=CARTESIAN_POINT('Ctrl Pts',(-74.3817437289633,6.06793252119795,
133.414768775364));
#259057=CARTESIAN_POINT('Ctrl Pts',(-74.6601913527762,5.47607605895596,
127.110226506756));
#259058=CARTESIAN_POINT('Ctrl Pts',(-74.9386389765891,-0.148026780279403,
124.200413017498));
#259059=CARTESIAN_POINT('Ctrl Pts',(-75.217086600402,-5.63610023994771,
127.359304751927));
#259060=CARTESIAN_POINT('Ctrl Pts',(-75.4955342242149,-5.94487291790794,
133.684034526541));
#259061=CARTESIAN_POINT('Ctrl Pts',(-75.7739818480278,-0.790597807498519,
137.362484658699));
#259062=CARTESIAN_POINT('Ctrl Pts',(-76.0524294718406,5.09019806515201,
135.014339179226));
#259063=CARTESIAN_POINT('Ctrl Pts',(-76.3308770956536,6.29335058592772,
128.797429070474));
#259064=CARTESIAN_POINT('Ctrl Pts',(-76.6093247194664,1.71322136550425,
124.424791009442));
#259065=CARTESIAN_POINT('Ctrl Pts',(-76.8877723432794,-4.44127459430165,
125.914665758975));
#259066=CARTESIAN_POINT('Ctrl Pts',(-77.1662199670922,-6.51445617026952,
131.89793120868));
#259067=CARTESIAN_POINT('Ctrl Pts',(-77.4446675909052,-2.60117077463652,
136.876258709042));
#259068=CARTESIAN_POINT('Ctrl Pts',(-77.7231152147181,3.7024634886308,136.274808492052));
#259069=CARTESIAN_POINT('Ctrl Pts',(-78.0015628385308,6.60371468124315,
130.646283924643));
#259070=CARTESIAN_POINT('Ctrl Pts',(-78.2800104623438,3.43647469119047,
125.163024115555));
#259071=CARTESIAN_POINT('Ctrl Pts',(-78.5584580861567,-2.88871765894464,
124.863876957204));
#259072=CARTESIAN_POINT('Ctrl Pts',(-78.8369057099696,-6.55931960221255,
130.023744073965));
#259073=CARTESIAN_POINT('Ctrl Pts',(-79.1153533337825,-4.20222727162433,
135.900959659057));
#259074=CARTESIAN_POINT('Ctrl Pts',(-79.3938009575953,2.01650663137172,
137.094649707722));
#259075=CARTESIAN_POINT('Ctrl Pts',(-79.6722485814083,6.38216945196263,
132.507871380239));
#259076=CARTESIAN_POINT('Ctrl Pts',(-79.9506962052212,4.88293033251105,
126.355649882987));
#259077=CARTESIAN_POINT('Ctrl Pts',(-80.229143829034,-1.10348321810992,
124.29157621921));
#259078=CARTESIAN_POINT('Ctrl Pts',(-80.507591452847,-6.07584959944043,
128.212433250316));
#259079=CARTESIAN_POINT('Ctrl Pts',(-80.7860390766598,-5.46480702063872,
134.515144909234));
#259080=CARTESIAN_POINT('Ctrl Pts',(-81.0644867004727,0.168126239464741,
137.407827085998));
#259081=CARTESIAN_POINT('Ctrl Pts',(-81.3429343242857,5.64655969892388,
134.232246175545));
#259082=CARTESIAN_POINT('Ctrl Pts',(-81.6213819480984,5.93608064484842,
127.906605898828));
#259083=CARTESIAN_POINT('Ctrl Pts',(-81.8998295719115,0.770633471818905,
124.243860645443));
#259084=CARTESIAN_POINT('Ctrl Pts',(-82.1782771957242,-5.10298821427442,
126.609894368197));
#259085=CARTESIAN_POINT('Ctrl Pts',(-82.4567248195372,-6.28721302628274,
132.830437663053));
#259086=CARTESIAN_POINT('Ctrl Pts',(-82.7351724433501,-1.69379621456928,
137.189115132473));
#259087=CARTESIAN_POINT('Ctrl Pts',(-83.0136200671628,4.45613657178832,
135.680515115291));
#259088=CARTESIAN_POINT('Ctrl Pts',(-83.2920676909759,6.51109754304618,
129.690967328089));
#259089=CARTESIAN_POINT('Ctrl Pts',(-83.5705153147887,2.58267795704331,
124.724573581631));
#259090=CARTESIAN_POINT('Ctrl Pts',(-83.8489629386017,-3.71909650065006,
125.345207107088));
#259091=CARTESIAN_POINT('Ctrl Pts',(-84.1274105624144,-6.60320296221082,
130.982536014198));
#259092=CARTESIAN_POINT('Ctrl Pts',(-84.4058581862275,-3.41928848589759,
136.456130436155));
#259093=CARTESIAN_POINT('Ctrl Pts',(-84.6843058100402,2.90678506742617,
136.736024499134));
#259094=CARTESIAN_POINT('Ctrl Pts',(-84.9627534338533,6.56166514813073,
131.565009232842));
#259095=CARTESIAN_POINT('Ctrl Pts',(-85.241201057666,4.1866955128661,125.694995048862));
#259096=CARTESIAN_POINT('Ctrl Pts',(-85.519648681479,-2.03564276727566,
124.520238216135));
#259097=CARTESIAN_POINT('Ctrl Pts',(-85.7980963052919,-6.38732479096924,
129.120282873878));
#259098=CARTESIAN_POINT('Ctrl Pts',(-86.0765439291047,-4.8693673699251,
135.267912706297));
#259099=CARTESIAN_POINT('Ctrl Pts',(-86.3549915529177,1.12330078225909,
137.313756225814));
#259100=CARTESIAN_POINT('Ctrl Pts',(-86.6334391767305,6.08371039184151,
133.377783183006));
#259101=CARTESIAN_POINT('Ctrl Pts',(-86.9118868005434,5.45348735709659,
127.076960521238));
#259102=CARTESIAN_POINT('Ctrl Pts',(-87.1903344243564,-0.188224141151809,
124.201436454379));
#259103=CARTESIAN_POINT('Ctrl Pts',(-87.4687820481692,-5.65696684894189,
127.39367712271));
#259104=CARTESIAN_POINT('Ctrl Pts',(-87.7472296719821,-5.92723338074904,
133.720169301662));
#259105=CARTESIAN_POINT('Ctrl Pts',(-88.0256772957949,-0.750661997095914,
137.367175745102));
#259106=CARTESIAN_POINT('Ctrl Pts',(-88.3041249196079,5.11573109001074,
134.983275697681));
#259107=CARTESIAN_POINT('Ctrl Pts',(-88.5825725434208,6.28101722275544,
128.759156842984));
#259108=CARTESIAN_POINT('Ctrl Pts',(-88.8610201672337,1.67435537253749,
124.414480343369));
#259109=CARTESIAN_POINT('Ctrl Pts',(-89.1394677910466,-4.47095726823472,
125.941791652735));
#259110=CARTESIAN_POINT('Ctrl Pts',(-89.4179154148595,-6.50767859790483,
131.93756629108));
#259111=CARTESIAN_POINT('Ctrl Pts',(-89.6963630386723,-2.56416121387375,
136.891980275641));
#259112=CARTESIAN_POINT('Ctrl Pts',(-89.9748106624853,3.73569505946763,
136.252169191183));
#259113=CARTESIAN_POINT('Ctrl Pts',(-90.253258286298,6.60263007200808,130.606088167816));
#259114=CARTESIAN_POINT('Ctrl Pts',(-90.5317059101111,3.40207060478355,
125.142209839621));
#259115=CARTESIAN_POINT('Ctrl Pts',(-90.8101535339238,-2.9248255478482,
124.881571464914));
#259116=CARTESIAN_POINT('Ctrl Pts',(-91.0886011577368,-6.56394990767886,
130.063686977158));
#259117=CARTESIAN_POINT('Ctrl Pts',(-91.3670487815497,-4.17112496913288,
135.926445381018));
#259118=CARTESIAN_POINT('Ctrl Pts',(-91.6454964053626,2.05476004526333,
137.082258115016));
#259119=CARTESIAN_POINT('Ctrl Pts',(-91.9239440291755,6.39242095867105,
132.468989741201));
#259120=CARTESIAN_POINT('Ctrl Pts',(-92.2023916529884,4.85575929818535,
126.326008524418));
#259121=CARTESIAN_POINT('Ctrl Pts',(-92.4808392768012,-1.14310794030347,
124.298414101576));
#259122=CARTESIAN_POINT('Ctrl Pts',(-92.7592869006141,-6.09151482558059,
128.249466693771));
#259123=CARTESIAN_POINT('Ctrl Pts',(-93.0377345244271,-5.44211717319261,
134.548341988427));
#259124=CARTESIAN_POINT('Ctrl Pts',(-93.3161821482399,0.208320299155509,
137.406681306919));
#259125=CARTESIAN_POINT('Ctrl Pts',(-93.5946297720528,5.6673215935918,134.197810453193));
#259126=CARTESIAN_POINT('Ctrl Pts',(-93.8730773958657,5.91833120756931,
127.870524979765));
#259127=CARTESIAN_POINT('Ctrl Pts',(-94.1515250196785,0.730683568342929,
124.239291131637));
#259128=CARTESIAN_POINT('Ctrl Pts',(-94.4299726434915,-5.12842657431339,
126.641035419604));
#259129=CARTESIAN_POINT('Ctrl Pts',(-94.7084202673044,-6.27476323274215,
132.868672174754));
#259130=CARTESIAN_POINT('Ctrl Pts',(-94.9868678911172,-1.6548990195065,
137.199307456074));
#259131=CARTESIAN_POINT('Ctrl Pts',(-95.2653155149302,4.48573654634406,
135.653299003326));
#259132=CARTESIAN_POINT('Ctrl Pts',(-95.543763138743,6.50419936651746,129.651353057874));
#259133=CARTESIAN_POINT('Ctrl Pts',(-95.822210762556,2.54562071666526,124.708964732227));
#259134=CARTESIAN_POINT('Ctrl Pts',(-96.1006583863688,-3.75225901131679,
125.367947448562));
#259135=CARTESIAN_POINT('Ctrl Pts',(-96.3791060101818,-6.60199601594203,
131.022728283664));
#259136=CARTESIAN_POINT('Ctrl Pts',(-96.6575536339946,-3.38482120735248,
136.476839901474));
#259137=CARTESIAN_POINT('Ctrl Pts',(-96.9360012578075,2.94283893308538,
136.718220173391));
#259138=CARTESIAN_POINT('Ctrl Pts',(-97.2144488816204,6.5661738596919,131.525052421605));
#259139=CARTESIAN_POINT('Ctrl Pts',(-97.4928965054334,4.15551578466796,
125.669604109659));
#259140=CARTESIAN_POINT('Ctrl Pts',(-97.771344129246,-2.07385828823457,
124.532746181678));
#259141=CARTESIAN_POINT('Ctrl Pts',(-98.0497917530593,-6.39745790785863,
129.15919553488));
#259142=CARTESIAN_POINT('Ctrl Pts',(-98.3282393768718,-4.84210624335443,
135.297471228287));
#259143=CARTESIAN_POINT('Ctrl Pts',(-98.606687000685,1.16290450875192,137.306797771098));
#259144=CARTESIAN_POINT('Ctrl Pts',(-98.8851346244975,6.09926282835875,
133.340702231527));
#259145=CARTESIAN_POINT('Ctrl Pts',(-99.1635822483109,5.43069657425812,
127.043832655902));
#259146=CARTESIAN_POINT('Ctrl Pts',(-99.4420298721233,-0.228414527308866,
124.202704565042));
#259147=CARTESIAN_POINT('Ctrl Pts',(-99.7204774959365,-5.67762383694899,
127.428175877623));
#259148=CARTESIAN_POINT('Ctrl Pts',(-99.9989251197493,-5.90937420777732,
133.756196030418));
#259149=CARTESIAN_POINT('Ctrl Pts',(-100.277372743562,-0.710698370637635,
137.371623643978));
#259150=CARTESIAN_POINT('Ctrl Pts',(-100.555820367375,5.14107454957247,
134.9520573649));
#259151=CARTESIAN_POINT('Ctrl Pts',(-100.834267991188,6.26845111417983,
128.720960401273));
#259152=CARTESIAN_POINT('Ctrl Pts',(-101.112715615001,1.63542733571746,
124.404406456659));
#259153=CARTESIAN_POINT('Ctrl Pts',(-101.391163238814,-4.50047426920288,
125.969097730777));
#259154=CARTESIAN_POINT('Ctrl Pts',(-101.669610862627,-6.50065988111587,
131.977159382129));
#259155=CARTESIAN_POINT('Ctrl Pts',(-101.94805848644,-2.52705663717401,
136.907476263252));
#259156=CARTESIAN_POINT('Ctrl Pts',(-102.226506110253,3.76878820275105,
136.229328019765));
#259157=CARTESIAN_POINT('Ctrl Pts',(-102.504953734065,6.60130079988703,
130.565899758046));
#259158=CARTESIAN_POINT('Ctrl Pts',(-102.783401357878,3.36754045339959,
125.121605376767));
#259159=CARTESIAN_POINT('Ctrl Pts',(-103.061848981691,-2.96082505626518,
124.899485443752));
#259160=CARTESIAN_POINT('Ctrl Pts',(-103.340296605504,-6.56833698356739,
130.103657326284));
#259161=CARTESIAN_POINT('Ctrl Pts',(-103.618744229317,-4.13986810407194,
135.951741302244));
#259162=CARTESIAN_POINT('Ctrl Pts',(-103.89719185313,2.0929373192654,137.06963389251));
#259163=CARTESIAN_POINT('Ctrl Pts',(-104.175639476943,6.40243559186997,
132.430046418718));
#259164=CARTESIAN_POINT('Ctrl Pts',(-104.454087100755,4.82840833191319,
126.296533112833));
#259165=CARTESIAN_POINT('Ctrl Pts',(-104.732534724569,-1.18269030421136,
124.305493064181));
#259166=CARTESIAN_POINT('Ctrl Pts',(-105.010982348381,-6.10695432839948,
128.286594809759));
#259167=CARTESIAN_POINT('Ctrl Pts',(-105.289429972194,-5.41922566609253,
134.581400333014));
#259168=CARTESIAN_POINT('Ctrl Pts',(-105.567877596007,0.248506639461218,
137.40529087642));
#259169=CARTESIAN_POINT('Ctrl Pts',(-105.84632521982,5.68787348357469,134.163248985309));
#259170=CARTESIAN_POINT('Ctrl Pts',(-106.124772843633,5.90036246435008,
127.834552775061));
#259171=CARTESIAN_POINT('Ctrl Pts',(-106.403220467446,0.690706589119241,
124.234964888896));
#259172=CARTESIAN_POINT('Ctrl Pts',(-106.681668091259,-5.1536748986197,
126.672330744555));
#259173=CARTESIAN_POINT('Ctrl Pts',(-106.960115715072,-6.26208092554253,
132.906830192629));
#259174=CARTESIAN_POINT('Ctrl Pts',(-107.238563338885,-1.61594050155245,
137.209262812568));
#259175=CARTESIAN_POINT('Ctrl Pts',(-107.517010962697,4.51517030028232,
135.625903212168));
#259176=CARTESIAN_POINT('Ctrl Pts',(-107.79545858651,6.49706017448951,129.611781512777));
#259177=CARTESIAN_POINT('Ctrl Pts',(-108.073906210323,2.50846914737518,
124.69358174996));
#259178=CARTESIAN_POINT('Ctrl Pts',(-108.352353834136,-3.78528248064593,
125.390889238328));
#259179=CARTESIAN_POINT('Ctrl Pts',(-108.630801457949,-6.60054443028347,
131.062912461436));
#259180=CARTESIAN_POINT('Ctrl Pts',(-108.909249081762,-3.35022850301195,
136.497339170987));
#259181=CARTESIAN_POINT('Ctrl Pts',(-109.187696705575,2.97878375076591,
136.700196707408));
#259182=CARTESIAN_POINT('Ctrl Pts',(-109.466144329388,6.57043925926657,
131.485068904869));
#259183=CARTESIAN_POINT('Ctrl Pts',(-109.7445919532,4.12418207230337,125.644403440746));
#259184=CARTESIAN_POINT('Ctrl Pts',(-110.023039577014,-2.11199696161116,
124.5454865442));
#259185=CARTESIAN_POINT('Ctrl Pts',(-110.301487200826,-6.40735396459295,
129.198169158078));
#259186=CARTESIAN_POINT('Ctrl Pts',(-110.579934824639,-4.81466569075636,
135.326863256411));
#259187=CARTESIAN_POINT('Ctrl Pts',(-110.858382448452,1.20246514338981,
137.299598366182));
#259188=CARTESIAN_POINT('Ctrl Pts',(-111.136830072265,6.11458925444912,
133.303527294979));
#259189=CARTESIAN_POINT('Ctrl Pts',(-111.415277696078,5.407704554961,127.010844138312));
#259190=CARTESIAN_POINT('Ctrl Pts',(-111.693725319891,-0.268596449482207,
124.204217302498));
#259191=CARTESIAN_POINT('Ctrl Pts',(-111.972172943703,-5.69807043851701,
127.462799738304));
#259192=CARTESIAN_POINT('Ctrl Pts',(-112.250620567517,-5.89129606077132,
133.792113377828));
#259193=CARTESIAN_POINT('Ctrl Pts',(-112.529068191329,-0.670708408989202,
137.375828190507));
#259194=CARTESIAN_POINT('Ctrl Pts',(-112.807515815142,5.16622750472631,
134.920685337692));
#259195=CARTESIAN_POINT('Ctrl Pts',(-113.085963438955,6.25565272584325,
128.682841160722));
#259196=CARTESIAN_POINT('Ctrl Pts',(-113.364411062768,1.5964386975353,124.394569722605));
#259197=CARTESIAN_POINT('Ctrl Pts',(-113.642858686581,-4.52982450344111,
125.996582981263));
#259198=CARTESIAN_POINT('Ctrl Pts',(-113.921306310394,-6.49340027998504,
132.016709014688));
#259199=CARTESIAN_POINT('Ctrl Pts',(-114.199753934207,-2.48985841946147,
136.922746097669));
#259200=CARTESIAN_POINT('Ctrl Pts',(-114.47820155802,3.80174169220082,136.206285824184));
#259201=CARTESIAN_POINT('Ctrl Pts',(-114.756649181833,6.59972691413776,
130.525720184532));
#259202=CARTESIAN_POINT('Ctrl Pts',(-115.035096805645,3.3328855165654,125.101211490497));
#259203=CARTESIAN_POINT('Ctrl Pts',(-115.313544429458,-2.99671485022117,
124.917618229914));
#259204=CARTESIAN_POINT('Ctrl Pts',(-115.591992053271,-6.57248066731354,
130.143653640229));
#259205=CARTESIAN_POINT('Ctrl Pts',(-115.870439677084,-4.10845783467579,
135.976846485386));
#259206=CARTESIAN_POINT('Ctrl Pts',(-116.148887300897,2.13103703870585,
137.056777507999));
#259207=CARTESIAN_POINT('Ctrl Pts',(-116.42733492471,6.41221298046361,132.391042855849));
#259208=CARTESIAN_POINT('Ctrl Pts',(-116.705782548523,4.8008784471946,126.267224740454));
#259209=CARTESIAN_POINT('Ctrl Pts',(-116.984230172336,-1.22222884309565,
124.312812844714));
#259210=CARTESIAN_POINT('Ctrl Pts',(-117.262677796149,-6.12216753577917,
128.323816222486));
#259211=CARTESIAN_POINT('Ctrl Pts',(-117.541125419961,-5.39613334759327,
134.614318718005));
#259212=CARTESIAN_POINT('Ctrl Pts',(-117.819573043774,0.288683771261777,
137.403655846021));
#259213=CARTESIAN_POINT('Ctrl Pts',(-118.098020667587,5.70821460731317,
134.128563052582));
#259214=CARTESIAN_POINT('Ctrl Pts',(-118.3764682914,5.88217508103065,127.79869061768));
#259215=CARTESIAN_POINT('Ctrl Pts',(-118.654915915213,0.650704015508265,
124.230882077529));
#259216=CARTESIAN_POINT('Ctrl Pts',(-118.933363539026,-5.17873225160735,
126.703779183394));
#259217=CARTESIAN_POINT('Ctrl Pts',(-119.211811162839,-6.24916657463125,
132.944910302722));
#259218=CARTESIAN_POINT('Ctrl Pts',(-119.490258786652,-1.57692210432836,
137.218980833058));
#259219=CARTESIAN_POINT('Ctrl Pts',(-119.768706410464,4.54443674292479,
135.598328756974));
#259220=CARTESIAN_POINT('Ctrl Pts',(-120.047154034278,6.48968023150711,
129.572254159139));
#259221=CARTESIAN_POINT('Ctrl Pts',(-120.32560165809,2.47122462583917,124.67842520485));
#259222=CARTESIAN_POINT('Ctrl Pts',(-120.604049281903,-3.81816568494053,
125.414031626265));
#259223=CARTESIAN_POINT('Ctrl Pts',(-120.882496905716,-6.59884825902321,
131.103087058474));
#259224=CARTESIAN_POINT('Ctrl Pts',(-121.160944529529,-3.31551165472302,
136.517627485086));
#259225=CARTESIAN_POINT('Ctrl Pts',(-121.439392153342,3.0146181885189,136.68195476905));
#259226=CARTESIAN_POINT('Ctrl Pts',(-121.717839777155,6.57446118879764,
131.445060164237));
#259227=CARTESIAN_POINT('Ctrl Pts',(-121.996287400968,4.0926955368563,125.619393975946));
#259228=CARTESIAN_POINT('Ctrl Pts',(-122.274735024781,-2.15005737416446,
124.5584588316));
#259229=CARTESIAN_POINT('Ctrl Pts',(-122.553182648593,-6.41701259446945,
129.237202299292));
#259230=CARTESIAN_POINT('Ctrl Pts',(-122.831630272406,-4.7870467289504,
135.356087701536));
#259231=CARTESIAN_POINT('Ctrl Pts',(-123.110077896219,1.24198122024032,
137.292158277842));
#259232=CARTESIAN_POINT('Ctrl Pts',(-123.388525520032,6.1296891021858,133.266259750888));
#259233=CARTESIAN_POINT('Ctrl Pts',(-123.666973143845,5.38451215118288,
126.97799619087));
#259234=CARTESIAN_POINT('Ctrl Pts',(-123.945420767658,-0.30876841871475,
124.20597461069));
#259235=CARTESIAN_POINT('Ctrl Pts',(-124.223868391471,-5.71830589598935,
127.497547421752));
#259236=CARTESIAN_POINT('Ctrl Pts',(-124.502316015284,-5.87299960962311,
133.827920012961));
#259237=CARTESIAN_POINT('Ctrl Pts',(-124.780763639097,-0.630693593994696,
137.379789228888));
#259238=CARTESIAN_POINT('Ctrl Pts',(-125.059211262909,5.19118902341993,
134.889160778557));
#259239=CARTESIAN_POINT('Ctrl Pts',(-125.337658886723,6.24262253199412,
128.644800533857));
#259240=CARTESIAN_POINT('Ctrl Pts',(-125.616106510535,1.55739090273089,
124.384970505708));
#259241=CARTESIAN_POINT('Ctrl Pts',(-125.894554134348,-4.55900688336737,
126.024246385717));
#259242=CARTESIAN_POINT('Ctrl Pts',(-126.173001758161,-6.48590006351826,
132.056213723232));
#259243=CARTESIAN_POINT('Ctrl Pts',(-126.451449381974,-2.45256793912933,
136.937789213063));
#259244=CARTESIAN_POINT('Ctrl Pts',(-126.729897005787,3.83455430671493,
136.183043458277));
#259245=CARTESIAN_POINT('Ctrl Pts',(-127.0083446296,6.5979084730801,130.485550936142));
#259246=CARTESIAN_POINT('Ctrl Pts',(-127.286792253413,3.29810707843306,
125.081028936517));
#259247=CARTESIAN_POINT('Ctrl Pts',(-127.565239877225,-3.03249359980603,
124.935969151478));
#259248=CARTESIAN_POINT('Ctrl Pts',(-127.843687501038,-6.57638080537151,
130.183674436914));
#259249=CARTESIAN_POINT('Ctrl Pts',(-128.122135124851,-4.07689532486387,
136.001760000162));
#259250=CARTESIAN_POINT('Ctrl Pts',(-128.400582748664,2.1690577917847,137.043689437881));
#259251=CARTESIAN_POINT('Ctrl Pts',(-128.679030372477,6.42175276214748,
132.351980497887));
#259252=CARTESIAN_POINT('Ctrl Pts',(-128.95747799629,4.77317066415926,126.238084493312));
#259253=CARTESIAN_POINT('Ctrl Pts',(-129.235925620103,-1.26172209184052,
124.320373171937));
#259254=CARTESIAN_POINT('Ctrl Pts',(-129.514373243916,-6.13715388399014,
128.361129552696));
#259255=CARTESIAN_POINT('Ctrl Pts',(-129.792820867728,-5.37284107338758,
134.647095923599));
#259256=CARTESIAN_POINT('Ctrl Pts',(-130.071268491542,0.328850205779251,
137.401776276312));
#259257=CARTESIAN_POINT('Ctrl Pts',(-130.349716115354,5.72834421106097,
134.093753940311));
#259258=CARTESIAN_POINT('Ctrl Pts',(-130.628163739167,5.86376973154965,
127.762939836503));
#259259=CARTESIAN_POINT('Ctrl Pts',(-130.90661136298,0.610677329821333,
124.227042848828));
#259260=CARTESIAN_POINT('Ctrl Pts',(-131.185058986793,-5.20359770476699,
126.735379570785));
#259261=CARTESIAN_POINT('Ctrl Pts',(-131.463506610606,-6.23602065855449,
132.982911093959));
#259262=CARTESIAN_POINT('Ctrl Pts',(-131.741954234419,-1.53784527367628,
137.228461157434));
#259263=CARTESIAN_POINT('Ctrl Pts',(-132.020401858232,4.57353478979242,
135.57057665953));
#259264=CARTESIAN_POINT('Ctrl Pts',(-132.298849482045,6.48205981103755,
129.532772461657));
#259265=CARTESIAN_POINT('Ctrl Pts',(-132.577297105858,2.43388853216508,
124.66349565853));
#259266=CARTESIAN_POINT('Ctrl Pts',(-132.85574472967,-3.85090740570176,
125.437373754826));
#259267=CARTESIAN_POINT('Ctrl Pts',(-133.134192353483,-6.59690756501448,
131.143250586095));
#259268=CARTESIAN_POINT('Ctrl Pts',(-133.412639977296,-3.28067194892964,
136.53770409198));
#259269=CARTESIAN_POINT('Ctrl Pts',(-133.691087601109,3.0503409184865,136.663495034279));
#259270=CARTESIAN_POINT('Ctrl Pts',(-133.969535224922,6.5782394992522,131.405027682246));
#259271=CARTESIAN_POINT('Ctrl Pts',(-134.247982848735,4.06105734507014,
125.59457664199));
#259272=CARTESIAN_POINT('Ctrl Pts',(-134.526430472548,-2.18803811555026,
124.57166256319));
#259273=CARTESIAN_POINT('Ctrl Pts',(-134.804878096361,-6.42643343958478,
129.276293512134));
#259274=CARTESIAN_POINT('Ctrl Pts',(-135.083325720174,-4.75925038136761,
135.385143480741));
#259275=CARTESIAN_POINT('Ctrl Pts',(-135.361773343986,1.28145127501926,
137.284477781773));
#259276=CARTESIAN_POINT('Ctrl Pts',(-135.640220967799,6.14456181203885,
133.228900980221));
#259277=CARTESIAN_POINT('Ctrl Pts',(-135.918668591612,5.36112022232688,
126.945290030769));
#259278=CARTESIAN_POINT('Ctrl Pts',(-136.197116215425,-0.348928946420584,
124.207976424505));
#259279=CARTESIAN_POINT('Ctrl Pts',(-136.475563839238,-5.73832945953392,
127.53241764038));
#259280=CARTESIAN_POINT('Ctrl Pts',(-136.754011463051,-5.85448553231475,
133.863614608987));
#259281=CARTESIAN_POINT('Ctrl Pts',(-137.032459086864,-0.590655408416443,
137.383506612345));
#259282=CARTESIAN_POINT('Ctrl Pts',(-137.310906710677,5.21595818069537,
134.857484855651));
#259283=CARTESIAN_POINT('Ctrl Pts',(-137.58935433449,6.22936101547165,128.606839930282));
#259284=CARTESIAN_POINT('Ctrl Pts',(-137.867801958302,1.51828539823306,
124.375609161675));
#259285=CARTESIAN_POINT('Ctrl Pts',(-138.146249582115,-4.58802032761614,
126.052086919061));
#259286=CARTESIAN_POINT('Ctrl Pts',(-138.424697205928,-6.47815950964009,
132.095672043897));
#259287=CARTESIAN_POINT('Ctrl Pts',(-138.703144829741,-2.41518657799051,
136.952605052004));
#259288=CARTESIAN_POINT('Ctrl Pts',(-138.981592453554,3.86722483040823,
136.159601783301));
#259289=CARTESIAN_POINT('Ctrl Pts',(-139.260040077367,6.59584554409815,
130.445393501362));
#259290=CARTESIAN_POINT('Ctrl Pts',(-139.53848770118,3.26320642772972,125.061058462695));
#259291=CARTESIAN_POINT('Ctrl Pts',(-139.816935324993,-3.06815997922566,
124.954537528447));
#259292=CARTESIAN_POINT('Ctrl Pts',(-140.095382948806,-6.58003725322031,
130.223718233352));
#259293=CARTESIAN_POINT('Ctrl Pts',(-140.373830572619,-4.04518174419624,
136.026480923393));
#259294=CARTESIAN_POINT('Ctrl Pts',(-140.652278196431,2.20699816962987,
137.030370167137));
#259295=CARTESIAN_POINT('Ctrl Pts',(-140.930725820244,6.43105458342049,
132.312860792301));
#259296=CARTESIAN_POINT('Ctrl Pts',(-141.209173444057,4.74528600953044,
126.209113451214));
#259297=CARTESIAN_POINT('Ctrl Pts',(-141.48762106787,-1.30116858700904,
124.328173765698));
#259298=CARTESIAN_POINT('Ctrl Pts',(-141.766068691683,-6.15191281770628,
128.398533417733));
#259299=CARTESIAN_POINT('Ctrl Pts',(-142.044516315496,-5.34934970658085,
134.679730735221));
#259300=CARTESIAN_POINT('Ctrl Pts',(-142.322963939309,0.369004454631186,
137.399652236939));
#259301=CARTESIAN_POINT('Ctrl Pts',(-142.601411563122,5.74826154890666,
134.058822938361));
#259302=CARTESIAN_POINT('Ctrl Pts',(-142.879859186934,5.84514709792562,
127.727301756295));
#259303=CARTESIAN_POINT('Ctrl Pts',(-143.158306810748,0.570628015260733,
124.223447345055));
#259304=CARTESIAN_POINT('Ctrl Pts',(-143.43675443456,-5.22827033670001,
126.767130735766));
#259305=CARTESIAN_POINT('Ctrl Pts',(-143.715202058373,-6.22264366443886,
133.020831158207));
#259306=CARTESIAN_POINT('Ctrl Pts',(-143.993649682186,-1.49871145760156,
137.237703434405));
#259307=CARTESIAN_POINT('Ctrl Pts',(-144.272097305999,4.60246336264661,
135.542647948195));
#259308=CARTESIAN_POINT('Ctrl Pts',(-144.550544929812,6.47419919545755,
129.493337883343));
#259309=CARTESIAN_POINT('Ctrl Pts',(-144.828992553625,2.39646224985712,
124.648793664219));
#259310=CARTESIAN_POINT('Ctrl Pts',(-145.107440177438,-3.8835064296727,
125.460914759058));
#259311=CARTESIAN_POINT('Ctrl Pts',(-145.38588780125,-6.59472242016944,
131.183401556022));
#259312=CARTESIAN_POINT('Ctrl Pts',(-145.664335425064,-3.24571067663155,
136.557568247724));
#259313=CARTESIAN_POINT('Ctrl Pts',(-145.942783048876,3.08595061694992,
136.644818187128));
#259314=CARTESIAN_POINT('Ctrl Pts',(-146.221230672689,6.58177405062243,
131.364972942318));
#259315=CARTESIAN_POINT('Ctrl Pts',(-146.499678296502,4.02926866931097,
125.569952358496));
#259316=CARTESIAN_POINT('Ctrl Pts',(-146.778125920315,-2.22593777837984,
124.585097249699));
#259317=CARTESIAN_POINT('Ctrl Pts',(-147.056573544128,-6.43561615084533,
129.315441348065));
#259318=CARTESIAN_POINT('Ctrl Pts',(-147.335021167941,-4.73127767801157,
135.414029517352));
#259319=CARTESIAN_POINT('Ctrl Pts',(-147.613468791753,1.32087384515067,
137.276557162581));
#259320=CARTESIAN_POINT('Ctrl Pts',(-147.891916415567,6.15920683289404,
133.191452367319));
#259321=CARTESIAN_POINT('Ctrl Pts',(-148.170364039379,5.33752963518947,
126.91272686995));
#259322=CARTESIAN_POINT('Ctrl Pts',(-148.448811663193,-0.389076544435395,
124.210222669761));
#259323=CARTESIAN_POINT('Ctrl Pts',(-148.727259287005,-5.75814038716998,
127.567409102056));
#259324=CARTESIAN_POINT('Ctrl Pts',(-149.005706910818,-5.83575451489182,
133.899195843233));
#259325=CARTESIAN_POINT('Ctrl Pts',(-149.284154534631,-0.550595335885521,
137.386980203127));
#259326=CARTESIAN_POINT('Ctrl Pts',(-149.562602158444,5.24053405872261,
134.825658742734));
#259327=CARTESIAN_POINT('Ctrl Pts',(-149.841049782257,6.21586866768539,
128.568960756646));
#259328=CARTESIAN_POINT('Ctrl Pts',(-150.119497406069,1.47912363311174,
124.366486037389));
#259329=CARTESIAN_POINT('Ctrl Pts',(-150.397945029883,-4.61686376108527,
126.080103549656));
#259330=CARTESIAN_POINT('Ctrl Pts',(-150.676392653695,-6.4701789051783,
132.135082514543));
#259331=CARTESIAN_POINT('Ctrl Pts',(-150.954840277509,-2.37771572122463,
136.967193065487));
#259332=CARTESIAN_POINT('Ctrl Pts',(-151.233287901321,3.89975205266408,
136.135961667893));
#259333=CARTESIAN_POINT('Ctrl Pts',(-151.511735525134,6.59353820363339,
130.405249368239));
#259334=CARTESIAN_POINT('Ctrl Pts',(-151.790183148947,3.22818485771248,
125.041300809049));
#259335=CARTESIAN_POINT('Ctrl Pts',(-152.06863077276,-3.10371266684865,
124.97332267276));
#259336=CARTESIAN_POINT('Ctrl Pts',(-152.347078396573,-6.58344987536885,
130.263783545709));
#259337=CARTESIAN_POINT('Ctrl Pts',(-152.625526020386,-4.01331826783166,
136.051008339035));
#259338=CARTESIAN_POINT('Ctrl Pts',(-152.903973644199,2.24485676634579,
137.016820189321));
#259339=CARTESIAN_POINT('Ctrl Pts',(-153.182421268012,6.44011809960154,
132.273685188686));
#259340=CARTESIAN_POINT('Ctrl Pts',(-153.460868891824,4.71722551658265,
126.180312687687));
#259341=CARTESIAN_POINT('Ctrl Pts',(-153.739316515637,-1.34056686689732,
124.336214336947));
#259342=CARTESIAN_POINT('Ctrl Pts',(-154.01776413945,-6.16644379003131,
128.436026431582));
#259343=CARTESIAN_POINT('Ctrl Pts',(-154.296211763263,-5.32566011765276,
134.712221943579));
#259344=CARTESIAN_POINT('Ctrl Pts',(-154.574659387076,0.409145029887599,
137.397283806609));
#259345=CARTESIAN_POINT('Ctrl Pts',(-154.853107010889,5.7679658828075,134.023771341112));
#259346=CARTESIAN_POINT('Ctrl Pts',(-155.131554634702,5.82630787022557,
127.691777697632));
#259347=CARTESIAN_POINT('Ctrl Pts',(-155.410002258515,0.530557555869813,
124.220095699443));
#259348=CARTESIAN_POINT('Ctrl Pts',(-155.688449882327,-5.25274923315307,
126.799031501784));
#259349=CARTESIAN_POINT('Ctrl Pts',(-155.96689750614,-6.20903608797397,
133.058669090323));
#259350=CARTESIAN_POINT('Ctrl Pts',(-156.245345129953,-1.4595221062231,
137.246707321489));
#259351=CARTESIAN_POINT('Ctrl Pts',(-156.523792753766,4.63122138952822,
135.514543657883));
#259352=CARTESIAN_POINT('Ctrl Pts',(-156.802240377579,6.46609867604585,
129.453951885458));
#259353=CARTESIAN_POINT('Ctrl Pts',(-157.080688001392,2.35894716575843,
124.634319766706));
#259354=CARTESIAN_POINT('Ctrl Pts',(-157.359135625205,-3.9159615488849,
125.484653766641));
#259355=CARTESIAN_POINT('Ctrl Pts',(-157.637583249018,-6.59229290546042,
131.223538480449));
#259356=CARTESIAN_POINT('Ctrl Pts',(-157.916030872831,-3.21062913332988,
136.577219216243));
#259357=CARTESIAN_POINT('Ctrl Pts',(-158.194478496644,3.12144596437753,
136.625924919674));
#259358=CARTESIAN_POINT('Ctrl Pts',(-158.472926120456,6.58506471193526,
131.324897428694));
#259359=CARTESIAN_POINT('Ctrl Pts',(-158.751373744269,3.99733068751967,
125.545522037924));
#259360=CARTESIAN_POINT('Ctrl Pts',(-159.029821368082,-2.26375495826568,
124.598762393297));
#259361=CARTESIAN_POINT('Ctrl Pts',(-159.308268991895,-6.44456038798308,
129.354644356446));
#259362=CARTESIAN_POINT('Ctrl Pts',(-159.586716615708,-4.7031296554214,
135.442744740987));
#259363=CARTESIAN_POINT('Ctrl Pts',(-159.865164239521,1.36024746981527,
137.268396713766));
#259364=CARTESIAN_POINT('Ctrl Pts',(-160.143611863334,6.17362362207528,
133.153915299856));
#259365=CARTESIAN_POINT('Ctrl Pts',(-160.422059487147,5.31374126392856,
126.880307915048));
#259366=CARTESIAN_POINT('Ctrl Pts',(-160.70050711096,-0.429209725076344,
124.212713263223));
#259367=CARTESIAN_POINT('Ctrl Pts',(-160.978954734773,-5.77773794479658,
127.602520510164));
#259368=CARTESIAN_POINT('Ctrl Pts',(-161.257402358585,-5.81680725143943,
133.934662397221));
#259369=CARTESIAN_POINT('Ctrl Pts',(-161.535849982398,-0.51051486084124,
137.390209872519));
#259370=CARTESIAN_POINT('Ctrl Pts',(-161.814297606211,5.26491574683228,
134.793683619137));
#259371=CARTESIAN_POINT('Ctrl Pts',(-162.092745230024,6.20214598860049,
128.531164416574));
#259372=CARTESIAN_POINT('Ctrl Pts',(-162.371192853837,1.43990705852047,
124.357601470914));
#259373=CARTESIAN_POINT('Ctrl Pts',(-162.64964047765,-4.64553611496906,
126.108295239334));
#259374=CARTESIAN_POINT('Ctrl Pts',(-162.928088101462,-6.46195854585841,
132.1744436748));
#259375=CARTESIAN_POINT('Ctrl Pts',(-163.206535725276,-2.34015675732853,
136.981552712947));
#259376=CARTESIAN_POINT('Ctrl Pts',(-163.484983349088,3.93213476817268,
136.112123988049));
#259377=CARTESIAN_POINT('Ctrl Pts',(-163.763430972902,6.5909865371863,130.365120024332));
#259378=CARTESIAN_POINT('Ctrl Pts',(-164.041878596714,3.19304366611785,
125.021756707701));
#259379=CARTESIAN_POINT('Ctrl Pts',(-164.320326220527,-3.13915034525769,
124.99232388833));
#259380=CARTESIAN_POINT('Ctrl Pts',(-164.59877384434,-6.58661854536123,
130.303868889347));
#259381=CARTESIAN_POINT('Ctrl Pts',(-164.877221468153,-3.98130607648258,
136.075341338217));
#259382=CARTESIAN_POINT('Ctrl Pts',(-165.155669091966,2.28263217906914,
137.003040006531));
#259383=CARTESIAN_POINT('Ctrl Pts',(-165.434116715779,6.44894297483741,
132.23445513871));
#259384=CARTESIAN_POINT('Ctrl Pts',(-165.712564339591,4.6889902251094,126.151683269957));
#259385=CARTESIAN_POINT('Ctrl Pts',(-165.991011963405,-1.37991547158711,
124.344494587733));
#259386=CARTESIAN_POINT('Ctrl Pts',(-166.269459587217,-6.18074626251326,
128.473607204924));
#259387=CARTESIAN_POINT('Ctrl Pts',(-166.54790721103,-5.3017731844313,134.744568344699));
#259388=CARTESIAN_POINT('Ctrl Pts',(-166.826354834843,0.449270444124704,
137.394671073086));
#259389=CARTESIAN_POINT('Ctrl Pts',(-167.104802458656,5.78745648261092,
133.988600447415));
#259390=CARTESIAN_POINT('Ctrl Pts',(-167.383250082469,5.8072527465451,127.656368976875));
#259391=CARTESIAN_POINT('Ctrl Pts',(-167.661697706282,0.490467436472931,
124.216988036188));
#259392=CARTESIAN_POINT('Ctrl Pts',(-167.940145330095,-5.27703348705155,
126.831080686747));
#259393=CARTESIAN_POINT('Ctrl Pts',(-168.218592953908,-6.19519843339338,
133.096423488211));
#259394=CARTESIAN_POINT('Ctrl Pts',(-168.49704057772,-1.42027867171577,
137.255472485049));
#259395=CARTESIAN_POINT('Ctrl Pts',(-168.775488201534,4.65980780479824,
135.486264830004));
#259396=CARTESIAN_POINT('Ctrl Pts',(-169.053935825346,6.45775855296945,
129.414615927465));
#259397=CARTESIAN_POINT('Ctrl Pts',(-169.332383449159,2.32134467000579,
124.620074502325));
#259398=CARTESIAN_POINT('Ctrl Pts',(-169.610831072972,-3.94827156070164,
125.508589897919));
#259399=CARTESIAN_POINT('Ctrl Pts',(-169.889278696785,-6.58961911091297,
131.263659872085));
#259400=CARTESIAN_POINT('Ctrl Pts',(-170.167726320598,-3.17542861898582,
136.596656269364));
#259401=CARTESIAN_POINT('Ctrl Pts',(-170.446173944411,3.15682564547787,
136.606815932013));
#259402=CARTESIAN_POINT('Ctrl Pts',(-170.724621568223,6.58811136125304,
131.284802626386));
#259403=CARTESIAN_POINT('Ctrl Pts',(-171.003069192037,3.96524458316956,
125.521286585549));
#259404=CARTESIAN_POINT('Ctrl Pts',(-171.28151681585,-2.30148825387982,
124.612657487621));
#259405=CARTESIAN_POINT('Ctrl Pts',(-171.559964439662,-6.45326581956532,
129.393901084596));
#259406=CARTESIAN_POINT('Ctrl Pts',(-171.838412063475,-4.67480735663214,
135.471288087592));
#259407=CARTESIAN_POINT('Ctrl Pts',(-172.116859687288,1.39957069001038,
137.259996737715));
#259408=CARTESIAN_POINT('Ctrl Pts',(-172.395307311101,6.18781164536257,
133.116291168777));
#259409=CARTESIAN_POINT('Ctrl Pts',(-172.673754934914,5.289755990031,126.848034367363));
#259410=CARTESIAN_POINT('Ctrl Pts',(-172.952202558727,-0.469327001192524,
124.215448112602));
#259411=CARTESIAN_POINT('Ctrl Pts',(-173.23065018254,-5.79712140621875,
127.637750563632));
#259412=CARTESIAN_POINT('Ctrl Pts',(-173.509097806352,-5.79764444405506,
133.970012956726));
#259413=CARTESIAN_POINT('Ctrl Pts',(-173.787545430165,-0.470415468481743,
137.393195500846));
#259414=CARTESIAN_POINT('Ctrl Pts',(-174.065993053978,5.28910234155359,
134.76156066971));
#259415=CARTESIAN_POINT('Ctrl Pts',(-174.344440677791,6.18819348671444,
128.493452310623));
#259416=CARTESIAN_POINT('Ctrl Pts',(-174.622888301604,1.40063712764339,
124.34895579147));
#259417=CARTESIAN_POINT('Ctrl Pts',(-174.901335925417,-4.67403632680454,
126.13666094344));
#259418=CARTESIAN_POINT('Ctrl Pts',(-175.17978354923,-6.45349873628761,
132.213754066126));
#259419=CARTESIAN_POINT('Ctrl Pts',(-175.458231173043,-2.30251107806296,
136.995683462282));
#259420=CARTESIAN_POINT('Ctrl Pts',(-175.736678796856,3.96437177698222,
136.088089627079));
#259421=CARTESIAN_POINT('Ctrl Pts',(-176.015126420669,6.58819063930867,
130.325006956645));
#259422=CARTESIAN_POINT('Ctrl Pts',(-176.293574044481,3.15778415511627,
125.002426882869));
#259423=CARTESIAN_POINT('Ctrl Pts',(-176.572021668294,-3.17447170129595,
125.011540471058));
#259424=CARTESIAN_POINT('Ctrl Pts',(-176.850469292107,-6.58954314578118,
130.343972778891));
#259425=CARTESIAN_POINT('Ctrl Pts',(-177.12891691592,-3.94914635637289,
136.099479019269));
#259426=CARTESIAN_POINT('Ctrl Pts',(-177.407364539733,2.32032300801719,
136.989030129397));
#259427=CARTESIAN_POINT('Ctrl Pts',(-177.685812163546,6.45752888212044,
132.195172096054));
#259428=CARTESIAN_POINT('Ctrl Pts',(-177.964259787359,4.66058118137817,
126.123226258898));
#259429=CARTESIAN_POINT('Ctrl Pts',(-178.242707411172,-1.41921294300185,
124.353014211231));
#259430=CARTESIAN_POINT('Ctrl Pts',(-178.521155034985,-6.19481970517025,
128.511274345191));
#259431=CARTESIAN_POINT('Ctrl Pts',(-178.799602658797,-5.27768979205393,
134.776768739972));
#259432=CARTESIAN_POINT('Ctrl Pts',(-179.078050282611,0.489379210479558,
137.391814133187));
#259433=CARTESIAN_POINT('Ctrl Pts',(-179.356497906423,5.80673262608622,
133.95331156054));
#259434=CARTESIAN_POINT('Ctrl Pts',(-179.634945530236,5.7879824329786,127.621076906106));
#259435=CARTESIAN_POINT('Ctrl Pts',(-179.913393154049,0.450359142625426,
124.214124470449));
#259436=CARTESIAN_POINT('Ctrl Pts',(-180.191840777862,-5.30112219853358,
126.863277103057));
#259437=CARTESIAN_POINT('Ctrl Pts',(-180.470288401675,-6.18113121345664,
133.134092952866));
#259438=CARTESIAN_POINT('Ctrl Pts',(-180.748736025488,-1.38098260826046,
137.263998600285));
#259439=CARTESIAN_POINT('Ctrl Pts',(-181.0271836493,4.68822154917632,135.457812512445));
#259440=CARTESIAN_POINT('Ctrl Pts',(-181.305631273113,6.44917913527537,
129.375331466973));
#259441=CARTESIAN_POINT('Ctrl Pts',(-181.584078896926,2.28365615597197,
124.606058398942));
#259442=CARTESIAN_POINT('Ctrl Pts',(-181.862526520739,-3.98043526786393,
125.532722265928));
#259443=CARTESIAN_POINT('Ctrl Pts',(-182.140974144552,-6.58670113560653,
131.303764244219));
#259444=CARTESIAN_POINT('Ctrl Pts',(-182.419421768365,-3.14011043796568,
136.615878686839));
#259445=CARTESIAN_POINT('Ctrl Pts',(-182.697869392178,3.19208834924215,
136.587491932238));
#259446=CARTESIAN_POINT('Ctrl Pts',(-182.976317015991,6.59091388568205,
131.244690021124));
#259447=CARTESIAN_POINT('Ctrl Pts',(-183.254764639804,3.93301154522339,
125.497246899427));
#259448=CARTESIAN_POINT('Ctrl Pts',(-183.533212263617,-2.33913626699958,
124.626782017781));
#259449=CARTESIAN_POINT('Ctrl Pts',(-183.811659887429,-6.46173212300977,
129.433210077844));
#259450=CARTESIAN_POINT('Ctrl Pts',(-184.090107511242,-4.64631183113728,
135.499658499484));
#259451=CARTESIAN_POINT('Ctrl Pts',(-184.368555135055,1.43884204859816,
137.251357545694));
#259452=CARTESIAN_POINT('Ctrl Pts',(-184.647002758868,6.20177037701405,
133.078581368264));
#259453=CARTESIAN_POINT('Ctrl Pts',(-184.925450382681,5.26557470227994,
126.815907422802));
#259454=CARTESIAN_POINT('Ctrl Pts',(-185.203898006494,-0.50942688622466,
124.218427116558));
#259455=CARTESIAN_POINT('Ctrl Pts',(-185.482345630307,-5.81629005317544,
127.673097957001));
#259456=CARTESIAN_POINT('Ctrl Pts',(-185.76079325412,-5.77826680282389,
134.005246211819));
#259457=CARTESIAN_POINT('Ctrl Pts',(-186.039240877932,-0.430298644703365,
137.395936977472));
#259458=CARTESIAN_POINT('Ctrl Pts',(-186.317688501746,5.31309294664177,
134.729291084778));
#259459=CARTESIAN_POINT('Ctrl Pts',(-186.596136125558,6.17401167904375,
128.455825836229));
#259460=CARTESIAN_POINT('Ctrl Pts',(-186.874583749371,1.36131529564269,
124.340549319425));
#259461=CARTESIAN_POINT('Ctrl Pts',(-187.153031373184,-4.70236334050424,
126.165199610876));
#259462=CARTESIAN_POINT('Ctrl Pts',(-187.431478996997,-6.44479978994851,
132.253012231859));
#259463=CARTESIAN_POINT('Ctrl Pts',(-187.70992662081,-2.26478007840253,
137.009584789872));
#259464=CARTESIAN_POINT('Ctrl Pts',(-187.988374244623,3.99646188453734,
136.063859475589));
#259465=CARTESIAN_POINT('Ctrl Pts',(-188.266821868436,6.58515061360439,
130.284911651585));
#259466=CARTESIAN_POINT('Ctrl Pts',(-188.545269492249,3.12240763126122,
124.983312050825));
#259467=CARTESIAN_POINT('Ctrl Pts',(-188.823717116061,-3.20967542611822,
125.030971708867));
#259468=CARTESIAN_POINT('Ctrl Pts',(-189.102164739874,-6.59222356825658,
130.384093728275));
#259469=CARTESIAN_POINT('Ctrl Pts',(-189.380612363687,-3.91684029919248,
136.123420487763));
#259470=CARTESIAN_POINT('Ctrl Pts',(-189.6590599875,2.35792785654334,136.974791077059));
#259471=CARTESIAN_POINT('Ctrl Pts',(-189.937507611313,6.46587550329532,
132.155837516369));
#259472=CARTESIAN_POINT('Ctrl Pts',(-190.215955235126,4.63199943809816,
126.094942708994));
#259473=CARTESIAN_POINT('Ctrl Pts',(-190.494402858939,-1.45845782495887,
124.361772891742));
#259474=CARTESIAN_POINT('Ctrl Pts',(-190.772850482752,-6.2086635965042,
128.549026456613));
#259475=CARTESIAN_POINT('Ctrl Pts',(-191.051298106565,-5.25341083294129,
134.808821936201));
#259476=CARTESIAN_POINT('Ctrl Pts',(-191.329745730377,0.529469842708527,
137.388713092773));
#259477=CARTESIAN_POINT('Ctrl Pts',(-191.60819335419,5.82579359894846,133.91790598813));
#259478=CARTESIAN_POINT('Ctrl Pts',(-191.886640978003,5.76849764359442,
127.585902793086));
#259479=CARTESIAN_POINT('Ctrl Pts',(-192.165088601816,0.410234160553658,
124.211505108333));
#259480=CARTESIAN_POINT('Ctrl Pts',(-192.443536225629,-5.32501447498302,
126.895619557667));
#259481=CARTESIAN_POINT('Ctrl Pts',(-192.721983849442,-6.16683494942961,
133.171676088433));
#259482=CARTESIAN_POINT('Ctrl Pts',(-193.000431473255,-1.34163537198624,
137.272285351261));
#259483=CARTESIAN_POINT('Ctrl Pts',(-193.278879097068,4.71646156978089,
135.429187759513));
#259484=CARTESIAN_POINT('Ctrl Pts',(-193.557326720881,6.44036074087642,
129.336099959682));
#259485=CARTESIAN_POINT('Ctrl Pts',(-193.835774344694,2.24588302022023,
124.592271975924));
#259486=CARTESIAN_POINT('Ctrl Pts',(-194.114221968506,-4.01245147853337,
125.557049976435));
#259487=CARTESIAN_POINT('Ctrl Pts',(-194.392669592319,-6.58353908766677,
131.343850110767));
#259488=CARTESIAN_POINT('Ctrl Pts',(-194.671117216133,-3.10467589899933,
136.634885756375));
#259489=CARTESIAN_POINT('Ctrl Pts',(-194.949564839945,3.22723276899961,
136.567953636405));
#259490=CARTESIAN_POINT('Ctrl Pts',(-195.228012463758,6.59347218137276,
131.204561099293));
#259491=CARTESIAN_POINT('Ctrl Pts',(-195.506460087571,3.90063276808784,
125.473403870355));
#259492=CARTESIAN_POINT('Ctrl Pts',(-195.784907711384,-2.3766976025655,
124.641135460387));
#259493=CARTESIAN_POINT('Ctrl Pts',(-196.063355335197,-6.46995898459376,
129.472569879579));
#259494=CARTESIAN_POINT('Ctrl Pts',(-196.34180295901,-4.61764413484867,
135.527854925386));
#259495=CARTESIAN_POINT('Ctrl Pts',(-196.620250582823,1.47806009036541,
137.242479457832));
#259496=CARTESIAN_POINT('Ctrl Pts',(-196.898698206635,6.21549929978325,
133.040787295662));
#259497=CARTESIAN_POINT('Ctrl Pts',(-197.177145830448,5.24119829672186,
126.783928271841));
#259498=CARTESIAN_POINT('Ctrl Pts',(-197.455593454261,-0.5495078942556,
124.2216501647));
#259499=CARTESIAN_POINT('Ctrl Pts',(-197.734041078074,-5.83524317536515,
127.708561380459));
#259500=CARTESIAN_POINT('Ctrl Pts',(-198.012488701887,-5.75867504579123,
134.040360856918));
#259501=CARTESIAN_POINT('Ctrl Pts',(-198.2909363257,-0.390165876051177,
137.398434200813));
#259502=CARTESIAN_POINT('Ctrl Pts',(-198.569383949513,5.33688667311775,
134.696876060105));
#259503=CARTESIAN_POINT('Ctrl Pts',(-198.847831573325,6.15960109109908,
128.418286387655));
#259504=CARTESIAN_POINT('Ctrl Pts',(-199.126279197139,1.32194301960288,
124.332382366286));
#259505=CARTESIAN_POINT('Ctrl Pts',(-199.404726820951,-4.73051610640191,
126.193910184127));
#259506=CARTESIAN_POINT('Ctrl Pts',(-199.683174444764,-6.43586202918244,
132.292216717274));
#259507=CARTESIAN_POINT('Ctrl Pts',(-199.961622068577,-2.22696515648391,
137.023256180599));
#259508=CARTESIAN_POINT('Ctrl Pts',(-200.24006969239,4.02840390172748,136.039434431435));
#259509=CARTESIAN_POINT('Ctrl Pts',(-200.518517316203,6.58186657272242,
130.244835594899));
#259510=CARTESIAN_POINT('Ctrl Pts',(-200.796964940016,3.08691540544346,
124.964412919876));
#259511=CARTESIAN_POINT('Ctrl Pts',(-201.075412563829,-3.24476021523692,
125.050616881724));
#259512=CARTESIAN_POINT('Ctrl Pts',(-201.353860187642,-6.59465971346335,
130.424230250803));
#259513=CARTESIAN_POINT('Ctrl Pts',(-201.632307811455,-3.88438910205457,
136.147164856536));
#259514=CARTESIAN_POINT('Ctrl Pts',(-201.910755435267,2.39544533118521,
136.960323377152));
#259515=CARTESIAN_POINT('Ctrl Pts',(-202.18920305908,6.47398252907625,132.116452857208));
#259516=CARTESIAN_POINT('Ctrl Pts',(-202.467650682893,4.60324605437475,
126.066833668302));
#259517=CARTESIAN_POINT('Ctrl Pts',(-202.746098306706,-1.49764866322506,
124.370770304711));
#259518=CARTESIAN_POINT('Ctrl Pts',(-203.024545930519,-6.22227742352606,
128.586862140274));
#259519=CARTESIAN_POINT('Ctrl Pts',(-203.302993554332,-5.22893720675747,
134.840726745644));
#259520=CARTESIAN_POINT('Ctrl Pts',(-203.581441178145,0.569540855237039,
137.385368066758));
#259521=CARTESIAN_POINT('Ctrl Pts',(-203.859888801958,5.84463869488665,
133.882385042152));
#259522=CARTESIAN_POINT('Ctrl Pts',(-204.138336425771,5.7487991004088,127.550847941203));
#259523=CARTESIAN_POINT('Ctrl Pts',(-204.416784049583,0.370093977104817,
124.209130046901));
#259524=CARTESIAN_POINT('Ctrl Pts',(-204.695231673396,-5.34870943106288,
126.928106852114));
#259525=CARTESIAN_POINT('Ctrl Pts',(-204.973679297209,-6.15231017106575,
133.209171502253));
#259526=CARTESIAN_POINT('Ctrl Pts',(-205.252126921022,-1.30223842092043,
137.280332430907));
#259527=CARTESIAN_POINT('Ctrl Pts',(-205.530574544835,4.74452682016742,
135.400391631911));
#259528=CARTESIAN_POINT('Ctrl Pts',(-205.809022168648,6.43130369654214,
129.296922859329));
#259529=CARTESIAN_POINT('Ctrl Pts',(-206.087469792461,2.20802666244648,
124.578715744137));
#259530=CARTESIAN_POINT('Ctrl Pts',(-206.365917416273,-4.04431900633787,
125.581572127967));
#259531=CARTESIAN_POINT('Ctrl Pts',(-206.644365040087,-6.58013308426553,
131.383915986335));
#259532=CARTESIAN_POINT('Ctrl Pts',(-206.922812663899,-3.06912631512495,
136.653676773657));
#259533=CARTESIAN_POINT('Ctrl Pts',(-207.201260287713,3.26225760245914,
136.548201768512));
#259534=CARTESIAN_POINT('Ctrl Pts',(-207.479707911525,6.59578615352751,
131.164417347887));
#259535=CARTESIAN_POINT('Ctrl Pts',(-207.758155535338,3.86810945157081,
125.449758381845));
#259536=CARTESIAN_POINT('Ctrl Pts',(-208.036603159151,-2.41417086872696,
124.655717283569));
#259537=CARTESIAN_POINT('Ctrl Pts',(-208.315050782964,-6.47794609946865,
129.511979031309));
#259538=CARTESIAN_POINT('Ctrl Pts',(-208.593498406777,-4.58880533005852,
135.555876320469));
#259539=CARTESIAN_POINT('Ctrl Pts',(-208.87194603059,1.51722336207232,137.233362803106));
#259540=CARTESIAN_POINT('Ctrl Pts',(-209.150393654402,6.22899790494034,
133.00291035145));
#259541=CARTESIAN_POINT('Ctrl Pts',(-209.428841278216,5.21662767663345,
126.752098099478));
#259542=CARTESIAN_POINT('Ctrl Pts',(-209.707288902028,-0.589568540070009,
124.225117137599));
#259543=CARTESIAN_POINT('Ctrl Pts',(-209.985736525842,-5.85398007047323,
127.744139519898));
#259544=CARTESIAN_POINT('Ctrl Pts',(-210.264184149654,-5.73886989893714,
134.07535559084));
#259545=CARTESIAN_POINT('Ctrl Pts',(-210.542631773467,-0.350018649658268,
137.400687078332));
#259546=CARTESIAN_POINT('Ctrl Pts',(-210.82107939728,5.36048263929459,134.664316796842));
#259547=CARTESIAN_POINT('Ctrl Pts',(-211.099527021093,6.14496225687153,
128.38083535594));
#259548=CARTESIAN_POINT('Ctrl Pts',(-211.377974644906,1.28252175847855,
124.324455234681));
#259549=CARTESIAN_POINT('Ctrl Pts',(-211.656422268719,-4.75849358128477,
126.222791599316));
#259550=CARTESIAN_POINT('Ctrl Pts',(-211.934869892531,-6.4266857851828,
132.331366069634));
#259551=CARTESIAN_POINT('Ctrl Pts',(-212.213317516344,-2.18906771355195,
137.036697127864));
#259552=CARTESIAN_POINT('Ctrl Pts',(-212.491765140157,4.06019664492976,
136.014815399695));
#259553=CARTESIAN_POINT('Ctrl Pts',(-212.770212763971,6.57833863835413,
130.204780271616));
#259554=CARTESIAN_POINT('Ctrl Pts',(-213.048660387783,3.05130879283982,
124.945730190337));
#259555=CARTESIAN_POINT('Ctrl Pts',(-213.327108011596,-3.27972476857289,
125.070475261673));
#259556=CARTESIAN_POINT('Ctrl Pts',(-213.605555635409,-6.59685149112928,
130.464380859201));
#259557=CARTESIAN_POINT('Ctrl Pts',(-213.884003259222,-3.85179396744981,
136.170711245733));
#259558=CARTESIAN_POINT('Ctrl Pts',(-214.162450883035,2.43287404171984,
136.94562756578));
#259559=CARTESIAN_POINT('Ctrl Pts',(-214.440898506847,6.48184965905313,
132.077019577989));
#259560=CARTESIAN_POINT('Ctrl Pts',(-214.71934613066,4.57432209567675,126.038900178414));
#259561=CARTESIAN_POINT('Ctrl Pts',(-214.997793754473,-1.53678400556905,
124.380006116735));
#259562=CARTESIAN_POINT('Ctrl Pts',(-215.276241378286,-6.23566068176903,
128.624779994154));
#259563=CARTESIAN_POINT('Ctrl Pts',(-215.554689002099,-5.20426982038336,
134.872481986055));
#259564=CARTESIAN_POINT('Ctrl Pts',(-215.833136625912,0.609590763220439,
137.381779179092));
#259565=CARTESIAN_POINT('Ctrl Pts',(-216.111584249725,5.86326721558844,
133.846750038845));
#259566=CARTESIAN_POINT('Ctrl Pts',(-216.390031873537,5.72888753335829,
127.51591364943));
#259567=CARTESIAN_POINT('Ctrl Pts',(-216.668479497351,0.329940079686948,
124.206999374164));
#259568=CARTESIAN_POINT('Ctrl Pts',(-216.946927121163,-5.37220618874772,
126.960737782571));
#259569=CARTESIAN_POINT('Ctrl Pts',(-217.225374744977,-6.13755741658593,
133.246577804923));
#259570=CARTESIAN_POINT('Ctrl Pts',(-217.503822368789,-1.26279321493052,
137.288139541036));
#259571=CARTESIAN_POINT('Ctrl Pts',(-217.782269992602,4.77241626036792,
135.37142519669));
#259572=CARTESIAN_POINT('Ctrl Pts',(-218.060717616415,6.4220083378839,129.257801617636));
#259573=CARTESIAN_POINT('Ctrl Pts',(-218.339165240228,2.17008848543354,
124.565390205911));
#259574=CARTESIAN_POINT('Ctrl Pts',(-218.617612864041,-4.07603667041411,
125.606287811847));
#259575=CARTESIAN_POINT('Ctrl Pts',(-218.896060487854,-6.57648325161253,
131.423960386264));
#259576=CARTESIAN_POINT('Ctrl Pts',(-219.174508111666,-3.03346300364714,
136.672251042379));
#259577=CARTESIAN_POINT('Ctrl Pts',(-219.45295573548,3.29716155176439,136.528237060474));
#259578=CARTESIAN_POINT('Ctrl Pts',(-219.731403359293,6.59785571640026,
131.124260254445));
#259579=CARTESIAN_POINT('Ctrl Pts',(-220.009850983105,3.83544280083539,
125.426311310091));
#259580=CARTESIAN_POINT('Ctrl Pts',(-220.288298606918,-2.45155467689987,
124.67052694699));
#259581=CARTESIAN_POINT('Ctrl Pts',(-220.566746230731,-6.48569317166813,
129.551436072715));
#259582=CARTESIAN_POINT('Ctrl Pts',(-220.845193854544,-4.55979648539947,
135.58372164639));
#259583=CARTESIAN_POINT('Ctrl Pts',(-221.123641478357,1.55633041250914,
137.224007919343));
#259584=CARTESIAN_POINT('Ctrl Pts',(-221.40208910217,6.24226569228925,132.964951939167));
#259585=CARTESIAN_POINT('Ctrl Pts',(-221.680536725983,5.19186375248807,
126.720418085194));
#259586=CARTESIAN_POINT('Ctrl Pts',(-221.958984349796,-0.629607339204784,
124.228827906785));
#259587=CARTESIAN_POINT('Ctrl Pts',(-222.237431973609,-5.87250004419688,
127.779831056953));
#259588=CARTESIAN_POINT('Ctrl Pts',(-222.515879597421,-5.71885209614835,
134.110229116839));
#259589=CARTESIAN_POINT('Ctrl Pts',(-222.794327221234,-0.309858453196267,
137.402695526548));
#259590=CARTESIAN_POINT('Ctrl Pts',(-223.072774845047,5.38387997081673,
134.631614501482));
#259591=CARTESIAN_POINT('Ctrl Pts',(-223.35122246886,6.13009571880702,128.343474128844));
#259592=CARTESIAN_POINT('Ctrl Pts',(-223.629670092673,1.24305297303857,
124.316768218352));
#259593=CARTESIAN_POINT('Ctrl Pts',(-223.908117716486,-4.78629472843886,
126.25184278623));
#259594=CARTESIAN_POINT('Ctrl Pts',(-224.186565340298,-6.41727139797729,
132.370458838244));
#259595=CARTESIAN_POINT('Ctrl Pts',(-224.465012964112,-2.15108915391133,
137.049907133607));
#259596=CARTESIAN_POINT('Ctrl Pts',(-224.743460587925,4.09183893605206,
135.990003292637));
#259597=CARTESIAN_POINT('Ctrl Pts',(-225.021908211737,6.57456694122844,
130.164747166004));
#259598=CARTESIAN_POINT('Ctrl Pts',(-225.300355835551,3.01558911286705,
124.927264554503));
#259599=CARTESIAN_POINT('Ctrl Pts',(-225.578803459363,-3.31456779050113,
125.090546112851));
#259600=CARTESIAN_POINT('Ctrl Pts',(-225.857251083176,-6.5987988200372,
130.504544065675));
#259601=CARTESIAN_POINT('Ctrl Pts',(-226.135698706989,-3.8190561032033,
136.194058782834));
#259602=CARTESIAN_POINT('Ctrl Pts',(-226.414146330802,2.47021260121173,
136.930704187504));
#259603=CARTESIAN_POINT('Ctrl Pts',(-226.692593954615,6.48947660170784,
132.037539139922));
#259604=CARTESIAN_POINT('Ctrl Pts',(-226.971041578427,4.54522863379049,
126.011143274415));
#259605=CARTESIAN_POINT('Ctrl Pts',(-227.24948920224,-1.57586240181677,
124.389479985577));
#259606=CARTESIAN_POINT('Ctrl Pts',(-227.527936826054,-6.24881287531301,
128.662778613197));
#259607=CARTESIAN_POINT('Ctrl Pts',(-227.806384449866,-5.17940958787633,
134.904086480733));
#259608=CARTESIAN_POINT('Ctrl Pts',(-228.084832073679,0.649618082593193,
137.377946562762));
#259609=CARTESIAN_POINT('Ctrl Pts',(-228.363279697492,5.88167847076755,
133.811002298682));
#259610=CARTESIAN_POINT('Ctrl Pts',(-228.641727321305,5.70876368027354,
127.481101212267));
#259611=CARTESIAN_POINT('Ctrl Pts',(-228.920174945118,0.289773956218704,
124.205113169075));
#259612=CARTESIAN_POINT('Ctrl Pts',(-229.198622568931,-5.39550387735667,
126.993511139885));
#259613=CARTESIAN_POINT('Ctrl Pts',(-229.477070192744,-6.12257723265909,
133.283893610337));
#259614=CARTESIAN_POINT('Ctrl Pts',(-229.755517816557,-1.22330121567356,
137.295706392352));
#259615=CARTESIAN_POINT('Ctrl Pts',(-230.033965440369,4.80012885692891,
135.34228952721));
#259616=CARTESIAN_POINT('Ctrl Pts',(-230.312413064183,6.41247500934538,
129.218737684256));
#259617=CARTESIAN_POINT('Ctrl Pts',(-230.590860687995,2.13206989499296,
124.552295855027));
#259618=CARTESIAN_POINT('Ctrl Pts',(-230.869308311808,-4.10760329545278,
125.631196112227));
#259619=CARTESIAN_POINT('Ctrl Pts',(-231.147755935621,-6.5725897249546,
131.463981826697));
#259620=CARTESIAN_POINT('Ctrl Pts',(-231.426203559434,-2.99768728608136,
136.690607874263));
#259621=CARTESIAN_POINT('Ctrl Pts',(-231.704651183247,3.33194332353496,
136.508060252089));
#259622=CARTESIAN_POINT('Ctrl Pts',(-231.98309880706,6.59968079330357,131.084091307006));
#259623=CARTESIAN_POINT('Ctrl Pts',(-232.261546430872,3.80263402635669,
125.403063523931));
#259624=CARTESIAN_POINT('Ctrl Pts',(-232.539994054686,-2.48884764181187,
124.685563901874));
#259625=CARTESIAN_POINT('Ctrl Pts',(-232.818441678498,-6.49319991412244,
129.5909395417));
#259626=CARTESIAN_POINT('Ctrl Pts',(-233.096889302311,-4.53061867580467,
135.611389871331));
#259627=CARTESIAN_POINT('Ctrl Pts',(-233.375336926124,1.59537979255065,
137.214415153187));
#259628=CARTESIAN_POINT('Ctrl Pts',(-233.653784549937,6.25530217018742,
132.926913465378));
#259629=CARTESIAN_POINT('Ctrl Pts',(-233.93223217375,5.16690744192206,126.688889402902));
#259630=CARTESIAN_POINT('Ctrl Pts',(-234.210679797563,-0.669622808008655,
124.232782334755));
#259631=CARTESIAN_POINT('Ctrl Pts',(-234.489127421376,-5.89080241027189,
127.815634669064));
#259632=CARTESIAN_POINT('Ctrl Pts',(-234.767575045188,-5.69862237919218,
134.144980142666));
#259633=CARTESIAN_POINT('Ctrl Pts',(-235.046022669002,-0.269686774814632,
137.404459471037));
#259634=CARTESIAN_POINT('Ctrl Pts',(-235.324470292814,5.40707780068583,
134.598770385822));
#259635=CARTESIAN_POINT('Ctrl Pts',(-235.602917916627,6.11500202779203,
128.306204090801));
#259636=CARTESIAN_POINT('Ctrl Pts',(-235.88136554044,1.20353812581378,124.309321602146));
#259637=CARTESIAN_POINT('Ctrl Pts',(-236.159813164253,-4.81391851768082,
126.281062668365));
#259638=CARTESIAN_POINT('Ctrl Pts',(-236.438260788066,-6.40761921642086,
132.40949357451));
#259639=CARTESIAN_POINT('Ctrl Pts',(-236.716708411879,-2.11303088487057,
137.062885708328));
#259640=CARTESIAN_POINT('Ctrl Pts',(-236.995156035692,4.12332960257798,
135.964999029683));
#259641=CARTESIAN_POINT('Ctrl Pts',(-237.273603659505,6.57055162110693,
130.124737761504));
#259642=CARTESIAN_POINT('Ctrl Pts',(-237.552051283318,2.97975768913041,
124.909016696624));
#259643=CARTESIAN_POINT('Ctrl Pts',(-237.83049890713,-3.34928798990126,
125.110828691528));
#259644=CARTESIAN_POINT('Ctrl Pts',(-238.108946530943,-6.60050162802816,
130.544718381962));
#259645=CARTESIAN_POINT('Ctrl Pts',(-238.387394154756,-3.7861767224282,
136.217206602688));
#259646=CARTESIAN_POINT('Ctrl Pts',(-238.665841778569,2.5074596260677,136.915553795314));
#259647=CARTESIAN_POINT('Ctrl Pts',(-238.944289402382,6.49686307441993,
131.998013005973));
#259648=CARTESIAN_POINT('Ctrl Pts',(-239.222737026195,4.51596674678651,
125.983563984846));
#259649=CARTESIAN_POINT('Ctrl Pts',(-239.501184650008,-1.61488240390346,
124.399191560181));
#259650=CARTESIAN_POINT('Ctrl Pts',(-239.77963227382,-6.26173351679718,
128.700856589348));
#259651=CARTESIAN_POINT('Ctrl Pts',(-240.058079897633,-5.15435743044315,
134.935539058562));
#259652=CARTESIAN_POINT('Ctrl Pts',(-240.336527521446,0.689621330129741,
137.373870359787));
#259653=CARTESIAN_POINT('Ctrl Pts',(-240.614975145259,5.89987177818775,
133.775143146303));
#259654=CARTESIAN_POINT('Ctrl Pts',(-240.893422769072,5.68842828685113,
127.446411919705));
#259655=CARTESIAN_POINT('Ctrl Pts',(-241.171870392886,0.249597095069331,
124.203471501526));
#259656=CARTESIAN_POINT('Ctrl Pts',(-241.450318016698,-5.41860163358522,
127.026425709627));
#259657=CARTESIAN_POINT('Ctrl Pts',(-241.728765640511,-6.10737017438111,
133.321117535742));
#259658=CARTESIAN_POINT('Ctrl Pts',(-242.007213264324,-1.18376388654087,
137.303032704464));
#259659=CARTESIAN_POINT('Ctrl Pts',(-242.285660888137,4.82766358294966,
135.312985703106));
#259660=CARTESIAN_POINT('Ctrl Pts',(-242.56410851195,6.40270406418687,129.179732506718));
#259661=CARTESIAN_POINT('Ctrl Pts',(-242.842556135762,2.09397229991911,
124.539433176702));
#259662=CARTESIAN_POINT('Ctrl Pts',(-243.121003759575,-4.13901771174057,
125.65629610612));
#259663=CARTESIAN_POINT('Ctrl Pts',(-243.399451383388,-6.56845264856689,
131.503978824623));
#259664=CARTESIAN_POINT('Ctrl Pts',(-243.677899007202,-2.9618004881116,
136.70874658909));
#259665=CARTESIAN_POINT('Ctrl Pts',(-243.956346631013,3.36660162892119,
136.487672091016));
#259666=CARTESIAN_POINT('Ctrl Pts',(-244.234794254827,6.60126131660758,
131.043911994042));
#259667=CARTESIAN_POINT('Ctrl Pts',(-244.513241878639,3.76968434387551,
125.380015884821));
#259668=CARTESIAN_POINT('Ctrl Pts',(-244.791689502453,-2.52604838156001,
124.70082759102));
#259669=CARTESIAN_POINT('Ctrl Pts',(-245.070137126265,-6.50046604866569,
129.630487974449));
#259670=CARTESIAN_POINT('Ctrl Pts',(-245.348584750079,-4.50127298246883,
135.638879970036));
#259671=CARTESIAN_POINT('Ctrl Pts',(-245.627032373891,1.63437005520677,
137.204584860103));
#259672=CARTESIAN_POINT('Ctrl Pts',(-245.905479997704,6.26810685556324,
132.888796339615));
#259673=CARTESIAN_POINT('Ctrl Pts',(-246.183927621517,5.14175966970064,
126.65751322091));
#259674=CARTESIAN_POINT('Ctrl Pts',(-246.46237524533,-0.709613463692526,
124.236980274974));
#259675=CARTESIAN_POINT('Ctrl Pts',(-246.740822869143,-5.90888649049716,
127.851549029514));
#259676=CARTESIAN_POINT('Ctrl Pts',(-247.019270492956,-5.67818149768794,
134.179607380607));
#259677=CARTESIAN_POINT('Ctrl Pts',(-247.297718116769,-0.229505103091092,
137.405978846438));
#259678=CARTESIAN_POINT('Ctrl Pts',(-247.576165740581,5.43007526929941,
134.565785666913));
#259679=CARTESIAN_POINT('Ctrl Pts',(-247.854613364394,6.09968174312738,
128.269026622868));
#259680=CARTESIAN_POINT('Ctrl Pts',(-248.133060988207,1.16397868104094,
124.302115661998));
#259681=CARTESIAN_POINT('Ctrl Pts',(-248.41150861202,-4.84136392540264,
126.31045016297));
#259682=CARTESIAN_POINT('Ctrl Pts',(-248.689956235833,-6.39772959817725,
132.448468831983));
#259683=CARTESIAN_POINT('Ctrl Pts',(-248.968403859646,-2.07489431669385,
137.075632371099));
#259684=CARTESIAN_POINT('Ctrl Pts',(-249.246851483459,4.15466747760909,
135.939803537374));
#259685=CARTESIAN_POINT('Ctrl Pts',(-249.525299107272,6.56629282677857,
130.08475354068));
#259686=CARTESIAN_POINT('Ctrl Pts',(-249.803746731085,2.94381584937754,
124.890987292882));
#259687=CARTESIAN_POINT('Ctrl Pts',(-250.082194354898,-3.38388408020374,
125.131322246124));
#259688=CARTESIAN_POINT('Ctrl Pts',(-250.36064197871,-6.60195985200274,
130.584902319384));
#259689=CARTESIAN_POINT('Ctrl Pts',(-250.639089602524,-3.75315704348482,
136.240153847548));
#259690=CARTESIAN_POINT('Ctrl Pts',(-250.917537226336,2.54461373609029,
136.900176950603));
#259691=CARTESIAN_POINT('Ctrl Pts',(-251.19598485015,6.50400880347224,131.958442640812));
#259692=CARTESIAN_POINT('Ctrl Pts',(-251.474432473962,4.48653751899202,
125.956163331638));
#259693=CARTESIAN_POINT('Ctrl Pts',(-251.752880097775,-1.65384256596459,
124.409140480742));
#259694=CARTESIAN_POINT('Ctrl Pts',(-252.031327721588,-6.27442212737671,
128.739012511497));
#259695=CARTESIAN_POINT('Ctrl Pts',(-252.309775345401,-5.12911427652582,
134.966838554275));
#259696=CARTESIAN_POINT('Ctrl Pts',(-252.588222969213,0.729599023732927,
137.369550720794));
#259697=CARTESIAN_POINT('Ctrl Pts',(-252.866670593027,5.91784646323776,
133.739173911277));
#259698=CARTESIAN_POINT('Ctrl Pts',(-253.145118216839,5.66788210748017,
127.411847055674));
#259699=CARTESIAN_POINT('Ctrl Pts',(-253.423565840652,0.209410983396998,
124.20207443517));
#259700=CARTESIAN_POINT('Ctrl Pts',(-253.702013464465,-5.44149859849489,
127.059480266814));
#259701=CARTESIAN_POINT('Ctrl Pts',(-253.980461088278,-6.0919368110008,
133.358248211846));
#259702=CARTESIAN_POINT('Ctrl Pts',(-254.258908712091,-1.1441826817532,
137.310118186916));
#259703=CARTESIAN_POINT('Ctrl Pts',(-254.537356335904,4.85501939763767,
135.283514846073));
#259704=CARTESIAN_POINT('Ctrl Pts',(-254.815803959717,6.39269590315201,
129.140787462715));
#259705=CARTESIAN_POINT('Ctrl Pts',(-255.09425158353,2.05579703890082,124.526802775315));
#259706=CARTESIAN_POINT('Ctrl Pts',(-255.372699207342,-4.17027861730954,
125.681586622223));
#259707=CARTESIAN_POINT('Ctrl Pts',(-255.651146831155,-6.5640724361261,
131.5439503534));
#259708=CARTESIAN_POINT('Ctrl Pts',(-255.929594454968,-2.925803447894,136.726665654721));
#259709=CARTESIAN_POINT('Ctrl Pts',(-256.208042078781,3.40113425532747,
136.467074956607));
#259710=CARTESIAN_POINT('Ctrl Pts',(-256.486489702594,6.60259898059897,
131.003720738236));
#259711=CARTESIAN_POINT('Ctrl Pts',(-256.764937326407,3.73659166461274,
125.357175036369));
#259712=CARTESIAN_POINT('Ctrl Pts',(-257.04338495022,-2.56314926818932,
124.716306516944));
#259713=CARTESIAN_POINT('Ctrl Pts',(-257.321832574033,-6.5075031063131,
129.670100547101));
#259714=CARTESIAN_POINT('Ctrl Pts',(-257.600280197845,-4.47173821150659,
135.666151948257));
#259715=CARTESIAN_POINT('Ctrl Pts',(-257.878727821659,1.67325768403046,
137.194590998305));
#259716=CARTESIAN_POINT('Ctrl Pts',(-258.157175445471,6.28075871394982,
132.850463013089));
#259717=CARTESIAN_POINT('Ctrl Pts',(-258.435623069284,5.1162713672671,126.626553096149));
#259718=CARTESIAN_POINT('Ctrl Pts',(-258.714070693097,-0.749294580734974,
124.240926059104));
#259719=CARTESIAN_POINT('Ctrl Pts',(-258.99251831691,-5.92728653745133,
127.888508918958));
#259720=CARTESIAN_POINT('Ctrl Pts',(-259.270965940723,-5.656519339957,134.212338033208));
#259721=CARTESIAN_POINT('Ctrl Pts',(-259.549413564536,-0.191230405826049,
137.41063083554));
#259722=CARTESIAN_POINT('Ctrl Pts',(-259.827861188349,5.45654320709978,
134.526020746857));
#259723=CARTESIAN_POINT('Ctrl Pts',(-260.059900874859,5.97341346954355,
129.293215926205));
#259724=CARTESIAN_POINT('Ctrl Pts',(-260.245542550368,3.60742224527213,
126.247226657536));
#259725=CARTESIAN_POINT('Ctrl Pts',(-260.338368351272,1.86717727106152,
125.459413119698));
#259726=CARTESIAN_POINT('Ctrl Pts',(-260.384786214875,0.950008195528324,
125.301089073499));
#259727=CARTESIAN_POINT('Ctrl Pts',(209.997886486728,-2.58542267678463,
125.478296443779));
#259728=CARTESIAN_POINT('Ctrl Pts',(209.951476810375,-3.47289965896197,
125.909102290886));
#259729=CARTESIAN_POINT('Ctrl Pts',(209.85865919672,-5.01373755653622,127.222906143875));
#259730=CARTESIAN_POINT('Ctrl Pts',(209.67302570846,-6.52844908712303,131.020616473957));
#259731=CARTESIAN_POINT('Ctrl Pts',(209.440986021949,-4.4641631800594,136.198709217918));
#259732=CARTESIAN_POINT('Ctrl Pts',(209.162538398136,2.13623200523086,137.47712630299));
#259733=CARTESIAN_POINT('Ctrl Pts',(208.884090774324,6.76311047611758,132.61329501932));
#259734=CARTESIAN_POINT('Ctrl Pts',(208.60564315051,5.180460236421,126.09244423763));
#259735=CARTESIAN_POINT('Ctrl Pts',(208.327195526698,-1.16565068102074,
123.898824768668));
#259736=CARTESIAN_POINT('Ctrl Pts',(208.048747902884,-6.43906639651766,
128.052530506575));
#259737=CARTESIAN_POINT('Ctrl Pts',(207.770300279072,-5.79609906993421,
134.734252735451));
#259738=CARTESIAN_POINT('Ctrl Pts',(207.491852655259,0.173626147510206,
137.805009652024));
#259739=CARTESIAN_POINT('Ctrl Pts',(207.213405031446,5.98357180802623,134.442293088818));
#259740=CARTESIAN_POINT('Ctrl Pts',(206.934957407633,6.29502677410122,127.736610299611));
#259741=CARTESIAN_POINT('Ctrl Pts',(206.65650978382,0.821596385081328,123.849978754804));
#259742=CARTESIAN_POINT('Ctrl Pts',(206.378062160007,-5.40680743188727,
126.354116934927));
#259743=CARTESIAN_POINT('Ctrl Pts',(206.099614536195,-6.66663710465116,
132.947794423038));
#259744=CARTESIAN_POINT('Ctrl Pts',(205.821166912381,-1.80014356190772,
137.571770081489));
#259745=CARTESIAN_POINT('Ctrl Pts',(205.542719288569,4.72058899422897,135.976822216287));
#259746=CARTESIAN_POINT('Ctrl Pts',(205.264271664756,6.90333351468265,129.628637390042));
#259747=CARTESIAN_POINT('Ctrl Pts',(204.985824040943,2.74225038547515,124.360883417158));
#259748=CARTESIAN_POINT('Ctrl Pts',(204.70737641713,-3.93882614214087,125.014370927945));
#259749=CARTESIAN_POINT('Ctrl Pts',(204.428928793317,-7.00031425910704,
130.988575726592));
#259750=CARTESIAN_POINT('Ctrl Pts',(204.150481169504,-3.62885534891233,
136.793496040797));
#259751=CARTESIAN_POINT('Ctrl Pts',(203.872033545692,3.07734423765085,137.09469337995));
#259752=CARTESIAN_POINT('Ctrl Pts',(203.593585921878,6.95561486460971,131.615382266785));
#259753=CARTESIAN_POINT('Ctrl Pts',(203.315138298066,4.44201520086038,125.390781848689));
#259754=CARTESIAN_POINT('Ctrl Pts',(203.036690674253,-2.15357941165663,
124.140995867004));
#259755=CARTESIAN_POINT('Ctrl Pts',(202.75824305044,-6.77013976170558,129.014516559232));
#259756=CARTESIAN_POINT('Ctrl Pts',(202.479795426627,-5.16527240588502,
135.532816506767));
#259757=CARTESIAN_POINT('Ctrl Pts',(202.201347802814,1.18622795093483,137.705896487686));
#259758=CARTESIAN_POINT('Ctrl Pts',(201.922900179001,6.44764277258624,133.536802163981));
#259759=CARTESIAN_POINT('Ctrl Pts',(201.644452555188,5.78398887041165,126.856727545651));
#259760=CARTESIAN_POINT('Ctrl Pts',(201.366004931376,-0.194868239746226,
123.804334868162));
#259761=CARTESIAN_POINT('Ctrl Pts',(201.087557307562,-5.99465095761073,
127.184623883922));
#259762=CARTESIAN_POINT('Ctrl Pts',(200.80910968375,-6.2856423003101,133.891274124028));
#259763=CARTESIAN_POINT('Ctrl Pts',(200.530662059936,-0.80043543977546,
137.76120165575));
#259764=CARTESIAN_POINT('Ctrl Pts',(200.252214436124,5.42033248649604,135.238132133988));
#259765=CARTESIAN_POINT('Ctrl Pts',(199.973766812311,6.66007965562565,128.640643190398));
#259766=CARTESIAN_POINT('Ctrl Pts',(199.695319188498,1.77953898422249,124.031504858911));
#259767=CARTESIAN_POINT('Ctrl Pts',(199.416871564685,-4.73631107837294,
125.646290097223));
#259768=CARTESIAN_POINT('Ctrl Pts',(199.138423940872,-6.89972264160091,
132.00109015798));
#259769=CARTESIAN_POINT('Ctrl Pts',(198.859976317059,-2.72262616738874,
137.256154234582));
#259770=CARTESIAN_POINT('Ctrl Pts',(198.581528693247,3.95643074697165,136.582335164788));
#259771=CARTESIAN_POINT('Ctrl Pts',(198.303081069434,6.999721087252,130.598839755845));
#259772=CARTESIAN_POINT('Ctrl Pts',(198.024633445621,3.61060970373355,124.804207978572));
#259773=CARTESIAN_POINT('Ctrl Pts',(197.746185821808,-3.09647560942607,
124.523423352781));
#259774=CARTESIAN_POINT('Ctrl Pts',(197.467738197995,-6.9580511087663,130.014513232485));
#259775=CARTESIAN_POINT('Ctrl Pts',(197.189290574182,-4.4255175588443,136.231434272887));
#259776=CARTESIAN_POINT('Ctrl Pts',(196.910842950369,2.17385042910367,137.461139751337));
#259777=CARTESIAN_POINT('Ctrl Pts',(196.632395326556,6.77555607120273,132.573590407591));
#259778=CARTESIAN_POINT('Ctrl Pts',(196.353947702743,5.15085668818228,126.060205318492));
#259779=CARTESIAN_POINT('Ctrl Pts',(196.07550007893,-1.20722835793932,123.90646718437));
#259780=CARTESIAN_POINT('Ctrl Pts',(195.797052455118,-6.45592951949867,
128.091556134528));
#259781=CARTESIAN_POINT('Ctrl Pts',(195.518604831305,-5.77194684232935,
134.769579876729));
#259782=CARTESIAN_POINT('Ctrl Pts',(195.240157207492,0.216173007661386,
137.80376083149));
#259783=CARTESIAN_POINT('Ctrl Pts',(194.961709583679,6.00564042424985,134.405834929363));
#259784=CARTESIAN_POINT('Ctrl Pts',(194.683261959866,6.2762176827981,127.698330076496));
#259785=CARTESIAN_POINT('Ctrl Pts',(194.404814336053,0.779257501134259,
123.845115552844));
#259786=CARTESIAN_POINT('Ctrl Pts',(194.12636671224,-5.43380225522669,126.387107265649));
#259787=CARTESIAN_POINT('Ctrl Pts',(193.847919088427,-6.65346319503207,
132.988339014042));
#259788=CARTESIAN_POINT('Ctrl Pts',(193.569471464615,-1.75891649835014,
137.58260130935));
#259789=CARTESIAN_POINT('Ctrl Pts',(193.291023840801,4.75198853246758,135.947991544374));
#259790=CARTESIAN_POINT('Ctrl Pts',(193.012576216989,6.89604824949333,129.586636238002));
#259791=CARTESIAN_POINT('Ctrl Pts',(192.734128593176,2.70297651592057,124.344310147306));
#259792=CARTESIAN_POINT('Ctrl Pts',(192.455680969363,-3.97399858803937,
125.038454847768));
#259793=CARTESIAN_POINT('Ctrl Pts',(192.17723334555,-6.99906313021511,131.031185270517));
#259794=CARTESIAN_POINT('Ctrl Pts',(191.898785721737,-3.59233057896577,
136.815474918205));
#259795=CARTESIAN_POINT('Ctrl Pts',(191.620338097924,3.11557827924791,137.075844182864));
#259796=CARTESIAN_POINT('Ctrl Pts',(191.341890474111,6.96042290329331,131.573026430018));
#259797=CARTESIAN_POINT('Ctrl Pts',(191.063442850298,4.40897891477476,125.363842346942));
#259798=CARTESIAN_POINT('Ctrl Pts',(190.784995226486,-2.19410130582752,
124.154228770475));
#259799=CARTESIAN_POINT('Ctrl Pts',(190.506547602672,-6.78090961418206,
129.055761484483));
#259800=CARTESIAN_POINT('Ctrl Pts',(190.22809997886,-5.13639325295408,135.564171377977));
#259801=CARTESIAN_POINT('Ctrl Pts',(189.949652355047,1.22821758097839,137.698547712335));
#259802=CARTESIAN_POINT('Ctrl Pts',(189.671204731234,6.46415645975623,133.497502906364));
#259803=CARTESIAN_POINT('Ctrl Pts',(189.392757107421,5.75985134361714,126.821591904301));
#259804=CARTESIAN_POINT('Ctrl Pts',(189.114309483608,-0.237475772924818,
123.80565078066));
#259805=CARTESIAN_POINT('Ctrl Pts',(188.835861859795,-6.01657425548534,
127.221182091151));
#259806=CARTESIAN_POINT('Ctrl Pts',(188.557414235982,-6.2667349232476,133.929479419415));
#259807=CARTESIAN_POINT('Ctrl Pts',(188.278966612169,-0.758072343566082,
137.76594523932));
#259808=CARTESIAN_POINT('Ctrl Pts',(188.000518988357,5.44722168595988,135.205054884148));
#259809=CARTESIAN_POINT('Ctrl Pts',(187.722071364544,6.64678509766207,128.600141483854));
#259810=CARTESIAN_POINT('Ctrl Pts',(187.443623740731,1.73827771811677,124.02079778535));
#259811=CARTESIAN_POINT('Ctrl Pts',(187.165176116918,-4.76762196479028,
125.675216934184));
#259812=CARTESIAN_POINT('Ctrl Pts',(186.886728493105,-6.89230997333645,
132.043068555446));
#259813=CARTESIAN_POINT('Ctrl Pts',(186.608280869292,-2.68330182444739,
137.272608096043));
#259814=CARTESIAN_POINT('Ctrl Pts',(186.329833245479,3.99152961452714,136.558144195375));
#259815=CARTESIAN_POINT('Ctrl Pts',(186.051385621667,6.99834033481346,130.556234274655));
#259816=CARTESIAN_POINT('Ctrl Pts',(185.772937997853,3.5740181753383,124.782340341422));
#259817=CARTESIAN_POINT('Ctrl Pts',(185.494490374041,-3.13465208677821,
124.542388849921));
#259818=CARTESIAN_POINT('Ctrl Pts',(185.216042750227,-6.96273021741339,
130.056883498557));
#259819=CARTESIAN_POINT('Ctrl Pts',(184.937595126415,-4.39239942652681,
136.258273103275));
#259820=CARTESIAN_POINT('Ctrl Pts',(184.659147502602,2.21433185669671,137.447783572063));
#259821=CARTESIAN_POINT('Ctrl Pts',(184.380699878789,6.78620033974098,132.532312894923));
#259822=CARTESIAN_POINT('Ctrl Pts',(184.102252254976,5.12188223488049,126.028938490053));
#259823=CARTESIAN_POINT('Ctrl Pts',(183.823804631163,-1.24919542597752,
123.913943728027));
#259824=CARTESIAN_POINT('Ctrl Pts',(183.54535700735,-6.47232351695142,128.130905471908));
#259825=CARTESIAN_POINT('Ctrl Pts',(183.266909383538,-5.74770248642891,
134.804641889104));
#259826=CARTESIAN_POINT('Ctrl Pts',(182.988461759724,0.258776338245136,
137.80231524236));
#259827=CARTESIAN_POINT('Ctrl Pts',(182.710014135912,6.02745234999885,134.369210164519));
#259828=CARTESIAN_POINT('Ctrl Pts',(182.431566512099,6.25719410952084,127.66018250561));
#259829=CARTESIAN_POINT('Ctrl Pts',(182.153118888286,0.73688016331929,123.840500929948));
#259830=CARTESIAN_POINT('Ctrl Pts',(181.874671264473,-5.46059065437546,
126.420266203747));
#259831=CARTESIAN_POINT('Ctrl Pts',(181.59622364066,-6.64004542538295,133.028800068927));
#259832=CARTESIAN_POINT('Ctrl Pts',(181.317776016847,-1.71762283471616,
137.593182748215));
#259833=CARTESIAN_POINT('Ctrl Pts',(181.039328393035,4.78321123051439,135.918969541833));
#259834=CARTESIAN_POINT('Ctrl Pts',(180.760880769221,6.88850784776155,129.544680596588));
#259835=CARTESIAN_POINT('Ctrl Pts',(180.482433145409,2.66360227523266,124.32797605183));
#259836=CARTESIAN_POINT('Ctrl Pts',(180.203985521595,-4.00902366402984,
125.062752534008));
#259837=CARTESIAN_POINT('Ctrl Pts',(179.925537897783,-6.99755270774298,
131.073786351827));
#259838=CARTESIAN_POINT('Ctrl Pts',(179.64709027397,-3.5556726624947,136.837231082039));
#259839=CARTESIAN_POINT('Ctrl Pts',(179.368642650157,3.15369685531979,137.056762577506));
#259840=CARTESIAN_POINT('Ctrl Pts',(179.090195026344,6.96497302975191,131.530642118605));
#259841=CARTESIAN_POINT('Ctrl Pts',(178.811747402531,4.37577924769062,125.337104441072));
#259842=CARTESIAN_POINT('Ctrl Pts',(178.533299778718,-2.23454189429802,
124.167708099424));
#259843=CARTESIAN_POINT('Ctrl Pts',(178.254852154906,-6.79142819886702,
129.097071203448));
#259844=CARTESIAN_POINT('Ctrl Pts',(177.976404531092,-5.10732376838957,
135.595349873321));
#259845=CARTESIAN_POINT('Ctrl Pts',(177.69795690728,1.27016169860089,137.690943469992));
#259846=CARTESIAN_POINT('Ctrl Pts',(177.419509283467,6.48043061542571,133.458103853558));
#259847=CARTESIAN_POINT('Ctrl Pts',(177.141061659654,5.73550038331004,126.786603845811));
#259848=CARTESIAN_POINT('Ctrl Pts',(176.862614035841,-0.280074506296806,
123.807226032976));
#259849=CARTESIAN_POINT('Ctrl Pts',(176.584166412028,-6.0382746070172,127.257873074351));
#259850=CARTESIAN_POINT('Ctrl Pts',(176.305718788215,-6.24759533000263,
133.967568912391));
#259851=CARTESIAN_POINT('Ctrl Pts',(176.027271164402,-0.71568115671533,
137.770430858802));
#259852=CARTESIAN_POINT('Ctrl Pts',(175.748823540589,5.4739090366252,135.171814564968));
#259853=CARTESIAN_POINT('Ctrl Pts',(175.470375916777,6.63324424063007,128.559721455457));
#259854=CARTESIAN_POINT('Ctrl Pts',(175.191928292964,1.69695203949225,124.010342079205));
#259855=CARTESIAN_POINT('Ctrl Pts',(174.913480669151,-4.79875618522306,
125.704333833448));
#259856=CARTESIAN_POINT('Ctrl Pts',(174.635033045338,-6.88464190799096,
132.085001052137));
#259857=CARTESIAN_POINT('Ctrl Pts',(174.356585421525,-2.64387805077028,
137.288822274217));
#259858=CARTESIAN_POINT('Ctrl Pts',(174.078137797712,4.02648057448505,136.533740017397));
#259859=CARTESIAN_POINT('Ctrl Pts',(173.799690173899,6.99670025630013,130.513637987877));
#259860=CARTESIAN_POINT('Ctrl Pts',(173.521242550086,3.53729421038521,124.76069585245));
#259861=CARTESIAN_POINT('Ctrl Pts',(173.242794926273,-3.17271240844464,
124.561586386726));
#259862=CARTESIAN_POINT('Ctrl Pts',(172.96434730246,-6.96715131953175,130.099281462668));
#259863=CARTESIAN_POINT('Ctrl Pts',(172.685899678648,-4.35911853223319,
136.284909836929));
#259864=CARTESIAN_POINT('Ctrl Pts',(172.407452054835,2.25473123140845,137.434181218309));
#259865=CARTESIAN_POINT('Ctrl Pts',(172.129004431022,6.79659314313001,132.490971352347));
#259866=CARTESIAN_POINT('Ctrl Pts',(171.850556807209,5.09271798834896,125.997848616637));
#259867=CARTESIAN_POINT('Ctrl Pts',(171.572109183396,-1.29111620461978,
123.921675598615));
#259868=CARTESIAN_POINT('Ctrl Pts',(171.293661559583,-6.48847768007612,
128.170353875152));
#259869=CARTESIAN_POINT('Ctrl Pts',(171.01521393577,-5.72324514729908,134.839555669585));
#259870=CARTESIAN_POINT('Ctrl Pts',(170.736766311957,0.301370079776633,
137.800610341449));
#259871=CARTESIAN_POINT('Ctrl Pts',(170.458318688145,6.04904092628448,134.332453302864));
#259872=CARTESIAN_POINT('Ctrl Pts',(170.179871064331,6.23793867361471,127.6221514434));
#259873=CARTESIAN_POINT('Ctrl Pts',(169.901423440519,0.694475520138818,
123.836144355433));
#259874=CARTESIAN_POINT('Ctrl Pts',(169.622975816706,-5.4871767093294,126.453587596077));
#259875=CARTESIAN_POINT('Ctrl Pts',(169.344528192893,-6.62638160640872,
133.06917869639));
#259876=CARTESIAN_POINT('Ctrl Pts',(169.06608056908,-1.67626552393645,137.603512624779));
#259877=CARTESIAN_POINT('Ctrl Pts',(168.787632945267,4.81425668490999,135.88975801558));
#259878=CARTESIAN_POINT('Ctrl Pts',(168.509185321454,6.88071218983824,129.50277163308));
#259879=CARTESIAN_POINT('Ctrl Pts',(168.230737697641,2.62412933378287,124.311881941165));
#259880=CARTESIAN_POINT('Ctrl Pts',(167.952290073828,-4.0439001841742,125.087262977647));
#259881=CARTESIAN_POINT('Ctrl Pts',(167.673842450016,-6.99578298838191,
131.116377449467));
#259882=CARTESIAN_POINT('Ctrl Pts',(167.395394826203,-3.51888298926545,
136.858763695638));
#259883=CARTESIAN_POINT('Ctrl Pts',(167.11694720239,3.19169856999505,137.037449287095));
#259884=CARTESIAN_POINT('Ctrl Pts',(166.838499578577,6.96926506657354,131.488230894564));
#259885=CARTESIAN_POINT('Ctrl Pts',(166.560051954764,4.34241743449723,125.310569126392));
#259886=CARTESIAN_POINT('Ctrl Pts',(166.281604330951,-2.27489968099678,
124.181433351974));
#259887=CARTESIAN_POINT('Ctrl Pts',(166.003156707138,-6.80169512468258,
129.13844418665));
#259888=CARTESIAN_POINT('Ctrl Pts',(165.724709083325,-5.0780650300646,135.626350836796));
#259889=CARTESIAN_POINT('Ctrl Pts',(165.446261459512,1.31205874991464,137.683084042787));
#259890=CARTESIAN_POINT('Ctrl Pts',(165.1678138357,6.49646463635559,133.418606465321));
#259891=CARTESIAN_POINT('Ctrl Pts',(164.889366211887,5.71093689192698,126.751764666776));
#259892=CARTESIAN_POINT('Ctrl Pts',(164.610918588074,-0.322662861405092,
123.809060566689));
#259893=CARTESIAN_POINT('Ctrl Pts',(164.332470964261,-6.05975120806294,
127.29469547395));
#259894=CARTESIAN_POINT('Ctrl Pts',(164.054023340448,-6.22822422981513,
134.00554119152));
#259895=CARTESIAN_POINT('Ctrl Pts',(163.775575716635,-0.673263450036036,
137.774658347991));
#259896=CARTESIAN_POINT('Ctrl Pts',(163.497128092822,5.50039354957815,135.138412408175));
#259897=CARTESIAN_POINT('Ctrl Pts',(163.218680469009,6.61945758629338,128.51938460299));
#259898=CARTESIAN_POINT('Ctrl Pts',(162.940232845196,1.65556347968583,124.000138127916));
#259899=CARTESIAN_POINT('Ctrl Pts',(162.661785221384,-4.82971258598073,
125.733639716082));
#259900=CARTESIAN_POINT('Ctrl Pts',(162.383337597571,-6.87671872970774,
132.126886094224));
#259901=CARTESIAN_POINT('Ctrl Pts',(162.104889973758,-2.60435630721971,
137.304796168278));
#259902=CARTESIAN_POINT('Ctrl Pts',(161.826442349945,4.06128233172446,136.509123535159));
#259903=CARTESIAN_POINT('Ctrl Pts',(161.547994726132,6.99480091248578,130.471052473933));
#259904=CARTESIAN_POINT('Ctrl Pts',(161.269547102319,3.50043916969439,124.739275313697));
#259905=CARTESIAN_POINT('Ctrl Pts',(160.991099478506,-3.21065516408591,
124.581015251828));
#259906=CARTESIAN_POINT('Ctrl Pts',(160.712651854693,-6.97131425129578,
130.141705553748));
#259907=CARTESIAN_POINT('Ctrl Pts',(160.434204230881,-4.32567610919938,
136.311343486817));
#259908=CARTESIAN_POINT('Ctrl Pts',(160.155756607067,2.29504705622523,137.420333194114));
#259909=CARTESIAN_POINT('Ctrl Pts',(159.877308983254,6.80673409626067,132.449567311792));
#259910=CARTESIAN_POINT('Ctrl Pts',(159.598861359442,5.06336502927952,125.966936850291));
#259911=CARTESIAN_POINT('Ctrl Pts',(159.320413735629,-1.33298914047637,
123.929662509627));
#259912=CARTESIAN_POINT('Ctrl Pts',(159.041966111816,-6.50439141027418,
128.209899882485));
#259913=CARTESIAN_POINT('Ctrl Pts',(158.763518488003,-5.69857573121565,
134.874319924428));
#259914=CARTESIAN_POINT('Ctrl Pts',(158.48507086419,0.343952653928878,137.798646191931));
#259915=CARTESIAN_POINT('Ctrl Pts',(158.206623240377,6.07040535313402,134.295565706438));
#259916=CARTESIAN_POINT('Ctrl Pts',(157.928175616564,6.2184520885971,127.584238299121));
#259917=CARTESIAN_POINT('Ctrl Pts',(157.649727992752,0.652045142912632,
123.832045990734));
#259918=CARTESIAN_POINT('Ctrl Pts',(157.371280368939,-5.51355943493244,
126.487070207899));
#259919=CARTESIAN_POINT('Ctrl Pts',(157.092832745126,-6.61247224442723,
133.109473400187));
#259920=CARTESIAN_POINT('Ctrl Pts',(156.814385121313,-1.63484609852131,
137.613590556265));
#259921=CARTESIAN_POINT('Ctrl Pts',(156.5359374975,4.84512374525377,135.860358048054));
#259922=CARTESIAN_POINT('Ctrl Pts',(156.257489873687,6.87266156459436,129.46091090043));
#259923=CARTESIAN_POINT('Ctrl Pts',(155.979042249874,2.58455915425555,124.296028411687));
#259924=CARTESIAN_POINT('Ctrl Pts',(155.700594626061,-4.07862685611001,
125.111985270442));
#259925=CARTESIAN_POINT('Ctrl Pts',(155.422147002248,-6.99375403770952,
131.158956985208));
#259926=CARTESIAN_POINT('Ctrl Pts',(155.143699378435,-3.48196292253304,
136.880071961106));
#259927=CARTESIAN_POINT('Ctrl Pts',(154.865251754623,3.22958201510593,137.017905027291));
#259928=CARTESIAN_POINT('Ctrl Pts',(154.58680413081,6.97329885471516,131.445794329457));
#259929=CARTESIAN_POINT('Ctrl Pts',(154.308356506997,4.30889471142897,125.284237386175));
#259930=CARTESIAN_POINT('Ctrl Pts',(154.029908883184,-2.31517317045128,
124.195404019528));
#259931=CARTESIAN_POINT('Ctrl Pts',(153.751461259371,-6.81171001118396,
129.179878900999));
#259932=CARTESIAN_POINT('Ctrl Pts',(153.473013635558,-5.04861812217248,
135.65717311965));
#259933=CARTESIAN_POINT('Ctrl Pts',(153.194566011745,1.3539071824088,137.674969721956));
#259934=CARTESIAN_POINT('Ctrl Pts',(152.916118387933,6.51225792839928,133.379012205241));
#259935=CARTESIAN_POINT('Ctrl Pts',(152.637670764119,5.68616177967723,126.717075658174));
#259936=CARTESIAN_POINT('Ctrl Pts',(152.359223140307,-0.365239260122265,
123.811154313817));
#259937=CARTESIAN_POINT('Ctrl Pts',(152.080775516494,-6.08100326279917,
127.331647925483));
#259938=CARTESIAN_POINT('Ctrl Pts',(151.802327892681,-6.20862234048841,
134.043394849727));
#259939=CARTESIAN_POINT('Ctrl Pts',(151.523880268868,-0.630820795332096,
137.778627550233));
#259940=CARTESIAN_POINT('Ctrl Pts',(151.245432645055,5.52667424342534,135.104849651499));
#259941=CARTESIAN_POINT('Ctrl Pts',(150.966985021242,6.60542564552152,128.479132421149));
#259942=CARTESIAN_POINT('Ctrl Pts',(150.688537397429,1.61411357236584,123.990186309594));
#259943=CARTESIAN_POINT('Ctrl Pts',(150.410089773616,-4.86049001996232,
125.763133496143));
#259944=CARTESIAN_POINT('Ctrl Pts',(150.131642149803,-6.8685407320831,132.168722129643));
#259945=CARTESIAN_POINT('Ctrl Pts',(149.853194525991,-2.56473805828847,
137.32052918631));
#259946=CARTESIAN_POINT('Ctrl Pts',(149.574746902178,4.09593359665354,136.484295660832));
#259947=CARTESIAN_POINT('Ctrl Pts',(149.296299278365,6.99264237375128,130.428479310845));
#259948=CARTESIAN_POINT('Ctrl Pts',(149.017851654552,3.46345441894284,124.718079518912));
#259949=CARTESIAN_POINT('Ctrl Pts',(148.739404030739,-3.24847894771935,
124.600674725279));
#259950=CARTESIAN_POINT('Ctrl Pts',(148.460956406926,-6.97521885844655,
130.184154199754));
#259951=CARTESIAN_POINT('Ctrl Pts',(148.182508783113,-4.29207339664657,
136.337573073429));
#259952=CARTESIAN_POINT('Ctrl Pts',(147.9040611593,2.33527783722936,137.406240012622));
#259953=CARTESIAN_POINT('Ctrl Pts',(147.625613535487,6.81662282335624,132.408102307496));
#259954=CARTESIAN_POINT('Ctrl Pts',(147.347165911675,5.03382444535687,125.936204336462));
#259955=CARTESIAN_POINT('Ctrl Pts',(147.068718287862,-1.37481268193005,
123.937904165105));
#259956=CARTESIAN_POINT('Ctrl Pts',(146.790270664049,-6.52006411785656,
128.249542028514));
#259957=CARTESIAN_POINT('Ctrl Pts',(146.511823040236,-5.67369515231286,
134.908933365434));
#259958=CARTESIAN_POINT('Ctrl Pts',(146.233375416423,0.386522482789046,
137.796422866589));
#259959=CARTESIAN_POINT('Ctrl Pts',(145.95492779261,6.09154483888081,134.258548742122));
#259960=CARTESIAN_POINT('Ctrl Pts',(145.676480168797,6.19873507655051,127.546444477659));
#259961=CARTESIAN_POINT('Ctrl Pts',(145.398032544984,0.609590603913882,
123.828205987717));
#259962=CARTESIAN_POINT('Ctrl Pts',(145.119584921171,-5.53973785356302,
126.520712798507));
#259963=CARTESIAN_POINT('Ctrl Pts',(144.841137297358,-6.59831785485502,
133.149682687181));
#259964=CARTESIAN_POINT('Ctrl Pts',(144.562689673546,-1.59336609328267,
137.623416169231));
#259965=CARTESIAN_POINT('Ctrl Pts',(144.284242049733,4.87581126775532,135.830770728684));
#259966=CARTESIAN_POINT('Ctrl Pts',(144.00579442592,6.86435627034879,129.419099949804));
#259967=CARTESIAN_POINT('Ctrl Pts',(143.727346802107,2.54489320293839,124.280416050852));
#259968=CARTESIAN_POINT('Ctrl Pts',(143.448899178294,-4.11320239302776,
125.136918496298));
#259969=CARTESIAN_POINT('Ctrl Pts',(143.170451554481,-6.99146593090932,
131.201523381251));
#259970=CARTESIAN_POINT('Ctrl Pts',(142.892003930668,-3.44491383038404,
136.901155088855));
#259971=CARTESIAN_POINT('Ctrl Pts',(142.613556306855,3.26734578686757,136.998130522314));
#259972=CARTESIAN_POINT('Ctrl Pts',(142.335108683042,6.97707424470332,131.403333995789));
#259973=CARTESIAN_POINT('Ctrl Pts',(142.05666105923,4.27521232068256,125.258110196154));
#259974=CARTESIAN_POINT('Ctrl Pts',(141.778213435417,-2.35536087031262,
124.209619584399));
#259975=CARTESIAN_POINT('Ctrl Pts',(141.499765811604,-6.8214724872659,129.221373811115));
#259976=CARTESIAN_POINT('Ctrl Pts',(141.221318187791,-5.01898413587917,
135.687815579753));
#259977=CARTESIAN_POINT('Ctrl Pts',(140.942870563978,1.39570544537436,137.666600808179));
#259978=CARTESIAN_POINT('Ctrl Pts',(140.664422940165,6.52780990633047,133.339322540502));
#259979=CARTESIAN_POINT('Ctrl Pts',(140.385975316352,5.66117596461176,126.68253810542));
#259980=CARTESIAN_POINT('Ctrl Pts',(140.10752769254,-0.407802124764288,
123.813507196776));
#259981=CARTESIAN_POINT('Ctrl Pts',(139.829080068726,-6.10202998372316,
127.368729059661));
#259982=CARTESIAN_POINT('Ctrl Pts',(139.550632444914,-6.18879038837768,
134.081128484328));
#259983=CARTESIAN_POINT('Ctrl Pts',(139.272184821101,-0.588354765331746,
137.78233831845));
#259984=CARTESIAN_POINT('Ctrl Pts',(138.993737197288,5.55275014432601,135.071127538621));
#259985=CARTESIAN_POINT('Ctrl Pts',(138.715289573475,6.59114893827324,128.438966401494));
#259986=CARTESIAN_POINT('Ctrl Pts',(138.436841949662,1.57260385347371,123.980486993006));
#259987=CARTESIAN_POINT('Ctrl Pts',(138.158394325849,-4.8910873466988,125.792814080728));
#259988=CARTESIAN_POINT('Ctrl Pts',(137.879946702036,-6.86010821815569,
132.210507608145));
#259989=CARTESIAN_POINT('Ctrl Pts',(137.601499078223,-2.52502477204539,
137.336020745319));
#259990=CARTESIAN_POINT('Ctrl Pts',(137.32305145441,4.13043308525698,136.459257314423));
#259991=CARTESIAN_POINT('Ctrl Pts',(137.044603830598,6.99022472008204,130.385920076178));
#259992=CARTESIAN_POINT('Ctrl Pts',(136.766156206785,3.42634132861412,124.69710925351));
#259993=CARTESIAN_POINT('Ctrl Pts',(136.487708582972,-3.28618235777073,
124.620564078594));
#259994=CARTESIAN_POINT('Ctrl Pts',(136.209260959159,-6.97886499629743,
130.226625827737));
#259995=CARTESIAN_POINT('Ctrl Pts',(135.930813335346,-4.25831163973555,
136.363597624819));
#259996=CARTESIAN_POINT('Ctrl Pts',(135.652365711533,2.37542208365453,137.391902196061));
#259997=CARTESIAN_POINT('Ctrl Pts',(135.37391808772,6.82625895798624,132.366577875963));
#259998=CARTESIAN_POINT('Ctrl Pts',(135.095470463907,5.00409733121823,125.905652213954));
#259999=CARTESIAN_POINT('Ctrl Pts',(134.817022840094,-1.4165852791943,123.946400259653));
#260000=CARTESIAN_POINT('Ctrl Pts',(134.538575216282,-6.53549522206528,
128.289278844285));
#260001=CARTESIAN_POINT('Ctrl Pts',(134.260127592469,-5.64860433254967,
134.943394709987));
#260002=CARTESIAN_POINT('Ctrl Pts',(133.981679968656,0.429077988916399,
137.793940447809));
#260003=CARTESIAN_POINT('Ctrl Pts',(133.703232344843,6.1124586001935,134.221403781595));
#260004=CARTESIAN_POINT('Ctrl Pts',(133.42478472103,6.17878836809604,127.508771379477));
#260005=CARTESIAN_POINT('Ctrl Pts',(133.146337097217,0.567113476311158,
123.824624488677));
#260006=CARTESIAN_POINT('Ctrl Pts',(132.867889473404,-5.5657109951702,126.554514121259));
#260007=CARTESIAN_POINT('Ctrl Pts',(132.589441849591,-6.58391896218814,
133.189805067404));
#260008=CARTESIAN_POINT('Ctrl Pts',(132.310994225778,-1.55182704527753,
137.632989099587));
#260009=CARTESIAN_POINT('Ctrl Pts',(132.032546601965,4.90631811527725,135.800997153839));
#260010=CARTESIAN_POINT('Ctrl Pts',(131.754098978153,6.85579661485726,129.377340330521));
#260011=CARTESIAN_POINT('Ctrl Pts',(131.47565135434,2.50513294966777,124.265045437181));
#260012=CARTESIAN_POINT('Ctrl Pts',(131.197203730527,-4.14762551371829,
125.162061731307));
#260013=CARTESIAN_POINT('Ctrl Pts',(130.918756106714,-6.98891875276791,
131.244075060281));
#260014=CARTESIAN_POINT('Ctrl Pts',(130.640308482901,-3.4077370856862,136.922012297644));
#260015=CARTESIAN_POINT('Ctrl Pts',(130.361860859088,3.30498848592948,136.978126504915));
#260016=CARTESIAN_POINT('Ctrl Pts',(130.083413235275,6.98059109663955,131.360851466943));
#260017=CARTESIAN_POINT('Ctrl Pts',(129.804965611462,4.24137151037132,125.232188524482));
#260018=CARTESIAN_POINT('Ctrl Pts',(129.526517987649,-2.39546129141071,
124.224079519825));
#260019=CARTESIAN_POINT('Ctrl Pts',(129.248070363836,-6.83098219117618,
129.262927379388));
#260020=CARTESIAN_POINT('Ctrl Pts',(128.969622740024,-4.98916416928312,
135.718277081636));
#260021=CARTESIAN_POINT('Ctrl Pts',(128.691175116211,1.43745198996158,137.657977611568));
#260022=CARTESIAN_POINT('Ctrl Pts',(128.412727492398,6.54311999386511,133.299538941816));
#260023=CARTESIAN_POINT('Ctrl Pts',(128.134279868585,5.63598037258881,126.648153288314));
#260024=CARTESIAN_POINT('Ctrl Pts',(127.855832244772,-0.450349878148651,
123.81611912838));
#260025=CARTESIAN_POINT('Ctrl Pts',(127.577384620959,-6.12283059168226,
127.40593750243));
#260026=CARTESIAN_POINT('Ctrl Pts',(127.298936997146,-6.16872910836309,
134.118740697091));
#260027=CARTESIAN_POINT('Ctrl Pts',(127.020489373333,-0.545866933628919,
137.785790515136));
#260028=CARTESIAN_POINT('Ctrl Pts',(126.742041749521,5.57862028602806,135.037247319125));
#260029=CARTESIAN_POINT('Ctrl Pts',(126.463594125708,6.57662799357718,128.398888032392));
#260030=CARTESIAN_POINT('Ctrl Pts',(126.185146501895,1.53103586116759,123.971040537565));
#260031=CARTESIAN_POINT('Ctrl Pts',(125.906698878082,-4.92150343239493,
125.822680370014));
#260032=CARTESIAN_POINT('Ctrl Pts',(125.628251254269,-6.85142150039552,
132.252240981353));
#260033=CARTESIAN_POINT('Ctrl Pts',(125.349803630456,-2.48521792008072,
137.351270271259));
#260034=CARTESIAN_POINT('Ctrl Pts',(125.071356006643,4.16477951914341,136.434009423738));
#260035=CARTESIAN_POINT('Ctrl Pts',(124.79290838283,6.98754804106521,130.343376346978));
#260036=CARTESIAN_POINT('Ctrl Pts',(124.514460759018,3.38910127394743,124.676365294554));
#260037=CARTESIAN_POINT('Ctrl Pts',(124.236013135205,-3.32376399712637,
124.640682574762));
#260038=CARTESIAN_POINT('Ctrl Pts',(123.957565511392,-6.98225252973936,
130.269118863895));
#260039=CARTESIAN_POINT('Ctrl Pts',(123.679117887579,-4.22439208952083,
136.389416176637));
#260040=CARTESIAN_POINT('Ctrl Pts',(123.400670263766,2.41547830794073,137.377320275725));
#260041=CARTESIAN_POINT('Ctrl Pts',(123.122222639953,6.83564214308024,132.324995555895));
#260042=CARTESIAN_POINT('Ctrl Pts',(122.84377501614,4.97418478841272,125.875281614887));
#260043=CARTESIAN_POINT('Ctrl Pts',(122.565327392328,-1.45830538437,123.955150478444));
#260044=CARTESIAN_POINT('Ctrl Pts',(122.286879768514,-6.55068415109515,
128.329108857337));
#260045=CARTESIAN_POINT('Ctrl Pts',(122.008432144702,-5.62330420167569,
134.977702681109));
#260046=CARTESIAN_POINT('Ctrl Pts',(121.729984520888,0.471617595401148,
137.791199027578));
#260047=CARTESIAN_POINT('Ctrl Pts',(121.451536897076,6.13314586210485,134.184132201278));
#260048=CARTESIAN_POINT('Ctrl Pts',(121.173089273263,6.15861270236637,127.471220400567));
#260049=CARTESIAN_POINT('Ctrl Pts',(120.89464164945,0.52461533410983,123.821301626325));
#260050=CARTESIAN_POINT('Ctrl Pts',(120.616194025637,-5.5914778973097,126.588472923636));
#260051=CARTESIAN_POINT('Ctrl Pts',(120.337746401824,-6.56927609998288,
133.229839054105));
#260052=CARTESIAN_POINT('Ctrl Pts',(120.059298778011,-1.51023049375061,
137.642308992603));
#260053=CARTESIAN_POINT('Ctrl Pts',(119.780851154198,4.93664315737715,135.77103842679));
#260054=CARTESIAN_POINT('Ctrl Pts',(119.502403530385,6.84698291530094,129.33563359));
#260055=CARTESIAN_POINT('Ctrl Pts',(119.223955906573,2.46527986777437,124.249917140239));
#260056=CARTESIAN_POINT('Ctrl Pts',(118.94550828276,-4.18189494262004,125.187414043775));
#260057=CARTESIAN_POINT('Ctrl Pts',(118.667060658947,-6.98611259767199,
131.28661044553));
#260058=CARTESIAN_POINT('Ctrl Pts',(118.388613035134,-3.37043406603744,
136.942642814599));
#260059=CARTESIAN_POINT('Ctrl Pts',(118.110165411321,3.34250871742766,136.95789371635));
#260060=CARTESIAN_POINT('Ctrl Pts',(117.831717787508,6.98384928020556,131.318348317123));
#260061=CARTESIAN_POINT('Ctrl Pts',(117.553270163695,4.20737353447909,125.206473331696));
#260062=CARTESIAN_POINT('Ctrl Pts',(117.274822539882,-2.43547294780967,
124.238783289987));
#260063=CARTESIAN_POINT('Ctrl Pts',(116.99637491607,-6.84023877052931,129.304538066038));
#260064=CARTESIAN_POINT('Ctrl Pts',(116.717927292256,-4.95915932737393,
135.748556496538));
#260065=CARTESIAN_POINT('Ctrl Pts',(116.439479668444,1.47914526923655,137.649100451659));
#260066=CARTESIAN_POINT('Ctrl Pts',(116.161032044631,6.55818762368211,133.259662883379));
#260067=CARTESIAN_POINT('Ctrl Pts',(115.882584420818,5.61057593724064,126.613922481));
#260068=CARTESIAN_POINT('Ctrl Pts',(115.604136797005,-0.49288094365267,
123.818990011842));
#260069=CARTESIAN_POINT('Ctrl Pts',(115.325689173192,-6.14340431590201,
127.443271875017));
#260070=CARTESIAN_POINT('Ctrl Pts',(115.047241549379,-6.14843924382291,
134.156230094282));
#260071=CARTESIAN_POINT('Ctrl Pts',(114.768793925566,-0.5033588746261,137.78898401237));
#260072=CARTESIAN_POINT('Ctrl Pts',(114.490346301753,5.60428370990391,135.003210248456));
#260073=CARTESIAN_POINT('Ctrl Pts',(114.211898677941,6.56186334951224,128.358898798961));
#260074=CARTESIAN_POINT('Ctrl Pts',(113.933451054127,1.48941113576461,123.961847293312));
#260075=CARTESIAN_POINT('Ctrl Pts',(113.655003430315,-4.95173714997151,
125.852731257293));
#260076=CARTESIAN_POINT('Ctrl Pts',(113.376555806502,-6.84248090069202,
132.293920702821));
#260077=CARTESIAN_POINT('Ctrl Pts',(113.098108182689,-2.4453189774521,137.366277199056));
#260078=CARTESIAN_POINT('Ctrl Pts',(112.819660558876,4.19897162559319,136.408552924347));
#260079=CARTESIAN_POINT('Ctrl Pts',(112.541212935063,6.98461243588604,130.300849699721));
#260080=CARTESIAN_POINT('Ctrl Pts',(112.26276531125,3.35173563488669,124.655848410718));
#260081=CARTESIAN_POINT('Ctrl Pts',(111.984317687437,-3.3612224731848,124.661029468288));
#260082=CARTESIAN_POINT('Ctrl Pts',(111.705870063624,-6.98538133324609,
130.311631733633));
#260083=CARTESIAN_POINT('Ctrl Pts',(111.427422439812,-4.1903160029037,136.415027772168));
#260084=CARTESIAN_POINT('Ctrl Pts',(111.148974815999,2.45544502578993,137.362494791951));
#260085=CARTESIAN_POINT('Ctrl Pts',(110.870527192186,6.84477203094083,132.28335688814));
#260086=CARTESIAN_POINT('Ctrl Pts',(110.592079568373,4.94408792536061,125.845093664656));
#260087=CARTESIAN_POINT('Ctrl Pts',(110.31363194456,-1.49997145150339,123.964154497236));
#260088=CARTESIAN_POINT('Ctrl Pts',(110.035184320747,-6.56563034211481,
128.369030591753));
#260089=CARTESIAN_POINT('Ctrl Pts',(109.756736696934,-5.59779569719655,
135.011856007506));
#260090=CARTESIAN_POINT('Ctrl Pts',(109.478289073121,0.514139725922464,
137.788198707481));
#260091=CARTESIAN_POINT('Ctrl Pts',(109.199841449309,6.15360585804082,134.146735382281));
#260092=CARTESIAN_POINT('Ctrl Pts',(108.921393825496,6.13820882697821,127.433792932393));
#260093=CARTESIAN_POINT('Ctrl Pts',(108.642946201683,0.482097752094529,
123.818237523792));
#260094=CARTESIAN_POINT('Ctrl Pts',(108.36449857787,-5.61703760517944,126.622587947283));
#260095=CARTESIAN_POINT('Ctrl Pts',(108.086050954057,-6.5543898108359,133.26978316381));
#260096=CARTESIAN_POINT('Ctrl Pts',(107.807603330244,-1.46857798007734,
137.651375502926));
#260097=CARTESIAN_POINT('Ctrl Pts',(107.529155706431,4.96678527034939,135.740895657668));
#260098=CARTESIAN_POINT('Ctrl Pts',(107.250708082618,6.83791549827476,129.2939812737));
#260099=CARTESIAN_POINT('Ctrl Pts',(106.972260458805,2.42533543402888,124.23503172061));
#260100=CARTESIAN_POINT('Ctrl Pts',(106.693812834992,-4.21600940986681,
125.212974494265));
#260101=CARTESIAN_POINT('Ctrl Pts',(106.415365211179,-6.98304756960462,
131.329127960835));
#260102=CARTESIAN_POINT('Ctrl Pts',(106.136917587367,-3.33300615371489,
136.96304587525));
#260103=CARTESIAN_POINT('Ctrl Pts',(105.858469963554,3.37990509103613,136.937432906355));
#260104=CARTESIAN_POINT('Ctrl Pts',(105.580022339741,6.98684867466819,131.275826121299));
#260105=CARTESIAN_POINT('Ctrl Pts',(105.301574715928,4.1732196528133,125.180965570684));
#260106=CARTESIAN_POINT('Ctrl Pts',(105.023127092115,-2.4753943568629,124.253730350031));
#260107=CARTESIAN_POINT('Ctrl Pts',(104.744679468302,-6.84924188231931,
129.346204329164));
#260108=CARTESIAN_POINT('Ctrl Pts',(104.466231844489,-4.92897072199215,
135.778652702442));
#260109=CARTESIAN_POINT('Ctrl Pts',(104.187784220676,1.52078373823962,137.639969657397));
#260110=CARTESIAN_POINT('Ctrl Pts',(103.909336596864,6.57301223744494,133.219695842813));
#260111=CARTESIAN_POINT('Ctrl Pts',(103.63088897305,5.58496359993783,126.579846951912));
#260112=CARTESIAN_POINT('Ctrl Pts',(103.352441349238,-0.535393745272065,
123.82211974078));
#260113=CARTESIAN_POINT('Ctrl Pts',(103.073993725425,-6.1637503940156,127.480730793984));
#260114=CARTESIAN_POINT('Ctrl Pts',(102.795546101612,-6.12792154660547,
134.193595286717));
#260115=CARTESIAN_POINT('Ctrl Pts',(102.517098477799,-0.460832163475232,
137.791918691816));
#260116=CARTESIAN_POINT('Ctrl Pts',(102.238650853986,5.6297394649859,134.96901758787));
#260117=CARTESIAN_POINT('Ctrl Pts',(101.960203230173,6.54685555318778,128.319000183017));
#260118=CARTESIAN_POINT('Ctrl Pts',(101.68175560636,1.44773121968427,123.952907600908));
#260119=CARTESIAN_POINT('Ctrl Pts',(101.403307982548,-4.981787379107,125.882965629019));
#260120=CARTESIAN_POINT('Ctrl Pts',(101.124860358735,-6.83328675034245,
132.335545228093));
#260121=CARTESIAN_POINT('Ctrl Pts',(100.846412734922,-2.4053294226295,137.38104097262));
#260122=CARTESIAN_POINT('Ctrl Pts',(100.567965111109,4.23300813760519,136.382888759548));
#260123=CARTESIAN_POINT('Ctrl Pts',(100.289517487296,6.98141801332452,130.258341710245));
#260124=CARTESIAN_POINT('Ctrl Pts',(100.011069863483,3.31424579602927,124.635559362262));
#260125=CARTESIAN_POINT('Ctrl Pts',(99.7326222396699,-3.39855639790849,
124.681604005209));
#260126=CARTESIAN_POINT('Ctrl Pts',(99.4541746158571,-6.98825129087862,
130.354162861621));
#260127=CARTESIAN_POINT('Ctrl Pts',(99.1757269920442,-4.15608464258612,
136.440431462363));
#260128=CARTESIAN_POINT('Ctrl Pts',(98.8972793682313,2.49532075622072,137.347426294104));
#260129=CARTESIAN_POINT('Ctrl Pts',(98.6188317444184,6.85364828325664,132.241663415635));
#260130=CARTESIAN_POINT('Ctrl Pts',(98.3403841206056,4.91380785731226,125.815089481885));
#260131=CARTESIAN_POINT('Ctrl Pts',(98.0619364967926,-1.54158193664305,
123.97341198238));
#260132=CARTESIAN_POINT('Ctrl Pts',(97.7834888729798,-6.58033324128762,
128.409042568218));
#260133=CARTESIAN_POINT('Ctrl Pts',(97.5050412491668,-5.57207976433927,
135.045853423614));
#260134=CARTESIAN_POINT('Ctrl Pts',(97.226593625354,0.55664280480716,137.784939598694));
#260135=CARTESIAN_POINT('Ctrl Pts',(96.948146001541,6.17383782984873,134.109214710358));
#260136=CARTESIAN_POINT('Ctrl Pts',(96.6696983777281,6.11757749800464,127.396490361844));
#260137=CARTESIAN_POINT('Ctrl Pts',(96.3912507539153,0.43956230576973,123.815432294619));
#260138=CARTESIAN_POINT('Ctrl Pts',(96.1128031301024,-5.64238917165504,
126.656857928054));
#260139=CARTESIAN_POINT('Ctrl Pts',(95.8343555062895,-6.53926064636413,
133.309635916377));
#260140=CARTESIAN_POINT('Ctrl Pts',(95.5559078824767,-1.42687104770695,
137.660188294596));
#260141=CARTESIAN_POINT('Ctrl Pts',(95.2774602586637,4.99674333726689,135.710569963425));
#260142=CARTESIAN_POINT('Ctrl Pts',(94.9990126348508,6.82859469977515,129.252384925061));
#260143=CARTESIAN_POINT('Ctrl Pts',(94.720565011038,2.38530112858694,124.22038972988));
#260144=CARTESIAN_POINT('Ctrl Pts',(94.442117387225,-4.24996765133445,125.238742135624));
#260145=CARTESIAN_POINT('Ctrl Pts',(94.1636697634123,-6.97972378214161,
131.371626030693));
#260146=CARTESIAN_POINT('Ctrl Pts',(93.885222139599,-3.29545473562348,136.983220723554));
#260147=CARTESIAN_POINT('Ctrl Pts',(93.6067745157866,3.41717622101856,136.91674483311));
#260148=CARTESIAN_POINT('Ctrl Pts',(93.3283268919733,6.98958916888377,131.233286455149));
#260149=CARTESIAN_POINT('Ctrl Pts',(93.0498792681607,4.13891113095855,125.155666186642));
#260150=CARTESIAN_POINT('Ctrl Pts',(92.7714316443476,-2.51522403926791,
124.268920146089));
#260151=CARTESIAN_POINT('Ctrl Pts',(92.4929840205349,-6.85799119293255,
129.387924624807));
#260152=CARTESIAN_POINT('Ctrl Pts',(92.2145363967218,-4.89859947178764,
135.808564584124));
#260153=CARTESIAN_POINT('Ctrl Pts',(91.9360887729091,1.562365854042,137.63058556713));
#260154=CARTESIAN_POINT('Ctrl Pts',(91.6576411490961,6.58759328582208,133.179639301113));
#260155=CARTESIAN_POINT('Ctrl Pts',(91.3791935252832,5.55914430975498,126.545927963732));
#260156=CARTESIAN_POINT('Ctrl Pts',(91.1007459014705,-0.57788670767935,
123.825508199223));
#260157=CARTESIAN_POINT('Ctrl Pts',(90.8222982776573,-6.18386807209161,
127.518312871276));
#260158=CARTESIAN_POINT('Ctrl Pts',(90.5438506538447,-6.10717677700159,
134.230834889814));
#260159=CARTESIAN_POINT('Ctrl Pts',(90.2654030300316,-0.41828837601907,
137.794594444728));
#260160=CARTESIAN_POINT('Ctrl Pts',(89.9869554062187,5.65498660800168,134.934670604388));
#260161=CARTESIAN_POINT('Ctrl Pts',(89.708507782406,6.53160516072318,128.279193663018));
#260162=CARTESIAN_POINT('Ctrl Pts',(89.430060158593,1.40599765739116,123.944221791613));
#260163=CARTESIAN_POINT('Ctrl Pts',(89.1516125347801,-5.01165300627911,
125.913382364846));
#260164=CARTESIAN_POINT('Ctrl Pts',(88.8731649109673,-6.82383939003939,
132.377113014756));
#260165=CARTESIAN_POINT('Ctrl Pts',(88.5947172871542,-2.36525073744058,
137.395561044874));
#260166=CARTESIAN_POINT('Ctrl Pts',(88.3162696633415,4.26688779394398,136.357017880338));
#260167=CARTESIAN_POINT('Ctrl Pts',(88.0378220395285,6.97796489175107,130.2158539537));
#260168=CARTESIAN_POINT('Ctrl Pts',(87.7593744157156,3.2766331465752,124.615498901007));
#260169=CARTESIAN_POINT('Ctrl Pts',(87.4809267919028,-3.43576438787495,
124.702405423128));
#260170=CARTESIAN_POINT('Ctrl Pts',(87.2024791680898,-6.99086229628967,
130.396710671853));
#260171=CARTESIAN_POINT('Ctrl Pts',(86.924031544277,-4.1216992770237,136.465626305881));
#260172=CARTESIAN_POINT('Ctrl Pts',(86.6455839204641,2.53510402162323,137.332115340552));
#260173=CARTESIAN_POINT('Ctrl Pts',(86.3671362966513,6.8622705711149,132.199916683345));
#260174=CARTESIAN_POINT('Ctrl Pts',(86.0886886728382,4.88334570630671,125.785270178391));
#260175=CARTESIAN_POINT('Ctrl Pts',(85.8102410490255,-1.58313529789712,
123.982922590838));
#260176=CARTESIAN_POINT('Ctrl Pts',(85.5317934252125,-6.59479230379227,
128.449143304076));
#260177=CARTESIAN_POINT('Ctrl Pts',(85.2533458013996,-5.5461573560172,135.079693669646));
#260178=CARTESIAN_POINT('Ctrl Pts',(84.9748981775869,0.599125257088023,
137.781421821987));
#260179=CARTESIAN_POINT('Ctrl Pts',(84.6964505537737,6.19384102782544,134.071571575853));
#260180=CARTESIAN_POINT('Ctrl Pts',(84.418002929961,6.09671947994716,127.359314071181));
#260181=CARTESIAN_POINT('Ctrl Pts',(84.1395553061481,0.397010571302045,
123.812886042756));
#260182=CARTESIAN_POINT('Ctrl Pts',(83.8611076823352,-5.66753165732491,
126.691281596061));
#260183=CARTESIAN_POINT('Ctrl Pts',(83.5826600585222,-6.52388916718428,
133.349395835046));
#260184=CARTESIAN_POINT('Ctrl Pts',(83.3042124347095,-1.38511124210516,
137.66874704105));
#260185=CARTESIAN_POINT('Ctrl Pts',(83.0257648108964,5.02651624802251,135.68006246779));
#260186=CARTESIAN_POINT('Ctrl Pts',(82.7473171870836,6.81902086518772,129.210846085452));
#260187=CARTESIAN_POINT('Ctrl Pts',(82.4688695632707,2.34517843493451,124.205991710613));
#260188=CARTESIAN_POINT('Ctrl Pts',(82.1904219394578,-4.28376840868787,
125.264716013022));
#260189=CARTESIAN_POINT('Ctrl Pts',(81.9119743156449,-6.97614135844701,
131.414103080323));
#260190=CARTESIAN_POINT('Ctrl Pts',(81.6335266918322,-3.25778120324508,
137.003166611925));
#260191=CARTESIAN_POINT('Ctrl Pts',(81.355079068019,3.45432072627939,136.895830263219));
#260192=CARTESIAN_POINT('Ctrl Pts',(81.0766314442065,6.99207066130227,131.190730894994));
#260193=CARTESIAN_POINT('Ctrl Pts',(80.7981838203932,4.10444924022979,125.130576117049));
#260194=CARTESIAN_POINT('Ctrl Pts',(80.5197361965806,-2.55496051912119,
124.284352115297));
#260195=CARTESIAN_POINT('Ctrl Pts',(80.2412885727675,-6.86648637816013,
129.429697407007));
#260196=CARTESIAN_POINT('Ctrl Pts',(79.9628409489547,-4.86804670217826,
135.838291033188));
#260197=CARTESIAN_POINT('Ctrl Pts',(79.6843933251418,1.6038900758031,137.620948528586));
#260198=CARTESIAN_POINT('Ctrl Pts',(79.405945701329,6.60193022850756,133.139494742587));
#260199=CARTESIAN_POINT('Ctrl Pts',(79.1274980775159,5.53311902343524,126.512166773338));
#260200=CARTESIAN_POINT('Ctrl Pts',(78.8490504537032,-0.620358256282274,
123.829155261608));
#260201=CARTESIAN_POINT('Ctrl Pts',(78.5706028298902,-6.2037566046621,127.556016714277));
#260202=CARTESIAN_POINT('Ctrl Pts',(78.2921552060774,-6.08620570371632,
134.267947523646));
#260203=CARTESIAN_POINT('Ctrl Pts',(78.0137075822645,-0.375729088733312,
137.797011171955));
#260204=CARTESIAN_POINT('Ctrl Pts',(77.7352599584516,5.68002420340909,134.90017057075));
#260205=CARTESIAN_POINT('Ctrl Pts',(77.4568123346387,6.51611273722737,128.23948071401));
#260206=CARTESIAN_POINT('Ctrl Pts',(77.1783647108257,1.36421199533782,123.935790187287));
#260207=CARTESIAN_POINT('Ctrl Pts',(76.8999170870129,-5.04133292480603,
125.94398033767));
#260208=CARTESIAN_POINT('Ctrl Pts',(76.6214694632,-6.81413916985829,132.418622522501));
#260209=CARTESIAN_POINT('Ctrl Pts',(76.3430218393871,-2.32508440701577,
137.409836877774));
#260210=CARTESIAN_POINT('Ctrl Pts',(76.0645742155741,4.30060933918641,136.33094124537));
#260211=CARTESIAN_POINT('Ctrl Pts',(75.7861265917614,6.97425319912241,130.173388004487));
#260212=CARTESIAN_POINT('Ctrl Pts',(75.5076789679483,3.23889908027492,124.595667770297));
#260213=CARTESIAN_POINT('Ctrl Pts',(75.2292313441357,-3.47284506432852,
124.72343295124));
#260214=CARTESIAN_POINT('Ctrl Pts',(74.9507837203226,-6.99321425272744,
130.439273587703));
#260215=CARTESIAN_POINT('Ctrl Pts',(74.6723360965098,-4.08716118037883,
136.490611369118));
#260216=CARTESIAN_POINT('Ctrl Pts',(74.3938884726969,2.57479334781394,137.316562498648));
#260217=CARTESIAN_POINT('Ctrl Pts',(74.1154408488841,6.87063857501356,132.158118238212));
#260218=CARTESIAN_POINT('Ctrl Pts',(73.836993225071,4.85270260113016,125.755636859138));
#260219=CARTESIAN_POINT('Ctrl Pts',(73.5585456012583,-1.62462999549052,
123.992685970191));
#260220=CARTESIAN_POINT('Ctrl Pts',(73.2800979774453,-6.60900699384299,
128.489331313375));
#260221=CARTESIAN_POINT('Ctrl Pts',(73.0016503536324,-5.52002943279461,
135.113375491641));
#260222=CARTESIAN_POINT('Ctrl Pts',(72.7232027298196,0.641585508562261,
137.777645507711));
#260223=CARTESIAN_POINT('Ctrl Pts',(72.4447551060067,6.21361471074508,134.033807373642));
#260224=CARTESIAN_POINT('Ctrl Pts',(72.1663074821937,6.07563554570727,127.322265437984));
#260225=CARTESIAN_POINT('Ctrl Pts',(71.8878598583809,0.354444125461637,
123.810598862555));
#260226=CARTESIAN_POINT('Ctrl Pts',(71.609412234568,-5.69246413052499,126.725857675724));
#260227=CARTESIAN_POINT('Ctrl Pts',(71.330964610755,-6.5082759428922,133.3890614465));
#260228=CARTESIAN_POINT('Ctrl Pts',(71.0525169869423,-1.34330011069692,
137.677051425141));
#260229=CARTESIAN_POINT('Ctrl Pts',(70.7740693631292,5.05610289937005,135.649374301231));
#260230=CARTESIAN_POINT('Ctrl Pts',(70.4956217393166,6.80919434927445,129.16936629411));
#260231=CARTESIAN_POINT('Ctrl Pts',(70.2171741155033,2.30496883983272,124.191838196331));
#260232=CARTESIAN_POINT('Ctrl Pts',(69.9387264916908,-4.31741042942741,
125.290895163988));
#260233=CARTESIAN_POINT('Ctrl Pts',(69.6602788678776,-6.97230043126892,
131.456557535721));
#260234=CARTESIAN_POINT('Ctrl Pts',(69.3818312440649,-3.21998695258627,
137.02288280126));
#260235=CARTESIAN_POINT('Ctrl Pts',(69.1033836202519,3.49133723041524,136.874689971681));
#260236=CARTESIAN_POINT('Ctrl Pts',(68.8249359964391,6.9942930599711,131.148161017746));
#260237=CARTESIAN_POINT('Ctrl Pts',(68.5464883726262,4.0698352576252,125.105696291628));
#260238=CARTESIAN_POINT('Ctrl Pts',(68.2680407488133,-2.59460232397255,
124.300025685817));
#260239=CARTESIAN_POINT('Ctrl Pts',(67.9895931250004,-6.87472712320984,
129.471521127857));
#260240=CARTESIAN_POINT('Ctrl Pts',(67.7111455011875,-4.83731354530826,
135.867830948109));
#260241=CARTESIAN_POINT('Ctrl Pts',(67.4326978773747,1.64535486482719,137.61105889887));
#260242=CARTESIAN_POINT('Ctrl Pts',(67.1542502535617,6.61602253424027,133.099263654809));
#260243=CARTESIAN_POINT('Ctrl Pts',(66.8758026297489,5.50688870535577,126.478564631767));
#260244=CARTESIAN_POINT('Ctrl Pts',(66.5973550059358,-0.662806817281494,
123.833060792792));
#260245=CARTESIAN_POINT('Ctrl Pts',(66.3189073821232,-6.22341525475008,
127.593840925854));
#260246=CARTESIAN_POINT('Ctrl Pts',(66.0404597583101,-6.0650091038406,134.304931812993));
#260247=CARTESIAN_POINT('Ctrl Pts',(65.7620121344974,-0.333155878668442,
137.799168783944));
#260248=CARTESIAN_POINT('Ctrl Pts',(65.4835645106842,5.70485132343066,134.865518765369));
#260249=CARTESIAN_POINT('Ctrl Pts',(65.2051168868716,6.50037885677781,128.199862807569));
#260250=CARTESIAN_POINT('Ctrl Pts',(64.9266692630585,1.32237578190785,123.927613100363));
#260251=CARTESIAN_POINT('Ctrl Pts',(64.6482216392459,-5.07082603488719,
125.974758413674));
#260252=CARTESIAN_POINT('Ctrl Pts',(64.3697740154327,-6.80418644924447,
132.460072213177));
#260253=CARTESIAN_POINT('Ctrl Pts',(64.09132639162,-2.28483191973344,137.423867942321));
#260254=CARTESIAN_POINT('Ctrl Pts',(63.812878767807,4.33417152376786,136.304659820925));
#260255=CARTESIAN_POINT('Ctrl Pts',(63.5344311439942,6.97028307297671,130.130945436197));
#260256=CARTESIAN_POINT('Ctrl Pts',(63.2559835201813,3.20104499537862,124.576066704985));
#260257=CARTESIAN_POINT('Ctrl Pts',(62.9775358963684,-3.5097970532309,124.744685810362));
#260258=CARTESIAN_POINT('Ctrl Pts',(62.6990882725555,-6.9953070730393,130.481850031987));
#260259=CARTESIAN_POINT('Ctrl Pts',(62.4206406487427,-4.05247163247362,
136.51538572624));
#260260=CARTESIAN_POINT('Ctrl Pts',(62.1421930249296,2.61438726408988,137.300768344709));
#260261=CARTESIAN_POINT('Ctrl Pts',(61.8637454011169,6.87875198487314,132.116269629093));
#260262=CARTESIAN_POINT('Ctrl Pts',(61.5852977773038,4.82187967727427,125.726190622201));
#260263=CARTESIAN_POINT('Ctrl Pts',(61.3068501534911,-1.66606449182178,
124.002701758653));
#260264=CARTESIAN_POINT('Ctrl Pts',(61.0284025296781,-6.62297678470872,
128.529605106938));
#260265=CARTESIAN_POINT('Ctrl Pts',(60.7499549058653,-5.49369696285183,
135.146897641504));
#260266=CARTESIAN_POINT('Ctrl Pts',(60.4715072820523,0.684021985849089,
137.773610795799));
#260267=CARTESIAN_POINT('Ctrl Pts',(60.1930596582395,6.23315814588628,133.995923503096));
#260268=CARTESIAN_POINT('Ctrl Pts',(59.9146120344266,6.05432647655821,127.285345835106));
#260269=CARTESIAN_POINT('Ctrl Pts',(59.6361644106137,0.311864545564345,
123.808570838767));
#260270=CARTESIAN_POINT('Ctrl Pts',(59.3577167868007,-5.71718566737322,
126.760584885814));
#260271=CARTESIAN_POINT('Ctrl Pts',(59.0792691629879,-6.49242155204172,
133.428631280914));
#260272=CARTESIAN_POINT('Ctrl Pts',(58.800821539175,-1.30143920280946,137.685101139145));
#260273=CARTESIAN_POINT('Ctrl Pts',(58.5223739153621,5.08550219496502,135.618506600908));
#260274=CARTESIAN_POINT('Ctrl Pts',(58.2439262915492,6.79911551616065,129.127947088084));
#260275=CARTESIAN_POINT('Ctrl Pts',(57.9654786677363,2.26467383326308,124.1779297115));
#260276=CARTESIAN_POINT('Ctrl Pts',(57.6870310439234,-4.35089246693584,
125.317278618444));
#260277=CARTESIAN_POINT('Ctrl Pts',(57.4085834201106,-6.96820114293417,
131.498987823723));
#260278=CARTESIAN_POINT('Ctrl Pts',(57.1301357962976,-3.18207338412696,
137.042368560968));
#260279=CARTESIAN_POINT('Ctrl Pts',(56.8516881724848,3.52822436176609,136.853324741857));
#260280=CARTESIAN_POINT('Ctrl Pts',(56.5732405486719,6.9962562825383,131.105578400848));
#260281=CARTESIAN_POINT('Ctrl Pts',(56.294792924859,4.03507046577855,125.081027632309));
#260282=CARTESIAN_POINT('Ctrl Pts',(56.0163453010462,-2.63414798488075,
124.315940276861));
#260283=CARTESIAN_POINT('Ctrl Pts',(55.7378976772331,-6.8827131227178,129.513394237565));
#260284=CARTESIAN_POINT('Ctrl Pts',(55.4594500534204,-4.80640114000575,
135.897183234276));
#260285=CARTESIAN_POINT('Ctrl Pts',(55.1810024296073,1.68675868462211,137.600917044446));
#260286=CARTESIAN_POINT('Ctrl Pts',(54.9025548057946,6.62986968082513,133.058947528554));
#260287=CARTESIAN_POINT('Ctrl Pts',(54.6241071819816,5.4804543274898,126.445122784157));
#260288=CARTESIAN_POINT('Ctrl Pts',(54.3456595581689,-0.705230817730614,
123.837224648055));
#260289=CARTESIAN_POINT('Ctrl Pts',(54.0672119343557,-6.24284329389726,
127.63178410442));
#260290=CARTESIAN_POINT('Ctrl Pts',(53.7887643105431,-6.04358776282204,
134.341786387386));
#260291=CARTESIAN_POINT('Ctrl Pts',(53.51031668673,-0.290570323389535,137.801067200743));
#260292=CARTESIAN_POINT('Ctrl Pts',(53.2318690629172,5.72946704808866,134.830716472279));
#260293=CARTESIAN_POINT('Ctrl Pts',(52.9534214391043,6.48440410239917,128.160341411752));
#260294=CARTESIAN_POINT('Ctrl Pts',(52.6749738152913,1.28049056735643,123.919690833848));
#260295=CARTESIAN_POINT('Ctrl Pts',(52.3965261914786,-5.10013124364513,
126.005715452363));
#260296=CARTESIAN_POINT('Ctrl Pts',(52.1180785676656,-6.79398159699943,
132.501460550851));
#260297=CARTESIAN_POINT('Ctrl Pts',(51.8396309438527,-2.24449476716385,
137.43765371859));
#260298=CARTESIAN_POINT('Ctrl Pts',(51.5611833200399,4.36757310402998,136.278174580871));
#260299=CARTESIAN_POINT('Ctrl Pts',(51.2827356962269,6.96605466042841,130.088527821552));
#260300=CARTESIAN_POINT('Ctrl Pts',(51.0042880724141,3.16307229458231,124.556696431394));
#260301=CARTESIAN_POINT('Ctrl Pts',(50.7258404486012,-3.54661898531293,
124.766163212963));
#260302=CARTESIAN_POINT('Ctrl Pts',(50.4473928247883,-6.99714067967511,
130.52443842702));
#260303=CARTESIAN_POINT('Ctrl Pts',(50.1689452009753,-4.0176319187415,136.539948459229));
#260304=CARTESIAN_POINT('Ctrl Pts',(49.8904975771625,2.65388430328469,137.284733463992));
#260305=CARTESIAN_POINT('Ctrl Pts',(49.6120499533496,6.88661050004828,132.074372406703));
#260306=CARTESIAN_POINT('Ctrl Pts',(49.3336023295367,4.79087807689359,125.696932558722));
#260307=CARTESIAN_POINT('Ctrl Pts',(49.0551547057238,-1.7074372515208,124.012969585086));
#260308=CARTESIAN_POINT('Ctrl Pts',(48.776707081911,-6.63670115873435,128.569963192402));
#260309=CARTESIAN_POINT('Ctrl Pts',(48.498259458098,-5.46716092194746,135.180258877061));
#260310=CARTESIAN_POINT('Ctrl Pts',(48.2198118342852,0.72643311645002,137.769317835757));
#260311=CARTESIAN_POINT('Ctrl Pts',(47.9413642104722,6.25247060906043,133.957921368012));
#260312=CARTESIAN_POINT('Ctrl Pts',(47.6629165866595,6.03279306211481,127.248556630613));
#260313=CARTESIAN_POINT('Ctrl Pts',(47.3844689628464,0.269273409411107,
123.806802046542));
#260314=CARTESIAN_POINT('Ctrl Pts',(47.1060213390337,-5.74169535180415,
126.7954619395));
#260315=CARTESIAN_POINT('Ctrl Pts',(46.8275737152206,-6.47632658212296,
133.468103872012));
#260316=CARTESIAN_POINT('Ctrl Pts',(46.5491260914079,-1.25953006961336,
137.69289588478));
#260317=CARTESIAN_POINT('Ctrl Pts',(46.2706784675948,5.11471304540623,135.587460510634));
#260318=CARTESIAN_POINT('Ctrl Pts',(45.9922308437821,6.78878473932087,129.086590002178));
#260319=CARTESIAN_POINT('Ctrl Pts',(45.7137832199691,2.22429490837156,124.164266771503));
#260320=CARTESIAN_POINT('Ctrl Pts',(45.4353355961562,-4.38421328052394,
125.343865398741));
#260321=CARTESIAN_POINT('Ctrl Pts',(45.1568879723434,-6.96384364534361,
131.541392372057));
#260322=CARTESIAN_POINT('Ctrl Pts',(44.8784403485304,-3.1440419027679,137.061623168999));
#260323=CARTESIAN_POINT('Ctrl Pts',(44.5999927247176,3.56498075346585,136.831735365442));
#260324=CARTESIAN_POINT('Ctrl Pts',(44.3215451009046,6.99796025625624,131.062984622213));
#260325=CARTESIAN_POINT('Ctrl Pts',(44.0430974770918,4.00015615291162,125.056571053198));
#260326=CARTESIAN_POINT('Ctrl Pts',(43.7646498532789,-2.67359603646683,
124.332095298706));
#260327=CARTESIAN_POINT('Ctrl Pts',(43.486202229466,-6.8904440807599,129.555315184507));
#260328=CARTESIAN_POINT('Ctrl Pts',(43.2077546056531,-4.77531063174146,
135.926346804027));
#260329=CARTESIAN_POINT('Ctrl Pts',(42.9293069818402,1.72810000095366,137.590523341125));
#260330=CARTESIAN_POINT('Ctrl Pts',(42.6508593580274,6.64347115515083,133.018547857752));
#260331=CARTESIAN_POINT('Ctrl Pts',(42.3724117342144,5.4538168693733,126.411842469708));
#260332=CARTESIAN_POINT('Ctrl Pts',(42.0939641104015,-0.74762868559244,
123.841646673103));
#260333=CARTESIAN_POINT('Ctrl Pts',(41.8155164865887,-6.26204000219037,
127.669844843974));
#260334=CARTESIAN_POINT('Ctrl Pts',(41.5370688627757,-6.02194247443641,
134.378509881167));
#260335=CARTESIAN_POINT('Ctrl Pts',(41.2586212389629,-0.247974000920424,
137.802706352008));
#260336=CARTESIAN_POINT('Ctrl Pts',(40.9801736151499,5.75387046523817,134.795764981093));
#260337=CARTESIAN_POINT('Ctrl Pts',(40.7017259913371,6.46818906604193,128.120917991039));
#260338=CARTESIAN_POINT('Ctrl Pts',(40.4232783675241,1.23855790375582,123.912023681303));
#260339=CARTESIAN_POINT('Ctrl Pts',(40.1448307437113,-5.12924746516435,
126.036850306614));
#260340=CARTESIAN_POINT('Ctrl Pts',(39.8663831198984,-6.78352499126783,
132.542786001862));
#260341=CARTESIAN_POINT('Ctrl Pts',(39.5879354960856,-2.20407444401526,
137.451193695743));
#260342=CARTESIAN_POINT('Ctrl Pts',(39.3094878722726,4.40081284226458,136.251486506627));
#260343=CARTESIAN_POINT('Ctrl Pts',(39.0310402484598,6.96156811816289,130.046136732356));
#260344=CARTESIAN_POINT('Ctrl Pts',(38.7525926246468,3.12498238497894,124.537557667297));
#260345=CARTESIAN_POINT('Ctrl Pts',(38.474145000834,-3.58330949612422,124.78786436319));
#260346=CARTESIAN_POINT('Ctrl Pts',(38.195697377021,-6.9987150046898,130.567037194673));
#260347=CARTESIAN_POINT('Ctrl Pts',(37.9172497532082,-3.98264333018119,
136.564298657899));
#260348=CARTESIAN_POINT('Ctrl Pts',(37.6388021293952,2.69328300182069,137.268458450676));
#260349=CARTESIAN_POINT('Ctrl Pts',(37.3603545055824,6.89421382933879,132.032428123559));
#260350=CARTESIAN_POINT('Ctrl Pts',(37.0819068817695,4.7596989487639,125.667863752866));
#260351=CARTESIAN_POINT('Ctrl Pts',(36.8034592579566,-1.74874674150458,
124.02348906901));
#260352=CARTESIAN_POINT('Ctrl Pts',(36.5250116341437,-6.65017960735793,
128.610404074285));
#260353=CARTESIAN_POINT('Ctrl Pts',(36.2465640103308,-5.44042229338459,
135.213457962098));
#260354=CARTESIAN_POINT('Ctrl Pts',(35.968116386518,0.768817328804687,137.764766786667));
#260355=CARTESIAN_POINT('Ctrl Pts',(35.689668762705,6.27155138463682,133.919802376575));
#260356=CARTESIAN_POINT('Ctrl Pts',(35.4112211388921,6.01103610030595,127.211899187745));
#260357=CARTESIAN_POINT('Ctrl Pts',(35.1327735150793,0.226672295232647,
123.805292551423));
#260358=CARTESIAN_POINT('Ctrl Pts',(34.8543258912663,-5.76599227560232,
126.830487544402));
#260359=CARTESIAN_POINT('Ctrl Pts',(34.5758782674535,-6.45999162954105,
133.507477757125));
#260360=CARTESIAN_POINT('Ctrl Pts',(34.2974306436406,-1.21757426406734,
137.700435373207));
#260361=CARTESIAN_POINT('Ctrl Pts',(34.0189830198277,5.1437343682746,135.556237180835));
#260362=CARTESIAN_POINT('Ctrl Pts',(33.7405353960148,6.778202401566,129.045296568894));
#260363=CARTESIAN_POINT('Ctrl Pts',(33.4620877722019,2.18383356141425,124.150849882625));
#260364=CARTESIAN_POINT('Ctrl Pts',(33.1836401483891,-4.41737163547663,
125.370654519698));
#260365=CARTESIAN_POINT('Ctrl Pts',(32.9051925245761,-6.95922809996586,
131.58376960941));
#260366=CARTESIAN_POINT('Ctrl Pts',(32.6267449007632,-3.10589391777991,
137.080645911863));
#260367=CARTESIAN_POINT('Ctrl Pts',(32.3482972769504,3.60160504349277,136.80992264244));
#260368=CARTESIAN_POINT('Ctrl Pts',(32.0698496531375,6.99940491798352,131.020381260171));
#260369=CARTESIAN_POINT('Ctrl Pts',(31.7914020293246,3.96509361278713,125.032327460544));
#260370=CARTESIAN_POINT('Ctrl Pts',(31.5129544055117,-2.71294501696876,
124.348490152723));
#260371=CARTESIAN_POINT('Ctrl Pts',(31.2345067816988,-6.89791971086261,
129.597282415287));
#260372=CARTESIAN_POINT('Ctrl Pts',(30.9560591578859,-4.74404317258561,
135.955320576696));
#260373=CARTESIAN_POINT('Ctrl Pts',(30.677611534073,1.76937728190418,137.579878174048));
#260374=CARTESIAN_POINT('Ctrl Pts',(30.3991639102601,6.65682645320975,132.978066139427));
#260375=CARTESIAN_POINT('Ctrl Pts',(30.1207162864473,5.42697731806706,126.378724921634));
#260376=CARTESIAN_POINT('Ctrl Pts',(29.8422686626343,-0.789998849798377,
123.846326704078));
#260377=CARTESIAN_POINT('Ctrl Pts',(29.5638210388214,-6.28100466828836,
127.708021734164));
#260378=CARTESIAN_POINT('Ctrl Pts',(29.2853734150086,-6.00007404075783,
134.415100933532));
#260379=CARTESIAN_POINT('Ctrl Pts',(29.0069257911957,-0.205368489683527,
137.804086176998));
#260380=CARTESIAN_POINT('Ctrl Pts',(28.7284781673828,5.77806067060162,134.760665586949));
#260381=CARTESIAN_POINT('Ctrl Pts',(28.4500305435699,6.45173434856014,128.08159400628));
#260382=CARTESIAN_POINT('Ctrl Pts',(28.171582919757,1.19657934493693,123.904611926838));
#260383=CARTESIAN_POINT('Ctrl Pts',(27.8931352959441,-5.15817362053239,
126.068161822712));
#260384=CARTESIAN_POINT('Ctrl Pts',(27.6146876721312,-6.77281701952304,
132.584047034882));
#260385=CARTESIAN_POINT('Ctrl Pts',(27.3362400483183,-2.16357244807759,
137.464487372053));
#260386=CARTESIAN_POINT('Ctrl Pts',(27.0577924245054,4.4338895067609,136.22459658713));
#260387=CARTESIAN_POINT('Ctrl Pts',(26.7793448006925,6.95682361243065,130.003773739425));
#260388=CARTESIAN_POINT('Ctrl Pts',(26.5008971768797,3.08677667800406,124.518651121888));
#260389=CARTESIAN_POINT('Ctrl Pts',(26.2224495530668,-3.61986722608435,
124.809788456898));
#260390=CARTESIAN_POINT('Ctrl Pts',(25.9440019292538,-7.00002998974624,
130.609644756432));
#260391=CARTESIAN_POINT('Ctrl Pts',(25.665554305441,-3.94750716330764,136.588435419948));
#260392=CARTESIAN_POINT('Ctrl Pts',(25.3871066816281,2.7325818997646,137.251943907838));
#260393=CARTESIAN_POINT('Ctrl Pts',(25.1086590578152,6.90156169100052,131.990438333922));
#260394=CARTESIAN_POINT('Ctrl Pts',(24.8302114340022,4.72834344823931,125.638985281792));
#260395=CARTESIAN_POINT('Ctrl Pts',(24.5517638101894,-1.78999143103474,
124.034259820624));
#260396=CARTESIAN_POINT('Ctrl Pts',(24.2733161863765,-6.66341163113055,
128.650926254035));
#260397=CARTESIAN_POINT('Ctrl Pts',(23.9948685625636,-5.41348206797292,
135.246493666413));
#260398=CARTESIAN_POINT('Ctrl Pts',(23.7164209387507,0.811173052350488,
137.759957817164));
#260399=CARTESIAN_POINT('Ctrl Pts',(23.4379733149379,6.29039976557031,133.881567941299));
#260400=CARTESIAN_POINT('Ctrl Pts',(23.159525691125,5.98905639734383,127.175374864857));
#260401=CARTESIAN_POINT('Ctrl Pts',(22.8810780673121,0.184062781628937,
123.804042409345));
#260402=CARTESIAN_POINT('Ctrl Pts',(22.6026304434992,-5.79007553843628,
126.865660402631));
#260403=CARTESIAN_POINT('Ctrl Pts',(22.3241828196863,-6.44341729959363,
133.546751477239));
#260404=CARTESIAN_POINT('Ctrl Pts',(22.0457351958734,-1.17557334085921,
137.707719325048));
#260405=CARTESIAN_POINT('Ctrl Pts',(21.7672875720605,5.17256508817436,135.524837768503));
#260406=CARTESIAN_POINT('Ctrl Pts',(21.4888399482477,6.76736889502847,129.004068318375));
#260407=CARTESIAN_POINT('Ctrl Pts',(21.2103923244347,2.14329129170119,124.137679542035));
#260408=CARTESIAN_POINT('Ctrl Pts',(20.9319447006219,-4.45036630309889,
125.397644988631));
#260409=CARTESIAN_POINT('Ctrl Pts',(20.6534970768089,-6.95435467783159,
131.626117965476));
#260410=CARTESIAN_POINT('Ctrl Pts',(20.3750494529961,-3.06763084275059,
137.099436084669));
#260411=CARTESIAN_POINT('Ctrl Pts',(20.0966018291831,3.6380958747203,136.787887381128));
#260412=CARTESIAN_POINT('Ctrl Pts',(19.8181542053702,7.00059021418742,130.977769893405));
#260413=CARTESIAN_POINT('Ctrl Pts',(19.5397065815574,3.92988414466092,125.0082977527));
#260414=CARTESIAN_POINT('Ctrl Pts',(19.2612589577445,-2.75219346829522,
124.365124231394));
#260415=CARTESIAN_POINT('Ctrl Pts',(18.9828113339316,-6.90513973601376,
129.639294374793));
#260416=CARTESIAN_POINT('Ctrl Pts',(18.7043637101187,-4.71259992116536,
135.98410347865));
#260417=CARTESIAN_POINT('Ctrl Pts',(18.4259160863058,1.81058899792882,137.568981937677));
#260418=CARTESIAN_POINT('Ctrl Pts',(18.1474684624929,6.6699350801164,132.937503873645));
#260419=CARTESIAN_POINT('Ctrl Pts',(17.86902083868,5.39993666812053,126.345771367118));
#260420=CARTESIAN_POINT('Ctrl Pts',(17.5905732148672,-0.832339740306418,
123.851264567558));
#260421=CARTESIAN_POINT('Ctrl Pts',(17.3121255910542,-6.29973658944851,
127.746313360329));
#260422=CARTESIAN_POINT('Ctrl Pts',(17.0336779672413,-5.97798327212915,
134.451558188587));
#260423=CARTESIAN_POINT('Ctrl Pts',(16.7552303434285,-0.162755368441711,
137.805206624583));
#260424=CARTESIAN_POINT('Ctrl Pts',(16.4767827196156,5.80203676780203,134.72541959047));
#260425=CARTESIAN_POINT('Ctrl Pts',(16.1983350958026,6.43504055968944,128.042370914639));
#260426=CARTESIAN_POINT('Ctrl Pts',(15.9198874719898,1.15455644643036,123.897455845098));
#260427=CARTESIAN_POINT('Ctrl Pts',(15.6414398481769,-5.18690863788001,
126.0996488404));
#260428=CARTESIAN_POINT('Ctrl Pts',(15.362992224364,-6.7618580785529,132.625242120967));
#260429=CARTESIAN_POINT('Ctrl Pts',(15.0845446005511,-2.12299028016722,
137.477534254917));
#260430=CARTESIAN_POINT('Ctrl Pts',(14.8060969767383,4.466801871851,136.197505818795));
#260431=CARTESIAN_POINT('Ctrl Pts',(14.5276493529253,6.95182131904109,129.961440412534));
#260432=CARTESIAN_POINT('Ctrl Pts',(14.2492017291125,3.04845658938423,124.499977495755));
#260433=CARTESIAN_POINT('Ctrl Pts',(13.9707541052995,-3.65629082053323,
124.831934681683));
#260434=CARTESIAN_POINT('Ctrl Pts',(13.6923064814867,-7.00108558611715,
130.652259533458));
#260435=CARTESIAN_POINT('Ctrl Pts',(13.4138588576738,-3.91222472010448,
136.612357850978));
#260436=CARTESIAN_POINT('Ctrl Pts',(13.1354112338608,2.77177954088132,137.23519044743));
#260437=CARTESIAN_POINT('Ctrl Pts',(12.856963610048,6.90865381275575,131.94840459374));
#260438=CARTESIAN_POINT('Ctrl Pts',(12.5785159862351,4.6968127372094,125.6102982156));
#260439=CARTESIAN_POINT('Ctrl Pts',(12.3000683624222,-1.83116979177416,
124.045281440813));
#260440=CARTESIAN_POINT('Ctrl Pts',(12.0216207386093,-6.67639673973472,
128.691528230086));
#260441=CARTESIAN_POINT('Ctrl Pts',(11.7431731147965,-5.38634124399241,
135.279364765853));
#260442=CARTESIAN_POINT('Ctrl Pts',(11.4647254909835,0.853498717580522,
137.75489110545));
#260443=CARTESIAN_POINT('Ctrl Pts',(11.1862778671706,6.30901505342741,133.843219478972));
#260444=CARTESIAN_POINT('Ctrl Pts',(10.9078302433578,5.96685476769427,127.13898501537));
#260445=CARTESIAN_POINT('Ctrl Pts',(10.6293826195448,0.141446447510913,
123.803051666633));
#260446=CARTESIAN_POINT('Ctrl Pts',(10.350934995732,-5.81394424789186,126.900979210845));
#260447=CARTESIAN_POINT('Ctrl Pts',(10.0724873719191,-6.42660420644864,
133.585923577051));
#260448=CARTESIAN_POINT('Ctrl Pts',(9.79403974810624,-1.1335288563486,137.714747470394));
#260449=CARTESIAN_POINT('Ctrl Pts',(9.51559212429333,5.20120413677258,135.493263437154));
#260450=CARTESIAN_POINT('Ctrl Pts',(9.23714450048043,6.75628462114785,128.962906778349));
#260451=CARTESIAN_POINT('Ctrl Pts',(8.95869687666756,2.10266960154115,124.124756237763));
#260452=CARTESIAN_POINT('Ctrl Pts',(8.68024925285465,-4.48319606076117,
125.4248358054));
#260453=CARTESIAN_POINT('Ctrl Pts',(8.40180162904178,-6.94922355952728,
131.66843587102));
#260454=CARTESIAN_POINT('Ctrl Pts',(8.12335400522884,-3.0292540955323,137.117992991138));
#260455=CARTESIAN_POINT('Ctrl Pts',(7.84490638141603,3.67445189496732,136.765630398031));
#260456=CARTESIAN_POINT('Ctrl Pts',(7.56645875760307,7.00151610094645,130.935152100895));
#260457=CARTESIAN_POINT('Ctrl Pts',(7.2880111337902,3.89452905323253,124.984482820099));
#260458=CARTESIAN_POINT('Ctrl Pts',(7.00956350997733,-2.79133993608059,
124.381996918337));
#260459=CARTESIAN_POINT('Ctrl Pts',(6.73111588616443,-6.91210388867261,
129.681349506257));
#260460=CARTESIAN_POINT('Ctrl Pts',(6.45266826235151,-4.68098204262199,
136.012694443327));
#260461=CARTESIAN_POINT('Ctrl Pts',(6.17422063853866,1.85173362191231,137.557835035774));
#260462=CARTESIAN_POINT('Ctrl Pts',(5.89577301472578,6.68279655012581,132.896862563455));
#260463=CARTESIAN_POINT('Ctrl Pts',(5.61732539091285,5.37269592153495,126.312983027266));
#260464=CARTESIAN_POINT('Ctrl Pts',(5.33887776709996,-0.874649788159289,
123.856460080569));
#260465=CARTESIAN_POINT('Ctrl Pts',(5.06043014328709,-6.31823507155263,
127.784718303561));
#260466=CARTESIAN_POINT('Ctrl Pts',(4.7819825194742,-5.95567098713191,134.487880295395));
#260467=CARTESIAN_POINT('Ctrl Pts',(4.50353489566127,-0.120136216239877,
137.806067653244));
#260468=CARTESIAN_POINT('Ctrl Pts',(4.22508727184843,5.82579786839633,134.690028297709));
#260469=CARTESIAN_POINT('Ctrl Pts',(3.94663964803551,6.41810831802433,128.003250169541));
#260470=CARTESIAN_POINT('Ctrl Pts',(3.66819202422262,1.11249076541009,123.890555701254));
#260471=CARTESIAN_POINT('Ctrl Pts',(3.3897444004097,-5.21545145242058,126.131310192911));
#260472=CARTESIAN_POINT('Ctrl Pts',(3.11129677659686,-6.75064857444498,
132.666369733619));
#260473=CARTESIAN_POINT('Ctrl Pts',(2.83284915278395,-2.08232944407128,
137.490333860877));
#260474=CARTESIAN_POINT('Ctrl Pts',(2.55440152897106,4.49954871795507,136.170215205482));
#260475=CARTESIAN_POINT('Ctrl Pts',(2.27595390515816,6.94656142335602,129.919138320362));
#260476=CARTESIAN_POINT('Ctrl Pts',(1.9975062813453,3.01002353908442,124.481537480858));
#260477=CARTESIAN_POINT('Ctrl Pts',(1.71905865753238,-3.69257892978116,
124.854302216906));
#260478=CARTESIAN_POINT('Ctrl Pts',(1.44061103371947,-7.00188175468703,
130.694879946647));
#260479=CARTESIAN_POINT('Ctrl Pts',(1.16216340990662,-3.87679730797559,
136.636065064534));
#260480=CARTESIAN_POINT('Ctrl Pts',(0.883715786093727,2.81087447268782,
137.218198690258));
#260481=CARTESIAN_POINT('Ctrl Pts',(0.605268162280799,6.91548993180329,
131.906328460586));
#260482=CARTESIAN_POINT('Ctrl Pts',(0.326820538467947,4.66510798405627,
125.5818036173));
#260483=CARTESIAN_POINT('Ctrl Pts',(0.0483729146550416,-1.87228029784353,
124.056553521165));
#260484=CARTESIAN_POINT('Ctrl Pts',(-0.23007470915786,-6.68913445200245,
128.732208497919));
#260485=CARTESIAN_POINT('Ctrl Pts',(-0.508522332970751,-5.35900082715629,
135.312070042369));
#260486=CARTESIAN_POINT('Ctrl Pts',(-0.786969956783612,0.895792756101716,
137.749566839272));
#260487=CARTESIAN_POINT('Ctrl Pts',(-1.06541758059653,6.32739655841135,
133.804758410613));
#260488=CARTESIAN_POINT('Ctrl Pts',(-1.34386520440944,5.94443203404716,
127.102730987725));
#260489=CARTESIAN_POINT('Ctrl Pts',(-1.62231282822229,0.0988248720430084,
123.802320359999));
#260490=CARTESIAN_POINT('Ctrl Pts',(-1.90076045203519,-5.83759751950527,
126.936442660293));
#260491=CARTESIAN_POINT('Ctrl Pts',(-2.17920807584809,-6.40955297312139,
133.624992605024));
#260492=CARTESIAN_POINT('Ctrl Pts',(-2.45765569966099,-1.09144236850938,
137.721519548813));
#260493=CARTESIAN_POINT('Ctrl Pts',(-2.73610332347384,5.22965045283876,
135.461515356786));
#260494=CARTESIAN_POINT('Ctrl Pts',(-3.01455094728676,6.74494999065597,
128.921813474073));
#260495=CARTESIAN_POINT('Ctrl Pts',(-3.29299857109967,2.06196999618574,
124.112080448687));
#260496=CARTESIAN_POINT('Ctrl Pts',(-3.57144619491253,-4.51585969194472,
125.452225962441));
#260497=CARTESIAN_POINT('Ctrl Pts',(-3.84989381872542,-6.94383493518842,
131.710721757939));
#260498=CARTESIAN_POINT('Ctrl Pts',(-4.12834144253832,-2.99076509818949,
137.136315943637));
#260499=CARTESIAN_POINT('Ctrl Pts',(-4.40678906635123,3.71067175704807,
136.743152517891));
#260500=CARTESIAN_POINT('Ctrl Pts',(-4.68523669016409,7.00218254395157,
130.892529461858));
#260501=CARTESIAN_POINT('Ctrl Pts',(-4.963684313977,3.85902964859785,124.960883545208));
#260502=CARTESIAN_POINT('Ctrl Pts',(-5.24213193778992,-2.83038296973812,
124.399107588329));
#260503=CARTESIAN_POINT('Ctrl Pts',(-5.52057956160276,-6.91881191077996,
129.723446251312));
#260504=CARTESIAN_POINT('Ctrl Pts',(-5.79902718541567,-4.6491907085676,
136.041092411279));
#260505=CARTESIAN_POINT('Ctrl Pts',(-6.07747480922856,1.89280962922548,
137.546437881394));
#260506=CARTESIAN_POINT('Ctrl Pts',(-6.35592243304147,6.69541038665145,
132.856143714835));
#260507=CARTESIAN_POINT('Ctrl Pts',(-6.63437005685431,5.34525608772619,
126.280361117063));
#260508=CARTESIAN_POINT('Ctrl Pts',(-6.91281768066725,-0.916927425542613,
123.86191305059));
#260509=CARTESIAN_POINT('Ctrl Pts',(-7.19126530448013,-6.33649942913263,
127.823235140749));
#260510=CARTESIAN_POINT('Ctrl Pts',(-7.469712928293,-5.93313801255607,134.524065908027));
#260511=CARTESIAN_POINT('Ctrl Pts',(-7.74816055210589,-0.0775126123463511,
137.806669231077));
#260512=CARTESIAN_POINT('Ctrl Pts',(-8.02660817591882,5.84934309190818,
134.654493020103));
#260513=CARTESIAN_POINT('Ctrl Pts',(-8.3050557997317,6.40093825099524,127.964233220621));
#260514=CARTESIAN_POINT('Ctrl Pts',(-8.58350342354456,1.07038386063539,
123.883911750995));
#260515=CARTESIAN_POINT('Ctrl Pts',(-8.86195104735747,-5.2438010064896,
126.163144707024));
#260516=CARTESIAN_POINT('Ctrl Pts',(-9.14039867117038,-6.73918892257159,
132.707428348838));
#260517=CARTESIAN_POINT('Ctrl Pts',(-9.41884629498326,-2.04159144649203,
137.50288571564));
#260518=CARTESIAN_POINT('Ctrl Pts',(-9.69729391879612,4.53212883162697,
136.142725758454));
#260519=CARTESIAN_POINT('Ctrl Pts',(-9.97574154260907,6.94104412028278,
129.876869030427));
#260520=CARTESIAN_POINT('Ctrl Pts',(-10.254189166422,2.97147895125515,124.463331760497));
#260521=CARTESIAN_POINT('Ctrl Pts',(-10.5326367902348,-3.72873020915888,
124.876890233732));
#260522=CARTESIAN_POINT('Ctrl Pts',(-10.8110844140478,-7.00241846595355,
130.737504416682));
#260523=CARTESIAN_POINT('Ctrl Pts',(-11.0895320378606,-3.84122623969676,
136.659556182137));
#260524=CARTESIAN_POINT('Ctrl Pts',(-11.3679796616735,2.84986524650705,
137.200969265957));
#260525=CARTESIAN_POINT('Ctrl Pts',(-11.6464272854864,6.92206979482823,
131.864211493609));
#260526=CARTESIAN_POINT('Ctrl Pts',(-11.9248749092993,4.6332303636112,125.553502542771));
#260527=CARTESIAN_POINT('Ctrl Pts',(-12.2033225331122,-1.91332142587795,
124.068075643991));
#260528=CARTESIAN_POINT('Ctrl Pts',(-12.4817701569251,-6.70162429593314,
128.77296555011));
#260529=CARTESIAN_POINT('Ctrl Pts',(-12.760217780738,-5.33146183057377,
135.344608284054));
#260530=CARTESIAN_POINT('Ctrl Pts',(-13.0386654045509,0.938053600692905,
137.743985215925));
#260531=CARTESIAN_POINT('Ctrl Pts',(-13.3171130283637,6.34554359938892,
133.766186161411));
#260532=CARTESIAN_POINT('Ctrl Pts',(-13.5955606521767,5.92178902728497,
127.066614125326));
#260533=CARTESIAN_POINT('Ctrl Pts',(-13.8740082759896,0.0561996345831295,
123.801848516541));
#260534=CARTESIAN_POINT('Ctrl Pts',(-14.1524558998025,-5.86103447679583,
126.972049436864));
#260535=CARTESIAN_POINT('Ctrl Pts',(-14.4309035236153,-6.39226423145161,
133.663957113442));
#260536=CARTESIAN_POINT('Ctrl Pts',(-14.7093511474282,-1.04931543687181,
137.728035309365));
#260537=CARTESIAN_POINT('Ctrl Pts',(-14.9877987712411,5.25790298228423,
135.429594703837));
#260538=CARTESIAN_POINT('Ctrl Pts',(-15.266246395054,6.73336542356173,128.880789928272));
#260539=CARTESIAN_POINT('Ctrl Pts',(-15.5446940188669,2.02119398377386,
124.099652644515));
#260540=CARTESIAN_POINT('Ctrl Pts',(-15.8231416426798,-4.54835598628669,
125.479814444798));
#260541=CARTESIAN_POINT('Ctrl Pts',(-16.1015892664927,-6.93818900449243,
131.752974059312));
#260542=CARTESIAN_POINT('Ctrl Pts',(-16.3800368903055,-2.95216527694612,
137.154404263204));
#260543=CARTESIAN_POINT('Ctrl Pts',(-16.6584845141185,3.74675411882228,
136.720454573632));
#260544=CARTESIAN_POINT('Ctrl Pts',(-16.9369321379314,7.00258951850748,
130.849903555692));
#260545=CARTESIAN_POINT('Ctrl Pts',(-17.2153797617442,3.82338724620039,
124.93750080251));
#260546=CARTESIAN_POINT('Ctrl Pts',(-17.4938273855571,-2.86932112251383,
124.416455607327));
#260547=CARTESIAN_POINT('Ctrl Pts',(-17.77227500937,-6.92526355376757,129.765583050046));
#260548=CARTESIAN_POINT('Ctrl Pts',(-18.0507226331829,-4.61722709704176,
136.069296330209));
#260549=CARTESIAN_POINT('Ctrl Pts',(-18.3291702569958,1.93381549778173,
137.534790896862));
#260550=CARTESIAN_POINT('Ctrl Pts',(-18.6076178808087,6.70777612228299,
132.81534883664));
#260551=CARTESIAN_POINT('Ctrl Pts',(-18.8860655046216,5.31761818348739,
126.247906845325));
#260552=CARTESIAN_POINT('Ctrl Pts',(-19.1645131284344,-0.959171085842972,
123.867623275557));
#260553=CARTESIAN_POINT('Ctrl Pts',(-19.4429607522474,-6.35452898539608,
127.861862444637));
#260554=CARTESIAN_POINT('Ctrl Pts',(-19.7214083760603,-5.91038518336925,
134.560113685611));
#260555=CARTESIAN_POINT('Ctrl Pts',(-19.9998559998732,-0.0348861361944895,
137.807011335788));
#260556=CARTESIAN_POINT('Ctrl Pts',(-20.278303623686,5.87267156586067,134.618815074426));
#260557=CARTESIAN_POINT('Ctrl Pts',(-20.5567512474989,6.38353099484532,
127.925321513668));
#260558=CARTESIAN_POINT('Ctrl Pts',(-20.8351988713118,1.02823729239309,
123.877524240513));
#260559=CARTESIAN_POINT('Ctrl Pts',(-21.1136464951247,-5.27195624958391,
126.1951512031));
#260560=CARTESIAN_POINT('Ctrl Pts',(-21.3920941189376,-6.72747954757436,
132.748416445183));
#260561=CARTESIAN_POINT('Ctrl Pts',(-21.6705417427505,-2.00077779699093,
137.515189354092));
#260562=CARTESIAN_POINT('Ctrl Pts',(-21.9489893665634,4.56454100559805,
136.115038496344));
#260563=CARTESIAN_POINT('Ctrl Pts',(-22.2274369903762,6.93526961426714,
129.834634109035));
#260564=CARTESIAN_POINT('Ctrl Pts',(-22.5058846141892,2.93282425418085,
124.445361009293));
#260565=CARTESIAN_POINT('Ctrl Pts',(-22.784332238002,-3.76474331906749,
124.899697895151));
#260566=CARTESIAN_POINT('Ctrl Pts',(-23.062779861815,-7.0026957000287,130.780131364099));
#260567=CARTESIAN_POINT('Ctrl Pts',(-23.3412274856278,-3.80551283336702,
136.682830333316));
#260568=CARTESIAN_POINT('Ctrl Pts',(-23.6196751094408,2.88875041752152,
137.183502812971));
#260569=CARTESIAN_POINT('Ctrl Pts',(-23.8981227332536,6.92839315801137,
131.822055253468));
#260570=CARTESIAN_POINT('Ctrl Pts',(-24.1765703570665,4.60118105711114,
125.525396040718));
#260571=CARTESIAN_POINT('Ctrl Pts',(-24.4550179808794,-1.95429165508329,
124.079847382335));
#260572=CARTESIAN_POINT('Ctrl Pts',(-24.7334656046923,-6.71386580871103,
128.813797876394));
#260573=CARTESIAN_POINT('Ctrl Pts',(-25.0119132285052,-5.30372527471246,
135.376978285193));
#260574=CARTESIAN_POINT('Ctrl Pts',(-25.290360852318,0.980279685362951,
137.738146442235));
#260575=CARTESIAN_POINT('Ctrl Pts',(-25.568808476131,6.36345550391485,133.727504160674));
#260576=CARTESIAN_POINT('Ctrl Pts',(-25.8472560999438,5.89892658645264,
127.030635766497));
#260577=CARTESIAN_POINT('Ctrl Pts',(-26.1257037237567,0.0135723146251221,
123.801636153745));
#260578=CARTESIAN_POINT('Ctrl Pts',(-26.4041513475696,-5.88425425129846,
127.007798221134));
#260579=CARTESIAN_POINT('Ctrl Pts',(-26.6825989713826,-6.37473862207999,
133.70281565846));
#260580=CARTESIAN_POINT('Ctrl Pts',(-26.9610465951954,-1.00714962246484,
137.734294510605));
#260581=CARTESIAN_POINT('Ctrl Pts',(-27.2394942190083,5.28596067820108,
135.397502661138));
#260582=CARTESIAN_POINT('Ctrl Pts',(-27.5179418428212,6.72153134913555,
128.839837661092));
#260583=CARTESIAN_POINT('Ctrl Pts',(-27.7963894666341,1.98034307527561,
124.087473285763));
#260584=CARTESIAN_POINT('Ctrl Pts',(-28.0748370904469,-4.58068373962494,
125.507600230172));
#260585=CARTESIAN_POINT('Ctrl Pts',(-28.3532847142599,-6.93228597665136,
131.795191209466));
#260586=CARTESIAN_POINT('Ctrl Pts',(-28.6317323380727,-2.91345606213275,
137.172257279568));
#260587=CARTESIAN_POINT('Ctrl Pts',(-28.9101799618857,3.78269764324474,
136.697537406337));
#260588=CARTESIAN_POINT('Ctrl Pts',(-29.1886275856985,7.00273700953358,
130.807275961916));
#260589=CARTESIAN_POINT('Ctrl Pts',(-29.4670752095115,3.78760316678249,
124.914335458459));
#260590=CARTESIAN_POINT('Ctrl Pts',(-29.7455228333243,-2.90815295154017,
124.434040332496));
#260591=CARTESIAN_POINT('Ctrl Pts',(-30.0239704571372,-6.93145857856742,
129.807758341064));
#260592=CARTESIAN_POINT('Ctrl Pts',(-30.3024180809501,-4.5850923924679,
136.097305155009));
#260593=CARTESIAN_POINT('Ctrl Pts',(-30.580865704763,1.97474970809384,137.52289451376));
#260594=CARTESIAN_POINT('Ctrl Pts',(-30.8593133285759,6.71989329880362,
132.774479440534));
#260595=CARTESIAN_POINT('Ctrl Pts',(-31.1377609523888,5.28978323295099,
126.215621414657));
#260596=CARTESIAN_POINT('Ctrl Pts',(-31.4162085762017,-1.00137920370602,
123.873590543879));
#260597=CARTESIAN_POINT('Ctrl Pts',(-31.6946562000146,-6.37232307225107,
127.900598783877));
#260598=CARTESIAN_POINT('Ctrl Pts',(-31.9731038238274,-5.88741334268594,
134.596022292384));
#260599=CARTESIAN_POINT('Ctrl Pts',(-32.2515514476404,0.00774163267598956,
137.807093954702));
#260600=CARTESIAN_POINT('Ctrl Pts',(-32.5299990714533,5.89578242580862,
134.582995782735));
#260601=CARTESIAN_POINT('Ctrl Pts',(-32.8084466952661,6.36588719460685,
127.886516490566));
#260602=CARTESIAN_POINT('Ctrl Pts',(-33.086894319079,0.9860526224398,123.8713934065));
#260603=CARTESIAN_POINT('Ctrl Pts',(-33.365341942892,-5.29991613840065,
126.227328495126));
#260604=CARTESIAN_POINT('Ctrl Pts',(-33.6437895667048,-6.71552088334846,
132.789332503824));
#260605=CARTESIAN_POINT('Ctrl Pts',(-33.9222371905177,-1.95989000793276,
137.527244320318));
#260606=CARTESIAN_POINT('Ctrl Pts',(-34.2006848143306,4.59678403882356,
136.08715444511));
#260607=CARTESIAN_POINT('Ctrl Pts',(-34.4791324381435,6.9292381192855,129.792435121214));
#260608=CARTESIAN_POINT('Ctrl Pts',(-34.7575800619564,2.89406088022529,
124.427625893158));
#260609=CARTESIAN_POINT('Ctrl Pts',(-35.0360276857693,-3.80061692502793,
124.922724356021));
#260610=CARTESIAN_POINT('Ctrl Pts',(-35.3144753095821,-7.00271344663942,
130.822759209339));
#260611=CARTESIAN_POINT('Ctrl Pts',(-35.592922933395,-3.76965841235978,
136.705886655638));
#260612=CARTESIAN_POINT('Ctrl Pts',(-35.8713705572079,2.92752854482695,
137.165799978524));
#260613=CARTESIAN_POINT('Ctrl Pts',(-36.1498181810209,6.9344597870381,131.779861302279));
#260614=CARTESIAN_POINT('Ctrl Pts',(-36.4282658048337,4.56896125215494,
125.49748515264));
#260615=CARTESIAN_POINT('Ctrl Pts',(-36.7067134286466,-1.99518946729269,
124.091868299989));
#260616=CARTESIAN_POINT('Ctrl Pts',(-36.9851610524595,-6.72585853672236,
128.854703963711));
#260617=CARTESIAN_POINT('Ctrl Pts',(-37.2636086762724,-5.27579218736066,
135.409178846303));
#260618=CARTESIAN_POINT('Ctrl Pts',(-37.5420563000852,1.02246944540875,
137.732050734562));
#260619=CARTESIAN_POINT('Ctrl Pts',(-37.8205039238982,6.38113160825695,
133.688713841779));
#260620=CARTESIAN_POINT('Ctrl Pts',(-38.0989515477111,5.87584555872632,
126.994797244432));
#260621=CARTESIAN_POINT('Ctrl Pts',(-38.377399171524,-0.0290555082599903,
123.801683279478));
#260622=CARTESIAN_POINT('Ctrl Pts',(-38.6558467953367,-5.90725598259587,
127.04368768842));
#260623=CARTESIAN_POINT('Ctrl Pts',(-38.9342944191497,-6.35697679442443,
133.741566800161));
#260624=CARTESIAN_POINT('Ctrl Pts',(-39.2127420429625,-0.964946487758246,
137.740296920595));
#260625=CARTESIAN_POINT('Ctrl Pts',(-39.4911896667755,5.31382250090111,
135.365240417872));
#260626=CARTESIAN_POINT('Ctrl Pts',(-39.7696372905882,6.70944820589337,
128.798958190032));
#260627=CARTESIAN_POINT('Ctrl Pts',(-40.0480849144012,1.93941878443644,
124.07554282374));
#260628=CARTESIAN_POINT('Ctrl Pts',(-40.3265325382142,-4.61284175404266,
125.535582288951));
#260629=CARTESIAN_POINT('Ctrl Pts',(-40.604980162027,-6.9261260704041,131.837371644027));
#260630=CARTESIAN_POINT('Ctrl Pts',(-40.8834277858398,-2.87463888813357,
137.18987433118));
#260631=CARTESIAN_POINT('Ctrl Pts',(-41.1618754096529,3.81850099841496,
136.674401865208));
#260632=CARTESIAN_POINT('Ctrl Pts',(-41.4403230334656,7.00262501156454,
130.76464826011));
#260633=CARTESIAN_POINT('Ctrl Pts',(-41.7187706572786,3.75167873633635,
124.891388371457));
#260634=CARTESIAN_POINT('Ctrl Pts',(-41.9972182810916,-2.94687701788942,
124.451861112224));
#260635=CARTESIAN_POINT('Ctrl Pts',(-42.2756659049044,-6.93739675562063,
129.849970561546));
#260636=CARTESIAN_POINT('Ctrl Pts',(-42.5541135287174,-4.55278778560923,
136.125117847804));
#260637=CARTESIAN_POINT('Ctrl Pts',(-42.8325611525302,2.01561074332903,
137.510749172913));
#260638=CARTESIAN_POINT('Ctrl Pts',(-43.1110087763431,6.73176146720674,
132.733537040953));
#260639=CARTESIAN_POINT('Ctrl Pts',(-43.389456400156,5.26175226755184,126.183506021407));
#260640=CARTESIAN_POINT('Ctrl Pts',(-43.6679040239687,-1.0435502150944,
123.879814634434));
#260641=CARTESIAN_POINT('Ctrl Pts',(-43.9463516477818,-6.38988103033122,
127.93944272308));
#260642=CARTESIAN_POINT('Ctrl Pts',(-44.2247992715946,-5.86422334173611,
134.631790397739));
#260643=CARTESIAN_POINT('Ctrl Pts',(-44.5032468954075,0.050369114677416,
137.806917084757));
#260644=CARTESIAN_POINT('Ctrl Pts',(-44.7816945192204,5.91867481537061,
134.547036472328));
#260645=CARTESIAN_POINT('Ctrl Pts',(-45.0601421430334,6.34800750407734,
127.847819589252));
#260646=CARTESIAN_POINT('Ctrl Pts',(-45.3385897668461,0.943831413943965,
123.865519476137));
#260647=CARTESIAN_POINT('Ctrl Pts',(-45.6170373906592,-5.32767963687585,
126.25967539076));
#260648=CARTESIAN_POINT('Ctrl Pts',(-45.895485014472,-6.7033133730266,132.830175008601));
#260649=CARTESIAN_POINT('Ctrl Pts',(-46.1739326382849,-1.91892959442962,
137.539050167615));
#260650=CARTESIAN_POINT('Ctrl Pts',(-46.4523802620978,4.62885673652604,
136.059074638009));
#260651=CARTESIAN_POINT('Ctrl Pts',(-46.7308278859106,6.92294985883713,
129.750273630666));
#260652=CARTESIAN_POINT('Ctrl Pts',(-47.0092755097235,2.8551902657795,124.410127069272));
#260653=CARTESIAN_POINT('Ctrl Pts',(-47.2877231335364,-3.83634969773052,
124.945968763085));
#260654=CARTESIAN_POINT('Ctrl Pts',(-47.5661707573492,-7.00247170512816,
130.865386372813));
#260655=CARTESIAN_POINT('Ctrl Pts',(-47.8446183811622,-3.73366430527375,
136.728724294741));
#260656=CARTESIAN_POINT('Ctrl Pts',(-48.123066004975,2.96619819148554,137.147861418602));
#260657=CARTESIAN_POINT('Ctrl Pts',(-48.4015136287881,6.9402694571073,131.737631203552));
#260658=CARTESIAN_POINT('Ctrl Pts',(-48.6799612526008,4.53657214265928,
125.469770912784));
#260659=CARTESIAN_POINT('Ctrl Pts',(-48.9584088764139,-2.03601334702262,
124.104137951514));
#260660=CARTESIAN_POINT('Ctrl Pts',(-49.2368565002267,-6.7376020355722,
128.895682296272));
#260661=CARTESIAN_POINT('Ctrl Pts',(-49.5153041240395,-5.24766360358919,
135.441208774179));
#260662=CARTESIAN_POINT('Ctrl Pts',(-49.7937517478526,1.06462131747325,
137.725698318783));
#260663=CARTESIAN_POINT('Ctrl Pts',(-50.0721993716652,6.39857125742062,
133.649816642113));
#260664=CARTESIAN_POINT('Ctrl Pts',(-50.3506469954783,5.85254679938199,
126.959099887138));
#260665=CARTESIAN_POINT('Ctrl Pts',(-50.6290946192911,-0.0716822544825644,
123.801989891996));
#260666=CARTESIAN_POINT('Ctrl Pts',(-50.907542243104,-5.93003881835047,
127.079716508824));
#260667=CARTESIAN_POINT('Ctrl Pts',(-51.1859898669169,-6.33897940665598,
133.780209102606));
#260668=CARTESIAN_POINT('Ctrl Pts',(-51.4644374907297,-0.922707596604453,
137.746042316915));
#260669=CARTESIAN_POINT('Ctrl Pts',(-51.7428851145428,5.34148741795441,
135.332809169526));
#260670=CARTESIAN_POINT('Ctrl Pts',(-52.0213327383556,6.69711644158035,
128.758153029896));
#260671=CARTESIAN_POINT('Ctrl Pts',(-52.2997803621686,1.89842262772099,
124.063861700536));
#260672=CARTESIAN_POINT('Ctrl Pts',(-52.5782279859813,-4.64482883791282,
125.563759584248));
#260673=CARTESIAN_POINT('Ctrl Pts',(-52.8566756097944,-6.91970951400822,
131.879513799985));
#260674=CARTESIAN_POINT('Ctrl Pts',(-53.135123233607,-2.83571519333325,
137.207254765232));
#260675=CARTESIAN_POINT('Ctrl Pts',(-53.4135708574202,3.85416285762642,
136.651048807542));
#260676=CARTESIAN_POINT('Ctrl Pts',(-53.6920184812329,7.0022535287505,130.72202202986));
#260677=CARTESIAN_POINT('Ctrl Pts',(-53.9704661050458,3.71561528605495,
124.868660391816));
#260678=CARTESIAN_POINT('Ctrl Pts',(-54.2489137288587,-2.98549188662705,
124.469917286158));
#260679=CARTESIAN_POINT('Ctrl Pts',(-54.5273613526715,-6.94307786488582,
129.892218147303));
#260680=CARTESIAN_POINT('Ctrl Pts',(-54.8058089764845,-4.5203144735249,
136.152733377983));
#260681=CARTESIAN_POINT('Ctrl Pts',(-55.0842566002972,2.05639708936689,
137.498355324372));
#260682=CARTESIAN_POINT('Ctrl Pts',(-55.3627042241104,6.74338018771311,
132.69252315503));
#260683=CARTESIAN_POINT('Ctrl Pts',(-55.6411518479232,5.23352632598741,
126.151561855625));
#260684=CARTESIAN_POINT('Ctrl Pts',(-55.919599471736,-1.08568255734582,
123.886295316588));
#260685=CARTESIAN_POINT('Ctrl Pts',(-56.1980470955489,-6.40720220901991,
127.978392822871));
#260686=CARTESIAN_POINT('Ctrl Pts',(-56.4764947193619,-5.8408160398338,
134.667416676276));
#260687=CARTESIAN_POINT('Ctrl Pts',(-56.7549423431748,0.0929947302327828,
137.806480732508));
#260688=CARTESIAN_POINT('Ctrl Pts',(-57.0333899669875,5.94134788626073,
134.510938475691));
#260689=CARTESIAN_POINT('Ctrl Pts',(-57.3118375908005,6.32989258579528,
127.809232243652));
#260690=CARTESIAN_POINT('Ctrl Pts',(-57.5902852146133,0.901575231427987,
123.859902667085));
#260691=CARTESIAN_POINT('Ctrl Pts',(-57.8687328384263,-5.35524571622284,
126.292190691378));
#260692=CARTESIAN_POINT('Ctrl Pts',(-58.1471804622391,-6.69085746896258,
132.870942446081));
#260693=CARTESIAN_POINT('Ctrl Pts',(-58.4256280860521,-1.87789807428466,
137.550606458515));
#260694=CARTESIAN_POINT('Ctrl Pts',(-58.7040757098649,4.6607579102399,136.030800115547));
#260695=CARTESIAN_POINT('Ctrl Pts',(-58.9825233336777,6.91640506593584,
129.708151199698));
#260696=CARTESIAN_POINT('Ctrl Pts',(-59.2609709574908,2.81621385120844,
124.392865186062));
#260697=CARTESIAN_POINT('Ctrl Pts',(-59.5394185813036,-3.87194031308425,
124.969430255013));
#260698=CARTESIAN_POINT('Ctrl Pts',(-59.8178662051166,-7.00197048445272,
130.908011274954));
#260699=CARTESIAN_POINT('Ctrl Pts',(-60.0963138289294,-3.69753184588372,
136.751342404371));
#260700=CARTESIAN_POINT('Ctrl Pts',(-60.3747614527424,3.00475792457964,
137.129687797925));
#260701=CARTESIAN_POINT('Ctrl Pts',(-60.6532090765552,6.94582195293937,
131.695366522141));
#260702=CARTESIAN_POINT('Ctrl Pts',(-60.9316567003681,4.50401492881459,
125.442254348109));
#260703=CARTESIAN_POINT('Ctrl Pts',(-61.210104324181,-2.07676178152925,
124.116655882255));
#260704=CARTESIAN_POINT('Ctrl Pts',(-61.4885519479939,-6.74909587010084,
128.93673135561));
#260705=CARTESIAN_POINT('Ctrl Pts',(-61.7669995718066,-5.21934056571308,
135.473066881942));
#260706=CARTESIAN_POINT('Ctrl Pts',(-62.0454471956197,1.10673373960332,
137.719089430292));
#260707=CARTESIAN_POINT('Ctrl Pts',(-62.3238948194324,6.41577380517329,
133.610814003028));
#260708=CARTESIAN_POINT('Ctrl Pts',(-62.6023424432454,5.82903117176375,
126.923545017394));
#260709=CARTESIAN_POINT('Ctrl Pts',(-62.8807900670583,-0.114306344492842,
123.802555979936));
#260710=CARTESIAN_POINT('Ctrl Pts',(-63.1592376908712,-5.95260191433588,
127.115883347286));
#260711=CARTESIAN_POINT('Ctrl Pts',(-63.4376853146842,-6.32074712567447,
133.818741133891));
#260712=CARTESIAN_POINT('Ctrl Pts',(-63.716132938497,-0.880434514181572,
137.751530486667));
#260713=CARTESIAN_POINT('Ctrl Pts',(-63.99458056231,5.36895440422691,135.300210117855));
#260714=CARTESIAN_POINT('Ctrl Pts',(-64.2730281861228,6.6845365131549,128.717423692735));
#260715=CARTESIAN_POINT('Ctrl Pts',(-64.5514758099358,1.85735612425694,
124.052430348997));
#260716=CARTESIAN_POINT('Ctrl Pts',(-64.8299234337484,-4.67664380594228,
125.592131071942));
#260717=CARTESIAN_POINT('Ctrl Pts',(-65.1083710575615,-6.91303654523158,
131.921616115747));
#260718=CARTESIAN_POINT('Ctrl Pts',(-65.3868186813742,-2.79668642006362,
137.224397937687));
#260719=CARTESIAN_POINT('Ctrl Pts',(-65.6652663051872,3.88968189941585,
136.627479098696));
#260720=CARTESIAN_POINT('Ctrl Pts',(-65.9437139290001,7.00162257485687,
130.679398850698));
#260721=CARTESIAN_POINT('Ctrl Pts',(-66.2221615528129,3.67941415228271,
124.846152361731));
#260722=CARTESIAN_POINT('Ctrl Pts',(-66.500609176626,-3.02399612686491,
124.48820818522));
#260723=CARTESIAN_POINT('Ctrl Pts',(-66.7790568004388,-6.94850169584742,
129.934499532835));
#260724=CARTESIAN_POINT('Ctrl Pts',(-67.0575044242516,-4.48767365952541,
136.180150722241));
#260725=CARTESIAN_POINT('Ctrl Pts',(-67.3359520480646,2.09710723485436,
137.485713427398));
#260726=CARTESIAN_POINT('Ctrl Pts',(-67.6143996718775,6.75474902978674,
132.651439302549));
#260727=CARTESIAN_POINT('Ctrl Pts',(-67.8928472956903,5.20510645418034,
126.119790101011));
#260728=CARTESIAN_POINT('Ctrl Pts',(-68.1712949195033,-1.12777466923081,
123.893032350195));
#260729=CARTESIAN_POINT('Ctrl Pts',(-68.449742543316,-6.42428596647451,
128.017447639935));
#260730=CARTESIAN_POINT('Ctrl Pts',(-68.728190167129,-5.81719230434518,
134.702899807851));
#260731=CARTESIAN_POINT('Ctrl Pts',(-69.0066377909419,0.135616899834216,
137.805784914121));
#260732=CARTESIAN_POINT('Ctrl Pts',(-69.2850854147548,5.96380079832,134.474703130449));
#260733=CARTESIAN_POINT('Ctrl Pts',(-69.5635330385676,6.31154311101565,
127.770755883637));
#260734=CARTESIAN_POINT('Ctrl Pts',(-69.8419806623805,0.859285640710264,
123.854543187474));
#260735=CARTESIAN_POINT('Ctrl Pts',(-70.1204282861936,-5.38261335497044,
126.324873192109));
#260736=CARTESIAN_POINT('Ctrl Pts',(-70.3988759100064,-6.67815363271447,
132.911633305611));
#260737=CARTESIAN_POINT('Ctrl Pts',(-70.6773235338194,-1.83679696793597,
137.561912764793));
#260738=CARTESIAN_POINT('Ctrl Pts',(-70.9557711576322,4.69248637785542,
136.002331925448));
#260739=CARTESIAN_POINT('Ctrl Pts',(-71.2342187814451,6.90960398310133,
129.666069389173));
#260740=CARTESIAN_POINT('Ctrl Pts',(-71.5126664052579,2.77713308079745,
124.375840883174));
#260741=CARTESIAN_POINT('Ctrl Pts',(-71.7911140290708,-3.90738745226578,
124.993107962432));
#260742=CARTESIAN_POINT('Ctrl Pts',(-72.0695616528837,-7.00120980318599,
130.950632336283));
#260743=CARTESIAN_POINT('Ctrl Pts',(-72.3480092766965,-3.66126237309149,
136.773740146404));
#260744=CARTESIAN_POINT('Ctrl Pts',(-72.6264569005095,3.04320631526353,
137.111279789924));
#260745=CARTESIAN_POINT('Ctrl Pts',(-72.9049045243223,6.95111706878496,
131.653068824177));
#260746=CARTESIAN_POINT('Ctrl Pts',(-73.1833521481353,4.47129081703998,
125.414936478256));
#260747=CARTESIAN_POINT('Ctrl Pts',(-73.4617997719481,-2.11743326086482,
124.129421628353));
#260748=CARTESIAN_POINT('Ctrl Pts',(-73.7402473957612,-6.76033961440018,
128.977849620639));
#260749=CARTESIAN_POINT('Ctrl Pts',(-74.018695019574,-5.19082412325261,
135.504751989078));
#260750=CARTESIAN_POINT('Ctrl Pts',(-74.2971426433868,1.14880515130821,
137.712224313981));
#260751=CARTESIAN_POINT('Ctrl Pts',(-74.5755902671998,6.43273861406817,
133.571707369781));
#260752=CARTESIAN_POINT('Ctrl Pts',(-74.8540378910127,5.80529954725181,
126.8881339527));
#260753=CARTESIAN_POINT('Ctrl Pts',(-75.1324855148255,-0.156926198840311,
123.803381522322));
#260754=CARTESIAN_POINT('Ctrl Pts',(-75.4109331386384,-5.97494443446864,
127.15218686363));
#260755=CARTESIAN_POINT('Ctrl Pts',(-75.6893807624512,-6.30228062708332,
133.857161466198));
#260756=CARTESIAN_POINT('Ctrl Pts',(-75.9678283862644,-0.838128806933456,
137.756761226486));
#260757=CARTESIAN_POINT('Ctrl Pts',(-76.2462760100769,5.3962224419198,135.267444470826));
#260758=CARTESIAN_POINT('Ctrl Pts',(-76.52472363389,6.67170888677059,128.676771687789));
#260759=CARTESIAN_POINT('Ctrl Pts',(-76.8031712577027,1.81622079577817,
124.041249192718));
#260760=CARTESIAN_POINT('Ctrl Pts',(-77.0816188815158,-4.70828547921653,
125.620695700721));
#260761=CARTESIAN_POINT('Ctrl Pts',(-77.3600665053286,-6.90610741134329,
131.963677031195));
#260762=CARTESIAN_POINT('Ctrl Pts',(-77.6385141291417,-2.75755401454922,
137.241303213299));
#260763=CARTESIAN_POINT('Ctrl Pts',(-77.9169617529544,3.92505680761298,
136.603693612052));
#260764=CARTESIAN_POINT('Ctrl Pts',(-78.1954093767674,7.00073217326374,
130.636780302039));
#260765=CARTESIAN_POINT('Ctrl Pts',(-78.4738570005803,3.6430766764653,124.823865115242));
#260766=CARTESIAN_POINT('Ctrl Pts',(-78.7523046243931,-3.06238831181505,
124.506733131632));
#260767=CARTESIAN_POINT('Ctrl Pts',(-79.0307522482061,-6.95366804752337,
129.976813151389));
#260768=CARTESIAN_POINT('Ctrl Pts',(-79.3091998720188,-4.45486655312747,
136.207368864621));
#260769=CARTESIAN_POINT('Ctrl Pts',(-79.5876474958318,2.13773967126259,
137.472823950436));
#260770=CARTESIAN_POINT('Ctrl Pts',(-79.8660951196445,6.76586757215105,
132.610287005887));
#260771=CARTESIAN_POINT('Ctrl Pts',(-80.1445427434577,5.17649370523912,
126.08819193488));
#260772=CARTESIAN_POINT('Ctrl Pts',(-80.4229903672703,-1.16982499101125,
123.900025485612));
#260773=CARTESIAN_POINT('Ctrl Pts',(-80.7014379910835,-6.44113166965063,
128.056605727087));
#260774=CARTESIAN_POINT('Ctrl Pts',(-80.9798856148961,-5.7933530106558,
134.738238477622));
#260775=CARTESIAN_POINT('Ctrl Pts',(-81.2583332387092,0.17823404410257,
137.804829655383));
#260776=CARTESIAN_POINT('Ctrl Pts',(-81.5367808625219,5.98603271954817,
134.438331779315));
#260777=CARTESIAN_POINT('Ctrl Pts',(-81.815228486335,6.29295975968447,127.732391934959));
#260778=CARTESIAN_POINT('Ctrl Pts',(-82.0936761101477,0.816964208846405,
123.849441235906));
#260779=CARTESIAN_POINT('Ctrl Pts',(-82.3721237339607,-5.40978153900143,
126.357721681897));
#260780=CARTESIAN_POINT('Ctrl Pts',(-82.6505713577735,-6.66520233502723,
132.952246079378));
#260781=CARTESIAN_POINT('Ctrl Pts',(-82.9290189815866,-1.79562779839943,
137.572968667493));
#260782=CARTESIAN_POINT('Ctrl Pts',(-83.2074666053992,4.72404096366304,
135.97367112261));
#260783=CARTESIAN_POINT('Ctrl Pts',(-83.4859142292123,6.90254686235,129.624029758449));
#260784=CARTESIAN_POINT('Ctrl Pts',(-83.7643618530252,2.73794940269844,
124.359054791448));
#260785=CARTESIAN_POINT('Ctrl Pts',(-84.0428094768383,-3.94268980176888,
125.017001007954));
#260786=CARTESIAN_POINT('Ctrl Pts',(-84.3212571006508,-7.00018968951541,
130.99324797746));
#260787=CARTESIAN_POINT('Ctrl Pts',(-84.5997047244641,-3.62485723087481,
136.795916690882));
#260788=CARTESIAN_POINT('Ctrl Pts',(-84.8781523482765,3.08154193881888,
137.092638076712));
#260789=CARTESIAN_POINT('Ctrl Pts',(-85.1565999720898,6.95615460843127,
131.61073967702));
#260790=CARTESIAN_POINT('Ctrl Pts',(-85.4350475959023,4.4384010199398,125.387818315495));
#260791=CARTESIAN_POINT('Ctrl Pts',(-85.7134952197154,-2.1580262779319,
124.142434716771));
#260792=CARTESIAN_POINT('Ctrl Pts',(-85.9919428435283,-6.7713328518292,
129.019035567703));
#260793=CARTESIAN_POINT('Ctrl Pts',(-86.2703904673411,-5.16211533289519,
135.536262921482));
#260794=CARTESIAN_POINT('Ctrl Pts',(-86.5488380911541,1.19083399361533,
137.70510322424));
#260795=CARTESIAN_POINT('Ctrl Pts',(-86.827285714967,6.4494650554685,133.532498191482));
#260796=CARTESIAN_POINT('Ctrl Pts',(-87.1057333387799,5.78135280522977,
126.852868005224));
#260797=CARTESIAN_POINT('Ctrl Pts',(-87.3841809625928,-0.199540238229241,
123.804466488563));
#260798=CARTESIAN_POINT('Ctrl Pts',(-87.6626285864056,-5.99706555083783,
127.188625712615));
#260799=CARTESIAN_POINT('Ctrl Pts',(-87.9410762102187,-6.28358059516641,
133.895468675847));
#260800=CARTESIAN_POINT('Ctrl Pts',(-88.2195238340314,-0.795792042514341,
137.761734342542));
#260801=CARTESIAN_POINT('Ctrl Pts',(-88.4979714578443,5.42329052060546,
135.234513442586));
#260802=CARTESIAN_POINT('Ctrl Pts',(-88.7764190816572,6.65863403776028,
128.636198521433));
#260803=CARTESIAN_POINT('Ctrl Pts',(-89.0548667054699,1.77501816656995,
124.03031864602));
#260804=CARTESIAN_POINT('Ctrl Pts',(-89.3333143292831,-4.73975268523957,
125.649452412109));
#260805=CARTESIAN_POINT('Ctrl Pts',(-89.6117619530957,-6.8989223691057,
132.005694987746));
#260806=CARTESIAN_POINT('Ctrl Pts',(-89.8902095769088,-2.71831942685781,
137.257969965635));
#260807=CARTESIAN_POINT('Ctrl Pts',(-90.1686572007216,3.9602862713853,136.579693228991));
#260808=CARTESIAN_POINT('Ctrl Pts',(-90.4471048245344,6.99958235696585,
130.59416796313));
#260809=CARTESIAN_POINT('Ctrl Pts',(-90.7255524483476,3.60660420510239,
124.801799478213));
#260810=CARTESIAN_POINT('Ctrl Pts',(-91.0040000721602,-3.10066701883943,
124.525491438947));
#260811=CARTESIAN_POINT('Ctrl Pts',(-91.2824476959735,-6.95857672847263,
130.019157435019));
#260812=CARTESIAN_POINT('Ctrl Pts',(-91.560895319786,-4.4218943700117,136.234386796543));
#260813=CARTESIAN_POINT('Ctrl Pts',(-91.8393429435991,2.17829289294083,
137.459687371113));
#260814=CARTESIAN_POINT('Ctrl Pts',(-92.1177905674117,6.77673540280433,
132.56906778996));
#260815=CARTESIAN_POINT('Ctrl Pts',(-92.3962381912249,5.14768913942031,
126.056768528114));
#260816=CARTESIAN_POINT('Ctrl Pts',(-92.6746858150375,-1.21183196449619,
123.907274463707));
#260817=CARTESIAN_POINT('Ctrl Pts',(-92.9531334388505,-6.45773869432309,
128.095865633305));
#260818=CARTESIAN_POINT('Ctrl Pts',(-93.2315810626634,-5.76929904214118,
134.773431376103));
#260819=CARTESIAN_POINT('Ctrl Pts',(-93.5100286864763,0.220844583841736,
137.803614991691));
#260820=CARTESIAN_POINT('Ctrl Pts',(-93.7884763102892,6.00804282613147,
134.401825770043));
#260821=CARTESIAN_POINT('Ctrl Pts',(-94.0669239341021,6.27414322041607,
127.694141819211));
#260822=CARTESIAN_POINT('Ctrl Pts',(-94.3453715579151,0.774612504073732,
123.844597001431));
#260823=CARTESIAN_POINT('Ctrl Pts',(-94.6238191817278,-5.43674926158731,
126.390734943524));
#260824=CARTESIAN_POINT('Ctrl Pts',(-94.9022668055408,-6.65200405581671,
132.99277926246));
#260825=CARTESIAN_POINT('Ctrl Pts',(-95.1807144293538,-1.75439209121494,
137.583773756932));
#260826=CARTESIAN_POINT('Ctrl Pts',(-95.4591620531666,4.75542049839504,
135.94481876907));
#260827=CARTESIAN_POINT('Ctrl Pts',(-95.7376096769794,6.89523396518648,
129.582033865318));
#260828=CARTESIAN_POINT('Ctrl Pts',(-96.0160573007924,2.69866426887766,
124.342507532899));
#260829=CARTESIAN_POINT('Ctrl Pts',(-96.2945049246052,-3.97784605345104,
125.041108506217));
#260830=CARTESIAN_POINT('Ctrl Pts',(-96.5729525484182,-6.99891018124123,
131.035856619345));
#260831=CARTESIAN_POINT('Ctrl Pts',(-96.8514001722308,-3.58831776824163,
136.817871216047));
#260832=CARTESIAN_POINT('Ctrl Pts',(-97.129847796044,3.11976337470375,137.073763349068));
#260833=CARTESIAN_POINT('Ctrl Pts',(-97.4082954198568,6.96093438520996,
131.56838064919));
#260834=CARTESIAN_POINT('Ctrl Pts',(-97.6867430436697,4.40534675625846,
125.360900864701));
#260835=CARTESIAN_POINT('Ctrl Pts',(-97.9651906674826,-2.1985393285419,
124.155694665303));
#260836=CARTESIAN_POINT('Ctrl Pts',(-98.2436382912955,-6.78207517502872,
129.060287670645));
#260837=CARTESIAN_POINT('Ctrl Pts',(-98.5220859151084,-5.13321525845608,
135.567598511506));
#260838=CARTESIAN_POINT('Ctrl Pts',(-98.8005335389213,1.23281870913114,
137.697726424945));
#260839=CARTESIAN_POINT('Ctrl Pts',(-99.0789811627341,6.4659525095689,133.493187921042));
#260840=CARTESIAN_POINT('Ctrl Pts',(-99.3574287865471,5.7571918330539,126.817748481762));
#260841=CARTESIAN_POINT('Ctrl Pts',(-99.6358764103599,-0.242146883580649,
123.805810838454));
#260842=CARTESIAN_POINT('Ctrl Pts',(-99.9143240341728,-6.01896444373747,
127.225198543987));
#260843=CARTESIAN_POINT('Ctrl Pts',(-100.192771657986,-6.26464772285957,
133.93366134335));
#260844=CARTESIAN_POINT('Ctrl Pts',(-100.471219281798,-0.753425789729175,
137.766449650557));
#260845=CARTESIAN_POINT('Ctrl Pts',(-100.749666905611,5.45015763726631,
135.201418253402));
#260846=CARTESIAN_POINT('Ctrl Pts',(-101.028114529424,6.64531245061667,
128.595705697122));
#260847=CARTESIAN_POINT('Ctrl Pts',(-101.306562153237,1.73374976341167,
124.019639113937));
#260848=CARTESIAN_POINT('Ctrl Pts',(-101.58500977705,-4.77104425798471,
125.678400140516));
#260849=CARTESIAN_POINT('Ctrl Pts',(-101.863457400863,-6.89148168476197,
132.047668428412));
#260850=CARTESIAN_POINT('Ctrl Pts',(-102.141905024676,-2.67898411084018,
137.274397577103));
#260851=CARTESIAN_POINT('Ctrl Pts',(-102.420352648489,3.99536898529432,
136.555478838857));
#260852=CARTESIAN_POINT('Ctrl Pts',(-102.698800272302,6.99817316856906,
130.551563412989));
#260853=CARTESIAN_POINT('Ctrl Pts',(-102.977247896115,3.56999808969468,
124.779956268296));
#260854=CARTESIAN_POINT('Ctrl Pts',(-103.255695519928,-3.13883082950684,
124.544482412068));
#260855=CARTESIAN_POINT('Ctrl Pts',(-103.53414314374,-6.96322755680218,
130.061530814641));
#260856=CARTESIAN_POINT('Ctrl Pts',(-103.812590767553,-4.38875833197407,
136.261203516848));
#260857=CARTESIAN_POINT('Ctrl Pts',(-104.091038391366,2.21876539717438,
137.44630417621));
#260858=CARTESIAN_POINT('Ctrl Pts',(-104.369486015179,6.78735211903507,
132.52778318216));
#260859=CARTESIAN_POINT('Ctrl Pts',(-104.647933638992,5.11869382408742,
126.02552104512));
#260860=CARTESIAN_POINT('Ctrl Pts',(-104.926381262805,-1.25379403310144,
123.914779015865));
#260861=CARTESIAN_POINT('Ctrl Pts',(-105.204828886617,-6.47410642511416,
128.135225903801));
#260862=CARTESIAN_POINT('Ctrl Pts',(-105.483276510431,-5.74503129012806,
134.808477199207));
#260863=CARTESIAN_POINT('Ctrl Pts',(-105.761724134243,0.263446940103889,
137.802140968053));
#260864=CARTESIAN_POINT('Ctrl Pts',(-106.040171758056,6.02983030247923,
134.365186455377));
#260865=CARTESIAN_POINT('Ctrl Pts',(-106.318619381869,6.25509419046252,
127.656006953765));
#260866=CARTESIAN_POINT('Ctrl Pts',(-106.597067005682,0.732232095750508,
123.840010663559));
#260867=CARTESIAN_POINT('Ctrl Pts',(-106.875514629495,-5.46351552342998,
126.423911753675));
#260868=CARTESIAN_POINT('Ctrl Pts',(-107.153962253308,-6.63855928414971,
133.033231352883));
#260869=CARTESIAN_POINT('Ctrl Pts',(-107.432409877121,-1.71309137438684,
137.594327632723));
#260870=CARTESIAN_POINT('Ctrl Pts',(-107.710857500934,4.78662381927155,
135.915775933963));
#260871=CARTESIAN_POINT('Ctrl Pts',(-107.989305124746,6.8876655625929,129.540083265954));
#260872=CARTESIAN_POINT('Ctrl Pts',(-108.26775274856,2.65927913505975,124.326199720693));
#260873=CARTESIAN_POINT('Ctrl Pts',(-108.546200372372,-4.0128549045848,
125.065429563905));
#260874=CARTESIAN_POINT('Ctrl Pts',(-108.824647996185,-6.99737132577695,
131.078456683062));
#260875=CARTESIAN_POINT('Ctrl Pts',(-109.103095619998,-3.5516453391731,
136.839602908365));
#260876=CARTESIAN_POINT('Ctrl Pts',(-109.381543243811,3.1578692066097,137.054656306401));
#260877=CARTESIAN_POINT('Ctrl Pts',(-109.659990867624,6.96545622200577,
131.525993310316));
#260878=CARTESIAN_POINT('Ctrl Pts',(-109.938438491437,4.37212925083209,
125.334185123311));
#260879=CARTESIAN_POINT('Ctrl Pts',(-110.21688611525,-2.23897091146772,
124.169200982596));
#260880=CARTESIAN_POINT('Ctrl Pts',(-110.495333739063,-6.79256618593892,
129.10160440085));
#260881=CARTESIAN_POINT('Ctrl Pts',(-110.773781362875,-5.10412497083799,
135.598757597999));
#260882=CARTESIAN_POINT('Ctrl Pts',(-111.052228986688,1.27475774209554,
137.690094189444));
#260883=CARTESIAN_POINT('Ctrl Pts',(-111.330676610501,6.48220036542147,
133.453778015119));
#260884=CARTESIAN_POINT('Ctrl Pts',(-111.609124234314,5.73281752601749,
126.782776683677));
#260885=CARTESIAN_POINT('Ctrl Pts',(-111.887571858127,-0.284744556090853,
123.807414522182));
#260886=CARTESIAN_POINT('Ctrl Pts',(-112.16601948194,-6.04064030169634,
127.261904002525));
#260887=CARTESIAN_POINT('Ctrl Pts',(-112.444467105753,-6.24548271172772,
133.971738053464));
#260888=CARTESIAN_POINT('Ctrl Pts',(-112.722914729566,-0.71103161847358,
137.770906975801));
#260889=CARTESIAN_POINT('Ctrl Pts',(-113.001362353379,5.47682279633179,
135.16816012963));
#260890=CARTESIAN_POINT('Ctrl Pts',(-113.279809977192,6.63174461897671,
128.55529471533));
#260891=CARTESIAN_POINT('Ctrl Pts',(-113.558257601004,1.69241711551747,
124.009210992206));
#260892=CARTESIAN_POINT('Ctrl Pts',(-113.836705224817,-4.80215903792943,
125.707537813274));
#260893=CARTESIAN_POINT('Ctrl Pts',(-114.11515284863,-6.88378563403075,
132.089595797848));
#260894=CARTESIAN_POINT('Ctrl Pts',(-114.393600472443,-2.63954952408134,
137.290585438973));
#260895=CARTESIAN_POINT('Ctrl Pts',(-114.672048096256,4.03030364933543,
136.531051338922));
#260896=CARTESIAN_POINT('Ctrl Pts',(-114.950495720069,6.99650466029252,
130.508968230339));
#260897=CARTESIAN_POINT('Ctrl Pts',(-115.228943343882,3.53325968669456,
124.758336294896));
#260898=CARTESIAN_POINT('Ctrl Pts',(-115.507390967695,-3.17687832964389,
124.563705347279));
#260899=CARTESIAN_POINT('Ctrl Pts',(-115.785838591507,-6.96762036017394,
130.103931720095));
#260900=CARTESIAN_POINT('Ctrl Pts',(-116.06428621532,-4.35545966688232,
136.287818031834));
#260901=CARTESIAN_POINT('Ctrl Pts',(-116.342733839133,2.25915568424066,
137.432674861647));
#260902=CARTESIAN_POINT('Ctrl Pts',(-116.621181462946,6.79771732743703,
132.486434712303));
#260903=CARTESIAN_POINT('Ctrl Pts',(-116.899629086759,5.08950883367243,
125.994450643782));
#260904=CARTESIAN_POINT('Ctrl Pts',(-117.178076710572,-1.2957096419083,
123.922538864004));
#260905=CARTESIAN_POINT('Ctrl Pts',(-117.456524334385,-6.49023425551004,
128.174685080065));
#260906=CARTESIAN_POINT('Ctrl Pts',(-117.734971958198,-5.7205506538686,
134.843374648297));
#260907=CARTESIAN_POINT('Ctrl Pts',(-118.013419582011,0.306039534242538,
137.800407639092));
#260908=CARTESIAN_POINT('Ctrl Pts',(-118.291867205823,6.05139434124684,
134.328415193001));
#260909=CARTESIAN_POINT('Ctrl Pts',(-118.570314829636,6.23581337569426,
127.617988751722));
#260910=CARTESIAN_POINT('Ctrl Pts',(-118.848762453449,0.689824554297045,
123.835682392233));
#260911=CARTESIAN_POINT('Ctrl Pts',(-119.127210077262,-5.49007933269568,
126.457250882969));
#260912=CARTESIAN_POINT('Ctrl Pts',(-119.405657701075,-6.62486851822702,
133.073600851681));
#260913=CARTESIAN_POINT('Ctrl Pts',(-119.684105324888,-1.67172717832737,
137.60462990379));
#260914=CARTESIAN_POINT('Ctrl Pts',(-119.962552948701,4.81764977004229,
135.886543693482));
#260915=CARTESIAN_POINT('Ctrl Pts',(-120.241000572514,6.87984193501854,
129.498179514853));
#260916=CARTESIAN_POINT('Ctrl Pts',(-120.519448196327,2.61979546067638,
124.310131959122));
#260917=CARTESIAN_POINT('Ctrl Pts',(-120.79789582014,-4.04771505790416,
125.089963279793));
#260918=CARTESIAN_POINT('Ctrl Pts',(-121.076343443952,-6.9955731801444,
131.121046590047));
#260919=CARTESIAN_POINT('Ctrl Pts',(-121.354791067765,-3.51484130258126,
136.86111096256));
#260920=CARTESIAN_POINT('Ctrl Pts',(-121.633238691578,3.19585802251066,
137.035317656727));
#260921=CARTESIAN_POINT('Ctrl Pts',(-121.911686315391,6.96971995125911,
131.483579231079));
#260922=CARTESIAN_POINT('Ctrl Pts',(-122.190133939204,4.3387497345494,125.307672081285));
#260923=CARTESIAN_POINT('Ctrl Pts',(-122.468581563017,-2.2793195285039,
124.182953168171));
#260924=CARTESIAN_POINT('Ctrl Pts',(-122.74702918683,-6.80280549581075,
129.142984227312));
#260925=CARTESIAN_POINT('Ctrl Pts',(-123.025476810643,-5.07484554799192,
135.629739026348));
#260926=CARTESIAN_POINT('Ctrl Pts',(-123.303924434456,1.31664953844379,
137.682206800553));
#260927=CARTESIAN_POINT('Ctrl Pts',(-123.582372058268,6.49820802095541,
133.414269934058));
#260928=CARTESIAN_POINT('Ctrl Pts',(-123.860819682081,5.7082307873194,126.747953906865));
#260929=CARTESIAN_POINT('Ctrl Pts',(-124.139267305894,-0.327331677286216,
123.809277480321));
#260930=CARTESIAN_POINT('Ctrl Pts',(-124.417714929707,-6.06209232150722,
127.298740728095));
#260931=CARTESIAN_POINT('Ctrl Pts',(-124.69616255352,-6.22608627193705,
134.009697395242));
#260932=CARTESIAN_POINT('Ctrl Pts',(-124.974610177333,-0.668611099680587,
137.77510615311));
#260933=CARTESIAN_POINT('Ctrl Pts',(-125.253057801146,5.50328500971429,
135.134740303665));
#260934=CARTESIAN_POINT('Ctrl Pts',(-125.531505424959,6.61793104560076,
128.514967073503));
#260935=CARTESIAN_POINT('Ctrl Pts',(-125.809953048772,1.6510217544855,123.999034667242));
#260936=CARTESIAN_POINT('Ctrl Pts',(-126.088400672584,-4.8330958721059,
125.736864350674));
#260937=CARTESIAN_POINT('Ctrl Pts',(-126.366848296398,-6.87583450209069,
132.131475542423));
#260938=CARTESIAN_POINT('Ctrl Pts',(-126.64529592021,-2.60001712784396,
137.306532951397));
#260939=CARTESIAN_POINT('Ctrl Pts',(-126.923743544023,4.06508896899354,
136.506411634357));
#260940=CARTESIAN_POINT('Ctrl Pts',(-127.202191167836,6.99457689396224,
130.466383993564));
#260941=CARTESIAN_POINT('Ctrl Pts',(-127.480638791649,3.49639035745773,
124.736940359153));
#260942=CARTESIAN_POINT('Ctrl Pts',(-127.759086415462,-3.21480810938582,
124.583159532264));
#260943=CARTESIAN_POINT('Ctrl Pts',(-128.037534039275,-6.97175497581086,
130.146358580199));
#260944=CARTESIAN_POINT('Ctrl Pts',(-128.315981663087,-4.32199960863106,
136.314229355287));
#260945=CARTESIAN_POINT('Ctrl Pts',(-128.594429286901,2.29946225746178,
137.418799932461));
#260946=CARTESIAN_POINT('Ctrl Pts',(-128.872876910713,6.80783064392392,
132.44502391257));
#260947=CARTESIAN_POINT('Ctrl Pts',(-129.151324534526,5.06013524963555,
125.963558475429));
#260948=CARTESIAN_POINT('Ctrl Pts',(-129.429772158339,-1.33757723771771,
123.930553720578));
#260949=CARTESIAN_POINT('Ctrl Pts',(-129.708219782152,-6.50612158788957,
128.214241699924));
#260950=CARTESIAN_POINT('Ctrl Pts',(-129.986667405965,-5.69585804050008,
134.878122430239));
#260951=CARTESIAN_POINT('Ctrl Pts',(-130.265115029778,0.348620787973942,
137.798415069035));
#260952=CARTESIAN_POINT('Ctrl Pts',(-130.543562653591,6.07273414337257,
134.291513345486));
#260953=CARTESIAN_POINT('Ctrl Pts',(-130.822010277403,6.21630149056731,
127.58008862186));
#260954=CARTESIAN_POINT('Ctrl Pts',(-131.100457901217,0.647391451141708,
123.831612347843));
#260955=CARTESIAN_POINT('Ctrl Pts',(-131.378905525029,-5.5164397050528,
126.490751096011));
#260956=CARTESIAN_POINT('Ctrl Pts',(-131.657353148842,-6.61093226536518,
133.113886262947));
#260957=CARTESIAN_POINT('Ctrl Pts',(-131.935800772655,-1.63030103580305,
137.614680188378));
#260958=CARTESIAN_POINT('Ctrl Pts',(-132.214248396468,4.848497201029,135.857123130838));
#260959=CARTESIAN_POINT('Ctrl Pts',(-132.492696020281,6.87176337237162,
129.456324164773));
#260960=CARTESIAN_POINT('Ctrl Pts',(-132.771143644094,2.58021470880796,
124.294304843582));
#260961=CARTESIAN_POINT('Ctrl Pts',(-133.049591267907,-4.08242522165371,
125.114708744776));
#260962=CARTESIAN_POINT('Ctrl Pts',(-133.32803889172,-6.99351581097555,
131.163624762118));
#260963=CARTESIAN_POINT('Ctrl Pts',(-133.606486515532,-3.47790702225152,
136.882394581644));
#260964=CARTESIAN_POINT('Ctrl Pts',(-133.884934139345,3.23372841471757,
137.015748116649));
#260965=CARTESIAN_POINT('Ctrl Pts',(-134.163381763158,6.97372541497715,
131.441139983145));
#260966=CARTESIAN_POINT('Ctrl Pts',(-134.441829386971,4.30520944429882,
125.281362721075));
#260967=CARTESIAN_POINT('Ctrl Pts',(-134.720277010784,-2.31958368451587,
124.196950712432));
#260968=CARTESIAN_POINT('Ctrl Pts',(-134.998724634597,-6.81279272522359,
129.184425616688));
#260969=CARTESIAN_POINT('Ctrl Pts',(-135.27717225841,-5.04537807487797,
135.660541648527));
#260970=CARTESIAN_POINT('Ctrl Pts',(-135.555619882223,1.35849254585843,
137.674064550544));
#260971=CARTESIAN_POINT('Ctrl Pts',(-135.834067506036,6.51397488300169,
133.374665141848));
#260972=CARTESIAN_POINT('Ctrl Pts',(-136.112515129848,5.68343252803032,
126.713281441693));
#260973=CARTESIAN_POINT('Ctrl Pts',(-136.390962753662,-0.369906669086523,
123.811399643837));
#260974=CARTESIAN_POINT('Ctrl Pts',(-136.669410377474,-6.08331970825794,
127.335707355701));
#260975=CARTESIAN_POINT('Ctrl Pts',(-136.947858001288,-6.20645912223011,
134.047537962086));
#260976=CARTESIAN_POINT('Ctrl Pts',(-137.2263056251,-0.626165805256695,
137.779047026878));
#260977=CARTESIAN_POINT('Ctrl Pts',(-137.504753248913,5.52954329684707,
135.101160013885));
#260978=CARTESIAN_POINT('Ctrl Pts',(-137.783200872726,6.60387224235649,
128.474724265995));
#260979=CARTESIAN_POINT('Ctrl Pts',(-138.061648496539,1.60956521423443,
123.989110516135));
#260980=CARTESIAN_POINT('Ctrl Pts',(-138.340096120352,-4.86385361413656,
125.766378666012));
#260981=CARTESIAN_POINT('Ctrl Pts',(-138.618543744165,-6.86762858357524,
132.173306110266));
#260982=CARTESIAN_POINT('Ctrl Pts',(-138.896991367977,-2.56038838701599,
137.322239523433));
#260983=CARTESIAN_POINT('Ctrl Pts',(-139.17543899179,4.09972365528409,136.481560638194));
#260984=CARTESIAN_POINT('Ctrl Pts',(-139.453886615603,6.99238994101352,
130.423812280637));
#260985=CARTESIAN_POINT('Ctrl Pts',(-139.732334239416,3.45939146819007,
124.715769253897));
#260986=CARTESIAN_POINT('Ctrl Pts',(-140.010781863229,-3.25261876323132,
124.602844246145));
#260987=CARTESIAN_POINT('Ctrl Pts',(-140.289229487042,-6.97563125050334,
130.188809822811));
#260988=CARTESIAN_POINT('Ctrl Pts',(-140.567677110855,-4.28837939709471,
136.340436508528));
#260989=CARTESIAN_POINT('Ctrl Pts',(-140.846124734668,2.33968362326381,
137.404679902793));
#260990=CARTESIAN_POINT('Ctrl Pts',(-141.124572358481,6.81769169374202,
132.403552317457));
#260991=CARTESIAN_POINT('Ctrl Pts',(-141.403019982293,5.03057416042698,
125.932845684778));
#260992=CARTESIAN_POINT('Ctrl Pts',(-141.681467606106,-1.37939526911043,
123.938823288595));
#260993=CARTESIAN_POINT('Ctrl Pts',(-141.959915229919,-6.52176783354029,
128.253894297592));
#260994=CARTESIAN_POINT('Ctrl Pts',(-142.238362853732,-5.67095436501806,
134.912719257437));
#260995=CARTESIAN_POINT('Ctrl Pts',(-142.516810477545,0.39118912343359,
137.796163331718));
#260996=CARTESIAN_POINT('Ctrl Pts',(-142.795258101358,6.09384891810056,
134.254482280245));
#260997=CARTESIAN_POINT('Ctrl Pts',(-143.073705725171,6.19655925810344,
127.542307968582));
#260998=CARTESIAN_POINT('Ctrl Pts',(-143.352153348984,0.604934358657401,
123.827800681205));
#260999=CARTESIAN_POINT('Ctrl Pts',(-143.630600972796,-5.54259566370794,
126.524411151443));
#261000=CARTESIAN_POINT('Ctrl Pts',(-143.90904859661,-6.59675104197701,
133.154086093891));
#261001=CARTESIAN_POINT('Ctrl Pts',(-144.187496220422,-1.58881448187379,
137.624478114069));
#261002=CARTESIAN_POINT('Ctrl Pts',(-144.465943844235,4.87916496916901,
135.827515336221));
#261003=CARTESIAN_POINT('Ctrl Pts',(-144.744391468048,6.86343017400547,
129.41451876668));
#261004=CARTESIAN_POINT('Ctrl Pts',(-145.022839091861,2.54053834613545,
124.278718960552));
#261005=CARTESIAN_POINT('Ctrl Pts',(-145.301286715674,-4.11698410963516,
125.139665041902));
#261006=CARTESIAN_POINT('Ctrl Pts',(-145.579734339487,-6.99119929450595,
131.206189621523));
#261007=CARTESIAN_POINT('Ctrl Pts',(-145.8581819633,-3.44084386679896,136.903452976945));
#261008=CARTESIAN_POINT('Ctrl Pts',(-146.136629587113,3.27147897992919,
136.995948411323));
#261009=CARTESIAN_POINT('Ctrl Pts',(-146.415077210925,6.97747246473481,
131.398677139117));
#261010=CARTESIAN_POINT('Ctrl Pts',(-146.693524834738,4.27150962292939,
125.255258017582));
#261011=CARTESIAN_POINT('Ctrl Pts',(-146.971972458551,-2.35976188750221,
124.211193096699));
#261012=CARTESIAN_POINT('Ctrl Pts',(-147.250420082364,-6.82252750409623,
129.225927033352));
#261013=CARTESIAN_POINT('Ctrl Pts',(-147.528867706177,-5.01572364342383,
135.69116432313));
#261014=CARTESIAN_POINT('Ctrl Pts',(-147.80731532999,1.40028521383297,137.665667741127));
#261015=CARTESIAN_POINT('Ctrl Pts',(-148.085762953803,6.52950036731291,
133.334965106058));
#261016=CARTESIAN_POINT('Ctrl Pts',(-148.364210577616,5.65842366705879,
126.678760572968));
#261017=CARTESIAN_POINT('Ctrl Pts',(-148.642658201429,-0.412467953858535,
123.813780934094));
#261018=CARTESIAN_POINT('Ctrl Pts',(-148.921105825242,-6.10432167535963,
127.372802515528));
#261019=CARTESIAN_POINT('Ctrl Pts',(-149.199553449054,-6.18660198989778,
134.085258351801));
#261020=CARTESIAN_POINT('Ctrl Pts',(-149.478001072867,-0.583697308029368,
137.782729451077));
#261021=CARTESIAN_POINT('Ctrl Pts',(-149.75644869668,5.55559668471987,135.067420504625));
#261022=CARTESIAN_POINT('Ctrl Pts',(-150.034896320493,6.58956873019717,
128.434567784019));
#261023=CARTESIAN_POINT('Ctrl Pts',(-150.313343944306,1.56804903095274,
123.979438906626));
#261024=CARTESIAN_POINT('Ctrl Pts',(-150.591791568119,-4.89443112428377,
125.796079665625));
#261025=CARTESIAN_POINT('Ctrl Pts',(-150.870239191931,-6.85916818255639,
132.21508595133));
#261026=CARTESIAN_POINT('Ctrl Pts',(-151.148686815745,-2.52066477005453,
137.33770457307));
#261027=CARTESIAN_POINT('Ctrl Pts',(-151.427134439557,4.13420642480782,
136.456499271296));
#261028=CARTESIAN_POINT('Ctrl Pts',(-151.705582063371,6.98994388248347,
130.381254669068));
#261029=CARTESIAN_POINT('Ctrl Pts',(-151.984029687183,3.42226438989971,
124.694823763634));
#261030=CARTESIAN_POINT('Ctrl Pts',(-152.262477310996,-3.29030889009209,
124.622758759495));
#261031=CARTESIAN_POINT('Ctrl Pts',(-152.540924934809,-6.97924904061452,
130.231283874884));
#261032=CARTESIAN_POINT('Ctrl Pts',(-152.819372558622,-4.25460027808296,
136.366438520441));
#261033=CARTESIAN_POINT('Ctrl Pts',(-153.097820182435,2.37981829122829,
137.390315295868));
#261034=CARTESIAN_POINT('Ctrl Pts',(-153.376267806248,6.82730011148789,
132.362021463707));
#261035=CARTESIAN_POINT('Ctrl Pts',(-153.654715430061,5.00082666144207,
125.902313409905));
#261036=CARTESIAN_POINT('Ctrl Pts',(-153.933163053873,-1.42116218650446,
123.947347261623));
#261037=CARTESIAN_POINT('Ctrl Pts',(-154.211610677687,-6.53717241268631,
128.293641403726));
#261038=CARTESIAN_POINT('Ctrl Pts',(-154.490058301499,-5.64584055023574,
134.947163847896));
#261039=CARTESIAN_POINT('Ctrl Pts',(-154.768505925312,0.433742963236675,
137.79365251058));
#261040=CARTESIAN_POINT('Ctrl Pts',(-155.046953549125,6.11473788301669,
134.217323369476));
#261041=CARTESIAN_POINT('Ctrl Pts',(-155.325401172938,6.17658740985663,
127.504648191865));
#261042=CARTESIAN_POINT('Ctrl Pts',(-155.603848796751,0.562454850108638,
123.824247533559));
#261043=CARTESIAN_POINT('Ctrl Pts',(-155.882296420564,-5.5685462394425,
126.558229801974));
#261044=CARTESIAN_POINT('Ctrl Pts',(-156.160744044376,-6.5823253735531,
133.194198854895));
#261045=CARTESIAN_POINT('Ctrl Pts',(-156.43919166819,-1.54726905384013,
137.634023317798));
#261046=CARTESIAN_POINT('Ctrl Pts',(-156.717639292002,4.90965193805665,
135.79772140676));
#261047=CARTESIAN_POINT('Ctrl Pts',(-156.996086915816,6.8548426487106,129.372764869687));
#261048=CARTESIAN_POINT('Ctrl Pts',(-157.274534539628,2.50076784287941,
124.263374887574));
#261049=CARTESIAN_POINT('Ctrl Pts',(-157.552982163441,-4.15139044125659,
125.164831246407));
#261050=CARTESIAN_POINT('Ctrl Pts',(-157.831429787254,-6.98862371657603,
131.248739591007));
#261051=CARTESIAN_POINT('Ctrl Pts',(-158.109877411067,-3.40365320961064,
136.924285368134));
#261052=CARTESIAN_POINT('Ctrl Pts',(-158.38832503488,3.30910831928323,136.975919274434));
#261053=CARTESIAN_POINT('Ctrl Pts',(-158.666772658693,6.98096096168483,
131.356192272474));
#261054=CARTESIAN_POINT('Ctrl Pts',(-158.945220282506,4.23765151920024,
125.229358938127));
#261055=CARTESIAN_POINT('Ctrl Pts',(-159.223667906319,-2.39985264864321,
124.225679793212));
#261056=CARTESIAN_POINT('Ctrl Pts',(-159.502115530131,-6.8320094717036,
129.267486939452));
#261057=CARTESIAN_POINT('Ctrl Pts',(-159.780563153944,-4.98588335248574,
135.721605915426));
#261058=CARTESIAN_POINT('Ctrl Pts',(-160.059010777757,1.44202599372318,
137.657016683454));
#261059=CARTESIAN_POINT('Ctrl Pts',(-160.33745840157,6.54478389858708,133.295171297791));
#261060=CARTESIAN_POINT('Ctrl Pts',(-160.615906025383,5.63320513111742,
126.644392579866));
#261061=CARTESIAN_POINT('Ctrl Pts',(-160.894353649196,-0.455013954479453,
123.816421262852));
#261062=CARTESIAN_POINT('Ctrl Pts',(-161.172801273009,-6.12509744457689,
127.410024833003));
#261063=CARTESIAN_POINT('Ctrl Pts',(-161.451248896821,-6.16651561075379,
134.122857166646));
#261064=CARTESIAN_POINT('Ctrl Pts',(-161.729696520635,-0.541207181682879,
137.786153289251));
#261065=CARTESIAN_POINT('Ctrl Pts',(-162.008144144447,5.58144420791359,
135.033523026113));
#261066=CARTESIAN_POINT('Ctrl Pts',(-162.286591768261,6.57502103914602,
128.394499115588));
#261067=CARTESIAN_POINT('Ctrl Pts',(-162.565039392073,1.52647474303778,
123.970020197102));
#261068=CARTESIAN_POINT('Ctrl Pts',(-162.843487015886,-4.92482726948487,
125.825966248931));
#261069=CARTESIAN_POINT('Ctrl Pts',(-163.121934639699,-6.85045361253876,
132.256813517449));
#261070=CARTESIAN_POINT('Ctrl Pts',(-163.400382263512,-2.48084774893327,
137.352927527244));
#261071=CARTESIAN_POINT('Ctrl Pts',(-163.678829887325,4.16853599979124,
136.431228462323));
#261072=CARTESIAN_POINT('Ctrl Pts',(-163.957277511138,6.98723880901292,
130.338712735846));
#261073=CARTESIAN_POINT('Ctrl Pts',(-164.23572513495,3.3850104983435,124.674104664506));
#261074=CARTESIAN_POINT('Ctrl Pts',(-164.514172758764,-3.32787709334726,
124.642902334375));
#261075=CARTESIAN_POINT('Ctrl Pts',(-164.792620382576,-6.98260821208591,
130.273779162525));
#261076=CARTESIAN_POINT('Ctrl Pts',(-165.07106800639,-4.22066350329308,
136.392234427513));
#261077=CARTESIAN_POINT('Ctrl Pts',(-165.349515630202,2.4198647741513,137.37570664397));
#261078=CARTESIAN_POINT('Ctrl Pts',(-165.627963254015,6.83665554111671,
132.320432890263));
#261079=CARTESIAN_POINT('Ctrl Pts',(-165.906410877828,4.97089385498702,
125.871962782194));
#261080=CARTESIAN_POINT('Ctrl Pts',(-166.184858501641,-1.46287644221077,
123.956125323802));
#261081=CARTESIAN_POINT('Ctrl Pts',(-166.463306125454,-6.55233475450377,
128.333481545486));
#261082=CARTESIAN_POINT('Ctrl Pts',(-166.741753749267,-5.62051752675643,
134.981454925258));
#261083=CARTESIAN_POINT('Ctrl Pts',(-167.020201373079,0.476280730534997,
137.790882698662));
#261084=CARTESIAN_POINT('Ctrl Pts',(-167.298648996893,6.13540026407138,
134.180037990117));
#261085=CARTESIAN_POINT('Ctrl Pts',(-167.577096620705,6.15638668589229,
127.467110687205));
#261086=CARTESIAN_POINT('Ctrl Pts',(-167.855544244518,0.519954499587912,
123.820953036571));
#261087=CARTESIAN_POINT('Ctrl Pts',(-168.133991868331,-5.5942904706483,
126.592205794446));
#261088=CARTESIAN_POINT('Ctrl Pts',(-168.412439492144,-6.56765579464175,
133.234223059563));
#261089=CARTESIAN_POINT('Ctrl Pts',(-168.690887115956,-1.50566629118217,
137.643315445865));
#261090=CARTESIAN_POINT('Ctrl Pts',(-168.96933473977,4.93995697798634,135.767742446477));
#261091=CARTESIAN_POINT('Ctrl Pts',(-169.247782363582,6.84600111470013,
129.331064021001));
#261092=CARTESIAN_POINT('Ctrl Pts',(-169.526229987396,2.46090467275213,
124.248273193229));
#261093=CARTESIAN_POINT('Ctrl Pts',(-169.804677611208,-4.18564294157836,
125.190206425745));
#261094=CARTESIAN_POINT('Ctrl Pts',(-170.083125235021,-6.98578917262369,
131.291273093865));
#261095=CARTESIAN_POINT('Ctrl Pts',(-170.361572858834,-3.36633642880185,
136.944890983262));
#261096=CARTESIAN_POINT('Ctrl Pts',(-170.640020482647,3.34661503841248,
136.955661448171));
#261097=CARTESIAN_POINT('Ctrl Pts',(-170.91846810646,6.98419077655865,131.313686957504));
#261098=CARTESIAN_POINT('Ctrl Pts',(-171.196915730273,4.20363638773547,
125.203666442409));
#261099=CARTESIAN_POINT('Ctrl Pts',(-171.475363354086,-2.43985448236259,
124.240410265162));
#261100=CARTESIAN_POINT('Ctrl Pts',(-171.753810977898,-6.84123827668714,
129.309103794972));
#261101=CARTESIAN_POINT('Ctrl Pts',(-172.032258601712,-4.9558583078063,
135.751865297389));
#261102=CARTESIAN_POINT('Ctrl Pts',(-172.310706225524,1.48371333881067,
137.648111698089));
#261103=CARTESIAN_POINT('Ctrl Pts',(-172.589153849337,6.55982491048677,
133.255285191615));
#261104=CARTESIAN_POINT('Ctrl Pts',(-172.86760147315,5.60777785468832,126.610178735912));
#261105=CARTESIAN_POINT('Ctrl Pts',(-173.146049096963,-0.497543094390354,
123.819320532272));
#261106=CARTESIAN_POINT('Ctrl Pts',(-173.424496720776,-6.14564624605571,
127.447372928838));
#261107=CARTESIAN_POINT('Ctrl Pts',(-173.702944344589,-6.14620072910595,
134.160333013378));
#261108=CARTESIAN_POINT('Ctrl Pts',(-173.981391968402,-0.498697000705985,
137.789318414533));
#261109=CARTESIAN_POINT('Ctrl Pts',(-174.259839592215,5.60708490864046,
134.999468834432));
#261110=CARTESIAN_POINT('Ctrl Pts',(-174.538287216028,6.56022970827155,
128.354519745462));
#261111=CARTESIAN_POINT('Ctrl Pts',(-174.81673483984,1.48484389103961,123.960854736574));
#261112=CARTESIAN_POINT('Ctrl Pts',(-175.095182463654,-4.95504092340126,
125.85603730847));
#261113=CARTESIAN_POINT('Ctrl Pts',(-175.373630087466,-6.8414851964426,
132.298487262391));
#261114=CARTESIAN_POINT('Ctrl Pts',(-175.652077711279,-2.44093879908611,
137.367907821863));
#261115=CARTESIAN_POINT('Ctrl Pts',(-175.930525335092,4.20271110814107,
136.405749147692));
#261116=CARTESIAN_POINT('Ctrl Pts',(-176.208972958905,6.98427482083815,
130.296188057377));
#261117=CARTESIAN_POINT('Ctrl Pts',(-176.487420582718,3.3476311739788,124.653612724266));
#261118=CARTESIAN_POINT('Ctrl Pts',(-176.765868206531,-3.36532198089259,
124.663274224357));
#261119=CARTESIAN_POINT('Ctrl Pts',(-177.044315830343,-6.98570864044213,
130.316294111058));
#261120=CARTESIAN_POINT('Ctrl Pts',(-177.322763454156,-4.18657033026512,
136.417823273865));
#261121=CARTESIAN_POINT('Ctrl Pts',(-177.601211077969,2.4598215880947,137.360854488428));
#261122=CARTESIAN_POINT('Ctrl Pts',(-177.879658701782,6.84575763596098,
132.278788138201));
#261123=CARTESIAN_POINT('Ctrl Pts',(-178.158106325595,4.94077685023126,
125.841794926299));
#261124=CARTESIAN_POINT('Ctrl Pts',(-178.436553949408,-1.50453649049278,
123.965157149858));
#261125=CARTESIAN_POINT('Ctrl Pts',(-178.715001573221,-6.56725429714808,
128.373413246577));
#261126=CARTESIAN_POINT('Ctrl Pts',(-178.993449197033,-5.59498623293233,
135.015591218853));
#261127=CARTESIAN_POINT('Ctrl Pts',(-179.271896820847,0.518800849074927,
137.787853998597));
#261128=CARTESIAN_POINT('Ctrl Pts',(-179.550344444659,6.15583529561319,
134.142627523792));
#261129=CARTESIAN_POINT('Ctrl Pts',(-179.828792068472,6.13595783475539,
127.429696845569));
#261130=CARTESIAN_POINT('Ctrl Pts',(-180.107239692285,0.477434881962636,
123.81791731232));
#261131=CARTESIAN_POINT('Ctrl Pts',(-180.385687316098,-5.61982740336347,
126.626337869861));
#261132=CARTESIAN_POINT('Ctrl Pts',(-180.664134939911,-6.55274284882976,
133.274157224785));
#261133=CARTESIAN_POINT('Ctrl Pts',(-180.942582563724,-1.4640077355066,
137.652354153945));
#261134=CARTESIAN_POINT('Ctrl Pts',(-181.221030187537,4.97007896599344,
135.737579566256));
#261135=CARTESIAN_POINT('Ctrl Pts',(-181.499477811349,6.83690589960112,
129.289417765863));
#261136=CARTESIAN_POINT('Ctrl Pts',(-181.777925435163,2.42095031289641,
124.233414437113));
#261137=CARTESIAN_POINT('Ctrl Pts',(-182.056373058975,-4.21974034136189,
125.215789639631));
#261138=CARTESIAN_POINT('Ctrl Pts',(-182.334820682789,-6.98269576768506,
131.333788554001));
#261139=CARTESIAN_POINT('Ctrl Pts',(-182.613268306601,-3.32889490715784,
136.965269058779));
#261140=CARTESIAN_POINT('Ctrl Pts',(-182.891715930414,3.38399774748988,
136.935175683191));
#261141=CARTESIAN_POINT('Ctrl Pts',(-183.170163554227,6.98716178967534,
131.27116276926));
#261142=CARTESIAN_POINT('Ctrl Pts',(-183.44861117804,4.16946548897866,125.178181482475));
#261143=CARTESIAN_POINT('Ctrl Pts',(-183.727058801853,-2.47976590637605,
124.255383966707));
#261144=CARTESIAN_POINT('Ctrl Pts',(-184.005506425666,-6.85021357707087,
129.350776057783));
#261145=CARTESIAN_POINT('Ctrl Pts',(-184.283954049479,-4.92564962197493,
135.781941347746));
#261146=CARTESIAN_POINT('Ctrl Pts',(-184.562401673291,1.52534570435398,
137.63895311501));
#261147=CARTESIAN_POINT('Ctrl Pts',(-184.840849297105,6.5746228456623,133.215308265529));
#261148=CARTESIAN_POINT('Ctrl Pts',(-185.119296920917,5.58214277998856,
126.576120308909));
#261149=CARTESIAN_POINT('Ctrl Pts',(-185.39774454473,-0.540053797659538,
123.822478634922));
#261150=CARTESIAN_POINT('Ctrl Pts',(-185.676192168543,-6.16596731835295,
127.484845419088));
#261151=CARTESIAN_POINT('Ctrl Pts',(-185.954639792356,-6.12565809773001,
134.197684503321));
#261152=CARTESIAN_POINT('Ctrl Pts',(-186.233087416169,-0.456168340327589,
137.792224709632));
#261153=CARTESIAN_POINT('Ctrl Pts',(-186.511535039982,5.63251783677319,
134.965259191474));
#261154=CARTESIAN_POINT('Ctrl Pts',(-186.789982663795,6.54519528567348,
128.314631155089));
#261155=CARTESIAN_POINT('Ctrl Pts',(-187.068430287608,1.44315801760525,
123.951942864674));
#261156=CARTESIAN_POINT('Ctrl Pts',(-187.346877911421,-4.98507096645316,
125.886291729948));
#261157=CARTESIAN_POINT('Ctrl Pts',(-187.625325535233,-6.83226326659722,
132.340105641921));
#261158=CARTESIAN_POINT('Ctrl Pts',(-187.903773159046,-2.40093939935397,
137.382644901827));
#261159=CARTESIAN_POINT('Ctrl Pts',(-188.182220782859,4.23673048348491,
136.380062271549));
#261160=CARTESIAN_POINT('Ctrl Pts',(-188.460668406672,6.98105202779173,
130.25368220943));
#261161=CARTESIAN_POINT('Ctrl Pts',(-188.739116030485,3.31012780190951,
124.633348702251));
#261162=CARTESIAN_POINT('Ctrl Pts',(-189.017563654298,-3.40264216519462,
124.683873674555));
#261163=CARTESIAN_POINT('Ctrl Pts',(-189.296011278111,-6.98855021079573,
130.358827145076));
#261164=CARTESIAN_POINT('Ctrl Pts',(-189.574458901924,-4.15232202233378,
136.443204111294));
#261165=CARTESIAN_POINT('Ctrl Pts',(-189.852906525736,2.49968725244504,
137.345759379595));
#261166=CARTESIAN_POINT('Ctrl Pts',(-190.13135414955,6.85460605873784,132.237088750687));
#261167=CARTESIAN_POINT('Ctrl Pts',(-190.409801773362,4.91047676317321,
125.8118109601));
#261168=CARTESIAN_POINT('Ctrl Pts',(-190.688249397175,-1.5461407876216,
123.974442405114));
#261169=CARTESIAN_POINT('Ctrl Pts',(-190.966697020988,-6.58193048776853,
128.413435027317));
#261170=CARTESIAN_POINT('Ctrl Pts',(-191.245144644801,-5.56924761483672,
135.049571463749));
#261171=CARTESIAN_POINT('Ctrl Pts',(-191.523592268614,0.561301743259386,
137.784566522618));
#261172=CARTESIAN_POINT('Ctrl Pts',(-191.802039892427,6.17604222041412,
134.105093356759));
#261173=CARTESIAN_POINT('Ctrl Pts',(-192.08048751624,6.11530161344434,127.39240805334));
#261174=CARTESIAN_POINT('Ctrl Pts',(-192.358935140053,0.43489757281158,
123.815140473294));
#261175=CARTESIAN_POINT('Ctrl Pts',(-192.637382763865,-5.64515609130746,
126.660624763449));
#261176=CARTESIAN_POINT('Ctrl Pts',(-192.915830387678,-6.53758708872167,
133.313999870785));
#261177=CARTESIAN_POINT('Ctrl Pts',(-193.194278011491,-1.42229493048546,
137.661139107108));
#261178=CARTESIAN_POINT('Ctrl Pts',(-193.472725635304,5.00001678589681,
135.707233883791));
#261179=CARTESIAN_POINT('Ctrl Pts',(-193.751173259117,6.82755734043935,
129.247827647489));
#261180=CARTESIAN_POINT('Ctrl Pts',(-194.02962088293,2.38090624383734,124.218799169824));
#261181=CARTESIAN_POINT('Ctrl Pts',(-194.308068506743,-4.25368137711504,
125.241579940071));
#261182=CARTESIAN_POINT('Ctrl Pts',(-194.586516130556,-6.97934361638637,
131.376284395991));
#261183=CARTESIAN_POINT('Ctrl Pts',(-194.864963754369,-3.29133003208973,
136.985418839569));
#261184=CARTESIAN_POINT('Ctrl Pts',(-195.143411378181,3.42125506128717,
136.914462738605));
#261185=CARTESIAN_POINT('Ctrl Pts',(-195.421859001994,6.98987389094189,
131.22862128349));
#261186=CARTESIAN_POINT('Ctrl Pts',(-195.700306625807,4.13514008914463,
125.152905002676));
#261187=CARTESIAN_POINT('Ctrl Pts',(-195.97875424962,-2.51958544175274,
124.270600342989));
#261188=CARTESIAN_POINT('Ctrl Pts',(-196.257201873433,-6.85893504027095,
129.392502183704));
#261189=CARTESIAN_POINT('Ctrl Pts',(-196.535649497246,-4.89525841438522,
135.811832952018));
#261190=CARTESIAN_POINT('Ctrl Pts',(-196.814097121059,1.56692154765205,
137.629541273595));
#261191=CARTESIAN_POINT('Ctrl Pts',(-197.092544744872,6.58917715577019,
133.175242000891));
#261192=CARTESIAN_POINT('Ctrl Pts',(-197.370992368684,5.55630085693524,
126.542218560906));
#261193=CARTESIAN_POINT('Ctrl Pts',(-197.649439992498,-0.582544489036021,
123.825895453776));
#261194=CARTESIAN_POINT('Ctrl Pts',(-197.92788761631,-6.18605990846357,
127.522440915193));
#261195=CARTESIAN_POINT('Ctrl Pts',(-198.206335240123,-6.10488847784037,
134.234910252398));
#261196=CARTESIAN_POINT('Ctrl Pts',(-198.484782863936,-0.413622776464342,
137.79487206686));
#261197=CARTESIAN_POINT('Ctrl Pts',(-198.763230487749,5.657742049887,134.930895364888));
#261198=CARTESIAN_POINT('Ctrl Pts',(-199.041678111562,6.52991832845634,
128.274834822558));
#261199=CARTESIAN_POINT('Ctrl Pts',(-199.320125735375,1.40141866741961,
123.943284911633));
#261200=CARTESIAN_POINT('Ctrl Pts',(-199.598573359188,-5.01491628586802,
125.916728392279));
#261201=CARTESIAN_POINT('Ctrl Pts',(-199.877020983,-6.82278816472322,132.381667113854));
#261202=CARTESIAN_POINT('Ctrl Pts',(-200.155468606814,-2.36085103192995,
137.397138221046));
#261203=CARTESIAN_POINT('Ctrl Pts',(-200.433916230626,4.27059286522247,
136.354168785731));
#261204=CARTESIAN_POINT('Ctrl Pts',(-200.712363854439,6.97757054929515,
130.211196767073));
#261205=CARTESIAN_POINT('Ctrl Pts',(-200.990811478252,3.27250177183757,
124.613313349352));
#261206=CARTESIAN_POINT('Ctrl Pts',(-201.269259102065,-3.43983626333961,
124.704699921646));
#261207=CARTESIAN_POINT('Ctrl Pts',(-201.547706725878,-6.9911328178512,
130.401376688499));
#261208=CARTESIAN_POINT('Ctrl Pts',(-201.826154349691,-4.1179198485831,
136.468375999304));
#261209=CARTESIAN_POINT('Ctrl Pts',(-202.104601973504,2.53946028996452,
137.330421876826));
#261210=CARTESIAN_POINT('Ctrl Pts',(-202.383049597317,6.86320048156709,
132.195336272904));
#261211=CARTESIAN_POINT('Ctrl Pts',(-202.66149722113,4.87999471659204,125.782011994664));
#261212=CARTESIAN_POINT('Ctrl Pts',(-202.939944844942,-1.5876877919352,
123.983980745501));
#261213=CARTESIAN_POINT('Ctrl Pts',(-203.218392468755,-6.59636278253501,
128.453545404684));
#261214=CARTESIAN_POINT('Ctrl Pts',(-203.496840092568,-5.54330262622176,
135.083394400798));
#261215=CARTESIAN_POINT('Ctrl Pts',(-203.775287716381,0.603781838200554,
137.781020392543));
#261216=CARTESIAN_POINT('Ctrl Pts',(-204.053735340194,6.19602028969954,
134.067436879861));
#261217=CARTESIAN_POINT('Ctrl Pts',(-204.332182964007,6.09441878738321,
127.355245692268));
#261218=CARTESIAN_POINT('Ctrl Pts',(-204.61063058782,0.392344148371673,
123.812622622391));
#261219=CARTESIAN_POINT('Ctrl Pts',(-204.889078211633,-5.67027559591653,
126.69506520469));
#261220=CARTESIAN_POINT('Ctrl Pts',(-205.167525835445,-6.5221890759199,
133.353749521179));
#261221=CARTESIAN_POINT('Ctrl Pts',(-205.445973459259,-1.38052942180316,
137.66966997982));
#261222=CARTESIAN_POINT('Ctrl Pts',(-205.724421083071,5.02976932833932,
135.676706523556));
#261223=CARTESIAN_POINT('Ctrl Pts',(-206.002868706884,6.8179557836299,129.206295207017));
#261224=CARTESIAN_POINT('Ctrl Pts',(-206.281316330697,2.340773949421,124.204427932937));
#261225=CARTESIAN_POINT('Ctrl Pts',(-206.55976395451,-4.28746479114066,
125.267576371395));
#261226=CARTESIAN_POINT('Ctrl Pts',(-206.838211578323,-6.97573284294384,
131.418759045136));
#261227=CARTESIAN_POINT('Ctrl Pts',(-207.116659202136,-3.253643195576,137.005339578972));
#261228=CARTESIAN_POINT('Ctrl Pts',(-207.395106825949,3.4583855992191,136.893523381939));
#261229=CARTESIAN_POINT('Ctrl Pts',(-207.673554449762,6.99232697986142,
131.186064076586));
#261230=CARTESIAN_POINT('Ctrl Pts',(-207.952002073574,4.10066146017411,
125.127837939644));
#261231=CARTESIAN_POINT('Ctrl Pts',(-208.230449697387,-2.55931161296347,
124.286058830161));
#261232=CARTESIAN_POINT('Ctrl Pts',(-208.5088973212,-6.86740234311116,129.434280626559));
#261233=CARTESIAN_POINT('Ctrl Pts',(-208.787344945013,-4.86468581119477,
135.841539002563));
#261234=CARTESIAN_POINT('Ctrl Pts',(-209.065792568826,1.60843932809579,
137.619876522599));
#261235=CARTESIAN_POINT('Ctrl Pts',(-209.344240192639,6.60348730149562,
133.135087882371));
#261236=CARTESIAN_POINT('Ctrl Pts',(-209.622687816452,5.53025304311036,
126.508474748144));
#261237=CARTESIAN_POINT('Ctrl Pts',(-209.901135440264,-0.625013594012848,
123.829570862223));
#261238=CARTESIAN_POINT('Ctrl Pts',(-210.179583064078,-6.20592327184948,
127.56015802404));
#261239=CARTESIAN_POINT('Ctrl Pts',(-210.45803068789,-6.08389263906328,
134.272008881199));
#261240=CARTESIAN_POINT('Ctrl Pts',(-210.736478311703,-0.371061885656257,
137.797260388114));
#261241=CARTESIAN_POINT('Ctrl Pts',(-211.014925935516,5.68275661328764,
134.896378628042));
#261242=CARTESIAN_POINT('Ctrl Pts',(-211.293373559329,6.51439940271492,
128.235132222534));
#261243=CARTESIAN_POINT('Ctrl Pts',(-211.571821183142,1.35962738715011,
123.934881198276));
#261244=CARTESIAN_POINT('Ctrl Pts',(-211.850268806955,-5.04457577571481,
125.947346167619));
#261245=CARTESIAN_POINT('Ctrl Pts',(-212.128716430768,-6.81306024192543,
132.423170138115));
#261246=CARTESIAN_POINT('Ctrl Pts',(-212.40716405458,-2.32067518230222,
137.411387242468));
#261247=CARTESIAN_POINT('Ctrl Pts',(-212.685611678394,4.30429699857105,
136.32806964973));
#261248=CARTESIAN_POINT('Ctrl Pts',(-212.964059302206,6.97383051435588,
130.168733304621));
#261249=CARTESIAN_POINT('Ctrl Pts',(-213.24250692602,3.23475447800865,124.593507407987));
#261250=CARTESIAN_POINT('Ctrl Pts',(-213.520954549832,-3.47690289708716,
124.725752193909));
#261251=CARTESIAN_POINT('Ctrl Pts',(-213.799402173646,-6.99345636590915,
130.443941164641));
#261252=CARTESIAN_POINT('Ctrl Pts',(-214.077849797458,-4.08336508379785,
136.49333800514));
#261253=CARTESIAN_POINT('Ctrl Pts',(-214.356297421271,2.57913922684953,
137.314842548456));
#261254=CARTESIAN_POINT('Ctrl Pts',(-214.634745045084,6.87154058597789,
132.153532252007));
#261255=CARTESIAN_POINT('Ctrl Pts',(-214.913192668897,4.84933184001288,
125.752399134204));
#261256=CARTESIAN_POINT('Ctrl Pts',(-215.19164029271,-1.62917596389355,
123.993771817573));
#261257=CARTESIAN_POINT('Ctrl Pts',(-215.470087916522,-6.61055064665203,
128.493742892374));
#261258=CARTESIAN_POINT('Ctrl Pts',(-215.748535540335,-5.51715222849034,
135.117058776675));
#261259=CARTESIAN_POINT('Ctrl Pts',(-216.026983164148,0.646239559784443,
137.777215739773));
#261260=CARTESIAN_POINT('Ctrl Pts',(-216.305430787961,6.21576876317433,
134.029659488472));
#261261=CARTESIAN_POINT('Ctrl Pts',(-216.583878411774,6.0733101303926,127.318211139417));
#261262=CARTESIAN_POINT('Ctrl Pts',(-216.862326035587,0.349776185474419,
123.810363852911));
#261263=CARTESIAN_POINT('Ctrl Pts',(-217.1407736594,-5.69518498637811,126.729657917385));
#261264=CARTESIAN_POINT('Ctrl Pts',(-217.419221283213,-6.50654938100331,
133.393404703032));
#261265=CARTESIAN_POINT('Ctrl Pts',(-217.697668907026,-1.33871275709491,
137.67794645597));
#261266=CARTESIAN_POINT('Ctrl Pts',(-217.976116530838,5.05933549082977,
135.64599861675));
#261267=CARTESIAN_POINT('Ctrl Pts',(-218.254564154652,6.80810158496121,
129.164821983446));
#261268=CARTESIAN_POINT('Ctrl Pts',(-218.533011778464,2.30055491676597,
124.190301258982));
#261269=CARTESIAN_POINT('Ctrl Pts',(-218.811459402277,-4.32108933158155,
125.293777970294));
#261270=CARTESIAN_POINT('Ctrl Pts',(-219.08990702609,-6.97186358115499,
131.461210927519));
#261271=CARTESIAN_POINT('Ctrl Pts',(-219.368354649903,-3.21583579411804,
137.02503053882));
#261272=CARTESIAN_POINT('Ctrl Pts',(-219.646802273716,3.49538798540175,
136.872358389107));
#261273=CARTESIAN_POINT('Ctrl Pts',(-219.925249897529,6.99452096553273,
131.143492725519));
#261274=CARTESIAN_POINT('Ctrl Pts',(-220.203697521342,4.06603087968498,
125.102981222246));
#261275=CARTESIAN_POINT('Ctrl Pts',(-220.482145145155,-2.59894294794204,
124.301758855404));
#261276=CARTESIAN_POINT('Ctrl Pts',(-220.760592768967,-6.87561517183164,
129.476109838232));
#261277=CARTESIAN_POINT('Ctrl Pts',(-221.03904039278,-4.83393294528274,
135.87105839861));
#261278=CARTESIAN_POINT('Ctrl Pts',(-221.317488016593,1.64989750722823,
137.609959220154));
#261279=CARTESIAN_POINT('Ctrl Pts',(-221.595935640406,6.61755275257056,
133.094847397895));
#261280=CARTESIAN_POINT('Ctrl Pts',(-221.874383264219,5.5040003037252,126.474890121013));
#261281=CARTESIAN_POINT('Ctrl Pts',(-222.152830888031,-0.667459538880483,
123.83350472407));
#261282=CARTESIAN_POINT('Ctrl Pts',(-222.431278511845,-6.22555667246622,
127.597995348007));
#261283=CARTESIAN_POINT('Ctrl Pts',(-222.709726135657,-6.06267135940695,
134.308979015016));
#261284=CARTESIAN_POINT('Ctrl Pts',(-222.988173759471,-0.328487245014279,
137.799389584896));
#261285=CARTESIAN_POINT('Ctrl Pts',(-223.266621383283,5.70756060005303,
134.861710259961));
#261286=CARTESIAN_POINT('Ctrl Pts',(-223.545069007096,6.49863908350723,
128.195524826214));
#261287=CARTESIAN_POINT('Ctrl Pts',(-223.823516630909,1.31778572538753,
123.926732036005));
#261288=CARTESIAN_POINT('Ctrl Pts',(-224.101964254722,-5.07404833695195,
125.978143921416));
#261289=CARTESIAN_POINT('Ctrl Pts',(-224.380411878535,-6.80307985867417,
132.464613176793));
#261290=CARTESIAN_POINT('Ctrl Pts',(-224.658859502348,-2.28041333920269,
137.425391438088));
#261291=CARTESIAN_POINT('Ctrl Pts',(-224.937307126161,4.33784163461131,
136.30176583066));
#261292=CARTESIAN_POINT('Ctrl Pts',(-225.215754749974,6.96983206156226,
130.126293395573));
#261293=CARTESIAN_POINT('Ctrl Pts',(-225.494202373786,3.19688731916334,
124.573931612073));
#261294=CARTESIAN_POINT('Ctrl Pts',(-225.7726499976,-3.51384069291894,124.747029711241));
#261295=CARTESIAN_POINT('Ctrl Pts',(-226.051097621412,-6.9955207688696,
130.486518996257));
#261296=CARTESIAN_POINT('Ctrl Pts',(-226.329545245225,-4.04865900841799,
136.518089203828));
#261297=CARTESIAN_POINT('Ctrl Pts',(-226.607992869038,2.61872259278156,
137.299021971784));
#261298=CARTESIAN_POINT('Ctrl Pts',(-226.886440492851,6.87962606292594,
132.111678237058));
#261299=CARTESIAN_POINT('Ctrl Pts',(-227.164888116664,4.81848926965818,
125.722973476035));
#261300=CARTESIAN_POINT('Ctrl Pts',(-227.443335740477,-1.67060376613766,
124.003815258517));
#261301=CARTESIAN_POINT('Ctrl Pts',(-227.72178336429,-6.62449355438458,
128.534026000853));
#261302=CARTESIAN_POINT('Ctrl Pts',(-228.000230988102,-5.49079739065326,
135.150563343936));
#261303=CARTESIAN_POINT('Ctrl Pts',(-228.278678611916,0.688673334723007,
137.773152705292));
#261304=CARTESIAN_POINT('Ctrl Pts',(-228.557126235728,6.23528690905198,
133.991762582447));
#261305=CARTESIAN_POINT('Ctrl Pts',(-228.835573859542,6.05197642466173,
127.281305767118));
#261306=CARTESIAN_POINT('Ctrl Pts',(-229.114021483354,0.307195261492642,
123.808364248553));
#261307=CARTESIAN_POINT('Ctrl Pts',(-229.392469107167,-5.7198833396657,
126.764401619687));
#261308=CARTESIAN_POINT('Ctrl Pts',(-229.670916730979,-6.49066858350677,
133.432963946903));
#261309=CARTESIAN_POINT('Ctrl Pts',(-229.949364354793,-1.29684648589306,
137.685968228869));
#261310=CARTESIAN_POINT('Ctrl Pts',(-230.227811978605,5.0887141777831,135.615111301269));
#261311=CARTESIAN_POINT('Ctrl Pts',(-230.506259602419,6.79799510958498,
129.123409513582));
#261312=CARTESIAN_POINT('Ctrl Pts',(-230.784707226231,2.26025063620168,
124.176419671429));
#261313=CARTESIAN_POINT('Ctrl Pts',(-231.063154850045,-4.35455375246839,
125.32018376586));
#261314=CARTESIAN_POINT('Ctrl Pts',(-231.341602473857,-6.96773597439774,
131.503638470075));
#261315=CARTESIAN_POINT('Ctrl Pts',(-231.62005009767,-3.17790922868121,
137.044490989456));
#261316=CARTESIAN_POINT('Ctrl Pts',(-231.898497721483,3.53226084869627,
136.850968544386));
#261317=CARTESIAN_POINT('Ctrl Pts',(-232.176945345296,6.99645576665798,
131.100908807788));
#261318=CARTESIAN_POINT('Ctrl Pts',(-232.455392969109,4.03124963092651,
125.078335771559));
#261319=CARTESIAN_POINT('Ctrl Pts',(-232.733840592922,-2.63847797813309,
124.317699836946));
#261320=CARTESIAN_POINT('Ctrl Pts',(-233.012288216734,-6.88357322210384,
129.517988268725));
#261321=CARTESIAN_POINT('Ctrl Pts',(-233.290735840548,-4.80300095620762,
135.900390046307));
#261322=CARTESIAN_POINT('Ctrl Pts',(-233.56918346436,1.6912945488023,137.599789733751));
#261323=CARTESIAN_POINT('Ctrl Pts',(-233.847631088173,6.63137298779474,
133.05452203859));
#261324=CARTESIAN_POINT('Ctrl Pts',(-234.126078711986,5.47754361158473,
126.441465924004));
#261325=CARTESIAN_POINT('Ctrl Pts',(-234.404526335799,-0.709880750790079,
123.837696893545));
#261326=CARTESIAN_POINT('Ctrl Pts',(-234.682973959612,-6.24495938279112,
127.635951485018));
#261327=CARTESIAN_POINT('Ctrl Pts',(-234.961421583425,-6.04122542523402,
134.345819283911));
#261328=CARTESIAN_POINT('Ctrl Pts',(-235.239869207238,-0.285900432155891,
137.801259578306));
#261329=CARTESIAN_POINT('Ctrl Pts',(-235.518316831051,5.73215309106056,
134.826891545298));
#261330=CARTESIAN_POINT('Ctrl Pts',(-235.796764454864,6.48263795483918,
128.156014101264));
#261331=CARTESIAN_POINT('Ctrl Pts',(-236.075212078676,1.27589523259052,
123.918837726791));
#261332=CARTESIAN_POINT('Ctrl Pts',(-236.353659702489,-5.10333287746112,
126.009120512446));
#261333=CARTESIAN_POINT('Ctrl Pts',(-236.632107326302,-6.79284738479763,
132.505994694203));
#261334=CARTESIAN_POINT('Ctrl Pts',(-236.910554950115,-2.24006699454776,
137.439150288976));
#261335=CARTESIAN_POINT('Ctrl Pts',(-237.189002573928,4.3712255303347,136.275258303218));
#261336=CARTESIAN_POINT('Ctrl Pts',(-237.467450197741,6.96557533907847,
130.083878612554));
#261337=CARTESIAN_POINT('Ctrl Pts',(-237.745897821554,3.15890169848239,
124.554586686994));
#261338=CARTESIAN_POINT('Ctrl Pts',(-238.024345445366,-3.55064828209192,
124.768531685198));
#261339=CARTESIAN_POINT('Ctrl Pts',(-238.30279306918,-6.99732595023538,
130.529108605612));
#261340=CARTESIAN_POINT('Ctrl Pts',(-238.581240692992,-4.01380290848946,
136.542628678202));
#261341=CARTESIAN_POINT('Ctrl Pts',(-238.859688316805,2.65820892098533,
137.282960733047));
#261342=CARTESIAN_POINT('Ctrl Pts',(-239.138135940618,6.88745661279959,
132.069775778975));
#261343=CARTESIAN_POINT('Ctrl Pts',(-239.416583564431,4.78746814841248,
125.693736110535));
#261344=CARTESIAN_POINT('Ctrl Pts',(-239.695031188244,-1.71196966354462,
124.014110696169));
#261345=CARTESIAN_POINT('Ctrl Pts',(-239.973478812057,-6.63819098907155,
128.574393237416));
#261346=CARTESIAN_POINT('Ctrl Pts',(-240.25192643587,-5.46423908930053,
135.183906861057));
#261347=CARTESIAN_POINT('Ctrl Pts',(-240.530374059683,0.731081590618679,
137.768831439659));
#261348=CARTESIAN_POINT('Ctrl Pts',(-240.808821683496,6.25457400407998,
133.95374756607));
#261349=CARTESIAN_POINT('Ctrl Pts',(-241.087269307308,6.03041846071876,
127.244530942912));
#261350=CARTESIAN_POINT('Ctrl Pts',(-241.365716931122,0.264602954276818,
123.806623883412));
#261351=CARTESIAN_POINT('Ctrl Pts',(-241.644164554934,-5.74436974057257,
126.799295024156));
#261352=CARTESIAN_POINT('Ctrl Pts',(-241.922612178747,-6.47454727189872,
133.472425786911));
#261353=CARTESIAN_POINT('Ctrl Pts',(-242.20105980256,-1.25493215956847,
137.693735001267));
#261354=CARTESIAN_POINT('Ctrl Pts',(-242.479507426373,5.11790430056101,
135.584045721651));
#261355=CARTESIAN_POINT('Ctrl Pts',(-242.757955050186,6.78763673199965,
129.082059331979));
#261356=CARTESIAN_POINT('Ctrl Pts',(-243.036402673998,2.21986260121965,
124.162783684665));
#261357=CARTESIAN_POINT('Ctrl Pts',(-243.314850297812,-4.38785681376436,
125.346792779616));
#261358=CARTESIAN_POINT('Ctrl Pts',(-243.593297921624,-6.96335017562108,
131.54604010063));
#261359=CARTESIAN_POINT('Ctrl Pts',(-243.871745545438,-3.13986490465013,
137.063720209766));
#261360=CARTESIAN_POINT('Ctrl Pts',(-244.15019316925,3.56900282276695,136.829354640385));
#261361=CARTESIAN_POINT('Ctrl Pts',(-244.428640793064,6.99813131154132,
131.058313901354));
#261362=CARTESIAN_POINT('Ctrl Pts',(-244.707088416876,3.99631900273028,
125.053902500829));
#261363=CARTESIAN_POINT('Ctrl Pts',(-244.985536040689,-2.67791523855318,
124.333881184089));
#261364=CARTESIAN_POINT('Ctrl Pts',(-245.263983664501,-6.89127619903846,
129.559914366219));
#261365=CARTESIAN_POINT('Ctrl Pts',(-245.542431288315,-4.7718909901659,
135.929532858758));
#261366=CARTESIAN_POINT('Ctrl Pts',(-245.820878912128,1.73262891883438,
137.589368440225));
#261367=CARTESIAN_POINT('Ctrl Pts',(-246.09932653594,6.6449474950541,133.014113298726));
#261368=CARTESIAN_POINT('Ctrl Pts',(-246.377774159753,5.45088394705135,
126.408203395661));
#261369=CARTESIAN_POINT('Ctrl Pts',(-246.656221783566,-0.752275657806765,
123.842147215306));
#261370=CARTESIAN_POINT('Ctrl Pts',(-246.934669407379,-6.26413068384941,
127.674025028594));
#261371=CARTESIAN_POINT('Ctrl Pts',(-247.213117031192,-6.01955563123113,
134.382528322752));
#261372=CARTESIAN_POINT('Ctrl Pts',(-247.491564655005,-0.243303025152602,
137.802870299053));
#261373=CARTESIAN_POINT('Ctrl Pts',(-247.770012278818,5.75653317502817,
134.791923774272));
#261374=CARTESIAN_POINT('Ctrl Pts',(-248.048459902631,6.46639660963695,
128.116601511768));
#261375=CARTESIAN_POINT('Ctrl Pts',(-248.326907526444,1.23395746102625,
123.91119856316));
#261376=CARTESIAN_POINT('Ctrl Pts',(-248.605355150257,-5.13242831209467,
126.040274792862));
#261377=CARTESIAN_POINT('Ctrl Pts',(-248.883802774069,-6.78236319946242,
132.547313156937));
#261378=CARTESIAN_POINT('Ctrl Pts',(-249.162250397883,-2.19963764338714,
137.452663285294));
#261379=CARTESIAN_POINT('Ctrl Pts',(-249.440698021695,4.40444744868852,
136.24854804965));
#261380=CARTESIAN_POINT('Ctrl Pts',(-249.719145645508,6.96106050463867,
130.041490527264));
#261381=CARTESIAN_POINT('Ctrl Pts',(-249.997593269321,3.12079902353814,
124.535473349588));
#261382=CARTESIAN_POINT('Ctrl Pts',(-250.276040893134,-3.58732430068758,
124.790257319018));
#261383=CARTESIAN_POINT('Ctrl Pts',(-250.554488516946,-6.99887184311352,
130.571708414529));
#261384=CARTESIAN_POINT('Ctrl Pts',(-250.83293614076,-3.97879807562073,
136.566955518948));
#261385=CARTESIAN_POINT('Ctrl Pts',(-251.111383764572,2.69759674828547,
137.26665942739));
#261386=CARTESIAN_POINT('Ctrl Pts',(-251.389831388386,6.89503194542569,
132.027826430486));
#261387=CARTESIAN_POINT('Ctrl Pts',(-251.668279012198,4.75626962579305,
125.66468812107));
#261388=CARTESIAN_POINT('Ctrl Pts',(-251.946726636011,-1.75327212332407,
124.024657749096));
#261389=CARTESIAN_POINT('Ctrl Pts',(-252.225174259824,-6.65164244307981,
128.614843106116));
#261390=CARTESIAN_POINT('Ctrl Pts',(-252.503621883637,-5.43747830869239,
135.217088092717));
#261391=CARTESIAN_POINT('Ctrl Pts',(-252.78206950745,0.773462756270139,
137.764252102553));
#261392=CARTESIAN_POINT('Ctrl Pts',(-253.060517131263,6.2736293330892,133.91561584884));
#261393=CARTESIAN_POINT('Ctrl Pts',(-253.338964755075,6.00863703830687,
127.207888027921));
#261394=CARTESIAN_POINT('Ctrl Pts',(-253.617412378889,0.222000840393564,
123.805142824969));
#261395=CARTESIAN_POINT('Ctrl Pts',(-253.895860002702,-5.76864327852066,
126.83433683216));
#261396=CARTESIAN_POINT('Ctrl Pts',(-254.174307626514,-6.45818604965135,
133.511788771436));
#261397=CARTESIAN_POINT('Ctrl Pts',(-254.452755250327,-1.21297131977014,
137.701246465247));
#261398=CARTESIAN_POINT('Ctrl Pts',(-254.73120287414,5.14690475579816,135.55280306703));
#261399=CARTESIAN_POINT('Ctrl Pts',(-255.009650497953,6.7770268770417,129.040772899161));
#261400=CARTESIAN_POINT('Ctrl Pts',(-255.288098121766,2.17939223099114,
124.149393939406));
#261401=CARTESIAN_POINT('Ctrl Pts',(-255.566545745579,-4.42099713522674,
125.37360376984));
#261402=CARTESIAN_POINT('Ctrl Pts',(-255.844993369392,-6.95870662337211,
131.588414730824));
#261403=CARTESIAN_POINT('Ctrl Pts',(-256.123440993205,-3.10170371057109,
137.082716575498));
#261404=CARTESIAN_POINT('Ctrl Pts',(-256.401888617018,3.60561156199617,
136.807519199501));
#261405=CARTESIAN_POINT('Ctrl Pts',(-256.68033624083,6.99954939633056,131.01570633407));
#261406=CARTESIAN_POINT('Ctrl Pts',(-256.958783864643,3.96123678073902,
125.029688453078));
#261407=CARTESIAN_POINT('Ctrl Pts',(-257.237231488456,-2.71724664265218,
124.350290708114));
#261408=CARTESIAN_POINT('Ctrl Pts',(-257.515679112269,-6.89873632689917,
129.601908459729));
#261409=CARTESIAN_POINT('Ctrl Pts',(-257.794126736082,-4.74058057908887,
135.958444437253));
#261410=CARTESIAN_POINT('Ctrl Pts',(-258.072574359895,1.77385448465437,
137.578773744179));
#261411=CARTESIAN_POINT('Ctrl Pts',(-258.351021983707,6.6583599873155,132.973475360041));
#261412=CARTESIAN_POINT('Ctrl Pts',(-258.629469607521,5.42386327951784,
126.375381938049));
#261413=CARTESIAN_POINT('Ctrl Pts',(-258.907917231333,-0.794342416617398,
123.846330221273));
#261414=CARTESIAN_POINT('Ctrl Pts',(-259.186364855146,-6.28363694765996,
127.713206958712));
#261415=CARTESIAN_POINT('Ctrl Pts',(-259.464812478959,-5.99659113747434,
134.41722675292));
#261416=CARTESIAN_POINT('Ctrl Pts',(-259.743260102772,-0.202727240537578,
137.807801967267));
#261417=CARTESIAN_POINT('Ctrl Pts',(-260.021707726585,5.7845923739281,134.749768174183));
#261418=CARTESIAN_POINT('Ctrl Pts',(-260.253747413096,6.33253704604016,
129.202365411857));
#261419=CARTESIAN_POINT('Ctrl Pts',(-260.439389088604,3.82430165355141,
125.973250269562));
#261420=CARTESIAN_POINT('Ctrl Pts',(-260.532214889509,1.97943258085903,
125.138073123498));
#261421=CARTESIAN_POINT('Ctrl Pts',(-260.578632753112,1.00712299976162,
124.970230583726));
#261422=CARTESIAN_POINT('',(-207.496424161897,4.58867628645328,134.536649434892));
#261423=CARTESIAN_POINT('',(-207.098616372022,-3.0618288645252,135.866570130891));
#261424=CARTESIAN_POINT('Ctrl Pts',(-207.495564181254,4.5776766096747,134.540053362101));
#261425=CARTESIAN_POINT('Ctrl Pts',(-207.425200105323,4.24191465405194,
134.818390223685));
#261426=CARTESIAN_POINT('Ctrl Pts',(-207.354706723523,3.87623645141089,
135.064257236424));
#261427=CARTESIAN_POINT('Ctrl Pts',(-207.211655246581,3.02401286069414,
135.53061445367));
#261428=CARTESIAN_POINT('Ctrl Pts',(-207.102465536533,2.31383710832897,
135.85051720249));
#261429=CARTESIAN_POINT('Ctrl Pts',(-207.017121680554,1.17680919028678,
136.083357503381));
#261430=CARTESIAN_POINT('Ctrl Pts',(-207.006414015297,1.01191707037494,
136.112213427934));
#261431=CARTESIAN_POINT('Ctrl Pts',(-206.996499081377,0.830830033328691,
136.138764692487));
#261432=CARTESIAN_POINT('Ctrl Pts',(-206.99566378727,0.815305079975026,
136.140999872962));
#261433=CARTESIAN_POINT('Ctrl Pts',(-206.994721821372,0.797482985899804,
136.143518759038));
#261434=CARTESIAN_POINT('Ctrl Pts',(-206.994601057751,0.795192058160855,
136.14384165627));
#261435=CARTESIAN_POINT('Ctrl Pts',(-206.994400925956,0.791385379449218,
136.144376712743));
#261436=CARTESIAN_POINT('Ctrl Pts',(-206.994321381524,0.789869706459846,
136.144589361887));
#261437=CARTESIAN_POINT('Ctrl Pts',(-206.994102307967,0.785688008384046,
136.145174979795));
#261438=CARTESIAN_POINT('Ctrl Pts',(-206.993963066015,0.783021855901667,
136.145547150697));
#261439=CARTESIAN_POINT('Ctrl Pts',(-206.993788136427,0.779661891522758,
136.146014653447));
#261440=CARTESIAN_POINT('Ctrl Pts',(-206.993752052949,0.778968252786303,
136.146111084266));
#261441=CARTESIAN_POINT('Ctrl Pts',(-206.993692234991,0.777817424895901,
136.146270939059));
#261442=CARTESIAN_POINT('Ctrl Pts',(-206.993668484286,0.777360243378844,
136.146334408072));
#261443=CARTESIAN_POINT('Ctrl Pts',(-206.993631449345,0.776646967855322,
136.146433374546));
#261444=CARTESIAN_POINT('Ctrl Pts',(-206.993618156518,0.776390877127087,
136.146468895845));
#261445=CARTESIAN_POINT('Ctrl Pts',(-206.993593676555,0.775919120366145,
136.146534310839));
#261446=CARTESIAN_POINT('Ctrl Pts',(-206.993582488265,0.775703454517646,
136.146564207738));
#261447=CARTESIAN_POINT('Ctrl Pts',(-206.993558003594,0.77523136736309,
136.14662963406));
#261448=CARTESIAN_POINT('Ctrl Pts',(-206.993544708385,0.774974945987442,
136.146665160236));
#261449=CARTESIAN_POINT('Ctrl Pts',(-206.993507616273,0.774259343522897,
136.146764273078));
#261450=CARTESIAN_POINT('Ctrl Pts',(-206.993483828071,0.773800159351325,
136.146827835603));
#261451=CARTESIAN_POINT('Ctrl Pts',(-206.99334996496,0.771214797369116,
136.147185513093));
#261452=CARTESIAN_POINT('Ctrl Pts',(-206.99324014741,0.769088506791007,
136.147478913998));
#261453=CARTESIAN_POINT('Ctrl Pts',(-206.992930672986,0.763081351255442,
136.148305663398));
#261454=CARTESIAN_POINT('Ctrl Pts',(-206.99273164549,0.759200212159492,
136.148837266646));
#261455=CARTESIAN_POINT('Ctrl Pts',(-206.986814011646,0.64326756001477,
136.164640627143));
#261456=CARTESIAN_POINT('Ctrl Pts',(-206.98184368946,0.530869304321618,
136.177840879035));
#261457=CARTESIAN_POINT('Ctrl Pts',(-206.96770201674,0.152471010400863,
136.215289979218));
#261458=CARTESIAN_POINT('Ctrl Pts',(-206.962007786316,-0.114938494561283,
136.230190105475));
#261459=CARTESIAN_POINT('Ctrl Pts',(-206.956679741253,-1.16160653569181,
136.244166478728));
#261460=CARTESIAN_POINT('Ctrl Pts',(-206.990483565803,-2.08084265314269,
136.163862496972));
#261461=CARTESIAN_POINT('Ctrl Pts',(-207.093821477621,-3.06040702803123,
135.870644567327));
#261462=CARTESIAN_POINT('',(-207.794902692642,5.47563200354658,128.562623629372));
#261463=CARTESIAN_POINT('Ctrl Pts',(-207.496674502688,4.59187829781673,
134.535658549994));
#261464=CARTESIAN_POINT('Ctrl Pts',(-207.504071625027,4.69122528656847,
134.41339833656));
#261465=CARTESIAN_POINT('Ctrl Pts',(-207.511468747366,4.78572386629805,
134.287121160146));
#261466=CARTESIAN_POINT('Ctrl Pts',(-207.518865869706,4.87504241186802,
134.157253703393));
#261467=CARTESIAN_POINT('Ctrl Pts',(-207.526262173893,4.96435107844546,
134.027400610507));
#261468=CARTESIAN_POINT('Ctrl Pts',(-207.53365847808,5.04848063920308,133.89395833482));
#261469=CARTESIAN_POINT('Ctrl Pts',(-207.541054782268,5.12714203594177,
133.757383662816));
#261470=CARTESIAN_POINT('Ctrl Pts',(-207.548451728743,5.20581026355275,
133.620797130813));
#261471=CARTESIAN_POINT('Ctrl Pts',(-207.555848675217,5.27900919514005,
133.481077984293));
#261472=CARTESIAN_POINT('Ctrl Pts',(-207.563245621692,5.34649516678223,
133.338708658794));
#261473=CARTESIAN_POINT('Ctrl Pts',(-207.570644671,5.4140003236014,133.196298859983));
#261474=CARTESIAN_POINT('Ctrl Pts',(-207.578043720307,5.47578912705761,
133.051237719391));
#261475=CARTESIAN_POINT('Ctrl Pts',(-207.585442769615,5.5316656567057,132.904028597253));
#261476=CARTESIAN_POINT('Ctrl Pts',(-207.59284975434,5.58760211345569,132.756661594586));
#261477=CARTESIAN_POINT('Ctrl Pts',(-207.600256739065,5.6376134973471,132.607142358003));
#261478=CARTESIAN_POINT('Ctrl Pts',(-207.60766372379,5.6815532323365,132.455991154528));
#261479=CARTESIAN_POINT('Ctrl Pts',(-207.615074827247,5.72551740048127,
132.304755901825));
#261480=CARTESIAN_POINT('Ctrl Pts',(-207.622485930705,5.763403101635,132.151887235657));
#261481=CARTESIAN_POINT('Ctrl Pts',(-207.629897034162,5.79511482293229,
131.997916125923));
#261482=CARTESIAN_POINT('Ctrl Pts',(-207.637319414593,5.8268747978075,131.843710728783));
#261483=CARTESIAN_POINT('Ctrl Pts',(-207.644741795025,5.85244196061352,
131.688399904348));
#261484=CARTESIAN_POINT('Ctrl Pts',(-207.652164175456,5.87177252105169,
131.532521330268));
#261485=CARTESIAN_POINT('Ctrl Pts',(-207.658588023416,5.88850254215265,
131.397613093029));
#261486=CARTESIAN_POINT('Ctrl Pts',(-207.665011871376,5.90056194097322,
131.262279799072));
#261487=CARTESIAN_POINT('Ctrl Pts',(-207.671435719336,5.90795384954832,
131.126869336994));
#261488=CARTESIAN_POINT('Ctrl Pts',(-207.67885957275,5.91649646233298,130.970379422006));
#261489=CARTESIAN_POINT('Ctrl Pts',(-207.686283426164,5.91883003966297,
130.813313207788));
#261490=CARTESIAN_POINT('Ctrl Pts',(-207.693707279578,5.91489478641788,
130.656204523845));
#261491=CARTESIAN_POINT('Ctrl Pts',(-207.701122589545,5.91096406190258,
130.499276642187));
#261492=CARTESIAN_POINT('Ctrl Pts',(-207.708537899512,5.90077887436122,
130.34230675777));
#261493=CARTESIAN_POINT('Ctrl Pts',(-207.715953209479,5.88433125073,130.185833096608));
#261494=CARTESIAN_POINT('Ctrl Pts',(-207.723359919502,5.86790270231684,
130.029540906599));
#261495=CARTESIAN_POINT('Ctrl Pts',(-207.730766629524,5.84522622595717,
129.873744162186));
#261496=CARTESIAN_POINT('Ctrl Pts',(-207.738173339547,5.81634586531258,
129.718979883648));
#261497=CARTESIAN_POINT('Ctrl Pts',(-207.745575077389,5.78748489227169,
129.564319499536));
#261498=CARTESIAN_POINT('Ctrl Pts',(-207.752976815231,5.75242839154114,
129.410690567196));
#261499=CARTESIAN_POINT('Ctrl Pts',(-207.760378553073,5.71127211818421,
129.258624108794));
#261500=CARTESIAN_POINT('Ctrl Pts',(-207.767776495132,5.67013695072318,
129.106635633615));
#261501=CARTESIAN_POINT('Ctrl Pts',(-207.77517443719,5.62290833687531,128.956208396221));
#261502=CARTESIAN_POINT('Ctrl Pts',(-207.782572379249,5.56973288860237,
128.807862154726));
#261503=CARTESIAN_POINT('Ctrl Pts',(-207.786682483713,5.54018999064428,
128.725444835883));
#261504=CARTESIAN_POINT('Ctrl Pts',(-207.790792588177,5.50881243015012,
128.643669624847));
#261505=CARTESIAN_POINT('Ctrl Pts',(-207.794902692642,5.47563200354658,
128.562623629372));
#261506=CARTESIAN_POINT('Ctrl Pts',(-207.386269723983,2.6533283127961,126.660259061981));
#261507=CARTESIAN_POINT('Ctrl Pts',(-207.393495255289,2.73186345863168,
126.685833507559));
#261508=CARTESIAN_POINT('Ctrl Pts',(-207.401071667583,2.80988843464172,
126.712904578486));
#261509=CARTESIAN_POINT('Ctrl Pts',(-207.437853940591,3.17010229530851,
126.845902326529));
#261510=CARTESIAN_POINT('Ctrl Pts',(-207.471155685021,3.44464862169167,
126.970579878808));
#261511=CARTESIAN_POINT('Ctrl Pts',(-207.539861816086,3.95135827120292,
127.245868129711));
#261512=CARTESIAN_POINT('Ctrl Pts',(-207.575105779606,4.18647404634928,
127.394611394059));
#261513=CARTESIAN_POINT('Ctrl Pts',(-207.673664526471,4.8027720530598,127.846802047319));
#261514=CARTESIAN_POINT('Ctrl Pts',(-207.738601360219,5.1630678639706,128.184811296776));
#261515=CARTESIAN_POINT('Ctrl Pts',(-207.795193373066,5.46743686141374,
128.565993481731));
#261516=CARTESIAN_POINT('',(-178.235140563957,-4.91824875847738,130.800866016629));
#261517=CARTESIAN_POINT('Ctrl Pts',(-178.235140564012,-4.91824875847807,
130.800866017606));
#261518=CARTESIAN_POINT('Ctrl Pts',(-178.242912059243,-4.91834661808309,
130.938592191243));
#261519=CARTESIAN_POINT('Ctrl Pts',(-178.250683554473,-4.91265502275465,
131.076364389796));
#261520=CARTESIAN_POINT('Ctrl Pts',(-178.258455049704,-4.90118910695513,
131.213662951256));
#261521=CARTESIAN_POINT('Ctrl Pts',(-178.266226229677,-4.8897236562809,
131.350955943075));
#261522=CARTESIAN_POINT('Ctrl Pts',(-178.27399740965,-4.87248438266389,
131.487774950232));
#261523=CARTESIAN_POINT('Ctrl Pts',(-178.281768589622,-4.84953840587296,
131.623604361798));
#261524=CARTESIAN_POINT('Ctrl Pts',(-178.289541094918,-4.82658851579851,
131.759456938165));
#261525=CARTESIAN_POINT('Ctrl Pts',(-178.297313600214,-4.79793004946218,
131.894319201245));
#261526=CARTESIAN_POINT('Ctrl Pts',(-178.30508610551,-4.76368139923051,
132.027685018175));
#261527=CARTESIAN_POINT('Ctrl Pts',(-178.31286157721,-4.72941967788061,
132.161101734639));
#261528=CARTESIAN_POINT('Ctrl Pts',(-178.32063704891,-4.68956362187731,
132.293020493378));
#261529=CARTESIAN_POINT('Ctrl Pts',(-178.328412520609,-4.64428160317825,
132.422949957973));
#261530=CARTESIAN_POINT('Ctrl Pts',(-178.33619753434,-4.59894401455087,
132.553038871534));
#261531=CARTESIAN_POINT('Ctrl Pts',(-178.34398254807,-4.54816729194925,
132.68113324938));
#261532=CARTESIAN_POINT('Ctrl Pts',(-178.351767561801,-4.49216835570908,
132.806760808953));
#261533=CARTESIAN_POINT('Ctrl Pts',(-178.359557729245,-4.43613234792204,
132.932471534533));
#261534=CARTESIAN_POINT('Ctrl Pts',(-178.36734789669,-4.37486741040936,
133.055711842143));
#261535=CARTESIAN_POINT('Ctrl Pts',(-178.375138064134,-4.30863618326705,
133.176034562851));
#261536=CARTESIAN_POINT('Ctrl Pts',(-178.38294095569,-4.24229677699919,
133.296553813311));
#261537=CARTESIAN_POINT('Ctrl Pts',(-178.390743847245,-4.17097507715918,
133.414145626664));
#261538=CARTESIAN_POINT('Ctrl Pts',(-178.398546738801,-4.09497718847947,
133.528391617451));
#261539=CARTESIAN_POINT('Ctrl Pts',(-178.403979900142,-4.04205978115932,
133.607941217238));
#261540=CARTESIAN_POINT('Ctrl Pts',(-178.409413061482,-3.98687607958372,
133.685869291158));
#261541=CARTESIAN_POINT('Ctrl Pts',(-178.414846222822,-3.92954049509117,
133.76204460338));
#261542=CARTESIAN_POINT('Ctrl Pts',(-178.422620556941,-3.84749875864512,
133.871044187919));
#261543=CARTESIAN_POINT('Ctrl Pts',(-178.430394891061,-3.76078840842461,
133.976800260166));
#261544=CARTESIAN_POINT('Ctrl Pts',(-178.43816922518,-3.66969498233147,
134.078886812171));
#261545=CARTESIAN_POINT('Ctrl Pts',(-178.445933978127,-3.57871382074449,
134.180847551624));
#261546=CARTESIAN_POINT('Ctrl Pts',(-178.453698731074,-3.48336058895814,
134.279147480063));
#261547=CARTESIAN_POINT('Ctrl Pts',(-178.461463484021,-3.38396310956101,
134.373390840978));
#261548=CARTESIAN_POINT('Ctrl Pts',(-178.469220524906,-3.28466435314195,
134.467540598059));
#261549=CARTESIAN_POINT('Ctrl Pts',(-178.476977565791,-3.18132962460898,
134.557641538328));
#261550=CARTESIAN_POINT('Ctrl Pts',(-178.484734606676,-3.07432564361539,
134.643332472049));
#261551=CARTESIAN_POINT('Ctrl Pts',(-178.492485797916,-2.96740235515608,
134.728958785569));
#261552=CARTESIAN_POINT('Ctrl Pts',(-178.500236989156,-2.856815625741,134.81018146859));
#261553=CARTESIAN_POINT('Ctrl Pts',(-178.507988180396,-2.74296724005992,
134.886677825042));
#261554=CARTESIAN_POINT('Ctrl Pts',(-178.515736077173,-2.6291672429796,
134.963141668503));
#261555=CARTESIAN_POINT('Ctrl Pts',(-178.523483973951,-2.51210867069543,
135.034882963187));
#261556=CARTESIAN_POINT('Ctrl Pts',(-178.531231870728,-2.39222425946025,
135.101620925594));
#261557=CARTESIAN_POINT('Ctrl Pts',(-178.538978146812,-2.27236492545981,
135.168344927857));
#261558=CARTESIAN_POINT('Ctrl Pts',(-178.546724422896,-2.14968126963242,
135.230067489522));
#261559=CARTESIAN_POINT('Ctrl Pts',(-178.55447069898,-2.0246323815396,135.286552802437));
#261560=CARTESIAN_POINT('Ctrl Pts',(-178.562217032245,-1.89958257036413,
135.343038532314));
#261561=CARTESIAN_POINT('Ctrl Pts',(-178.569963365511,-1.77216784838562,
135.394286775354));
#261562=CARTESIAN_POINT('Ctrl Pts',(-178.577709698776,-1.64286875422958,
135.440109243072));
#261563=CARTESIAN_POINT('Ctrl Pts',(-178.585457766779,-1.51354070443772,
135.485941972413));
#261564=CARTESIAN_POINT('Ctrl Pts',(-178.593205834782,-1.38232781119079,
135.526346378023));
#261565=CARTESIAN_POINT('Ctrl Pts',(-178.600953902785,-1.24972691011741,
135.561183686866));
#261566=CARTESIAN_POINT('Ctrl Pts',(-178.608710205527,-1.11698507922857,
135.596058021216));
#261567=CARTESIAN_POINT('Ctrl Pts',(-178.616466508269,-0.982852672395769,
135.625353339897));
#261568=CARTESIAN_POINT('Ctrl Pts',(-178.62422281101,-0.847838434771901,
135.648981660643));
#261569=CARTESIAN_POINT('Ctrl Pts',(-178.631983253525,-0.712752135984214,
135.672622592535));
#261570=CARTESIAN_POINT('Ctrl Pts',(-178.639743696039,-0.576783455982213,
135.690590448432));
#261571=CARTESIAN_POINT('Ctrl Pts',(-178.647504138553,-0.440446459232609,
135.702849157825));
#261572=CARTESIAN_POINT('Ctrl Pts',(-178.655277038818,-0.303890602232393,
135.715127545987));
#261573=CARTESIAN_POINT('Ctrl Pts',(-178.663049939084,-0.166965637712462,
135.721678454702));
#261574=CARTESIAN_POINT('Ctrl Pts',(-178.670822839349,-0.03018673474577,
135.722517978158));
#261575=CARTESIAN_POINT('Ctrl Pts',(-178.678313175112,0.101619910576147,
135.723326982821));
#261576=CARTESIAN_POINT('Ctrl Pts',(-178.685803510874,0.233290621547758,
135.718832649925));
#261577=CARTESIAN_POINT('Ctrl Pts',(-178.693293846636,0.364370681277128,
135.709094766236));
#261578=CARTESIAN_POINT('Ctrl Pts',(-178.701068180755,0.500420681308806,
135.698987667727));
#261579=CARTESIAN_POINT('Ctrl Pts',(-178.708842514874,0.63626532236978,
135.683199534606));
#261580=CARTESIAN_POINT('Ctrl Pts',(-178.716616848993,0.77139185169714,
135.661740330295));
#261581=CARTESIAN_POINT('Ctrl Pts',(-178.72438160194,0.906351849653709,
135.640307572536));
#261582=CARTESIAN_POINT('Ctrl Pts',(-178.732146354887,1.04059511436018,
135.61321771052));
#261583=CARTESIAN_POINT('Ctrl Pts',(-178.739911107835,1.17361148854135,
135.580532634617));
#261584=CARTESIAN_POINT('Ctrl Pts',(-178.74766814872,1.30649574898521,135.547880021992));
#261585=CARTESIAN_POINT('Ctrl Pts',(-178.755425189605,1.43815516668883,
135.509643347339));
#261586=CARTESIAN_POINT('Ctrl Pts',(-178.76318223049,1.56808764156665,135.465935910411));
#261587=CARTESIAN_POINT('Ctrl Pts',(-178.77093342173,1.6979221333539,135.422261433602));
#261588=CARTESIAN_POINT('Ctrl Pts',(-178.77868461297,1.82603190540451,135.373124530313));
#261589=CARTESIAN_POINT('Ctrl Pts',(-178.78643580421,1.95192828993981,135.318688808275));
#261590=CARTESIAN_POINT('Ctrl Pts',(-178.794183700987,2.07777116515346,
135.264276222872));
#261591=CARTESIAN_POINT('Ctrl Pts',(-178.801931597764,2.20140216582424,
135.204569452893));
#261592=CARTESIAN_POINT('Ctrl Pts',(-178.809679494541,2.32235115632627,
135.139780801263));
#261593=CARTESIAN_POINT('Ctrl Pts',(-178.817425770625,2.44327484690683,
135.075005702023));
#261594=CARTESIAN_POINT('Ctrl Pts',(-178.82517204671,2.56151729879949,135.005151020031));
#261595=CARTESIAN_POINT('Ctrl Pts',(-178.832918322794,2.6766319708055,134.93047554027));
#261596=CARTESIAN_POINT('Ctrl Pts',(-178.840664656059,2.79174749256172,
134.855799509272));
#261597=CARTESIAN_POINT('Ctrl Pts',(-178.848410989325,2.90373486036354,
134.77630282227));
#261598=CARTESIAN_POINT('Ctrl Pts',(-178.85615732259,3.01217591891128,134.692287995493));
#261599=CARTESIAN_POINT('Ctrl Pts',(-178.863905390593,3.12064126208234,
134.608254354177));
#261600=CARTESIAN_POINT('Ctrl Pts',(-178.871653458596,3.22555840668735,
134.519700799111));
#261601=CARTESIAN_POINT('Ctrl Pts',(-178.879401526599,3.32654204724801,
134.426970321963));
#261602=CARTESIAN_POINT('Ctrl Pts',(-178.887157829341,3.42763301442343,
134.334141289761));
#261603=CARTESIAN_POINT('Ctrl Pts',(-178.894914132082,3.52478183797542,
134.23712673239));
#261604=CARTESIAN_POINT('Ctrl Pts',(-178.902670434824,3.61763950674951,
134.136307114991));
#261605=CARTESIAN_POINT('Ctrl Pts',(-178.910430877338,3.71054673645731,
134.035433687128));
#261606=CARTESIAN_POINT('Ctrl Pts',(-178.918191319852,3.79915799525986,
133.93075145081));
#261607=CARTESIAN_POINT('Ctrl Pts',(-178.925951762367,3.88316507161623,
133.822673406042));
#261608=CARTESIAN_POINT('Ctrl Pts',(-178.933724662632,3.96730700358959,
133.714421864802));
#261609=CARTESIAN_POINT('Ctrl Pts',(-178.941497562898,4.04682975652453,
133.60276394041));
#261610=CARTESIAN_POINT('Ctrl Pts',(-178.949270463163,4.12146840944813,
133.488141758498));
#261611=CARTESIAN_POINT('Ctrl Pts',(-178.956760798925,4.19339375933312,
133.377686381616));
#261612=CARTESIAN_POINT('Ctrl Pts',(-178.964251134687,4.26078378529405,
133.264478786661));
#261613=CARTESIAN_POINT('Ctrl Pts',(-178.971741470449,4.32344300204487,
133.14893385604));
#261614=CARTESIAN_POINT('Ctrl Pts',(-178.979515804568,4.38847796204466,
133.029008004254));
#261615=CARTESIAN_POINT('Ctrl Pts',(-178.987290138687,4.44862230519032,
132.906184188811));
#261616=CARTESIAN_POINT('Ctrl Pts',(-178.995064472806,4.50360725859762,
132.780899188606));
#261617=CARTESIAN_POINT('Ctrl Pts',(-179.002829225753,4.55852444796399,
132.655768590966));
#261618=CARTESIAN_POINT('Ctrl Pts',(-179.0105939787,4.60829474347329,132.528183198275));
#261619=CARTESIAN_POINT('Ctrl Pts',(-179.018358731647,4.65269446277708,
132.398605673554));
#261620=CARTESIAN_POINT('Ctrl Pts',(-179.026115772532,4.69705008365385,
132.269156847057));
#261621=CARTESIAN_POINT('Ctrl Pts',(-179.033872813417,4.73604561757761,
132.137720193522));
#261622=CARTESIAN_POINT('Ctrl Pts',(-179.041629854302,4.76950498948021,
132.004779385256));
#261623=CARTESIAN_POINT('Ctrl Pts',(-179.049381045542,4.80293912941014,
131.871938828688));
#261624=CARTESIAN_POINT('Ctrl Pts',(-179.057132236782,4.83084532209175,
131.737596752741));
#261625=CARTESIAN_POINT('Ctrl Pts',(-179.064883428023,4.85309707847332,
131.602252721433));
#261626=CARTESIAN_POINT('Ctrl Pts',(-179.0726313248,4.87533937726481,131.466966214949));
#261627=CARTESIAN_POINT('Ctrl Pts',(-179.080379221577,4.89193195641557,
131.330678985081));
#261628=CARTESIAN_POINT('Ctrl Pts',(-179.088127118354,4.90279931259945,
131.193901325162));
#261629=CARTESIAN_POINT('Ctrl Pts',(-179.095873394438,4.91366439556669,
131.057152276181));
#261630=CARTESIAN_POINT('Ctrl Pts',(-179.103619670522,4.91880660669958,
130.919913390691));
#261631=CARTESIAN_POINT('Ctrl Pts',(-179.111365946606,4.91820230270907,
130.782700236056));
#261632=CARTESIAN_POINT('Ctrl Pts',(-179.119112279871,4.91759799425773,
130.645486068543));
#261633=CARTESIAN_POINT('Ctrl Pts',(-179.126858613137,4.91124708775985,
130.508298023225));
#261634=CARTESIAN_POINT('Ctrl Pts',(-179.134604946402,4.89917807553393,
130.371651423409));
#261635=CARTESIAN_POINT('Ctrl Pts',(-179.142353014405,4.88710636053639,
130.234974222535));
#261636=CARTESIAN_POINT('Ctrl Pts',(-179.150101082408,4.86931402609475,
130.098839097816));
#261637=CARTESIAN_POINT('Ctrl Pts',(-179.157849150411,4.84588137379236,
129.963755613041));
#261638=CARTESIAN_POINT('Ctrl Pts',(-179.165605453153,4.82242381698827,
129.828528559931));
#261639=CARTESIAN_POINT('Ctrl Pts',(-179.173361755895,4.79331403439889,
129.694355765308));
#261640=CARTESIAN_POINT('Ctrl Pts',(-179.181118058636,4.75868347306896,
129.561736512842));
#261641=CARTESIAN_POINT('Ctrl Pts',(-179.188878501151,4.72403442836585,
129.429046477489));
#261642=CARTESIAN_POINT('Ctrl Pts',(-179.196638943665,4.68385884803004,
129.297912010122));
#261643=CARTESIAN_POINT('Ctrl Pts',(-179.204399386179,4.63833760479553,
129.16881565443));
#261644=CARTESIAN_POINT('Ctrl Pts',(-179.212172286444,4.59274328682007,
129.039512061807));
#261645=CARTESIAN_POINT('Ctrl Pts',(-179.21994518671,4.54178630312496,128.912253482031));
#261646=CARTESIAN_POINT('Ctrl Pts',(-179.227718086975,4.48569543026932,
128.787501780324));
#261647=CARTESIAN_POINT('Ctrl Pts',(-179.235208422737,4.43164360192636,
128.667285117205));
#261648=CARTESIAN_POINT('Ctrl Pts',(-179.242698758499,4.37282480120875,
128.549396509455));
#261649=CARTESIAN_POINT('Ctrl Pts',(-179.250189094261,4.30948241586416,
128.434224678457));
#261650=CARTESIAN_POINT('Ctrl Pts',(-179.25796342838,4.24373838472681,128.314686072481));
#261651=CARTESIAN_POINT('Ctrl Pts',(-179.265737762499,4.17291271682093,
128.197695660831));
#261652=CARTESIAN_POINT('Ctrl Pts',(-179.273512096618,4.09722760829128,
128.083715659407));
#261653=CARTESIAN_POINT('Ctrl Pts',(-179.281276849565,4.02163577489393,
127.969876128149));
#261654=CARTESIAN_POINT('Ctrl Pts',(-179.289041602512,3.94119663104747,
127.859039947773));
#261655=CARTESIAN_POINT('Ctrl Pts',(-179.29680635546,3.85617852248092,127.751645389239));
#261656=CARTESIAN_POINT('Ctrl Pts',(-179.304563396344,3.77124485509857,
127.644357496495));
#261657=CARTESIAN_POINT('Ctrl Pts',(-179.31232043723,3.6817415146055,127.540504727641));
#261658=CARTESIAN_POINT('Ctrl Pts',(-179.320077478115,3.58798025533687,
127.440496656314));
#261659=CARTESIAN_POINT('Ctrl Pts',(-179.327828669355,3.49428970216282,
127.340564001851));
#261660=CARTESIAN_POINT('Ctrl Pts',(-179.335579860595,3.39634788769476,
127.244470558066));
#261661=CARTESIAN_POINT('Ctrl Pts',(-179.343331051835,3.29450673886711,
127.152592770336));
#261662=CARTESIAN_POINT('Ctrl Pts',(-179.351078948612,3.19270887524427,
127.060754033117));
#261663=CARTESIAN_POINT('Ctrl Pts',(-179.358826845389,3.08701526322851,
126.973127649607));
#261664=CARTESIAN_POINT('Ctrl Pts',(-179.366574742166,2.97781441566159,
126.890052968903));
#261665=CARTESIAN_POINT('Ctrl Pts',(-179.37432101825,2.86863641055788,126.806995665632));
#261666=CARTESIAN_POINT('Ctrl Pts',(-179.382067294334,2.75595294011129,
126.728488407918));
#261667=CARTESIAN_POINT('Ctrl Pts',(-179.389813570418,2.64018498597006,
126.654829764282));
#261668=CARTESIAN_POINT('Ctrl Pts',(-179.397559903684,2.52441617725656,
126.581170576914));
#261669=CARTESIAN_POINT('Ctrl Pts',(-179.405306236949,2.40556316927225,
126.512360284919));
#261670=CARTESIAN_POINT('Ctrl Pts',(-179.413052570214,2.28407491890505,
126.448653461738));
#261671=CARTESIAN_POINT('Ctrl Pts',(-179.420800638217,2.16255946208602,
126.384932371855));
#261672=CARTESIAN_POINT('Ctrl Pts',(-179.42854870622,2.03840793474619,126.326317206531));
#261673=CARTESIAN_POINT('Ctrl Pts',(-179.436296774223,1.9120924522984,126.273015837441));
#261674=CARTESIAN_POINT('Ctrl Pts',(-179.444053076965,1.78564272025286,
126.219657819023));
#261675=CARTESIAN_POINT('Ctrl Pts',(-179.451809379707,1.65702479963027,
126.1716250307));
#261676=CARTESIAN_POINT('Ctrl Pts',(-179.459565682449,1.52672980226203,
126.129076757373));
#261677=CARTESIAN_POINT('Ctrl Pts',(-179.467326124963,1.39636526253059,
126.08650577475));
#261678=CARTESIAN_POINT('Ctrl Pts',(-179.475086567477,1.26432223869915,
126.049425245569));
#261679=CARTESIAN_POINT('Ctrl Pts',(-179.482847009991,1.13110447457022,
126.017943823125));
#261680=CARTESIAN_POINT('Ctrl Pts',(-179.490619910257,0.997672857459797,
125.986411863907));
#261681=CARTESIAN_POINT('Ctrl Pts',(-179.498392810522,0.863063115764055,
125.960497046634));
#261682=CARTESIAN_POINT('Ctrl Pts',(-179.506165710787,0.727787489092654,
125.940256544541));
#261683=CARTESIAN_POINT('Ctrl Pts',(-179.51365604655,0.597429472185839,
125.920751835681));
#261684=CARTESIAN_POINT('Ctrl Pts',(-179.521146382312,0.466453449186646,
125.906516086481));
#261685=CARTESIAN_POINT('Ctrl Pts',(-179.528636718074,0.335318019426584,
125.897554641338));
#261686=CARTESIAN_POINT('Ctrl Pts',(-179.536411052193,0.199210549992686,
125.888253420279));
#261687=CARTESIAN_POINT('Ctrl Pts',(-179.544185386312,0.0625001998143731,
125.884604885428));
#261688=CARTESIAN_POINT('Ctrl Pts',(-179.551959720431,-0.074304053336741,
125.886671935862));
#261689=CARTESIAN_POINT('Ctrl Pts',(-179.559724473378,-0.210939707472022,
125.888736438841));
#261690=CARTESIAN_POINT('Ctrl Pts',(-179.567489226326,-0.347668647150042,
125.896502505897));
#261691=CARTESIAN_POINT('Ctrl Pts',(-179.575253979273,-0.483977095179842,
125.909981266326));
#261692=CARTESIAN_POINT('Ctrl Pts',(-179.583011020158,-0.620150159737818,
125.923446639461));
#261693=CARTESIAN_POINT('Ctrl Pts',(-179.590768061043,-0.75590317721648,
125.942613376373));
#261694=CARTESIAN_POINT('Ctrl Pts',(-179.598525101928,-0.890723050881356,
125.967440573868));
#261695=CARTESIAN_POINT('Ctrl Pts',(-179.606276293168,-1.0254412558302,
125.99224904898));
#261696=CARTESIAN_POINT('Ctrl Pts',(-179.614027484408,-1.15922733467526,
126.02270941777));
#261697=CARTESIAN_POINT('Ctrl Pts',(-179.621778675648,-1.29157434815609,
126.058729072062));
#261698=CARTESIAN_POINT('Ctrl Pts',(-179.629526572425,-1.42386511062591,
126.09473341704));
#261699=CARTESIAN_POINT('Ctrl Pts',(-179.637274469202,-1.55471764778564,
126.136292245547));
#261700=CARTESIAN_POINT('Ctrl Pts',(-179.645022365979,-1.68363645494728,
126.183262117201));
#261701=CARTESIAN_POINT('Ctrl Pts',(-179.652768642063,-1.81252829507363,
126.230222163771));
#261702=CARTESIAN_POINT('Ctrl Pts',(-179.660514918148,-1.9394868426528,
126.282590868379));
#261703=CARTESIAN_POINT('Ctrl Pts',(-179.668261194232,-2.06403335266789,
126.340175430819));
#261704=CARTESIAN_POINT('Ctrl Pts',(-179.676007527497,-2.18858078205719,
126.397760418335));
#261705=CARTESIAN_POINT('Ctrl Pts',(-179.683753860762,-2.31071578348326,
126.460561176436));
#261706=CARTESIAN_POINT('Ctrl Pts',(-179.691500194028,-2.429981504936,126.528337588141));
#261707=CARTESIAN_POINT('Ctrl Pts',(-179.699248262031,-2.54927393512061,
126.596129177904));
#261708=CARTESIAN_POINT('Ctrl Pts',(-179.706996330034,-2.66569546687332,
126.668898445397));
#261709=CARTESIAN_POINT('Ctrl Pts',(-179.714744398037,-2.77881602195207,
126.746360546269));
#261710=CARTESIAN_POINT('Ctrl Pts',(-179.722500700779,-2.89205680290245,
126.823904974785));
#261711=CARTESIAN_POINT('Ctrl Pts',(-179.73025700352,-3.00198927584127,
126.906151978699));
#261712=CARTESIAN_POINT('Ctrl Pts',(-179.738013306262,-3.10821397193136,
126.992774469098));
#261713=CARTESIAN_POINT('Ctrl Pts',(-179.745773748776,-3.21449536334011,
127.079443192529));
#261714=CARTESIAN_POINT('Ctrl Pts',(-179.753534191291,-3.31706474242677,
127.170491796366));
#261715=CARTESIAN_POINT('Ctrl Pts',(-179.761294633805,-3.41555841026557,
127.265555196444));
#261716=CARTESIAN_POINT('Ctrl Pts',(-179.76906753407,-3.51421018888385,
127.36077120073));
#261717=CARTESIAN_POINT('Ctrl Pts',(-179.776840434336,-3.60877291201382,
127.460014597025));
#261718=CARTESIAN_POINT('Ctrl Pts',(-179.784613334601,-3.69892160017226,
127.562885327165));
#261719=CARTESIAN_POINT('Ctrl Pts',(-179.792103670363,-3.78579315644455,
127.662016447149));
#261720=CARTESIAN_POINT('Ctrl Pts',(-179.799594006125,-3.86856583511938,
127.764515514558));
#261721=CARTESIAN_POINT('Ctrl Pts',(-179.807084341887,-3.94698725566329,
127.869999585564));
#261722=CARTESIAN_POINT('Ctrl Pts',(-179.81489938152,-4.02880822192404,
127.980056360295));
#261723=CARTESIAN_POINT('Ctrl Pts',(-179.822714421154,-4.10615277853036,
128.093713091792));
#261724=CARTESIAN_POINT('Ctrl Pts',(-179.830529460787,-4.17868931704032,
128.210572142352));
#261725=CARTESIAN_POINT('Ctrl Pts',(-179.838331509096,-4.25110527449914,
128.327236932372));
#261726=CARTESIAN_POINT('Ctrl Pts',(-179.846133557405,-4.31872893195353,
128.447093113703));
#261727=CARTESIAN_POINT('Ctrl Pts',(-179.853935605714,-4.38126988870761,
128.569711377796));
#261728=CARTESIAN_POINT('Ctrl Pts',(-179.861730173332,-4.44375088049264,
128.692212074126));
#261729=CARTESIAN_POINT('Ctrl Pts',(-179.86952474095,-4.50115869139553,
128.817469244293));
#261730=CARTESIAN_POINT('Ctrl Pts',(-179.877319308568,-4.55324684430206,
128.945025726441));
#261731=CARTESIAN_POINT('Ctrl Pts',(-179.885106751938,-4.60528738855242,
129.072465621758));
#261732=CARTESIAN_POINT('Ctrl Pts',(-179.892894195309,-4.65201781159595,
129.202200288788));
#261733=CARTESIAN_POINT('Ctrl Pts',(-179.900681638679,-4.6932383823034,
129.333749673307));
#261734=CARTESIAN_POINT('Ctrl Pts',(-179.90555036806,-4.71900958783941,
129.415994682738));
#261735=CARTESIAN_POINT('Ctrl Pts',(-179.910419097441,-4.74262803915595,
129.498948563585));
#261736=CARTESIAN_POINT('Ctrl Pts',(-179.915287826822,-4.76405452823417,
129.582490119309));
#261737=CARTESIAN_POINT('Ctrl Pts',(-178.165366640417,-4.76405452823403,
129.582490119308));
#261738=CARTESIAN_POINT('Ctrl Pts',(-178.174286102188,-4.80301964378508,
129.734414513464));
#261739=CARTESIAN_POINT('Ctrl Pts',(-178.18320556396,-4.83475684527663,
129.888373267217));
#261740=CARTESIAN_POINT('Ctrl Pts',(-178.192125025732,-4.85907467737619,
130.043718558394));
#261741=CARTESIAN_POINT('Ctrl Pts',(-178.200980669897,-4.88321851850083,
130.197952373904));
#261742=CARTESIAN_POINT('Ctrl Pts',(-178.209836314062,-4.90004869699476,
130.353552808266));
#261743=CARTESIAN_POINT('Ctrl Pts',(-178.218691958226,-4.9094252417917,
130.509866376946));
#261744=CARTESIAN_POINT('Ctrl Pts',(-178.224174826803,-4.91523061990645,
130.606646095947));
#261745=CARTESIAN_POINT('Ctrl Pts',(-178.22965769538,-4.91817971751586,
130.70369880656));
#261746=CARTESIAN_POINT('Ctrl Pts',(-178.235140563957,-4.91824875847738,
130.80086601663));
#261747=CARTESIAN_POINT('',(-178.485270545702,-2.29572256715808,125.351142443209));
#261748=CARTESIAN_POINT('Ctrl Pts',(-178.48283591081,-2.30474777596774,
125.357501197005));
#261749=CARTESIAN_POINT('Ctrl Pts',(-178.439259969146,-2.35809653341986,
125.471388554306));
#261750=CARTESIAN_POINT('Ctrl Pts',(-178.397030602778,-2.41201111853674,
125.585847534594));
#261751=CARTESIAN_POINT('Ctrl Pts',(-178.311610003403,-2.52439778012099,
125.826246106787));
#261752=CARTESIAN_POINT('Ctrl Pts',(-178.268672143037,-2.58283994140754,
125.952273103513));
#261753=CARTESIAN_POINT('Ctrl Pts',(-178.183448400479,-2.70162741425541,
126.21363850387));
#261754=CARTESIAN_POINT('Ctrl Pts',(-178.141394739096,-2.76182193325093,
126.348942022816));
#261755=CARTESIAN_POINT('Ctrl Pts',(-178.059030111423,-2.88183628638349,
126.627709334455));
#261756=CARTESIAN_POINT('Ctrl Pts',(-178.018924422453,-2.94145364433504,
126.771074158801));
#261757=CARTESIAN_POINT('Ctrl Pts',(-177.980719892801,-2.99891973414341,
126.915872442133));
#261758=CARTESIAN_POINT('',(-178.811624764632,-5.91430460988513,130.800157362323));
#261759=CARTESIAN_POINT('Ctrl Pts',(-178.485270545702,-2.29572256715808,
125.351142443209));
#261760=CARTESIAN_POINT('Ctrl Pts',(-178.492676155995,-2.44062366529699,
125.412143619096));
#261761=CARTESIAN_POINT('Ctrl Pts',(-178.500081766289,-2.58322966273536,
125.478982251567));
#261762=CARTESIAN_POINT('Ctrl Pts',(-178.507487376582,-2.72303992747434,
125.551458170739));
#261763=CARTESIAN_POINT('Ctrl Pts',(-178.514887922563,-2.86275458323872,
125.623884527396));
#261764=CARTESIAN_POINT('Ctrl Pts',(-178.522288468545,-2.99967698309288,
125.701940323268));
#261765=CARTESIAN_POINT('Ctrl Pts',(-178.529689014526,-3.13332760890747,
125.785377786577));
#261766=CARTESIAN_POINT('Ctrl Pts',(-178.537322090704,-3.27117762843923,
125.871436911829));
#261767=CARTESIAN_POINT('Ctrl Pts',(-178.544955166882,-3.40554653031744,
125.963221272439));
#261768=CARTESIAN_POINT('Ctrl Pts',(-178.55258824306,-3.53593626550598,
126.060408121094));
#261769=CARTESIAN_POINT('Ctrl Pts',(-178.559984666331,-3.6622834483718,
126.154581826727));
#261770=CARTESIAN_POINT('Ctrl Pts',(-178.567381089602,-3.78489421730117,
126.253827766868));
#261771=CARTESIAN_POINT('Ctrl Pts',(-178.574777512873,-3.90334590563519,
126.357808998225));
#261772=CARTESIAN_POINT('Ctrl Pts',(-178.582174070057,-4.02179973853031,
126.461792112157));
#261773=CARTESIAN_POINT('Ctrl Pts',(-178.58957062724,-4.13609406001072,
126.570510442079));
#261774=CARTESIAN_POINT('Ctrl Pts',(-178.596967184423,-4.24584063293858,
126.683587888794));
#261775=CARTESIAN_POINT('Ctrl Pts',(-178.604365335927,-4.35561086164749,
126.796689709258));
#261776=CARTESIAN_POINT('Ctrl Pts',(-178.611763487432,-4.46083113010824,
126.91415224943));
#261777=CARTESIAN_POINT('Ctrl Pts',(-178.619161638937,-4.56115140711873,
127.03556393907));
#261778=CARTESIAN_POINT('Ctrl Pts',(-178.62656284585,-4.66151311601725,
127.157025771272));
#261779=CARTESIAN_POINT('Ctrl Pts',(-178.633964052763,-4.7569705667546,
127.282439712767));
#261780=CARTESIAN_POINT('Ctrl Pts',(-178.641365259675,-4.84721530679233,
127.411362779061));
#261781=CARTESIAN_POINT('Ctrl Pts',(-178.648774778471,-4.9375613956671,
127.540430631664));
#261782=CARTESIAN_POINT('Ctrl Pts',(-178.656184297267,-5.02268287156556,
127.673015171635));
#261783=CARTESIAN_POINT('Ctrl Pts',(-178.663593816062,-5.10231539881571,
127.808645655573));
#261784=CARTESIAN_POINT('Ctrl Pts',(-178.67100831022,-5.18200139790702,
127.944367212995));
#261785=CARTESIAN_POINT('Ctrl Pts',(-178.678422804377,-5.25619092940608,
128.083138461444));
#261786=CARTESIAN_POINT('Ctrl Pts',(-178.685837298534,-5.32466681106959,
128.224466450436));
#261787=CARTESIAN_POINT('Ctrl Pts',(-178.693261769769,-5.393234835119,128.365984612928));
#261788=CARTESIAN_POINT('Ctrl Pts',(-178.700686241004,-5.45607371265313,
128.510066043443));
#261789=CARTESIAN_POINT('Ctrl Pts',(-178.708110712239,-5.51301510408258,
128.656199770549));
#261790=CARTESIAN_POINT('Ctrl Pts',(-178.709701422424,-5.52521492929238,
128.687509260591));
#261791=CARTESIAN_POINT('Ctrl Pts',(-178.71129213261,-5.53714422039791,
128.718912912318));
#261792=CARTESIAN_POINT('Ctrl Pts',(-178.712882842796,-5.54880162463143,
128.750405629503));
#261793=CARTESIAN_POINT('Ctrl Pts',(-178.721434613827,-5.6114726584305,
128.919712715677));
#261794=CARTESIAN_POINT('Ctrl Pts',(-178.729986384858,-5.66643819996979,
129.092017853483));
#261795=CARTESIAN_POINT('Ctrl Pts',(-178.738538155888,-5.71344087978109,
129.266659776783));
#261796=CARTESIAN_POINT('Ctrl Pts',(-178.747059185309,-5.76027459598887,
129.440673903352));
#261797=CARTESIAN_POINT('Ctrl Pts',(-178.75558021473,-5.79920250282132,
129.617007918382));
#261798=CARTESIAN_POINT('Ctrl Pts',(-178.764101244151,-5.8300165114818,
129.79498554439));
#261799=CARTESIAN_POINT('Ctrl Pts',(-178.772561766365,-5.86061171211978,
129.971699364288));
#261800=CARTESIAN_POINT('Ctrl Pts',(-178.781022288578,-5.88320776267822,
130.150033394033));
#261801=CARTESIAN_POINT('Ctrl Pts',(-178.789482810792,-5.89764813416367,
130.329305833256));
#261802=CARTESIAN_POINT('Ctrl Pts',(-178.796863453485,-5.91024537338731,
130.485696394633));
#261803=CARTESIAN_POINT('Ctrl Pts',(-178.804244096178,-5.91663666015527,
130.642800748583));
#261804=CARTESIAN_POINT('Ctrl Pts',(-178.811624738871,-5.91674850538075,
130.800155076613));
#261805=CARTESIAN_POINT('',(-180.561624807791,-5.90996050472777,130.808431327307));
#261806=CARTESIAN_POINT('Ctrl Pts',(-178.811624807791,-5.91021030986751,
130.800161191611));
#261807=CARTESIAN_POINT('Ctrl Pts',(-178.871526694064,-5.90189013011824,
132.075856832088));
#261808=CARTESIAN_POINT('Ctrl Pts',(-179.024244454939,-4.86928404315109,
135.340473970702));
#261809=CARTESIAN_POINT('Ctrl Pts',(-179.269778090423,0.518479272423054,
137.783525307874));
#261810=CARTESIAN_POINT('Ctrl Pts',(-179.548225714233,6.15201962547423,
134.140558312264));
#261811=CARTESIAN_POINT('Ctrl Pts',(-179.826673338048,6.13215448558245,
127.431788617551));
#261812=CARTESIAN_POINT('Ctrl Pts',(-180.10512096186,0.477138945842835,
123.822247831545));
#261813=CARTESIAN_POINT('Ctrl Pts',(-180.350104785108,-4.88402996107005,
126.29162117749));
#261814=CARTESIAN_POINT('Ctrl Pts',(-180.502272733752,-5.90199055707381,
129.544310586215));
#261815=CARTESIAN_POINT('Ctrl Pts',(-180.561624807791,-5.90996050472777,
130.808431327307));
#261816=CARTESIAN_POINT('',(-182.311624807792,-5.92507812272359,130.807023572335));
#261817=CARTESIAN_POINT('Ctrl Pts',(-180.561624807791,-5.90996050472777,
130.808431327307));
#261818=CARTESIAN_POINT('Ctrl Pts',(-180.595088608356,-5.9144541090899,
131.521166055697));
#261819=CARTESIAN_POINT('Ctrl Pts',(-180.721368283525,-5.46467200361853,
134.2052756912));
#261820=CARTESIAN_POINT('Ctrl Pts',(-180.9404638333,-1.46310027610978,137.648109452265));
#261821=CARTESIAN_POINT('Ctrl Pts',(-181.218911457112,4.96699828222215,
135.734521730019));
#261822=CARTESIAN_POINT('Ctrl Pts',(-181.497359080924,6.83266807054414,
129.290356797193));
#261823=CARTESIAN_POINT('Ctrl Pts',(-181.775806704738,2.41944969642949,
124.23748741209));
#261824=CARTESIAN_POINT('Ctrl Pts',(-182.047228613693,-4.04967250708035,
125.19448203293));
#261825=CARTESIAN_POINT('Ctrl Pts',(-182.225834648045,-5.91491065230807,
128.991748760208));
#261826=CARTESIAN_POINT('Ctrl Pts',(-182.311624807792,-5.92507812272359,
130.807023572335));
#261827=CARTESIAN_POINT('',(-184.061624807792,-5.91793140692411,130.798997977614));
#261828=CARTESIAN_POINT('Ctrl Pts',(-182.311624807792,-5.92507812272359,
130.807023572335));
#261829=CARTESIAN_POINT('Ctrl Pts',(-182.318650522649,-5.92591077938457,
130.955684016088));
#261830=CARTESIAN_POINT('Ctrl Pts',(-182.325676237506,-5.920802909146,131.104286291747));
#261831=CARTESIAN_POINT('Ctrl Pts',(-182.425517826968,-5.76118888251318,
133.209457008152));
#261832=CARTESIAN_POINT('Ctrl Pts',(-182.611149576176,-3.32683150482748,
136.961450244072));
#261833=CARTESIAN_POINT('Ctrl Pts',(-182.88959719999,3.38190018988211,136.931375521743));
#261834=CARTESIAN_POINT('Ctrl Pts',(-183.168044823802,6.98283082510118,
131.270873423793));
#261835=CARTESIAN_POINT('Ctrl Pts',(-183.446492447615,4.16688106229984,
125.181668847338));
#261836=CARTESIAN_POINT('Ctrl Pts',(-183.724940071428,-2.47822883329544,
124.259443323958));
#261837=CARTESIAN_POINT('Ctrl Pts',(-183.929984191486,-5.69455770389321,
128.0092781062));
#261838=CARTESIAN_POINT('Ctrl Pts',(-184.042212436941,-5.92199600856727,
130.386992623478));
#261839=CARTESIAN_POINT('Ctrl Pts',(-184.061624807792,-5.9181658456461,
130.798997765173));
#261840=CARTESIAN_POINT('',(-185.811624807754,-5.91674999671234,130.804163375351));
#261841=CARTESIAN_POINT('Ctrl Pts',(-184.061624807792,-5.91674757076024,
130.798999050368));
#261842=CARTESIAN_POINT('Ctrl Pts',(-184.068928931162,-5.91688801138847,
130.953982046063));
#261843=CARTESIAN_POINT('Ctrl Pts',(-184.076233054531,-5.91093487072381,
131.109156665659));
#261844=CARTESIAN_POINT('Ctrl Pts',(-184.083537177901,-5.89886979863471,
131.263997062221));
#261845=CARTESIAN_POINT('Ctrl Pts',(-184.090835650274,-5.88681406095517,
131.41871766309));
#261846=CARTESIAN_POINT('Ctrl Pts',(-184.098134122647,-5.86865583195702,
131.57310417378));
#261847=CARTESIAN_POINT('Ctrl Pts',(-184.10543259502,-5.84442882662681,
131.726630780259));
#261848=CARTESIAN_POINT('Ctrl Pts',(-184.112782708521,-5.8200304005078,
131.881243680798));
#261849=CARTESIAN_POINT('Ctrl Pts',(-184.120132822023,-5.78947697807806,
132.034984065929));
#261850=CARTESIAN_POINT('Ctrl Pts',(-184.127482935524,-5.75285625138199,
132.187319587831));
#261851=CARTESIAN_POINT('Ctrl Pts',(-184.134776202234,-5.71651875443688,
132.338476925796));
#261852=CARTESIAN_POINT('Ctrl Pts',(-184.142069468944,-5.67420758047763,
132.488250678532));
#261853=CARTESIAN_POINT('Ctrl Pts',(-184.149362735654,-5.62605967323285,
132.636131104205));
#261854=CARTESIAN_POINT('Ctrl Pts',(-184.1566557956,-5.57791313097582,132.784007337485));
#261855=CARTESIAN_POINT('Ctrl Pts',(-184.163948855547,-5.52393030354824,
132.929989984487));
#261856=CARTESIAN_POINT('Ctrl Pts',(-184.171241915494,-5.46429776820347,
133.073585256712));
#261857=CARTESIAN_POINT('Ctrl Pts',(-184.178536303616,-5.40465437287707,
133.217206679795));
#261858=CARTESIAN_POINT('Ctrl Pts',(-184.185830691739,-5.33935937028289,
133.358439507777));
#261859=CARTESIAN_POINT('Ctrl Pts',(-184.193125079861,-5.26864703532705,
133.49681098473));
#261860=CARTESIAN_POINT('Ctrl Pts',(-184.200517599794,-5.19698340338551,
133.637043980879));
#261861=CARTESIAN_POINT('Ctrl Pts',(-184.207910119727,-5.11975580564257,
133.774337715552));
#261862=CARTESIAN_POINT('Ctrl Pts',(-184.215302639659,-5.03725512909461,
133.908227774342));
#261863=CARTESIAN_POINT('Ctrl Pts',(-184.222607901079,-4.95572825936504,
134.040537445459));
#261864=CARTESIAN_POINT('Ctrl Pts',(-184.2299131625,-4.86905238698824,134.16952307254));
#261865=CARTESIAN_POINT('Ctrl Pts',(-184.23721842392,-4.7775502821432,134.294768024172));
#261866=CARTESIAN_POINT('Ctrl Pts',(-184.244654573109,-4.68440874160218,
134.422256979315));
#261867=CARTESIAN_POINT('Ctrl Pts',(-184.252090722298,-4.58626664978123,
134.545869616373));
#261868=CARTESIAN_POINT('Ctrl Pts',(-184.259526871487,-4.48350479392226,
134.665204479389));
#261869=CARTESIAN_POINT('Ctrl Pts',(-184.266963020676,-4.38074293806359,
134.784539342404));
#261870=CARTESIAN_POINT('Ctrl Pts',(-184.274399169865,-4.27336164917223,
134.899596175744));
#261871=CARTESIAN_POINT('Ctrl Pts',(-184.281835319054,-4.161777721421,135.010015948187));
#261872=CARTESIAN_POINT('Ctrl Pts',(-184.289258585459,-4.05038710764862,
135.120244423497));
#261873=CARTESIAN_POINT('Ctrl Pts',(-184.296681851865,-3.93444578121529,
135.226211097442));
#261874=CARTESIAN_POINT('Ctrl Pts',(-184.30410511827,-3.81431332688993,
135.327517082559));
#261875=CARTESIAN_POINT('Ctrl Pts',(-184.311519610991,-3.6943228591492,
135.428703332415));
#261876=CARTESIAN_POINT('Ctrl Pts',(-184.318934103712,-3.57015140620211,
135.525239619935));
#261877=CARTESIAN_POINT('Ctrl Pts',(-184.326348596433,-3.44219618145469,
135.616762929393));
#261878=CARTESIAN_POINT('Ctrl Pts',(-184.333755942787,-3.31436428477031,
135.70819802524));
#261879=CARTESIAN_POINT('Ctrl Pts',(-184.341163289141,-3.18275617821301,
135.794629546266));
#261880=CARTESIAN_POINT('Ctrl Pts',(-184.348570635494,-3.04780293399889,
135.8757339856));
#261881=CARTESIAN_POINT('Ctrl Pts',(-184.35597245717,-2.91295034300579,
135.956777934184));
#261882=CARTESIAN_POINT('Ctrl Pts',(-184.363374278845,-2.77475790068248,
136.032502520666));
#261883=CARTESIAN_POINT('Ctrl Pts',(-184.370776100521,-2.63368641439405,
136.102626978663));
#261884=CARTESIAN_POINT('Ctrl Pts',(-184.378174014832,-2.49268939864553,
136.172714418505));
#261885=CARTESIAN_POINT('Ctrl Pts',(-184.385571929143,-2.34881669916657,
136.237207451659));
#261886=CARTESIAN_POINT('Ctrl Pts',(-184.392969843455,-2.20255442484518,
136.295870844097));
#261887=CARTESIAN_POINT('Ctrl Pts',(-184.400366528367,-2.05631645666011,
136.354524487743));
#261888=CARTESIAN_POINT('Ctrl Pts',(-184.407763213279,-1.90769004789607,
136.407350274588));
#261889=CARTESIAN_POINT('Ctrl Pts',(-184.415159898191,-1.75718213247968,
136.454160748172));
#261890=CARTESIAN_POINT('Ctrl Pts',(-184.422556255127,-1.60668089074197,
136.50096914613));
#261891=CARTESIAN_POINT('Ctrl Pts',(-184.429952612062,-1.45429866469017,
136.541762650303));
#261892=CARTESIAN_POINT('Ctrl Pts',(-184.437348968997,-1.30055816731291,
136.576403498205));
#261893=CARTESIAN_POINT('Ctrl Pts',(-184.444746458334,-1.14679413187302,
136.611049649709));
#261894=CARTESIAN_POINT('Ctrl Pts',(-184.45214394767,-0.991671775233469,
136.63954118726));
#261895=CARTESIAN_POINT('Ctrl Pts',(-184.459541437007,-0.835724485702392,
136.661791380836));
#261896=CARTESIAN_POINT('Ctrl Pts',(-184.466941519522,-0.679722529091387,
136.684049374182));
#261897=CARTESIAN_POINT('Ctrl Pts',(-184.474341602037,-0.522895433160513,
136.70006161478));
#261898=CARTESIAN_POINT('Ctrl Pts',(-184.481741684552,-0.365782046711605,
136.709793206022));
#261899=CARTESIAN_POINT('Ctrl Pts',(-184.489149904218,-0.208495897941526,
136.71953549815));
#261900=CARTESIAN_POINT('Ctrl Pts',(-184.496558123885,-0.0509232027779254,
136.722983325656));
#261901=CARTESIAN_POINT('Ctrl Pts',(-184.503966343551,0.106396107174741,
136.720153922853));
#261902=CARTESIAN_POINT('Ctrl Pts',(-184.511379122853,0.263812244537669,
136.717322778599));
#261903=CARTESIAN_POINT('Ctrl Pts',(-184.518791902155,0.420974314123582,
136.708206727033));
#261904=CARTESIAN_POINT('Ctrl Pts',(-184.526204681458,0.577347679482734,
136.692874880052));
#261905=CARTESIAN_POINT('Ctrl Pts',(-184.533628052486,0.733944478439272,
136.677521126208));
#261906=CARTESIAN_POINT('Ctrl Pts',(-184.541051423515,0.889749953635859,
136.655933889856));
#261907=CARTESIAN_POINT('Ctrl Pts',(-184.548474794544,1.04423900632314,
136.628233509394));
#261908=CARTESIAN_POINT('Ctrl Pts',(-184.552410843985,1.1261528089723,136.613546103012));
#261909=CARTESIAN_POINT('Ctrl Pts',(-184.556346893425,1.20769674862925,
136.59714091264));
#261910=CARTESIAN_POINT('Ctrl Pts',(-184.560282942866,1.28879442450105,
136.579041517311));
#261911=CARTESIAN_POINT('Ctrl Pts',(-184.567706209272,1.44174211022288,
136.544906622583));
#261912=CARTESIAN_POINT('Ctrl Pts',(-184.575129475677,1.59356399310633,
136.504639476673));
#261913=CARTESIAN_POINT('Ctrl Pts',(-184.582552742083,1.74373011348117,
136.458327000013));
#261914=CARTESIAN_POINT('Ctrl Pts',(-184.589967234804,1.89371874997225,
136.412069260854));
#261915=CARTESIAN_POINT('Ctrl Pts',(-184.597381727525,2.04205516608679,
136.359780522206));
#261916=CARTESIAN_POINT('Ctrl Pts',(-184.604796220246,2.18821924286488,
136.301598752089));
#261917=CARTESIAN_POINT('Ctrl Pts',(-184.612203566599,2.33424244120238,
136.243473059753));
#261918=CARTESIAN_POINT('Ctrl Pts',(-184.619610912953,2.47809712401023,
136.179465780693));
#261919=CARTESIAN_POINT('Ctrl Pts',(-184.627018259307,2.6192781107327,136.109764724808));
#261920=CARTESIAN_POINT('Ctrl Pts',(-184.634420080982,2.76035379934881,
136.040115654599));
#261921=CARTESIAN_POINT('Ctrl Pts',(-184.641821902658,2.89875942920178,
135.964781427729));
#261922=CARTESIAN_POINT('Ctrl Pts',(-184.649223724333,3.03400970594374,
135.883997973396));
#261923=CARTESIAN_POINT('Ctrl Pts',(-184.656621638644,3.16918858511778,
135.803257164018));
#261924=CARTESIAN_POINT('Ctrl Pts',(-184.664019552956,3.30121510880317,
135.71707304701));
#261925=CARTESIAN_POINT('Ctrl Pts',(-184.671417467267,3.42962861422033,
135.625727449806));
#261926=CARTESIAN_POINT('Ctrl Pts',(-184.678814152179,3.55802077964237,
135.534397032583));
#261927=CARTESIAN_POINT('Ctrl Pts',(-184.686210837092,3.68280081455794,
135.437907053702));
#261928=CARTESIAN_POINT('Ctrl Pts',(-184.693607522004,3.80353699636812,
135.336582686238));
#261929=CARTESIAN_POINT('Ctrl Pts',(-184.701003878939,3.92426782460947,
135.235262811603));
#261930=CARTESIAN_POINT('Ctrl Pts',(-184.708400235875,4.04095487032625,
135.129109214579));
#261931=CARTESIAN_POINT('Ctrl Pts',(-184.71579659281,4.15319969089864,135.018487204419));
#261932=CARTESIAN_POINT('Ctrl Pts',(-184.723194082147,4.2654616964396,134.907848257747));
#261933=CARTESIAN_POINT('Ctrl Pts',(-184.730591571483,4.37327985674116,
134.792739797803));
#261934=CARTESIAN_POINT('Ctrl Pts',(-184.73798906082,4.47629289397063,134.673563699583));
#261935=CARTESIAN_POINT('Ctrl Pts',(-184.745389143335,4.57934204226076,
134.554345824366));
#261936=CARTESIAN_POINT('Ctrl Pts',(-184.75278922585,4.67758246983172,134.431057754148));
#261937=CARTESIAN_POINT('Ctrl Pts',(-184.760189308365,4.77069355624095,
134.304133975219));
#261938=CARTESIAN_POINT('Ctrl Pts',(-184.767597528031,4.86390702786161,
134.177070630548));
#261939=CARTESIAN_POINT('Ctrl Pts',(-184.775005747698,4.95197967345292,
134.046363894402));
#261940=CARTESIAN_POINT('Ctrl Pts',(-184.782413967364,5.03463414650848,
133.912477342097));
#261941=CARTESIAN_POINT('Ctrl Pts',(-184.789826746667,5.11733949201328,
133.778508384854));
#261942=CARTESIAN_POINT('Ctrl Pts',(-184.797239525968,5.194619837159,133.641356036106));
#261943=CARTESIAN_POINT('Ctrl Pts',(-184.804652305271,5.26624434368106,
133.501507457311));
#261944=CARTESIAN_POINT('Ctrl Pts',(-184.812075676299,5.3379711906568,133.361459056308));
#261945=CARTESIAN_POINT('Ctrl Pts',(-184.819499047328,5.4040259024361,133.21870706884));
#261946=CARTESIAN_POINT('Ctrl Pts',(-184.826922418357,5.46422589442022,
133.073758321197));
#261947=CARTESIAN_POINT('Ctrl Pts',(-184.830858467798,5.49614537464935,
132.9969030172));
#261948=CARTESIAN_POINT('Ctrl Pts',(-184.834794517239,5.52641971457611,
132.919430385207));
#261949=CARTESIAN_POINT('Ctrl Pts',(-184.838730566679,5.55502745541382,
132.841417448413));
#261950=CARTESIAN_POINT('Ctrl Pts',(-184.846153833085,5.60898076181651,
132.69428748432));
#261951=CARTESIAN_POINT('Ctrl Pts',(-184.85357709949,5.65716630769147,132.544790058487));
#261952=CARTESIAN_POINT('Ctrl Pts',(-184.861000365896,5.69937076551409,
132.39341802361));
#261953=CARTESIAN_POINT('Ctrl Pts',(-184.868414858617,5.74152534117242,
132.242224897908));
#261954=CARTESIAN_POINT('Ctrl Pts',(-184.875829351338,5.7777128006819,132.089161929462));
#261955=CARTESIAN_POINT('Ctrl Pts',(-184.883243844059,5.80776808344369,
131.93474128417));
#261956=CARTESIAN_POINT('Ctrl Pts',(-184.890651190412,5.83779439779231,
131.78046947531));
#261957=CARTESIAN_POINT('Ctrl Pts',(-184.898058536766,5.86170023104261,
131.624842958691));
#261958=CARTESIAN_POINT('Ctrl Pts',(-184.90546588312,5.87937053055049,131.468388272859));
#261959=CARTESIAN_POINT('Ctrl Pts',(-184.912867704795,5.89702765088234,
131.312050276835));
#261960=CARTESIAN_POINT('Ctrl Pts',(-184.920269526471,5.9084584559214,131.154885710824));
#261961=CARTESIAN_POINT('Ctrl Pts',(-184.927671348146,5.91359912613479,
130.997430392202));
#261962=CARTESIAN_POINT('Ctrl Pts',(-184.935069262458,5.91873708262841,
130.840058193015));
#261963=CARTESIAN_POINT('Ctrl Pts',(-184.942467176769,5.91759150510721,
130.682395919046));
#261964=CARTESIAN_POINT('Ctrl Pts',(-184.94986509108,5.91015050348987,130.52498347355));
#261965=CARTESIAN_POINT('Ctrl Pts',(-184.957261775993,5.90271073843201,
130.367597187147));
#261966=CARTESIAN_POINT('Ctrl Pts',(-184.964658460905,5.88897764325531,
130.210461019335));
#261967=CARTESIAN_POINT('Ctrl Pts',(-184.972055145817,5.86899143866611,
130.054113954552));
#261968=CARTESIAN_POINT('Ctrl Pts',(-184.979451502752,5.84900612028617,
129.897773822362));
#261969=CARTESIAN_POINT('Ctrl Pts',(-184.986847859688,5.82276829113332,
129.742223093914));
#261970=CARTESIAN_POINT('Ctrl Pts',(-184.994244216623,5.79036992825915,
129.587994448844));
#261971=CARTESIAN_POINT('Ctrl Pts',(-185.00164170596,5.75796660511301,129.433742190975));
#261972=CARTESIAN_POINT('Ctrl Pts',(-185.009039195297,5.71940094696954,
129.280812784864));
#261973=CARTESIAN_POINT('Ctrl Pts',(-185.016436684633,5.67481578315034,
129.129727407037));
#261974=CARTESIAN_POINT('Ctrl Pts',(-185.023836767148,5.63021499007076,
128.978589066463));
#261975=CARTESIAN_POINT('Ctrl Pts',(-185.031236849663,5.57959059565481,
128.829296399002));
#261976=CARTESIAN_POINT('Ctrl Pts',(-185.038636932178,5.52313484234269,
128.682354002166));
#261977=CARTESIAN_POINT('Ctrl Pts',(-185.046045151844,5.46661701012626,
128.535250027059));
#261978=CARTESIAN_POINT('Ctrl Pts',(-185.053453371511,5.40425514743527,
128.3905018324));
#261979=CARTESIAN_POINT('Ctrl Pts',(-185.060861591177,5.33628936075163,
128.248593331441));
#261980=CARTESIAN_POINT('Ctrl Pts',(-185.06827437048,5.26828174226036,128.106597488167));
#261981=CARTESIAN_POINT('Ctrl Pts',(-185.075687149781,5.19466350113199,
127.967445150473));
#261982=CARTESIAN_POINT('Ctrl Pts',(-185.083099929084,5.11571972637515,
127.831593851794));
#261983=CARTESIAN_POINT('Ctrl Pts',(-185.090523300112,5.03666315305096,
127.69554844241));
#261984=CARTESIAN_POINT('Ctrl Pts',(-185.097946671141,4.95226604824019,
127.562813806486));
#261985=CARTESIAN_POINT('Ctrl Pts',(-185.10537004217,4.86285612782121,127.433817509607));
#261986=CARTESIAN_POINT('Ctrl Pts',(-185.109306091611,4.81544884265258,
127.365420577777));
#261987=CARTESIAN_POINT('Ctrl Pts',(-185.113242141051,4.76663294343972,
127.298074068215));
#261988=CARTESIAN_POINT('Ctrl Pts',(-185.117178190492,4.71646163297881,
127.231837667725));
#261989=CARTESIAN_POINT('Ctrl Pts',(-185.124601456898,4.62184010724392,
127.10691788357));
#261990=CARTESIAN_POINT('Ctrl Pts',(-185.132024723303,4.52210915344613,
126.9855710088));
#261991=CARTESIAN_POINT('Ctrl Pts',(-185.139447989709,4.41756811377999,
126.868242920823));
#261992=CARTESIAN_POINT('Ctrl Pts',(-185.14686248243,4.31315063294114,126.751053504903));
#261993=CARTESIAN_POINT('Ctrl Pts',(-185.154276975151,4.20393462841209,
126.637873697119));
#261994=CARTESIAN_POINT('Ctrl Pts',(-185.161691467872,4.09026178058174,
126.529119205808));
#261995=CARTESIAN_POINT('Ctrl Pts',(-185.169098814225,3.97669849492183,
126.420469536169));
#261996=CARTESIAN_POINT('Ctrl Pts',(-185.176506160579,3.85868718572215,
126.316236947986));
#261997=CARTESIAN_POINT('Ctrl Pts',(-185.183913506933,3.73660865600951,
126.21680284525));
#261998=CARTESIAN_POINT('Ctrl Pts',(-185.191315328609,3.61462117706974,
126.11744290422));
#261999=CARTESIAN_POINT('Ctrl Pts',(-185.198717150284,3.48857280588916,
126.022874557316));
#262000=CARTESIAN_POINT('Ctrl Pts',(-185.206118971959,3.35887984478284,
125.933441120098));
#262001=CARTESIAN_POINT('Ctrl Pts',(-185.213516886271,3.2292553475808,125.844054894095));
#262002=CARTESIAN_POINT('Ctrl Pts',(-185.220914800582,3.09599039862963,
125.759798390713));
#262003=CARTESIAN_POINT('Ctrl Pts',(-185.228312714894,2.95953280695017,
125.68097344431));
#262004=CARTESIAN_POINT('Ctrl Pts',(-185.235709399806,2.82309789204744,
125.602161597183));
#262005=CARTESIAN_POINT('Ctrl Pts',(-185.243106084718,2.68347171034644,
125.52877970213));
#262006=CARTESIAN_POINT('Ctrl Pts',(-185.25050276963,2.54112946499453,125.461085254585));
#262007=CARTESIAN_POINT('Ctrl Pts',(-185.257899126566,2.39879353124695,
125.393393808683));
#262008=CARTESIAN_POINT('Ctrl Pts',(-185.265295483501,2.25374211042627,
125.33138946918));
#262009=CARTESIAN_POINT('Ctrl Pts',(-185.272691840437,2.10647307683844,
125.275282779531));
#262010=CARTESIAN_POINT('Ctrl Pts',(-185.280089329773,1.95918149598603,
125.219167499804));
#262011=CARTESIAN_POINT('Ctrl Pts',(-185.28748681911,1.80967197519407,125.168951800726));
#262012=CARTESIAN_POINT('Ctrl Pts',(-185.294884308446,1.65846019776952,
125.124797224583));
#262013=CARTESIAN_POINT('Ctrl Pts',(-185.302284390961,1.50719541329015,
125.080627170122));
#262014=CARTESIAN_POINT('Ctrl Pts',(-185.309684473476,1.35422754221607,
125.042522573463));
#262015=CARTESIAN_POINT('Ctrl Pts',(-185.317084555991,1.2000850284593,125.010594442877));
#262016=CARTESIAN_POINT('Ctrl Pts',(-185.324492775658,1.04577301916263,
124.97863120403));
#262017=CARTESIAN_POINT('Ctrl Pts',(-185.331900995324,0.890284153455571,
124.952858070407));
#262018=CARTESIAN_POINT('Ctrl Pts',(-185.339309214991,0.734155344681294,
124.933334600559));
#262019=CARTESIAN_POINT('Ctrl Pts',(-185.346721994293,0.577930441230811,
124.913799114341));
#262020=CARTESIAN_POINT('Ctrl Pts',(-185.354134773595,0.421065180974498,
124.900520988071));
#262021=CARTESIAN_POINT('Ctrl Pts',(-185.361547552897,0.264098597322687,
124.89350767629));
#262022=CARTESIAN_POINT('Ctrl Pts',(-185.368970923926,0.106907732454928,
124.88648434356));
#262023=CARTESIAN_POINT('Ctrl Pts',(-185.376394294955,-0.0503843726528677,
124.885743705147));
#262024=CARTESIAN_POINT('Ctrl Pts',(-185.383817665983,-0.207240856527645,
124.891241154044));
#262025=CARTESIAN_POINT('Ctrl Pts',(-185.387753715424,-0.290409927994593,
124.894156033358));
#262026=CARTESIAN_POINT('Ctrl Pts',(-185.391689764865,-0.373456639755591,
124.898823798456));
#262027=CARTESIAN_POINT('Ctrl Pts',(-185.395625814305,-0.456302018202181,
124.905231950493));
#262028=CARTESIAN_POINT('Ctrl Pts',(-185.403049080711,-0.612545816442367,
124.917317525243));
#262029=CARTESIAN_POINT('Ctrl Pts',(-185.410472347116,-0.768545395500247,
124.935633051325));
#262030=CARTESIAN_POINT('Ctrl Pts',(-185.417895613522,-0.923763824315242,
124.960167691303));
#262031=CARTESIAN_POINT('Ctrl Pts',(-185.425310106243,-1.07879879783747,
124.984673333373));
#262032=CARTESIAN_POINT('Ctrl Pts',(-185.432724598964,-1.23305409374088,
125.015383400464));
#262033=CARTESIAN_POINT('Ctrl Pts',(-185.440139091685,-1.38599527823421,
125.052235127696));
#262034=CARTESIAN_POINT('Ctrl Pts',(-185.447546438038,-1.53878905225622,
125.089051335846));
#262035=CARTESIAN_POINT('Ctrl Pts',(-185.454953784392,-1.69027087592442,
125.131997332593));
#262036=CARTESIAN_POINT('Ctrl Pts',(-185.462361130746,-1.83991402991944,
125.180958895743));
#262037=CARTESIAN_POINT('Ctrl Pts',(-185.469762952421,-1.98944557440407,
125.229883941511));
#262038=CARTESIAN_POINT('Ctrl Pts',(-185.477164774097,-2.1371408264938,
125.284815504598));
#262039=CARTESIAN_POINT('Ctrl Pts',(-185.484566595772,-2.28248592351566,
125.345588908523));
#262040=CARTESIAN_POINT('Ctrl Pts',(-185.491964510084,-2.42775429399301,
125.40633023064));
#262041=CARTESIAN_POINT('Ctrl Pts',(-185.499362424395,-2.57067463664222,
125.472907108294));
#262042=CARTESIAN_POINT('Ctrl Pts',(-185.506760338706,-2.7107509579538,
125.545105935916));
#262043=CARTESIAN_POINT('Ctrl Pts',(-185.514157023618,-2.85080400112102,
125.617292765403));
#262044=CARTESIAN_POINT('Ctrl Pts',(-185.521553708531,-2.98801362948039,
125.695099519758));
#262045=CARTESIAN_POINT('Ctrl Pts',(-185.528950393443,-3.12190634592099,
125.778265579686));
#262046=CARTESIAN_POINT('Ctrl Pts',(-185.536346750378,-3.25579312541823,
125.861427951945));
#262047=CARTESIAN_POINT('Ctrl Pts',(-185.543743107314,-3.38636296832752,
125.949948960309));
#262048=CARTESIAN_POINT('Ctrl Pts',(-185.551139464249,-3.51316962525318,
126.043523532903));
#262049=CARTESIAN_POINT('Ctrl Pts',(-185.558536953586,-3.6399956966021,
126.137112432005));
#262050=CARTESIAN_POINT('Ctrl Pts',(-185.565934442922,-3.7630571343807,
126.235756214237));
#262051=CARTESIAN_POINT('Ctrl Pts',(-185.573331932259,-3.88193928906325,
126.339108338184));
#262052=CARTESIAN_POINT('Ctrl Pts',(-185.580732014774,-4.00086311770033,
126.442496692057));
#262053=CARTESIAN_POINT('Ctrl Pts',(-185.588132097289,-4.1156044648104,
126.550596429015));
#262054=CARTESIAN_POINT('Ctrl Pts',(-185.595532179804,-4.22578429914888,
126.66302295691));
#262055=CARTESIAN_POINT('Ctrl Pts',(-185.60294039947,-4.33608528754245,
126.775573109331));
#262056=CARTESIAN_POINT('Ctrl Pts',(-185.610348619137,-4.44181448473375,
126.892459287456));
#262057=CARTESIAN_POINT('Ctrl Pts',(-185.617756838803,-4.54263156765102,
127.013261963735));
#262058=CARTESIAN_POINT('Ctrl Pts',(-185.625169618105,-4.64351070180004,
127.134138992044));
#262059=CARTESIAN_POINT('Ctrl Pts',(-185.632582397407,-4.73947147030228,
127.258937026566));
#262060=CARTESIAN_POINT('Ctrl Pts',(-185.639995176709,-4.8302162407166,
127.387206592589));
#262061=CARTESIAN_POINT('Ctrl Pts',(-185.647418547738,-4.92109067151479,
127.515659436183));
#262062=CARTESIAN_POINT('Ctrl Pts',(-185.654841918766,-5.00673401647177,
127.6475934058));
#262063=CARTESIAN_POINT('Ctrl Pts',(-185.662265289795,-5.08689361798639,
127.7825327135));
#262064=CARTESIAN_POINT('Ctrl Pts',(-185.666201339236,-5.12939616211485,
127.854080772271));
#262065=CARTESIAN_POINT('Ctrl Pts',(-185.670137388677,-5.17035781537923,
127.926473363939));
#262066=CARTESIAN_POINT('Ctrl Pts',(-185.674073438118,-5.20974640624689,
127.999637289839));
#262067=CARTESIAN_POINT('Ctrl Pts',(-185.681900715772,-5.288075055757,128.145131997376));
#262068=CARTESIAN_POINT('Ctrl Pts',(-185.689727993426,-5.36039597288839,
128.294079034415));
#262069=CARTESIAN_POINT('Ctrl Pts',(-185.69755527108,-5.42640910216598,
128.445968195082));
#262070=CARTESIAN_POINT('Ctrl Pts',(-185.705369342796,-5.49231085616024,
128.597601093116));
#262071=CARTESIAN_POINT('Ctrl Pts',(-185.713183414512,-5.55192591167538,
128.752165934091));
#262072=CARTESIAN_POINT('Ctrl Pts',(-185.720997486229,-5.60499975256745,
128.909127561655));
#262073=CARTESIAN_POINT('Ctrl Pts',(-185.728793533698,-5.6579511712372,
129.065727135315));
#262074=CARTESIAN_POINT('Ctrl Pts',(-185.736589581167,-5.70439137034077,
129.22471217246));
#262075=CARTESIAN_POINT('Ctrl Pts',(-185.744385628636,-5.7441138651048,
129.38552783418));
#262076=CARTESIAN_POINT('Ctrl Pts',(-185.752171064916,-5.78378229363978,
129.54612460994));
#262077=CARTESIAN_POINT('Ctrl Pts',(-185.759956501197,-5.81675116516731,
129.708546741938));
#262078=CARTESIAN_POINT('Ctrl Pts',(-185.767741937477,-5.842863099156,129.872222555356));
#262079=CARTESIAN_POINT('Ctrl Pts',(-185.775512714118,-5.86892586550339,
130.035590174303));
#262080=CARTESIAN_POINT('Ctrl Pts',(-185.783283490759,-5.88815739778654,
130.200206457726));
#262081=CARTESIAN_POINT('Ctrl Pts',(-185.7910542674,-5.90045097199386,130.365488324528));
#262082=CARTESIAN_POINT('Ctrl Pts',(-185.797911114185,-5.9112986849928,
130.511331203479));
#262083=CARTESIAN_POINT('Ctrl Pts',(-185.804767960969,-5.91674511390588,
130.657691966486));
#262084=CARTESIAN_POINT('Ctrl Pts',(-185.811624807754,-5.91674999671234,
130.804163375351));
#262085=CARTESIAN_POINT('',(-187.561624807792,-5.91674750900767,130.809789904034));
#262086=CARTESIAN_POINT('Ctrl Pts',(-185.811624807791,-5.91674999671237,
130.804163376133));
#262087=CARTESIAN_POINT('Ctrl Pts',(-185.819353984328,-5.91675550068887,
130.969268914026));
#262088=CARTESIAN_POINT('Ctrl Pts',(-185.827083160864,-5.90984584058032,
131.134248349692));
#262089=CARTESIAN_POINT('Ctrl Pts',(-185.834812337401,-5.89607849221174,
131.298515427497));
#262090=CARTESIAN_POINT('Ctrl Pts',(-185.84255057446,-5.88229500507678,
131.462975067292));
#262091=CARTESIAN_POINT('Ctrl Pts',(-185.85028881152,-5.86163781335462,
131.626720362507));
#262092=CARTESIAN_POINT('Ctrl Pts',(-185.858027048579,-5.83421588616898,
131.789173064722));
#262093=CARTESIAN_POINT('Ctrl Pts',(-185.865901549692,-5.80631108117604,
131.954486426734));
#262094=CARTESIAN_POINT('Ctrl Pts',(-185.873776050805,-5.77140116501924,
132.118460904788));
#262095=CARTESIAN_POINT('Ctrl Pts',(-185.881650551917,-5.72965398230494,
132.28050282127));
#262096=CARTESIAN_POINT('Ctrl Pts',(-185.889414944337,-5.68849054802612,
132.44027891503));
#262097=CARTESIAN_POINT('Ctrl Pts',(-185.897179336757,-5.64067998075974,
132.59817586172));
#262098=CARTESIAN_POINT('Ctrl Pts',(-185.904943729177,-5.58643216126939,
132.753644144925));
#262099=CARTESIAN_POINT('Ctrl Pts',(-185.912873284636,-5.53103038996559,
132.91241952709));
#262100=CARTESIAN_POINT('Ctrl Pts',(-185.920802840095,-5.46891459747241,
133.068661436369));
#262101=CARTESIAN_POINT('Ctrl Pts',(-185.928732395554,-5.40035816938212,
133.221810142352));
#262102=CARTESIAN_POINT('Ctrl Pts',(-185.936661951013,-5.33180174129202,
133.374958848335));
#262103=CARTESIAN_POINT('Ctrl Pts',(-185.944591506471,-5.25680489255712,
133.525014066598));
#262104=CARTESIAN_POINT('Ctrl Pts',(-185.95252106193,-5.17568835721522,
133.671446349016));
#262105=CARTESIAN_POINT('Ctrl Pts',(-185.959944328336,-5.09975097902817,
133.808529171427));
#262106=CARTESIAN_POINT('Ctrl Pts',(-185.967367594741,-5.01824886787116,
133.942800289093));
#262107=CARTESIAN_POINT('Ctrl Pts',(-185.974790861147,-4.93141506493196,
134.073775858838));
#262108=CARTESIAN_POINT('Ctrl Pts',(-185.982205353868,-4.84468389233649,
134.204596626337));
#262109=CARTESIAN_POINT('Ctrl Pts',(-185.989619846589,-4.75263377562075,
134.332129290969));
#262110=CARTESIAN_POINT('Ctrl Pts',(-185.99703433931,-4.65554394683494,
134.455913865376));
#262111=CARTESIAN_POINT('Ctrl Pts',(-186.004441685664,-4.55854769688175,
134.579579131549));
#262112=CARTESIAN_POINT('Ctrl Pts',(-186.011849032018,-4.45652163394964,
134.699503207619));
#262113=CARTESIAN_POINT('Ctrl Pts',(-186.019256378371,-4.34978858474558,
134.815254511764));
#262114=CARTESIAN_POINT('Ctrl Pts',(-186.026658200047,-4.24313514107611,
134.930919484221));
#262115=CARTESIAN_POINT('Ctrl Pts',(-186.034060021722,-4.13178195327352,
135.042417608329));
#262116=CARTESIAN_POINT('Ctrl Pts',(-186.041461843398,-4.0160923929967,
135.149349967773));
#262117=CARTESIAN_POINT('Ctrl Pts',(-186.048859757709,-3.90046390433854,
135.256225878457));
#262118=CARTESIAN_POINT('Ctrl Pts',(-186.056257672021,-3.78050387557164,
135.358540571827));
#262119=CARTESIAN_POINT('Ctrl Pts',(-186.063655586332,-3.65661275257442,
135.455931722065));
#262120=CARTESIAN_POINT('Ctrl Pts',(-186.071052271244,-3.53274221803405,
135.553306687661));
#262121=CARTESIAN_POINT('Ctrl Pts',(-186.078448956157,-3.4049421790122,
135.645759503541));
#262122=CARTESIAN_POINT('Ctrl Pts',(-186.085845641069,-3.27364649016796,
135.732967846785));
#262123=CARTESIAN_POINT('Ctrl Pts',(-186.093241998004,-3.14235662311216,
135.820172323119));
#262124=CARTESIAN_POINT('Ctrl Pts',(-186.10063835494,-3.00757172538186,
135.902132582656));
#262125=CARTESIAN_POINT('Ctrl Pts',(-186.108034711876,-2.86975475604621,
135.978569562192));
#262126=CARTESIAN_POINT('Ctrl Pts',(-186.115432201212,-2.73191668658033,
136.055018244425));
#262127=CARTESIAN_POINT('Ctrl Pts',(-186.122829690549,-2.59104594766015,
136.125941781829));
#262128=CARTESIAN_POINT('Ctrl Pts',(-186.130227179886,-2.44763008059823,
136.191107089329));
#262129=CARTESIAN_POINT('Ctrl Pts',(-186.137627262401,-2.30416393932624,
136.256295240426));
#262130=CARTESIAN_POINT('Ctrl Pts',(-186.145027344916,-2.15815123321437,
136.315720988395));
#262131=CARTESIAN_POINT('Ctrl Pts',(-186.152427427431,-2.01009930602779,
136.369199460013));
#262132=CARTESIAN_POINT('Ctrl Pts',(-186.159835647097,-1.8618845805278,
136.422736736708));
#262133=CARTESIAN_POINT('Ctrl Pts',(-186.167243866764,-1.71162650717714,
136.47031355006));
#262134=CARTESIAN_POINT('Ctrl Pts',(-186.174652086431,-1.5598481143866,
136.511794754071));
#262135=CARTESIAN_POINT('Ctrl Pts',(-186.182064865733,-1.40797630452743,
136.553301489072));
#262136=CARTESIAN_POINT('Ctrl Pts',(-186.189477645035,-1.25458267355879,
136.588705055152));
#262137=CARTESIAN_POINT('Ctrl Pts',(-186.196890424337,-1.10019974227204,
136.617921582208));
#262138=CARTESIAN_POINT('Ctrl Pts',(-186.204313795366,-0.94559622141344,
136.647179855207));
#262139=CARTESIAN_POINT('Ctrl Pts',(-186.211737166394,-0.790000945331487,
136.67023337849));
#262140=CARTESIAN_POINT('Ctrl Pts',(-186.219160537423,-0.633951672601608,
136.687050124867));
#262141=CARTESIAN_POINT('Ctrl Pts',(-186.223096586864,-0.551210603860005,
136.695966767307));
#262142=CARTESIAN_POINT('Ctrl Pts',(-186.227032636304,-0.468341915081361,
136.703130899092));
#262143=CARTESIAN_POINT('Ctrl Pts',(-186.230968685744,-0.385425554330736,
136.708543685914));
#262144=CARTESIAN_POINT('Ctrl Pts',(-186.23839195215,-0.229047885666553,
136.718752032934));
#262145=CARTESIAN_POINT('Ctrl Pts',(-186.245815218555,-0.0720279097393259,
136.72275881741));
#262146=CARTESIAN_POINT('Ctrl Pts',(-186.253238484961,0.0851013380298015,
136.72049857444));
#262147=CARTESIAN_POINT('Ctrl Pts',(-186.260652977682,0.242044872077285,
136.718241002889));
#262148=CARTESIAN_POINT('Ctrl Pts',(-186.268067470403,0.399097051278048,
136.709731153093));
#262149=CARTESIAN_POINT('Ctrl Pts',(-186.275481963124,0.555719943496593,
136.694955316482));
#262150=CARTESIAN_POINT('Ctrl Pts',(-186.282889309477,0.712191876675316,
136.680193721379));
#262151=CARTESIAN_POINT('Ctrl Pts',(-186.290296655831,0.868234977439624,
136.65917819753));
#262152=CARTESIAN_POINT('Ctrl Pts',(-186.297704002185,1.02331164805928,
136.631947067671));
#262153=CARTESIAN_POINT('Ctrl Pts',(-186.30510582386,1.1782726566464,136.604736247816));
#262154=CARTESIAN_POINT('Ctrl Pts',(-186.312507645536,1.33226830420908,
136.571319116806));
#262155=CARTESIAN_POINT('Ctrl Pts',(-186.319909467211,1.48476655989437,
136.531785765494));
#262156=CARTESIAN_POINT('Ctrl Pts',(-186.327307381523,1.63718431293841,
136.492273283531));
#262157=CARTESIAN_POINT('Ctrl Pts',(-186.334705295834,1.78810588790865,
136.446651104826));
#262158=CARTESIAN_POINT('Ctrl Pts',(-186.342103210145,1.93700999905407,
136.395060289885));
#262159=CARTESIAN_POINT('Ctrl Pts',(-186.349499895057,2.08588936503698,
136.343478048401));
#262160=CARTESIAN_POINT('Ctrl Pts',(-186.35689657997,2.23275158021718,136.285929261356));
#262161=CARTESIAN_POINT('Ctrl Pts',(-186.364293264882,2.37709095615206,
136.22260471955));
#262162=CARTESIAN_POINT('Ctrl Pts',(-186.371689621817,2.52142393192816,
136.15928298562));
#262163=CARTESIAN_POINT('Ctrl Pts',(-186.379085978753,2.66323394903901,
136.090186156123));
#262164=CARTESIAN_POINT('Ctrl Pts',(-186.386482335688,2.80203598302284,
136.015552891158));
#262165=CARTESIAN_POINT('Ctrl Pts',(-186.393879825025,2.94085926795201,
135.94090819965));
#262166=CARTESIAN_POINT('Ctrl Pts',(-186.401277314361,3.07667332397372,
135.860725561701));
#262167=CARTESIAN_POINT('Ctrl Pts',(-186.408674803698,3.20901852202426,
135.775289171449));
#262168=CARTESIAN_POINT('Ctrl Pts',(-186.416074886213,3.34141011347863,
135.689822831602));
#262169=CARTESIAN_POINT('Ctrl Pts',(-186.423474968728,3.47033011248045,
135.599099274988));
#262170=CARTESIAN_POINT('Ctrl Pts',(-186.430875051243,3.59534874825436,
135.503445415793));
#262171=CARTESIAN_POINT('Ctrl Pts',(-186.438283270909,3.72050485487072,
135.407686375345));
#262172=CARTESIAN_POINT('Ctrl Pts',(-186.445691490576,3.84175073429224,
135.306986432451));
#262173=CARTESIAN_POINT('Ctrl Pts',(-186.453099710242,3.95868997473241,
135.201712576012));
#262174=CARTESIAN_POINT('Ctrl Pts',(-186.460512489544,4.07570118932416,
135.096373925272));
#262175=CARTESIAN_POINT('Ctrl Pts',(-186.467925268846,4.18840021653473,
134.986456011451));
#262176=CARTESIAN_POINT('Ctrl Pts',(-186.475338048148,4.29642865357484,
134.872361525536));
#262177=CARTESIAN_POINT('Ctrl Pts',(-186.482761419177,4.40461144671197,
134.758104016068));
#262178=CARTESIAN_POINT('Ctrl Pts',(-186.490184790206,4.50811007610825,
134.639658296061));
#262179=CARTESIAN_POINT('Ctrl Pts',(-186.497608161235,4.60660692473589,
134.517459485557));
#262180=CARTESIAN_POINT('Ctrl Pts',(-186.501544210675,4.65883231727349,
134.452666744113));
#262181=CARTESIAN_POINT('Ctrl Pts',(-186.505480260116,4.7096522547113,134.386819357501));
#262182=CARTESIAN_POINT('Ctrl Pts',(-186.509416309556,4.75902450389532,
134.319985218377));
#262183=CARTESIAN_POINT('Ctrl Pts',(-186.516839575961,4.85213902500785,
134.193938117801));
#262184=CARTESIAN_POINT('Ctrl Pts',(-186.524262842367,4.94038317868034,
134.063998529898));
#262185=CARTESIAN_POINT('Ctrl Pts',(-186.531686108772,5.02341376877007,
133.930579527085));
#262186=CARTESIAN_POINT('Ctrl Pts',(-186.539100601493,5.10634622359734,
133.797318214453));
#262187=CARTESIAN_POINT('Ctrl Pts',(-186.546515094214,5.18407718502282,
133.660585986465));
#262188=CARTESIAN_POINT('Ctrl Pts',(-186.553929586935,5.25630435417878,
133.520828010844));
#262189=CARTESIAN_POINT('Ctrl Pts',(-186.561336933289,5.3284619080698,133.381204739222));
#262190=CARTESIAN_POINT('Ctrl Pts',(-186.568744279642,5.39512606019245,
133.238561855208));
#262191=CARTESIAN_POINT('Ctrl Pts',(-186.576151625996,5.45603846784417,
133.093372369372));
#262192=CARTESIAN_POINT('Ctrl Pts',(-186.583553447672,5.51690544472435,
132.948291171332));
#262193=CARTESIAN_POINT('Ctrl Pts',(-186.590955269347,5.57202907504359,
132.800667496085));
#262194=CARTESIAN_POINT('Ctrl Pts',(-186.598357091022,5.6211975791176,132.650997652563));
#262195=CARTESIAN_POINT('Ctrl Pts',(-186.605755005334,5.67034012752104,
132.501406818586));
#262196=CARTESIAN_POINT('Ctrl Pts',(-186.613152919645,5.71353369422572,
132.349772321271));
#262197=CARTESIAN_POINT('Ctrl Pts',(-186.620550833956,5.75061518974696,
132.196608979731));
#262198=CARTESIAN_POINT('Ctrl Pts',(-186.627947518869,5.78769052299643,
132.043471091159));
#262199=CARTESIAN_POINT('Ctrl Pts',(-186.635344203781,5.81865571320347,
131.88880522507));
#262200=CARTESIAN_POINT('Ctrl Pts',(-186.642740888693,5.84339794111647,
131.733139958559));
#262201=CARTESIAN_POINT('Ctrl Pts',(-186.650137245628,5.86813907193316,
131.577481594409));
#262202=CARTESIAN_POINT('Ctrl Pts',(-186.657533602564,5.88665773050493,
131.42082428662));
#262203=CARTESIAN_POINT('Ctrl Pts',(-186.664929959499,5.89889254076296,
131.26370510162));
#262204=CARTESIAN_POINT('Ctrl Pts',(-186.672327448836,5.91112922420171,
131.106561861272));
#262205=CARTESIAN_POINT('Ctrl Pts',(-186.679724938173,5.91708011472825,
130.948956975106));
#262206=CARTESIAN_POINT('Ctrl Pts',(-186.687122427509,5.91673587218311,
130.791430755944));
#262207=CARTESIAN_POINT('Ctrl Pts',(-186.694522510024,5.91639150896428,
130.633849316211));
#262208=CARTESIAN_POINT('Ctrl Pts',(-186.701922592539,5.90974761986768,
130.47634697145));
#262209=CARTESIAN_POINT('Ctrl Pts',(-186.709322675054,5.89684694545481,
130.319462005091));
#262210=CARTESIAN_POINT('Ctrl Pts',(-186.716730894721,5.88393208542427,
130.162404527584));
#262211=CARTESIAN_POINT('Ctrl Pts',(-186.724139114387,5.86474673092027,
130.005966156498));
#262212=CARTESIAN_POINT('Ctrl Pts',(-186.731547334054,5.83938536984659,
129.850678770763));
#262213=CARTESIAN_POINT('Ctrl Pts',(-186.738960113356,5.81400839927836,
129.695295808233));
#262214=CARTESIAN_POINT('Ctrl Pts',(-186.746372892658,5.78244792237959,
129.541065607525));
#262215=CARTESIAN_POINT('Ctrl Pts',(-186.75378567196,5.7448490090175,129.38850736737));
#262216=CARTESIAN_POINT('Ctrl Pts',(-186.761209042988,5.70719637256474,
129.235731144846));
#262217=CARTESIAN_POINT('Ctrl Pts',(-186.768632414017,5.66348817105071,
129.084632011842));
#262218=CARTESIAN_POINT('Ctrl Pts',(-186.776055785046,5.61391880352735,
128.935712381567));
#262219=CARTESIAN_POINT('Ctrl Pts',(-186.779991834487,5.58763593546334,
128.856751620311));
#262220=CARTESIAN_POINT('Ctrl Pts',(-186.783927883928,5.55970608173856,
128.77840324676));
#262221=CARTESIAN_POINT('Ctrl Pts',(-186.787863933369,5.53016353431541,
128.700739490502));
#262222=CARTESIAN_POINT('Ctrl Pts',(-186.795287199775,5.47444721187183,
128.554268070017));
#262223=CARTESIAN_POINT('Ctrl Pts',(-186.80271046618,5.41282347703181,128.409790243116));
#262224=CARTESIAN_POINT('Ctrl Pts',(-186.810133732586,5.34545435342012,
128.267818026163));
#262225=CARTESIAN_POINT('Ctrl Pts',(-186.817548225307,5.27816485451769,
128.12601360858));
#262226=CARTESIAN_POINT('Ctrl Pts',(-186.824962718028,5.20514364198745,
127.986709240179));
#262227=CARTESIAN_POINT('Ctrl Pts',(-186.832377210749,5.12660184812075,
127.850399877586));
#262228=CARTESIAN_POINT('Ctrl Pts',(-186.839784557103,5.04813575579202,
127.714221895088));
#262229=CARTESIAN_POINT('Ctrl Pts',(-186.847191903456,4.96415986019837,
127.581033492824));
#262230=CARTESIAN_POINT('Ctrl Pts',(-186.85459924981,4.87493247798782,127.451307695592));
#262231=CARTESIAN_POINT('Ctrl Pts',(-186.862001071486,4.78577164492528,
127.321678652754));
#262232=CARTESIAN_POINT('Ctrl Pts',(-186.869402893161,4.69136733467664,
127.195507379004));
#262233=CARTESIAN_POINT('Ctrl Pts',(-186.876804714836,4.59202263391012,
127.073240317689));
#262234=CARTESIAN_POINT('Ctrl Pts',(-186.884202629148,4.4927303764384,126.951037800204));
#262235=CARTESIAN_POINT('Ctrl Pts',(-186.891600543459,4.38850315720013,
126.832735679553));
#262236=CARTESIAN_POINT('Ctrl Pts',(-186.89899845777,4.27968595424607,126.718749439844));
#262237=CARTESIAN_POINT('Ctrl Pts',(-186.906395142683,4.17088683473652,
126.604782142579));
#262238=CARTESIAN_POINT('Ctrl Pts',(-186.913791827595,4.05749950290368,
126.495129572533));
#262239=CARTESIAN_POINT('Ctrl Pts',(-186.921188512507,3.93990768406763,
126.390172356569));
#262240=CARTESIAN_POINT('Ctrl Pts',(-186.928584869443,3.82232107937571,
126.285219794517));
#262241=CARTESIAN_POINT('Ctrl Pts',(-186.935981226378,3.70053063686753,
126.184962421158));
#262242=CARTESIAN_POINT('Ctrl Pts',(-186.943377583313,3.57495503047606,
126.089742171438));
#262243=CARTESIAN_POINT('Ctrl Pts',(-186.95077507265,3.4493601981394,125.994507343255));
#262244=CARTESIAN_POINT('Ctrl Pts',(-186.958172561986,3.31997934549403,
125.904311399832));
#262245=CARTESIAN_POINT('Ctrl Pts',(-186.965570051323,3.18726200443501,
125.819454251586));
#262246=CARTESIAN_POINT('Ctrl Pts',(-186.972970133838,3.05449813951574,
125.734567356798));
#262247=CARTESIAN_POINT('Ctrl Pts',(-186.980370216353,2.91839577182612,
125.655023184307));
#262248=CARTESIAN_POINT('Ctrl Pts',(-186.987770298868,2.77943087677651,
125.581076730611));
#262249=CARTESIAN_POINT('Ctrl Pts',(-186.995178518535,2.64031317554104,
125.507048965188));
#262250=CARTESIAN_POINT('Ctrl Pts',(-187.002586738201,2.49832699064388,
125.438631386499));
#262251=CARTESIAN_POINT('Ctrl Pts',(-187.009994957867,2.35397087991152,
125.376031992747));
#262252=CARTESIAN_POINT('Ctrl Pts',(-187.017407737169,2.20952592040129,
125.313394070112));
#262253=CARTESIAN_POINT('Ctrl Pts',(-187.024820516472,2.06270847584779,
125.256581602402));
#262254=CARTESIAN_POINT('Ctrl Pts',(-187.032233295774,1.91403377665382,
125.205753177825));
#262255=CARTESIAN_POINT('Ctrl Pts',(-187.039656666802,1.76514664407727,
125.15485212721));
#262256=CARTESIAN_POINT('Ctrl Pts',(-187.047080037831,1.61439731357947,
125.109952302834));
#262257=CARTESIAN_POINT('Ctrl Pts',(-187.05450340886,1.46231355706026,125.071161717882));
#262258=CARTESIAN_POINT('Ctrl Pts',(-187.058439458301,1.38167510015412,
125.050594018973));
#262259=CARTESIAN_POINT('Ctrl Pts',(-187.062375507741,1.30066162638929,
125.031742986259));
#262260=CARTESIAN_POINT('Ctrl Pts',(-187.066311557182,1.21935244020638,
125.014618810796));
#262261=CARTESIAN_POINT('Ctrl Pts',(-187.073734823588,1.06600585263888,
124.9823231503));
#262262=CARTESIAN_POINT('Ctrl Pts',(-187.081158089993,0.911143431117751,
124.956075149189));
#262263=CARTESIAN_POINT('Ctrl Pts',(-187.088581356398,0.755283527239422,
124.936015249749));
#262264=CARTESIAN_POINT('Ctrl Pts',(-187.095995849119,0.599607836824118,
124.915979059444));
#262265=CARTESIAN_POINT('Ctrl Pts',(-187.10341034184,0.442937377369268,
124.902116459795));
#262266=CARTESIAN_POINT('Ctrl Pts',(-187.110824834561,0.285802692063943,
124.894517355371));
#262267=CARTESIAN_POINT('Ctrl Pts',(-187.118232180915,0.128819459083885,
124.88692557525));
#262268=CARTESIAN_POINT('Ctrl Pts',(-187.125639527269,-0.0286267386259374,
124.885585289803));
#262269=CARTESIAN_POINT('Ctrl Pts',(-187.133046873623,-0.185998305446971,
124.890534851374));
#262270=CARTESIAN_POINT('Ctrl Pts',(-187.140448695298,-0.343252498615732,
124.895480721376));
#262271=CARTESIAN_POINT('Ctrl Pts',(-187.147850516973,-0.500431800219757,
124.906707085891));
#262272=CARTESIAN_POINT('Ctrl Pts',(-187.155252338649,-0.656996779079823,
124.924200263054));
#262273=CARTESIAN_POINT('Ctrl Pts',(-187.16265025296,-0.813479108507141,
124.941684205705));
#262274=CARTESIAN_POINT('Ctrl Pts',(-187.170048167272,-0.969347390991606,
124.965428331216));
#262275=CARTESIAN_POINT('Ctrl Pts',(-187.177446081583,-1.12406559892257,
124.995366979093));
#262276=CARTESIAN_POINT('Ctrl Pts',(-187.184842766495,-1.27875809549403,
125.02530065171));
#262277=CARTESIAN_POINT('Ctrl Pts',(-187.192239451407,-1.43230053069113,
125.061426732754));
#262278=CARTESIAN_POINT('Ctrl Pts',(-187.199636136319,-1.58416525944525,
125.103628121363));
#262279=CARTESIAN_POINT('Ctrl Pts',(-187.207032493255,-1.73602325435815,
125.145827638718));
#262280=CARTESIAN_POINT('Ctrl Pts',(-187.21442885019,-1.88620333107437,
125.194101828061));
#262281=CARTESIAN_POINT('Ctrl Pts',(-187.221825207126,-2.03419150655014,
125.248283271346));
#262282=CARTESIAN_POINT('Ctrl Pts',(-187.229222696462,-2.18220233939295,
125.302473009948));
#262283=CARTESIAN_POINT('Ctrl Pts',(-187.236620185799,-2.32802025223464,
125.362571674956));
#262284=CARTESIAN_POINT('Ctrl Pts',(-187.244017675135,-2.4711499389764,
125.428363171362));
#262285=CARTESIAN_POINT('Ctrl Pts',(-187.25141775765,-2.61432979960858,
125.494177730874));
#262286=CARTESIAN_POINT('Ctrl Pts',(-187.258817840165,-2.75481921895261,
125.565688939224));
#262287=CARTESIAN_POINT('Ctrl Pts',(-187.26621792268,-2.89214638489867,
125.642634176653));
#262288=CARTESIAN_POINT('Ctrl Pts',(-187.273626142347,-3.02962455618108,
125.719664023281));
#262289=CARTESIAN_POINT('Ctrl Pts',(-187.281034362013,-3.16393320396151,
125.802139649419));
#262290=CARTESIAN_POINT('Ctrl Pts',(-187.28844258168,-3.29462785077745,
125.889754032357));
#262291=CARTESIAN_POINT('Ctrl Pts',(-187.295855360982,-3.42540293796775,
125.977422340486));
#262292=CARTESIAN_POINT('Ctrl Pts',(-187.303268140284,-3.55255929106162,
126.070235488155));
#262293=CARTESIAN_POINT('Ctrl Pts',(-187.310680919586,-3.67568499069044,
126.167845718236));
#262294=CARTESIAN_POINT('Ctrl Pts',(-187.318104290615,-3.79898661809308,
126.26559541839));
#262295=CARTESIAN_POINT('Ctrl Pts',(-187.325527661644,-3.91824580736076,
126.368155647766));
#262296=CARTESIAN_POINT('Ctrl Pts',(-187.332951032672,-4.03308641033856,
126.475140760682));
#262297=CARTESIAN_POINT('Ctrl Pts',(-187.336887082113,-4.09397765360244,
126.531866834624));
#262298=CARTESIAN_POINT('Ctrl Pts',(-187.340823131554,-4.1536273227506,
126.589836320882));
#262299=CARTESIAN_POINT('Ctrl Pts',(-187.344759180995,-4.21198397777087,
126.648988006897));
#262300=CARTESIAN_POINT('Ctrl Pts',(-187.352082400964,-4.32055949944319,
126.759042724129));
#262301=CARTESIAN_POINT('Ctrl Pts',(-187.359405620933,-4.42500455681407,
126.873544452405));
#262302=CARTESIAN_POINT('Ctrl Pts',(-187.366728840903,-4.52492539990628,
126.992145947878));
#262303=CARTESIAN_POINT('Ctrl Pts',(-187.374043222144,-4.62472564397862,
127.1106042978));
#262304=CARTESIAN_POINT('Ctrl Pts',(-187.381357603385,-4.72001229335793,
127.233152278661));
#262305=CARTESIAN_POINT('Ctrl Pts',(-187.388671984626,-4.81042708213411,
127.3594046164));
#262306=CARTESIAN_POINT('Ctrl Pts',(-187.395978017208,-4.90073867116098,
127.485512849288));
#262307=CARTESIAN_POINT('Ctrl Pts',(-187.403284049789,-4.98618925122516,
127.615316708677));
#262308=CARTESIAN_POINT('Ctrl Pts',(-187.410590082371,-5.06645997052641,
127.748396951297));
#262309=CARTESIAN_POINT('Ctrl Pts',(-187.417891395085,-5.14667883307661,
127.881391220987));
#262310=CARTESIAN_POINT('Ctrl Pts',(-187.4251927078,-5.22172429356674,128.017657336095));
#262311=CARTESIAN_POINT('Ctrl Pts',(-187.432494020514,-5.29131999812529,
128.156745985498));
#262312=CARTESIAN_POINT('Ctrl Pts',(-187.439792150053,-5.36088536083589,
128.295773996006));
#262313=CARTESIAN_POINT('Ctrl Pts',(-187.447090279593,-5.42500552334415,
128.437621749531));
#262314=CARTESIAN_POINT('Ctrl Pts',(-187.454388409132,-5.48344955540227,
128.581814434501));
#262315=CARTESIAN_POINT('Ctrl Pts',(-187.461684889562,-5.54188038124945,
128.725974537204));
#262316=CARTESIAN_POINT('Ctrl Pts',(-187.468981369991,-5.59463748570317,
128.87247816067));
#262317=CARTESIAN_POINT('Ctrl Pts',(-187.47627785042,-5.64153778312993,
129.020829848553));
#262318=CARTESIAN_POINT('Ctrl Pts',(-187.483576690867,-5.68845325027215,
129.169229520201));
#262319=CARTESIAN_POINT('Ctrl Pts',(-187.490875531314,-5.7295080036463,
129.319478085701));
#262320=CARTESIAN_POINT('Ctrl Pts',(-187.498174371761,-5.76456856275173,
129.471064008467));
#262321=CARTESIAN_POINT('Ctrl Pts',(-187.505474224208,-5.79963398307961,
129.62267094895));
#262322=CARTESIAN_POINT('Ctrl Pts',(-187.512774076655,-5.82870347565599,
129.775615239507));
#262323=CARTESIAN_POINT('Ctrl Pts',(-187.520073929102,-5.85169470676966,
129.929375119821));
#262324=CARTESIAN_POINT('Ctrl Pts',(-187.527380321913,-5.87470653706738,
130.083272762574));
#262325=CARTESIAN_POINT('Ctrl Pts',(-187.534686714723,-5.89162917731749,
130.237987073307));
#262326=CARTESIAN_POINT('Ctrl Pts',(-187.541993107533,-5.9024321476053,
130.392990582907));
#262327=CARTESIAN_POINT('Ctrl Pts',(-187.54853700762,-5.91210772350591,
130.531817977784));
#262328=CARTESIAN_POINT('Ctrl Pts',(-187.555080907706,-5.91687497723714,
130.670877114353));
#262329=CARTESIAN_POINT('Ctrl Pts',(-187.561624807792,-5.91674750900767,
130.809789904034));
#262330=CARTESIAN_POINT('',(-189.311624807792,-5.92158926949562,130.802089018337));
#262331=CARTESIAN_POINT('Ctrl Pts',(-187.561624807792,-5.91744066498834,
130.809790540083));
#262332=CARTESIAN_POINT('Ctrl Pts',(-187.582152140131,-5.92149194206913,
131.245596366776));
#262333=CARTESIAN_POINT('Ctrl Pts',(-187.695495347076,-5.67831340457064,
133.64744955503));
#262334=CARTESIAN_POINT('Ctrl Pts',(-187.90165442862,-2.39945118657061,
137.378567378342));
#262335=CARTESIAN_POINT('Ctrl Pts',(-188.180102052435,4.23410436286723,
136.376606194958));
#262336=CARTESIAN_POINT('Ctrl Pts',(-188.458549676247,6.97672485032798,
130.254023545258));
#262337=CARTESIAN_POINT('Ctrl Pts',(-188.73699730006,3.3080760322958,124.637173779559));
#262338=CARTESIAN_POINT('Ctrl Pts',(-189.015444923873,-3.40053305091948,
124.687667434156));
#262339=CARTESIAN_POINT('Ctrl Pts',(-189.20698742645,-5.86572937063765,
128.589015218929));
#262340=CARTESIAN_POINT('Ctrl Pts',(-189.305714054423,-5.92609167912231,
130.677041554188));
#262341=CARTESIAN_POINT('Ctrl Pts',(-189.311624807792,-5.92547957657923,
130.802087525964));
#262342=CARTESIAN_POINT('',(-191.061624793292,-5.91313729896144,130.80003214728));
#262343=CARTESIAN_POINT('Ctrl Pts',(-189.311624807792,-5.91674956464851,
130.802090874911));
#262344=CARTESIAN_POINT('Ctrl Pts',(-189.318977448973,-5.91680914766334,
130.957411468767));
#262345=CARTESIAN_POINT('Ctrl Pts',(-189.326330090154,-5.91074854494049,
131.112981837623));
#262346=CARTESIAN_POINT('Ctrl Pts',(-189.333682731335,-5.89853497471983,
131.268274094959));
#262347=CARTESIAN_POINT('Ctrl Pts',(-189.341027006048,-5.88633530215123,
131.42338964739));
#262348=CARTESIAN_POINT('Ctrl Pts',(-189.348371280761,-5.86799662359575,
131.578227341974));
#262349=CARTESIAN_POINT('Ctrl Pts',(-189.355715555474,-5.8435381292413,
131.732257537813));
#262350=CARTESIAN_POINT('Ctrl Pts',(-189.363053149278,-5.81910188418644,
131.886147616115));
#262351=CARTESIAN_POINT('Ctrl Pts',(-189.370390743082,-5.78855696232474,
132.039231283816));
#262352=CARTESIAN_POINT('Ctrl Pts',(-189.377728336886,-5.75197447447406,
132.190982486533));
#262353=CARTESIAN_POINT('Ctrl Pts',(-189.385060929245,-5.71541692194747,
132.342630252726));
#262354=CARTESIAN_POINT('Ctrl Pts',(-189.392393521605,-5.67283008434618,
132.492946992982));
#262355=CARTESIAN_POINT('Ctrl Pts',(-189.399726113965,-5.62433638296606,
132.641415546996));
#262356=CARTESIAN_POINT('Ctrl Pts',(-189.407056104548,-5.57585988828992,
132.789831420881));
#262357=CARTESIAN_POINT('Ctrl Pts',(-189.414386095132,-5.52148081560047,
132.936400051107));
#262358=CARTESIAN_POINT('Ctrl Pts',(-189.421716085716,-5.46137178798303,
133.080618238294));
#262359=CARTESIAN_POINT('Ctrl Pts',(-189.429044866575,-5.40127268062225,
133.224812624041));
#262360=CARTESIAN_POINT('Ctrl Pts',(-189.436373647433,-5.33544564582625,
133.366656986859));
#262361=CARTESIAN_POINT('Ctrl Pts',(-189.443702428292,-5.26411181390032,
133.505667222388));
#262362=CARTESIAN_POINT('Ctrl Pts',(-189.45103151263,-5.19277502809146,
133.644683214231));
#262363=CARTESIAN_POINT('Ctrl Pts',(-189.458360596969,-5.11593116510898,
133.780864506177));
#262364=CARTESIAN_POINT('Ctrl Pts',(-189.465689681307,-5.03384764105057,
133.913750990162));
#262365=CARTESIAN_POINT('Ctrl Pts',(-189.473020582319,-4.95174377079516,
134.046670412968));
#262366=CARTESIAN_POINT('Ctrl Pts',(-189.480351483332,-4.86439785503814,
134.176293078574));
#262367=CARTESIAN_POINT('Ctrl Pts',(-189.487682384344,-4.77212086708803,
134.302187513283));
#262368=CARTESIAN_POINT('Ctrl Pts',(-189.495020896959,-4.6797480688371,
134.428212662962));
#262369=CARTESIAN_POINT('Ctrl Pts',(-189.502359409575,-4.5824341979447,
134.550501542638));
#262370=CARTESIAN_POINT('Ctrl Pts',(-189.509697922191,-4.48053120714239,
134.668654946978));
#262371=CARTESIAN_POINT('Ctrl Pts',(-189.517040396452,-4.37857320471192,
134.78687213562));
#262372=CARTESIAN_POINT('Ctrl Pts',(-189.524382870713,-4.27202140698691,
134.900949123779));
#262373=CARTESIAN_POINT('Ctrl Pts',(-189.531725344974,-4.16126441642406,
135.010523835881));
#262374=CARTESIAN_POINT('Ctrl Pts',(-189.539078893906,-4.05034037083163,
135.120263819778));
#262375=CARTESIAN_POINT('Ctrl Pts',(-189.546432442839,-3.93519874240669,
135.225487704928));
#262376=CARTESIAN_POINT('Ctrl Pts',(-189.553785991771,-3.81626167847011,
135.325873347167));
#262377=CARTESIAN_POINT('Ctrl Pts',(-189.559970718347,-3.71622926868426,
135.410303022565));
#262378=CARTESIAN_POINT('Ctrl Pts',(-189.566155444922,-3.61351273278213,
135.491310933321));
#262379=CARTESIAN_POINT('Ctrl Pts',(-189.572340171498,-3.50837810462016,
135.568729792758));
#262380=CARTESIAN_POINT('Ctrl Pts',(-189.579763437904,-3.38218944555196,
135.661652383818));
#262381=CARTESIAN_POINT('Ctrl Pts',(-189.587186704309,-3.25211571553351,
135.749698689375));
#262382=CARTESIAN_POINT('Ctrl Pts',(-189.594609970715,-3.11857050878932,
135.832526142309));
#262383=CARTESIAN_POINT('Ctrl Pts',(-189.602024463436,-2.98518314138887,
135.915255700071));
#262384=CARTESIAN_POINT('Ctrl Pts',(-189.609438956157,-2.84833277843893,
135.992778488313));
#262385=CARTESIAN_POINT('Ctrl Pts',(-189.616853448878,-2.70846504719477,
136.064792885985));
#262386=CARTESIAN_POINT('Ctrl Pts',(-189.624260795232,-2.5687321257355,
136.13673787347));
#262387=CARTESIAN_POINT('Ctrl Pts',(-189.631668141586,-2.42598795540314,
136.203184870211));
#262388=CARTESIAN_POINT('Ctrl Pts',(-189.63907548794,-2.28070593937386,
136.263876253646));
#262389=CARTESIAN_POINT('Ctrl Pts',(-189.646477309616,-2.13553228015454,
136.324522371158));
#262390=CARTESIAN_POINT('Ctrl Pts',(-189.653879131291,-1.98782488706824,
136.379421279541));
#262391=CARTESIAN_POINT('Ctrl Pts',(-189.661280952967,-1.83808039076475,
136.428361954656));
#262392=CARTESIAN_POINT('Ctrl Pts',(-189.668678867278,-1.68841494341483,
136.477276794369));
#262393=CARTESIAN_POINT('Ctrl Pts',(-189.67607678159,-1.53671488843013,
136.520239549164));
#262394=CARTESIAN_POINT('Ctrl Pts',(-189.683474695901,-1.38349529252278,
136.557087913212));
#262395=CARTESIAN_POINT('Ctrl Pts',(-189.690871380814,-1.23030115893236,
136.59393015373));
#262396=CARTESIAN_POINT('Ctrl Pts',(-189.698268065726,-1.07558834819108,
136.62465993296));
#262397=CARTESIAN_POINT('Ctrl Pts',(-189.705664750638,-0.919885608475016,
136.649165236184));
#262398=CARTESIAN_POINT('Ctrl Pts',(-189.713061107574,-0.7641897727816,
136.673669452817));
#262399=CARTESIAN_POINT('Ctrl Pts',(-189.72045746451,-0.607504464148897,
136.691949684189));
#262400=CARTESIAN_POINT('Ctrl Pts',(-189.727853821445,-0.450366841788114,
136.703945371624));
#262401=CARTESIAN_POINT('Ctrl Pts',(-189.735251310782,-0.293205161256196,
136.71594289563));
#262402=CARTESIAN_POINT('Ctrl Pts',(-189.742648800119,-0.135591401348304,
136.721653931456));
#262403=CARTESIAN_POINT('Ctrl Pts',(-189.750046289455,0.021934111525369,
136.721069961217));
#262404=CARTESIAN_POINT('Ctrl Pts',(-189.75744637197,0.179514844723607,
136.720485786269));
#262405=CARTESIAN_POINT('Ctrl Pts',(-189.764846454486,0.337006896234077,
136.713602213106));
#262406=CARTESIAN_POINT('Ctrl Pts',(-189.772246537001,0.493872048296028,
136.700462801417));
#262407=CARTESIAN_POINT('Ctrl Pts',(-189.779654756667,0.650909689718572,
136.687308941594));
#262408=CARTESIAN_POINT('Ctrl Pts',(-189.787062976334,0.807318682811136,
136.667885536733));
#262409=CARTESIAN_POINT('Ctrl Pts',(-189.794471196001,0.962567293055188,
136.642287884057));
#262410=CARTESIAN_POINT('Ctrl Pts',(-189.801883975303,1.11791145622882,
136.616674476453));
#262411=CARTESIAN_POINT('Ctrl Pts',(-189.809296754605,1.27209344867101,
136.584879323986));
#262412=CARTESIAN_POINT('Ctrl Pts',(-189.816709533907,1.4245942930246,136.547048286487));
#262413=CARTESIAN_POINT('Ctrl Pts',(-189.824132904936,1.57731303773595,
136.509163194228));
#262414=CARTESIAN_POINT('Ctrl Pts',(-189.831556275965,1.72834547933129,
136.465225096164));
#262415=CARTESIAN_POINT('Ctrl Pts',(-189.838979646994,1.87718950102327,
136.41542915571));
#262416=CARTESIAN_POINT('Ctrl Pts',(-189.842915696433,1.95611017275407,
136.389026153255));
#262417=CARTESIAN_POINT('Ctrl Pts',(-189.846851745872,2.03441595105685,
136.360977098998));
#262418=CARTESIAN_POINT('Ctrl Pts',(-189.850787795312,2.11203465861468,
136.331316394783));
#262419=CARTESIAN_POINT('Ctrl Pts',(-189.858211061717,2.25842111873141,
136.275377232289));
#262420=CARTESIAN_POINT('Ctrl Pts',(-189.865634328123,2.40280499749717,
136.213533698149));
#262421=CARTESIAN_POINT('Ctrl Pts',(-189.873057594528,2.54467452571146,
136.145948595003));
#262422=CARTESIAN_POINT('Ctrl Pts',(-189.880472087249,2.68637637592454,
136.078443371836));
#262423=CARTESIAN_POINT('Ctrl Pts',(-189.88788657997,2.82556945715901,136.005210246327));
#262424=CARTESIAN_POINT('Ctrl Pts',(-189.895301072691,2.96175913466819,
135.926461103764));
#262425=CARTESIAN_POINT('Ctrl Pts',(-189.902708419045,3.09781754743913,
135.847787862589));
#262426=CARTESIAN_POINT('Ctrl Pts',(-189.910115765399,3.23087799845622,
135.763609374162));
#262427=CARTESIAN_POINT('Ctrl Pts',(-189.917523111753,3.36046785658173,
135.674184674694));
#262428=CARTESIAN_POINT('Ctrl Pts',(-189.924924933428,3.48996106170153,
135.584826671541));
#262429=CARTESIAN_POINT('Ctrl Pts',(-189.932326755103,3.61598852205761,
135.49023045941));
#262430=CARTESIAN_POINT('Ctrl Pts',(-189.939728576779,3.73810425606627,
135.390699804028));
#262431=CARTESIAN_POINT('Ctrl Pts',(-189.94712649109,3.86015552612914,135.291221690105));
#262432=CARTESIAN_POINT('Ctrl Pts',(-189.954524405402,3.97829889370356,
135.18681455587));
#262433=CARTESIAN_POINT('Ctrl Pts',(-189.961922319713,4.09211940015992,
135.077824011271));
#262434=CARTESIAN_POINT('Ctrl Pts',(-189.969319004625,4.20592099171351,
134.968851578922));
#262435=CARTESIAN_POINT('Ctrl Pts',(-189.976715689538,4.31540087856674,
134.855297505843));
#262436=CARTESIAN_POINT('Ctrl Pts',(-189.98411237445,4.42017901826155,134.73754609616));
#262437=CARTESIAN_POINT('Ctrl Pts',(-189.991508731385,4.52495251198384,
134.619799907697));
#262438=CARTESIAN_POINT('Ctrl Pts',(-189.998905088321,4.62502442492598,
134.497857031564));
#262439=CARTESIAN_POINT('Ctrl Pts',(-190.006301445256,4.72005345968584,
134.372136661575));
#262440=CARTESIAN_POINT('Ctrl Pts',(-190.013698934593,4.81509704363352,
134.246397043477));
#262441=CARTESIAN_POINT('Ctrl Pts',(-190.02109642393,4.90509598697833,134.11687907778));
#262442=CARTESIAN_POINT('Ctrl Pts',(-190.028493913266,4.98975106375987,
133.984032752269));
#262443=CARTESIAN_POINT('Ctrl Pts',(-190.035893995781,5.07443581624746,
133.851139857685));
#262444=CARTESIAN_POINT('Ctrl Pts',(-190.043294078296,5.15377277199098,
133.71491659491));
#262445=CARTESIAN_POINT('Ctrl Pts',(-190.050694160811,5.22750765914304,
133.575839326866));
#262446=CARTESIAN_POINT('Ctrl Pts',(-190.058102380478,5.30132362538356,
133.436609129067));
#262447=CARTESIAN_POINT('Ctrl Pts',(-190.065510600145,5.36952504604308,
133.294518988678));
#262448=CARTESIAN_POINT('Ctrl Pts',(-190.072918819811,5.43190468187914,
133.150067779485));
#262449=CARTESIAN_POINT('Ctrl Pts',(-190.080331599113,5.49432271134037,
133.005527662983));
#262450=CARTESIAN_POINT('Ctrl Pts',(-190.087744378416,5.55091168210434,
132.858623929535));
#262451=CARTESIAN_POINT('Ctrl Pts',(-190.095157157718,5.60151379023981,
132.709872050293));
#262452=CARTESIAN_POINT('Ctrl Pts',(-190.102580528747,5.65218820104032,
132.56090762739));
#262453=CARTESIAN_POINT('Ctrl Pts',(-190.110003899775,5.69685855860319,
132.410090141567));
#262454=CARTESIAN_POINT('Ctrl Pts',(-190.117427270804,5.73541765304766,
132.25794752849));
#262455=CARTESIAN_POINT('Ctrl Pts',(-190.121363320244,5.7558626101311,132.17727786444));
#262456=CARTESIAN_POINT('Ctrl Pts',(-190.125299369684,5.77459033229658,
132.096235796439));
#262457=CARTESIAN_POINT('Ctrl Pts',(-190.129235419124,5.79159074918677,
132.014900644345));
#262458=CARTESIAN_POINT('Ctrl Pts',(-190.13665868553,5.82365300488208,131.861505085854));
#262459=CARTESIAN_POINT('Ctrl Pts',(-190.144081951935,5.84966530135562,
131.706602898674));
#262460=CARTESIAN_POINT('Ctrl Pts',(-190.15150521834,5.86948798532478,131.550712647528));
#262461=CARTESIAN_POINT('Ctrl Pts',(-190.158919711061,5.88928724052766,
131.395006645713));
#262462=CARTESIAN_POINT('Ctrl Pts',(-190.166334203782,5.90291139835537,
131.238315271165));
#262463=CARTESIAN_POINT('Ctrl Pts',(-190.173748696503,5.9102713617377,131.081169203277));
#262464=CARTESIAN_POINT('Ctrl Pts',(-190.181156042857,5.91762423131021,
130.924174598686));
#262465=CARTESIAN_POINT('Ctrl Pts',(-190.18856338921,5.91872490889553,130.766726543612));
#262466=CARTESIAN_POINT('Ctrl Pts',(-190.195970735564,5.91353586032059,
130.609362691417));
#262467=CARTESIAN_POINT('Ctrl Pts',(-190.203372557239,5.90835068193385,
130.45211620712));
#262468=CARTESIAN_POINT('Ctrl Pts',(-190.210774378915,5.8968851302798,130.294954172144));
#262469=CARTESIAN_POINT('Ctrl Pts',(-190.21817620059,5.8791537081288,130.138415996223));
#262470=CARTESIAN_POINT('Ctrl Pts',(-190.225574114901,5.86143164625758,
129.981960455587));
#262471=CARTESIAN_POINT('Ctrl Pts',(-190.232972029212,5.83745034325019,
129.826128488115));
#262472=CARTESIAN_POINT('Ctrl Pts',(-190.240369943524,5.80727627526828,
129.671456020874));
#262473=CARTESIAN_POINT('Ctrl Pts',(-190.247766628436,5.77710722166901,
129.51680925739));
#262474=CARTESIAN_POINT('Ctrl Pts',(-190.255163313348,5.74074751701105,
129.36332197774));
#262475=CARTESIAN_POINT('Ctrl Pts',(-190.26255999826,5.69831506500718,129.211521648174));
#262476=CARTESIAN_POINT('Ctrl Pts',(-190.269956355195,5.6558844945027,129.059728049594));
#262477=CARTESIAN_POINT('Ctrl Pts',(-190.277352712131,5.60738181255083,
128.909621611885));
#262478=CARTESIAN_POINT('Ctrl Pts',(-190.284749069066,5.55297521919776,
128.761716062712));
#262479=CARTESIAN_POINT('Ctrl Pts',(-190.292146558402,5.49856029605635,
128.613787868822));
#262480=CARTESIAN_POINT('Ctrl Pts',(-190.299544047739,5.43823979060307,
128.468061584774));
#262481=CARTESIAN_POINT('Ctrl Pts',(-190.306941537075,5.37223055136691,
128.325032187232));
#262482=CARTESIAN_POINT('Ctrl Pts',(-190.31434161959,5.30619817269379,128.181952650957));
#262483=CARTESIAN_POINT('Ctrl Pts',(-190.321741702105,5.23447324617382,
128.041572222184));
#262484=CARTESIAN_POINT('Ctrl Pts',(-190.32914178462,5.15731910927882,127.904362312813));
#262485=CARTESIAN_POINT('Ctrl Pts',(-190.336550004286,5.08008013347921,
127.767001527043));
#262486=CARTESIAN_POINT('Ctrl Pts',(-190.343958223952,4.99740020795088,
127.632818548654));
#262487=CARTESIAN_POINT('Ctrl Pts',(-190.351366443619,4.90958703146701,
127.502257387358));
#262488=CARTESIAN_POINT('Ctrl Pts',(-190.358779222921,4.82171980743826,
127.371615867845));
#262489=CARTESIAN_POINT('Ctrl Pts',(-190.366192002223,4.72871325692401,
127.244600907808));
#262490=CARTESIAN_POINT('Ctrl Pts',(-190.373604781525,4.63091576352256,
127.121623896911));
#262491=CARTESIAN_POINT('Ctrl Pts',(-190.381028152553,4.53297853247616,
126.998471170694));
#262492=CARTESIAN_POINT('Ctrl Pts',(-190.388451523582,4.43023692968165,
126.879368198737));
#262493=CARTESIAN_POINT('Ctrl Pts',(-190.395874894611,4.32307717280776,
126.764690541873));
#262494=CARTESIAN_POINT('Ctrl Pts',(-190.399810944053,4.26625849842815,
126.703885696528));
#262495=CARTESIAN_POINT('Ctrl Pts',(-190.403746993495,4.20819830263757,
126.644324316123));
#262496=CARTESIAN_POINT('Ctrl Pts',(-190.407683042937,4.14895787620481,
126.586057747456));
#262497=CARTESIAN_POINT('Ctrl Pts',(-190.415106309343,4.03723228082388,
126.476168817428));
#262498=CARTESIAN_POINT('Ctrl Pts',(-190.422529575748,3.92096896531795,
126.370555519829));
#262499=CARTESIAN_POINT('Ctrl Pts',(-190.429952842154,3.80052872686658,
126.269615645822));
#262500=CARTESIAN_POINT('Ctrl Pts',(-190.437367334875,3.68023083877513,
126.168795074362));
#262501=CARTESIAN_POINT('Ctrl Pts',(-190.444781827596,3.55576613772917,
126.072637169181));
#262502=CARTESIAN_POINT('Ctrl Pts',(-190.452196320317,3.42753294018989,
125.981503735342));
#262503=CARTESIAN_POINT('Ctrl Pts',(-190.459603666671,3.29942333863392,
125.890458139337));
#262504=CARTESIAN_POINT('Ctrl Pts',(-190.467011013024,3.16755277385676,
125.804427588461));
#262505=CARTESIAN_POINT('Ctrl Pts',(-190.474418359378,3.03235330072144,
125.72373427605));
#262506=CARTESIAN_POINT('Ctrl Pts',(-190.481820181054,2.89725466445357,
125.643101147756));
#262507=CARTESIAN_POINT('Ctrl Pts',(-190.489222002729,2.75883238263387,
125.567797522283));
#262508=CARTESIAN_POINT('Ctrl Pts',(-190.496623824405,2.61754811504931,
125.498102762175));
#262509=CARTESIAN_POINT('Ctrl Pts',(-190.504021738716,2.47633843033066,
125.428444793389));
#262510=CARTESIAN_POINT('Ctrl Pts',(-190.511419653028,2.33227010265108,
125.364389957968));
#262511=CARTESIAN_POINT('Ctrl Pts',(-190.518817567339,2.18582995461846,
125.306172009307));
#262512=CARTESIAN_POINT('Ctrl Pts',(-190.526214252251,2.03941414228153,
125.247963735412));
#262513=CARTESIAN_POINT('Ctrl Pts',(-190.533610937163,1.89062763842013,
125.195590560915));
#262514=CARTESIAN_POINT('Ctrl Pts',(-190.541007622076,1.73997794516578,
125.149238398477));
#262515=CARTESIAN_POINT('Ctrl Pts',(-190.548403979011,1.58933493187669,
125.102888291342));
#262516=CARTESIAN_POINT('Ctrl Pts',(-190.555800335947,1.43682925025374,
125.0625587752));
#262517=CARTESIAN_POINT('Ctrl Pts',(-190.563196692882,1.28298403016603,
125.028386020943));
#262518=CARTESIAN_POINT('Ctrl Pts',(-190.570594182219,1.12911525598238,
124.994208034749));
#262519=CARTESIAN_POINT('Ctrl Pts',(-190.577991671555,0.97390689941849,
124.966188768263));
#262520=CARTESIAN_POINT('Ctrl Pts',(-190.585389160892,0.817892610288261,
124.944413327655));
#262521=CARTESIAN_POINT('Ctrl Pts',(-190.592789243407,0.661823630589273,
124.9226302537));
#262522=CARTESIAN_POINT('Ctrl Pts',(-190.600189325922,0.50494852531532,
124.907095415004));
#262523=CARTESIAN_POINT('Ctrl Pts',(-190.607589408437,0.347806246985612,
124.897842067942));
#262524=CARTESIAN_POINT('Ctrl Pts',(-190.614997628104,0.190491174567385,
124.888578545873));
#262525=CARTESIAN_POINT('Ctrl Pts',(-190.62240584777,0.0329087152680474,
124.885610331419));
#262526=CARTESIAN_POINT('Ctrl Pts',(-190.629814067437,-0.124401254264218,
124.888918546982));
#262527=CARTESIAN_POINT('Ctrl Pts',(-190.637226846739,-0.281808045457423,
124.892228798696));
#262528=CARTESIAN_POINT('Ctrl Pts',(-190.644639626041,-0.438941640954478,
124.901823155316));
#262529=CARTESIAN_POINT('Ctrl Pts',(-190.652052405343,-0.59526761713485,
124.917630878017));
#262530=CARTESIAN_POINT('Ctrl Pts',(-190.659475776372,-0.75181695920117,
124.933461187533));
#262531=CARTESIAN_POINT('Ctrl Pts',(-190.666899147401,-0.907556008596329,
124.955522542167));
#262532=CARTESIAN_POINT('Ctrl Pts',(-190.67432251843,-1.06196003527188,
124.983693005858));
#262533=CARTESIAN_POINT('Ctrl Pts',(-190.67825856787,-1.14382875507758,
124.998629661646));
#262534=CARTESIAN_POINT('Ctrl Pts',(-190.68219461731,-1.22532238526077,
125.015282967731));
#262535=CARTESIAN_POINT('Ctrl Pts',(-190.68613066675,-1.3063645971489,125.033629112651));
#262536=CARTESIAN_POINT('Ctrl Pts',(-190.693553933156,-1.45920767955153,
125.068229369412));
#262537=CARTESIAN_POINT('Ctrl Pts',(-190.700977199561,-1.61090629986719,
125.108958422396));
#262538=CARTESIAN_POINT('Ctrl Pts',(-190.708400465967,-1.76093076543627,
125.155727738555));
#262539=CARTESIAN_POINT('Ctrl Pts',(-190.715814958688,-1.91077791454581,
125.202441777267));
#262540=CARTESIAN_POINT('Ctrl Pts',(-190.723229451409,-2.05895449464387,
125.255181758744));
#262541=CARTESIAN_POINT('Ctrl Pts',(-190.73064394413,-2.20494080910687,
125.313808132539));
#262542=CARTESIAN_POINT('Ctrl Pts',(-190.738051290484,-2.35078641646454,
125.372378000029));
#262543=CARTESIAN_POINT('Ctrl Pts',(-190.745458636838,-2.49444561681005,
125.436822826783));
#262544=CARTESIAN_POINT('Ctrl Pts',(-190.752865983192,-2.63541380355637,
125.506953266179));
#262545=CARTESIAN_POINT('Ctrl Pts',(-190.760267804868,-2.7762768509102,
125.577031399648));
#262546=CARTESIAN_POINT('Ctrl Pts',(-190.767669626543,-2.91445254820704,
125.652786536705));
#262547=CARTESIAN_POINT('Ctrl Pts',(-190.775071448219,-3.04945632143417,
125.733981272175));
#262548=CARTESIAN_POINT('Ctrl Pts',(-190.78246936253,-3.18438882722145,
125.815133145578));
#262549=CARTESIAN_POINT('Ctrl Pts',(-190.789867276842,-3.31615242456538,
125.901718706713));
#262550=CARTESIAN_POINT('Ctrl Pts',(-190.797265191153,-3.44428731060594,
125.993454727352));
#262551=CARTESIAN_POINT('Ctrl Pts',(-190.804661876065,-3.5724009029514,
126.085175503127));
#262552=CARTESIAN_POINT('Ctrl Pts',(-190.812058560978,-3.69688667759057,
126.182044822578));
#262553=CARTESIAN_POINT('Ctrl Pts',(-190.81945524589,-3.81731390363919,
126.283736200123));
#262554=CARTESIAN_POINT('Ctrl Pts',(-190.826851602826,-3.9377357898191,
126.385423068566));
#262555=CARTESIAN_POINT('Ctrl Pts',(-190.834247959761,-4.05409920001659,
126.491931329125));
#262556=CARTESIAN_POINT('Ctrl Pts',(-190.841644316697,-4.16600680533306,
126.602894461518));
#262557=CARTESIAN_POINT('Ctrl Pts',(-190.849041806034,-4.27793154398928,
126.713874582649));
#262558=CARTESIAN_POINT('Ctrl Pts',(-190.85643929537,-4.38539885432859,
126.829310670813));
#262559=CARTESIAN_POINT('Ctrl Pts',(-190.863836784707,-4.48804868336094,
126.948799753271));
#262560=CARTESIAN_POINT('Ctrl Pts',(-190.871236867222,-4.59073449613216,
127.068330722442));
#262561=CARTESIAN_POINT('Ctrl Pts',(-190.878636949737,-4.68859922218421,
127.19191723167));
#262562=CARTESIAN_POINT('Ctrl Pts',(-190.886037032252,-4.78132356498639,
127.319123820818));
#262563=CARTESIAN_POINT('Ctrl Pts',(-190.893445251919,-4.87414986773537,
127.446470286688));
#262564=CARTESIAN_POINT('Ctrl Pts',(-190.900853471586,-4.9618242790364,
127.57744448025));
#262565=CARTESIAN_POINT('Ctrl Pts',(-190.908261691252,-5.04407086463152,
127.711581984189));
#262566=CARTESIAN_POINT('Ctrl Pts',(-190.915674470554,-5.12636807162771,
127.845802047523));
#262567=CARTESIAN_POINT('Ctrl Pts',(-190.923087249857,-5.20323061424422,
127.98318897578));
#262568=CARTESIAN_POINT('Ctrl Pts',(-190.930500029159,-5.27442913803752,
128.123254907169));
#262569=CARTESIAN_POINT('Ctrl Pts',(-190.937923400188,-5.3457293936204,
128.26352097133));
#262570=CARTESIAN_POINT('Ctrl Pts',(-190.945346771217,-5.41134931149239,
128.406473345405));
#262571=CARTESIAN_POINT('Ctrl Pts',(-190.952770142245,-5.47110785050535,
128.551604649726));
#262572=CARTESIAN_POINT('Ctrl Pts',(-190.956706191685,-5.50279326176559,
128.628556749628));
#262573=CARTESIAN_POINT('Ctrl Pts',(-190.960642241124,-5.53283166141068,
128.706121167425));
#262574=CARTESIAN_POINT('Ctrl Pts',(-190.964578290564,-5.56120182518544,
128.784220814965));
#262575=CARTESIAN_POINT('Ctrl Pts',(-190.973177240122,-5.62318112981626,
128.954842383627));
#262576=CARTESIAN_POINT('Ctrl Pts',(-190.98177618968,-5.67735007641122,
129.128443962409));
#262577=CARTESIAN_POINT('Ctrl Pts',(-190.990375139238,-5.72345280997876,
129.304354452763));
#262578=CARTESIAN_POINT('Ctrl Pts',(-190.998941388787,-5.76938022448008,
129.479595992265));
#262579=CARTESIAN_POINT('Ctrl Pts',(-191.007507638336,-5.80730256775135,
129.657128801406));
#262580=CARTESIAN_POINT('Ctrl Pts',(-191.016073887885,-5.83701346337239,
129.836267444927));
#262581=CARTESIAN_POINT('Ctrl Pts',(-191.024576231815,-5.8665027108652,
130.014069684944));
#262582=CARTESIAN_POINT('Ctrl Pts',(-191.033078575745,-5.88790249831863,
130.19345375926));
#262583=CARTESIAN_POINT('Ctrl Pts',(-191.041580919675,-5.90105816818685,
130.373729617549));
#262584=CARTESIAN_POINT('Ctrl Pts',(-191.048262204323,-5.91139611450565,
130.515393414546));
#262585=CARTESIAN_POINT('Ctrl Pts',(-191.054943488972,-5.9166441504911,
130.657607486087));
#262586=CARTESIAN_POINT('Ctrl Pts',(-191.06162477362,-5.91674841448608,
130.80002908476));
#262587=CARTESIAN_POINT('',(-192.811624807792,-5.9097125884178,130.808293688258));
#262588=CARTESIAN_POINT('Ctrl Pts',(-191.061624807792,-5.91047567621124,
130.800034404554));
#262589=CARTESIAN_POINT('Ctrl Pts',(-191.12209184332,-5.90179870917759,
132.087620467717));
#262590=CARTESIAN_POINT('Ctrl Pts',(-191.275374753451,-4.85401633074215,
135.36448301843));
#262591=CARTESIAN_POINT('Ctrl Pts',(-191.52147353819,0.560953822592365,
137.780239869629));
#262592=CARTESIAN_POINT('Ctrl Pts',(-191.799921162001,6.17221402509524,
134.103047410633));
#262593=CARTESIAN_POINT('Ctrl Pts',(-192.078368785815,6.11151106794695,
127.394522938632));
#262594=CARTESIAN_POINT('Ctrl Pts',(-192.356816409627,0.434628003272854,
123.819472713731));
#262595=CARTESIAN_POINT('Ctrl Pts',(-192.601235083619,-4.89907710821755,
126.315663527414));
#262596=CARTESIAN_POINT('Ctrl Pts',(-192.752837883008,-5.902105290066,129.556078088356));
#262597=CARTESIAN_POINT('Ctrl Pts',(-192.811624807792,-5.9097125884178,
130.808293688258));
#262598=CARTESIAN_POINT('',(-194.561624807792,-5.92485436802142,130.807214191615));
#262599=CARTESIAN_POINT('Ctrl Pts',(-192.811624807792,-5.9097125884178,
130.808293688258));
#262600=CARTESIAN_POINT('Ctrl Pts',(-192.845653757612,-5.91411609097954,
131.533141636508));
#262601=CARTESIAN_POINT('Ctrl Pts',(-192.972498582038,-5.45424420182938,
134.22966001815));
#262602=CARTESIAN_POINT('Ctrl Pts',(-193.192159281066,-1.42141332660588,
137.656888960118));
#262603=CARTESIAN_POINT('Ctrl Pts',(-193.47060690488,4.99691754528912,135.704194857198));
#262604=CARTESIAN_POINT('Ctrl Pts',(-193.749054528692,6.82332530604844,
129.248792458293));
#262605=CARTESIAN_POINT('Ctrl Pts',(-194.027502152505,2.37943044852847,
124.222881204015));
#262606=CARTESIAN_POINT('Ctrl Pts',(-194.298358912204,-4.07028890202498,
125.217162883923));
#262607=CARTESIAN_POINT('Ctrl Pts',(-194.476399797301,-5.91415325007818,
129.003717447568));
#262608=CARTESIAN_POINT('Ctrl Pts',(-194.561624807792,-5.92485436802142,
130.807214191615));
#262609=CARTESIAN_POINT('',(-196.311624807792,-5.91811478187531,130.799043979201));
#262610=CARTESIAN_POINT('Ctrl Pts',(-194.561624807792,-5.92485436802142,
130.807214191615));
#262611=CARTESIAN_POINT('Ctrl Pts',(-194.569215671905,-5.92580750057834,
130.96784894699));
#262612=CARTESIAN_POINT('Ctrl Pts',(-194.576806536018,-5.91984348713247,
131.128411830021));
#262613=CARTESIAN_POINT('Ctrl Pts',(-194.677213274735,-5.74644163664981,
133.244482439234));
#262614=CARTESIAN_POINT('Ctrl Pts',(-194.862845023943,-3.28928991419861,
136.981587535098));
#262615=CARTESIAN_POINT('Ctrl Pts',(-195.141292647756,3.41913440987934,
136.910675415994));
#262616=CARTESIAN_POINT('Ctrl Pts',(-195.419740271569,6.98554124528268,
131.228358307197));
#262617=CARTESIAN_POINT('Ctrl Pts',(-195.698187895382,4.13257693892937,
125.156408035065));
#262618=CARTESIAN_POINT('Ctrl Pts',(-195.976635519195,-2.5180236866903,
124.27465026843));
#262619=CARTESIAN_POINT('Ctrl Pts',(-196.181114489998,-5.70266478639503,
128.033605093401));
#262620=CARTESIAN_POINT('Ctrl Pts',(-196.292777586197,-5.92224318811939,
130.39909676226));
#262621=CARTESIAN_POINT('Ctrl Pts',(-196.311624807792,-5.91853255389597,
130.799043603888));
#262622=CARTESIAN_POINT('',(-198.061624807755,-5.91674998668501,130.803963675558));
#262623=CARTESIAN_POINT('Ctrl Pts',(-196.311624807792,-5.91674761240624,
130.79904520742));
#262624=CARTESIAN_POINT('Ctrl Pts',(-196.318927817343,-5.91688679200283,
130.953970325757));
#262625=CARTESIAN_POINT('Ctrl Pts',(-196.326230826894,-5.91093694148842,
131.109091464218));
#262626=CARTESIAN_POINT('Ctrl Pts',(-196.333533836445,-5.89887867729289,
131.263883101324));
#262627=CARTESIAN_POINT('Ctrl Pts',(-196.340831042499,-5.88682999546239,
131.41855172985));
#262628=CARTESIAN_POINT('Ctrl Pts',(-196.348128248553,-5.86868258965433,
131.572890996276));
#262629=CARTESIAN_POINT('Ctrl Pts',(-196.355425454607,-5.84446913863302,
131.726375286683));
#262630=CARTESIAN_POINT('Ctrl Pts',(-196.362846509282,-5.81984473545903,
131.882464521733));
#262631=CARTESIAN_POINT('Ctrl Pts',(-196.370267563958,-5.78894650617216,
132.037669091922));
#262632=CARTESIAN_POINT('Ctrl Pts',(-196.377688618634,-5.75186394852528,
132.191440889272));
#262633=CARTESIAN_POINT('Ctrl Pts',(-196.3849802672,-5.71542802531407,132.342531260482));
#262634=CARTESIAN_POINT('Ctrl Pts',(-196.392271915766,-5.67302179942338,
132.492238033825));
#262635=CARTESIAN_POINT('Ctrl Pts',(-196.399563564333,-5.62478171151197,
132.640051566593));
#262636=CARTESIAN_POINT('Ctrl Pts',(-196.40685488677,-5.57654378120929,
132.787858488184));
#262637=CARTESIAN_POINT('Ctrl Pts',(-196.414146209206,-5.52247262718137,
132.933771971568));
#262638=CARTESIAN_POINT('Ctrl Pts',(-196.421437531643,-5.46275434354564,
133.077298263999));
#262639=CARTESIAN_POINT('Ctrl Pts',(-196.428730063846,-5.40302615153141,
133.220848370123));
#262640=CARTESIAN_POINT('Ctrl Pts',(-196.43602259605,-5.3376491138028,133.362010141883));
#262641=CARTESIAN_POINT('Ctrl Pts',(-196.443315128253,-5.26685704862626,
133.500310801052));
#262642=CARTESIAN_POINT('Ctrl Pts',(-196.450833098134,-5.19387655310716,
133.642886817326));
#262643=CARTESIAN_POINT('Ctrl Pts',(-196.458351068014,-5.11514103364721,
133.782421580859));
#262644=CARTESIAN_POINT('Ctrl Pts',(-196.465869037895,-5.03095663489101,
133.918426432597));
#262645=CARTESIAN_POINT('Ctrl Pts',(-196.473172341532,-4.9491760165358,
134.050547835598));
#262646=CARTESIAN_POINT('Ctrl Pts',(-196.480475645169,-4.86225370657967,
134.179337872425));
#262647=CARTESIAN_POINT('Ctrl Pts',(-196.487778948806,-4.77051280347123,
134.304380353856));
#262648=CARTESIAN_POINT('Ctrl Pts',(-196.495404251808,-4.67472708529593,
134.434935901931));
#262649=CARTESIAN_POINT('Ctrl Pts',(-196.503029554811,-4.57368851682401,
134.561405546719));
#262650=CARTESIAN_POINT('Ctrl Pts',(-196.510654857813,-4.467808907599,134.683357153744));
#262651=CARTESIAN_POINT('Ctrl Pts',(-196.518280160816,-4.361929298374,134.805308760768));
#262652=CARTESIAN_POINT('Ctrl Pts',(-196.525905463818,-4.25120902523955,
134.922742040811));
#262653=CARTESIAN_POINT('Ctrl Pts',(-196.53353076682,-4.13609959561202,
135.035271949381));
#262654=CARTESIAN_POINT('Ctrl Pts',(-196.540954033226,-4.024040053635,135.144820316129));
#262655=CARTESIAN_POINT('Ctrl Pts',(-196.548377299631,-3.90745582610583,
135.250079258993));
#262656=CARTESIAN_POINT('Ctrl Pts',(-196.555800566037,-3.78670891927233,
135.350652086797));
#262657=CARTESIAN_POINT('Ctrl Pts',(-196.563215058758,-3.66610472525497,
135.451106045871));
#262658=CARTESIAN_POINT('Ctrl Pts',(-196.570629551479,-3.5413479291358,
135.546884677918));
#262659=CARTESIAN_POINT('Ctrl Pts',(-196.578044044199,-3.41283794674118,
135.63762739189));
#262660=CARTESIAN_POINT('Ctrl Pts',(-196.585451390553,-3.28445182710626,
135.728282644617));
#262661=CARTESIAN_POINT('Ctrl Pts',(-196.592858736907,-3.15232002574301,
135.813911428368));
#262662=CARTESIAN_POINT('Ctrl Pts',(-196.60026608326,-3.0168755761589,135.894192866322));
#262663=CARTESIAN_POINT('Ctrl Pts',(-196.607667904936,-2.88153214615492,
135.974414427351));
#262664=CARTESIAN_POINT('Ctrl Pts',(-196.615069726611,-2.74288130716737,
136.049296394212));
#262665=CARTESIAN_POINT('Ctrl Pts',(-196.622471548287,-2.60138556712834,
136.118560810788));
#262666=CARTESIAN_POINT('Ctrl Pts',(-196.629869462598,-2.45996452158867,
136.187788663217));
#262667=CARTESIAN_POINT('Ctrl Pts',(-196.637267376909,-2.31570190033966,
136.251404707507));
#262668=CARTESIAN_POINT('Ctrl Pts',(-196.644665291221,-2.1690852351992,
136.309176673071));
#262669=CARTESIAN_POINT('Ctrl Pts',(-196.652061976133,-2.02249293508921,
136.366939037981));
#262670=CARTESIAN_POINT('Ctrl Pts',(-196.659458661045,-1.87354771447102,
136.418859114951));
#262671=CARTESIAN_POINT('Ctrl Pts',(-196.666855345957,-1.72275763897961,
136.464752536845));
#262672=CARTESIAN_POINT('Ctrl Pts',(-196.674251702893,-1.57197424967773,
136.510643923776));
#262673=CARTESIAN_POINT('Ctrl Pts',(-196.681648059828,-1.41934652527773,
136.550509078279));
#262674=CARTESIAN_POINT('Ctrl Pts',(-196.689044416763,-1.26539800768293,
136.584213422323));
#262675=CARTESIAN_POINT('Ctrl Pts',(-196.6964419061,-1.11142592017751,136.617922926587));
#262676=CARTESIAN_POINT('Ctrl Pts',(-196.703839395436,-0.956133001520995,
136.645469662442));
#262677=CARTESIAN_POINT('Ctrl Pts',(-196.711236884773,-0.800053158089319,
136.666770148359));
#262678=CARTESIAN_POINT('Ctrl Pts',(-196.718636967288,-0.643918601110704,
136.688078101128));
#262679=CARTESIAN_POINT('Ctrl Pts',(-196.726037049803,-0.486996939769862,
136.703135394011));
#262680=CARTESIAN_POINT('Ctrl Pts',(-196.733437132318,-0.329827225310558,
136.711910411173));
#262681=CARTESIAN_POINT('Ctrl Pts',(-196.740845351984,-0.172484686592092,
136.720695077368));
#262682=CARTESIAN_POINT('Ctrl Pts',(-196.748253571651,-0.0148939229818671,
136.723183651275));
#262683=CARTESIAN_POINT('Ctrl Pts',(-196.755661791317,0.142405248829505,
136.719396653602));
#262684=CARTESIAN_POINT('Ctrl Pts',(-196.763074570619,0.299801235656451,
136.715607325096));
#262685=CARTESIAN_POINT('Ctrl Pts',(-196.770487349921,0.456904901399012,
136.705534752304));
#262686=CARTESIAN_POINT('Ctrl Pts',(-196.777900129223,0.613182040216748,
136.689251300328));
#262687=CARTESIAN_POINT('Ctrl Pts',(-196.785323500252,0.769682475138877,
136.672944581791));
#262688=CARTESIAN_POINT('Ctrl Pts',(-196.792746871281,0.925353655985176,
136.650409313252));
#262689=CARTESIAN_POINT('Ctrl Pts',(-196.80017024231,1.07967122626914,136.621769027302));
#262690=CARTESIAN_POINT('Ctrl Pts',(-196.804106291751,1.16149410484353,
136.606583260475));
#262691=CARTESIAN_POINT('Ctrl Pts',(-196.808042341192,1.24293667063961,
136.589681992946));
#262692=CARTESIAN_POINT('Ctrl Pts',(-196.811978390633,1.32392266781222,
136.571089268383));
#262693=CARTESIAN_POINT('Ctrl Pts',(-196.819401657039,1.47665973097384,
136.536023970121));
#262694=CARTESIAN_POINT('Ctrl Pts',(-196.826824923444,1.62823368340216,
136.494833387375));
#262695=CARTESIAN_POINT('Ctrl Pts',(-196.83424818985,1.7781151043552,136.447607664982));
#262696=CARTESIAN_POINT('Ctrl Pts',(-196.841662682571,1.92781937791556,
136.40043775947));
#262697=CARTESIAN_POINT('Ctrl Pts',(-196.849077175292,2.07583474930553,
136.347247023744));
#262698=CARTESIAN_POINT('Ctrl Pts',(-196.856491668013,2.22164194905233,
136.288176589379));
#262699=CARTESIAN_POINT('Ctrl Pts',(-196.863899014366,2.36730861433047,
136.229163089323));
#262700=CARTESIAN_POINT('Ctrl Pts',(-196.87130636072,2.51077100136879,136.164281311885));
#262701=CARTESIAN_POINT('Ctrl Pts',(-196.878713707074,2.65152508222352,
136.093722138661));
#262702=CARTESIAN_POINT('Ctrl Pts',(-196.886115528749,2.79217418337481,
136.02321559113));
#262703=CARTESIAN_POINT('Ctrl Pts',(-196.893517350425,2.93011866807073,
135.947040245676));
#262704=CARTESIAN_POINT('Ctrl Pts',(-196.9009191721,3.06487468712279,135.865434981249));
#262705=CARTESIAN_POINT('Ctrl Pts',(-196.908317086411,3.19955956952096,
135.783872795607));
#262706=CARTESIAN_POINT('Ctrl Pts',(-196.915715000723,3.33105901987783,
135.696886592468));
#262707=CARTESIAN_POINT('Ctrl Pts',(-196.923112915034,3.45891409951243,
135.604760998232));
#262708=CARTESIAN_POINT('Ctrl Pts',(-196.930509599946,3.5867479319525,135.512650713597));
#262709=CARTESIAN_POINT('Ctrl Pts',(-196.937906284858,3.7109382930943,135.415402950964));
#262710=CARTESIAN_POINT('Ctrl Pts',(-196.94530296977,3.83105544775849,135.313345505398));
#262711=CARTESIAN_POINT('Ctrl Pts',(-196.952699326706,3.95116727630217,
135.211292585167));
#262712=CARTESIAN_POINT('Ctrl Pts',(-196.960095683641,4.0672059730031,135.104430647757));
#262713=CARTESIAN_POINT('Ctrl Pts',(-196.967492040577,4.17877532636475,
134.993127421085));
#262714=CARTESIAN_POINT('Ctrl Pts',(-196.974889529913,4.29036176127955,
134.881807153605));
#262715=CARTESIAN_POINT('Ctrl Pts',(-196.98228701925,4.39747722609323,134.766044506611));
#262716=CARTESIAN_POINT('Ctrl Pts',(-196.989684508586,4.49976289599391,
134.646243546852));
#262717=CARTESIAN_POINT('Ctrl Pts',(-196.997084591101,4.60208442197746,
134.526400591052));
#262718=CARTESIAN_POINT('Ctrl Pts',(-197.004484673616,4.69957253990412,
134.40251678771));
#262719=CARTESIAN_POINT('Ctrl Pts',(-197.011884756131,4.79190928011303,
134.275028566775));
#262720=CARTESIAN_POINT('Ctrl Pts',(-197.019292975798,4.88434755406011,
134.147400159435));
#262721=CARTESIAN_POINT('Ctrl Pts',(-197.026701195464,4.97162291886746,
134.01615972179));
#262722=CARTESIAN_POINT('Ctrl Pts',(-197.034109415131,5.05346085508178,
133.881772508856));
#262723=CARTESIAN_POINT('Ctrl Pts',(-197.041522194433,5.13534916118031,
133.747302582836));
#262724=CARTESIAN_POINT('Ctrl Pts',(-197.048934973735,5.2117931892249,133.609682347809));
#262725=CARTESIAN_POINT('Ctrl Pts',(-197.056347753037,5.28256507071789,
133.469400361384));
#262726=CARTESIAN_POINT('Ctrl Pts',(-197.063771124065,5.35343807439412,
133.328917933479));
#262727=CARTESIAN_POINT('Ctrl Pts',(-197.071194495094,5.41862259046731,
133.185766497095));
#262728=CARTESIAN_POINT('Ctrl Pts',(-197.078617866123,5.47793912291705,
133.04045398058));
#262729=CARTESIAN_POINT('Ctrl Pts',(-197.082553915564,5.50939017170535,
132.963405797591));
#262730=CARTESIAN_POINT('Ctrl Pts',(-197.086489965005,5.53919235282093,
132.88575031248));
#262731=CARTESIAN_POINT('Ctrl Pts',(-197.090426014446,5.56732467673674,
132.80756467764));
#262732=CARTESIAN_POINT('Ctrl Pts',(-197.097849280852,5.62038136165785,
132.660109010435));
#262733=CARTESIAN_POINT('Ctrl Pts',(-197.105272547257,5.66765598150285,
132.510321035348));
#262734=CARTESIAN_POINT('Ctrl Pts',(-197.112695813663,5.70893821283385,
132.35869489453));
#262735=CARTESIAN_POINT('Ctrl Pts',(-197.120110306384,5.75017165199582,
132.207247963219));
#262736=CARTESIAN_POINT('Ctrl Pts',(-197.127524799105,5.7854267033022,132.053967547337));
#262737=CARTESIAN_POINT('Ctrl Pts',(-197.134939291826,5.81454142691153,
131.899366808064));
#262738=CARTESIAN_POINT('Ctrl Pts',(-197.14234663818,5.84362808865393,131.744915078805));
#262739=CARTESIAN_POINT('Ctrl Pts',(-197.149753984533,5.86658613620568,
131.589145923993));
#262740=CARTESIAN_POINT('Ctrl Pts',(-197.157161330887,5.88330372424391,
131.432586572775));
#262741=CARTESIAN_POINT('Ctrl Pts',(-197.164563152563,5.90000884367436,
131.276143989427));
#262742=CARTESIAN_POINT('Ctrl Pts',(-197.171964974238,5.91048273160501,
131.118912752756));
#262743=CARTESIAN_POINT('Ctrl Pts',(-197.179366795914,5.91466483135784,
130.961429058695));
#262744=CARTESIAN_POINT('Ctrl Pts',(-197.186764710225,5.91884472341276,
130.804028499051));
#262745=CARTESIAN_POINT('Ctrl Pts',(-197.194162624536,5.91673943210462,
130.646376119654));
#262746=CARTESIAN_POINT('Ctrl Pts',(-197.201560538848,5.90834035411677,
130.489011886135));
#262747=CARTESIAN_POINT('Ctrl Pts',(-197.20895722376,5.8999426719033,130.331673803696));
#262748=CARTESIAN_POINT('Ctrl Pts',(-197.216353908672,5.8852532987146,130.1746241445));
#262749=CARTESIAN_POINT('Ctrl Pts',(-197.223750593585,5.86431573546309,
130.018401638166));
#262750=CARTESIAN_POINT('Ctrl Pts',(-197.23114695052,5.84337910060514,129.862186058901));
#262751=CARTESIAN_POINT('Ctrl Pts',(-197.238543307455,5.81619487614345,
129.706797929561));
#262752=CARTESIAN_POINT('Ctrl Pts',(-197.245939664391,5.7828582799976,129.552769360021));
#262753=CARTESIAN_POINT('Ctrl Pts',(-197.253337153727,5.74951657993387,
129.398717208314));
#262754=CARTESIAN_POINT('Ctrl Pts',(-197.260734643064,5.71002071162072,
129.246025395738));
#262755=CARTESIAN_POINT('Ctrl Pts',(-197.268132132401,5.66451667428286,
129.09521421972));
#262756=CARTESIAN_POINT('Ctrl Pts',(-197.275532214916,5.61899668557493,
128.944350177076));
#262757=CARTESIAN_POINT('Ctrl Pts',(-197.282932297431,5.56746444227009,
128.79536844072));
#262758=CARTESIAN_POINT('Ctrl Pts',(-197.290332379946,5.51011525487502,
128.648772428581));
#262759=CARTESIAN_POINT('Ctrl Pts',(-197.297740599612,5.45270300615285,
128.502015219055));
#262760=CARTESIAN_POINT('Ctrl Pts',(-197.305148819279,5.38946117553666,
128.357649320603));
#262761=CARTESIAN_POINT('Ctrl Pts',(-197.312557038945,5.32063281077705,
128.216157175913));
#262762=CARTESIAN_POINT('Ctrl Pts',(-197.319969818248,5.2517620833074,128.07457794517));
#262763=CARTESIAN_POINT('Ctrl Pts',(-197.32738259755,5.17729814637798,127.935876320775));
#262764=CARTESIAN_POINT('Ctrl Pts',(-197.334795376852,5.09752886885128,
127.80050809227));
#262765=CARTESIAN_POINT('Ctrl Pts',(-197.34221874788,5.01764561323994,127.664946443292));
#262766=CARTESIAN_POINT('Ctrl Pts',(-197.349642118909,4.93244207870739,
127.532728015764));
#262767=CARTESIAN_POINT('Ctrl Pts',(-197.357065489938,4.84224857777326,
127.40427837245));
#262768=CARTESIAN_POINT('Ctrl Pts',(-197.361001539378,4.79442581941926,
127.336171289465));
#262769=CARTESIAN_POINT('Ctrl Pts',(-197.364937588819,4.74520086733818,
127.26912318392));
#262770=CARTESIAN_POINT('Ctrl Pts',(-197.368873638259,4.69462728667099,
127.203193417651));
#262771=CARTESIAN_POINT('Ctrl Pts',(-197.376296904665,4.59924709187124,
127.078851936054));
#262772=CARTESIAN_POINT('Ctrl Pts',(-197.38372017107,4.49877931298799,126.958114400183));
#262773=CARTESIAN_POINT('Ctrl Pts',(-197.391143437476,4.39352600085202,
126.841424857004));
#262774=CARTESIAN_POINT('Ctrl Pts',(-197.398557930197,4.28839708939024,
126.724873231176));
#262775=CARTESIAN_POINT('Ctrl Pts',(-197.405972422918,4.17849415076658,
126.612360349171));
#262776=CARTESIAN_POINT('Ctrl Pts',(-197.413386915639,4.06416138957402,
126.504299831717));
#262777=CARTESIAN_POINT('Ctrl Pts',(-197.420794261992,3.94993882660157,
126.396343467059));
#262778=CARTESIAN_POINT('Ctrl Pts',(-197.428201608346,3.83129521052947,
126.292831178398));
#262779=CARTESIAN_POINT('Ctrl Pts',(-197.4356089547,3.70861365904349,126.194142044607));
#262780=CARTESIAN_POINT('Ctrl Pts',(-197.443010776375,3.58602360808748,
126.095526516895));
#262781=CARTESIAN_POINT('Ctrl Pts',(-197.450412598051,3.45940190792309,
126.001727214337));
#262782=CARTESIAN_POINT('Ctrl Pts',(-197.457814419726,3.32916694301156,
125.91308491198));
#262783=CARTESIAN_POINT('Ctrl Pts',(-197.465212334038,3.19900072812314,
125.824489403203));
#262784=CARTESIAN_POINT('Ctrl Pts',(-197.472610248349,3.06522535501235,
125.741045682467));
#262785=CARTESIAN_POINT('Ctrl Pts',(-197.48000816266,2.92829046175452,125.6630528526));
#262786=CARTESIAN_POINT('Ctrl Pts',(-197.487404847572,2.79137832459229,
125.585072983727));
#262787=CARTESIAN_POINT('Ctrl Pts',(-197.494801532485,2.65130803341802,
125.512542392469));
#262788=CARTESIAN_POINT('Ctrl Pts',(-197.502198217397,2.50855635002252,
125.445715676794));
#262789=CARTESIAN_POINT('Ctrl Pts',(-197.509594574332,2.36581099638625,
125.378891924286));
#262790=CARTESIAN_POINT('Ctrl Pts',(-197.516990931268,2.22038482501944,
125.317771702748));
#262791=CARTESIAN_POINT('Ctrl Pts',(-197.524387288203,2.0727769826413,125.262562521033));
#262792=CARTESIAN_POINT('Ctrl Pts',(-197.53178477754,1.9251465411261,125.207344886652));
#262793=CARTESIAN_POINT('Ctrl Pts',(-197.539182266876,1.77533411318653,
125.158040224843));
#262794=CARTESIAN_POINT('Ctrl Pts',(-197.546579756213,1.62385635592891,
125.11480693579));
#262795=CARTESIAN_POINT('Ctrl Pts',(-197.553979838728,1.47232549837808,
125.071558491375));
#262796=CARTESIAN_POINT('Ctrl Pts',(-197.561379921243,1.31912850795002,
125.034385759555));
#262797=CARTESIAN_POINT('Ctrl Pts',(-197.568780003758,1.16479449450476,
125.003396529755));
#262798=CARTESIAN_POINT('Ctrl Pts',(-197.576188223424,1.01029077494556,
124.972373224112));
#262799=CARTESIAN_POINT('Ctrl Pts',(-197.583596443091,0.854647901707854,
124.947547072864));
#262800=CARTESIAN_POINT('Ctrl Pts',(-197.591004662757,0.698403140736846,
124.928974365113));
#262801=CARTESIAN_POINT('Ctrl Pts',(-197.598417442059,0.542062213722543,
124.910390226172));
#262802=CARTESIAN_POINT('Ctrl Pts',(-197.605830221361,0.38511903209279,
124.898067229277));
#262803=CARTESIAN_POINT('Ctrl Pts',(-197.613243000663,0.228112664648767,
124.892009547583));
#262804=CARTESIAN_POINT('Ctrl Pts',(-197.620666371692,0.0708819591442937,
124.88594321039));
#262805=CARTESIAN_POINT('Ctrl Pts',(-197.628089742721,-0.0864117401809329,
124.886160067387));
#262806=CARTESIAN_POINT('Ctrl Pts',(-197.63551311375,-0.243231853336173,
124.892612244367));
#262807=CARTESIAN_POINT('Ctrl Pts',(-197.639449163191,-0.326381640180508,
124.896033343419));
#262808=CARTESIAN_POINT('Ctrl Pts',(-197.643385212631,-0.409398399272633,
124.901206550941));
#262809=CARTESIAN_POINT('Ctrl Pts',(-197.647321262072,-0.492203234551277,
124.908118887583));
#262810=CARTESIAN_POINT('Ctrl Pts',(-197.654744528478,-0.64837056963286,
124.921155338763));
#262811=CARTESIAN_POINT('Ctrl Pts',(-197.662167794883,-0.804255766574924,
124.940420139216));
#262812=CARTESIAN_POINT('Ctrl Pts',(-197.669591061289,-0.959321970235522,
124.965899183256));
#262813=CARTESIAN_POINT('Ctrl Pts',(-197.67700555401,-1.11420489852084,
124.991348113182));
#262814=CARTESIAN_POINT('Ctrl Pts',(-197.684420046731,-1.26827039553683,
125.022996607056));
#262815=CARTESIAN_POINT('Ctrl Pts',(-197.691834539452,-1.42098441946168,
125.060778647911));
#262816=CARTESIAN_POINT('Ctrl Pts',(-197.699241885806,-1.57355125186026,
125.098524273012));
#262817=CARTESIAN_POINT('Ctrl Pts',(-197.706649232159,-1.72476884444938,
125.142391586927));
#262818=CARTESIAN_POINT('Ctrl Pts',(-197.714056578513,-1.87411118297151,
125.192263163284));
#262819=CARTESIAN_POINT('Ctrl Pts',(-197.721458400189,-2.02334213634406,
125.242097543538));
#262820=CARTESIAN_POINT('Ctrl Pts',(-197.728860221864,-2.17070026796815,
125.297927151792));
#262821=CARTESIAN_POINT('Ctrl Pts',(-197.73626204354,-2.31567272712397,
125.359584186586));
#262822=CARTESIAN_POINT('Ctrl Pts',(-197.743659957851,-2.46056865644708,
125.421208673112));
#262823=CARTESIAN_POINT('Ctrl Pts',(-197.751057872162,-2.60308107876267,
125.488654313942));
#262824=CARTESIAN_POINT('Ctrl Pts',(-197.758455786474,-2.74271531002859,
125.561704488214));
#262825=CARTESIAN_POINT('Ctrl Pts',(-197.765852471386,-2.88232633661789,
125.634742522872));
#262826=CARTESIAN_POINT('Ctrl Pts',(-197.773249156298,-3.01905979100342,
125.713383069601));
#262827=CARTESIAN_POINT('Ctrl Pts',(-197.780645841211,-3.15244377131063,
125.797362631624));
#262828=CARTESIAN_POINT('Ctrl Pts',(-197.788042198146,-3.28582183723238,
125.881338469906));
#262829=CARTESIAN_POINT('Ctrl Pts',(-197.795438555081,-3.41585040848234,
125.970652653875));
#262830=CARTESIAN_POINT('Ctrl Pts',(-197.802834912017,-3.54208510099192,
126.064997400864));
#262831=CARTESIAN_POINT('Ctrl Pts',(-197.810232401353,-3.66833912035446,
126.159356592273));
#262832=CARTESIAN_POINT('Ctrl Pts',(-197.81762989069,-3.79079780538828,
126.258747656766));
#262833=CARTESIAN_POINT('Ctrl Pts',(-197.825027380027,-3.90904862374609,
126.362821535256));
#262834=CARTESIAN_POINT('Ctrl Pts',(-197.832427462542,-4.02734089474615,
126.466931896683));
#262835=CARTESIAN_POINT('Ctrl Pts',(-197.839827545057,-4.14142208218471,
126.575728093952));
#262836=CARTESIAN_POINT('Ctrl Pts',(-197.847227627572,-4.2509155029613,
126.688823234771));
#262837=CARTESIAN_POINT('Ctrl Pts',(-197.854635847238,-4.36052932300976,
126.802042735323));
#262838=CARTESIAN_POINT('Ctrl Pts',(-197.862044066905,-4.46554504194146,
126.919570351452));
#262839=CARTESIAN_POINT('Ctrl Pts',(-197.869452286571,-4.56562489677327,
127.040984491736));
#262840=CARTESIAN_POINT('Ctrl Pts',(-197.876865065873,-4.66576634908582,
127.162473360399));
#262841=CARTESIAN_POINT('Ctrl Pts',(-197.884277845175,-4.76096565859968,
127.287853223139));
#262842=CARTESIAN_POINT('Ctrl Pts',(-197.891690624478,-4.8509279344683,
127.416672801799));
#262843=CARTESIAN_POINT('Ctrl Pts',(-197.899113995506,-4.94101875265536,
127.545676443914));
#262844=CARTESIAN_POINT('Ctrl Pts',(-197.906537366535,-5.02585739131891,
127.678129304451));
#262845=CARTESIAN_POINT('Ctrl Pts',(-197.913960737564,-5.10519409379517,
127.813554066286));
#262846=CARTESIAN_POINT('Ctrl Pts',(-197.917896787004,-5.14726031710364,
127.88535952448));
#262847=CARTESIAN_POINT('Ctrl Pts',(-197.921832836445,-5.18778053718604,
127.958000120082));
#262848=CARTESIAN_POINT('Ctrl Pts',(-197.925768885886,-5.22672302868686,
128.031402459949));
#262849=CARTESIAN_POINT('Ctrl Pts',(-197.933618442971,-5.30438498764153,
128.177786763732));
#262850=CARTESIAN_POINT('Ctrl Pts',(-197.941468000057,-5.37598238513895,
128.327603249052));
#262851=CARTESIAN_POINT('Ctrl Pts',(-197.949317557143,-5.44121712518422,
128.480336788277));
#262852=CARTESIAN_POINT('Ctrl Pts',(-197.957153559567,-5.50633921749837,
128.632806586333));
#262853=CARTESIAN_POINT('Ctrl Pts',(-197.964989561992,-5.56512043354741,
128.788183113502));
#262854=CARTESIAN_POINT('Ctrl Pts',(-197.972825564417,-5.6173084054525,
128.94592664227));
#262855=CARTESIAN_POINT('Ctrl Pts',(-197.98064289557,-5.66937202622657,
129.103294306917));
#262856=CARTESIAN_POINT('Ctrl Pts',(-197.988460226724,-5.71487364188634,
129.263017430468));
#262857=CARTESIAN_POINT('Ctrl Pts',(-197.996277557878,-5.75360906848479,
129.424536987695));
#262858=CARTESIAN_POINT('Ctrl Pts',(-198.004083819218,-5.79228964337747,
129.585827823465));
#262859=CARTESIAN_POINT('Ctrl Pts',(-198.011890080558,-5.82422305311737,
129.748909723495));
#262860=CARTESIAN_POINT('Ctrl Pts',(-198.019696341898,-5.84925431259238,
129.913207123986));
#262861=CARTESIAN_POINT('Ctrl Pts',(-198.027487193755,-5.87423616060821,
130.07718020303));
#262862=CARTESIAN_POINT('Ctrl Pts',(-198.035278045612,-5.89234298762165,
130.242363691703));
#262863=CARTESIAN_POINT('Ctrl Pts',(-198.04306889747,-5.90347053031272,
130.40817094048));
#262864=CARTESIAN_POINT('Ctrl Pts',(-198.049254200898,-5.91230489518304,
130.539808425459));
#262865=CARTESIAN_POINT('Ctrl Pts',(-198.055439504327,-5.91674112270733,
130.671838733572));
#262866=CARTESIAN_POINT('Ctrl Pts',(-198.061624807755,-5.91674998668501,
130.803963675558));
#262867=CARTESIAN_POINT('',(-199.811624807792,-5.91674748832781,130.809812394026));
#262868=CARTESIAN_POINT('Ctrl Pts',(-198.061624807792,-5.91674998668506,
130.803963676344));
#262869=CARTESIAN_POINT('Ctrl Pts',(-198.069335284224,-5.91676103632174,
130.96866800542));
#262870=CARTESIAN_POINT('Ctrl Pts',(-198.077045760657,-5.90989046074581,
131.133254346916));
#262871=CARTESIAN_POINT('Ctrl Pts',(-198.084756237089,-5.89619368993992,
131.297138999004));
#262872=CARTESIAN_POINT('Ctrl Pts',(-198.09247513413,-5.88248196089642,
131.461202629451));
#262873=CARTESIAN_POINT('Ctrl Pts',(-198.10019403117,-5.86192918777857,
131.624562717793));
#262874=CARTESIAN_POINT('Ctrl Pts',(-198.107912928211,-5.83464232566053,
131.786643414988));
#262875=CARTESIAN_POINT('Ctrl Pts',(-198.115938226668,-5.80627231226227,
131.955157901231));
#262876=CARTESIAN_POINT('Ctrl Pts',(-198.123963525126,-5.77062274114287,
132.122288952053));
#262877=CARTESIAN_POINT('Ctrl Pts',(-198.131988823583,-5.72787106095795,
132.287406021976));
#262878=CARTESIAN_POINT('Ctrl Pts',(-198.13973298131,-5.68661704950663,
132.446738742092));
#262879=CARTESIAN_POINT('Ctrl Pts',(-198.147477139037,-5.63875026118319,
132.604195921967));
#262880=CARTESIAN_POINT('Ctrl Pts',(-198.155221296764,-5.58447970808055,
132.759230677835));
#262881=CARTESIAN_POINT('Ctrl Pts',(-198.162974554244,-5.53014538450852,
132.914447606882));
#262882=CARTESIAN_POINT('Ctrl Pts',(-198.170727811723,-5.46939239828204,
133.067236130232));
#262883=CARTESIAN_POINT('Ctrl Pts',(-198.178481069202,-5.40247702272164,
133.217071247017));
#262884=CARTESIAN_POINT('Ctrl Pts',(-198.186248543322,-5.33543894881967,
133.367181106642));
#262885=CARTESIAN_POINT('Ctrl Pts',(-198.194016017441,-5.26221604894185,
133.514326447479));
#262886=CARTESIAN_POINT('Ctrl Pts',(-198.201783491561,-5.18311009938688,
133.658007452781));
#262887=CARTESIAN_POINT('Ctrl Pts',(-198.202594497607,-5.17485060571508,
133.673009261883));
#262888=CARTESIAN_POINT('Ctrl Pts',(-198.203405503652,-5.16652701566992,
133.687973331658));
#262889=CARTESIAN_POINT('Ctrl Pts',(-198.204216509698,-5.15813969907268,
133.702899112627));
#262890=CARTESIAN_POINT('Ctrl Pts',(-198.211639776104,-5.08136926578121,
133.839517142834));
#262891=CARTESIAN_POINT('Ctrl Pts',(-198.219063042509,-4.9990513182663,
133.973289646283));
#262892=CARTESIAN_POINT('Ctrl Pts',(-198.226486308914,-4.91142183868873,
134.103734207348));
#262893=CARTESIAN_POINT('Ctrl Pts',(-198.233900801635,-4.82389592987909,
134.234024593775));
#262894=CARTESIAN_POINT('Ctrl Pts',(-198.241315294356,-4.73107119111244,
134.360994560333));
#262895=CARTESIAN_POINT('Ctrl Pts',(-198.248729787077,-4.63322964933905,
134.484185827951));
#262896=CARTESIAN_POINT('Ctrl Pts',(-198.256137133431,-4.53548241092728,
134.607258359188));
#262897=CARTESIAN_POINT('Ctrl Pts',(-198.263544479785,-4.43272822641348,
134.726559151738));
#262898=CARTESIAN_POINT('Ctrl Pts',(-198.270951826138,-4.32529254368441,
134.841658596914));
#262899=CARTESIAN_POINT('Ctrl Pts',(-198.278353647814,-4.21793699054084,
134.956672196582));
#262900=CARTESIAN_POINT('Ctrl Pts',(-198.285755469489,-4.10590714512817,
135.067490416427));
#262901=CARTESIAN_POINT('Ctrl Pts',(-198.293157291165,-3.98956880068971,
135.173716559471));
#262902=CARTESIAN_POINT('Ctrl Pts',(-198.300555205476,-3.87329187035737,
135.279886626562));
#262903=CARTESIAN_POINT('Ctrl Pts',(-198.307953119787,-3.75271124559411,
135.381469193533));
#262904=CARTESIAN_POINT('Ctrl Pts',(-198.315351034099,-3.62822957043913,
135.478104378909));
#262905=CARTESIAN_POINT('Ctrl Pts',(-198.322747719011,-3.50376858188041,
135.57472350527));
#262906=CARTESIAN_POINT('Ctrl Pts',(-198.330144403923,-3.37540812416725,
135.666396653101));
#262907=CARTESIAN_POINT('Ctrl Pts',(-198.337541088835,-3.24358400599151,
135.752804146452));
#262908=CARTESIAN_POINT('Ctrl Pts',(-198.344937445771,-3.11176573303569,
135.839207808404));
#262909=CARTESIAN_POINT('Ctrl Pts',(-198.352333802706,-2.97648441719638,
135.920346075478));
#262910=CARTESIAN_POINT('Ctrl Pts',(-198.359730159642,-2.83820470770205,
135.995942707804));
#262911=CARTESIAN_POINT('Ctrl Pts',(-198.367127648978,-2.69990382723119,
136.071550914167));
#262912=CARTESIAN_POINT('Ctrl Pts',(-198.374525138315,-2.55860396661923,
136.141615617351));
#262913=CARTESIAN_POINT('Ctrl Pts',(-198.381922627651,-2.41479407700068,
136.205906704399));
#262914=CARTESIAN_POINT('Ctrl Pts',(-198.389322710166,-2.27093377504764,
136.270220328589));
#262915=CARTESIAN_POINT('Ctrl Pts',(-198.396722792681,-2.12456203282009,
136.328756154751));
#262916=CARTESIAN_POINT('Ctrl Pts',(-198.404122875196,-1.97618731005907,
136.381332401434));
#262917=CARTESIAN_POINT('Ctrl Pts',(-198.411531094863,-1.82764943403772,
136.433966461105));
#262918=CARTESIAN_POINT('Ctrl Pts',(-198.418939314529,-1.67710453105635,
136.480627729429));
#262919=CARTESIAN_POINT('Ctrl Pts',(-198.426347534195,-1.52507644250729,
136.521184246734));
#262920=CARTESIAN_POINT('Ctrl Pts',(-198.433760313498,-1.37295478320602,
136.561765725898));
#262921=CARTESIAN_POINT('Ctrl Pts',(-198.441173092799,-1.21934848271258,
136.596234885463));
#262922=CARTESIAN_POINT('Ctrl Pts',(-198.448585872102,-1.06479056249309,
136.624511098484));
#262923=CARTESIAN_POINT('Ctrl Pts',(-198.45600924313,-0.910011802669364,
136.652827713883));
#262924=CARTESIAN_POINT('Ctrl Pts',(-198.463432614159,-0.754279076069821,
136.67493365743));
#262925=CARTESIAN_POINT('Ctrl Pts',(-198.470855985188,-0.598130326265068,
136.690800176017));
#262926=CARTESIAN_POINT('Ctrl Pts',(-198.474792034629,-0.515336512371863,
136.699212984885));
#262927=CARTESIAN_POINT('Ctrl Pts',(-198.47872808407,-0.432425748835829,
136.705872538709));
#262928=CARTESIAN_POINT('Ctrl Pts',(-198.482664133511,-0.349477975144942,
136.710780489823));
#262929=CARTESIAN_POINT('Ctrl Pts',(-198.490087399917,-0.193041062691021,
136.720036732451));
#262930=CARTESIAN_POINT('Ctrl Pts',(-198.497510666322,-0.0359996055459115,
136.72308761753));
#262931=CARTESIAN_POINT('Ctrl Pts',(-198.504933932728,0.1211129722417,136.719870926107));
#262932=CARTESIAN_POINT('Ctrl Pts',(-198.512348425449,0.278039856009755,
136.716658036546));
#262933=CARTESIAN_POINT('Ctrl Pts',(-198.51976291817,0.435037323525875,
136.707192323227));
#262934=CARTESIAN_POINT('Ctrl Pts',(-198.527177410891,0.591567369173254,
136.691463352378));
#262935=CARTESIAN_POINT('Ctrl Pts',(-198.534584757244,0.74794654526894,
136.675749541703));
#262936=CARTESIAN_POINT('Ctrl Pts',(-198.541992103598,0.903858827456171,
136.653784528579));
#262937=CARTESIAN_POINT('Ctrl Pts',(-198.549399449952,1.05876686124651,
136.62560990754));
#262938=CARTESIAN_POINT('Ctrl Pts',(-198.556801271627,1.2135593587809,136.597456300197));
#262939=CARTESIAN_POINT('Ctrl Pts',(-198.564203093303,1.36734873359921,
136.563102373113));
#262940=CARTESIAN_POINT('Ctrl Pts',(-198.571604914978,1.5196035131144,136.522641454096));
#262941=CARTESIAN_POINT('Ctrl Pts',(-198.57900282929,1.67177791851663,136.482201894084));
#262942=CARTESIAN_POINT('Ctrl Pts',(-198.586400743601,1.82241898210764,
136.43566185819));
#262943=CARTESIAN_POINT('Ctrl Pts',(-198.593798657912,1.97100628646992,
136.383165577519));
#262944=CARTESIAN_POINT('Ctrl Pts',(-198.601195342825,2.11956889831808,
136.330678020777));
#262945=CARTESIAN_POINT('Ctrl Pts',(-198.608592027737,2.26607807668035,
136.27223630799));
#262946=CARTESIAN_POINT('Ctrl Pts',(-198.615988712649,2.41002930388112,
136.208034304692));
#262947=CARTESIAN_POINT('Ctrl Pts',(-198.623385069584,2.55397414813362,
136.143835148178));
#262948=CARTESIAN_POINT('Ctrl Pts',(-198.63078142652,2.6953609258196,136.073876361061));
#262949=CARTESIAN_POINT('Ctrl Pts',(-198.638177783455,2.83370607425544,
135.998399551501));
#262950=CARTESIAN_POINT('Ctrl Pts',(-198.645575272792,2.97207240368668,
135.922911186248));
#262951=CARTESIAN_POINT('Ctrl Pts',(-198.652972762128,3.10739584891269,
135.84190329519));
#262952=CARTESIAN_POINT('Ctrl Pts',(-198.660370251465,3.23921851935599,
135.755662865093));
#262953=CARTESIAN_POINT('Ctrl Pts',(-198.66777033398,3.37108740003226,135.669392203545));
#262954=CARTESIAN_POINT('Ctrl Pts',(-198.675170416495,3.49945275040591,
135.577885555203));
#262955=CARTESIAN_POINT('Ctrl Pts',(-198.68257049901,3.62388679768368,135.481472444332));
#262956=CARTESIAN_POINT('Ctrl Pts',(-198.689978718676,3.74845767298839,
135.384953317334));
#262957=CARTESIAN_POINT('Ctrl Pts',(-198.697386938343,3.86908831687014,
135.283517182095));
#262958=CARTESIAN_POINT('Ctrl Pts',(-198.704795158009,3.98538455885265,
135.17753343379));
#262959=CARTESIAN_POINT('Ctrl Pts',(-198.712207937311,4.10175237923126,
135.071484454256));
#262960=CARTESIAN_POINT('Ctrl Pts',(-198.719620716613,4.21378021684949,
134.960882545995));
#262961=CARTESIAN_POINT('Ctrl Pts',(-198.727033495915,4.32111212685275,
134.846132574229));
#262962=CARTESIAN_POINT('Ctrl Pts',(-198.734456866944,4.42859739772255,
134.731218642321));
#262963=CARTESIAN_POINT('Ctrl Pts',(-198.741880237973,4.53137309681198,
134.612145091307));
#262964=CARTESIAN_POINT('Ctrl Pts',(-198.749303609002,4.62912426167716,
134.489348966591));
#262965=CARTESIAN_POINT('Ctrl Pts',(-198.753239658442,4.68095427479721,
134.424239514812));
#262966=CARTESIAN_POINT('Ctrl Pts',(-198.757175707883,4.73137243893255,
134.35808399281));
#262967=CARTESIAN_POINT('Ctrl Pts',(-198.761111757324,4.78033693499349,
134.290950549066));
#262968=CARTESIAN_POINT('Ctrl Pts',(-198.76853502373,4.87268244643274,134.164338969331));
#262969=CARTESIAN_POINT('Ctrl Pts',(-198.775958290135,4.9601339859933,134.033864621697));
#262970=CARTESIAN_POINT('Ctrl Pts',(-198.783381556541,5.04235087838011,
133.899942660058));
#262971=CARTESIAN_POINT('Ctrl Pts',(-198.790796049262,5.12447059722781,
133.766178983056));
#262972=CARTESIAN_POINT('Ctrl Pts',(-198.798210541983,5.20136779059828,
133.628976117973));
#262973=CARTESIAN_POINT('Ctrl Pts',(-198.805625034704,5.27274287508696,
133.488781064463));
#262974=CARTESIAN_POINT('Ctrl Pts',(-198.813032381058,5.34404916558199,
133.348721136224));
#262975=CARTESIAN_POINT('Ctrl Pts',(-198.820439727411,5.40984377485081,
133.205675091435));
#262976=CARTESIAN_POINT('Ctrl Pts',(-198.827847073765,5.46987124432698,
133.060117504508));
#262977=CARTESIAN_POINT('Ctrl Pts',(-198.835248895441,5.52985394305153,
132.914668479921));
#262978=CARTESIAN_POINT('Ctrl Pts',(-198.842650717116,5.58407792484558,
132.766711986614));
#262979=CARTESIAN_POINT('Ctrl Pts',(-198.850052538791,5.63233443512196,
132.616745613487));
#262980=CARTESIAN_POINT('Ctrl Pts',(-198.857450453103,5.68056547116234,
132.46685840644));
#262981=CARTESIAN_POINT('Ctrl Pts',(-198.864848367414,5.7228351953659,132.314963787059));
#262982=CARTESIAN_POINT('Ctrl Pts',(-198.872246281726,5.7589836551197,132.161577557692));
#262983=CARTESIAN_POINT('Ctrl Pts',(-198.879642966638,5.79512610765524,
132.008216818333));
#262984=CARTESIAN_POINT('Ctrl Pts',(-198.88703965155,5.82514922912225,131.853365323941));
#262985=CARTESIAN_POINT('Ctrl Pts',(-198.894436336462,5.84894341995819,
131.697552328582));
#262986=CARTESIAN_POINT('Ctrl Pts',(-198.901832693398,5.87273655573477,
131.541746242135));
#262987=CARTESIAN_POINT('Ctrl Pts',(-198.909229050333,5.89030125370091,
131.384979108511));
#262988=CARTESIAN_POINT('Ctrl Pts',(-198.916625407269,5.90157940820071,
131.227788357802));
#262989=CARTESIAN_POINT('Ctrl Pts',(-198.924022896605,5.9128592894148,131.070573540788));
#262990=CARTESIAN_POINT('Ctrl Pts',(-198.931420385942,5.91785068400867,
130.912935349915));
#262991=CARTESIAN_POINT('Ctrl Pts',(-198.938817875279,5.91654754103343,
130.75541414485));
#262992=CARTESIAN_POINT('Ctrl Pts',(-198.946217957794,5.91524394124343,
130.597837720972));
#262993=CARTESIAN_POINT('Ctrl Pts',(-198.953618040309,5.90764141376477,
130.440378737603));
#262994=CARTESIAN_POINT('Ctrl Pts',(-198.961018122824,5.89378597505109,
130.283575208025));
#262995=CARTESIAN_POINT('Ctrl Pts',(-198.96842634249,5.87991530085824,130.126599256847));
#262996=CARTESIAN_POINT('Ctrl Pts',(-198.975834562157,5.85977801704612,
129.970280570899));
#262997=CARTESIAN_POINT('Ctrl Pts',(-198.983242781823,5.83347184746589,
129.815150444083));
#262998=CARTESIAN_POINT('Ctrl Pts',(-198.990655561125,5.80714948687722,
129.659924837261));
#262999=CARTESIAN_POINT('Ctrl Pts',(-198.998068340427,5.77465075171243,
129.505889611662));
#263000=CARTESIAN_POINT('Ctrl Pts',(-199.005481119729,5.73612386966094,
129.353563073315));
#263001=CARTESIAN_POINT('Ctrl Pts',(-199.012904490758,5.6975419385936,129.201018883665));
#263002=CARTESIAN_POINT('Ctrl Pts',(-199.020327861787,5.65291476358045,
129.050188614405));
#263003=CARTESIAN_POINT('Ctrl Pts',(-199.027751232816,5.60243979840348,
128.901573486076));
#263004=CARTESIAN_POINT('Ctrl Pts',(-199.031687282256,5.57567676073842,
128.82277417907));
#263005=CARTESIAN_POINT('Ctrl Pts',(-199.035623331697,5.54727049570574,
128.744597274093));
#263006=CARTESIAN_POINT('Ctrl Pts',(-199.039559381137,5.51725573431446,
128.667114790649));
#263007=CARTESIAN_POINT('Ctrl Pts',(-199.046982647543,5.46064883105527,
128.520985245009));
#263008=CARTESIAN_POINT('Ctrl Pts',(-199.054405913948,5.39814676042029,
128.376885216112));
#263009=CARTESIAN_POINT('Ctrl Pts',(-199.061829180354,5.32991465982133,
128.235325724552));
#263010=CARTESIAN_POINT('Ctrl Pts',(-199.069243673075,5.26176320389876,
128.093933544556));
#263011=CARTESIAN_POINT('Ctrl Pts',(-199.076658165796,5.18789535905273,
127.955076257988));
#263012=CARTESIAN_POINT('Ctrl Pts',(-199.084072658517,5.10852526660425,
127.819247527084));
#263013=CARTESIAN_POINT('Ctrl Pts',(-199.09148000487,5.02923167403911,127.683549713025));
#263014=CARTESIAN_POINT('Ctrl Pts',(-199.098887351224,4.94444657871635,
127.550874963544));
#263015=CARTESIAN_POINT('Ctrl Pts',(-199.106294697578,4.85443117193422,
127.421694722232));
#263016=CARTESIAN_POINT('Ctrl Pts',(-199.113696519254,4.7644829020383,127.292610828418));
#263017=CARTESIAN_POINT('Ctrl Pts',(-199.121098340929,4.66931230052762,
127.16701655816));
#263018=CARTESIAN_POINT('Ctrl Pts',(-199.128500162604,4.56922516608224,
127.045356501561));
#263019=CARTESIAN_POINT('Ctrl Pts',(-199.135898076916,4.46919086685664,
126.92376066836));
#263020=CARTESIAN_POINT('Ctrl Pts',(-199.143295991227,4.36424544012047,
126.806095200239));
#263021=CARTESIAN_POINT('Ctrl Pts',(-199.150693905538,4.25473638670253,
126.692773473631));
#263022=CARTESIAN_POINT('Ctrl Pts',(-199.158090590451,4.14524553170241,
126.579470579038));
#263023=CARTESIAN_POINT('Ctrl Pts',(-199.165487275363,4.0311928143572,126.470510261472));
#263024=CARTESIAN_POINT('Ctrl Pts',(-199.172883960275,3.91296426986117,
126.3662708049));
#263025=CARTESIAN_POINT('Ctrl Pts',(-199.18028031721,3.79474096774303,126.262035970415));
#263026=CARTESIAN_POINT('Ctrl Pts',(-199.187676674146,3.67234248664227,
126.162521827584));
#263027=CARTESIAN_POINT('Ctrl Pts',(-199.195073031081,3.5461895741899,126.068067756434));
#263028=CARTESIAN_POINT('Ctrl Pts',(-199.202470520418,3.42001734740458,
125.973599224125));
#263029=CARTESIAN_POINT('Ctrl Pts',(-199.209868009754,3.29008984357849,
125.884192529796));
#263030=CARTESIAN_POINT('Ctrl Pts',(-199.217265499091,3.15685841191773,
125.800144841882));
#263031=CARTESIAN_POINT('Ctrl Pts',(-199.224665581606,3.02358027618456,
125.716067691181));
#263032=CARTESIAN_POINT('Ctrl Pts',(-199.232065664121,2.8869962222029,125.637353486203));
#263033=CARTESIAN_POINT('Ctrl Pts',(-199.239465746636,2.74758376880045,
125.564254321323));
#263034=CARTESIAN_POINT('Ctrl Pts',(-199.246873966302,2.60801801707374,
125.491074776397));
#263035=CARTESIAN_POINT('Ctrl Pts',(-199.254282185969,2.4656179856307,125.423522775534));
#263036=CARTESIAN_POINT('Ctrl Pts',(-199.261690405635,2.32088348920477,
125.361803278223));
#263037=CARTESIAN_POINT('Ctrl Pts',(-199.269103184937,2.1760599111109,125.300045793591));
#263038=CARTESIAN_POINT('Ctrl Pts',(-199.276515964239,2.028899353128,125.24412809794));
#263039=CARTESIAN_POINT('Ctrl Pts',(-199.283928743541,1.87991800148424,
125.194205640188));
#263040=CARTESIAN_POINT('Ctrl Pts',(-199.29135211457,1.73072377829936,125.144211850888));
#263041=CARTESIAN_POINT('Ctrl Pts',(-199.298775485599,1.57970392286291,
125.100230512364));
#263042=CARTESIAN_POINT('Ctrl Pts',(-199.306198856628,1.42738685480326,
125.062366423104));
#263043=CARTESIAN_POINT('Ctrl Pts',(-199.310134906068,1.34662469051819,
125.042289974441));
#263044=CARTESIAN_POINT('Ctrl Pts',(-199.314070955509,1.26549796615698,
125.023932443002));
#263045=CARTESIAN_POINT('Ctrl Pts',(-199.31800700495,1.18408604672678,125.007303536905));
#263046=CARTESIAN_POINT('Ctrl Pts',(-199.325430271356,1.03054570746349,
124.975941938976));
#263047=CARTESIAN_POINT('Ctrl Pts',(-199.332853537761,0.875526376150656,
124.950637115694));
#263048=CARTESIAN_POINT('Ctrl Pts',(-199.340276804166,0.719547249692918,
124.931526351391));
#263049=CARTESIAN_POINT('Ctrl Pts',(-199.347691296887,0.563752477609392,
124.912438174424));
#263050=CARTESIAN_POINT('Ctrl Pts',(-199.355105789608,0.407000535315681,
124.899529529172));
#263051=CARTESIAN_POINT('Ctrl Pts',(-199.362520282329,0.24982250344574,
124.892887088972));
#263052=CARTESIAN_POINT('Ctrl Pts',(-199.369927628683,0.0927959656810105,
124.886251051005));
#263053=CARTESIAN_POINT('Ctrl Pts',(-199.377334975037,-0.0646554736133486,
124.885869210084));
#263054=CARTESIAN_POINT('Ctrl Pts',(-199.38474232139,-0.221993995317587,
124.891776645347));
#263055=CARTESIAN_POINT('Ctrl Pts',(-199.392144143066,-0.379215168016295,
124.897679674621));
#263056=CARTESIAN_POINT('Ctrl Pts',(-199.399545964741,-0.536323219385118,
124.909862626159));
#263057=CARTESIAN_POINT('Ctrl Pts',(-199.406947786417,-0.692778811524635,
124.928308534679));
#263058=CARTESIAN_POINT('Ctrl Pts',(-199.414345700728,-0.84915181197491,
124.946744705747));
#263059=CARTESIAN_POINT('Ctrl Pts',(-199.421743615039,-1.00487266934929,
124.971437205811));
#263060=CARTESIAN_POINT('Ctrl Pts',(-199.429141529351,-1.15940576566253,
125.00231711264));
#263061=CARTESIAN_POINT('Ctrl Pts',(-199.436538214263,-1.3139131813789,
125.033191887789));
#263062=CARTESIAN_POINT('Ctrl Pts',(-199.443934899175,-1.46723286208119,
125.070251955885));
#263063=CARTESIAN_POINT('Ctrl Pts',(-199.451331584087,-1.61883788530298,
125.113377006308));
#263064=CARTESIAN_POINT('Ctrl Pts',(-199.458727941023,-1.7704361861996,
125.156500144521));
#263065=CARTESIAN_POINT('Ctrl Pts',(-199.466124297958,-1.92031962173487,
125.205687628209));
#263066=CARTESIAN_POINT('Ctrl Pts',(-199.473520654893,-2.06797523750912,
125.260768913666));
#263067=CARTESIAN_POINT('Ctrl Pts',(-199.48091814423,-2.21565345973426,
125.315858632208));
#263068=CARTESIAN_POINT('Ctrl Pts',(-199.488315633567,-2.36110283327585,
125.376843818751));
#263069=CARTESIAN_POINT('Ctrl Pts',(-199.495713122903,-2.50382937664356,
125.443505367221));
#263070=CARTESIAN_POINT('Ctrl Pts',(-199.503113205418,-2.64660595258121,
125.510190283794));
#263071=CARTESIAN_POINT('Ctrl Pts',(-199.510513287933,-2.78665745995995,
125.582555366178));
#263072=CARTESIAN_POINT('Ctrl Pts',(-199.517913370448,-2.92351369405257,
125.660335127428));
#263073=CARTESIAN_POINT('Ctrl Pts',(-199.525321590115,-3.06052041564315,
125.738200415521));
#263074=CARTESIAN_POINT('Ctrl Pts',(-199.532729809781,-3.1943245224501,
125.821492088438));
#263075=CARTESIAN_POINT('Ctrl Pts',(-199.540138029447,-3.3244834141804,
125.909900423496));
#263076=CARTESIAN_POINT('Ctrl Pts',(-199.54755080875,-3.45472241653674,
125.998363172409));
#263077=CARTESIAN_POINT('Ctrl Pts',(-199.554963588052,-3.58131143374482,
126.091948637279));
#263078=CARTESIAN_POINT('Ctrl Pts',(-199.562376367354,-3.7038406709643,
126.190306559949));
#263079=CARTESIAN_POINT('Ctrl Pts',(-199.569799738382,-3.82654498370379,
126.288805021032));
#263080=CARTESIAN_POINT('Ctrl Pts',(-199.577223109411,-3.94517765014855,
126.39208931474));
#263081=CARTESIAN_POINT('Ctrl Pts',(-199.58464648044,-4.05936487664758,
126.499771512815));
#263082=CARTESIAN_POINT('Ctrl Pts',(-199.588582529881,-4.11990968402192,
126.556867198033));
#263083=CARTESIAN_POINT('Ctrl Pts',(-199.592518579321,-4.17920537128048,
126.615198714714));
#263084=CARTESIAN_POINT('Ctrl Pts',(-199.596454628762,-4.23720087198234,
126.674704538306));
#263085=CARTESIAN_POINT('Ctrl Pts',(-199.603780504856,-4.3451435842251,
126.785458302217));
#263086=CARTESIAN_POINT('Ctrl Pts',(-199.611106380951,-4.44892529945081,
126.900636519193));
#263087=CARTESIAN_POINT('Ctrl Pts',(-199.618432257045,-4.54815423714637,
127.01988924132));
#263088=CARTESIAN_POINT('Ctrl Pts',(-199.625749275158,-4.64726319356173,
127.138997770688));
#263089=CARTESIAN_POINT('Ctrl Pts',(-199.633066293272,-4.74183008260889,
127.262170710391));
#263090=CARTESIAN_POINT('Ctrl Pts',(-199.640383311386,-4.83149884976926,
127.389020308435));
#263091=CARTESIAN_POINT('Ctrl Pts',(-199.647691937754,-4.9210647775684,
127.515724425147));
#263092=CARTESIAN_POINT('Ctrl Pts',(-199.655000564122,-5.00574355056634,
127.646096491343));
#263093=CARTESIAN_POINT('Ctrl Pts',(-199.66230919049,-5.08521874467687,
127.779715038116));
#263094=CARTESIAN_POINT('Ctrl Pts',(-199.669613071836,-5.1646423406467,
127.913246834945));
#263095=CARTESIAN_POINT('Ctrl Pts',(-199.676916953183,-5.23886888252049,
128.050020591129));
#263096=CARTESIAN_POINT('Ctrl Pts',(-199.684220834529,-5.30762463042162,
128.18958503541));
#263097=CARTESIAN_POINT('Ctrl Pts',(-199.691521506071,-5.37635016253885,
128.329088145923));
#263098=CARTESIAN_POINT('Ctrl Pts',(-199.698822177613,-5.43960951509057,
128.471379160608));
#263099=CARTESIAN_POINT('Ctrl Pts',(-199.706122849155,-5.49717452749041,
128.615981588053));
#263100=CARTESIAN_POINT('Ctrl Pts',(-199.713421843476,-5.55472631518357,
128.760550795239));
#263101=CARTESIAN_POINT('Ctrl Pts',(-199.720720837798,-5.60658622516097,
128.907430001561));
#263102=CARTESIAN_POINT('Ctrl Pts',(-199.728019832119,-5.6525740654497,
129.05612236232));
#263103=CARTESIAN_POINT('Ctrl Pts',(-199.735321043721,-5.69857587587576,
129.204859892687));
#263104=CARTESIAN_POINT('Ctrl Pts',(-199.742622255322,-5.73870193341256,
129.355411312575));
#263105=CARTESIAN_POINT('Ctrl Pts',(-199.749923466924,-5.77282175169358,
129.50726401913));
#263106=CARTESIAN_POINT('Ctrl Pts',(-199.757225668922,-5.80694619826219,
129.659137324213));
#263107=CARTESIAN_POINT('Ctrl Pts',(-199.764527870919,-5.83506270707501,
129.81231189086));
#263108=CARTESIAN_POINT('Ctrl Pts',(-199.771830072916,-5.85709199383315,
129.966265194433));
#263109=CARTESIAN_POINT('Ctrl Pts',(-199.779138508574,-5.87914008630182,
130.120349923109));
#263110=CARTESIAN_POINT('Ctrl Pts',(-199.786446944231,-5.8950905299074,
130.275214335113));
#263111=CARTESIAN_POINT('Ctrl Pts',(-199.793755379889,-5.90491592475032,
130.430330559776));
#263112=CARTESIAN_POINT('Ctrl Pts',(-199.799711855857,-5.91292375720509,
130.556752424544));
#263113=CARTESIAN_POINT('Ctrl Pts',(-199.805668331824,-5.9168640205334,
130.683341391447));
#263114=CARTESIAN_POINT('Ctrl Pts',(-199.811624807792,-5.91674748832781,
130.809812394026));
#263115=CARTESIAN_POINT('',(-201.561624807792,-5.9216802870108,130.802292919862));
#263116=CARTESIAN_POINT('Ctrl Pts',(-199.811624807792,-5.91707319532089,
130.809812694137));
#263117=CARTESIAN_POINT('Ctrl Pts',(-199.832717289386,-5.92122840583984,
131.257688120002));
#263118=CARTESIAN_POINT('Ctrl Pts',(-199.946625645587,-5.66995203506684,
133.671789078785));
#263119=CARTESIAN_POINT('Ctrl Pts',(-200.153349876387,-2.35938766776408,
137.393051713948));
#263120=CARTESIAN_POINT('Ctrl Pts',(-200.431797500202,4.26794575514161,
136.350728759107));
#263121=CARTESIAN_POINT('Ctrl Pts',(-200.710245124014,6.97324552981307,
130.211564437336));
#263122=CARTESIAN_POINT('Ctrl Pts',(-200.988692747828,3.27047332456854,
124.617150845494));
#263123=CARTESIAN_POINT('Ctrl Pts',(-201.26714037164,-3.43770409444905,
124.708480772182));
#263124=CARTESIAN_POINT('Ctrl Pts',(-201.458117724962,-5.87190273225,128.613207570693));
#263125=CARTESIAN_POINT('Ctrl Pts',(-201.556279203679,-5.9261716932185,
130.689210903785));
#263126=CARTESIAN_POINT('Ctrl Pts',(-201.561624807792,-5.92566153694035,
130.802291529712));
#263127=CARTESIAN_POINT('',(-203.31162480776,-5.91674832526764,130.799908882784));
#263128=CARTESIAN_POINT('Ctrl Pts',(-201.561624807792,-5.91674963930729,
130.802294641516));
#263129=CARTESIAN_POINT('Ctrl Pts',(-201.568982881734,-5.91680390723813,
130.957712590457));
#263130=CARTESIAN_POINT('Ctrl Pts',(-201.576340955677,-5.91073031198679,
131.113380258586));
#263131=CARTESIAN_POINT('Ctrl Pts',(-201.583699029619,-5.89849601535624,
131.26876918696));
#263132=CARTESIAN_POINT('Ctrl Pts',(-201.591048671187,-5.88627573926641,
131.423980039155));
#263133=CARTESIAN_POINT('Ctrl Pts',(-201.598398312754,-5.86790884059778,
131.578912411785));
#263134=CARTESIAN_POINT('Ctrl Pts',(-201.605747954322,-5.84341445076555,
131.733036082454));
#263135=CARTESIAN_POINT('Ctrl Pts',(-201.61309084544,-5.81894255837628,
131.887018194647));
#263136=CARTESIAN_POINT('Ctrl Pts',(-201.620433736558,-5.78835443516488,
132.040192709969));
#263137=CARTESIAN_POINT('Ctrl Pts',(-201.627776627676,-5.75172113270748,
132.192032975893));
#263138=CARTESIAN_POINT('Ctrl Pts',(-201.635114444198,-5.71511314714554,
132.343768306585));
#263139=CARTESIAN_POINT('Ctrl Pts',(-201.64245226072,-5.67246838760474,
132.494170855111));
#263140=CARTESIAN_POINT('Ctrl Pts',(-201.649790077242,-5.62390921912543,
132.642722839093));
#263141=CARTESIAN_POINT('Ctrl Pts',(-201.65712519342,-5.57536792060671,
132.791220155373));
#263142=CARTESIAN_POINT('Ctrl Pts',(-201.664460309597,-5.52091665958435,
132.937867900585));
#263143=CARTESIAN_POINT('Ctrl Pts',(-201.671795425774,-5.46072800920963,
133.082162226999));
#263144=CARTESIAN_POINT('Ctrl Pts',(-201.679129259572,-5.40054988146438,
133.2264313268));
#263145=CARTESIAN_POINT('Ctrl Pts',(-201.68646309337,-5.33463650595489,
133.368347475309));
#263146=CARTESIAN_POINT('Ctrl Pts',(-201.693796927167,-5.2632089776057,
133.507425881401));
#263147=CARTESIAN_POINT('Ctrl Pts',(-201.701130988438,-5.19177923379931,
133.646508601267));
#263148=CARTESIAN_POINT('Ctrl Pts',(-201.708465049707,-5.11483517035096,
133.782753065024));
#263149=CARTESIAN_POINT('Ctrl Pts',(-201.715799110978,-5.03264419073689,
133.915698434638));
#263150=CARTESIAN_POINT('Ctrl Pts',(-201.723134909502,-4.95043374214518,
134.04867529567));
#263151=CARTESIAN_POINT('Ctrl Pts',(-201.730470708027,-4.86297410395734,
134.178351183875));
#263152=CARTESIAN_POINT('Ctrl Pts',(-201.737806506552,-4.77057626898022,
134.304293848978));
#263153=CARTESIAN_POINT('Ctrl Pts',(-201.745149895269,-4.67808283196083,
134.430366824234));
#263154=CARTESIAN_POINT('Ctrl Pts',(-201.752493283986,-4.58064121767003,
134.55269855382));
#263155=CARTESIAN_POINT('Ctrl Pts',(-201.759836672703,-4.4786034494646,
134.67088899648));
#263156=CARTESIAN_POINT('Ctrl Pts',(-201.767183945264,-4.3765117145283,
134.789141948854));
#263157=CARTESIAN_POINT('Ctrl Pts',(-201.774531217824,-4.26981924252526,
134.903248973441));
#263158=CARTESIAN_POINT('Ctrl Pts',(-201.781878490384,-4.15891476263121,
135.012847110317));
#263159=CARTESIAN_POINT('Ctrl Pts',(-201.789236993135,-4.04784076697534,
135.12261276623));
#263160=CARTESIAN_POINT('Ctrl Pts',(-201.796595495886,-3.93254218153233,
135.227855508902));
#263161=CARTESIAN_POINT('Ctrl Pts',(-201.803953998638,-3.81344138899068,
135.328252231567));
#263162=CARTESIAN_POINT('Ctrl Pts',(-201.81064787218,-3.70509792958346,
135.419580996176));
#263163=CARTESIAN_POINT('Ctrl Pts',(-201.817341745723,-3.5936086492963,
135.506900002018));
#263164=CARTESIAN_POINT('Ctrl Pts',(-201.824035619266,-3.47931103503038,
135.589998013359));
#263165=CARTESIAN_POINT('Ctrl Pts',(-201.831458885672,-3.35255906776189,
135.682150736593));
#263166=CARTESIAN_POINT('Ctrl Pts',(-201.838882152077,-3.22195178485856,
135.769403615139));
#263167=CARTESIAN_POINT('Ctrl Pts',(-201.846305418483,-3.0879048581852,
135.851416605892));
#263168=CARTESIAN_POINT('Ctrl Pts',(-201.853719911204,-2.95401636384689,
135.933332664101));
#263169=CARTESIAN_POINT('Ctrl Pts',(-201.861134403924,-2.8166966332044,
136.010020969021));
#263170=CARTESIAN_POINT('Ctrl Pts',(-201.868548896646,-2.67639312130945,
136.081182617852));
#263171=CARTESIAN_POINT('Ctrl Pts',(-201.875956242999,-2.53622483922201,
136.152275678408));
#263172=CARTESIAN_POINT('Ctrl Pts',(-201.883363589353,-2.39307883188319,
136.217852519758));
#263173=CARTESIAN_POINT('Ctrl Pts',(-201.890770935707,-2.24743006191977,
136.277658405854));
#263174=CARTESIAN_POINT('Ctrl Pts',(-201.898172757382,-2.10188992230359,
136.337419686464));
#263175=CARTESIAN_POINT('Ctrl Pts',(-201.905574579058,-1.95385108065789,
136.391418440872));
#263176=CARTESIAN_POINT('Ctrl Pts',(-201.912976400733,-1.80381144299486,
136.439446671977));
#263177=CARTESIAN_POINT('Ctrl Pts',(-201.920374315044,-1.65385101008865,
136.487449549353));
#263178=CARTESIAN_POINT('Ctrl Pts',(-201.927772229356,-1.50189223927456,
136.529488066856));
#263179=CARTESIAN_POINT('Ctrl Pts',(-201.935170143667,-1.34845117572333,
136.56540305702));
#263180=CARTESIAN_POINT('Ctrl Pts',(-201.942566828579,-1.19503561129339,
136.601312078765));
#263181=CARTESIAN_POINT('Ctrl Pts',(-201.949963513491,-1.04013860613695,
136.631099507851));
#263182=CARTESIAN_POINT('Ctrl Pts',(-201.957360198404,-0.884289580498989,
136.654656550279));
#263183=CARTESIAN_POINT('Ctrl Pts',(-201.964756555339,-0.728447465370143,
136.678212548163));
#263184=CARTESIAN_POINT('Ctrl Pts',(-201.972152912275,-0.571653782799518,
136.695538652899));
#263185=CARTESIAN_POINT('Ctrl Pts',(-201.97954926921,-0.414446050683824,
136.706577576775));
#263186=CARTESIAN_POINT('Ctrl Pts',(-201.986946758547,-0.25721424966346,
136.717618190738));
#263187=CARTESIAN_POINT('Ctrl Pts',(-201.994344247883,-0.0995686452809479,
136.722369681061));
#263188=CARTESIAN_POINT('Ctrl Pts',(-202.00174173722,0.0579503942137365,
136.720826819135));
#263189=CARTESIAN_POINT('Ctrl Pts',(-202.009141819735,0.215524651763755,
136.719283416362));
#263190=CARTESIAN_POINT('Ctrl Pts',(-202.016541902249,0.372971883044187,
136.711441271919));
#263191=CARTESIAN_POINT('Ctrl Pts',(-202.023941984764,0.529754145426437,
136.69734722097));
#263192=CARTESIAN_POINT('Ctrl Pts',(-202.031350204431,0.686708806024008,
136.683237672164));
#263193=CARTESIAN_POINT('Ctrl Pts',(-202.038758424097,0.842996665438895,
136.662862521241));
#263194=CARTESIAN_POINT('Ctrl Pts',(-202.046166643764,0.998086579105648,
136.636320300478));
#263195=CARTESIAN_POINT('Ctrl Pts',(-202.053579423066,1.15327194802645,
136.609761743421));
#263196=CARTESIAN_POINT('Ctrl Pts',(-202.060992202368,1.30725753771265,
136.577028630497));
#263197=CARTESIAN_POINT('Ctrl Pts',(-202.06840498167,1.45952526831276,136.538269977999));
#263198=CARTESIAN_POINT('Ctrl Pts',(-202.075828352699,1.61201056618677,
136.49945594532));
#263199=CARTESIAN_POINT('Ctrl Pts',(-202.083251723727,1.76277274582379,
136.454599283991));
#263200=CARTESIAN_POINT('Ctrl Pts',(-202.090675094756,1.91131088775466,
136.403898210337));
#263201=CARTESIAN_POINT('Ctrl Pts',(-202.094611144197,1.99006937472724,
136.377015284531));
#263202=CARTESIAN_POINT('Ctrl Pts',(-202.098547193638,2.06820295967937,
136.34849008045));
#263203=CARTESIAN_POINT('Ctrl Pts',(-202.102483243078,2.14563967604513,
136.318357438664));
#263204=CARTESIAN_POINT('Ctrl Pts',(-202.109906509484,2.29168290639948,
136.261528216662));
#263205=CARTESIAN_POINT('Ctrl Pts',(-202.117329775889,2.43568765092004,
136.198806922689));
#263206=CARTESIAN_POINT('Ctrl Pts',(-202.124753042294,2.5771431409141,136.130359471653));
#263207=CARTESIAN_POINT('Ctrl Pts',(-202.132167535015,2.71843144226654,
136.06199291982));
#263208=CARTESIAN_POINT('Ctrl Pts',(-202.139582027737,2.85717615375475,
135.987913843359));
#263209=CARTESIAN_POINT('Ctrl Pts',(-202.146996520458,2.99288393960237,
135.908337134613));
#263210=CARTESIAN_POINT('Ctrl Pts',(-202.154403866811,3.12846092517669,
135.828837124895));
#263211=CARTESIAN_POINT('Ctrl Pts',(-202.161811213165,3.26100649253989,
135.743850219369));
#263212=CARTESIAN_POINT('Ctrl Pts',(-202.169218559519,3.39004959613795,
135.653638326486));
#263213=CARTESIAN_POINT('Ctrl Pts',(-202.176620381194,3.51899645452082,
135.563493717036));
#263214=CARTESIAN_POINT('Ctrl Pts',(-202.18402220287,3.64444574588738,135.468132092632));
#263215=CARTESIAN_POINT('Ctrl Pts',(-202.191424024545,3.76595334602514,
135.36785992819));
#263216=CARTESIAN_POINT('Ctrl Pts',(-202.198821938857,3.88739680324591,
135.267640696643));
#263217=CARTESIAN_POINT('Ctrl Pts',(-202.206219853168,4.00490242603697,
135.16251632462));
#263218=CARTESIAN_POINT('Ctrl Pts',(-202.213617767479,4.11805736728282,
135.052834941634));
#263219=CARTESIAN_POINT('Ctrl Pts',(-202.221014452392,4.23119350423076,
134.943171785704));
#263220=CARTESIAN_POINT('Ctrl Pts',(-202.228411137304,4.33998012680202,
134.828953381375));
#263221=CARTESIAN_POINT('Ctrl Pts',(-202.235807822216,4.44403953894811,
134.710566339077));
#263222=CARTESIAN_POINT('Ctrl Pts',(-202.243204179152,4.54809433699053,
134.592184546185));
#263223=CARTESIAN_POINT('Ctrl Pts',(-202.250600536087,4.64742209493324,
134.469634763234));
#263224=CARTESIAN_POINT('Ctrl Pts',(-202.257996893022,4.74168407344933,
134.343338253847));
#263225=CARTESIAN_POINT('Ctrl Pts',(-202.265394382359,4.83596048371523,
134.217022408141));
#263226=CARTESIAN_POINT('Ctrl Pts',(-202.272791871696,4.92516934696955,
134.086958992999));
#263227=CARTESIAN_POINT('Ctrl Pts',(-202.280189361032,5.00901418199923,
133.953599809344));
#263228=CARTESIAN_POINT('Ctrl Pts',(-202.287589443547,5.09288840870597,
133.820193876833));
#263229=CARTESIAN_POINT('Ctrl Pts',(-202.294989526062,5.17139466485451,
133.683490191393));
#263230=CARTESIAN_POINT('Ctrl Pts',(-202.302389608577,5.24428158306487,
133.543966654942));
#263231=CARTESIAN_POINT('Ctrl Pts',(-202.309797828244,5.31724864793465,
133.40428969802));
#263232=CARTESIAN_POINT('Ctrl Pts',(-202.31720604791,5.3845838619657,133.261787028827));
#263233=CARTESIAN_POINT('Ctrl Pts',(-202.324614267577,5.44608302654156,
133.116958773432));
#263234=CARTESIAN_POINT('Ctrl Pts',(-202.332027046879,5.50762004282705,
132.972041378663));
#263235=CARTESIAN_POINT('Ctrl Pts',(-202.339439826181,5.56331372040708,
132.824795893876));
#263236=CARTESIAN_POINT('Ctrl Pts',(-202.346852605483,5.61300939609337,
132.675738741267));
#263237=CARTESIAN_POINT('Ctrl Pts',(-202.354275976512,5.66277607929151,
132.526468608809));
#263238=CARTESIAN_POINT('Ctrl Pts',(-202.361699347541,5.70652754037334,
132.375381996141));
#263239=CARTESIAN_POINT('Ctrl Pts',(-202.36912271857,5.74415978513868,132.223007481763));
#263240=CARTESIAN_POINT('Ctrl Pts',(-202.37305876801,5.76411330428583,132.142214858066));
#263241=CARTESIAN_POINT('Ctrl Pts',(-202.376994817451,5.78234735340238,
132.061060290616));
#263242=CARTESIAN_POINT('Ctrl Pts',(-202.380930866892,5.79885234516005,
131.9796231591));
#263243=CARTESIAN_POINT('Ctrl Pts',(-202.388354133297,5.82998024451299,
131.82603527062));
#263244=CARTESIAN_POINT('Ctrl Pts',(-202.395777399702,5.85504912545923,
131.670977609184));
#263245=CARTESIAN_POINT('Ctrl Pts',(-202.403200666108,5.87392249395432,
131.514969580018));
#263246=CARTESIAN_POINT('Ctrl Pts',(-202.410615158829,5.89277355569518,
131.359145939387));
#263247=CARTESIAN_POINT('Ctrl Pts',(-202.41802965155,5.90544363622744,131.202374533849));
#263248=CARTESIAN_POINT('Ctrl Pts',(-202.425444144271,5.91184687052777,
131.045186575326));
#263249=CARTESIAN_POINT('Ctrl Pts',(-202.432851490625,5.91824393314985,
130.888150120474));
#263250=CARTESIAN_POINT('Ctrl Pts',(-202.440258836978,5.91838615934132,
130.730698282408));
#263251=CARTESIAN_POINT('Ctrl Pts',(-202.447666183332,5.91223928847316,
130.573368933009));
#263252=CARTESIAN_POINT('Ctrl Pts',(-202.455068005008,5.90609700217325,
130.416156925776));
#263253=CARTESIAN_POINT('Ctrl Pts',(-202.462469826683,5.8936749730336,130.259067596714));
#263254=CARTESIAN_POINT('Ctrl Pts',(-202.469871648358,5.87499098709605,
130.10264025728));
#263255=CARTESIAN_POINT('Ctrl Pts',(-202.47726956267,5.85631686428913,129.94629549462));
#263256=CARTESIAN_POINT('Ctrl Pts',(-202.484667476981,5.83138741218186,
129.790612395348));
#263257=CARTESIAN_POINT('Ctrl Pts',(-202.492065391293,5.80027236804441,
129.636126471943));
#263258=CARTESIAN_POINT('Ctrl Pts',(-202.499462076205,5.76916249466294,
129.481666221295));
#263259=CARTESIAN_POINT('Ctrl Pts',(-202.506858761117,5.73186914302823,
129.328403117249));
#263260=CARTESIAN_POINT('Ctrl Pts',(-202.514255446029,5.68851342550535,
129.176863898569));
#263261=CARTESIAN_POINT('Ctrl Pts',(-202.521651802964,5.64515963042055,
129.025331399297));
#263262=CARTESIAN_POINT('Ctrl Pts',(-202.5290481599,5.59574410661747,128.875522992302));
#263263=CARTESIAN_POINT('Ctrl Pts',(-202.536444516835,5.54043817823208,
128.727951371852));
#263264=CARTESIAN_POINT('Ctrl Pts',(-202.543842006172,5.48512378236803,
128.580357157809));
#263265=CARTESIAN_POINT('Ctrl Pts',(-202.551239495508,5.42391731725896,
128.435000761769));
#263266=CARTESIAN_POINT('Ctrl Pts',(-202.558636984845,5.35703864047963,
128.292375831205));
#263267=CARTESIAN_POINT('Ctrl Pts',(-202.56603706736,5.29013651948354,128.149700903693));
#263268=CARTESIAN_POINT('Ctrl Pts',(-202.573437149875,5.21755838634373,
128.009759685829));
#263269=CARTESIAN_POINT('Ctrl Pts',(-202.58083723239,5.13957044327107,127.873021977771));
#263270=CARTESIAN_POINT('Ctrl Pts',(-202.588245452056,5.06149674443775,
127.736133912546));
#263271=CARTESIAN_POINT('Ctrl Pts',(-202.595653671723,4.9780015408993,127.60245671643));
#263272=CARTESIAN_POINT('Ctrl Pts',(-202.603061891389,4.8893952285411,127.472432517859));
#263273=CARTESIAN_POINT('Ctrl Pts',(-202.610474670691,4.80073438047586,
127.342328291562));
#263274=CARTESIAN_POINT('Ctrl Pts',(-202.617887449993,4.70695637704169,
127.215881842089));
#263275=CARTESIAN_POINT('Ctrl Pts',(-202.625300229295,4.60841209962781,
127.093502430771));
#263276=CARTESIAN_POINT('Ctrl Pts',(-202.632723600324,4.50972701752896,
126.970948158011));
#263277=CARTESIAN_POINT('Ctrl Pts',(-202.640146971353,4.40626230469941,
126.852472810054));
#263278=CARTESIAN_POINT('Ctrl Pts',(-202.647570342382,4.29840645779756,
126.738449589756));
#263279=CARTESIAN_POINT('Ctrl Pts',(-202.651506391822,4.24121869980284,
126.677991742403));
#263280=CARTESIAN_POINT('Ctrl Pts',(-202.655442441263,4.18279701272454,
126.618784894444));
#263281=CARTESIAN_POINT('Ctrl Pts',(-202.659378490704,4.12320299875834,
126.560880018632));
#263282=CARTESIAN_POINT('Ctrl Pts',(-202.66680175711,4.01081054828672,126.451673230002));
#263283=CARTESIAN_POINT('Ctrl Pts',(-202.674225023515,3.89390648875168,
126.346769616974));
#263284=CARTESIAN_POINT('Ctrl Pts',(-202.681648289921,3.77285403211578,
126.246564767065));
#263285=CARTESIAN_POINT('Ctrl Pts',(-202.689062782642,3.65194464943049,
126.146478350966));
#263286=CARTESIAN_POINT('Ctrl Pts',(-202.696477275363,3.52689691396513,
126.051079879331));
#263287=CARTESIAN_POINT('Ctrl Pts',(-202.703891768084,3.39811133721108,
125.960728725853));
#263288=CARTESIAN_POINT('Ctrl Pts',(-202.711299114438,3.2694498888457,125.87046465622));
#263289=CARTESIAN_POINT('Ctrl Pts',(-202.718706460791,3.13705807494424,
125.785238432848));
#263290=CARTESIAN_POINT('Ctrl Pts',(-202.726113807145,3.00136990364706,
125.705369613065));
#263291=CARTESIAN_POINT('Ctrl Pts',(-202.733515628821,2.86578293370648,
125.625560362461));
#263292=CARTESIAN_POINT('Ctrl Pts',(-202.740917450496,2.7269048219899,125.551100747908));
#263293=CARTESIAN_POINT('Ctrl Pts',(-202.748319272171,2.5851989202899,125.482267316521));
#263294=CARTESIAN_POINT('Ctrl Pts',(-202.755717186483,2.44356782403319,
125.413470221767));
#263295=CARTESIAN_POINT('Ctrl Pts',(-202.763115100794,2.29911224564274,
125.350293557936));
#263296=CARTESIAN_POINT('Ctrl Pts',(-202.770513015105,2.15232042163001,
125.292968110664));
#263297=CARTESIAN_POINT('Ctrl Pts',(-202.777909700018,2.00555299175515,
125.235652189841));
#263298=CARTESIAN_POINT('Ctrl Pts',(-202.78530638493,1.85645043418548,125.184185691378));
#263299=CARTESIAN_POINT('Ctrl Pts',(-202.792703069842,1.70552137335281,
125.13875143518));
#263300=CARTESIAN_POINT('Ctrl Pts',(-202.800099426778,1.55459900487243,
125.093319193584));
#263301=CARTESIAN_POINT('Ctrl Pts',(-202.807495783713,1.40185065161534,
125.053918770026));
#263302=CARTESIAN_POINT('Ctrl Pts',(-202.814892140649,1.2478002626691,125.020683148431));
#263303=CARTESIAN_POINT('Ctrl Pts',(-202.822289629985,1.09372628821504,
124.987442438377));
#263304=CARTESIAN_POINT('Ctrl Pts',(-202.829687119322,0.938350246075035,
124.960368488343));
#263305=CARTESIAN_POINT('Ctrl Pts',(-202.837084608658,0.782206294241051,
124.939543154443));
#263306=CARTESIAN_POINT('Ctrl Pts',(-202.844484691173,0.626007606387029,
124.918710520255));
#263307=CARTESIAN_POINT('Ctrl Pts',(-202.851884773688,0.469040842675188,
124.904130912675));
#263308=CARTESIAN_POINT('Ctrl Pts',(-202.859284856203,0.311845148080142,
124.895834306707));
#263309=CARTESIAN_POINT('Ctrl Pts',(-202.86669307587,0.154476600659004,
124.887528577766));
#263310=CARTESIAN_POINT('Ctrl Pts',(-202.874101295536,-0.00312100736494086,
124.885519667463));
#263311=CARTESIAN_POINT('Ctrl Pts',(-202.881509515203,-0.160407924259452,
124.889785412166));
#263312=CARTESIAN_POINT('Ctrl Pts',(-202.888922294505,-0.317791648627735,
124.894053782363));
#263313=CARTESIAN_POINT('Ctrl Pts',(-202.896335073807,-0.474863929231365,
124.904604478017));
#263314=CARTESIAN_POINT('Ctrl Pts',(-202.903747853109,-0.631090782958744,
124.921363508425));
#263315=CARTESIAN_POINT('Ctrl Pts',(-202.911171224138,-0.787540860940819,
124.938146484921));
#263316=CARTESIAN_POINT('Ctrl Pts',(-202.918594595167,-0.943142731124381,
124.961155458605));
#263317=CARTESIAN_POINT('Ctrl Pts',(-202.926017966195,-1.09737241544244,
124.990265301498));
#263318=CARTESIAN_POINT('Ctrl Pts',(-202.929954015636,-1.17914869475504,
125.00570003868));
#263319=CARTESIAN_POINT('Ctrl Pts',(-202.933890065077,-1.260539441657,125.022849111077));
#263320=CARTESIAN_POINT('Ctrl Pts',(-202.937826114517,-1.34146847383707,
125.041688243033));
#263321=CARTESIAN_POINT('Ctrl Pts',(-202.945249380923,-1.49409810282559,
125.077218257956));
#263322=CARTESIAN_POINT('Ctrl Pts',(-202.952672647328,-1.64554598320926,
125.118869988883));
#263323=CARTESIAN_POINT('Ctrl Pts',(-202.960095913734,-1.79528297106824,
125.166551680018));
#263324=CARTESIAN_POINT('Ctrl Pts',(-202.967510406455,-1.94484298224202,
125.214177015355));
#263325=CARTESIAN_POINT('Ctrl Pts',(-202.974924899176,-2.0926957737322,
125.267818012581));
#263326=CARTESIAN_POINT('Ctrl Pts',(-202.982339391897,-2.23832250802715,
125.327331960296));
#263327=CARTESIAN_POINT('Ctrl Pts',(-202.98974673825,-2.38380888179367,
125.386788546228));
#263328=CARTESIAN_POINT('Ctrl Pts',(-202.997154084604,-2.52707312651263,
125.452106673295));
#263329=CARTESIAN_POINT('Ctrl Pts',(-203.004561430958,-2.66761179755283,
125.523093926699));
#263330=CARTESIAN_POINT('Ctrl Pts',(-203.011963252633,-2.80804564954954,
125.594028235132));
#263331=CARTESIAN_POINT('Ctrl Pts',(-203.019365074309,-2.94575764374757,
125.670623083307));
#263332=CARTESIAN_POINT('Ctrl Pts',(-203.026766895984,-3.08026466026495,
125.752638120712));
#263333=CARTESIAN_POINT('Ctrl Pts',(-203.034164810295,-3.21470067157453,
125.834609863016));
#263334=CARTESIAN_POINT('Ctrl Pts',(-203.041562724607,-3.34593475675407,
125.921995902334));
#263335=CARTESIAN_POINT('Ctrl Pts',(-203.048960638918,-3.47350884555318,
126.014510216733));
#263336=CARTESIAN_POINT('Ctrl Pts',(-203.05635732383,-3.60106173385371,
126.107009156931));
#263337=CARTESIAN_POINT('Ctrl Pts',(-203.063754008742,-3.72495553101644,
126.20463446186));
#263338=CARTESIAN_POINT('Ctrl Pts',(-203.071150693655,-3.84476150154799,
126.307057030002));
#263339=CARTESIAN_POINT('Ctrl Pts',(-203.07854705059,-3.96456215975726,
126.409475056621));
#263340=CARTESIAN_POINT('Ctrl Pts',(-203.085943407525,-4.08027506799617,
126.516689680931));
#263341=CARTESIAN_POINT('Ctrl Pts',(-203.093339764461,-4.19150513584072,
126.628331970787));
#263342=CARTESIAN_POINT('Ctrl Pts',(-203.100737253797,-4.3027522332923,
126.739991353362));
#263343=CARTESIAN_POINT('Ctrl Pts',(-203.108134743134,-4.40951486027692,
126.85607948678));
#263344=CARTESIAN_POINT('Ctrl Pts',(-203.11553223247,-4.51143542348493,
126.976191214023));
#263345=CARTESIAN_POINT('Ctrl Pts',(-203.122932314985,-4.61339171478823,
127.096345046245));
#263346=CARTESIAN_POINT('Ctrl Pts',(-203.1303323975,-4.71050232147278,127.220524996061));
#263347=CARTESIAN_POINT('Ctrl Pts',(-203.137732480015,-4.80245060369318,
127.348293667753));
#263348=CARTESIAN_POINT('Ctrl Pts',(-203.145140699682,-4.89449999250279,
127.476202834236));
#263349=CARTESIAN_POINT('Ctrl Pts',(-203.152548919348,-4.98137550230915,
127.607708300172));
#263350=CARTESIAN_POINT('Ctrl Pts',(-203.159957139014,-5.06280403100677,
127.74234397716));
#263351=CARTESIAN_POINT('Ctrl Pts',(-203.167369918316,-5.14428267760486,
127.87706252016));
#263352=CARTESIAN_POINT('Ctrl Pts',(-203.174782697619,-5.22030748290961,
128.014914787064));
#263353=CARTESIAN_POINT('Ctrl Pts',(-203.182195476921,-5.29065206648016,
128.155411528975));
#263354=CARTESIAN_POINT('Ctrl Pts',(-203.189618847949,-5.36109716169105,
128.296109019219));
#263355=CARTESIAN_POINT('Ctrl Pts',(-203.197042218978,-5.42584567210385,
128.43945819178));
#263356=CARTESIAN_POINT('Ctrl Pts',(-203.204465590007,-5.48471964848875,
128.584950574338));
#263357=CARTESIAN_POINT('Ctrl Pts',(-203.208401639448,-5.51593604343254,
128.662094126619));
#263358=CARTESIAN_POINT('Ctrl Pts',(-203.212337688889,-5.54550172992229,
128.739839959623));
#263359=CARTESIAN_POINT('Ctrl Pts',(-203.21627373833,-5.5733959533535,128.818110857429));
#263360=CARTESIAN_POINT('Ctrl Pts',(-203.224921721089,-5.63468297906373,
128.990081607504));
#263361=CARTESIAN_POINT('Ctrl Pts',(-203.233569703848,-5.68805083248295,
129.165014549172));
#263362=CARTESIAN_POINT('Ctrl Pts',(-203.242217686606,-5.73324512702968,
129.342228313056));
#263363=CARTESIAN_POINT('Ctrl Pts',(-203.250830811819,-5.77825725629626,
129.518727778925));
#263364=CARTESIAN_POINT('Ctrl Pts',(-203.259443937031,-5.81516149890193,
129.697489615715));
#263365=CARTESIAN_POINT('Ctrl Pts',(-203.268057062243,-5.84375315109936,
129.877818836794));
#263366=CARTESIAN_POINT('Ctrl Pts',(-203.276602616523,-5.87212049858119,
130.056733354925));
#263367=CARTESIAN_POINT('Ctrl Pts',(-203.285148170803,-5.89230509977486,
130.237190643914));
#263368=CARTESIAN_POINT('Ctrl Pts',(-203.293693725083,-5.90415413278233,
130.418492066309));
#263369=CARTESIAN_POINT('Ctrl Pts',(-203.299670752642,-5.91244171653796,
130.545299943557));
#263370=CARTESIAN_POINT('Ctrl Pts',(-203.305647780201,-5.91665247871619,
130.672520358863));
#263371=CARTESIAN_POINT('Ctrl Pts',(-203.31162480776,-5.91674832526764,
130.799908882784));
#263372=CARTESIAN_POINT('',(-205.061626015508,-5.91263662896126,130.80817859488));
#263373=CARTESIAN_POINT('Ctrl Pts',(-203.311624807792,-5.91674832526815,
130.799908883463));
#263374=CARTESIAN_POINT('Ctrl Pts',(-203.31925383089,-5.91687066290775,
130.962506425771));
#263375=CARTESIAN_POINT('Ctrl Pts',(-203.326882853988,-5.91028565918037,
131.125172439786));
#263376=CARTESIAN_POINT('Ctrl Pts',(-203.334511877086,-5.8970065749038,
131.287314050147));
#263377=CARTESIAN_POINT('Ctrl Pts',(-203.341914747701,-5.88412113183752,
131.444649183011));
#263378=CARTESIAN_POINT('Ctrl Pts',(-203.349317618315,-5.86493289222459,
131.601490170919));
#263379=CARTESIAN_POINT('Ctrl Pts',(-203.35672048893,-5.83950678773434,
131.757298725999));
#263380=CARTESIAN_POINT('Ctrl Pts',(-203.364124032299,-5.81407837258119,
131.913121440585));
#263381=CARTESIAN_POINT('Ctrl Pts',(-203.371527575669,-5.78241102307281,
132.067911168375));
#263382=CARTESIAN_POINT('Ctrl Pts',(-203.378931119038,-5.7446210682295,
132.22113842123));
#263383=CARTESIAN_POINT('Ctrl Pts',(-203.386336782644,-5.70682029105092,
132.374409555499));
#263384=CARTESIAN_POINT('Ctrl Pts',(-203.39374244625,-5.66289350593888,
132.526116962837));
#263385=CARTESIAN_POINT('Ctrl Pts',(-203.401148109856,-5.61300728187641,
132.675745082635));
#263386=CARTESIAN_POINT('Ctrl Pts',(-203.40894588088,-5.56047973361094,
132.833295557386));
#263387=CARTESIAN_POINT('Ctrl Pts',(-203.416743651903,-5.5013446649065,
132.988540125356));
#263388=CARTESIAN_POINT('Ctrl Pts',(-203.424541422927,-5.43585428549973,
133.1409005272));
#263389=CARTESIAN_POINT('Ctrl Pts',(-203.431959917198,-5.37354930079099,
133.285850252536));
#263390=CARTESIAN_POINT('Ctrl Pts',(-203.439378411468,-5.305492808283,133.428189425049));
#263391=CARTESIAN_POINT('Ctrl Pts',(-203.446796905739,-5.23194910023918,
133.567445700405));
#263392=CARTESIAN_POINT('Ctrl Pts',(-203.454220864128,-5.15835122331424,
133.706804545468));
#263393=CARTESIAN_POINT('Ctrl Pts',(-203.461644822517,-5.07925826396159,
133.84307564888));
#263394=CARTESIAN_POINT('Ctrl Pts',(-203.469068780906,-4.99497801599823,
133.975815359825));
#263395=CARTESIAN_POINT('Ctrl Pts',(-203.47650313371,-4.91057976578007,
134.108740921968));
#263396=CARTESIAN_POINT('Ctrl Pts',(-203.483937486513,-4.82097993977899,
134.238124918073));
#263397=CARTESIAN_POINT('Ctrl Pts',(-203.491371839317,-4.72652713722884,
134.363556001854));
#263398=CARTESIAN_POINT('Ctrl Pts',(-203.492488346925,-4.71234200565376,
134.382393520477));
#263399=CARTESIAN_POINT('Ctrl Pts',(-203.493604854534,-4.69804748499611,
134.401141949454));
#263400=CARTESIAN_POINT('Ctrl Pts',(-203.494721362142,-4.68364482727004,
134.419799967699));
#263401=CARTESIAN_POINT('Ctrl Pts',(-203.502144628548,-4.58788662156608,
134.543850568851));
#263402=CARTESIAN_POINT('Ctrl Pts',(-203.509567894953,-4.48705182451503,
134.664281756115));
#263403=CARTESIAN_POINT('Ctrl Pts',(-203.516991161359,-4.38144383707481,
134.78065040392));
#263404=CARTESIAN_POINT('Ctrl Pts',(-203.52440565408,-4.27596066950554,
134.896881513646));
#263405=CARTESIAN_POINT('Ctrl Pts',(-203.531820146801,-4.16571578943428,
135.009059367759));
#263406=CARTESIAN_POINT('Ctrl Pts',(-203.539234639522,-4.05105465877887,
135.116771395088));
#263407=CARTESIAN_POINT('Ctrl Pts',(-203.546641985876,-3.93650404283811,
135.22437960551));
#263408=CARTESIAN_POINT('Ctrl Pts',(-203.55404933223,-3.81754592051431,
135.327530304353));
#263409=CARTESIAN_POINT('Ctrl Pts',(-203.561456678584,-3.69456456150438,
135.425845580581));
#263410=CARTESIAN_POINT('Ctrl Pts',(-203.568858500259,-3.57167492663218,
135.524087529567));
#263411=CARTESIAN_POINT('Ctrl Pts',(-203.576260321934,-3.44476832015857,
135.617501004755));
#263412=CARTESIAN_POINT('Ctrl Pts',(-203.58366214361,-3.31426416180886,
135.705746506093));
#263413=CARTESIAN_POINT('Ctrl Pts',(-203.591060057921,-3.18382889558812,
135.793945423318));
#263414=CARTESIAN_POINT('Ctrl Pts',(-203.598457972233,-3.04980016813304,
135.876981591329));
#263415=CARTESIAN_POINT('Ctrl Pts',(-203.605855886544,-2.91262852580243,
135.954557277227));
#263416=CARTESIAN_POINT('Ctrl Pts',(-203.613252571456,-2.77547967891002,
136.032120071453));
#263417=CARTESIAN_POINT('Ctrl Pts',(-203.620649256369,-2.63518927836053,
136.104224000971));
#263418=CARTESIAN_POINT('Ctrl Pts',(-203.628045941281,-2.49223485864503,
136.170615920089));
#263419=CARTESIAN_POINT('Ctrl Pts',(-203.635442298216,-2.3492867776783,
136.23700489532));
#263420=CARTESIAN_POINT('Ctrl Pts',(-203.642838655152,-2.20367525098471,
136.297682206512));
#263421=CARTESIAN_POINT('Ctrl Pts',(-203.650235012087,-2.05590005455707,
136.352441865004));
#263422=CARTESIAN_POINT('Ctrl Pts',(-203.657632501424,-1.90810223337002,
136.40720990734));
#263423=CARTESIAN_POINT('Ctrl Pts',(-203.665029990761,-1.75814043291998,
136.456058363276));
#263424=CARTESIAN_POINT('Ctrl Pts',(-203.672427480097,-1.60653179003577,
136.498830405887));
#263425=CARTESIAN_POINT('Ctrl Pts',(-203.679827562612,-1.45487000097703,
136.541617442172));
#263426=CARTESIAN_POINT('Ctrl Pts',(-203.687227645127,-1.30156057913766,
136.578323722869));
#263427=CARTESIAN_POINT('Ctrl Pts',(-203.694627727642,-1.14713296000083,
136.60884306948));
#263428=CARTESIAN_POINT('Ctrl Pts',(-203.702035947309,-0.992535531820553,
136.63939597525));
#263429=CARTESIAN_POINT('Ctrl Pts',(-203.709444166976,-0.836817817244495,
136.663748288138));
#263430=CARTESIAN_POINT('Ctrl Pts',(-203.716852386642,-0.680517251053971,
136.681845354553));
#263431=CARTESIAN_POINT('Ctrl Pts',(-203.724265165944,-0.524120484472526,
136.699953559411));
#263432=CARTESIAN_POINT('Ctrl Pts',(-203.731677945247,-0.367140522827894,
136.711798818167));
#263433=CARTESIAN_POINT('Ctrl Pts',(-203.739090724549,-0.210116445125973,
136.717378598427));
#263434=CARTESIAN_POINT('Ctrl Pts',(-203.746514095577,-0.0528680040588055,
136.722966351339));
#263435=CARTESIAN_POINT('Ctrl Pts',(-203.753937466606,0.104424306655523,
136.722270747431));
#263436=CARTESIAN_POINT('Ctrl Pts',(-203.761360837635,0.261224055224296,
136.715341293856));
#263437=CARTESIAN_POINT('Ctrl Pts',(-203.765296887076,0.344363044267299,
136.711667131301));
#263438=CARTESIAN_POINT('Ctrl Pts',(-203.769232936516,0.427363673358813,
136.706241273284));
#263439=CARTESIAN_POINT('Ctrl Pts',(-203.773168985957,0.510147086307701,
136.699076939225));
#263440=CARTESIAN_POINT('Ctrl Pts',(-203.780592252362,0.666274019559398,
136.68556522878));
#263441=CARTESIAN_POINT('Ctrl Pts',(-203.788015518767,0.822099859025682,
136.665826056643));
#263442=CARTESIAN_POINT('Ctrl Pts',(-203.795438785173,0.977087794984135,
136.639875162436));
#263443=CARTESIAN_POINT('Ctrl Pts',(-203.802853277894,1.13189254807323,
136.613954940032));
#263444=CARTESIAN_POINT('Ctrl Pts',(-203.810267770615,1.28586100433918,
136.581837670375));
#263445=CARTESIAN_POINT('Ctrl Pts',(-203.817682263336,1.43845932536675,
136.543590995567));
#263446=CARTESIAN_POINT('Ctrl Pts',(-203.82508960969,1.59091056638773,136.505381184343));
#263447=CARTESIAN_POINT('Ctrl Pts',(-203.832496956044,1.74199394153385,
136.461053819284));
#263448=CARTESIAN_POINT('Ctrl Pts',(-203.839904302397,1.8911837963895,136.410727927222));
#263449=CARTESIAN_POINT('Ctrl Pts',(-203.847306124073,2.04026237982279,
136.360439570108));
#263450=CARTESIAN_POINT('Ctrl Pts',(-203.854707945748,2.18744990277064,
136.30416171299));
#263451=CARTESIAN_POINT('Ctrl Pts',(-203.862109767424,2.33223402761866,
136.24206371749));
#263452=CARTESIAN_POINT('Ctrl Pts',(-203.869507681735,2.47694172205335,
136.179998503038));
#263453=CARTESIAN_POINT('Ctrl Pts',(-203.876905596046,2.61924820292951,
136.112119415821));
#263454=CARTESIAN_POINT('Ctrl Pts',(-203.884303510358,2.7586594478157,136.038644581345));
#263455=CARTESIAN_POINT('Ctrl Pts',(-203.89170019527,2.89804752508276,135.965181957054));
#263456=CARTESIAN_POINT('Ctrl Pts',(-203.899096880182,3.03454099135519,
135.886125604982));
#263457=CARTESIAN_POINT('Ctrl Pts',(-203.906493565094,3.16766874893783,
135.801740456992));
#263458=CARTESIAN_POINT('Ctrl Pts',(-203.91388992203,3.30079060349657,135.717359050728));
#263459=CARTESIAN_POINT('Ctrl Pts',(-203.921286278965,3.43054673081018,
135.627649518213));
#263460=CARTESIAN_POINT('Ctrl Pts',(-203.928682635901,3.55649368565297,
135.532920993242));
#263461=CARTESIAN_POINT('Ctrl Pts',(-203.936080125237,3.68245992329573,
135.438177965092));
#263462=CARTESIAN_POINT('Ctrl Pts',(-203.943477614574,3.80461552889866,
135.338414638858));
#263463=CARTESIAN_POINT('Ctrl Pts',(-203.95087510391,3.92254903444112,135.233981327616));
#263464=CARTESIAN_POINT('Ctrl Pts',(-203.958275186425,4.04052388139095,
135.12951140744));
#263465=CARTESIAN_POINT('Ctrl Pts',(-203.96567526894,4.15427340221235,135.020368490215));
#263466=CARTESIAN_POINT('Ctrl Pts',(-203.973075351455,4.26342209311666,
134.906940612938));
#263467=CARTESIAN_POINT('Ctrl Pts',(-203.980483571122,4.37269080422754,
134.793388010048));
#263468=CARTESIAN_POINT('Ctrl Pts',(-203.987891790788,4.47734832309786,
134.675541306575));
#263469=CARTESIAN_POINT('Ctrl Pts',(-203.995300010455,4.57705817148828,
134.55382312002));
#263470=CARTESIAN_POINT('Ctrl Pts',(-204.002712789757,4.6768293896272,134.432030017952));
#263471=CARTESIAN_POINT('Ctrl Pts',(-204.010125569059,4.77164664501153,
134.306360982011));
#263472=CARTESIAN_POINT('Ctrl Pts',(-204.017538348361,4.8612164216961,134.177268185812));
#263473=CARTESIAN_POINT('Ctrl Pts',(-204.02496171939,4.95091417987762,134.047990935772));
#263474=CARTESIAN_POINT('Ctrl Pts',(-204.032385090419,5.03534928462894,
133.915280469116));
#263475=CARTESIAN_POINT('Ctrl Pts',(-204.039808461447,5.11427343323228,
133.779614860926));
#263476=CARTESIAN_POINT('Ctrl Pts',(-204.043744510888,5.15612091057836,
133.707681700217));
#263477=CARTESIAN_POINT('Ctrl Pts',(-204.047680560328,5.19641984998835,
133.634918111469));
#263478=CARTESIAN_POINT('Ctrl Pts',(-204.051616609769,5.23513874963715,
133.561397584048));
#263479=CARTESIAN_POINT('Ctrl Pts',(-204.059039876174,5.30816138600291,
133.422740163822));
#263480=CARTESIAN_POINT('Ctrl Pts',(-204.06646314258,5.3757819339304,133.280969967167));
#263481=CARTESIAN_POINT('Ctrl Pts',(-204.073886408985,5.437723476843,133.136547134955));
#263482=CARTESIAN_POINT('Ctrl Pts',(-204.081300901706,5.49959180999563,
132.992294998537));
#263483=CARTESIAN_POINT('Ctrl Pts',(-204.088715394427,5.5557943529252,132.845396806912));
#263484=CARTESIAN_POINT('Ctrl Pts',(-204.096129887148,5.60609946214324,
132.696338255663));
#263485=CARTESIAN_POINT('Ctrl Pts',(-204.103537233502,5.65635608540307,
132.547423372657));
#263486=CARTESIAN_POINT('Ctrl Pts',(-204.110944579855,5.70072647244532,
132.396352626674));
#263487=CARTESIAN_POINT('Ctrl Pts',(-204.118351926209,5.73902663486398,
132.243632602572));
#263488=CARTESIAN_POINT('Ctrl Pts',(-204.125753747884,5.77729823157674,
132.091026482824));
#263489=CARTESIAN_POINT('Ctrl Pts',(-204.13315556956,5.80950852791993,131.936773894766));
#263490=CARTESIAN_POINT('Ctrl Pts',(-204.140557391235,5.83552308162863,
131.781397426637));
#263491=CARTESIAN_POINT('Ctrl Pts',(-204.147955305546,5.86152390245685,
131.626102980537));
#263492=CARTESIAN_POINT('Ctrl Pts',(-204.155353219858,5.88133543288823,
131.469686203167));
#263493=CARTESIAN_POINT('Ctrl Pts',(-204.162751134169,5.89487415689882,
131.312680631756));
#263494=CARTESIAN_POINT('Ctrl Pts',(-204.170147819081,5.90841063101912,
131.155701151823));
#263495=CARTESIAN_POINT('Ctrl Pts',(-204.177544503993,5.9156763355876,130.998133443599));
#263496=CARTESIAN_POINT('Ctrl Pts',(-204.184941188905,5.91663952547246,
130.840517057061));
#263497=CARTESIAN_POINT('Ctrl Pts',(-204.192337545841,5.91760267264848,
130.682907659399));
#263498=CARTESIAN_POINT('Ctrl Pts',(-204.199733902776,5.91226385852082,
130.525249961006));
#263499=CARTESIAN_POINT('Ctrl Pts',(-204.207130259712,5.90064347312982,
130.368084139275));
#263500=CARTESIAN_POINT('Ctrl Pts',(-204.214527749048,5.8890213086282,130.210894255055));
#263501=CARTESIAN_POINT('Ctrl Pts',(-204.221925238385,5.87111568546889,
130.054196769752));
#263502=CARTESIAN_POINT('Ctrl Pts',(-204.229322727721,5.84699892344906,
129.898527215838));
#263503=CARTESIAN_POINT('Ctrl Pts',(-204.236722810236,5.82287370733566,
129.742803092204));
#263504=CARTESIAN_POINT('Ctrl Pts',(-204.244122892751,5.79253307447818,
129.58810798606));
#263505=CARTESIAN_POINT('Ctrl Pts',(-204.251522975266,5.75610052241988,
129.434967562853));
#263506=CARTESIAN_POINT('Ctrl Pts',(-204.258931194933,5.71962790902519,
129.281658746007));
#263507=CARTESIAN_POINT('Ctrl Pts',(-204.266339414599,5.67705008515344,
129.129908389533));
#263508=CARTESIAN_POINT('Ctrl Pts',(-204.273747634265,5.62854073617138,
128.980228017189));
#263509=CARTESIAN_POINT('Ctrl Pts',(-204.281160413567,5.58000153049444,
128.830455519072));
#263510=CARTESIAN_POINT('Ctrl Pts',(-204.288573192869,5.52552365400217,
128.682755893192));
#263511=CARTESIAN_POINT('Ctrl Pts',(-204.295985972171,5.46532888062469,
128.537620493708));
#263512=CARTESIAN_POINT('Ctrl Pts',(-204.3034093432,5.40504809813207,128.392277717958));
#263513=CARTESIAN_POINT('Ctrl Pts',(-204.310832714229,5.33903426053937,
128.249506824144));
#263514=CARTESIAN_POINT('Ctrl Pts',(-204.318256085258,5.26755537227114,
128.109775127633));
#263515=CARTESIAN_POINT('Ctrl Pts',(-204.322192134699,5.22965555059476,
128.035686029319));
#263516=CARTESIAN_POINT('Ctrl Pts',(-204.32612818414,5.19022004371018,127.962450893188));
#263517=CARTESIAN_POINT('Ctrl Pts',(-204.330064233581,5.14929365279669,
127.890135945416));
#263518=CARTESIAN_POINT('Ctrl Pts',(-204.337487499987,5.07210775681115,
127.753752210805));
#263519=CARTESIAN_POINT('Ctrl Pts',(-204.344910766392,4.98938303310252,
127.620230874498));
#263520=CARTESIAN_POINT('Ctrl Pts',(-204.352334032798,4.90135693104575,
127.490053631635));
#263521=CARTESIAN_POINT('Ctrl Pts',(-204.359748525519,4.81343486853123,
127.360030247463));
#263522=CARTESIAN_POINT('Ctrl Pts',(-204.367163018239,4.72022410681939,
127.233343395595));
#263523=CARTESIAN_POINT('Ctrl Pts',(-204.374577510961,4.62200806639798,
127.110450494586));
#263524=CARTESIAN_POINT('Ctrl Pts',(-204.381984857314,4.52388669029411,
126.987676042383));
#263525=CARTESIAN_POINT('Ctrl Pts',(-204.389392203668,4.42076987115514,
126.868688550817));
#263526=CARTESIAN_POINT('Ctrl Pts',(-204.396799550022,4.31298436294144,
126.753916636035));
#263527=CARTESIAN_POINT('Ctrl Pts',(-204.404201371697,4.20527924522689,
126.639230322478));
#263528=CARTESIAN_POINT('Ctrl Pts',(-204.411603193373,4.09291262618729,
126.528753596247));
#263529=CARTESIAN_POINT('Ctrl Pts',(-204.419005015048,3.97625150478076,
126.422882039137));
#263530=CARTESIAN_POINT('Ctrl Pts',(-204.42640292936,3.85965196787114,126.317066370797));
#263531=CARTESIAN_POINT('Ctrl Pts',(-204.433800843671,3.73876271923734,
126.215851280293));
#263532=CARTESIAN_POINT('Ctrl Pts',(-204.441198757982,3.61398749640891,
126.119595421924));
#263533=CARTESIAN_POINT('Ctrl Pts',(-204.448595442894,3.48923300895941,
126.023355559533));
#263534=CARTESIAN_POINT('Ctrl Pts',(-204.455992127807,3.36059412427482,
125.932073521404));
#263535=CARTESIAN_POINT('Ctrl Pts',(-204.463388812719,3.22850762201203,
125.846067655557));
#263536=CARTESIAN_POINT('Ctrl Pts',(-204.470785169654,3.0964269766028,125.7600656033));
#263537=CARTESIAN_POINT('Ctrl Pts',(-204.47818152659,2.9608993304014,125.679339461843));
#263538=CARTESIAN_POINT('Ctrl Pts',(-204.485577883525,2.82239017126325,
125.604164055545));
#263539=CARTESIAN_POINT('Ctrl Pts',(-204.492975372862,2.68385980601923,
125.5289771397));
#263540=CARTESIAN_POINT('Ctrl Pts',(-204.500372862198,2.54234734704194,
125.459342829222));
#263541=CARTESIAN_POINT('Ctrl Pts',(-204.507770351535,2.39834244358581,
125.395489747801));
#263542=CARTESIAN_POINT('Ctrl Pts',(-204.51517043405,2.25428705943503,125.331614282781));
#263543=CARTESIAN_POINT('Ctrl Pts',(-204.522570516565,2.1077378322723,125.273524232987));
#263544=CARTESIAN_POINT('Ctrl Pts',(-204.52997059908,1.95920377276374,125.221399831452));
#263545=CARTESIAN_POINT('Ctrl Pts',(-204.537378818746,1.81050638478601,
125.169218113778));
#263546=CARTESIAN_POINT('Ctrl Pts',(-204.544787038413,1.65982015826697,
125.123015268486));
#263547=CARTESIAN_POINT('Ctrl Pts',(-204.552195258079,1.5076693338124,125.082921660242));
#263548=CARTESIAN_POINT('Ctrl Pts',(-204.559608037382,1.35542486306415,
125.042803375052));
#263549=CARTESIAN_POINT('Ctrl Pts',(-204.567020816684,1.2017143617988,125.008801899886));
#263550=CARTESIAN_POINT('Ctrl Pts',(-204.574433595986,1.04707109441425,
124.980996238984));
#263551=CARTESIAN_POINT('Ctrl Pts',(-204.581856967014,0.89220686547698,
124.953150848049));
#263552=CARTESIAN_POINT('Ctrl Pts',(-204.589280338043,0.73640757733136,
124.931519003745));
#263553=CARTESIAN_POINT('Ctrl Pts',(-204.596703709072,0.580211258570826,
124.916127821733));
#263554=CARTESIAN_POINT('Ctrl Pts',(-204.600639758513,0.497392222485452,
124.907967047723));
#263555=CARTESIAN_POINT('Ctrl Pts',(-204.604575807954,0.414461573604239,
124.901559876592));
#263556=CARTESIAN_POINT('Ctrl Pts',(-204.608511857394,0.331499246015727,
124.896904412702));
#263557=CARTESIAN_POINT('Ctrl Pts',(-204.6159351238,0.175034885349205,124.888124353097));
#263558=CARTESIAN_POINT('Ctrl Pts',(-204.623358390205,0.017984869765548,
124.885551462325));
#263559=CARTESIAN_POINT('Ctrl Pts',(-204.630781656611,-0.139117189784255,
124.889246335491));
#263560=CARTESIAN_POINT('Ctrl Pts',(-204.638196149331,-0.296033567746183,
124.892936841624));
#263561=CARTESIAN_POINT('Ctrl Pts',(-204.645610642053,-0.453001497684593,
124.902880357385));
#263562=CARTESIAN_POINT('Ctrl Pts',(-204.653025134774,-0.609482944717867,
124.919085678993));
#263563=CARTESIAN_POINT('Ctrl Pts',(-204.660432481127,-0.765813569041512,
124.935275381302));
#263564=CARTESIAN_POINT('Ctrl Pts',(-204.667839827481,-0.92165827510939,
124.957714836041));
#263565=CARTESIAN_POINT('Ctrl Pts',(-204.675247173835,-1.07647983752149,
124.986360813346));
#263566=CARTESIAN_POINT('Ctrl Pts',(-204.68264899551,-1.23118592817213,
125.0149854254));
#263567=CARTESIAN_POINT('Ctrl Pts',(-204.690050817186,-1.38487002911259,
125.049807275314));
#263568=CARTESIAN_POINT('Ctrl Pts',(-204.697452638861,-1.53700095427533,
125.090731418094));
#263569=CARTESIAN_POINT('Ctrl Pts',(-204.704850553172,-1.689051570706,125.131633957337));
#263570=CARTESIAN_POINT('Ctrl Pts',(-204.712248467484,-1.83955028467765,
125.17863227724));
#263571=CARTESIAN_POINT('Ctrl Pts',(-204.719646381795,-1.98797712017319,
125.231580563395));
#263572=CARTESIAN_POINT('Ctrl Pts',(-204.727043066707,-2.1363792898212,
125.284520050505));
#263573=CARTESIAN_POINT('Ctrl Pts',(-204.734439751619,-2.28270991309183,
125.343407416136));
#263574=CARTESIAN_POINT('Ctrl Pts',(-204.741836436532,-2.42646506470635,
125.408047260073));
#263575=CARTESIAN_POINT('Ctrl Pts',(-204.749232793467,-2.57021384206722,
125.472684237812));
#263576=CARTESIAN_POINT('Ctrl Pts',(-204.756629150402,-2.711387034376,125.5430730336));
#263577=CARTESIAN_POINT('Ctrl Pts',(-204.764025507338,-2.84950181656107,
125.6189705686));
#263578=CARTESIAN_POINT('Ctrl Pts',(-204.771422996674,-2.98763774447108,
125.694879723706));
#263579=CARTESIAN_POINT('Ctrl Pts',(-204.778820486011,-3.12271400273242,
125.776299117558));
#263580=CARTESIAN_POINT('Ctrl Pts',(-204.786217975348,-3.25427357637751,
125.862940371059));
#263581=CARTESIAN_POINT('Ctrl Pts',(-204.793618057863,-3.38587926802739,
125.949611996517));
#263582=CARTESIAN_POINT('Ctrl Pts',(-204.801018140377,-3.5139655090601,
126.041508920977));
#263583=CARTESIAN_POINT('Ctrl Pts',(-204.808418222892,-3.63810553162232,
126.138300319705));
#263584=CARTESIAN_POINT('Ctrl Pts',(-204.815826442559,-3.76238205890143,
126.235198150526));
#263585=CARTESIAN_POINT('Ctrl Pts',(-204.823234662225,-3.88270340732681,
126.337000974104));
#263586=CARTESIAN_POINT('Ctrl Pts',(-204.830642881892,-3.99867653255975,
126.443338197255));
#263587=CARTESIAN_POINT('Ctrl Pts',(-204.838055661194,-4.11472103731682,
126.549740869193));
#263588=CARTESIAN_POINT('Ctrl Pts',(-204.845468440496,-4.22641172186707,
126.660683239356));
#263589=CARTESIAN_POINT('Ctrl Pts',(-204.852881219798,-4.33339387527508,
126.775759361022));
#263590=CARTESIAN_POINT('Ctrl Pts',(-204.860304590827,-4.44052888980039,
126.890999908847));
#263591=CARTESIAN_POINT('Ctrl Pts',(-204.867727961855,-4.54294169391004,
127.010385722194));
#263592=CARTESIAN_POINT('Ctrl Pts',(-204.875151332884,-4.64031865683491,
127.133478799047));
#263593=CARTESIAN_POINT('Ctrl Pts',(-204.879087382325,-4.69195025910903,
127.198745701977));
#263594=CARTESIAN_POINT('Ctrl Pts',(-204.883023431766,-4.74216683506,127.265054373102));
#263595=CARTESIAN_POINT('Ctrl Pts',(-204.886959481207,-4.79092677321238,
127.332336536973));
#263596=CARTESIAN_POINT('Ctrl Pts',(-204.894439644792,-4.88359133935193,
127.460201188986));
#263597=CARTESIAN_POINT('Ctrl Pts',(-204.901919808376,-4.97127200205635,
127.591969048914));
#263598=CARTESIAN_POINT('Ctrl Pts',(-204.909399971961,-5.05362495660158,
127.727218215838));
#263599=CARTESIAN_POINT('Ctrl Pts',(-204.916871063548,-5.13587803287105,
127.862303351566));
#263600=CARTESIAN_POINT('Ctrl Pts',(-204.924342155134,-5.21281607482848,
128.000861080831));
#263601=CARTESIAN_POINT('Ctrl Pts',(-204.931813246721,-5.28413634723124,
128.142437698628));
#263602=CARTESIAN_POINT('Ctrl Pts',(-204.939276676359,-5.35538347741398,
128.28386912309));
#263603=CARTESIAN_POINT('Ctrl Pts',(-204.946740105998,-5.42102414483629,
128.428312948119));
#263604=CARTESIAN_POINT('Ctrl Pts',(-204.954203535636,-5.48079969101944,
128.575287871014));
#263605=CARTESIAN_POINT('Ctrl Pts',(-204.961660708341,-5.5405251246347,
128.722139578124));
#263606=CARTESIAN_POINT('Ctrl Pts',(-204.969117881046,-5.59439509099741,
128.871517820658));
#263607=CARTESIAN_POINT('Ctrl Pts',(-204.976575053751,-5.64219757205847,
129.022918190667));
#263608=CARTESIAN_POINT('Ctrl Pts',(-204.984026968987,-5.68996635133299,
129.174211820128));
#263609=CARTESIAN_POINT('Ctrl Pts',(-204.991478884223,-5.73167605837681,
129.327524388969));
#263610=CARTESIAN_POINT('Ctrl Pts',(-204.99893079946,-5.76716343358339,
129.482333199984));
#263611=CARTESIAN_POINT('Ctrl Pts',(-205.006379560772,-5.80263578923023,
129.637076490228));
#263612=CARTESIAN_POINT('Ctrl Pts',(-205.013828322084,-5.83189097662629,
129.793314405558));
#263613=CARTESIAN_POINT('Ctrl Pts',(-205.021277083396,-5.85481604611657,
129.95051073109));
#263614=CARTESIAN_POINT('Ctrl Pts',(-205.028725022292,-5.87773858445527,
130.107689700612));
#263615=CARTESIAN_POINT('Ctrl Pts',(-205.036172961189,-5.89433233816279,
130.265826508781));
#263616=CARTESIAN_POINT('Ctrl Pts',(-205.043620900085,-5.90453575298649,
130.424376270251));
#263617=CARTESIAN_POINT('Ctrl Pts',(-205.049622202654,-5.91275732682686,
130.552130418624));
#263618=CARTESIAN_POINT('Ctrl Pts',(-205.055623505223,-5.91683088167834,
130.680152436099));
#263619=CARTESIAN_POINT('Ctrl Pts',(-205.061624807792,-5.91674878301709,
130.808155504365));
#263620=CARTESIAN_POINT('',(-206.811623324931,-5.92153837798521,130.807366761688));
#263621=CARTESIAN_POINT('Ctrl Pts',(-205.061626944303,-5.90947417380247,
130.808196352657));
#263622=CARTESIAN_POINT('Ctrl Pts',(-205.096220331209,-5.91377200472859,
131.545141902329));
#263623=CARTESIAN_POINT('Ctrl Pts',(-205.223629592719,-5.44370849995411,
134.254054771831));
#263624=CARTESIAN_POINT('Ctrl Pts',(-205.443854728833,-1.37967370610466,
137.665414544981));
#263625=CARTESIAN_POINT('Ctrl Pts',(-205.722302352646,5.0266516457322,135.673686419238));
#263626=CARTESIAN_POINT('Ctrl Pts',(-206.000749976459,6.813729700728,129.207285761534));
#263627=CARTESIAN_POINT('Ctrl Pts',(-206.279197600272,2.3393230299546,124.208518875085));
#263628=CARTESIAN_POINT('Ctrl Pts',(-206.549488398635,-4.09076040919075,
125.239883832662));
#263629=CARTESIAN_POINT('Ctrl Pts',(-206.726963322394,-5.91340440505827,
129.015638925646));
#263630=CARTESIAN_POINT('Ctrl Pts',(-206.811622371547,-5.92461749863669,
130.807348163968));
#263631=CARTESIAN_POINT('Ctrl Pts',(-206.811624807792,-5.91674922156144,
130.807395687932));
#263632=CARTESIAN_POINT('Ctrl Pts',(-206.819780821161,-5.91666079577132,
130.979778256311));
#263633=CARTESIAN_POINT('Ctrl Pts',(-206.827936834529,-5.90903961803116,
131.151962513016));
#263634=CARTESIAN_POINT('Ctrl Pts',(-206.836092847897,-5.89393313865187,
131.323477867907));
#263635=CARTESIAN_POINT('Ctrl Pts',(-206.843516422095,-5.88018327514893,
131.479590530506));
#263636=CARTESIAN_POINT('Ctrl Pts',(-206.850939996293,-5.86020589862519,
131.635392596784));
#263637=CARTESIAN_POINT('Ctrl Pts',(-206.858363570491,-5.83401756875813,
131.790347214798));
#263638=CARTESIAN_POINT('Ctrl Pts',(-206.865778303408,-5.80786042849981,
131.945117285957));
#263639=CARTESIAN_POINT('Ctrl Pts',(-206.873193036325,-5.77550712091378,
132.099041553354));
#263640=CARTESIAN_POINT('Ctrl Pts',(-206.880607769242,-5.73702611008395,
132.251586230494));
#263641=CARTESIAN_POINT('Ctrl Pts',(-206.888015288472,-5.69858253687992,
132.403982499097));
#263642=CARTESIAN_POINT('Ctrl Pts',(-206.895422807702,-5.65402321989905,
132.555001489991));
#263643=CARTESIAN_POINT('Ctrl Pts',(-206.902830326931,-5.60346799857048,
132.704117694536));
#263644=CARTESIAN_POINT('Ctrl Pts',(-206.910232254374,-5.55295094035424,
132.853121334279));
#263645=CARTESIAN_POINT('Ctrl Pts',(-206.917634181817,-5.49644710986732,
133.000224695794));
#263646=CARTESIAN_POINT('Ctrl Pts',(-206.925036109261,-5.43412666074035,
133.144915679412));
#263647=CARTESIAN_POINT('Ctrl Pts',(-206.932434348698,-5.37183726273652,
133.289534570841));
#263648=CARTESIAN_POINT('Ctrl Pts',(-206.939832588136,-5.30373716364741,
133.431743135487));
#263649=CARTESIAN_POINT('Ctrl Pts',(-206.947230827574,-5.23004527582684,
133.57104762106));
#263650=CARTESIAN_POINT('Ctrl Pts',(-206.954627182734,-5.15637215678872,
133.710316626804));
#263651=CARTESIAN_POINT('Ctrl Pts',(-206.962023537895,-5.07711025803544,
133.846682695997));
#263652=CARTESIAN_POINT('Ctrl Pts',(-206.969419893055,-4.99252519862058,
133.97967520098));
#263653=CARTESIAN_POINT('Ctrl Pts',(-206.976815824747,-4.9079449820142,
134.112660091648));
#263654=CARTESIAN_POINT('Ctrl Pts',(-206.984211756438,-4.81804241190689,
134.242271487812));
#263655=CARTESIAN_POINT('Ctrl Pts',(-206.99160768813,-4.72312724667466,
134.368066494069));
#263656=CARTESIAN_POINT('Ctrl Pts',(-206.999004656617,-4.62819877580896,
134.493879134833));
#263657=CARTESIAN_POINT('Ctrl Pts',(-207.006401625103,-4.52825653613315,
134.615874023046));
#263658=CARTESIAN_POINT('Ctrl Pts',(-207.01379859359,-4.42365139311575,
134.733640311694));
#263659=CARTESIAN_POINT('Ctrl Pts',(-207.021201700528,-4.31895944243015,
134.851504329924));
#263660=CARTESIAN_POINT('Ctrl Pts',(-207.028604807466,-4.20959710649542,
134.965132459073));
#263661=CARTESIAN_POINT('Ctrl Pts',(-207.036007914404,-4.09595347651789,
135.074149333732));
#263662=CARTESIAN_POINT('Ctrl Pts',(-207.043414228711,-3.98226061085117,
135.183213439556));
#263663=CARTESIAN_POINT('Ctrl Pts',(-207.050820543018,-3.86428303275637,
135.287662060798));
#263664=CARTESIAN_POINT('Ctrl Pts',(-207.058226857325,-3.74244355311888,
135.387159632821));
#263665=CARTESIAN_POINT('Ctrl Pts',(-207.065642606406,-3.62044886429578,
135.486783953063));
#263666=CARTESIAN_POINT('Ctrl Pts',(-207.073058355488,-3.49458274227156,
135.581444397463));
#263667=CARTESIAN_POINT('Ctrl Pts',(-207.08047410457,-3.36529835974214,
135.670847801605));
#263668=CARTESIAN_POINT('Ctrl Pts',(-207.086208830725,-3.26532052582677,
135.73998498984));
#263669=CARTESIAN_POINT('Ctrl Pts',(-207.091943556881,-3.16329913061462,
135.805979224788));
#263670=CARTESIAN_POINT('Ctrl Pts',(-207.097678283037,-3.05945365335209,
135.868713873954));
#263671=CARTESIAN_POINT('Origin',(210.,0.,130.804360617566));
#263672=CARTESIAN_POINT('',(-178.530629926805,1.98348391145776,125.240348466903));
#263673=CARTESIAN_POINT('Ctrl Pts',(-178.18410255161,3.73285074851184,126.213744553045));
#263674=CARTESIAN_POINT('Ctrl Pts',(-178.294692878395,3.30225397105088,
125.863605599916));
#263675=CARTESIAN_POINT('Ctrl Pts',(-178.403686871865,2.806068509165,125.563687251781));
#263676=CARTESIAN_POINT('Ctrl Pts',(-178.503050604127,2.18460962668051,
125.30481172624));
#263677=CARTESIAN_POINT('Ctrl Pts',(-178.516849507463,2.09302951709462,
125.269308805648));
#263678=CARTESIAN_POINT('Ctrl Pts',(-178.529878634857,2.00062638375932,
125.236109129432));
#263679=CARTESIAN_POINT('',(-177.987180129183,4.43101178267811,134.710827119055));
#263680=CARTESIAN_POINT('Ctrl Pts',(-177.98715711374,4.43823075232565,134.717165027655));
#263681=CARTESIAN_POINT('Ctrl Pts',(-177.917823106101,4.66836223140131,
134.456130613341));
#263682=CARTESIAN_POINT('Ctrl Pts',(-177.848712438811,4.88126271378723,
134.167633593295));
#263683=CARTESIAN_POINT('Ctrl Pts',(-177.785458995272,5.06765282954142,
133.85834577826));
#263684=CARTESIAN_POINT('Ctrl Pts',(-178.529931596729,1.99775342761758,
125.244229456078));
#263685=CARTESIAN_POINT('Ctrl Pts',(-178.491569805427,2.76854523389136,
125.517184209005));
#263686=CARTESIAN_POINT('Ctrl Pts',(-178.36039213952,5.21384277720883,126.968629961239));
#263687=CARTESIAN_POINT('Ctrl Pts',(-178.179474983672,6.55706668978598,
131.115450305371));
#263688=CARTESIAN_POINT('Ctrl Pts',(-178.036919619125,5.13087667649733,
133.913851480684));
#263689=CARTESIAN_POINT('Ctrl Pts',(-177.987180129183,4.43101178267811,
134.710827119055));
#263690=CARTESIAN_POINT('Origin',(210.,0.,130.804360617566));
#263691=CARTESIAN_POINT('',(-207.299567498839,-3.90840034609305,135.243902605346));
#263692=CARTESIAN_POINT('Ctrl Pts',(-207.097024439715,-3.07128565518615,
135.861547087012));
#263693=CARTESIAN_POINT('Ctrl Pts',(-207.161528107063,-3.37326783662078,
135.678149945624));
#263694=CARTESIAN_POINT('Ctrl Pts',(-207.230903561036,-3.65533760795257,
135.469418255391));
#263695=CARTESIAN_POINT('Ctrl Pts',(-207.299550587757,-3.91125355034577,
135.243958147456));
#263696=CARTESIAN_POINT('',(-178.657321351531,-0.670823532967099,124.921705606293));
#263697=CARTESIAN_POINT('Ctrl Pts',(-178.656496695459,-0.652296033834956,
124.923676945854));
#263698=CARTESIAN_POINT('Ctrl Pts',(-178.631041117028,-1.20105617910375,
124.984546410404));
#263699=CARTESIAN_POINT('Ctrl Pts',(-178.571675042675,-1.75540607403642,
125.126022270676));
#263700=CARTESIAN_POINT('Ctrl Pts',(-178.487473351945,-2.28203573490688,
125.345395642053));
#263701=CARTESIAN_POINT('Ctrl Pts',(-178.486373882786,-2.28888204220153,
125.348262685419));
#263702=CARTESIAN_POINT('Ctrl Pts',(-178.485270545702,-2.29572256715809,
125.351142443209));
#263703=CARTESIAN_POINT('',(-179.063374001572,-5.91358993803376,130.79964208133));
#263704=CARTESIAN_POINT('Ctrl Pts',(-179.063373167743,-5.91137817917409,
130.799626087985));
#263705=CARTESIAN_POINT('Ctrl Pts',(-179.032829268644,-5.91617425954304,
130.149473536606));
#263706=CARTESIAN_POINT('Ctrl Pts',(-178.909469494942,-5.51702945710787,
127.529389957826));
#263707=CARTESIAN_POINT('Ctrl Pts',(-178.774255230047,-3.11548842989244,
125.328065259864));
#263708=CARTESIAN_POINT('Ctrl Pts',(-178.66958486425,-0.929687989411222,
124.947409885417));
#263709=CARTESIAN_POINT('Ctrl Pts',(-178.657730373058,-0.680012995400244,
124.920727840718));
#263710=CARTESIAN_POINT('',(-180.813376354123,-5.91239331584027,130.807847145143));
#263711=CARTESIAN_POINT('Ctrl Pts',(-180.813375192208,-5.91674898580156,
130.807824938015));
#263712=CARTESIAN_POINT('Ctrl Pts',(-180.80590436759,-5.91684231226662,
130.648431696059));
#263713=CARTESIAN_POINT('Ctrl Pts',(-180.798433542972,-5.91049037800369,
130.489025468643));
#263714=CARTESIAN_POINT('Ctrl Pts',(-180.790962718354,-5.89771667312605,
130.330157490171));
#263715=CARTESIAN_POINT('Ctrl Pts',(-180.783490770938,-5.88494104847493,
130.171265635264));
#263716=CARTESIAN_POINT('Ctrl Pts',(-180.776018823522,-5.86574175873066,
130.012912552212));
#263717=CARTESIAN_POINT('Ctrl Pts',(-180.768546876106,-5.84019423006307,
129.855644686616));
#263718=CARTESIAN_POINT('Ctrl Pts',(-180.761072443837,-5.81463820537227,
129.698324520407));
#263719=CARTESIAN_POINT('Ctrl Pts',(-180.753598011569,-5.78272979363846,
129.542090648727));
#263720=CARTESIAN_POINT('Ctrl Pts',(-180.7461235793,-5.74459562263046,129.3874796434));
#263721=CARTESIAN_POINT('Ctrl Pts',(-180.738645298881,-5.70644181855295,
129.232789037847));
#263722=CARTESIAN_POINT('Ctrl Pts',(-180.731167018461,-5.66205595596423,
129.079723315102));
#263723=CARTESIAN_POINT('Ctrl Pts',(-180.723688738042,-5.61161462016539,
128.928804188864));
#263724=CARTESIAN_POINT('Ctrl Pts',(-180.716200537055,-5.56110636969527,
128.777684855721));
#263725=CARTESIAN_POINT('Ctrl Pts',(-180.708712336068,-5.50452671422177,
128.628718151764));
#263726=CARTESIAN_POINT('Ctrl Pts',(-180.701224135081,-5.4421008949015,
128.482407040896));
#263727=CARTESIAN_POINT('Ctrl Pts',(-180.693730469935,-5.37962952330192,
128.335989166437));
#263728=CARTESIAN_POINT('Ctrl Pts',(-180.686236804789,-5.31130363918635,
128.192231074739));
#263729=CARTESIAN_POINT('Ctrl Pts',(-180.678743139642,-5.23739446975496,
128.051611131928));
#263730=CARTESIAN_POINT('Ctrl Pts',(-180.67123737861,-5.16336599996819,
127.910764207684));
#263731=CARTESIAN_POINT('Ctrl Pts',(-180.663731617577,-5.0837364204128,
127.773065865971));
#263732=CARTESIAN_POINT('Ctrl Pts',(-180.656225856544,-4.99882089239424,
127.638966448073));
#263733=CARTESIAN_POINT('Ctrl Pts',(-180.651626308805,-4.9467844602118,
127.556790014292));
#263734=CARTESIAN_POINT('Ctrl Pts',(-180.647026761065,-4.89276383469503,
127.475964459253));
#263735=CARTESIAN_POINT('Ctrl Pts',(-180.642427213326,-4.83683886899804,
127.396587104281));
#263736=CARTESIAN_POINT('Ctrl Pts',(-180.63500394692,-4.74658088221714,
127.26847901934));
#263737=CARTESIAN_POINT('Ctrl Pts',(-180.627580680515,-4.65109331048002,
127.143765544506));
#263738=CARTESIAN_POINT('Ctrl Pts',(-180.62015741411,-4.55065994398724,
127.022902613477));
#263739=CARTESIAN_POINT('Ctrl Pts',(-180.612742921389,-4.45034528139318,
126.902182532395));
#263740=CARTESIAN_POINT('Ctrl Pts',(-180.605328428668,-4.34509669582955,
126.785304220586));
#263741=CARTESIAN_POINT('Ctrl Pts',(-180.597913935947,-4.23524133075553,
126.672694920446));
#263742=CARTESIAN_POINT('Ctrl Pts',(-180.590506589593,-4.12549184841834,
126.560194157389));
#263743=CARTESIAN_POINT('Ctrl Pts',(-180.583099243239,-4.01114468503391,
126.451954479988));
#263744=CARTESIAN_POINT('Ctrl Pts',(-180.575691896886,-3.89256726626094,
126.348370195658));
#263745=CARTESIAN_POINT('Ctrl Pts',(-180.56829007521,-3.77407828700056,
126.244863168396));
#263746=CARTESIAN_POINT('Ctrl Pts',(-180.560888253535,-3.65136561447588,
126.146004865181));
#263747=CARTESIAN_POINT('Ctrl Pts',(-180.55348643186,-3.52483346582677,
126.05215275167));
#263748=CARTESIAN_POINT('Ctrl Pts',(-180.546088517549,-3.39836811251472,
125.958350181959));
#263749=CARTESIAN_POINT('Ctrl Pts',(-180.538690603237,-3.26808759764599,
125.869548760655));
#263750=CARTESIAN_POINT('Ctrl Pts',(-180.531292688926,-3.13442905661681,
125.78606558324));
#263751=CARTESIAN_POINT('Ctrl Pts',(-180.523896004014,-3.00079272721176,
125.702596279216));
#263752=CARTESIAN_POINT('Ctrl Pts',(-180.516499319102,-2.86377980209576,
125.624443662571));
#263753=CARTESIAN_POINT('Ctrl Pts',(-180.50910263419,-2.72385632332298,
125.551881460787));
#263754=CARTESIAN_POINT('Ctrl Pts',(-180.501706277254,-2.58393904890388,
125.479322476488));
#263755=CARTESIAN_POINT('Ctrl Pts',(-180.494309920319,-2.44111180882452,
125.412353586024));
#263756=CARTESIAN_POINT('Ctrl Pts',(-180.486913563384,-2.29586492173638,
125.351202374526));
#263757=CARTESIAN_POINT('Ctrl Pts',(-180.479516074047,-2.15059579697861,
125.29004180062));
#263758=CARTESIAN_POINT('Ctrl Pts',(-180.472118584711,-2.0029066316598,
125.234700824044));
#263759=CARTESIAN_POINT('Ctrl Pts',(-180.464721095374,-1.85330723241896,
125.185358671956));
#263760=CARTESIAN_POINT('Ctrl Pts',(-180.457321012859,-1.70365539134041,
125.135999223054));
#263761=CARTESIAN_POINT('Ctrl Pts',(-180.449920930344,-1.55209233740366,
125.092642902312));
#263762=CARTESIAN_POINT('Ctrl Pts',(-180.442520847829,-1.39914237269438,
125.055418872912));
#263763=CARTESIAN_POINT('Ctrl Pts',(-180.435112628163,-1.24602422377592,
125.018153911864));
#263764=CARTESIAN_POINT('Ctrl Pts',(-180.427704408496,-1.0915164813912,
124.987034796868));
#263765=CARTESIAN_POINT('Ctrl Pts',(-180.42029618883,-0.936153686024078,
124.962139564007));
#263766=CARTESIAN_POINT('Ctrl Pts',(-180.412883409528,-0.780695267448333,
124.937229008546));
#263767=CARTESIAN_POINT('Ctrl Pts',(-180.405470630226,-0.624381117031028,
124.91855001255));
#263768=CARTESIAN_POINT('Ctrl Pts',(-180.398057850924,-0.467749690625702,
124.906128612175));
#263769=CARTESIAN_POINT('Ctrl Pts',(-180.390634479895,-0.310894461893262,
124.893689463521));
#263770=CARTESIAN_POINT('Ctrl Pts',(-180.383211108867,-0.153721423776527,
124.887525782551));
#263771=CARTESIAN_POINT('Ctrl Pts',(-180.375787737838,0.00323134341759472,
124.887611499941));
#263772=CARTESIAN_POINT('Ctrl Pts',(-180.371851688396,0.0864514666357916,
124.887656949358));
#263773=CARTESIAN_POINT('Ctrl Pts',(-180.367915638954,0.169609742978011,
124.889458461255));
#263774=CARTESIAN_POINT('Ctrl Pts',(-180.363979589513,0.252626814831058,
124.893006267256));
#263775=CARTESIAN_POINT('Ctrl Pts',(-180.356556323107,0.409194421432122,
124.899697318649));
#263776=CARTESIAN_POINT('Ctrl Pts',(-180.349133056702,0.565732764817981,
124.912623037657));
#263777=CARTESIAN_POINT('Ctrl Pts',(-180.341709790296,0.721704859521438,
124.931791106846));
#263778=CARTESIAN_POINT('Ctrl Pts',(-180.334295297575,0.877492608161631,
124.950936520968));
#263779=CARTESIAN_POINT('Ctrl Pts',(-180.326880804854,1.03271507339061,
124.976309554354));
#263780=CARTESIAN_POINT('Ctrl Pts',(-180.319466312133,1.18683597505039,
125.007865906896));
#263781=CARTESIAN_POINT('Ctrl Pts',(-180.31205896578,1.34080832918305,125.039391844237));
#263782=CARTESIAN_POINT('Ctrl Pts',(-180.304651619426,1.49368087018309,
125.077089161737));
#263783=CARTESIAN_POINT('Ctrl Pts',(-180.297244273072,1.6449232535122,125.120861866572));
#263784=CARTESIAN_POINT('Ctrl Pts',(-180.289842451397,1.79605283456535,
125.164601924071));
#263785=CARTESIAN_POINT('Ctrl Pts',(-180.282440629721,1.94555432179695,
125.214408243235));
#263786=CARTESIAN_POINT('Ctrl Pts',(-180.275038808046,2.09290847999003,
125.270133963653));
#263787=CARTESIAN_POINT('Ctrl Pts',(-180.267640893735,2.24018485107,125.325830266896));
#263788=CARTESIAN_POINT('Ctrl Pts',(-180.260242979423,2.38531580236709,
125.387439616482));
#263789=CARTESIAN_POINT('Ctrl Pts',(-180.252845065112,2.52779827011158,
125.454765635876));
#263790=CARTESIAN_POINT('Ctrl Pts',(-180.2454483802,2.67025705985461,125.522080466907));
#263791=CARTESIAN_POINT('Ctrl Pts',(-180.238051695287,2.81006790238803,
125.595109922935));
#263792=CARTESIAN_POINT('Ctrl Pts',(-180.230655010375,2.94674859591522,
125.673609865973));
#263793=CARTESIAN_POINT('Ctrl Pts',(-180.22325865344,3.08342322887723,125.752106328241));
#263794=CARTESIAN_POINT('Ctrl Pts',(-180.215862296504,3.21696766509498,
125.836072609297));
#263795=CARTESIAN_POINT('Ctrl Pts',(-180.208465939569,3.34692540154562,
125.925219205495));
#263796=CARTESIAN_POINT('Ctrl Pts',(-180.201068450232,3.47690303485747,
126.014379450264));
#263797=CARTESIAN_POINT('Ctrl Pts',(-180.193670960896,3.60329256715243,
126.108721378205));
#263798=CARTESIAN_POINT('Ctrl Pts',(-180.186273471559,3.72566764660411,
126.20791295121));
#263799=CARTESIAN_POINT('Ctrl Pts',(-180.178873389044,3.84808562445071,
126.307139295668));
#263800=CARTESIAN_POINT('Ctrl Pts',(-180.171473306529,3.96648605779236,
126.411218435038));
#263801=CARTESIAN_POINT('Ctrl Pts',(-180.164073224014,4.08047687990288,
126.519779074979));
#263802=CARTESIAN_POINT('Ctrl Pts',(-180.156665004348,4.19459304664037,
126.628459088503));
#263803=CARTESIAN_POINT('Ctrl Pts',(-180.149256784681,4.30428964824568,
126.741630186279));
#263804=CARTESIAN_POINT('Ctrl Pts',(-180.141848565015,4.40921209856459,
126.858884824665));
#263805=CARTESIAN_POINT('Ctrl Pts',(-180.134435785713,4.51419912690065,
126.976211631324));
#263806=CARTESIAN_POINT('Ctrl Pts',(-180.127023006411,4.61440591173413,
127.097626699522));
#263807=CARTESIAN_POINT('Ctrl Pts',(-180.119610227109,4.7095194995687,127.222691084278));
#263808=CARTESIAN_POINT('Ctrl Pts',(-180.11218685608,4.80476899015836,127.347934166893));
#263809=CARTESIAN_POINT('Ctrl Pts',(-180.104763485052,4.89491053578961,
127.476836675114));
#263810=CARTESIAN_POINT('Ctrl Pts',(-180.097340114023,4.97967522377445,
127.608931815632));
#263811=CARTESIAN_POINT('Ctrl Pts',(-180.093404064582,5.02461949524755,
127.678971828719));
#263812=CARTESIAN_POINT('Ctrl Pts',(-180.089468015141,5.06805291187504,
127.749909002942));
#263813=CARTESIAN_POINT('Ctrl Pts',(-180.0855319657,5.10994079734045,127.821671292448));
#263814=CARTESIAN_POINT('Ctrl Pts',(-180.078108699294,5.18894004204775,
127.957012730823));
#263815=CARTESIAN_POINT('Ctrl Pts',(-180.070685432889,5.2626780668334,128.095699539363));
#263816=CARTESIAN_POINT('Ctrl Pts',(-180.063262166483,5.33085815437477,
128.2372840896));
#263817=CARTESIAN_POINT('Ctrl Pts',(-180.055847673762,5.39895765871467,
128.378701298656));
#263818=CARTESIAN_POINT('Ctrl Pts',(-180.048433181041,5.46151214110167,
128.523009099099));
#263819=CARTESIAN_POINT('Ctrl Pts',(-180.04101868832,5.51826899994545,128.669732357952));
#263820=CARTESIAN_POINT('Ctrl Pts',(-180.033611341967,5.57497115439181,
128.816314199405));
#263821=CARTESIAN_POINT('Ctrl Pts',(-180.026203995613,5.62588667606558,
128.965306518641));
#263822=CARTESIAN_POINT('Ctrl Pts',(-180.018796649259,5.67080966227076,
129.116211235314));
#263823=CARTESIAN_POINT('Ctrl Pts',(-180.011394827583,5.71569914321786,
129.267003401556));
#263824=CARTESIAN_POINT('Ctrl Pts',(-180.003993005908,5.75460488194266,
129.419704768962));
#263825=CARTESIAN_POINT('Ctrl Pts',(-179.996591184232,5.78736977694945,
129.573799108599));
#263826=CARTESIAN_POINT('Ctrl Pts',(-179.989193269921,5.8201173756232,129.727812103033));
#263827=CARTESIAN_POINT('Ctrl Pts',(-179.98179535561,5.84673050914526,129.883216241026));
#263828=CARTESIAN_POINT('Ctrl Pts',(-179.974397441298,5.86710247640078,
130.039482134464));
#263829=CARTESIAN_POINT('Ctrl Pts',(-179.967000756386,5.88747105820495,
130.195722059347));
#263830=CARTESIAN_POINT('Ctrl Pts',(-179.959604071474,5.90160048400506,
130.352823085647));
#263831=CARTESIAN_POINT('Ctrl Pts',(-179.952207386562,5.9094355121563,130.51024756079));
#263832=CARTESIAN_POINT('Ctrl Pts',(-179.944811029626,5.91727019289419,
130.667665055567));
#263833=CARTESIAN_POINT('Ctrl Pts',(-179.937414672691,5.91881101237257,
130.825405597834));
#263834=CARTESIAN_POINT('Ctrl Pts',(-179.930018315755,5.91405478717383,
130.982928634877));
#263835=CARTESIAN_POINT('Ctrl Pts',(-179.922620826419,5.90929783378486,
131.140475789099));
#263836=CARTESIAN_POINT('Ctrl Pts',(-179.915223337082,5.89824192734704,
131.297804998638));
#263837=CARTESIAN_POINT('Ctrl Pts',(-179.907825847746,5.88093596734664,
131.454378086923));
#263838=CARTESIAN_POINT('Ctrl Pts',(-179.900425765231,5.86362394076881,
131.61100606166));
#263839=CARTESIAN_POINT('Ctrl Pts',(-179.893025682716,5.84005753945498,
131.766877016608));
#263840=CARTESIAN_POINT('Ctrl Pts',(-179.885625600201,5.81033722220633,
131.921460401266));
#263841=CARTESIAN_POINT('Ctrl Pts',(-179.878217380534,5.78058422441342,
132.076213766249));
#263842=CARTESIAN_POINT('Ctrl Pts',(-179.870809160868,5.74466386733851,
132.229676366655));
#263843=CARTESIAN_POINT('Ctrl Pts',(-179.863400941201,5.70272736651028,
132.381329591818));
#263844=CARTESIAN_POINT('Ctrl Pts',(-179.855988161899,5.66076505446567,
132.533076157011));
#263845=CARTESIAN_POINT('Ctrl Pts',(-179.848575382597,5.61277933382527,
132.683010773186));
#263846=CARTESIAN_POINT('Ctrl Pts',(-179.841162603295,5.55897034242447,
132.830632883217));
#263847=CARTESIAN_POINT('Ctrl Pts',(-179.833739232266,5.50508446621329,
132.978465922642));
#263848=CARTESIAN_POINT('Ctrl Pts',(-179.826315861237,5.44535884258079,
133.123979512235));
#263849=CARTESIAN_POINT('Ctrl Pts',(-179.818892490209,5.380040844081,133.266695094951));
#263850=CARTESIAN_POINT('Ctrl Pts',(-179.814956440768,5.34540767399451,
133.342366321317));
#263851=CARTESIAN_POINT('Ctrl Pts',(-179.811020391327,5.30920304288685,
133.417251360219));
#263852=CARTESIAN_POINT('Ctrl Pts',(-179.807084341887,5.27146882157906,
133.491282094949));
#263853=CARTESIAN_POINT('Ctrl Pts',(-179.799661075481,5.20030325783337,
133.630901750236));
#263854=CARTESIAN_POINT('Ctrl Pts',(-179.792237809076,5.12347932154279,
133.767903246486));
#263855=CARTESIAN_POINT('Ctrl Pts',(-179.784814542671,5.04121323225327,
133.901794992893));
#263856=CARTESIAN_POINT('Ctrl Pts',(-179.77740004995,4.95904437464975,134.035528490373));
#263857=CARTESIAN_POINT('Ctrl Pts',(-179.769985557229,4.87144636083707,
134.166159239093));
#263858=CARTESIAN_POINT('Ctrl Pts',(-179.762571064508,4.77868239631381,
134.293217897201));
#263859=CARTESIAN_POINT('Ctrl Pts',(-179.755163718154,4.68600784119206,
134.42015409139));
#263860=CARTESIAN_POINT('Ctrl Pts',(-179.7477563718,4.5881774664831,134.543524749663));
#263861=CARTESIAN_POINT('Ctrl Pts',(-179.740349025446,4.485499025852,134.662887415656));
#263862=CARTESIAN_POINT('Ctrl Pts',(-179.732947203771,4.38289716667605,
134.78216105647));
#263863=CARTESIAN_POINT('Ctrl Pts',(-179.725545382096,4.27545468365737,
134.897432375347));
#263864=CARTESIAN_POINT('Ctrl Pts',(-179.71814356042,4.16352097762122,135.008290164003));
#263865=CARTESIAN_POINT('Ctrl Pts',(-179.710745646109,4.05164636051687,
135.119089431696));
#263866=CARTESIAN_POINT('Ctrl Pts',(-179.703347731798,3.93528550668121,
135.225479547193));
#263867=CARTESIAN_POINT('Ctrl Pts',(-179.695949817487,3.81482613076614,
135.32708459262));
#263868=CARTESIAN_POINT('Ctrl Pts',(-179.688553132574,3.69438677301383,
135.428672753131));
#263869=CARTESIAN_POINT('Ctrl Pts',(-179.681156447662,3.56985053003108,
135.525477181344));
#263870=CARTESIAN_POINT('Ctrl Pts',(-179.67375976275,3.44163988469777,135.617160786548));
#263871=CARTESIAN_POINT('Ctrl Pts',(-179.666363405815,3.31343492435919,
135.708840326406));
#263872=CARTESIAN_POINT('Ctrl Pts',(-179.658967048879,3.18155618927124,
135.795399277593));
#263873=CARTESIAN_POINT('Ctrl Pts',(-179.651570691944,3.04645674102676,
135.876542779866));
#263874=CARTESIAN_POINT('Ctrl Pts',(-179.644173202607,2.91133660871186,
135.957698705416));
#263875=CARTESIAN_POINT('Ctrl Pts',(-179.636775713271,2.77299510144716,
136.033437338946));
#263876=CARTESIAN_POINT('Ctrl Pts',(-179.629378223934,2.63191143379257,
136.103508923395));
#263877=CARTESIAN_POINT('Ctrl Pts',(-179.621978141419,2.49077830947559,
136.17360507133));
#263878=CARTESIAN_POINT('Ctrl Pts',(-179.614578058904,2.3469014450307,136.23803004898));
#263879=CARTESIAN_POINT('Ctrl Pts',(-179.607177976389,2.20078150805586,
136.296581599673));
#263880=CARTESIAN_POINT('Ctrl Pts',(-179.599769756723,2.05450089718987,
136.355197533815));
#263881=CARTESIAN_POINT('Ctrl Pts',(-179.592361537056,1.90597263478008,
136.407927004143));
#263882=CARTESIAN_POINT('Ctrl Pts',(-179.58495331739,1.75571477835447,136.45461691083));
#263883=CARTESIAN_POINT('Ctrl Pts',(-179.577540538088,1.60536444072542,
136.501335554375));
#263884=CARTESIAN_POINT('Ctrl Pts',(-179.570127758786,1.45328274764712,
136.542007130973));
#263885=CARTESIAN_POINT('Ctrl Pts',(-179.562714979484,1.29999901139323,
136.576529458901));
#263886=CARTESIAN_POINT('Ctrl Pts',(-179.555291608455,1.14649625614847,
136.611101113949));
#263887=CARTESIAN_POINT('Ctrl Pts',(-179.547868237426,0.991788393612213,
136.639505904812));
#263888=CARTESIAN_POINT('Ctrl Pts',(-179.540444866397,0.836411758288183,
136.661693281253));
#263889=CARTESIAN_POINT('Ctrl Pts',(-179.536508816957,0.754027338025988,
136.673457560621));
#263890=CARTESIAN_POINT('Ctrl Pts',(-179.532572767516,0.671454946475021,
136.683474771799));
#263891=CARTESIAN_POINT('Ctrl Pts',(-179.528636718075,0.588774524354783,
136.691743323147));
#263892=CARTESIAN_POINT('Ctrl Pts',(-179.521213451669,0.432841828606704,
136.707337552936));
#263893=CARTESIAN_POINT('Ctrl Pts',(-179.513790185264,0.276053375632314,
136.716756054739));
#263894=CARTESIAN_POINT('Ctrl Pts',(-179.506366918858,0.118939626646369,
136.719915023343));
#263895=CARTESIAN_POINT('Ctrl Pts',(-179.498952426137,-0.0379884269357607,
136.723070258309));
#263896=CARTESIAN_POINT('Ctrl Pts',(-179.491537933416,-0.195240641656169,
136.7199806789));
#263897=CARTESIAN_POINT('Ctrl Pts',(-179.484123440695,-0.352279877922297,
136.710614036622));
#263898=CARTESIAN_POINT('Ctrl Pts',(-179.476716094341,-0.509167753859644,
136.701256422266));
#263899=CARTESIAN_POINT('Ctrl Pts',(-179.469308747988,-0.665842689874027,
136.685633811616));
#263900=CARTESIAN_POINT('Ctrl Pts',(-179.461901401634,-0.821766086522907,
136.663765968072));
#263901=CARTESIAN_POINT('Ctrl Pts',(-179.454499579958,-0.977573189619913,
136.641914434392));
#263902=CARTESIAN_POINT('Ctrl Pts',(-179.447097758283,-1.13262950134629,
136.61382699401));
#263903=CARTESIAN_POINT('Ctrl Pts',(-179.439695936607,-1.28640020084502,
136.579575339615));
#263904=CARTESIAN_POINT('Ctrl Pts',(-179.432298022296,-1.44008972598887,
136.545341766401));
#263905=CARTESIAN_POINT('Ctrl Pts',(-179.424900107985,-1.59249462705246,
136.504950540707));
#263906=CARTESIAN_POINT('Ctrl Pts',(-179.417502193673,-1.74308906444127,
136.458524665056));
#263907=CARTESIAN_POINT('Ctrl Pts',(-179.410105508761,-1.89365847576642,
136.412106504543));
#263908=CARTESIAN_POINT('Ctrl Pts',(-179.402708823849,-2.04241766416558,
136.3596557943));
#263909=CARTESIAN_POINT('Ctrl Pts',(-179.395312138936,-2.18885466336137,
136.301345775376));
#263910=CARTESIAN_POINT('Ctrl Pts',(-179.387915782001,-2.33528516938715,
136.243038341979));
#263911=CARTESIAN_POINT('Ctrl Pts',(-179.380519425065,-2.47939334413142,
136.178872254585));
#263912=CARTESIAN_POINT('Ctrl Pts',(-179.37312306813,-2.62068622246135,
136.109069307579));
#263913=CARTESIAN_POINT('Ctrl Pts',(-179.365725578793,-2.76200073309085,
136.039255673564));
#263914=CARTESIAN_POINT('Ctrl Pts',(-179.358328089457,-2.90049875436519,
135.963803626908));
#263915=CARTESIAN_POINT('Ctrl Pts',(-179.35093060012,-3.03571113142043,
135.882981344601));
#263916=CARTESIAN_POINT('Ctrl Pts',(-179.343530517605,-3.17097090696619,
135.802130730167));
#263917=CARTESIAN_POINT('Ctrl Pts',(-179.33613043509,-3.30294242489327,
135.715906323391));
#263918=CARTESIAN_POINT('Ctrl Pts',(-179.328730352575,-3.43118489787047,
135.624620025433));
#263919=CARTESIAN_POINT('Ctrl Pts',(-179.321322132908,-3.55956838662981,
135.533233348805));
#263920=CARTESIAN_POINT('Ctrl Pts',(-179.313913913242,-3.6842143372299,
135.4367738818));
#263921=CARTESIAN_POINT('Ctrl Pts',(-179.306505693575,-3.80471391970313,
135.335594726693));
#263922=CARTESIAN_POINT('Ctrl Pts',(-179.299092914273,-3.92528766765873,
135.234353297504));
#263923=CARTESIAN_POINT('Ctrl Pts',(-179.291680134971,-4.04170968684056,
135.128386642548));
#263924=CARTESIAN_POINT('Ctrl Pts',(-179.284267355669,-4.15360790265782,
135.018084855515));
#263925=CARTESIAN_POINT('Ctrl Pts',(-179.27684398464,-4.26566600389351,
134.907625464115));
#263926=CARTESIAN_POINT('Ctrl Pts',(-179.269420613611,-4.37318713756271,
134.792818841095));
#263927=CARTESIAN_POINT('Ctrl Pts',(-179.261997242582,-4.47583887241952,
134.674088896223));
#263928=CARTESIAN_POINT('Ctrl Pts',(-179.258061193142,-4.53026728532872,
134.611135430574));
#263929=CARTESIAN_POINT('Ctrl Pts',(-179.254125143702,-4.58332744336295,
134.547079486324));
#263930=CARTESIAN_POINT('Ctrl Pts',(-179.250189094261,-4.63497479752016,
134.481987459546));
#263931=CARTESIAN_POINT('Ctrl Pts',(-179.242405181676,-4.73711235857636,
134.35326177809));
#263932=CARTESIAN_POINT('Ctrl Pts',(-179.23462126909,-4.83405257557669,
134.220064488449));
#263933=CARTESIAN_POINT('Ctrl Pts',(-179.226837356504,-4.92538181691207,
134.082857913605));
#263934=CARTESIAN_POINT('Ctrl Pts',(-179.21943360423,-5.01225060826353,
133.952352402468));
#263935=CARTESIAN_POINT('Ctrl Pts',(-179.212029851955,-5.09404316262776,
133.818220254166));
#263936=CARTESIAN_POINT('Ctrl Pts',(-179.20462609968,-5.17044286712766,
133.680895185456));
#263937=CARTESIAN_POINT('Ctrl Pts',(-179.197229304088,-5.24677078525505,
133.543699149556));
#263938=CARTESIAN_POINT('Ctrl Pts',(-179.189832508496,-5.31771575753479,
133.403316488217));
#263939=CARTESIAN_POINT('Ctrl Pts',(-179.182435712904,-5.38300406071346,
133.260210337081));
#263940=CARTESIAN_POINT('Ctrl Pts',(-179.175044399858,-5.44824397184658,
133.117210257003));
#263941=CARTESIAN_POINT('Ctrl Pts',(-179.167653086811,-5.50783540530376,
132.971491044007));
#263942=CARTESIAN_POINT('Ctrl Pts',(-179.160261773764,-5.56155032784516,
132.82354077628));
#263943=CARTESIAN_POINT('Ctrl Pts',(-179.152874472875,-5.61523609281154,
132.67567081903));
#263944=CARTESIAN_POINT('Ctrl Pts',(-179.145487171987,-5.66305157103681,
132.525572568989));
#263945=CARTESIAN_POINT('Ctrl Pts',(-179.138099871098,-5.70481673901178,
132.373754302016));
#263946=CARTESIAN_POINT('Ctrl Pts',(-179.130714471695,-5.74657115666838,
132.221975112935));
#263947=CARTESIAN_POINT('Ctrl Pts',(-179.123329072291,-5.78227826278416,
132.068477147734));
#263948=CARTESIAN_POINT('Ctrl Pts',(-179.115943672887,-5.81180782512948,
131.913784056233));
#263949=CARTESIAN_POINT('Ctrl Pts',(-179.108559362774,-5.84133303208765,
131.759113780793));
#263950=CARTESIAN_POINT('Ctrl Pts',(-179.101175052661,-5.86468244308912,
131.603249097923));
#263951=CARTESIAN_POINT('Ctrl Pts',(-179.093790742548,-5.88177695426642,
131.446723772456));
#263952=CARTESIAN_POINT('Ctrl Pts',(-179.086404697669,-5.89887548138718,
131.290161675136));
#263953=CARTESIAN_POINT('Ctrl Pts',(-179.079018652791,-5.90971613497904,
131.132938997188));
#263954=CARTESIAN_POINT('Ctrl Pts',(-179.071632607912,-5.91427167588424,
130.975594686412));
#263955=CARTESIAN_POINT('Ctrl Pts',(-179.068880136011,-5.91596933661368,
130.916959002315));
#263956=CARTESIAN_POINT('Ctrl Pts',(-179.066127664109,-5.91679467625972,
130.858306445919));
#263957=CARTESIAN_POINT('Ctrl Pts',(-179.063375192208,-5.91674813668029,
130.799664918431));
#263958=CARTESIAN_POINT('',(-182.56337376072,-5.92087641190242,130.807755266905));
#263959=CARTESIAN_POINT('Ctrl Pts',(-182.56337265757,-5.92405711974599,
130.807733754196));
#263960=CARTESIAN_POINT('Ctrl Pts',(-182.479952757115,-5.91188579994225,
129.041809576944));
#263961=CARTESIAN_POINT('Ctrl Pts',(-182.303716982053,-4.13524844748988,
125.289854803609));
#263962=CARTESIAN_POINT('Ctrl Pts',(-182.034665332392,2.25108434336954,
124.177884947263));
#263963=CARTESIAN_POINT('Ctrl Pts',(-181.756217708577,6.79180772637146,
129.116489669186));
#263964=CARTESIAN_POINT('Ctrl Pts',(-181.477770084765,5.09119160707943,
135.60616533563));
#263965=CARTESIAN_POINT('Ctrl Pts',(-181.199322460952,-1.28798088058456,
137.683217047348));
#263966=CARTESIAN_POINT('Ctrl Pts',(-180.977858187196,-5.42030405385856,
134.307513343875));
#263967=CARTESIAN_POINT('Ctrl Pts',(-180.849209788043,-5.91302735279117,
131.571366059404));
#263968=CARTESIAN_POINT('Ctrl Pts',(-180.813377263496,-5.90898434920711,
130.80786452556));
#263969=CARTESIAN_POINT('',(-184.313376079986,-5.91869333543885,130.799262689142));
#263970=CARTESIAN_POINT('Ctrl Pts',(-184.313375192208,-5.91674778898835,
130.799245541667));
#263971=CARTESIAN_POINT('Ctrl Pts',(-184.30222306504,-5.91654340696533,
130.56283128179));
#263972=CARTESIAN_POINT('Ctrl Pts',(-184.291070937872,-5.90216644403423,
130.327006005632));
#263973=CARTESIAN_POINT('Ctrl Pts',(-184.279918810703,-5.87384581741895,
130.093118130302));
#263974=CARTESIAN_POINT('Ctrl Pts',(-184.274027981434,-5.85888616230683,
129.969572772447));
#263975=CARTESIAN_POINT('Ctrl Pts',(-184.268137152164,-5.84003663158251,
129.846567305077));
#263976=CARTESIAN_POINT('Ctrl Pts',(-184.262246322894,-5.81733560061832,
129.724297160042));
#263977=CARTESIAN_POINT('Ctrl Pts',(-184.254823056489,-5.78872913575387,
129.570219725698));
#263978=CARTESIAN_POINT('Ctrl Pts',(-184.247399790083,-5.75395386469645,
129.417046595923));
#263979=CARTESIAN_POINT('Ctrl Pts',(-184.239976523677,-5.71307757234325,
129.265310516079));
#263980=CARTESIAN_POINT('Ctrl Pts',(-184.232562030956,-5.67224959237304,
129.11375377568));
#263981=CARTESIAN_POINT('Ctrl Pts',(-184.225147538235,-5.6253350405974,
128.963631061319));
#263982=CARTESIAN_POINT('Ctrl Pts',(-184.217733045514,-5.5724530706871,
128.815467121803));
#263983=CARTESIAN_POINT('Ctrl Pts',(-184.21032569916,-5.51962207041052,
128.66744598827));
#263984=CARTESIAN_POINT('Ctrl Pts',(-184.202918352807,-5.46083522698721,
128.521380220278));
#263985=CARTESIAN_POINT('Ctrl Pts',(-184.195511006453,-5.39626204145504,
128.377781432282));
#263986=CARTESIAN_POINT('Ctrl Pts',(-184.188109184777,-5.33173701704084,
128.23428974568));
#263987=CARTESIAN_POINT('Ctrl Pts',(-184.180707363102,-5.26143439604173,
128.093261714445));
#263988=CARTESIAN_POINT('Ctrl Pts',(-184.173305541426,-5.18557248352986,
127.955190812069));
#263989=CARTESIAN_POINT('Ctrl Pts',(-184.165907627115,-5.1097506179311,
127.817192796247));
#263990=CARTESIAN_POINT('Ctrl Pts',(-184.158509712804,-5.02837548473259,
127.682149126725));
#263991=CARTESIAN_POINT('Ctrl Pts',(-184.151111798492,-4.94171214425669,
127.550530313785));
#263992=CARTESIAN_POINT('Ctrl Pts',(-184.14371511358,-4.85506320565538,
127.418933373503));
#263993=CARTESIAN_POINT('Ctrl Pts',(-184.136318428668,-4.76312800903145,
127.290760471687));
#263994=CARTESIAN_POINT('Ctrl Pts',(-184.128921743756,-4.66621597412815,
127.166454757694));
#263995=CARTESIAN_POINT('Ctrl Pts',(-184.12152538682,-4.56930823640603,
127.042154555547));
#263996=CARTESIAN_POINT('Ctrl Pts',(-184.114129029885,-4.46742432870891,
126.921721494671));
#263997=CARTESIAN_POINT('Ctrl Pts',(-184.106732672949,-4.36091497905957,
126.80556691097));
#263998=CARTESIAN_POINT('Ctrl Pts',(-184.099335183613,-4.25438932255719,
126.689394543706));
#263999=CARTESIAN_POINT('Ctrl Pts',(-184.091937694276,-4.14323706635495,
126.577502233055));
#264000=CARTESIAN_POINT('Ctrl Pts',(-184.084540204939,-4.02784681849153,
126.470265490637));
#264001=CARTESIAN_POINT('Ctrl Pts',(-184.077140122424,-3.91241612075543,
126.362991156545));
#264002=CARTESIAN_POINT('Ctrl Pts',(-184.069740039909,-3.79274474677175,
126.260375893956));
#264003=CARTESIAN_POINT('Ctrl Pts',(-184.062339957394,-3.66925535844911,
126.1627557575));
#264004=CARTESIAN_POINT('Ctrl Pts',(-184.054931737728,-3.54563018084883,
126.065028277668));
#264005=CARTESIAN_POINT('Ctrl Pts',(-184.047523518061,-3.41817889765681,
125.972307124804));
#264006=CARTESIAN_POINT('Ctrl Pts',(-184.040115298395,-3.28735479886558,
125.884886154895));
#264007=CARTESIAN_POINT('Ctrl Pts',(-184.032702519093,-3.15645018002447,
125.797411378838));
#264008=CARTESIAN_POINT('Ctrl Pts',(-184.025289739791,-3.02216892674676,
125.715243480416));
#264009=CARTESIAN_POINT('Ctrl Pts',(-184.017876960489,-2.88498957422633,
125.638630686655));
#264010=CARTESIAN_POINT('Ctrl Pts',(-184.01045358946,-2.74761421341414,
125.561908424942));
#264011=CARTESIAN_POINT('Ctrl Pts',(-184.003030218431,-2.60733281501413,
125.490757289058));
#264012=CARTESIAN_POINT('Ctrl Pts',(-183.995606847402,-2.46464530350015,
125.425377991601));
#264013=CARTESIAN_POINT('Ctrl Pts',(-183.991670797962,-2.38898896116109,
125.390712319337));
#264014=CARTESIAN_POINT('Ctrl Pts',(-183.987734748521,-2.31265646397017,
125.357668496352));
#264015=CARTESIAN_POINT('Ctrl Pts',(-183.983798699081,-2.23572401264854,
125.326270740449));
#264016=CARTESIAN_POINT('Ctrl Pts',(-183.976375432675,-2.09063181042523,
125.267055552704));
#264017=CARTESIAN_POINT('Ctrl Pts',(-183.96895216627,-1.94296603481777,
125.213519155027));
#264018=CARTESIAN_POINT('Ctrl Pts',(-183.961528899864,-1.79321153898064,
125.165892479945));
#264019=CARTESIAN_POINT('Ctrl Pts',(-183.954114407143,-1.64363404052125,
125.118322095638));
#264020=CARTESIAN_POINT('Ctrl Pts',(-183.946699914422,-1.49197308804768,
125.076647642673));
#264021=CARTESIAN_POINT('Ctrl Pts',(-183.939285421701,-1.33873457306213,
125.04105251324));
#264022=CARTESIAN_POINT('Ctrl Pts',(-183.931878075348,-1.18564375512665,
125.005491691733));
#264023=CARTESIAN_POINT('Ctrl Pts',(-183.924470728994,-1.03097876289946,
124.975998612581));
#264024=CARTESIAN_POINT('Ctrl Pts',(-183.91706338264,-0.875261651561804,
124.95270720987));
#264025=CARTESIAN_POINT('Ctrl Pts',(-183.909661560965,-0.71966067992065,
124.929433178765));
#264026=CARTESIAN_POINT('Ctrl Pts',(-183.902259739289,-0.563009519234663,
124.912351669202));
#264027=CARTESIAN_POINT('Ctrl Pts',(-183.894857917614,-0.405841341951333,
124.901545749415));
#264028=CARTESIAN_POINT('Ctrl Pts',(-183.887460003302,-0.248756132525396,
124.890745533989));
#264029=CARTESIAN_POINT('Ctrl Pts',(-183.880062088991,-0.091154821529368,
124.886214336211));
#264030=CARTESIAN_POINT('Ctrl Pts',(-183.87266417468,0.066423465832265,
124.887983475625));
#264031=CARTESIAN_POINT('Ctrl Pts',(-183.865267489768,0.223975566541075,
124.889752321039));
#264032=CARTESIAN_POINT('Ctrl Pts',(-183.857870804855,0.38150427830029,
124.89781942147));
#264033=CARTESIAN_POINT('Ctrl Pts',(-183.850474119943,0.538469518075691,
124.912163986376));
#264034=CARTESIAN_POINT('Ctrl Pts',(-183.843077763008,0.695427797847872,
124.92650791523));
#264035=CARTESIAN_POINT('Ctrl Pts',(-183.835681406072,0.851822283566282,
124.947128721133));
#264036=CARTESIAN_POINT('Ctrl Pts',(-183.828285049137,1.00711732962266,
124.97395366377));
#264037=CARTESIAN_POINT('Ctrl Pts',(-183.8208875598,1.16243615174704,125.000782713374));
#264038=CARTESIAN_POINT('Ctrl Pts',(-183.813490070464,1.31665483117389,
125.033817727484));
#264039=CARTESIAN_POINT('Ctrl Pts',(-183.806092581127,1.46924738720576,
125.072934732353));
#264040=CARTESIAN_POINT('Ctrl Pts',(-183.798692498612,1.6218934343218,125.112065449627));
#264041=CARTESIAN_POINT('Ctrl Pts',(-183.791292416097,1.77291186172737,
125.157282309882));
#264042=CARTESIAN_POINT('Ctrl Pts',(-183.783892333582,1.92179147805772,
125.20841136142));
#264043=CARTESIAN_POINT('Ctrl Pts',(-183.776484113915,2.07083480283121,
125.259596634606));
#264044=CARTESIAN_POINT('Ctrl Pts',(-183.769075894249,2.21773426647063,
125.316706960799));
#264045=CARTESIAN_POINT('Ctrl Pts',(-183.761667674582,2.3619976252977,125.379519810631));
#264046=CARTESIAN_POINT('Ctrl Pts',(-183.75425489528,2.50634977581538,125.442371320724));
#264047=CARTESIAN_POINT('Ctrl Pts',(-183.746842115978,2.64806225327137,
125.510932185989));
#264048=CARTESIAN_POINT('Ctrl Pts',(-183.739429336676,2.7866675572784,125.584933973986));
#264049=CARTESIAN_POINT('Ctrl Pts',(-183.732005965648,2.92547090704354,
125.659041499208));
#264050=CARTESIAN_POINT('Ctrl Pts',(-183.724582594619,3.06115789516633,
125.738605285748));
#264051=CARTESIAN_POINT('Ctrl Pts',(-183.71715922359,3.19328943506455,125.823313223051));
#264052=CARTESIAN_POINT('Ctrl Pts',(-183.713223174149,3.26334874797098,
125.868227403948));
#264053=CARTESIAN_POINT('Ctrl Pts',(-183.709287124708,3.33240903135922,
125.914587102222));
#264054=CARTESIAN_POINT('Ctrl Pts',(-183.705351075268,3.40040872175365,
125.962341298364));
#264055=CARTESIAN_POINT('Ctrl Pts',(-183.697927808862,3.52865401564075,
126.052404221932));
#264056=CARTESIAN_POINT('Ctrl Pts',(-183.690504542457,3.65351266188925,
126.147701890419));
#264057=CARTESIAN_POINT('Ctrl Pts',(-183.683081276051,3.77452829544996,
126.247951207806));
#264058=CARTESIAN_POINT('Ctrl Pts',(-183.67566678333,3.89540089858187,126.348082038826));
#264059=CARTESIAN_POINT('Ctrl Pts',(-183.668252290609,4.01243924548009,
126.453152633621));
#264060=CARTESIAN_POINT('Ctrl Pts',(-183.660837797888,4.12521559638735,
126.562836499301));
#264061=CARTESIAN_POINT('Ctrl Pts',(-183.653430451534,4.23788324920132,
126.672414647542));
#264062=CARTESIAN_POINT('Ctrl Pts',(-183.646023105181,4.34629681818062,
126.786596956152));
#264063=CARTESIAN_POINT('Ctrl Pts',(-183.638615758827,4.45006143720835,
126.905016599969));
#264064=CARTESIAN_POINT('Ctrl Pts',(-183.631213937151,4.55374866466839,
127.023347921947));
#264065=CARTESIAN_POINT('Ctrl Pts',(-183.623812115476,4.65279360120558,
127.145910006866));
#264066=CARTESIAN_POINT('Ctrl Pts',(-183.616410293801,4.74683816642942,
127.272299182054));
#264067=CARTESIAN_POINT('Ctrl Pts',(-183.609012379489,4.84083308625904,
127.398621637381));
#264068=CARTESIAN_POINT('Ctrl Pts',(-183.601614465178,4.92983266949919,
127.528766860743));
#264069=CARTESIAN_POINT('Ctrl Pts',(-183.594216550867,5.01351915578842,
127.662298199815));
#264070=CARTESIAN_POINT('Ctrl Pts',(-183.586819865954,5.09719173490199,
127.795807348402));
#264071=CARTESIAN_POINT('Ctrl Pts',(-183.579423181042,5.17555277139587,
127.932701179883));
#264072=CARTESIAN_POINT('Ctrl Pts',(-183.57202649613,5.24832782886879,128.072514069309));
#264073=CARTESIAN_POINT('Ctrl Pts',(-183.564630139194,5.32109965941941,
128.212320759286));
#264074=CARTESIAN_POINT('Ctrl Pts',(-183.557233782259,5.38828583108009,
128.355045918725));
#264075=CARTESIAN_POINT('Ctrl Pts',(-183.549837425324,5.44965801280331,
128.500199575888));
#264076=CARTESIAN_POINT('Ctrl Pts',(-183.542439935987,5.5110395907644,128.645375456446));
#264077=CARTESIAN_POINT('Ctrl Pts',(-183.53504244665,5.56660526102463,128.7929802312));
#264078=CARTESIAN_POINT('Ctrl Pts',(-183.527644957314,5.61617502079312,
128.942504366853));
#264079=CARTESIAN_POINT('Ctrl Pts',(-183.520244874799,5.665762157164,129.09208091796));
#264080=CARTESIAN_POINT('Ctrl Pts',(-183.512844792284,5.70934908086662,
129.243577815451));
#264081=CARTESIAN_POINT('Ctrl Pts',(-183.505444709769,5.74680583097126,
129.396470954412));
#264082=CARTESIAN_POINT('Ctrl Pts',(-183.498036490102,5.78430376862334,
129.549532215098));
#264083=CARTESIAN_POINT('Ctrl Pts',(-183.490628270436,5.81565798206432,
129.703992420572));
#264084=CARTESIAN_POINT('Ctrl Pts',(-183.483220050769,5.84078962182305,
129.859317149728));
#264085=CARTESIAN_POINT('Ctrl Pts',(-183.475807271467,5.8659367296867,130.014737478662));
#264086=CARTESIAN_POINT('Ctrl Pts',(-183.468394492165,5.88485358757889,
130.17102302182));
#264087=CARTESIAN_POINT('Ctrl Pts',(-183.460981712863,5.89751333993616,
130.327635363594));
#264088=CARTESIAN_POINT('Ctrl Pts',(-183.453558341834,5.91019118114126,
130.484471480425));
#264089=CARTESIAN_POINT('Ctrl Pts',(-183.446134970806,5.91659404558043,
130.641634956467));
#264090=CARTESIAN_POINT('Ctrl Pts',(-183.438711599777,5.91674718368156,
130.798587672361));
#264091=CARTESIAN_POINT('Ctrl Pts',(-183.434775550336,5.91682838117727,
130.881807768356));
#264092=CARTESIAN_POINT('Ctrl Pts',(-183.430839500895,5.9151534241066,130.964968689975));
#264093=CARTESIAN_POINT('Ctrl Pts',(-183.426903451455,5.91173196006602,
131.04799106483));
#264094=CARTESIAN_POINT('Ctrl Pts',(-183.419480185049,5.90527918566564,
131.204568672769));
#264095=CARTESIAN_POINT('Ctrl Pts',(-183.412056918644,5.8925917063369,131.36112650563));
#264096=CARTESIAN_POINT('Ctrl Pts',(-183.404633652238,5.87366102232141,
131.517127590259));
#264097=CARTESIAN_POINT('Ctrl Pts',(-183.397219159517,5.85475271280228,
131.672944294561));
#264098=CARTESIAN_POINT('Ctrl Pts',(-183.389804666796,5.82961593096655,
131.828205193483));
#264099=CARTESIAN_POINT('Ctrl Pts',(-183.382390174075,5.79829416074255,
131.982373940071));
#264100=CARTESIAN_POINT('Ctrl Pts',(-183.374982827722,5.76700257961994,
132.136394093016));
#264101=CARTESIAN_POINT('Ctrl Pts',(-183.367575481368,5.72953795175678,
132.289323825892));
#264102=CARTESIAN_POINT('Ctrl Pts',(-183.360168135014,5.68599546277168,
132.44063264869));
#264103=CARTESIAN_POINT('Ctrl Pts',(-183.352766313339,5.64248544941762,
132.59182861966));
#264104=CARTESIAN_POINT('Ctrl Pts',(-183.345364491663,5.59290670374262,
132.741405730511));
#264105=CARTESIAN_POINT('Ctrl Pts',(-183.337962669988,5.5374052957988,132.888844523131));
#264106=CARTESIAN_POINT('Ctrl Pts',(-183.330564755676,5.48193318661622,
133.03620548396));
#264107=CARTESIAN_POINT('Ctrl Pts',(-183.323166841365,5.42054477297452,
133.181430026141));
#264108=CARTESIAN_POINT('Ctrl Pts',(-183.315768927054,5.35343566560404,
133.324014787634));
#264109=CARTESIAN_POINT('Ctrl Pts',(-183.308372242142,5.28633771054982,
133.466575854126));
#264110=CARTESIAN_POINT('Ctrl Pts',(-183.300975557229,5.21352110739003,
133.606497673161));
#264111=CARTESIAN_POINT('Ctrl Pts',(-183.293578872317,5.13522926000215,
133.743297671965));
#264112=CARTESIAN_POINT('Ctrl Pts',(-183.286182515382,5.05694088415682,
133.880091604913));
#264113=CARTESIAN_POINT('Ctrl Pts',(-183.278786158446,4.97317793223063,
134.013763668875));
#264114=CARTESIAN_POINT('Ctrl Pts',(-183.271389801511,4.88422921281487,
134.143856920781));
#264115=CARTESIAN_POINT('Ctrl Pts',(-183.263992312174,4.7952668751231,134.273970090296));
#264116=CARTESIAN_POINT('Ctrl Pts',(-183.256594822838,4.70111739978136,
134.400503048588));
#264117=CARTESIAN_POINT('Ctrl Pts',(-183.249197333501,4.60211217567657,
134.523028939021));
#264118=CARTESIAN_POINT('Ctrl Pts',(-183.241797250986,4.50307224544381,
134.645597780714));
#264119=CARTESIAN_POINT('Ctrl Pts',(-183.234397168471,4.39917341190046,
134.764156467682));
#264120=CARTESIAN_POINT('Ctrl Pts',(-183.226997085956,4.29078637229727,
134.878312368607));
#264121=CARTESIAN_POINT('Ctrl Pts',(-183.219588866289,4.18228015000174,
134.99259379568));
#264122=CARTESIAN_POINT('Ctrl Pts',(-183.212180646623,4.06927612283048,
135.102462497404));
#264123=CARTESIAN_POINT('Ctrl Pts',(-183.204772426956,3.95218129433147,
135.207563267824));
#264124=CARTESIAN_POINT('Ctrl Pts',(-183.197359647654,3.83501439591901,
135.312728726014));
#264125=CARTESIAN_POINT('Ctrl Pts',(-183.189946868352,3.71375196598444,
135.413120167876));
#264126=CARTESIAN_POINT('Ctrl Pts',(-183.18253408905,3.58883247273898,135.508423972275));
#264127=CARTESIAN_POINT('Ctrl Pts',(-183.175110718021,3.46373448866361,
135.603863951219));
#264128=CARTESIAN_POINT('Ctrl Pts',(-183.167687346993,3.33496930979695,
135.694201560142));
#264129=CARTESIAN_POINT('Ctrl Pts',(-183.160263975964,3.20300331966732,
135.779167176288));
#264130=CARTESIAN_POINT('Ctrl Pts',(-183.156327926523,3.13303178521975,
135.82421798469));
#264131=CARTESIAN_POINT('Ctrl Pts',(-183.152391877082,3.06216079141112,
135.867759305324));
#264132=CARTESIAN_POINT('Ctrl Pts',(-183.148455827642,2.99046233124018,
135.90975635227));
#264133=CARTESIAN_POINT('Ctrl Pts',(-183.141032561236,2.85524127299102,
135.988961472127));
#264134=CARTESIAN_POINT('Ctrl Pts',(-183.133609294831,2.71666684177059,
136.062910469239));
#264135=CARTESIAN_POINT('Ctrl Pts',(-183.126186028425,2.57518621397406,
136.131305945412));
#264136=CARTESIAN_POINT('Ctrl Pts',(-183.118771535704,2.43387280453034,
136.199620583812));
#264137=CARTESIAN_POINT('Ctrl Pts',(-183.111357042983,2.28966036846826,
136.262394605668));
#264138=CARTESIAN_POINT('Ctrl Pts',(-183.103942550262,2.14302365379594,
136.319374686612));
#264139=CARTESIAN_POINT('Ctrl Pts',(-183.096535203909,1.99652827310958,
136.376299848008));
#264140=CARTESIAN_POINT('Ctrl Pts',(-183.089127857555,1.84761361116126,
136.427442051669));
#264141=CARTESIAN_POINT('Ctrl Pts',(-183.081720511201,1.69677743437165,
136.472594637145));
#264142=CARTESIAN_POINT('Ctrl Pts',(-183.074318689525,1.54605375689342,
136.517713546118));
#264143=CARTESIAN_POINT('Ctrl Pts',(-183.06691686785,1.39341177422502,136.556851625278));
#264144=CARTESIAN_POINT('Ctrl Pts',(-183.059515046175,1.23936747561927,
136.589850987697));
#264145=CARTESIAN_POINT('Ctrl Pts',(-183.052117131863,1.08540449579967,
136.622832930009));
#264146=CARTESIAN_POINT('Ctrl Pts',(-183.044719217552,0.930041038421735,
136.649682531358));
#264147=CARTESIAN_POINT('Ctrl Pts',(-183.037321303241,0.773806328602494,
136.670292285112));
#264148=CARTESIAN_POINT('Ctrl Pts',(-183.029924618328,0.617597582157862,
136.690898613898));
#264149=CARTESIAN_POINT('Ctrl Pts',(-183.022527933416,0.460518240359305,
136.705267104356));
#264150=CARTESIAN_POINT('Ctrl Pts',(-183.015131248504,0.303105871090587,
136.713341696687));
#264151=CARTESIAN_POINT('Ctrl Pts',(-183.007734891569,0.145700481651279,
136.721415930983));
#264152=CARTESIAN_POINT('Ctrl Pts',(-183.000338534633,-0.012037533089414,
136.72319680293));
#264153=CARTESIAN_POINT('Ctrl Pts',(-182.992942177698,-0.169567625887687,
136.718680306486));
#264154=CARTESIAN_POINT('Ctrl Pts',(-182.985544688361,-0.327121836945322,
136.714163118556));
#264155=CARTESIAN_POINT('Ctrl Pts',(-182.978147199025,-0.484467689507502,
136.703346653195));
#264156=CARTESIAN_POINT('Ctrl Pts',(-182.970749709688,-0.641066933207348,
136.686278990822));
#264157=CARTESIAN_POINT('Ctrl Pts',(-182.963349627173,-0.797721072529536,
136.669205345406));
#264158=CARTESIAN_POINT('Ctrl Pts',(-182.955949544658,-0.953627711032837,
136.645876180442));
#264159=CARTESIAN_POINT('Ctrl Pts',(-182.948549462143,-1.10825614594989,
136.616391147206));
#264160=CARTESIAN_POINT('Ctrl Pts',(-182.941141242476,-1.26305461072711,
136.586873692145));
#264161=CARTESIAN_POINT('Ctrl Pts',(-182.93373302281,-1.41657169809388,
136.551186920619));
#264162=CARTESIAN_POINT('Ctrl Pts',(-182.926324803144,-1.56828856786049,
136.509481258746));
#264163=CARTESIAN_POINT('Ctrl Pts',(-182.918912023842,-1.7200988168289,
136.467749927734));
#264164=CARTESIAN_POINT('Ctrl Pts',(-182.911499244539,-1.8701062854791,
136.419992437623));
#264165=CARTESIAN_POINT('Ctrl Pts',(-182.904086465237,-2.01781011269092,
136.366408164254));
#264166=CARTESIAN_POINT('Ctrl Pts',(-182.896663094209,-2.1657249860579,
136.312747327163));
#264167=CARTESIAN_POINT('Ctrl Pts',(-182.88923972318,-2.31132929938075,
136.253243219605));
#264168=CARTESIAN_POINT('Ctrl Pts',(-182.881816352151,-2.45414411970913,
136.188142485565));
#264169=CARTESIAN_POINT('Ctrl Pts',(-182.87788030271,-2.52986796424262,
136.153624514306));
#264170=CARTESIAN_POINT('Ctrl Pts',(-182.873944253269,-2.60480801371997,
136.117533887402));
#264171=CARTESIAN_POINT('Ctrl Pts',(-182.870008203829,-2.67889608778898,
136.079912371964));
#264172=CARTESIAN_POINT('Ctrl Pts',(-182.862584937423,-2.81862388327062,
136.008959367975));
#264173=CARTESIAN_POINT('Ctrl Pts',(-182.855161671018,-2.95574213382726,
135.932344013602));
#264174=CARTESIAN_POINT('Ctrl Pts',(-182.847738404613,-3.08975892017157,
135.850281780022));
#264175=CARTESIAN_POINT('Ctrl Pts',(-182.840323911892,-3.22361730980421,
135.768316537187));
#264176=CARTESIAN_POINT('Ctrl Pts',(-182.832909419171,-3.35438121652008,
135.680917422574));
#264177=CARTESIAN_POINT('Ctrl Pts',(-182.82549492645,-3.48158089845803,
135.588346927119));
#264178=CARTESIAN_POINT('Ctrl Pts',(-182.818087580096,-3.60865798055354,
135.495865654593));
#264179=CARTESIAN_POINT('Ctrl Pts',(-182.810680233742,-3.7321773771412,
135.398223142311));
#264180=CARTESIAN_POINT('Ctrl Pts',(-182.803272887389,-3.85169616402163,
135.295726470239));
#264181=CARTESIAN_POINT('Ctrl Pts',(-182.795871065713,-3.97112580928161,
135.193306244053));
#264182=CARTESIAN_POINT('Ctrl Pts',(-182.788469244038,-4.08656050384569,
135.086039308776));
#264183=CARTESIAN_POINT('Ctrl Pts',(-182.781067422363,-4.19758850817627,
134.974274439041));
#264184=CARTESIAN_POINT('Ctrl Pts',(-182.773669508051,-4.30855790168761,
134.86256856911));
#264185=CARTESIAN_POINT('Ctrl Pts',(-182.76627159374,-4.4151249753976,134.746369757665));
#264186=CARTESIAN_POINT('Ctrl Pts',(-182.758873679429,-4.51691322183099,
134.626065146824));
#264187=CARTESIAN_POINT('Ctrl Pts',(-182.751476994517,-4.61868455290431,
134.505780528426));
#264188=CARTESIAN_POINT('Ctrl Pts',(-182.744080309604,-4.71567839198069,
134.381391749517));
#264189=CARTESIAN_POINT('Ctrl Pts',(-182.736683624692,-4.80755700579362,
134.253320779491));
#264190=CARTESIAN_POINT('Ctrl Pts',(-182.729287267757,-4.89943154561279,
134.125255488265));
#264191=CARTESIAN_POINT('Ctrl Pts',(-182.721890910821,-4.98619109355161,
133.993508633881));
#264192=CARTESIAN_POINT('Ctrl Pts',(-182.714494553886,-5.06754010022365,
133.858532828677));
#264193=CARTESIAN_POINT('Ctrl Pts',(-182.70709706455,-5.14890156163604,
133.723536358334));
#264194=CARTESIAN_POINT('Ctrl Pts',(-182.699699575213,-5.22485063968611,
133.585310272575));
#264195=CARTESIAN_POINT('Ctrl Pts',(-182.692302085877,-5.29513684831921,
133.444333405318));
#264196=CARTESIAN_POINT('Ctrl Pts',(-182.684902003362,-5.36544769567369,
133.303307118839));
#264197=CARTESIAN_POINT('Ctrl Pts',(-182.677501920847,-5.43009155481507,
133.159528464853));
#264198=CARTESIAN_POINT('Ctrl Pts',(-182.670101838332,-5.48886540737634,
133.013497802579));
#264199=CARTESIAN_POINT('Ctrl Pts',(-182.662693618666,-5.54770388783085,
132.867306564579));
#264200=CARTESIAN_POINT('Ctrl Pts',(-182.655285398999,-5.6006593318303,
132.718858719442));
#264201=CARTESIAN_POINT('Ctrl Pts',(-182.647877179333,-5.6475778513308,
132.568672091104));
#264202=CARTESIAN_POINT('Ctrl Pts',(-182.640464400031,-5.69452524839718,
132.418393025403));
#264203=CARTESIAN_POINT('Ctrl Pts',(-182.633051620729,-5.73542822034687,
132.26637340365));
#264204=CARTESIAN_POINT('Ctrl Pts',(-182.625638841427,-5.77018378005181,
132.113142382005));
#264205=CARTESIAN_POINT('Ctrl Pts',(-182.618215470398,-5.80498900013038,
131.959692416689));
#264206=CARTESIAN_POINT('Ctrl Pts',(-182.61079209937,-5.83362919713295,
131.80502796056));
#264207=CARTESIAN_POINT('Ctrl Pts',(-182.603368728341,-5.85605300467136,
131.649685270572));
#264208=CARTESIAN_POINT('Ctrl Pts',(-182.5994326789,-5.86794264548235,131.567318848928));
#264209=CARTESIAN_POINT('Ctrl Pts',(-182.595496629458,-5.87808550618547,
131.484761797472));
#264210=CARTESIAN_POINT('Ctrl Pts',(-182.591560580017,-5.88647987348797,
131.40209405441));
#264211=CARTESIAN_POINT('Ctrl Pts',(-182.582165450747,-5.90651675745441,
131.204770788007));
#264212=CARTESIAN_POINT('Ctrl Pts',(-182.572770321477,-5.91663410596626,
131.006423364004));
#264213=CARTESIAN_POINT('Ctrl Pts',(-182.563375192208,-5.91674901010249,
130.807783182575));
#264214=CARTESIAN_POINT('',(-186.063375192208,-5.90709598019638,130.803332506185));
#264215=CARTESIAN_POINT('Ctrl Pts',(-186.063375192208,-5.90709598019638,
130.803332506185));
#264216=CARTESIAN_POINT('Ctrl Pts',(-186.019894150062,-5.90852920600748,
129.876120039144));
#264217=CARTESIAN_POINT('Ctrl Pts',(-185.883597233311,-5.26549744303905,
126.971533866971));
#264218=CARTESIAN_POINT('Ctrl Pts',(-185.654484441958,-0.717600748298859,
123.842851463917));
#264219=CARTESIAN_POINT('Ctrl Pts',(-185.376036818144,5.46903407832205,
126.437757042646));
#264220=CARTESIAN_POINT('Ctrl Pts',(-185.097589194332,6.62989376413611,
133.045357986287));
#264221=CARTESIAN_POINT('Ctrl Pts',(-184.819141570519,1.69820496902565,
137.593591826879));
#264222=CARTESIAN_POINT('Ctrl Pts',(-184.557737350984,-4.39666896695656,
136.006341653894));
#264223=CARTESIAN_POINT('Ctrl Pts',(-184.389149006053,-5.90500976629783,
132.406387652391));
#264224=CARTESIAN_POINT('Ctrl Pts',(-184.313376535726,-5.91969208008458,
130.799271491783));
#264225=CARTESIAN_POINT('',(-187.813375192208,-5.91590714834001,130.809830359851));
#264226=CARTESIAN_POINT('Ctrl Pts',(-187.813375192208,-5.91590714834001,
130.809830359851));
#264227=CARTESIAN_POINT('Ctrl Pts',(-187.743456064355,-5.90233112363404,
129.324427893846));
#264228=CARTESIAN_POINT('Ctrl Pts',(-187.580721061896,-4.58174601807203,
125.845682237925));
#264229=CARTESIAN_POINT('Ctrl Pts',(-187.325170184835,1.26703804199676,
123.92161587942));
#264230=CARTESIAN_POINT('Ctrl Pts',(-187.046722561023,6.47551308848548,
128.150063955324));
#264231=CARTESIAN_POINT('Ctrl Pts',(-186.768274937209,5.73330795305963,
134.817680994228));
#264232=CARTESIAN_POINT('Ctrl Pts',(-186.489827313397,-0.277527103565456,
137.797252668579));
#264233=CARTESIAN_POINT('Ctrl Pts',(-186.254860731729,-5.1345300677341,
134.88889554915));
#264234=CARTESIAN_POINT('Ctrl Pts',(-186.112710024666,-5.90546980125088,
131.855374257204));
#264235=CARTESIAN_POINT('Ctrl Pts',(-186.063375192208,-5.90709598019638,
130.803332506185));
#264236=CARTESIAN_POINT('',(-189.563375998339,-5.92191640313042,130.80298505409));
#264237=CARTESIAN_POINT('Ctrl Pts',(-189.563375192208,-5.91674983639772,
130.802969219882));
#264238=CARTESIAN_POINT('Ctrl Pts',(-189.559833853251,-5.91673225127943,
130.728190637922));
#264239=CARTESIAN_POINT('Ctrl Pts',(-189.556292514295,-5.91529709555501,
130.653430419199));
#264240=CARTESIAN_POINT('Ctrl Pts',(-189.552751175338,-5.91244610460354,
130.578724577319));
#264241=CARTESIAN_POINT('Ctrl Pts',(-189.545327908933,-5.90646992847011,
130.42212805461));
#264242=CARTESIAN_POINT('Ctrl Pts',(-189.537904642528,-5.89425901609847,
130.265532330591));
#264243=CARTESIAN_POINT('Ctrl Pts',(-189.530481376122,-5.87580323340804,
130.109474350058));
#264244=CARTESIAN_POINT('Ctrl Pts',(-189.523066883401,-5.85736926392009,
129.953600817098));
#264245=CARTESIAN_POINT('Ctrl Pts',(-189.51565239068,-5.832705159285,129.798264129616));
#264246=CARTESIAN_POINT('Ctrl Pts',(-189.508237897959,-5.80185277077408,
129.644000764434));
#264247=CARTESIAN_POINT('Ctrl Pts',(-189.500830551605,-5.77103011895677,
129.48988608409));
#264248=CARTESIAN_POINT('Ctrl Pts',(-189.493423205251,-5.73403113012844,
129.336843030134));
#264249=CARTESIAN_POINT('Ctrl Pts',(-189.486015858898,-5.69094937483769,
129.18540237983));
#264250=CARTESIAN_POINT('Ctrl Pts',(-189.478614037222,-5.64789975154543,
129.034074679676));
#264251=CARTESIAN_POINT('Ctrl Pts',(-189.471212215547,-5.59877649678882,
128.884347361008));
#264252=CARTESIAN_POINT('Ctrl Pts',(-189.463810393871,-5.54372409889164,
128.73674032412));
#264253=CARTESIAN_POINT('Ctrl Pts',(-189.45641247956,-5.48870076272677,
128.589211207839));
#264254=CARTESIAN_POINT('Ctrl Pts',(-189.449014565249,-5.42775464698324,
128.443800493114));
#264255=CARTESIAN_POINT('Ctrl Pts',(-189.441616650937,-5.36107982942442,
128.301012135025));
#264256=CARTESIAN_POINT('Ctrl Pts',(-189.434219966025,-5.29441609201077,
128.158247505772));
#264257=CARTESIAN_POINT('Ctrl Pts',(-189.426823281113,-5.22202570001855,
128.018104706153));
#264258=CARTESIAN_POINT('Ctrl Pts',(-189.419426596201,-5.14415058741227,
127.881067047545));
#264259=CARTESIAN_POINT('Ctrl Pts',(-189.412030239265,-5.06627892787009,
127.744035465331));
#264260=CARTESIAN_POINT('Ctrl Pts',(-189.40463388233,-4.98292321570959,
127.610109074916));
#264261=CARTESIAN_POINT('Ctrl Pts',(-189.397237525395,-4.89437086740681,
127.479745696289));
#264262=CARTESIAN_POINT('Ctrl Pts',(-189.389840036058,-4.80580496151345,
127.349362358695));
#264263=CARTESIAN_POINT('Ctrl Pts',(-189.382442546721,-4.71204104506515,
127.222543427878));
#264264=CARTESIAN_POINT('Ctrl Pts',(-189.375045057385,-4.61340920620913,
127.099716767131));
#264265=CARTESIAN_POINT('Ctrl Pts',(-189.36764497487,-4.51474279211475,
126.976847049689));
#264266=CARTESIAN_POINT('Ctrl Pts',(-189.360244892355,-4.41120529168435,
126.857972679567));
#264267=CARTESIAN_POINT('Ctrl Pts',(-189.35284480984,-4.30316620541695,
126.74348741454));
#264268=CARTESIAN_POINT('Ctrl Pts',(-189.345436590173,-4.19500831906767,
126.628876261194));
#264269=CARTESIAN_POINT('Ctrl Pts',(-189.338028370507,-4.08233921785816,
126.518664122988));
#264270=CARTESIAN_POINT('Ctrl Pts',(-189.33062015084,-3.96556482232641,
126.413207443008));
#264271=CARTESIAN_POINT('Ctrl Pts',(-189.323207371538,-3.84871855410236,
126.307685856202));
#264272=CARTESIAN_POINT('Ctrl Pts',(-189.315794592236,-3.72776224286292,
126.206925798223));
#264273=CARTESIAN_POINT('Ctrl Pts',(-189.308381812934,-3.6031334002335,
126.111242223297));
#264274=CARTESIAN_POINT('Ctrl Pts',(-189.300958441905,-3.4783264820694,
126.015421931193));
#264275=CARTESIAN_POINT('Ctrl Pts',(-189.293535070877,-3.349836856241,125.924692823797));
#264276=CARTESIAN_POINT('Ctrl Pts',(-189.286111699848,-3.21813008347746,
125.839325942126));
#264277=CARTESIAN_POINT('Ctrl Pts',(-189.282175650407,-3.14829599229798,
125.794062373115));
#264278=CARTESIAN_POINT('Ctrl Pts',(-189.278239600966,-3.07755785156217,
125.750305547236));
#264279=CARTESIAN_POINT('Ctrl Pts',(-189.274303551526,-3.00598754805893,
125.708090469368));
#264280=CARTESIAN_POINT('Ctrl Pts',(-189.26688028512,-2.8710081892836,125.628474149996));
#264281=CARTESIAN_POINT('Ctrl Pts',(-189.259457018715,-2.73265947523997,
125.55410372251));
#264282=CARTESIAN_POINT('Ctrl Pts',(-189.252033752309,-2.59138767507411,
125.485277944776));
#264283=CARTESIAN_POINT('Ctrl Pts',(-189.244619259588,-2.45028284644415,
125.416533513396));
#264284=CARTESIAN_POINT('Ctrl Pts',(-189.237204766867,-2.30626214089305,
125.353320849256));
#264285=CARTESIAN_POINT('Ctrl Pts',(-189.229790274146,-2.15979953319767,
125.295894720522));
#264286=CARTESIAN_POINT('Ctrl Pts',(-189.222382927793,-2.01347809167781,
125.238523941253));
#264287=CARTESIAN_POINT('Ctrl Pts',(-189.214975581439,-1.86471977876785,
125.186928729472));
#264288=CARTESIAN_POINT('Ctrl Pts',(-189.207568235085,-1.71402172957951,
125.141317259704));
#264289=CARTESIAN_POINT('Ctrl Pts',(-189.20016641341,-1.56343607668177,
125.09573980869));
#264290=CARTESIAN_POINT('Ctrl Pts',(-189.192764591734,-1.4109139238907,
125.056137321127));
#264291=CARTESIAN_POINT('Ctrl Pts',(-189.185362770059,-1.25697077751556,
125.022669253703));
#264292=CARTESIAN_POINT('Ctrl Pts',(-189.177964855747,-1.10310889652911,
124.989218853811));
#264293=CARTESIAN_POINT('Ctrl Pts',(-189.170566941436,-0.94782787973478,
124.961896503906));
#264294=CARTESIAN_POINT('Ctrl Pts',(-189.163169027125,-0.791656622585064,
124.940811320901));
#264295=CARTESIAN_POINT('Ctrl Pts',(-189.155772342213,-0.635511318265274,
124.919729641871));
#264296=CARTESIAN_POINT('Ctrl Pts',(-189.1483756573,-0.478476436789943,
124.904883122484));
#264297=CARTESIAN_POINT('Ctrl Pts',(-189.140978972388,-0.321089372926129,
124.896329458449));
#264298=CARTESIAN_POINT('Ctrl Pts',(-189.133582615453,-0.163709287769656,
124.887776173693));
#264299=CARTESIAN_POINT('Ctrl Pts',(-189.126186258517,-0.00597742402233353,
124.885515209737));
#264300=CARTESIAN_POINT('Ctrl Pts',(-189.118789901582,0.151565685768833,
124.889552217846));
#264301=CARTESIAN_POINT('Ctrl Pts',(-189.111392412245,0.309132915812747,
124.893589844031));
#264302=CARTESIAN_POINT('Ctrl Pts',(-189.103994922909,0.466510961159943,
124.90392735264));
#264303=CARTESIAN_POINT('Ctrl Pts',(-189.096597433572,0.623161427596432,
124.920518301727));
#264304=CARTESIAN_POINT('Ctrl Pts',(-189.089197351057,0.779866807610867,
124.937115066746));
#264305=CARTESIAN_POINT('Ctrl Pts',(-189.081797268542,0.935843729918489,
124.959969597473));
#264306=CARTESIAN_POINT('Ctrl Pts',(-189.074397186027,1.09056119090591,
124.988983858371));
#264307=CARTESIAN_POINT('Ctrl Pts',(-189.06698896636,1.24544877964724,125.018030023431));
#264308=CARTESIAN_POINT('Ctrl Pts',(-189.059580746694,1.39907377419055,
125.053249376451));
#264309=CARTESIAN_POINT('Ctrl Pts',(-189.052172527027,1.55091687890397,
125.094493071184));
#264310=CARTESIAN_POINT('Ctrl Pts',(-189.044759747725,1.7028534405147,125.135762150722));
#264311=CARTESIAN_POINT('Ctrl Pts',(-189.037346968423,1.85300557171295,
125.183062848489));
#264312=CARTESIAN_POINT('Ctrl Pts',(-189.029934189121,2.00087180686703,
125.236197314017));
#264313=CARTESIAN_POINT('Ctrl Pts',(-189.022510818092,2.14894932023193,
125.289407700562));
#264314=CARTESIAN_POINT('Ctrl Pts',(-189.015087447064,2.29473406916035,
125.348468363057));
#264315=CARTESIAN_POINT('Ctrl Pts',(-189.007664076035,2.43774637222091,
125.413134116368));
#264316=CARTESIAN_POINT('Ctrl Pts',(-189.003728026594,2.5135749268355,125.447421450406));
#264317=CARTESIAN_POINT('Ctrl Pts',(-188.999791977153,2.58862447664729,
125.483283818407));
#264318=CARTESIAN_POINT('Ctrl Pts',(-188.995855927713,2.66282671449517,
125.520679660972));
#264319=CARTESIAN_POINT('Ctrl Pts',(-188.988432661307,2.80276981930618,
125.591207052967));
#264320=CARTESIAN_POINT('Ctrl Pts',(-188.981009394902,2.94012062552616,
125.667404711676));
#264321=CARTESIAN_POINT('Ctrl Pts',(-188.973586128496,3.07438656032618,
125.749058664153));
#264322=CARTESIAN_POINT('Ctrl Pts',(-188.966171635775,3.20849380394173,
125.830616108438));
#264323=CARTESIAN_POINT('Ctrl Pts',(-188.958757143054,3.33952311781041,
125.917616817874));
#264324=CARTESIAN_POINT('Ctrl Pts',(-188.951342650333,3.46700396331473,
126.009799732473));
#264325=CARTESIAN_POINT('Ctrl Pts',(-188.943935303979,3.59436193798021,
126.101893797708));
#264326=CARTESIAN_POINT('Ctrl Pts',(-188.936527957626,3.71817795265517,
126.199159907163));
#264327=CARTESIAN_POINT('Ctrl Pts',(-188.929120611272,3.83800815054602,
126.301292330404));
#264328=CARTESIAN_POINT('Ctrl Pts',(-188.921718789596,3.95774897455468,
126.403348579431));
#264329=CARTESIAN_POINT('Ctrl Pts',(-188.914316967921,4.07350961808697,
126.510263674354));
#264330=CARTESIAN_POINT('Ctrl Pts',(-188.906915146246,4.1848772819624,126.62169009535));
#264331=CARTESIAN_POINT('Ctrl Pts',(-188.899517231934,4.29618615571496,
126.733057695206));
#264332=CARTESIAN_POINT('Ctrl Pts',(-188.892119317623,4.40310640502578,
126.848931614914));
#264333=CARTESIAN_POINT('Ctrl Pts',(-188.884721403311,4.50526034583612,
126.968925860105));
#264334=CARTESIAN_POINT('Ctrl Pts',(-188.877324718399,4.60739731051461,
127.08890016443));
#264335=CARTESIAN_POINT('Ctrl Pts',(-188.869928033487,4.70476929697789,
127.2129931513));
#264336=CARTESIAN_POINT('Ctrl Pts',(-188.862531348575,4.79703728919411,
127.340783881217));
#264337=CARTESIAN_POINT('Ctrl Pts',(-188.855134991639,4.88930119015086,
127.468568944758));
#264338=CARTESIAN_POINT('Ctrl Pts',(-188.847738634704,4.97646132833132,
127.600051122683));
#264339=CARTESIAN_POINT('Ctrl Pts',(-188.840342277768,5.05822077812171,
127.734778704295));
#264340=CARTESIAN_POINT('Ctrl Pts',(-188.832944788432,5.13999274549259,
127.869526913045));
#264341=CARTESIAN_POINT('Ctrl Pts',(-188.825547299095,5.21636218440918,
128.007521195684));
#264342=CARTESIAN_POINT('Ctrl Pts',(-188.818149809759,5.28707715257132,
128.148283482907));
#264343=CARTESIAN_POINT('Ctrl Pts',(-188.810749727244,5.35781690975603,
128.289095114132));
#264344=CARTESIAN_POINT('Ctrl Pts',(-188.803349644729,5.42289808223647,
128.432676348477));
#264345=CARTESIAN_POINT('Ctrl Pts',(-188.795949562214,5.48211612966465,
128.57852744696));
#264346=CARTESIAN_POINT('Ctrl Pts',(-188.788541342547,5.54139929342365,
128.724538923719));
#264347=CARTESIAN_POINT('Ctrl Pts',(-188.781133122881,5.59480631631315,
128.872824903103));
#264348=CARTESIAN_POINT('Ctrl Pts',(-188.773724903214,5.64218173492415,
129.022868031955));
#264349=CARTESIAN_POINT('Ctrl Pts',(-188.766312123912,5.68958631231479,
129.173003509849));
#264350=CARTESIAN_POINT('Ctrl Pts',(-188.75889934461,5.73095179023987,129.324897932882));
#264351=CARTESIAN_POINT('Ctrl Pts',(-188.751486565308,5.76617357147899,
129.478022460806));
#264352=CARTESIAN_POINT('Ctrl Pts',(-188.744063194279,5.80144567925094,
129.631365780237));
#264353=CARTESIAN_POINT('Ctrl Pts',(-188.73663982325,5.83055648899496,129.785942349065));
#264354=CARTESIAN_POINT('Ctrl Pts',(-188.729216452221,5.85345300237912,
129.941216069162));
#264355=CARTESIAN_POINT('Ctrl Pts',(-188.725280402781,5.86559328316901,
130.023545921295));
#264356=CARTESIAN_POINT('Ctrl Pts',(-188.72134435334,5.8759873721544,130.106071718954));
#264357=CARTESIAN_POINT('Ctrl Pts',(-188.7174083039,5.88463331274603,130.18871352952));
#264358=CARTESIAN_POINT('Ctrl Pts',(-188.709985037494,5.90093928687214,
130.344573405092));
#264359=CARTESIAN_POINT('Ctrl Pts',(-188.702561771089,5.91107350431225,
130.501317224105));
#264360=CARTESIAN_POINT('Ctrl Pts',(-188.695138504683,5.91494973892084,
130.658414913483));
#264361=CARTESIAN_POINT('Ctrl Pts',(-188.687724011962,5.91882139214203,
130.815326926438));
#264362=CARTESIAN_POINT('Ctrl Pts',(-188.680309519241,5.91644977602051,
130.972591607699));
#264363=CARTESIAN_POINT('Ctrl Pts',(-188.67289502652,5.90780019010058,131.1296719705));
#264364=CARTESIAN_POINT('Ctrl Pts',(-188.665487680167,5.89915894097722,
131.286600933333));
#264365=CARTESIAN_POINT('Ctrl Pts',(-188.658080333813,5.88425178867966,
131.443345561147));
#264366=CARTESIAN_POINT('Ctrl Pts',(-188.650672987459,5.86309603744215,
131.599367169885));
#264367=CARTESIAN_POINT('Ctrl Pts',(-188.643271165784,5.84195606496208,
131.75527241182));
#264368=CARTESIAN_POINT('Ctrl Pts',(-188.635869344108,5.81457682305113,
131.910455340087));
#264369=CARTESIAN_POINT('Ctrl Pts',(-188.628467522433,5.78102756193813,
132.064380812091));
#264370=CARTESIAN_POINT('Ctrl Pts',(-188.621069608122,5.74749601121893,
132.218225028037));
#264371=CARTESIAN_POINT('Ctrl Pts',(-188.61367169381,5.70780100727417,132.3708127459));
#264372=CARTESIAN_POINT('Ctrl Pts',(-188.606273779499,5.66206315063794,
132.521617570001));
#264373=CARTESIAN_POINT('Ctrl Pts',(-188.598877094587,5.61633289480377,
132.672397333077));
#264374=CARTESIAN_POINT('Ctrl Pts',(-188.591480409675,5.56456188758136,
132.821394433549));
#264375=CARTESIAN_POINT('Ctrl Pts',(-188.584083724762,5.50692103084546,
132.968096119547));
#264376=CARTESIAN_POINT('Ctrl Pts',(-188.576687367827,5.44928272996555,
133.114791300639));
#264377=CARTESIAN_POINT('Ctrl Pts',(-188.569291010892,5.38577523360099,
133.259190922191));
#264378=CARTESIAN_POINT('Ctrl Pts',(-188.561894653956,5.3166180832047,133.400801011613));
#264379=CARTESIAN_POINT('Ctrl Pts',(-188.55449716462,5.24745034467193,133.542432781902));
#264380=CARTESIAN_POINT('Ctrl Pts',(-188.547099675283,5.17263139364863,
133.681273834221));
#264381=CARTESIAN_POINT('Ctrl Pts',(-188.539702185946,5.09242726241424,
133.816853794242));
#264382=CARTESIAN_POINT('Ctrl Pts',(-188.532302103431,5.0121950157461,133.952481281607));
#264383=CARTESIAN_POINT('Ctrl Pts',(-188.524902020916,4.92657402028228,
134.084845079539));
#264384=CARTESIAN_POINT('Ctrl Pts',(-188.517501938401,4.83587416152764,
134.213502981324));
#264385=CARTESIAN_POINT('Ctrl Pts',(-188.510093718735,4.74507456895399,
134.342302355698));
#264386=CARTESIAN_POINT('Ctrl Pts',(-188.502685499068,4.64918517523304,
134.467387390564));
#264387=CARTESIAN_POINT('Ctrl Pts',(-188.495277279402,4.54855721245665,
134.588347648134));
#264388=CARTESIAN_POINT('Ctrl Pts',(-188.4878645001,4.44786731484825,134.709382354725));
#264389=CARTESIAN_POINT('Ctrl Pts',(-188.480451720798,4.34243328610366,
134.826286948712));
#264390=CARTESIAN_POINT('Ctrl Pts',(-188.473038941496,4.23264351714947,
134.938687578419));
#264391=CARTESIAN_POINT('Ctrl Pts',(-188.465615570467,4.12269687542492,
135.051248811416));
#264392=CARTESIAN_POINT('Ctrl Pts',(-188.458192199438,4.00838233397257,
135.159292971309));
#264393=CARTESIAN_POINT('Ctrl Pts',(-188.45076882841,3.89012228043788,135.262485694966));
#264394=CARTESIAN_POINT('Ctrl Pts',(-188.446832778969,3.82741796243955,
135.317200953127));
#264395=CARTESIAN_POINT('Ctrl Pts',(-188.442896729528,3.76360493059685,
135.370553004011));
#264396=CARTESIAN_POINT('Ctrl Pts',(-188.438960680087,3.69874937690234,
135.422496995951));
#264397=CARTESIAN_POINT('Ctrl Pts',(-188.431537413681,3.57643382671275,
135.520461743629));
#264398=CARTESIAN_POINT('Ctrl Pts',(-188.424114147276,3.45003860462953,
135.613711810634));
#264399=CARTESIAN_POINT('Ctrl Pts',(-188.41669088087,3.31996306880589,135.701888135025));
#264400=CARTESIAN_POINT('Ctrl Pts',(-188.409276388149,3.1900412714635,135.789960242322));
#264401=CARTESIAN_POINT('Ctrl Pts',(-188.401861895428,3.05644812470781,
135.872970336136));
#264402=CARTESIAN_POINT('Ctrl Pts',(-188.394447402707,2.91961665426848,
135.950598967528));
#264403=CARTESIAN_POINT('Ctrl Pts',(-188.387040056353,2.78291706715196,
136.028152777522));
#264404=CARTESIAN_POINT('Ctrl Pts',(-188.37963271,2.64298569258825,136.100335268136));
#264405=CARTESIAN_POINT('Ctrl Pts',(-188.372225363646,2.50028509409351,
136.16686982602));
#264406=CARTESIAN_POINT('Ctrl Pts',(-188.36482354197,2.35769092708891,136.233354759921));
#264407=CARTESIAN_POINT('Ctrl Pts',(-188.357421720295,2.2123319855006,136.294199991563));
#264408=CARTESIAN_POINT('Ctrl Pts',(-188.35001989862,2.06469593138949,136.349174525481));
#264409=CARTESIAN_POINT('Ctrl Pts',(-188.342621984308,1.91713781320257,
136.40412003877));
#264410=CARTESIAN_POINT('Ctrl Pts',(-188.335224069997,1.76730532541907,
136.453200896397));
#264411=CARTESIAN_POINT('Ctrl Pts',(-188.327826155686,1.61570652716677,
136.496234033285));
#264412=CARTESIAN_POINT('Ctrl Pts',(-188.320429470773,1.46413292188381,
136.539260018847));
#264413=CARTESIAN_POINT('Ctrl Pts',(-188.313032785861,1.31079394745819,
136.576240176501));
#264414=CARTESIAN_POINT('Ctrl Pts',(-188.305636100949,1.15621337319739,
136.607041135925));
#264415=CARTESIAN_POINT('Ctrl Pts',(-188.298239744013,1.00163965320169,
136.637840729602));
#264416=CARTESIAN_POINT('Ctrl Pts',(-188.290843387078,0.845824808937177,
136.662461596891));
#264417=CARTESIAN_POINT('Ctrl Pts',(-188.283447030143,0.689303101053426,
136.680821439981));
#264418=CARTESIAN_POINT('Ctrl Pts',(-188.276049540806,0.53275742929617,
136.69918409401));
#264419=CARTESIAN_POINT('Ctrl Pts',(-188.268652051469,0.375505049213833,
136.711283771691));
#264420=CARTESIAN_POINT('Ctrl Pts',(-188.261254562133,0.21808549699706,
136.7170900447));
#264421=CARTESIAN_POINT('Ctrl Pts',(-188.253854479618,0.060610761600514,
136.722898353089));
#264422=CARTESIAN_POINT('Ctrl Pts',(-188.246454397103,-0.0970308897949569,
136.72240885064));
#264423=CARTESIAN_POINT('Ctrl Pts',(-188.239054314588,-0.254299915471865,
136.715643229275));
#264424=CARTESIAN_POINT('Ctrl Pts',(-188.231646094921,-0.411741874610377,
136.708870168413));
#264425=CARTESIAN_POINT('Ctrl Pts',(-188.224237875255,-0.568810016570274,
136.695807222463));
#264426=CARTESIAN_POINT('Ctrl Pts',(-188.216829655588,-0.724969178892556,
136.676528041282));
#264427=CARTESIAN_POINT('Ctrl Pts',(-188.209416876286,-0.881224454573593,
136.657236994087));
#264428=CARTESIAN_POINT('Ctrl Pts',(-188.202004096984,-1.03656926831098,
136.631722148261));
#264429=CARTESIAN_POINT('Ctrl Pts',(-188.194591317682,-1.19047915331876,
136.600108192126));
#264430=CARTESIAN_POINT('Ctrl Pts',(-188.187167946653,-1.34460895198768,
136.568449064488));
#264431=CARTESIAN_POINT('Ctrl Pts',(-188.179744575625,-1.49729936561825,
136.530673510755));
#264432=CARTESIAN_POINT('Ctrl Pts',(-188.172321204596,-1.648040774199,136.486956166176));
#264433=CARTESIAN_POINT('Ctrl Pts',(-188.168385155155,-1.72796748601767,
136.463776181097));
#264434=CARTESIAN_POINT('Ctrl Pts',(-188.164449105714,-1.80734657986099,
136.438926556829));
#264435=CARTESIAN_POINT('Ctrl Pts',(-188.160513056274,-1.88610454236212,
136.412438739149));
#264436=CARTESIAN_POINT('Ctrl Pts',(-188.153089789868,-2.03463960169,136.36248354166));
#264437=CARTESIAN_POINT('Ctrl Pts',(-188.145666523463,-2.18141322895194,
136.306547600599));
#264438=CARTESIAN_POINT('Ctrl Pts',(-188.138243257057,-2.32590747232902,
136.244772825539));
#264439=CARTESIAN_POINT('Ctrl Pts',(-188.130828764336,-2.47023093550992,
136.183071063134));
#264440=CARTESIAN_POINT('Ctrl Pts',(-188.123414271615,-2.61228003741925,
136.115544348554));
#264441=CARTESIAN_POINT('Ctrl Pts',(-188.115999778894,-2.75155195563308,
136.042384328657));
#264442=CARTESIAN_POINT('Ctrl Pts',(-188.10859243254,-2.89068963832824,
135.969294823142));
#264443=CARTESIAN_POINT('Ctrl Pts',(-188.101185086187,-3.02705513796119,
135.890582993991));
#264444=CARTESIAN_POINT('Ctrl Pts',(-188.093777739833,-3.16016570500775,
135.80648849272));
#264445=CARTESIAN_POINT('Ctrl Pts',(-188.086375918158,-3.29317699317143,
135.722456712301));
#264446=CARTESIAN_POINT('Ctrl Pts',(-188.078974096482,-3.42293786829595,
135.633050451894));
#264447=CARTESIAN_POINT('Ctrl Pts',(-188.071572274807,-3.5489903940987,
135.53855513671));
#264448=CARTESIAN_POINT('Ctrl Pts',(-188.064174360495,-3.67497637775464,
135.444109704868));
#264449=CARTESIAN_POINT('Ctrl Pts',(-188.056776446184,-3.79725761282802,
135.344580791833));
#264450=CARTESIAN_POINT('Ctrl Pts',(-188.049378531873,-3.91540546311575,
135.240296890993));
#264451=CARTESIAN_POINT('Ctrl Pts',(-188.041981846961,-4.03353367937402,
135.136030320245));
#264452=CARTESIAN_POINT('Ctrl Pts',(-188.034585162048,-4.1475295945303,
135.027010576778));
#264453=CARTESIAN_POINT('Ctrl Pts',(-188.027188477136,-4.2569978902504,
134.913606232628));
#264454=CARTESIAN_POINT('Ctrl Pts',(-188.019792120201,-4.36646133203156,
134.800206916945));
#264455=CARTESIAN_POINT('Ctrl Pts',(-188.012395763265,-4.4713972942949,
134.682423655727));
#264456=CARTESIAN_POINT('Ctrl Pts',(-188.00499940633,-4.5714477566311,134.560661453614));
#264457=CARTESIAN_POINT('Ctrl Pts',(-187.997601916993,-4.67151353694821,
134.438880609397));
#264458=CARTESIAN_POINT('Ctrl Pts',(-187.990204427657,-4.76669209099886,
134.313119899753));
#264459=CARTESIAN_POINT('Ctrl Pts',(-187.98280693832,-4.85666618608259,
134.183816804508));
#264460=CARTESIAN_POINT('Ctrl Pts',(-187.975406855805,-4.94667182144627,
134.054468382263));
#264461=CARTESIAN_POINT('Ctrl Pts',(-187.96800677329,-5.03146915236339,
133.92157540827));
#264462=CARTESIAN_POINT('Ctrl Pts',(-187.960606690775,-5.11078479338413,
133.785603539271));
#264463=CARTESIAN_POINT('Ctrl Pts',(-187.953198471109,-5.19018765010589,
133.649482155223));
#264464=CARTESIAN_POINT('Ctrl Pts',(-187.945790251442,-5.26409659104829,
133.510275437626));
#264465=CARTESIAN_POINT('Ctrl Pts',(-187.938382031776,-5.3322843115409,
133.368473443359));
#264466=CARTESIAN_POINT('Ctrl Pts',(-187.930969252474,-5.40051400043771,
133.226584172331));
#264467=CARTESIAN_POINT('Ctrl Pts',(-187.923556473172,-5.46301530435872,
133.082096783536));
#264468=CARTESIAN_POINT('Ctrl Pts',(-187.91614369387,-5.51960964001329,
132.93551992282));
#264469=CARTESIAN_POINT('Ctrl Pts',(-187.908720322841,-5.57628484030872,
132.788733626212));
#264470=CARTESIAN_POINT('Ctrl Pts',(-187.901296951812,-5.62703609533202,
132.639852247296));
#264471=CARTESIAN_POINT('Ctrl Pts',(-187.893873580783,-5.67173486859993,
132.489398938438));
#264472=CARTESIAN_POINT('Ctrl Pts',(-187.889937531343,-5.6954352307193,
132.409624984003));
#264473=CARTESIAN_POINT('Ctrl Pts',(-187.886001481902,-5.71743487721036,
132.329409275315));
#264474=CARTESIAN_POINT('Ctrl Pts',(-187.882065432461,-5.73772052852476,
132.248830658462));
#264475=CARTESIAN_POINT('Ctrl Pts',(-187.872272656446,-5.78819063633813,
132.048353413881));
#264476=CARTESIAN_POINT('Ctrl Pts',(-187.862479880431,-5.82817280781611,
131.845137610024));
#264477=CARTESIAN_POINT('Ctrl Pts',(-187.852687104416,-5.85742459265489,
131.640128350768));
#264478=CARTESIAN_POINT('Ctrl Pts',(-187.843111607346,-5.88602734836112,
131.43966777059));
#264479=CARTESIAN_POINT('Ctrl Pts',(-187.833536110275,-5.90437066060156,
131.237492158579));
#264480=CARTESIAN_POINT('Ctrl Pts',(-187.823960613204,-5.91227224031638,
131.034507350944));
#264481=CARTESIAN_POINT('Ctrl Pts',(-187.820432147727,-5.915183885637,130.959709679258));
#264482=CARTESIAN_POINT('Ctrl Pts',(-187.81690368225,-5.91667814734567,
130.88480237372));
#264483=CARTESIAN_POINT('Ctrl Pts',(-187.813375216773,-5.91674747054566,
130.809831658736));
#264484=CARTESIAN_POINT('',(-191.313375192208,-5.91167657527647,130.799567797019));
#264485=CARTESIAN_POINT('Ctrl Pts',(-191.313375192208,-5.91167657527647,
130.799567797019));
#264486=CARTESIAN_POINT('Ctrl Pts',(-191.283395767544,-5.91650671956634,
130.161511730902));
#264487=CARTESIAN_POINT('Ctrl Pts',(-191.160600468276,-5.52689340955663,
127.553783705044));
#264488=CARTESIAN_POINT('Ctrl Pts',(-190.944989294402,-1.71886118746277,
124.020329607269));
#264489=CARTESIAN_POINT('Ctrl Pts',(-190.66654167059,4.77851096535738,125.691299549647));
#264490=CARTESIAN_POINT('Ctrl Pts',(-190.388094046777,6.88466498425298,
132.060922826512));
#264491=CARTESIAN_POINT('Ctrl Pts',(-190.109646422965,2.66414821720038,
137.275826819836));
#264492=CARTESIAN_POINT('Ctrl Pts',(-189.834740626303,-3.91976489026385,
136.553081220811));
#264493=CARTESIAN_POINT('Ctrl Pts',(-189.65265070425,-5.9201422633631,132.691092662961));
#264494=CARTESIAN_POINT('Ctrl Pts',(-189.563376656799,-5.92613653540298,
130.802997987718));
#264495=CARTESIAN_POINT('',(-193.063375192208,-5.90877653025682,130.807662282052));
#264496=CARTESIAN_POINT('Ctrl Pts',(-193.063375192208,-5.90877653025682,
130.807662282052));
#264497=CARTESIAN_POINT('Ctrl Pts',(-193.006957681836,-5.90270635330487,
129.605440343458));
#264498=CARTESIAN_POINT('Ctrl Pts',(-192.857724296862,-4.96095598029521,
126.416633059624));
#264499=CARTESIAN_POINT('Ctrl Pts',(-192.61567503728,0.256241860122023,
123.810656260109));
#264500=CARTESIAN_POINT('Ctrl Pts',(-192.337227413466,6.02250653238034,
127.239676115707));
#264501=CARTESIAN_POINT('Ctrl Pts',(-192.058779789655,6.25438191717603,
133.944466883987));
#264502=CARTESIAN_POINT('Ctrl Pts',(-191.780332165841,0.738785863635208,
137.763653396148));
#264503=CARTESIAN_POINT('Ctrl Pts',(-191.531863966693,-4.78877897888325,
135.464945051595));
#264504=CARTESIAN_POINT('Ctrl Pts',(-191.376211642148,-5.90155266118287,
132.136924284238));
#264505=CARTESIAN_POINT('Ctrl Pts',(-191.313375192208,-5.91167657527647,
130.799567797019));
#264506=CARTESIAN_POINT('',(-194.813375192208,-5.92378430407072,130.807954965743));
#264507=CARTESIAN_POINT('Ctrl Pts',(-194.813375192208,-5.92378430407072,
130.807954965743));
#264508=CARTESIAN_POINT('Ctrl Pts',(-194.730519596129,-5.91124949145352,
129.053764187153));
#264509=CARTESIAN_POINT('Ctrl Pts',(-194.554848125446,-4.15536005181142,
125.312715685492));
#264510=CARTESIAN_POINT('Ctrl Pts',(-194.286360780158,2.21070539777845,
124.164304731159));
#264511=CARTESIAN_POINT('Ctrl Pts',(-194.007913156345,6.78140734036955,
129.075177280167));
#264512=CARTESIAN_POINT('Ctrl Pts',(-193.729465532532,5.12032722732323,
135.575084840937));
#264513=CARTESIAN_POINT('Ctrl Pts',(-193.451017908719,-1.24608346573943,
137.690929903266));
#264514=CARTESIAN_POINT('Ctrl Pts',(-193.228987795278,-5.40948930689292,
134.331882897925));
#264515=CARTESIAN_POINT('Ctrl Pts',(-193.099773556441,-5.91269277027163,
131.5832887094));
#264516=CARTESIAN_POINT('Ctrl Pts',(-193.063375192208,-5.90877653025682,
130.807662282052));
#264517=CARTESIAN_POINT('',(-196.563375192208,-5.91754067440713,130.799324060973));
#264518=CARTESIAN_POINT('Ctrl Pts',(-196.563375192208,-5.92005028606524,
130.799321924984));
#264519=CARTESIAN_POINT('Ctrl Pts',(-196.546897385026,-5.92321501407519,
130.449886125491));
#264520=CARTESIAN_POINT('Ctrl Pts',(-196.530419577843,-5.89494931063627,
130.100961680412));
#264521=CARTESIAN_POINT('Ctrl Pts',(-196.421125896056,-5.48691602341415,
127.826183567757));
#264522=CARTESIAN_POINT('Ctrl Pts',(-196.235494146848,-2.68383279408233,
124.341033141431));
#264523=CARTESIAN_POINT('Ctrl Pts',(-195.957046523035,3.98710327515676,
125.052789701408));
#264524=CARTESIAN_POINT('Ctrl Pts',(-195.678598899222,6.99408621534913,
131.049958953475));
#264525=CARTESIAN_POINT('Ctrl Pts',(-195.400151275409,3.57384560374378,
136.821435332985));
#264526=CARTESIAN_POINT('Ctrl Pts',(-195.121703651596,-3.13058452563971,
137.063513999468));
#264527=CARTESIAN_POINT('Ctrl Pts',(-194.926111623863,-5.81921701947016,
133.19324015144));
#264528=CARTESIAN_POINT('Ctrl Pts',(-194.823335470733,-5.92529114525991,
131.018830628555));
#264529=CARTESIAN_POINT('Ctrl Pts',(-194.813375192208,-5.92378430407072,
130.807954965743));
#264530=CARTESIAN_POINT('',(-198.313375158537,-5.91281518750731,130.803135099679));
#264531=CARTESIAN_POINT('Ctrl Pts',(-198.313375135094,-5.91674987280848,
130.803133783915));
#264532=CARTESIAN_POINT('Ctrl Pts',(-198.305494209198,-5.91671497079014,
130.634808997274));
#264533=CARTESIAN_POINT('Ctrl Pts',(-198.297613283303,-5.90949285436914,
130.466668773567));
#264534=CARTESIAN_POINT('Ctrl Pts',(-198.289732357408,-5.89515605919228,
130.29932042088));
#264535=CARTESIAN_POINT('Ctrl Pts',(-198.281836630896,-5.88079233908077,
130.131657782929));
#264536=CARTESIAN_POINT('Ctrl Pts',(-198.273940904384,-5.85928727531646,
129.964790277688));
#264537=CARTESIAN_POINT('Ctrl Pts',(-198.266045177872,-5.83076466142615,
129.799316327217));
#264538=CARTESIAN_POINT('Ctrl Pts',(-198.258126453544,-5.80215896996073,
129.633360402175));
#264539=CARTESIAN_POINT('Ctrl Pts',(-198.250207729216,-5.76649488777139,
129.468806441626));
#264540=CARTESIAN_POINT('Ctrl Pts',(-198.242289004889,-5.72394703223156,
129.306241485218));
#264541=CARTESIAN_POINT('Ctrl Pts',(-198.234357905677,-5.6813326855795,
129.143422482521));
#264542=CARTESIAN_POINT('Ctrl Pts',(-198.226426806465,-5.63181316657086,
128.982598970972));
#264543=CARTESIAN_POINT('Ctrl Pts',(-198.218495707253,-5.57561197482526,
128.824339994268));
#264544=CARTESIAN_POINT('Ctrl Pts',(-198.210545405859,-5.51927471297368,
128.665697852811));
#264545=CARTESIAN_POINT('Ctrl Pts',(-198.202595104465,-5.45622353317009,
128.509632936207));
#264546=CARTESIAN_POINT('Ctrl Pts',(-198.194644803071,-5.38672971531874,
128.356693659706));
#264547=CARTESIAN_POINT('Ctrl Pts',(-198.19130570656,-5.35754257470302,
128.292459742115));
#264548=CARTESIAN_POINT('Ctrl Pts',(-198.187966610049,-5.32721951801162,
128.228776855833));
#264549=CARTESIAN_POINT('Ctrl Pts',(-198.184627513538,-5.29578296029053,
128.165684169042));
#264550=CARTESIAN_POINT('Ctrl Pts',(-198.177204247133,-5.22589521009871,
128.025420531639));
#264551=CARTESIAN_POINT('Ctrl Pts',(-198.169780980727,-5.15032541721235,
127.887723278348));
#264552=CARTESIAN_POINT('Ctrl Pts',(-198.162357714322,-5.06928530351928,
127.753085953754));
#264553=CARTESIAN_POINT('Ctrl Pts',(-198.154943221601,-4.98834097251064,
127.618607759295));
#264554=CARTESIAN_POINT('Ctrl Pts',(-198.14752872888,-4.90193938086913,
127.487182611414));
#264555=CARTESIAN_POINT('Ctrl Pts',(-198.14011423616,-4.8103394376285,127.359282235686));
#264556=CARTESIAN_POINT('Ctrl Pts',(-198.132706889806,-4.71882778186184,
127.231505135156));
#264557=CARTESIAN_POINT('Ctrl Pts',(-198.125299543452,-4.62212796504708,
127.107246344862));
#264558=CARTESIAN_POINT('Ctrl Pts',(-198.117892197099,-4.52054368801486,
126.986951112778));
#264559=CARTESIAN_POINT('Ctrl Pts',(-198.110490375423,-4.41903517636901,
126.866745601416));
#264560=CARTESIAN_POINT('Ctrl Pts',(-198.103088553748,-4.31264969804995,
126.750498046109));
#264561=CARTESIAN_POINT('Ctrl Pts',(-198.095686732073,-4.20173288463405,
126.638622828328));
#264562=CARTESIAN_POINT('Ctrl Pts',(-198.088288817762,-4.09087462334089,
126.526806668604));
#264563=CARTESIAN_POINT('Ctrl Pts',(-198.080890903451,-3.97549005300435,
126.419358514093));
#264564=CARTESIAN_POINT('Ctrl Pts',(-198.07349298914,-3.85596343966191,
126.316657807164));
#264565=CARTESIAN_POINT('Ctrl Pts',(-198.066096304228,-3.736456689474,126.213974167229));
#264566=CARTESIAN_POINT('Ctrl Pts',(-198.058699619315,-3.61280954527593,
126.116036652106));
#264567=CARTESIAN_POINT('Ctrl Pts',(-198.051302934403,-3.48544139440895,
126.023186196083));
#264568=CARTESIAN_POINT('Ctrl Pts',(-198.043906577468,-3.35807889117926,
125.930339857147));
#264569=CARTESIAN_POINT('Ctrl Pts',(-198.036510220533,-3.22699601099537,
125.842580348711));
#264570=CARTESIAN_POINT('Ctrl Pts',(-198.029113863598,-3.09264310423706,
125.76020665557));
#264571=CARTESIAN_POINT('Ctrl Pts',(-198.021716374261,-2.95826962770573,
125.677820350807));
#264572=CARTESIAN_POINT('Ctrl Pts',(-198.014318884925,-2.82062544600519,
125.600821698323));
#264573=CARTESIAN_POINT('Ctrl Pts',(-198.006921395588,-2.68018747322264,
125.529464820407));
#264574=CARTESIAN_POINT('Ctrl Pts',(-197.999521313073,-2.53970027012625,
125.458082928449));
#264575=CARTESIAN_POINT('Ctrl Pts',(-197.992121230558,-2.39641765864562,
125.392346917666));
#264576=CARTESIAN_POINT('Ctrl Pts',(-197.984721148044,-2.2508384387309,
125.332463607823));
#264577=CARTESIAN_POINT('Ctrl Pts',(-197.977312928377,-2.10509913949819,
125.272514450125));
#264578=CARTESIAN_POINT('Ctrl Pts',(-197.969904708711,-1.95705853397072,
125.21843098787));
#264579=CARTESIAN_POINT('Ctrl Pts',(-197.962496489045,-1.80723326014781,
125.170371044811));
#264580=CARTESIAN_POINT('Ctrl Pts',(-197.955083709743,-1.65731577136839,
125.122281521658));
#264581=CARTESIAN_POINT('Ctrl Pts',(-197.947670930441,-1.50561178442189,
125.080223004612));
#264582=CARTESIAN_POINT('Ctrl Pts',(-197.940258151139,-1.35264965650991,
125.04430250421));
#264583=CARTESIAN_POINT('Ctrl Pts',(-197.93283478011,-1.19946896913657,
125.008330678912));
#264584=CARTESIAN_POINT('Ctrl Pts',(-197.925411409082,-1.04502691596486,
124.97851445706));
#264585=CARTESIAN_POINT('Ctrl Pts',(-197.917988038053,-0.889859347573362,
124.954909283976));
#264586=CARTESIAN_POINT('Ctrl Pts',(-197.91405198861,-0.807585779573266,
124.942393254802));
#264587=CARTESIAN_POINT('Ctrl Pts',(-197.910115939167,-0.725108295893379,
124.931622504652));
#264588=CARTESIAN_POINT('Ctrl Pts',(-197.906179889724,-0.642506819387798,
124.922599355024));
#264589=CARTESIAN_POINT('Ctrl Pts',(-197.898756623319,-0.486723012682509,
124.905581976438));
#264590=CARTESIAN_POINT('Ctrl Pts',(-197.891333356914,-0.330027094746583,
124.894732254595));
#264591=CARTESIAN_POINT('Ctrl Pts',(-197.883910090508,-0.172948739468105,
124.890138834777));
#264592=CARTESIAN_POINT('Ctrl Pts',(-197.876495597787,-0.0160560377610202,
124.885550844));
#264593=CARTESIAN_POINT('Ctrl Pts',(-197.869081105066,0.141217832067213,
124.887204447401));
#264594=CARTESIAN_POINT('Ctrl Pts',(-197.861666612345,0.298336047272165,
124.895136796674));
#264595=CARTESIAN_POINT('Ctrl Pts',(-197.854259265991,0.455302826025905,
124.90306150045));
#264596=CARTESIAN_POINT('Ctrl Pts',(-197.846851919638,0.612113878507934,
124.917252883675));
#264597=CARTESIAN_POINT('Ctrl Pts',(-197.839444573284,0.768230447271629,
124.937696101643));
#264598=CARTESIAN_POINT('Ctrl Pts',(-197.832042751609,0.924230578407954,
124.958124072289));
#264599=CARTESIAN_POINT('Ctrl Pts',(-197.824640929933,1.07953688863353,
124.984794545045));
#264600=CARTESIAN_POINT('Ctrl Pts',(-197.817239108258,1.23361392477094,
125.017640713587));
#264601=CARTESIAN_POINT('Ctrl Pts',(-197.809841193946,1.38760962484074,
125.050469542891));
#264602=CARTESIAN_POINT('Ctrl Pts',(-197.802443279635,1.54037697901615,
125.089467497698));
#264603=CARTESIAN_POINT('Ctrl Pts',(-197.795045365324,1.69138904650517,
125.134516381975));
#264604=CARTESIAN_POINT('Ctrl Pts',(-197.787648680412,1.84237601852799,
125.179557779945));
#264605=CARTESIAN_POINT('Ctrl Pts',(-197.780251995499,1.99160792542631,
125.23064800505));
#264606=CARTESIAN_POINT('Ctrl Pts',(-197.772855310587,2.1385712404262,125.287618498152));
#264607=CARTESIAN_POINT('Ctrl Pts',(-197.765458953652,2.2855280389187,125.344586465122));
#264608=CARTESIAN_POINT('Ctrl Pts',(-197.758062596717,2.43021609746273,
125.407434046729));
#264609=CARTESIAN_POINT('Ctrl Pts',(-197.750666239781,2.57214044630336,
125.475943959028));
#264610=CARTESIAN_POINT('Ctrl Pts',(-197.743268750445,2.71408652412452,
125.544464360369));
#264611=CARTESIAN_POINT('Ctrl Pts',(-197.735871261108,2.8532677135316,125.618648656259));
#264612=CARTESIAN_POINT('Ctrl Pts',(-197.728473771771,2.98921243053313,
125.698232964672));
#264613=CARTESIAN_POINT('Ctrl Pts',(-197.721073689256,3.12520480274389,
125.777845171241));
#264614=CARTESIAN_POINT('Ctrl Pts',(-197.713673606741,3.25795812173416,
125.862860970739));
#264615=CARTESIAN_POINT('Ctrl Pts',(-197.706273524226,3.38702877062359,
125.952972499772));
#264616=CARTESIAN_POINT('Ctrl Pts',(-197.69886530456,3.51624134596045,126.043183115696));
#264617=CARTESIAN_POINT('Ctrl Pts',(-197.691457084894,3.64176285786007,
126.138500437448));
#264618=CARTESIAN_POINT('Ctrl Pts',(-197.684048865227,3.76318126927204,
126.238575110438));
#264619=CARTESIAN_POINT('Ctrl Pts',(-197.676636085925,3.88467441169026,
126.33871137772));
#264620=CARTESIAN_POINT('Ctrl Pts',(-197.669223306623,4.002059143761,126.443610582622));
#264621=CARTESIAN_POINT('Ctrl Pts',(-197.661810527321,4.11495984451519,
126.552886045076));
#264622=CARTESIAN_POINT('Ctrl Pts',(-197.654387156293,4.2280218630853,126.662317645436));
#264623=CARTESIAN_POINT('Ctrl Pts',(-197.646963785264,4.33658679716489,
126.776137722587));
#264624=CARTESIAN_POINT('Ctrl Pts',(-197.639540414235,4.4403183587074,126.893925419813));
#264625=CARTESIAN_POINT('Ctrl Pts',(-197.635604364794,4.49531932164588,
126.956379283164));
#264626=CARTESIAN_POINT('Ctrl Pts',(-197.631668315353,4.54896215332004,
127.019948072493));
#264627=CARTESIAN_POINT('Ctrl Pts',(-197.627732265912,4.60120170033201,
127.084565801267));
#264628=CARTESIAN_POINT('Ctrl Pts',(-197.620308999507,4.69972385564997,
127.206432821078));
#264629=CARTESIAN_POINT('Ctrl Pts',(-197.612885733101,4.79355000507247,
127.332400995022));
#264630=CARTESIAN_POINT('Ctrl Pts',(-197.605462466696,4.88231926713834,
127.462072608398));
#264631=CARTESIAN_POINT('Ctrl Pts',(-197.598047973975,4.97098361130828,
127.591590960695));
#264632=CARTESIAN_POINT('Ctrl Pts',(-197.590633481254,5.05460275620507,
127.72480373464));
#264633=CARTESIAN_POINT('Ctrl Pts',(-197.583218988533,5.13285527925053,
127.861279367452));
#264634=CARTESIAN_POINT('Ctrl Pts',(-197.575811642179,5.21103237956813,
127.997623459912));
#264635=CARTESIAN_POINT('Ctrl Pts',(-197.568404295825,5.28385297112994,
128.137223828763));
#264636=CARTESIAN_POINT('Ctrl Pts',(-197.560996949471,5.35103833164711,
128.279619178182));
#264637=CARTESIAN_POINT('Ctrl Pts',(-197.553595127796,5.41817358278764,
128.421908323777));
#264638=CARTESIAN_POINT('Ctrl Pts',(-197.54619330612,5.47968181295513,128.566987963062));
#264639=CARTESIAN_POINT('Ctrl Pts',(-197.538791484445,5.53532980268285,
128.714371493663));
#264640=CARTESIAN_POINT('Ctrl Pts',(-197.531393570133,5.59094841626997,
128.861677221646));
#264641=CARTESIAN_POINT('Ctrl Pts',(-197.523995655822,5.64071281889356,
129.011284070463));
#264642=CARTESIAN_POINT('Ctrl Pts',(-197.516597741511,5.6844376278525,129.162684822059));
#264643=CARTESIAN_POINT('Ctrl Pts',(-197.509201056598,5.72815517054139,
129.314060413596));
#264644=CARTESIAN_POINT('Ctrl Pts',(-197.501804371686,5.76583500808062,
129.467228957956));
#264645=CARTESIAN_POINT('Ctrl Pts',(-197.494407686774,5.79734138028169,
129.621667300187));
#264646=CARTESIAN_POINT('Ctrl Pts',(-197.487011329838,5.82884635545729,
129.77609879446));
#264647=CARTESIAN_POINT('Ctrl Pts',(-197.479614972903,5.85417833496008,
129.93179960889));
#264648=CARTESIAN_POINT('Ctrl Pts',(-197.472218615968,5.87325258268416,
130.088235864123));
#264649=CARTESIAN_POINT('Ctrl Pts',(-197.464821126631,5.89232975072421,
130.244696070146));
#264650=CARTESIAN_POINT('Ctrl Pts',(-197.457423637294,5.90514723414698,
130.401891570591));
#264651=CARTESIAN_POINT('Ctrl Pts',(-197.450026147958,5.91167214170678,
130.559282973812));
#264652=CARTESIAN_POINT('Ctrl Pts',(-197.442626065443,5.91819933656282,
130.716729550346));
#264653=CARTESIAN_POINT('Ctrl Pts',(-197.435225982928,5.9184295482666,130.874371793638));
#264654=CARTESIAN_POINT('Ctrl Pts',(-197.427825900413,5.91238200524872,
131.03167006856));
#264655=CARTESIAN_POINT('Ctrl Pts',(-197.420417680746,5.9063278123356,131.189141309106));
#264656=CARTESIAN_POINT('Ctrl Pts',(-197.41300946108,5.89398209323351,131.346267452684));
#264657=CARTESIAN_POINT('Ctrl Pts',(-197.405601241413,5.87541605376114,
131.502513006165));
#264658=CARTESIAN_POINT('Ctrl Pts',(-197.398188462111,5.85683858720126,
131.658854726177));
#264659=CARTESIAN_POINT('Ctrl Pts',(-197.390775682809,5.83203323018161,
131.814314408332));
#264660=CARTESIAN_POINT('Ctrl Pts',(-197.383362903507,5.80112227528612,
131.96836702205));
#264661=CARTESIAN_POINT('Ctrl Pts',(-197.375939532478,5.77016715336866,
132.122639753366));
#264662=CARTESIAN_POINT('Ctrl Pts',(-197.368516161449,5.73308909762374,
132.275501039037));
#264663=CARTESIAN_POINT('Ctrl Pts',(-197.361092790421,5.69006041482304,
132.426440467069));
#264664=CARTESIAN_POINT('Ctrl Pts',(-197.35715674098,5.66724557474622,132.506472173542));
#264665=CARTESIAN_POINT('Ctrl Pts',(-197.35322069154,5.64275861274537,132.585963890444));
#264666=CARTESIAN_POINT('Ctrl Pts',(-197.3492846421,5.6166306386455,132.664841961608));
#264667=CARTESIAN_POINT('Ctrl Pts',(-197.341861375694,5.56735409491276,
132.813603542143));
#264668=CARTESIAN_POINT('Ctrl Pts',(-197.334438109289,5.51208882816386,
132.960631013906));
#264669=CARTESIAN_POINT('Ctrl Pts',(-197.327014842883,5.45097438179734,
133.105405782592));
#264670=CARTESIAN_POINT('Ctrl Pts',(-197.319600350162,5.38993216763119,
133.250009439524));
#264671=CARTESIAN_POINT('Ctrl Pts',(-197.312185857442,5.32305467845807,
133.392365352562));
#264672=CARTESIAN_POINT('Ctrl Pts',(-197.304771364721,5.25053126351302,
133.531969829563));
#264673=CARTESIAN_POINT('Ctrl Pts',(-197.297364018367,5.17807774936575,
133.671439750514));
#264674=CARTESIAN_POINT('Ctrl Pts',(-197.289956672013,5.09998931384532,
133.808163185873));
#264675=CARTESIAN_POINT('Ctrl Pts',(-197.282549325659,5.01650340198775,
133.941656297024));
#264676=CARTESIAN_POINT('Ctrl Pts',(-197.275147503984,4.93307975707299,
134.075049843976));
#264677=CARTESIAN_POINT('Ctrl Pts',(-197.267745682308,4.84426684850198,
134.20521754882));
#264678=CARTESIAN_POINT('Ctrl Pts',(-197.260343860633,4.75034800781524,
134.331700176943));
#264679=CARTESIAN_POINT('Ctrl Pts',(-197.252945946322,4.65647874615343,
134.458116035871));
#264680=CARTESIAN_POINT('Ctrl Pts',(-197.24554803201,4.55750914234047,134.580850393335));
#264681=CARTESIAN_POINT('Ctrl Pts',(-197.238150117699,4.453765729412,134.699473117869));
#264682=CARTESIAN_POINT('Ctrl Pts',(-197.230753432787,4.3500395567568,134.818076129458));
#264683=CARTESIAN_POINT('Ctrl Pts',(-197.223356747875,4.24154139500116,
134.932568583504));
#264684=CARTESIAN_POINT('Ctrl Pts',(-197.215960062963,4.12863800752296,
135.042553483085));
#264685=CARTESIAN_POINT('Ctrl Pts',(-197.208563706027,4.01573962629928,
135.152533505821));
#264686=CARTESIAN_POINT('Ctrl Pts',(-197.201167349092,3.89843667513432,
135.258006111018));
#264687=CARTESIAN_POINT('Ctrl Pts',(-197.193770992156,3.77713251991294,
135.35861143296));
#264688=CARTESIAN_POINT('Ctrl Pts',(-197.18637350282,3.65580979271537,135.459232157834));
#264689=CARTESIAN_POINT('Ctrl Pts',(-197.178976013483,3.53048492905807,
135.554983877352));
#264690=CARTESIAN_POINT('Ctrl Pts',(-197.171578524146,3.40159395588911,
135.645547364817));
#264691=CARTESIAN_POINT('Ctrl Pts',(-197.164178441631,3.27265780018913,
135.736142599172));
#264692=CARTESIAN_POINT('Ctrl Pts',(-197.156778359116,3.14015335129741,
135.821545765924));
#264693=CARTESIAN_POINT('Ctrl Pts',(-197.149378276601,3.00454501296717,
135.901481356528));
#264694=CARTESIAN_POINT('Ctrl Pts',(-197.141970056935,2.86878755932826,
135.981504844531));
#264695=CARTESIAN_POINT('Ctrl Pts',(-197.134561837268,2.72991972195824,
136.056048560025));
#264696=CARTESIAN_POINT('Ctrl Pts',(-197.127153617602,2.58843051487615,
136.124882963366));
#264697=CARTESIAN_POINT('Ctrl Pts',(-197.1197408383,2.44685422354838,136.193759733134));
#264698=CARTESIAN_POINT('Ctrl Pts',(-197.112328058998,2.3026536887318,136.256920039268));
#264699=CARTESIAN_POINT('Ctrl Pts',(-197.104915279696,2.15633673565307,
136.31418297813));
#264700=CARTESIAN_POINT('Ctrl Pts',(-197.097491908667,2.00981071804999,
136.371527736965));
#264701=CARTESIAN_POINT('Ctrl Pts',(-197.090068537638,1.86116259434809,
136.422958177311));
#264702=CARTESIAN_POINT('Ctrl Pts',(-197.08264516661,1.71091492463178,136.468343375588));
#264703=CARTESIAN_POINT('Ctrl Pts',(-197.078709117169,1.63125000500077,
136.492407696719));
#264704=CARTESIAN_POINT('Ctrl Pts',(-197.074773067728,1.55113557114578,
136.514773336763));
#264705=CARTESIAN_POINT('Ctrl Pts',(-197.070837018287,1.47065040770534,
136.535426656342));
#264706=CARTESIAN_POINT('Ctrl Pts',(-197.063413751881,1.31885790131885,
136.574378172499));
#264707=CARTESIAN_POINT('Ctrl Pts',(-197.055990485476,1.16528729868185,
136.607353878223));
#264708=CARTESIAN_POINT('Ctrl Pts',(-197.04856721907,1.01045033448641,136.634190862439));
#264709=CARTESIAN_POINT('Ctrl Pts',(-197.041152726349,0.855796374724231,
136.660996127568));
#264710=CARTESIAN_POINT('Ctrl Pts',(-197.033738233628,0.699879396883509,
136.681677050091));
#264711=CARTESIAN_POINT('Ctrl Pts',(-197.026323740907,0.543225519315743,
136.696120676976));
#264712=CARTESIAN_POINT('Ctrl Pts',(-197.018916394553,0.38672263065309,
136.71055038255));
#264713=CARTESIAN_POINT('Ctrl Pts',(-197.011509048199,0.229484625460507,
136.718754726634));
#264714=CARTESIAN_POINT('Ctrl Pts',(-197.004101701846,0.072046915710644,
136.720671951872));
#264715=CARTESIAN_POINT('Ctrl Pts',(-196.99669988017,-0.0852733710555033,
136.722587747171));
#264716=CARTESIAN_POINT('Ctrl Pts',(-196.989298058495,-0.242792694141263,
136.718225755868));
#264717=CARTESIAN_POINT('Ctrl Pts',(-196.981896236819,-0.399971538843124,
136.707576125289));
#264718=CARTESIAN_POINT('Ctrl Pts',(-196.974498322508,-0.557067410055896,
136.696932116566));
#264719=CARTESIAN_POINT('Ctrl Pts',(-196.967100408196,-0.71382278933619,
136.680007104075));
#264720=CARTESIAN_POINT('Ctrl Pts',(-196.959702493885,-0.869699295819346,
136.656843312743));
#264721=CARTESIAN_POINT('Ctrl Pts',(-196.952305808973,-1.02554989845523,
136.633683370814));
#264722=CARTESIAN_POINT('Ctrl Pts',(-196.944909124061,-1.18052154928376,
136.604286762546));
#264723=CARTESIAN_POINT('Ctrl Pts',(-196.937512439148,-1.33408199898751,
136.568747469823));
#264724=CARTESIAN_POINT('Ctrl Pts',(-196.930116082213,-1.48763563966,136.533209752951));
#264725=CARTESIAN_POINT('Ctrl Pts',(-196.922719725277,-1.63977783994152,
136.491529977363));
#264726=CARTESIAN_POINT('Ctrl Pts',(-196.915323368342,-1.7899878054991,
136.443852989993));
#264727=CARTESIAN_POINT('Ctrl Pts',(-196.907925879005,-1.94022076858587,
136.396168703155));
#264728=CARTESIAN_POINT('Ctrl Pts',(-196.900528389669,-2.08852055208359,
136.34248548924));
#264729=CARTESIAN_POINT('Ctrl Pts',(-196.893130900332,-2.23438289831461,
136.28299764024));
#264730=CARTESIAN_POINT('Ctrl Pts',(-196.885730817817,-2.38029637636477,
136.223488937868));
#264731=CARTESIAN_POINT('Ctrl Pts',(-196.878330735302,-2.52377037052379,
136.158171690011));
#264732=CARTESIAN_POINT('Ctrl Pts',(-196.870930652787,-2.66432206607766,
136.087287693602));
#264733=CARTESIAN_POINT('Ctrl Pts',(-196.86352243312,-2.80502831267005,
136.016325752951));
#264734=CARTESIAN_POINT('Ctrl Pts',(-196.856114213454,-2.9428055098375,
135.939785007485));
#264735=CARTESIAN_POINT('Ctrl Pts',(-196.848705993787,-3.07719621535446,
135.857952806763));
#264736=CARTESIAN_POINT('Ctrl Pts',(-196.841293214485,-3.21166963610861,
135.776070239686));
#264737=CARTESIAN_POINT('Ctrl Pts',(-196.833880435183,-3.3427521018158,
135.688889934013));
#264738=CARTESIAN_POINT('Ctrl Pts',(-196.826467655881,-3.47001692118132,
135.596741354654));
#264739=CARTESIAN_POINT('Ctrl Pts',(-196.819044284852,-3.59746358248833,
135.504461109084));
#264740=CARTESIAN_POINT('Ctrl Pts',(-196.811620913823,-3.72108141033138,
135.407198641944));
#264741=CARTESIAN_POINT('Ctrl Pts',(-196.804197542794,-3.84047779850241,
135.305322830439));
#264742=CARTESIAN_POINT('Ctrl Pts',(-196.800261493354,-3.90378462838005,
135.251305830709));
#264743=CARTESIAN_POINT('Ctrl Pts',(-196.796325443914,-3.96590528316954,
135.195992463312));
#264744=CARTESIAN_POINT('Ctrl Pts',(-196.792389394474,-4.02678570265285,
135.139441639578));
#264745=CARTESIAN_POINT('Ctrl Pts',(-196.78507668251,-4.13989428490648,
135.034376931548));
#264746=CARTESIAN_POINT('Ctrl Pts',(-196.777763970547,-4.24908372070728,
134.924700531894));
#264747=CARTESIAN_POINT('Ctrl Pts',(-196.770451258584,-4.35394615139191,
134.810740963125));
#264748=CARTESIAN_POINT('Ctrl Pts',(-196.763147289429,-4.45868321243069,
134.696917640204));
#264749=CARTESIAN_POINT('Ctrl Pts',(-196.755843320274,-4.55910330236656,
134.578821616739));
#264750=CARTESIAN_POINT('Ctrl Pts',(-196.748539351119,-4.65483230230702,
134.456820993792));
#264751=CARTESIAN_POINT('Ctrl Pts',(-196.741242407847,-4.75046921796755,
134.3349377265));
#264752=CARTESIAN_POINT('Ctrl Pts',(-196.733945464575,-4.84142378676094,
134.209157634796));
#264753=CARTESIAN_POINT('Ctrl Pts',(-196.726648521302,-4.92735958258975,
134.079884714006));
#264754=CARTESIAN_POINT('Ctrl Pts',(-196.719357248112,-5.01322860210467,
133.950712244595));
#264755=CARTESIAN_POINT('Ctrl Pts',(-196.712065974921,-5.09408640058275,
133.818052669374));
#264756=CARTESIAN_POINT('Ctrl Pts',(-196.704774701731,-5.16963782844034,
133.682341730301));
#264757=CARTESIAN_POINT('Ctrl Pts',(-196.697486477277,-5.24515766559986,
133.546687536724));
#264758=CARTESIAN_POINT('Ctrl Pts',(-196.690198252823,-5.31537535882009,
133.407984853367));
#264759=CARTESIAN_POINT('Ctrl Pts',(-196.682910028369,-5.38004001794075,
133.266696900013));
#264760=CARTESIAN_POINT('Ctrl Pts',(-196.675623313027,-5.44469128748668,
133.125438201984));
#264761=CARTESIAN_POINT('Ctrl Pts',(-196.668336597685,-5.50379165095616,
132.98159564949));
#264762=CARTESIAN_POINT('Ctrl Pts',(-196.661049882344,-5.5571371184965,
132.835655182303));
#264763=CARTESIAN_POINT('Ctrl Pts',(-196.653763137853,-5.61048279943774,
132.689714131302));
#264764=CARTESIAN_POINT('Ctrl Pts',(-196.646476393361,-5.65807340793315,
132.541675511368));
#264765=CARTESIAN_POINT('Ctrl Pts',(-196.63918964887,-5.69975396984224,
132.392042967965));
#264766=CARTESIAN_POINT('Ctrl Pts',(-196.631898500147,-5.74145972418876,
132.242319984118));
#264767=CARTESIAN_POINT('Ctrl Pts',(-196.624607351424,-5.77724819432482,
132.091001524323));
#264768=CARTESIAN_POINT('Ctrl Pts',(-196.617316202701,-5.80701487487784,
131.938604332756));
#264769=CARTESIAN_POINT('Ctrl Pts',(-196.61002256742,-5.83679170699883,
131.786155167962));
#264770=CARTESIAN_POINT('Ctrl Pts',(-196.602728932139,-5.86054259825711,
131.632626918938));
#264771=CARTESIAN_POINT('Ctrl Pts',(-196.595435296857,-5.87821471232728,
131.478543351162));
#264772=CARTESIAN_POINT('Ctrl Pts',(-196.58813424297,-5.89590480130939,
131.324303059717));
#264773=CARTESIAN_POINT('Ctrl Pts',(-196.580833189082,-5.90750373817299,
131.169506705419));
#264774=CARTESIAN_POINT('Ctrl Pts',(-196.573532135195,-5.91301075271542,
131.014680375962));
#264775=CARTESIAN_POINT('Ctrl Pts',(-196.570146487533,-5.91556446772689,
130.942884247832));
#264776=CARTESIAN_POINT('Ctrl Pts',(-196.56676083987,-5.91680893090054,
130.871081648203));
#264777=CARTESIAN_POINT('Ctrl Pts',(-196.563375192208,-5.91674785692228,
130.799324735758));
#264778=CARTESIAN_POINT('',(-200.063375194059,-5.91567330630329,130.809819562943));
#264779=CARTESIAN_POINT('Ctrl Pts',(-200.063375192208,-5.91554583036233,
130.809819405987));
#264780=CARTESIAN_POINT('Ctrl Pts',(-199.994021213611,-5.90217632497919,
129.336193982877));
#264781=CARTESIAN_POINT('Ctrl Pts',(-199.831851360409,-4.59893760167832,
125.869330780398));
#264782=CARTESIAN_POINT('Ctrl Pts',(-199.576865632603,1.22511734593415,
123.91403058054));
#264783=CARTESIAN_POINT('Ctrl Pts',(-199.298418008789,6.45923565506566,
128.110694847157));
#264784=CARTESIAN_POINT('Ctrl Pts',(-199.019970384977,5.7576319483906,134.782706363876));
#264785=CARTESIAN_POINT('Ctrl Pts',(-198.741522761164,-0.234954242897439,
137.798812492739));
#264786=CARTESIAN_POINT('Ctrl Pts',(-198.505991030241,-5.12129580041003,
134.913151181637));
#264787=CARTESIAN_POINT('Ctrl Pts',(-198.363275173922,-5.90520520611573,
131.867199701326));
#264788=CARTESIAN_POINT('Ctrl Pts',(-198.313375192208,-5.90716405999748,
130.803136989425));
#264789=CARTESIAN_POINT('',(-201.813375867204,-5.92197308054016,130.803199987403));
#264790=CARTESIAN_POINT('Ctrl Pts',(-201.813375192208,-5.91674988355362,
130.803186748634));
#264791=CARTESIAN_POINT('Ctrl Pts',(-201.810399002507,-5.91673741614191,
130.740346209347));
#264792=CARTESIAN_POINT('Ctrl Pts',(-201.807422812807,-5.9157238558129,
130.677516728804));
#264793=CARTESIAN_POINT('Ctrl Pts',(-201.804446623105,-5.91371007129092,
130.614719495411));
#264794=CARTESIAN_POINT('Ctrl Pts',(-201.7970233567,-5.90868725336307,130.458089495395));
#264795=CARTESIAN_POINT('Ctrl Pts',(-201.789600090295,-5.89742980985056,
130.301422341445));
#264796=CARTESIAN_POINT('Ctrl Pts',(-201.782176823889,-5.87992433832519,
130.145254906719));
#264797=CARTESIAN_POINT('Ctrl Pts',(-201.774762331168,-5.86243955681343,
129.989272048933));
#264798=CARTESIAN_POINT('Ctrl Pts',(-201.767347838447,-5.83872148765387,
129.833788102077));
#264799=CARTESIAN_POINT('Ctrl Pts',(-201.759933345726,-5.80880871565572,
129.679339787793));
#264800=CARTESIAN_POINT('Ctrl Pts',(-201.752525999373,-5.77892477471341,
129.52504033661));
#264801=CARTESIAN_POINT('Ctrl Pts',(-201.745118653019,-5.74285808789947,
129.371774894843));
#264802=CARTESIAN_POINT('Ctrl Pts',(-201.737711306665,-5.70069899303698,
129.220074799512));
#264803=CARTESIAN_POINT('Ctrl Pts',(-201.73030948499,-5.658571342018,129.068487847836));
#264804=CARTESIAN_POINT('Ctrl Pts',(-201.722907663315,-5.6103604300888,
128.918464276076));
#264805=CARTESIAN_POINT('Ctrl Pts',(-201.715505841639,-5.55620757811541,
128.770524854434));
#264806=CARTESIAN_POINT('Ctrl Pts',(-201.708107927328,-5.50208331301106,
128.622663528862));
#264807=CARTESIAN_POINT('Ctrl Pts',(-201.700710013017,-5.44202348275199,
128.476884511958));
#264808=CARTESIAN_POINT('Ctrl Pts',(-201.693312098705,-5.37621909378814,
128.333692930869));
#264809=CARTESIAN_POINT('Ctrl Pts',(-201.685915413793,-5.31042564032021,
128.190525145624));
#264810=CARTESIAN_POINT('Ctrl Pts',(-201.678518728881,-5.23888967855432,
128.049944281665));
#264811=CARTESIAN_POINT('Ctrl Pts',(-201.671122043969,-5.16185019591898,
127.912435114136));
#264812=CARTESIAN_POINT('Ctrl Pts',(-201.663725687034,-5.08481412929481,
127.774932043906));
#264813=CARTESIAN_POINT('Ctrl Pts',(-201.656329330098,-5.00227520947535,
127.640500724959));
#264814=CARTESIAN_POINT('Ctrl Pts',(-201.648932973163,-4.91451806073126,
127.509600718386));
#264815=CARTESIAN_POINT('Ctrl Pts',(-201.641535483827,-4.82674747614365,
127.378680670687));
#264816=CARTESIAN_POINT('Ctrl Pts',(-201.63413799449,-4.73375727975254,
127.251293321958));
#264817=CARTESIAN_POINT('Ctrl Pts',(-201.626740505153,-4.635874949064,127.127868536908));
#264818=CARTESIAN_POINT('Ctrl Pts',(-201.619340422639,-4.53795830587631,
127.004400485491));
#264819=CARTESIAN_POINT('Ctrl Pts',(-201.611940340124,-4.43514634578947,
126.884898055683));
#264820=CARTESIAN_POINT('Ctrl Pts',(-201.604540257609,-4.32780616554116,
126.76975724722));
#264821=CARTESIAN_POINT('Ctrl Pts',(-201.597132037942,-4.22034795372998,
126.654489829602));
#264822=CARTESIAN_POINT('Ctrl Pts',(-201.589723818276,-4.10835183258725,
126.543593884573));
#264823=CARTESIAN_POINT('Ctrl Pts',(-201.58231559861,-3.99222154535993,
126.437428319572));
#264824=CARTESIAN_POINT('Ctrl Pts',(-201.574902819308,-3.87601978187823,
126.331197411437));
#264825=CARTESIAN_POINT('Ctrl Pts',(-201.567490040006,-3.7556790667533,
126.22970292491));
#264826=CARTESIAN_POINT('Ctrl Pts',(-201.560077260704,-3.63163498628868,
126.133262471641));
#264827=CARTESIAN_POINT('Ctrl Pts',(-201.552653889675,-3.50741366582499,
126.03668421973));
#264828=CARTESIAN_POINT('Ctrl Pts',(-201.545230518646,-3.3794787144427,
125.945174640511));
#264829=CARTESIAN_POINT('Ctrl Pts',(-201.537807147618,-3.24829403434159,
125.859007603982));
#264830=CARTESIAN_POINT('Ctrl Pts',(-201.533871098176,-3.17873676920309,
125.813319773655));
#264831=CARTESIAN_POINT('Ctrl Pts',(-201.529935048734,-3.10826629928466,
125.769133155338));
#264832=CARTESIAN_POINT('Ctrl Pts',(-201.525998999293,-3.03695429695874,
125.726483190857));
#264833=CARTESIAN_POINT('Ctrl Pts',(-201.518575732887,-2.90246208617211,
125.646046688922));
#264834=CARTESIAN_POINT('Ctrl Pts',(-201.511152466482,-2.76456864931066,
125.570835471457));
#264835=CARTESIAN_POINT('Ctrl Pts',(-201.503729200076,-2.6237184286282,
125.50115100736));
#264836=CARTESIAN_POINT('Ctrl Pts',(-201.496314707355,-2.4830346812097,
125.431548904513));
#264837=CARTESIAN_POINT('Ctrl Pts',(-201.488900214634,-2.3394014374572,
125.367460716645));
#264838=CARTESIAN_POINT('Ctrl Pts',(-201.481485721913,-2.1932911125198,
125.30914409242));
#264839=CARTESIAN_POINT('Ctrl Pts',(-201.47407837556,-2.04732161421452,
125.250883675953));
#264840=CARTESIAN_POINT('Ctrl Pts',(-201.466671029206,-1.89888013215013,
125.198383886038));
#264841=CARTESIAN_POINT('Ctrl Pts',(-201.459263682852,-1.74846252501016,
125.151855919546));
#264842=CARTESIAN_POINT('Ctrl Pts',(-201.451861861177,-1.5981571049961,
125.105362655367));
#264843=CARTESIAN_POINT('Ctrl Pts',(-201.444460039501,-1.44587884966913,
125.064832455911));
#264844=CARTESIAN_POINT('Ctrl Pts',(-201.437058217826,-1.29214228512928,
125.030427912946));
#264845=CARTESIAN_POINT('Ctrl Pts',(-201.429660303514,-1.13848687692604,
124.996041531872));
#264846=CARTESIAN_POINT('Ctrl Pts',(-201.422262389203,-0.983375056028614,
124.967774448564));
#264847=CARTESIAN_POINT('Ctrl Pts',(-201.414864474892,-0.827335043864665,
124.94573899745));
#264848=CARTESIAN_POINT('Ctrl Pts',(-201.40746778998,-0.67132096271966,
124.923707208227));
#264849=CARTESIAN_POINT('Ctrl Pts',(-201.400071105067,-0.514379365714424,
124.907905048017));
#264850=CARTESIAN_POINT('Ctrl Pts',(-201.392674420155,-0.357047286449173,
124.898393482732));
#264851=CARTESIAN_POINT('Ctrl Pts',(-201.38527806322,-0.199722183453189,
124.8888823392));
#264852=CARTESIAN_POINT('Ctrl Pts',(-201.377881706284,-0.0420070052413085,
124.88566125851));
#264853=CARTESIAN_POINT('Ctrl Pts',(-201.370485349349,0.115557760055124,
124.888739182198));
#264854=CARTESIAN_POINT('Ctrl Pts',(-201.363087860012,0.273146648919818,
124.891817577123));
#264855=CARTESIAN_POINT('Ctrl Pts',(-201.355690370676,0.430584705765377,
124.90119688937));
#264856=CARTESIAN_POINT('Ctrl Pts',(-201.348292881339,0.587333263647712,
124.916833955213));
#264857=CARTESIAN_POINT('Ctrl Pts',(-201.340892798824,0.744136769493798,
124.932476502606));
#264858=CARTESIAN_POINT('Ctrl Pts',(-201.333492716309,0.900249923925743,
124.954381134094));
#264859=CARTESIAN_POINT('Ctrl Pts',(-201.326092633794,1.05514113639827,
124.982453048325));
#264860=CARTESIAN_POINT('Ctrl Pts',(-201.318684414127,1.21020266768233,
125.010555830512));
#264861=CARTESIAN_POINT('Ctrl Pts',(-201.311276194461,1.36403920610859,
125.044839372054));
#264862=CARTESIAN_POINT('Ctrl Pts',(-201.303867974794,1.51613055959717,
125.08515799056));
#264863=CARTESIAN_POINT('Ctrl Pts',(-201.296455195492,1.66831552277604,
125.125501424502));
#264864=CARTESIAN_POINT('Ctrl Pts',(-201.28904241619,1.81875280477592,125.171887227256));
#264865=CARTESIAN_POINT('Ctrl Pts',(-201.281629636888,1.96693974488418,
125.224120604583));
#264866=CARTESIAN_POINT('Ctrl Pts',(-201.274206265859,2.11533842144153,
125.276428615409));
#264867=CARTESIAN_POINT('Ctrl Pts',(-201.266782894831,2.26147998833225,
125.334600750501));
#264868=CARTESIAN_POINT('Ctrl Pts',(-201.259359523802,2.4048832805008,125.398394749225));
#264869=CARTESIAN_POINT('Ctrl Pts',(-201.255423474361,2.48091914692211,
125.432219858064));
#264870=CARTESIAN_POINT('Ctrl Pts',(-201.25148742492,2.55618561065255,125.467624713707));
#264871=CARTESIAN_POINT('Ctrl Pts',(-201.24755137548,2.63061411281273,125.504568173331));
#264872=CARTESIAN_POINT('Ctrl Pts',(-201.240128109074,2.77098394505528,
125.574242385217));
#264873=CARTESIAN_POINT('Ctrl Pts',(-201.232704842669,2.908796043259,125.649602538817));
#264874=CARTESIAN_POINT('Ctrl Pts',(-201.225281576263,3.04355654120713,
125.730437663581));
#264875=CARTESIAN_POINT('Ctrl Pts',(-201.217867083542,3.17815776343784,
125.81117724794));
#264876=CARTESIAN_POINT('Ctrl Pts',(-201.210452590821,3.30971424764855,
125.89737873283));
#264877=CARTESIAN_POINT('Ctrl Pts',(-201.2030380981,3.43775387479355,125.988783927403));
#264878=CARTESIAN_POINT('Ctrl Pts',(-201.195630751746,3.56567009252529,
126.080101022208));
#264879=CARTESIAN_POINT('Ctrl Pts',(-201.188223405393,3.69007589959199,
126.176611626323));
#264880=CARTESIAN_POINT('Ctrl Pts',(-201.180816059039,3.81052558635577,
126.27801271686));
#264881=CARTESIAN_POINT('Ctrl Pts',(-201.173414237363,3.93088543719886,
126.379338178638));
#264882=CARTESIAN_POINT('Ctrl Pts',(-201.166012415688,4.04729475848319,
126.485546624777));
#264883=CARTESIAN_POINT('Ctrl Pts',(-201.158610594013,4.15933864322472,
126.59629305472));
#264884=CARTESIAN_POINT('Ctrl Pts',(-201.151212679701,4.27132338087164,
126.706981022484));
#264885=CARTESIAN_POINT('Ctrl Pts',(-201.14381476539,4.37894700663587,126.822201941411));
#264886=CARTESIAN_POINT('Ctrl Pts',(-201.136416851079,4.48182949379902,
126.941572123354));
#264887=CARTESIAN_POINT('Ctrl Pts',(-201.129020166166,4.58469488375913,
127.060922468139));
#264888=CARTESIAN_POINT('Ctrl Pts',(-201.121623481254,4.68282045537774,
127.184420424934));
#264889=CARTESIAN_POINT('Ctrl Pts',(-201.114226796342,4.77586463652599,
127.311647125726));
#264890=CARTESIAN_POINT('Ctrl Pts',(-201.106830439406,4.86890469199773,
127.438868185153));
#264891=CARTESIAN_POINT('Ctrl Pts',(-201.099434082471,4.95686358463872,
127.569817358517));
#264892=CARTESIAN_POINT('Ctrl Pts',(-201.092037725536,5.03944164464534,
127.704044750962));
#264893=CARTESIAN_POINT('Ctrl Pts',(-201.084640236199,5.12203234756399,
127.838292693965));
#264894=CARTESIAN_POINT('Ctrl Pts',(-201.077242746863,5.19924038189781,
127.975819537438));
#264895=CARTESIAN_POINT('Ctrl Pts',(-201.069845257526,5.27081089987097,
128.11614875458));
#264896=CARTESIAN_POINT('Ctrl Pts',(-201.062445175011,5.34240650677816,
128.25652716391));
#264897=CARTESIAN_POINT('Ctrl Pts',(-201.055045092496,5.40836049318189,
128.399709570458));
#264898=CARTESIAN_POINT('Ctrl Pts',(-201.047645009981,5.46846528047079,
128.545197489595));
#264899=CARTESIAN_POINT('Ctrl Pts',(-201.040236790314,5.52863615915231,
128.690845387655));
#264900=CARTESIAN_POINT('Ctrl Pts',(-201.032828570648,5.58294485137867,
128.838803515936));
#264901=CARTESIAN_POINT('Ctrl Pts',(-201.025420350982,5.63123274734572,
128.988555477216));
#264902=CARTESIAN_POINT('Ctrl Pts',(-201.01800757168,5.67955036370688,129.138399608329));
#264903=CARTESIAN_POINT('Ctrl Pts',(-201.010594792377,5.72183969969134,
129.290039413705));
#264904=CARTESIAN_POINT('Ctrl Pts',(-201.003182013075,5.75799294081597,
129.442946699607));
#264905=CARTESIAN_POINT('Ctrl Pts',(-200.995758642047,5.79419783938699,
129.596072466609));
#264906=CARTESIAN_POINT('Ctrl Pts',(-200.988335271018,5.82424906122381,
129.750468965729));
#264907=CARTESIAN_POINT('Ctrl Pts',(-200.980911899989,5.84809034559499,
129.905600431388));
#264908=CARTESIAN_POINT('Ctrl Pts',(-200.976975850548,5.86073156663221,
129.987854856808));
#264909=CARTESIAN_POINT('Ctrl Pts',(-200.973039801108,5.8716278209937,130.070315853689));
#264910=CARTESIAN_POINT('Ctrl Pts',(-200.969103751667,5.88077666555392,
130.152903502802));
#264911=CARTESIAN_POINT('Ctrl Pts',(-200.961680485262,5.898031100869,130.308661231559));
#264912=CARTESIAN_POINT('Ctrl Pts',(-200.954257218856,5.90911927466106,
130.465340456614));
#264913=CARTESIAN_POINT('Ctrl Pts',(-200.946833952451,5.91395173567687,
130.622411639596));
#264914=CARTESIAN_POINT('Ctrl Pts',(-200.93941945973,5.91877848512508,130.779297177483));
#264915=CARTESIAN_POINT('Ctrl Pts',(-200.932004967009,5.91736422769598,
130.936573381693));
#264916=CARTESIAN_POINT('Ctrl Pts',(-200.924590474288,5.90967099478593,
131.093703486643));
#264917=CARTESIAN_POINT('Ctrl Pts',(-200.917183127934,5.90198517690339,
131.250682143683));
#264918=CARTESIAN_POINT('Ctrl Pts',(-200.90977578158,5.88803244983971,131.40751461145));
#264919=CARTESIAN_POINT('Ctrl Pts',(-200.902368435227,5.86782683838578,
131.563662110531));
#264920=CARTESIAN_POINT('Ctrl Pts',(-200.894966613551,5.84763629703924,
131.719693148917));
#264921=CARTESIAN_POINT('Ctrl Pts',(-200.887564791876,5.82120220493272,
131.87503986722));
#264922=CARTESIAN_POINT('Ctrl Pts',(-200.880162970201,5.78859055344715,
132.029166711216));
#264923=CARTESIAN_POINT('Ctrl Pts',(-200.872765055889,5.75599611739846,
132.183212192852));
#264924=CARTESIAN_POINT('Ctrl Pts',(-200.865367141578,5.71723069365822,
132.336038718374));
#264925=CARTESIAN_POINT('Ctrl Pts',(-200.857969227266,5.67241167620617,
132.487119167727));
#264926=CARTESIAN_POINT('Ctrl Pts',(-200.850572542354,5.62760010686179,
132.63817451025));
#264927=CARTESIAN_POINT('Ctrl Pts',(-200.843175857442,5.57673704647701,
132.787483994966));
#264928=CARTESIAN_POINT('Ctrl Pts',(-200.83577917253,5.51999027249402,132.934533839178));
#264929=CARTESIAN_POINT('Ctrl Pts',(-200.828382815595,5.46324601472245,
133.081577163045));
#264930=CARTESIAN_POINT('Ctrl Pts',(-200.820986458659,5.40061869648633,
133.226360697364));
#264931=CARTESIAN_POINT('Ctrl Pts',(-200.813590101724,5.33232484821961,
133.368389142282));
#264932=CARTESIAN_POINT('Ctrl Pts',(-200.806192612387,5.26402054399037,
133.510439332119));
#264933=CARTESIAN_POINT('Ctrl Pts',(-200.79879512305,5.1900481440821,133.649733256226));
#264934=CARTESIAN_POINT('Ctrl Pts',(-200.791397633714,5.11067081254324,
133.785798929576));
#264935=CARTESIAN_POINT('Ctrl Pts',(-200.783997551199,5.03126565540398,
133.921912300536));
#264936=CARTESIAN_POINT('Ctrl Pts',(-200.776597468684,4.94645198230616,
134.054794845375));
#264937=CARTESIAN_POINT('Ctrl Pts',(-200.769197386169,4.85653698117537,
134.18400247921));
#264938=CARTESIAN_POINT('Ctrl Pts',(-200.761789166503,4.76652310925724,
134.313352190122));
#264939=CARTESIAN_POINT('Ctrl Pts',(-200.754380946836,4.67139692025517,
134.439018613408));
#264940=CARTESIAN_POINT('Ctrl Pts',(-200.74697272717,4.57150714130225,134.560589180836));
#264941=CARTESIAN_POINT('Ctrl Pts',(-200.739559947868,4.47155588185713,
134.682234572919));
#264942=CARTESIAN_POINT('Ctrl Pts',(-200.732147168566,4.36683543800591,
134.799778807794));
#264943=CARTESIAN_POINT('Ctrl Pts',(-200.724734389264,4.25773191773792,
134.912845676462));
#264944=CARTESIAN_POINT('Ctrl Pts',(-200.717311018235,4.14847250524356,
135.026074100376));
#264945=CARTESIAN_POINT('Ctrl Pts',(-200.709887647206,4.03481777724236,
135.134812123521));
#264946=CARTESIAN_POINT('Ctrl Pts',(-200.702464276177,3.91718807819064,
135.238722817768));
#264947=CARTESIAN_POINT('Ctrl Pts',(-200.698528226736,3.85481798926586,
135.293818761162));
#264948=CARTESIAN_POINT('Ctrl Pts',(-200.694592177296,3.79133090880903,
135.347558271593));
#264949=CARTESIAN_POINT('Ctrl Pts',(-200.690656127855,3.72679275456151,
135.399896095293));
#264950=CARTESIAN_POINT('Ctrl Pts',(-200.683232861449,3.60507580982061,
135.498603597382));
#264951=CARTESIAN_POINT('Ctrl Pts',(-200.675809595044,3.4792505691735,135.592621340272));
#264952=CARTESIAN_POINT('Ctrl Pts',(-200.668386328638,3.34971419766227,
135.681587837666));
#264953=CARTESIAN_POINT('Ctrl Pts',(-200.660971835917,3.22033092738485,
135.770449184047));
#264954=CARTESIAN_POINT('Ctrl Pts',(-200.653557343196,3.08724556180289,
135.854270959279));
#264955=CARTESIAN_POINT('Ctrl Pts',(-200.646142850475,2.95088917404671,
135.93273108439));
#264956=CARTESIAN_POINT('Ctrl Pts',(-200.638735504121,2.81466421171077,
136.011115586678));
#264957=CARTESIAN_POINT('Ctrl Pts',(-200.631328157768,2.67517482505955,
136.084148541912));
#264958=CARTESIAN_POINT('Ctrl Pts',(-200.623920811414,2.53288188521501,
136.151550526111));
#264959=CARTESIAN_POINT('Ctrl Pts',(-200.616518989738,2.3906950728134,136.218902239368));
#264960=CARTESIAN_POINT('Ctrl Pts',(-200.609117168063,2.24570920658458,
136.280631184824));
#264961=CARTESIAN_POINT('Ctrl Pts',(-200.601715346387,2.09841053341921,
136.336503402757));
#264962=CARTESIAN_POINT('Ctrl Pts',(-200.594317432076,1.95118961807727,
136.39234612618));
#264963=CARTESIAN_POINT('Ctrl Pts',(-200.586919517765,1.80165867545395,
136.442338147334));
#264964=CARTESIAN_POINT('Ctrl Pts',(-200.579521603453,1.65032464089478,
136.486293311831));
#264965=CARTESIAN_POINT('Ctrl Pts',(-200.572124918541,1.49901575530602,
136.530241171777));
#264966=CARTESIAN_POINT('Ctrl Pts',(-200.564728233629,1.34590473061233,
136.568154062135));
#264967=CARTESIAN_POINT('Ctrl Pts',(-200.557331548716,1.19151451455393,
136.599895426719));
#264968=CARTESIAN_POINT('Ctrl Pts',(-200.549935191781,1.03713114431951,
136.631635383858));
#264969=CARTESIAN_POINT('Ctrl Pts',(-200.542538834845,0.881469061150174,
136.657204284162));
#264970=CARTESIAN_POINT('Ctrl Pts',(-200.53514247791,0.725062014826754,
136.676516579149));
#264971=CARTESIAN_POINT('Ctrl Pts',(-200.527744988573,0.568631022185253,
136.695831830898));
#264972=CARTESIAN_POINT('Ctrl Pts',(-200.520347499237,0.411455209797665,
136.708888524271));
#264973=CARTESIAN_POINT('Ctrl Pts',(-200.5129500099,0.254073918632435,136.715652947198));
#264974=CARTESIAN_POINT('Ctrl Pts',(-200.505549927385,0.0966374576993343,
136.722419741384));
#264975=CARTESIAN_POINT('Ctrl Pts',(-200.49814984487,-0.0610042527022276,
136.72288985748));
#264976=CARTESIAN_POINT('Ctrl Pts',(-200.490749762355,-0.218311548806333,
136.717081702664));
#264977=CARTESIAN_POINT('Ctrl Pts',(-200.483341542688,-0.375791820453863,
136.711267161183));
#264978=CARTESIAN_POINT('Ctrl Pts',(-200.475933323022,-0.532936570164552,
136.699160575621));
#264979=CARTESIAN_POINT('Ctrl Pts',(-200.468525103355,-0.689210197067142,
136.680832336783));
#264980=CARTESIAN_POINT('Ctrl Pts',(-200.461112324053,-0.845580007779526,
136.66249281722));
#264981=CARTESIAN_POINT('Ctrl Pts',(-200.453699544751,-1.00107725944581,
136.637924072098));
#264982=CARTESIAN_POINT('Ctrl Pts',(-200.446286765449,-1.15517673598396,
136.607247594851));
#264983=CARTESIAN_POINT('Ctrl Pts',(-200.43886339442,-1.30949639708053,
136.576527285615));
#264984=CARTESIAN_POINT('Ctrl Pts',(-200.431440023392,-1.4624139322289,
136.539681901662));
#264985=CARTESIAN_POINT('Ctrl Pts',(-200.424016652363,-1.61341866780536,
136.496882972803));
#264986=CARTESIAN_POINT('Ctrl Pts',(-200.420080602922,-1.69348500191474,
136.474189953777));
#264987=CARTESIAN_POINT('Ctrl Pts',(-200.416144553482,-1.77301389176252,
136.449823992991));
#264988=CARTESIAN_POINT('Ctrl Pts',(-200.412208504041,-1.85193163392452,
136.423816088141));
#264989=CARTESIAN_POINT('Ctrl Pts',(-200.404785237635,-2.00076803270955,
136.37476599127));
#264990=CARTESIAN_POINT('Ctrl Pts',(-200.39736197123,-2.14787943854751,
136.3197245393));
#264991=CARTESIAN_POINT('Ctrl Pts',(-200.389938704824,-2.29274704537207,
136.258830486255));
#264992=CARTESIAN_POINT('Ctrl Pts',(-200.382524212103,-2.43744343071588,
136.198008404924));
#264993=CARTESIAN_POINT('Ctrl Pts',(-200.375109719382,-2.57990095506391,
136.131347634659));
#264994=CARTESIAN_POINT('Ctrl Pts',(-200.367695226661,-2.71961563869954,
136.059036757942));
#264995=CARTESIAN_POINT('Ctrl Pts',(-200.360287880307,-2.85919566006293,
135.986795577171));
#264996=CARTESIAN_POINT('Ctrl Pts',(-200.352880533953,-2.99603777440594,
135.908915301869));
#264997=CARTESIAN_POINT('Ctrl Pts',(-200.3454731876,-3.1296577823218,135.825632640475));
#264998=CARTESIAN_POINT('Ctrl Pts',(-200.338071365924,-3.26317813139457,
135.742412094433));
#264999=CARTESIAN_POINT('Ctrl Pts',(-200.330669544249,-3.39348084363586,
135.653797381792));
#265000=CARTESIAN_POINT('Ctrl Pts',(-200.323267722573,-3.52010625378327,
135.560071134889));
#265001=CARTESIAN_POINT('Ctrl Pts',(-200.315869808262,-3.64666481936232,
135.466394365342));
#265002=CARTESIAN_POINT('Ctrl Pts',(-200.30847189395,-3.76954964959203,
135.367611656931));
#265003=CARTESIAN_POINT('Ctrl Pts',(-200.301073979639,-3.88833011657844,
135.264048887727));
#265004=CARTESIAN_POINT('Ctrl Pts',(-200.293677294726,-4.00709084440596,
135.160503328776));
#265005=CARTESIAN_POINT('Ctrl Pts',(-200.286280609814,-4.12174828160482,
135.052179530682));
#265006=CARTESIAN_POINT('Ctrl Pts',(-200.278883924902,-4.23190487356255,
134.939443652236));
#265007=CARTESIAN_POINT('Ctrl Pts',(-200.271487567967,-4.34205658106188,
134.826712772617));
#265008=CARTESIAN_POINT('Ctrl Pts',(-200.264091211031,-4.44770757924775,
134.709570468634));
#265009=CARTESIAN_POINT('Ctrl Pts',(-200.256694854095,-4.5484973889659,
134.588419558052));
#265010=CARTESIAN_POINT('Ctrl Pts',(-200.249297364759,-4.64930262986123,
134.467250098956));
#265011=CARTESIAN_POINT('Ctrl Pts',(-200.241899875422,-4.74524496160936,
134.342071098237));
#265012=CARTESIAN_POINT('Ctrl Pts',(-200.234502386085,-4.83600449432356,
134.21331809653));
#265013=CARTESIAN_POINT('Ctrl Pts',(-200.22710230357,-4.92679584265112,
134.084519960658));
#265014=CARTESIAN_POINT('Ctrl Pts',(-200.219702221055,-5.01240055972236,
133.952145634283));
#265015=CARTESIAN_POINT('Ctrl Pts',(-200.21230213854,-5.09254243056786,
133.816659101343));
#265016=CARTESIAN_POINT('Ctrl Pts',(-200.204893918873,-5.17277242563903,
133.681023587033));
#265017=CARTESIAN_POINT('Ctrl Pts',(-200.197485699207,-5.24752738802124,
133.542269353312));
#265018=CARTESIAN_POINT('Ctrl Pts',(-200.19007747954,-5.31657703414016,
133.400885064313));
#265019=CARTESIAN_POINT('Ctrl Pts',(-200.182664700238,-5.38566917916411,
133.259413755643));
#265020=CARTESIAN_POINT('Ctrl Pts',(-200.175251920936,-5.44904886082607,
133.115309507039));
#265021=CARTESIAN_POINT('Ctrl Pts',(-200.167839141634,-5.50653440287247,
132.969079867834));
#265022=CARTESIAN_POINT('Ctrl Pts',(-200.160415770605,-5.56410208295706,
132.822641288864));
#265023=CARTESIAN_POINT('Ctrl Pts',(-200.152992399576,-5.615758680887,132.674071605666));
#265024=CARTESIAN_POINT('Ctrl Pts',(-200.145569028547,-5.66137247798355,
132.523893178476));
#265025=CARTESIAN_POINT('Ctrl Pts',(-200.141632979107,-5.68555800768561,
132.44426497292));
#265026=CARTESIAN_POINT('Ctrl Pts',(-200.137696929668,-5.70804554235413,
132.364184668557));
#265027=CARTESIAN_POINT('Ctrl Pts',(-200.133760880228,-5.7288213227283,
132.283731029178));
#265028=CARTESIAN_POINT('Ctrl Pts',(-200.124071939592,-5.77996277961027,
132.085687140804));
#265029=CARTESIAN_POINT('Ctrl Pts',(-200.114382998956,-5.82085499360012,
131.88489595805));
#265030=CARTESIAN_POINT('Ctrl Pts',(-200.10469405832,-5.85125580823402,
131.682276347638));
#265031=CARTESIAN_POINT('Ctrl Pts',(-200.095203709521,-5.88103350483466,
131.483809781632));
#265032=CARTESIAN_POINT('Ctrl Pts',(-200.085713360723,-5.90074552551159,
131.283588737847));
#265033=CARTESIAN_POINT('Ctrl Pts',(-200.076223011924,-5.91020894769956,
131.082498635521));
#265034=CARTESIAN_POINT('Ctrl Pts',(-200.071940411166,-5.91447939759482,
130.991755013462));
#265035=CARTESIAN_POINT('Ctrl Pts',(-200.067657810408,-5.91666348839728,
130.900834742462));
#265036=CARTESIAN_POINT('Ctrl Pts',(-200.06337520965,-5.91674748049752,
130.809820885532));
#265037=CARTESIAN_POINT('',(-203.563375192208,-5.91198242686231,130.79947290462));
#265038=CARTESIAN_POINT('Ctrl Pts',(-203.563375192208,-5.91198242686231,
130.79947290462));
#265039=CARTESIAN_POINT('Ctrl Pts',(-203.5339609168,-5.91683243646446,130.173526639722));
#265040=CARTESIAN_POINT('Ctrl Pts',(-203.504546641391,-5.82534361100667,
129.54896166662));
#265041=CARTESIAN_POINT('Ctrl Pts',(-203.382316491379,-5.02009495809496,
127.092968345155));
#265042=CARTESIAN_POINT('Ctrl Pts',(-203.196684742167,-1.76012566321133,
124.030918495546));
#265043=CARTESIAN_POINT('Ctrl Pts',(-202.918237118359,4.74729777661893,
125.662306130287));
#265044=CARTESIAN_POINT('Ctrl Pts',(-202.639789494544,6.89218647818192,
132.018990635446));
#265045=CARTESIAN_POINT('Ctrl Pts',(-202.361341870732,2.70349250829908,
137.25948949219));
#265046=CARTESIAN_POINT('Ctrl Pts',(-202.085870845849,-3.89824401710562,
136.575431840637));
#265047=CARTESIAN_POINT('Ctrl Pts',(-201.90321569557,-5.92108948216704,
132.703162475868));
#265048=CARTESIAN_POINT('Ctrl Pts',(-201.813376419895,-5.92624986544025,
130.803210827386));
#265049=CARTESIAN_POINT('',(-205.313375192208,-5.90857914829821,130.807499840963));
#265050=CARTESIAN_POINT('Ctrl Pts',(-205.313375192208,-5.90857914829821,
130.807499840963));
#265051=CARTESIAN_POINT('Ctrl Pts',(-205.257522831092,-5.90287670038602,
129.617221394239));
#265052=CARTESIAN_POINT('Ctrl Pts',(-205.108854595372,-4.97542928644342,
126.440754491598));
#265053=CARTESIAN_POINT('Ctrl Pts',(-204.867370485048,0.213664449080756,
123.809226020325));
#265054=CARTESIAN_POINT('Ctrl Pts',(-204.588922861234,6.00069570294186,
127.203081454398));
#265055=CARTESIAN_POINT('Ctrl Pts',(-204.310475237422,6.27338075607734,
133.906336507158));
#265056=CARTESIAN_POINT('Ctrl Pts',(-204.032027613609,0.781135366069192,
137.759027257328));
#265057=CARTESIAN_POINT('Ctrl Pts',(-203.782994265204,-4.77292417967637,
135.488857499412));
#265058=CARTESIAN_POINT('Ctrl Pts',(-203.626776791404,-5.90152837485451,
132.148681533904));
#265059=CARTESIAN_POINT('Ctrl Pts',(-203.563375192208,-5.91198242686231,
130.79947290462));
#265060=CARTESIAN_POINT('',(-207.063375192208,-5.92350094233479,130.808116397466));
#265061=CARTESIAN_POINT('Ctrl Pts',(-207.063375192208,-5.92350094233479,
130.808116397466));
#265062=CARTESIAN_POINT('Ctrl Pts',(-206.981084745385,-5.91062028060458,
129.06567203012));
#265063=CARTESIAN_POINT('Ctrl Pts',(-206.805978423956,-4.17532705327718,
125.335613429113));
#265064=CARTESIAN_POINT('Ctrl Pts',(-206.538056227925,2.17024453367553,
124.150970564787));
#265065=CARTESIAN_POINT('Ctrl Pts',(-206.259608604111,6.77075566682168,
129.033928966654));
#265066=CARTESIAN_POINT('Ctrl Pts',(-205.981160980299,5.14927311196064,
135.543827565311));
#265067=CARTESIAN_POINT('Ctrl Pts',(-205.702713356486,-1.20413987681471,
137.698387574825));
#265068=CARTESIAN_POINT('Ctrl Pts',(-205.480118093789,-5.39856531937876,
134.356261281287));
#265069=CARTESIAN_POINT('Ctrl Pts',(-205.350338705697,-5.91235307129998,
131.595235086907));
#265070=CARTESIAN_POINT('Ctrl Pts',(-205.313375192208,-5.90857914829821,
130.807499840963));
#265071=CARTESIAN_POINT('Ctrl Pts',(-207.299567498839,-3.90840034609405,
135.243902605345));
#265072=CARTESIAN_POINT('Ctrl Pts',(-207.231362157743,-4.98707972514044,
134.275313217871));
#265073=CARTESIAN_POINT('Ctrl Pts',(-207.152631388866,-5.83925384327957,
132.696773286164));
#265074=CARTESIAN_POINT('Ctrl Pts',(-207.073900619989,-5.92514845404535,
131.030985187931));
#265075=CARTESIAN_POINT('Ctrl Pts',(-207.063375192208,-5.92350094233479,
130.808116397466));
#265076=CARTESIAN_POINT('Origin',(213.235140564004,0.,130.804360617566));
#265077=CARTESIAN_POINT('',(-177.889859436045,-4.91824981877161,130.80302545727));
#265078=CARTESIAN_POINT('Ctrl Pts',(-177.889859436045,-4.91824981877161,
130.80302545727));
#265079=CARTESIAN_POINT('Ctrl Pts',(-177.897578984021,-4.91828660513675,
130.938533181825));
#265080=CARTESIAN_POINT('Ctrl Pts',(-177.905298531998,-4.91271888509105,
131.074267759702));
#265081=CARTESIAN_POINT('Ctrl Pts',(-177.913018079974,-4.90151653121722,
131.209723117934));
#265082=CARTESIAN_POINT('Ctrl Pts',(-177.920728283118,-4.89032773825667,
131.345014501845));
#265083=CARTESIAN_POINT('Ctrl Pts',(-177.928438486262,-4.87351791200395,
131.480026946718));
#265084=CARTESIAN_POINT('Ctrl Pts',(-177.936148689406,-4.85110890292581,
131.614252878582));
#265085=CARTESIAN_POINT('Ctrl Pts',(-177.943851468977,-4.82872146979285,
131.748349574418));
#265086=CARTESIAN_POINT('Ctrl Pts',(-177.951554248548,-4.80074564454809,
131.881660874833));
#265087=CARTESIAN_POINT('Ctrl Pts',(-177.959257028118,-4.76725516232351,
132.013683270872));
#265088=CARTESIAN_POINT('Ctrl Pts',(-177.966954298254,-4.73378863426308,
132.145611237511));
#265089=CARTESIAN_POINT('Ctrl Pts',(-177.974651568389,-4.69481539576988,
132.276251751023));
#265090=CARTESIAN_POINT('Ctrl Pts',(-177.982348838524,-4.65046036686952,
132.405110891243));
#265091=CARTESIAN_POINT('Ctrl Pts',(-177.990043303124,-4.60612150469107,
132.533923064299));
#265092=CARTESIAN_POINT('Ctrl Pts',(-177.997737767723,-4.55640488027498,
132.660954780006));
#265093=CARTESIAN_POINT('Ctrl Pts',(-178.005432232323,-4.5014853573474,
132.785726974424));
#265094=CARTESIAN_POINT('Ctrl Pts',(-178.013125478951,-4.44657452773564,
132.910479418413));
#265095=CARTESIAN_POINT('Ctrl Pts',(-178.020818725579,-4.38646259723445,
133.03297268916));
#265096=CARTESIAN_POINT('Ctrl Pts',(-178.028511972207,-4.32137249872143,
133.152747891802));
#265097=CARTESIAN_POINT('Ctrl Pts',(-178.036205725472,-4.25627811371228,
133.272530982217));
#265098=CARTESIAN_POINT('Ctrl Pts',(-178.043899478737,-4.18620509819149,
133.389595299688));
#265099=CARTESIAN_POINT('Ctrl Pts',(-178.051593232003,-4.11142201299136,
133.503507166679));
#265100=CARTESIAN_POINT('Ctrl Pts',(-178.059289216561,-4.03661723967682,
133.617452069665));
#265101=CARTESIAN_POINT('Ctrl Pts',(-178.06698520112,-3.95709989735997,
133.72824237193));
#265102=CARTESIAN_POINT('Ctrl Pts',(-178.074681185679,-3.87318119104158,
133.835474360708));
#265103=CARTESIAN_POINT('Ctrl Pts',(-178.082385491664,-3.78917174605771,
133.942822296072));
#265104=CARTESIAN_POINT('Ctrl Pts',(-178.09008979765,-3.70075168025727,
134.046603923423));
#265105=CARTESIAN_POINT('Ctrl Pts',(-178.097794103635,-3.60827196007457,
134.146449264601));
#265106=CARTESIAN_POINT('Ctrl Pts',(-178.105503084718,-3.5157361216954,
134.246355193554));
#265107=CARTESIAN_POINT('Ctrl Pts',(-178.113212065802,-3.41913600421425,
134.342319800581));
#265108=CARTESIAN_POINT('Ctrl Pts',(-178.120921046885,-3.31885770099228,
134.434011650801));
#265109=CARTESIAN_POINT('Ctrl Pts',(-178.128641384245,-3.21843167550299,
134.525838574388));
#265110=CARTESIAN_POINT('Ctrl Pts',(-178.136361721606,-3.11431694878514,
134.61337991927));
#265111=CARTESIAN_POINT('Ctrl Pts',(-178.144082058966,-3.00693114976664,
134.696345730983));
#265112=CARTESIAN_POINT('Ctrl Pts',(-178.148050571034,-2.9517312511805,
134.738992937919));
#265113=CARTESIAN_POINT('Ctrl Pts',(-178.152019083102,-2.89566748822361,
134.780431866513));
#265114=CARTESIAN_POINT('Ctrl Pts',(-178.15598759517,-2.83879919740751,
134.820627812275));
#265115=CARTESIAN_POINT('Ctrl Pts',(-178.163761929289,-2.72739394374767,
134.899371862246));
#265116=CARTESIAN_POINT('Ctrl Pts',(-178.171536263408,-2.61253338564665,
134.973601801254));
#265117=CARTESIAN_POINT('Ctrl Pts',(-178.179310597527,-2.49461950041102,
135.04299915024));
#265118=CARTESIAN_POINT('Ctrl Pts',(-178.187075350474,-2.37685093350067,
135.112310973196));
#265119=CARTESIAN_POINT('Ctrl Pts',(-178.194840103421,-2.25603686031665,
135.176801859868));
#265120=CARTESIAN_POINT('Ctrl Pts',(-178.202604856368,-2.13261028670629,
135.236195048988));
#265121=CARTESIAN_POINT('Ctrl Pts',(-178.210361897253,-2.00930630210852,
135.295529247955));
#265122=CARTESIAN_POINT('Ctrl Pts',(-178.218118938138,-1.88339533081727,
135.349775656748));
#265123=CARTESIAN_POINT('Ctrl Pts',(-178.225875979023,-1.75533686375186,
135.39870230678));
#265124=CARTESIAN_POINT('Ctrl Pts',(-178.233627170264,-1.6273749665728,
135.447592060845));
#265125=CARTESIAN_POINT('Ctrl Pts',(-178.241378361504,-1.49726916076229,
135.491169902165));
#265126=CARTESIAN_POINT('Ctrl Pts',(-178.249129552744,-1.36550057426087,
135.529251224151));
#265127=CARTESIAN_POINT('Ctrl Pts',(-178.256877449521,-1.23378799292357,
135.567316360559));
#265128=CARTESIAN_POINT('Ctrl Pts',(-178.264625346298,-1.10041441132796,
135.599889515772));
#265129=CARTESIAN_POINT('Ctrl Pts',(-178.272373243075,-0.965877633492174,
135.626835444833));
#265130=CARTESIAN_POINT('Ctrl Pts',(-178.280119519159,-0.831368997850033,
135.653775737386));
#265131=CARTESIAN_POINT('Ctrl Pts',(-178.287865795243,-0.695698033044637,
135.675091068361));
#265132=CARTESIAN_POINT('Ctrl Pts',(-178.295612071327,-0.559373905331694,
135.690697066945));
#265133=CARTESIAN_POINT('Ctrl Pts',(-178.303358404593,-0.423048771305566,
135.706303180729));
#265134=CARTESIAN_POINT('Ctrl Pts',(-178.311104737858,-0.286070853179251,
135.716199833558));
#265135=CARTESIAN_POINT('Ctrl Pts',(-178.318851071123,-0.148955232533464,
135.720354454137));
#265136=CARTESIAN_POINT('Ctrl Pts',(-178.326599139126,-0.01180890579494,
135.724510005114));
#265137=CARTESIAN_POINT('Ctrl Pts',(-178.334347207129,0.125474794115099,
135.722920953233));
#265138=CARTESIAN_POINT('Ctrl Pts',(-178.342095275132,0.262380385697254,
135.715606854083));
#265139=CARTESIAN_POINT('Ctrl Pts',(-178.349851577874,0.399431482171527,
135.708284981421));
#265140=CARTESIAN_POINT('Ctrl Pts',(-178.357607880616,0.536103276532238,
135.695225927641));
#265141=CARTESIAN_POINT('Ctrl Pts',(-178.365364183358,0.671884454715865,
135.676501249979));
#265142=CARTESIAN_POINT('Ctrl Pts',(-178.373124625872,0.807738103402582,
135.657766578393));
#265143=CARTESIAN_POINT('Ctrl Pts',(-178.380885068386,0.942699804202917,
135.63336032706));
#265144=CARTESIAN_POINT('Ctrl Pts',(-178.3886455109,1.0762690282611,135.603405110098));
#265145=CARTESIAN_POINT('Ctrl Pts',(-178.396418411166,1.21005266949546,
135.573401806363));
#265146=CARTESIAN_POINT('Ctrl Pts',(-178.404191311431,1.34243898930015,
135.537831838098));
#265147=CARTESIAN_POINT('Ctrl Pts',(-178.411964211697,1.47294233469106,
135.496867830259));
#265148=CARTESIAN_POINT('Ctrl Pts',(-178.419454547459,1.59870155475822,
135.457392967287));
#265149=CARTESIAN_POINT('Ctrl Pts',(-178.426944883221,1.72271203539251,
135.412909533879));
#265150=CARTESIAN_POINT('Ctrl Pts',(-178.434435218983,1.8445590297808,135.363613302837));
#265151=CARTESIAN_POINT('Ctrl Pts',(-178.442209553102,1.97102588999646,
135.312447990212));
#265152=CARTESIAN_POINT('Ctrl Pts',(-178.449983887221,2.09556257726352,
135.255935644863));
#265153=CARTESIAN_POINT('Ctrl Pts',(-178.45775822134,2.21768386757729,135.194242315971));
#265154=CARTESIAN_POINT('Ctrl Pts',(-178.465522974287,2.33965465431505,
135.132625018593));
#265155=CARTESIAN_POINT('Ctrl Pts',(-178.473287727234,2.45921562135268,
135.065839616714));
#265156=CARTESIAN_POINT('Ctrl Pts',(-178.481052480181,2.57589987136006,
134.994100814192));
#265157=CARTESIAN_POINT('Ctrl Pts',(-178.488809521066,2.69246822892538,
134.922433263661));
#265158=CARTESIAN_POINT('Ctrl Pts',(-178.496566561951,2.80616522451045,
134.845822306524));
#265159=CARTESIAN_POINT('Ctrl Pts',(-178.504323602836,2.91654733030766,
134.76452914082));
#265160=CARTESIAN_POINT('Ctrl Pts',(-178.512074794076,3.02684619610039,
134.683297278925));
#265161=CARTESIAN_POINT('Ctrl Pts',(-178.519825985316,3.13383483424316,
134.59739046739));
#265162=CARTESIAN_POINT('Ctrl Pts',(-178.527577176556,3.23709786857969,
134.507113708408));
#265163=CARTESIAN_POINT('Ctrl Pts',(-178.535325073334,3.34031701337215,
134.416875319456));
#265164=CARTESIAN_POINT('Ctrl Pts',(-178.543072970111,3.43981341005556,
134.322270933959));
#265165=CARTESIAN_POINT('Ctrl Pts',(-178.550820866888,3.53520419798672,
134.223646265335));
#265166=CARTESIAN_POINT('Ctrl Pts',(-178.558567142972,3.63057503222116,
134.125042226865));
#265167=CARTESIAN_POINT('Ctrl Pts',(-178.566313419056,3.72184169427708,
134.022419858821));
#265168=CARTESIAN_POINT('Ctrl Pts',(-178.57405969514,3.80865798380126,133.916161932709));
#265169=CARTESIAN_POINT('Ctrl Pts',(-178.581806028405,3.89547491418369,
133.809903222225));
#265170=CARTESIAN_POINT('Ctrl Pts',(-178.589552361671,3.97784115911567,
133.700009202882));
#265171=CARTESIAN_POINT('Ctrl Pts',(-178.597298694936,4.05545090126791,
133.586895621821));
#265172=CARTESIAN_POINT('Ctrl Pts',(-178.605046762939,4.1330780235839,133.473756709758));
#265173=CARTESIAN_POINT('Ctrl Pts',(-178.612794830942,4.20594630237465,
133.357397123591));
#265174=CARTESIAN_POINT('Ctrl Pts',(-178.620542898945,4.27379355996916,
133.238261122777));
#265175=CARTESIAN_POINT('Ctrl Pts',(-178.628299201687,4.34171292643635,
133.118998502804));
#265176=CARTESIAN_POINT('Ctrl Pts',(-178.636055504429,4.40460041788537,
132.996953913909));
#265177=CARTESIAN_POINT('Ctrl Pts',(-178.643811807171,4.46223985970607,
132.872596217528));
#265178=CARTESIAN_POINT('Ctrl Pts',(-178.651572249685,4.51991006543252,
132.7481721477));
#265179=CARTESIAN_POINT('Ctrl Pts',(-178.659332692199,4.57232649087066,
132.621432871501));
#265180=CARTESIAN_POINT('Ctrl Pts',(-178.667093134713,4.6193217466782,132.492865773959));
#265181=CARTESIAN_POINT('Ctrl Pts',(-178.674866034979,4.66639244344228,
132.364092289099));
#265182=CARTESIAN_POINT('Ctrl Pts',(-178.682638935244,4.70802446131689,
132.233485492179));
#265183=CARTESIAN_POINT('Ctrl Pts',(-178.69041183551,4.7441005272662,132.101547284817));
#265184=CARTESIAN_POINT('Ctrl Pts',(-178.697902171271,4.77886513734783,
131.974405363625));
#265185=CARTESIAN_POINT('Ctrl Pts',(-178.705392507033,4.80847065889238,
131.846027451783));
#265186=CARTESIAN_POINT('Ctrl Pts',(-178.712882842795,4.83285762032032,
131.716868307513));
#265187=CARTESIAN_POINT('Ctrl Pts',(-178.720657176914,4.85816922080323,
131.58281205503));
#265188=CARTESIAN_POINT('Ctrl Pts',(-178.728431511034,4.87793890559331,
131.447489509917));
#265189=CARTESIAN_POINT('Ctrl Pts',(-178.736205845153,4.89204410114357,
131.311398658512));
#265190=CARTESIAN_POINT('Ctrl Pts',(-178.7439705981,4.90613191330093,131.175475526918));
#265191=CARTESIAN_POINT('Ctrl Pts',(-178.751735351047,4.91456908636255,
131.038786358168));
#265192=CARTESIAN_POINT('Ctrl Pts',(-178.759500103994,4.91728388735268,
130.901840018886));
#265193=CARTESIAN_POINT('Ctrl Pts',(-178.767257144879,4.9199959919642,130.765029696639));
#265194=CARTESIAN_POINT('Ctrl Pts',(-178.775014185764,4.91699702730776,
130.627963100528));
#265195=CARTESIAN_POINT('Ctrl Pts',(-178.782771226649,4.90826700907514,
130.491154566979));
#265196=CARTESIAN_POINT('Ctrl Pts',(-178.790522417889,4.89954357421716,
130.354449201808));
#265197=CARTESIAN_POINT('Ctrl Pts',(-178.798273609129,4.88509771292451,
130.218001900438));
#265198=CARTESIAN_POINT('Ctrl Pts',(-178.806024800369,4.86496151122054,
130.082326991727));
#265199=CARTESIAN_POINT('Ctrl Pts',(-178.813772697147,4.84483386793941,
129.946709748471));
#265200=CARTESIAN_POINT('Ctrl Pts',(-178.821520593924,4.81902075182776,
129.811864630855));
#265201=CARTESIAN_POINT('Ctrl Pts',(-178.829268490701,4.78760607584458,
129.678300616928));
#265202=CARTESIAN_POINT('Ctrl Pts',(-178.837014766785,4.75619797113449,
129.544764541714));
#265203=CARTESIAN_POINT('Ctrl Pts',(-178.844761042869,4.71919072663617,
129.412509417502));
#265204=CARTESIAN_POINT('Ctrl Pts',(-178.852507318953,4.67671924911073,
129.282033409802));
#265205=CARTESIAN_POINT('Ctrl Pts',(-178.860253652219,4.63424745807043,
129.151556438958));
#265206=CARTESIAN_POINT('Ctrl Pts',(-178.867999985484,4.58631147452994,
129.022858982598));
#265207=CARTESIAN_POINT('Ctrl Pts',(-178.875746318749,4.53309577659699,
128.896423054987));
#265208=CARTESIAN_POINT('Ctrl Pts',(-178.883494386752,4.47986816137724,
128.769958812926));
#265209=CARTESIAN_POINT('Ctrl Pts',(-178.891242454755,4.42135863065274,
128.645757467678));
#265210=CARTESIAN_POINT('Ctrl Pts',(-178.898990522758,4.35779923905243,
128.524279729831));
#265211=CARTESIAN_POINT('Ctrl Pts',(-178.9067468255,4.29417229577462,128.402672883999));
#265212=CARTESIAN_POINT('Ctrl Pts',(-178.914503128242,4.22548495189499,
128.283795774974));
#265213=CARTESIAN_POINT('Ctrl Pts',(-178.922259430984,4.15201482616275,
128.168083707637));
#265214=CARTESIAN_POINT('Ctrl Pts',(-178.930019873498,4.07850548721226,
128.052309881286));
#265215=CARTESIAN_POINT('Ctrl Pts',(-178.937780316012,4.00020850299509,
127.93970478349));
#265216=CARTESIAN_POINT('Ctrl Pts',(-178.945540758526,3.91744344631057,
127.830672687157));
#265217=CARTESIAN_POINT('Ctrl Pts',(-178.953313658792,3.83454552780952,
127.721465562824));
#265218=CARTESIAN_POINT('Ctrl Pts',(-178.961086559057,3.74716545316439,
127.615843203123));
#265219=CARTESIAN_POINT('Ctrl Pts',(-178.968859459323,3.65566209747847,
127.514175563263));
#265220=CARTESIAN_POINT('Ctrl Pts',(-178.976349795085,3.56748511925551,
127.416203798198));
#265221=CARTESIAN_POINT('Ctrl Pts',(-178.983840130847,3.47547965372134,
127.321904437295));
#265222=CARTESIAN_POINT('Ctrl Pts',(-178.991330466609,3.37999615600626,
127.231573323606));
#265223=CARTESIAN_POINT('Ctrl Pts',(-178.999104800728,3.28089237245302,
127.137817278285));
#265224=CARTESIAN_POINT('Ctrl Pts',(-179.006879134847,3.17772768024682,
127.048039341494));
#265225=CARTESIAN_POINT('Ctrl Pts',(-179.014653468966,3.07085479539997,
126.962611811609));
#265226=CARTESIAN_POINT('Ctrl Pts',(-179.022418221913,2.9641136218319,126.87728956352));
#265227=CARTESIAN_POINT('Ctrl Pts',(-179.03018297486,2.85367365105237,126.796307296342));
#265228=CARTESIAN_POINT('Ctrl Pts',(-179.037947727807,2.73992423354038,
126.720000415899));
#265229=CARTESIAN_POINT('Ctrl Pts',(-179.045704768692,2.62628779355376,
126.643769324527));
#265230=CARTESIAN_POINT('Ctrl Pts',(-179.053461809577,2.50934877066748,
126.572204595192));
#265231=CARTESIAN_POINT('Ctrl Pts',(-179.061218850462,2.38952908867568,
126.50560105266));
#265232=CARTESIAN_POINT('Ctrl Pts',(-179.068970041702,2.26979976363732,
126.439047736377));
#265233=CARTESIAN_POINT('Ctrl Pts',(-179.076721232943,2.14719444371695,
126.377448349309));
#265234=CARTESIAN_POINT('Ctrl Pts',(-179.084472424183,2.02216319162956,
126.321053903887));
#265235=CARTESIAN_POINT('Ctrl Pts',(-179.09222032096,1.89718508116047,126.264683427609));
#265236=CARTESIAN_POINT('Ctrl Pts',(-179.099968217737,1.76978344491984,
126.213513653413));
#265237=CARTESIAN_POINT('Ctrl Pts',(-179.107716114514,1.64043185755897,
126.167749098018));
#265238=CARTESIAN_POINT('Ctrl Pts',(-179.115462390598,1.51110732776167,
126.121994115581));
#265239=CARTESIAN_POINT('Ctrl Pts',(-179.123208666682,1.37983402649866,
126.08164223333));
#265240=CARTESIAN_POINT('Ctrl Pts',(-179.130954942766,1.24710399492245,
126.046849221011));
#265241=CARTESIAN_POINT('Ctrl Pts',(-179.138701276032,1.11437298356347,
126.012055951859));
#265242=CARTESIAN_POINT('Ctrl Pts',(-179.146447609297,0.980185598621585,
125.982821733656));
#265243=CARTESIAN_POINT('Ctrl Pts',(-179.154193942562,0.845047087272823,
125.959251900231));
#265244=CARTESIAN_POINT('Ctrl Pts',(-179.161942010565,0.709878312591245,
125.935676788506));
#265245=CARTESIAN_POINT('Ctrl Pts',(-179.169690078568,0.573758372738378,
125.917768652887));
#265246=CARTESIAN_POINT('Ctrl Pts',(-179.177438146571,0.437200307775627,
125.905581284571));
#265247=CARTESIAN_POINT('Ctrl Pts',(-179.185194449313,0.300497107276185,
125.893380963375));
#265248=CARTESIAN_POINT('Ctrl Pts',(-179.192950752055,0.163355241530021,
125.886913589944));
#265249=CARTESIAN_POINT('Ctrl Pts',(-179.200707054797,0.0262910045776176,
125.886180888685));
#265250=CARTESIAN_POINT('Ctrl Pts',(-179.208467497311,-0.110846387685345,
125.885447796361));
#265251=CARTESIAN_POINT('Ctrl Pts',(-179.216227939825,-0.247905678082787,
125.890455460777));
#265252=CARTESIAN_POINT('Ctrl Pts',(-179.223988382339,-0.384374003464339,
125.901153535669));
#265253=CARTESIAN_POINT('Ctrl Pts',(-179.231761282605,-0.52106139991651,
125.911868784061));
#265254=CARTESIAN_POINT('Ctrl Pts',(-179.23953418287,-0.657155547236459,
125.928292650204));
#265255=CARTESIAN_POINT('Ctrl Pts',(-179.247307083135,-0.792151210869699,
125.950323172138));
#265256=CARTESIAN_POINT('Ctrl Pts',(-179.254797418897,-0.922239442095216,
125.971552829108));
#265257=CARTESIAN_POINT('Ctrl Pts',(-179.262287754659,-1.05130736659908,
125.997988525034));
#265258=CARTESIAN_POINT('Ctrl Pts',(-179.269778090421,-1.17891665368521,
126.029495322486));
#265259=CARTESIAN_POINT('Ctrl Pts',(-179.27755242454,-1.31136428567816,
126.062196709739));
#265260=CARTESIAN_POINT('Ctrl Pts',(-179.285326758659,-1.44266004261855,
126.100464919285));
#265261=CARTESIAN_POINT('Ctrl Pts',(-179.293101092779,-1.57230004771894,
126.144204437518));
#265262=CARTESIAN_POINT('Ctrl Pts',(-179.300865845726,-1.70178028309931,
126.187890050703));
#265263=CARTESIAN_POINT('Ctrl Pts',(-179.308630598673,-1.8296084598658,
126.237033432431));
#265264=CARTESIAN_POINT('Ctrl Pts',(-179.31639535162,-1.95529193815402,
126.291488306156));
#265265=CARTESIAN_POINT('Ctrl Pts',(-179.324152392505,-2.08085058584013,
126.345889094533));
#265266=CARTESIAN_POINT('Ctrl Pts',(-179.33190943339,-2.20426841771294,
126.405590722102));
#265267=CARTESIAN_POINT('Ctrl Pts',(-179.339666474275,-2.32506932923065,
126.470397572411));
#265268=CARTESIAN_POINT('Ctrl Pts',(-179.347417665515,-2.44577914384112,
126.53515555137));
#265269=CARTESIAN_POINT('Ctrl Pts',(-179.355168856755,-2.56387562298451,
126.605010906023));
#265270=CARTESIAN_POINT('Ctrl Pts',(-179.362920047995,-2.67890431290246,
126.679720664211));
#265271=CARTESIAN_POINT('Ctrl Pts',(-179.370667944772,-2.79388411255856,
126.754398668759));
#265272=CARTESIAN_POINT('Ctrl Pts',(-179.378415841549,-2.90579838913901,
126.833926760686));
#265273=CARTESIAN_POINT('Ctrl Pts',(-179.386163738326,-3.01421909826937,
126.918017054507));
#265274=CARTESIAN_POINT('Ctrl Pts',(-179.393910014411,-3.12261712812466,
127.002089758452));
#265275=CARTESIAN_POINT('Ctrl Pts',(-179.401656290495,-3.22752273534894,
127.090722526651));
#265276=CARTESIAN_POINT('Ctrl Pts',(-179.409402566579,-3.32853890617992,
127.183585588301));
#265277=CARTESIAN_POINT('Ctrl Pts',(-179.417148899844,-3.42955582268919,
127.276449335445));
#265278=CARTESIAN_POINT('Ctrl Pts',(-179.424895233109,-3.52668295768921,
127.373543173757));
#265279=CARTESIAN_POINT('Ctrl Pts',(-179.432641566375,-3.61955859240775,
127.474498959985));
#265280=CARTESIAN_POINT('Ctrl Pts',(-179.440389634378,-3.71245502598061,
127.575477354561));
#265281=CARTESIAN_POINT('Ctrl Pts',(-179.448137702381,-3.80109780006598,
127.680319130344));
#265282=CARTESIAN_POINT('Ctrl Pts',(-179.455885770384,-3.88516434792299,
127.788621727654));
#265283=CARTESIAN_POINT('Ctrl Pts',(-179.463642073126,-3.96932024270782,
127.897039430254));
#265284=CARTESIAN_POINT('Ctrl Pts',(-179.471398375867,-4.04888995545252,
128.008924992652));
#265285=CARTESIAN_POINT('Ctrl Pts',(-179.479154678609,-4.12359296582618,
128.123844974133));
#265286=CARTESIAN_POINT('Ctrl Pts',(-179.486915121123,-4.19833584744553,
128.238826291868));
#265287=CARTESIAN_POINT('Ctrl Pts',(-179.494675563638,-4.26820665186612,
128.356844919536));
#265288=CARTESIAN_POINT('Ctrl Pts',(-179.502436006152,-4.33297052176697,
128.477442157456));
#265289=CARTESIAN_POINT('Ctrl Pts',(-179.510208906417,-4.39783835638142,
128.59823298877));
#265290=CARTESIAN_POINT('Ctrl Pts',(-179.517981806683,-4.45758270355803,
128.721610350122));
#265291=CARTESIAN_POINT('Ctrl Pts',(-179.525754706948,-4.5120162551646,
128.847094060443));
#265292=CARTESIAN_POINT('Ctrl Pts',(-179.53324504271,-4.56447101006087,
128.968016121821));
#265293=CARTESIAN_POINT('Ctrl Pts',(-179.540735378472,-4.6119942762349,
129.090893761478));
#265294=CARTESIAN_POINT('Ctrl Pts',(-179.548225714234,-4.65446265192088,
129.215285262407));
#265295=CARTESIAN_POINT('Ctrl Pts',(-179.555502049297,-4.69571769586986,
129.336122868151));
#265296=CARTESIAN_POINT('Ctrl Pts',(-179.562778384359,-4.73228882758073,
129.458636134573));
#265297=CARTESIAN_POINT('Ctrl Pts',(-179.570054719422,-4.76405452823393,
129.582490119308));
#265298=CARTESIAN_POINT('Ctrl Pts',(-177.819765072025,-4.76405452823413,
129.582490119309));
#265299=CARTESIAN_POINT('Ctrl Pts',(-177.827528067606,-4.79810789403888,
129.715263675749));
#265300=CARTESIAN_POINT('Ctrl Pts',(-177.835291063187,-4.82657512862265,
129.849339500209));
#265301=CARTESIAN_POINT('Ctrl Pts',(-177.843054058769,-4.84938475087329,
129.984207826619));
#265302=CARTESIAN_POINT('Ctrl Pts',(-177.850828440854,-4.87222782952152,
130.119273973419));
#265303=CARTESIAN_POINT('Ctrl Pts',(-177.85860282294,-4.88939667628526,
130.255134556517));
#265304=CARTESIAN_POINT('Ctrl Pts',(-177.866377205026,-4.90087174218342,
130.39127560311));
#265305=CARTESIAN_POINT('Ctrl Pts',(-177.870098127136,-4.90636386052154,
130.456434508968));
#265306=CARTESIAN_POINT('Ctrl Pts',(-177.873819049247,-4.91055247038314,
130.52165766879));
#265307=CARTESIAN_POINT('Ctrl Pts',(-177.877539971357,-4.91343964523087,
130.586888975338));
#265308=CARTESIAN_POINT('Ctrl Pts',(-177.88164645957,-4.91662599235856,
130.658879622671));
#265309=CARTESIAN_POINT('Ctrl Pts',(-177.885752947782,-4.91823024989552,
130.730940811616));
#265310=CARTESIAN_POINT('Ctrl Pts',(-177.889859435994,-4.91824981877137,
130.803025456376));
#265311=CARTESIAN_POINT('Origin',(213.235140564004,0.,130.804360617566));
#265312=CARTESIAN_POINT('',(-207.7784959754,-4.32025079610558,133.152443722346));
#265313=CARTESIAN_POINT('',(-207.934947426862,-4.83864761984552,129.923070498784));
#265314=CARTESIAN_POINT('Ctrl Pts',(-207.778555181163,-4.32174403853603,
133.152064075816));
#265315=CARTESIAN_POINT('Ctrl Pts',(-207.801743821445,-4.40255038673971,
133.003312600242));
#265316=CARTESIAN_POINT('Ctrl Pts',(-207.823415744591,-4.47600032780121,
132.849732400647));
#265317=CARTESIAN_POINT('Ctrl Pts',(-207.918593342393,-4.79298445822066,
132.087388166203));
#265318=CARTESIAN_POINT('Ctrl Pts',(-207.96044672069,-4.91825,131.426623044073));
#265319=CARTESIAN_POINT('Ctrl Pts',(-207.96044672069,-4.91825,130.515843321034));
#265320=CARTESIAN_POINT('Ctrl Pts',(-207.9520747996,-4.89250964418619,130.218795312125));
#265321=CARTESIAN_POINT('Ctrl Pts',(-207.934947426862,-4.83864761984552,
129.923070498784));
#265322=CARTESIAN_POINT('',(-207.639859435957,-4.91824901139309,130.80747901955));
#265323=CARTESIAN_POINT('Ctrl Pts',(-207.639859435995,-4.91824901139267,
130.807479020212));
#265324=CARTESIAN_POINT('Ctrl Pts',(-207.650384863776,-4.91813168363402,
130.992524762711));
#265325=CARTESIAN_POINT('Ctrl Pts',(-207.660910291556,-4.90757161966847,
131.177239249296));
#265326=CARTESIAN_POINT('Ctrl Pts',(-207.671435719336,-4.88667662202955,
131.360754950939));
#265327=CARTESIAN_POINT('Ctrl Pts',(-207.679211362107,-4.87124047627466,
131.496326879103));
#265328=CARTESIAN_POINT('Ctrl Pts',(-207.686987004878,-4.85013380583299,
131.63147072125));
#265329=CARTESIAN_POINT('Ctrl Pts',(-207.694762647649,-4.82338668994206,
131.765674250981));
#265330=CARTESIAN_POINT('Ctrl Pts',(-207.702526426575,-4.79668038400811,
131.899673016942));
#265331=CARTESIAN_POINT('Ctrl Pts',(-207.7102902055,-4.76435084676709,132.032733947661));
#265332=CARTESIAN_POINT('Ctrl Pts',(-207.718053984426,-4.72647989782645,
132.164349896179));
#265333=CARTESIAN_POINT('Ctrl Pts',(-207.72581092684,-4.68864229671419,
132.295849948313));
#265334=CARTESIAN_POINT('Ctrl Pts',(-207.733567869255,-4.64527309585006,
132.425907175703));
#265335=CARTESIAN_POINT('Ctrl Pts',(-207.741324811669,-4.59650519091897,
132.554024325927));
#265336=CARTESIAN_POINT('Ctrl Pts',(-207.749075720058,-4.54777522191265,
132.682041815471));
#265337=CARTESIAN_POINT('Ctrl Pts',(-207.756826628447,-4.49365504758959,
132.808121868315));
#265338=CARTESIAN_POINT('Ctrl Pts',(-207.764577536836,-4.43432729007962,
132.931782660075));
#265339=CARTESIAN_POINT('Ctrl Pts',(-207.769236751612,-4.3986642747871,
133.006117455334));
#265340=CARTESIAN_POINT('Ctrl Pts',(-207.773895966387,-4.36112049094283,
133.079578367346));
#265341=CARTESIAN_POINT('Ctrl Pts',(-207.778555181163,-4.32174403853604,
133.152064075816));
#265342=CARTESIAN_POINT('',(-207.345738387465,-2.41370886482958,126.51939632007));
#265343=CARTESIAN_POINT('Ctrl Pts',(-207.344683452294,-2.4077731095894,
126.515793057735));
#265344=CARTESIAN_POINT('Ctrl Pts',(-207.352734226166,-2.53162780530793,
126.585330030555));
#265345=CARTESIAN_POINT('Ctrl Pts',(-207.360785000037,-2.65233540086029,
126.660162464917));
#265346=CARTESIAN_POINT('Ctrl Pts',(-207.368835773908,-2.76943374285605,
126.73995170526));
#265347=CARTESIAN_POINT('Ctrl Pts',(-207.37688654778,-2.88653208485212,
126.819740945603));
#265348=CARTESIAN_POINT('Ctrl Pts',(-207.384937321651,-3.00002084366859,
126.904486660409));
#265349=CARTESIAN_POINT('Ctrl Pts',(-207.392988095523,-3.10947838849646,
126.993805905457));
#265350=CARTESIAN_POINT('Ctrl Pts',(-207.400658416081,-3.21376332677892,
127.078904214322));
#265351=CARTESIAN_POINT('Ctrl Pts',(-207.408328736639,-3.31473885798247,
127.168439200213));
#265352=CARTESIAN_POINT('Ctrl Pts',(-207.415999057197,-3.41199622474628,
127.262120531855));
#265353=CARTESIAN_POINT('Ctrl Pts',(-207.423659876097,-3.5091331133442,
127.355685815167));
#265354=CARTESIAN_POINT('Ctrl Pts',(-207.431320694998,-3.6025607104101,
127.453386953501));
#265355=CARTESIAN_POINT('Ctrl Pts',(-207.438981513899,-3.69190164243585,
127.554892149481));
#265356=CARTESIAN_POINT('Ctrl Pts',(-207.446634794044,-3.78115465703662,
127.65629745759));
#265357=CARTESIAN_POINT('Ctrl Pts',(-207.454288074189,-3.86632874177754,
127.761499077257));
#265358=CARTESIAN_POINT('Ctrl Pts',(-207.461941354334,-3.94708224177111,
127.870127354992));
#265359=CARTESIAN_POINT('Ctrl Pts',(-207.469588971909,-4.02777599322606,
127.978675259977));
#265360=CARTESIAN_POINT('Ctrl Pts',(-207.477236589484,-4.10405542874681,
128.090644456684));
#265361=CARTESIAN_POINT('Ctrl Pts',(-207.48488420706,-4.17561853151846,
128.205631516305));
#265362=CARTESIAN_POINT('Ctrl Pts',(-207.492528815864,-4.24715347950354,
128.320573337026));
#265363=CARTESIAN_POINT('Ctrl Pts',(-207.500173424667,-4.31397557168506,
128.438530319058));
#265364=CARTESIAN_POINT('Ctrl Pts',(-207.507818033471,-4.37582579382953,
128.559069615367));
#265365=CARTESIAN_POINT('Ctrl Pts',(-207.515461394372,-4.43766591957205,
128.679589234896));
#265366=CARTESIAN_POINT('Ctrl Pts',(-207.523104755273,-4.49453560601694,
128.802689972396));
#265367=CARTESIAN_POINT('Ctrl Pts',(-207.530748116175,-4.54622180435359,
128.927914410471));
#265368=CARTESIAN_POINT('Ctrl Pts',(-207.538391988785,-4.59791146298729,
129.053147232095));
#265369=CARTESIAN_POINT('Ctrl Pts',(-207.546035861395,-4.64441679099704,
129.180503664702));
#265370=CARTESIAN_POINT('Ctrl Pts',(-207.553679734006,-4.68557310654164,
129.309506870287));
#265371=CARTESIAN_POINT('Ctrl Pts',(-207.561329824708,-4.72676290167804,
129.438615016623));
#265372=CARTESIAN_POINT('Ctrl Pts',(-207.568979915409,-4.76259487138462,
129.569372227599));
#265373=CARTESIAN_POINT('Ctrl Pts',(-207.576630006111,-4.79295434605128,
129.701286867009));
#265374=CARTESIAN_POINT('Ctrl Pts',(-207.584283333495,-4.82332666552696,
129.833257318266));
#265375=CARTESIAN_POINT('Ctrl Pts',(-207.591936660878,-4.84822180430393,
129.966385778011));
#265376=CARTESIAN_POINT('Ctrl Pts',(-207.599589988262,-4.86757658728517,
130.100172269598));
#265377=CARTESIAN_POINT('Ctrl Pts',(-207.607253582638,-4.88695733484313,
130.2341382367));
#265378=CARTESIAN_POINT('Ctrl Pts',(-207.614917177013,-4.9007828403537,
130.368763598783));
#265379=CARTESIAN_POINT('Ctrl Pts',(-207.622580771389,-4.90904194574255,
130.503544664797));
#265380=CARTESIAN_POINT('Ctrl Pts',(-207.628340326245,-4.91524905538563,
130.604839032065));
#265381=CARTESIAN_POINT('Ctrl Pts',(-207.634099881101,-4.91831321358352,
130.7062212724));
#265382=CARTESIAN_POINT('Ctrl Pts',(-207.639859435958,-4.91824901139309,
130.80747901955));
#265383=CARTESIAN_POINT('Ctrl Pts',(-207.934947426862,-4.83864761984552,
129.923070498784));
#265384=CARTESIAN_POINT('Ctrl Pts',(-207.915135175363,-4.77634221032461,
129.580988005111));
#265385=CARTESIAN_POINT('Ctrl Pts',(-207.88355659529,-4.67629636070848,
129.240699151234));
#265386=CARTESIAN_POINT('Ctrl Pts',(-207.767461666534,-4.28964812743423,
128.310813320659));
#265387=CARTESIAN_POINT('Ctrl Pts',(-207.660120443156,-3.91181434973351,
127.760719114158));
#265388=CARTESIAN_POINT('Ctrl Pts',(-207.48661174168,-3.17142674355786,
127.020331507982));
#265389=CARTESIAN_POINT('Ctrl Pts',(-207.410631570968,-2.80838203606073,
126.740710909013));
#265390=CARTESIAN_POINT('Ctrl Pts',(-207.344683452294,-2.40777310958941,
126.515793057735));
#265391=CARTESIAN_POINT('Ctrl Pts',(210.578629502474,3.43871735229388,135.623751273273));
#265392=CARTESIAN_POINT('Ctrl Pts',(210.532211638871,4.24191310225744,135.050661598608));
#265393=CARTESIAN_POINT('Ctrl Pts',(210.439385837966,5.5417116830592,133.497735776206));
#265394=CARTESIAN_POINT('Ctrl Pts',(210.253744162458,6.40049231640402,129.500124813146));
#265395=CARTESIAN_POINT('Ctrl Pts',(210.021704475947,3.49988613106459,124.739836436729));
#265396=CARTESIAN_POINT('Ctrl Pts',(209.743256852134,-3.22132718841443,
124.582443963435));
#265397=CARTESIAN_POINT('Ctrl Pts',(209.464809228321,-6.97029916743427,
130.151104711613));
#265398=CARTESIAN_POINT('Ctrl Pts',(209.186361604508,-4.320155850937,136.315756482887));
#265399=CARTESIAN_POINT('Ctrl Pts',(208.907913980696,2.30329626696544,137.417975354914));
#265400=CARTESIAN_POINT('Ctrl Pts',(208.629466356883,6.80838731381026,132.441404887444));
#265401=CARTESIAN_POINT('Ctrl Pts',(208.35101873307,5.05782663488002,125.961106241921));
#265402=CARTESIAN_POINT('Ctrl Pts',(208.072571109257,-1.34111875541754,
123.931185212061));
#265403=CARTESIAN_POINT('Ctrl Pts',(207.794123485444,-6.50738248846785,
128.217554840719));
#265404=CARTESIAN_POINT('Ctrl Pts',(207.515675861631,-5.69381680528821,
134.880978212762));
#265405=CARTESIAN_POINT('Ctrl Pts',(207.237228237818,0.352161018465804,
137.798239159538));
#265406=CARTESIAN_POINT('Ctrl Pts',(206.958780614005,6.07448159193836,134.288440920842));
#265407=CARTESIAN_POINT('Ctrl Pts',(206.680332990192,6.21467071562046,127.576957111676));
#265408=CARTESIAN_POINT('Ctrl Pts',(206.40188536638,0.643870262773591,123.831292031177));
#265409=CARTESIAN_POINT('Ctrl Pts',(206.123437742567,-5.51860979104455,
126.493540260974));
#265410=CARTESIAN_POINT('Ctrl Pts',(205.844990118754,-6.60976007302988,
133.117219720399));
#265411=CARTESIAN_POINT('Ctrl Pts',(205.566542494941,-1.62686214948821,
137.615495756827));
#265412=CARTESIAN_POINT('Ctrl Pts',(205.288094871128,4.8510417637676,135.85467075854));
#265413=CARTESIAN_POINT('Ctrl Pts',(205.009647247315,6.87107573233629,129.452857771449));
#265414=CARTESIAN_POINT('Ctrl Pts',(204.731199623502,2.57692653546199,124.293009711503));
#265415=CARTESIAN_POINT('Ctrl Pts',(204.452751999689,-4.08529213152394,
125.116775123829));
#265416=CARTESIAN_POINT('Ctrl Pts',(204.174304375876,-6.9933269740478,131.167153704944));
#265417=CARTESIAN_POINT('Ctrl Pts',(203.895856752063,-3.47483593506387,
136.884143186524));
#265418=CARTESIAN_POINT('Ctrl Pts',(203.617409128251,3.23685955433703,137.014109488232));
#265419=CARTESIAN_POINT('Ctrl Pts',(203.338961504438,6.97403925260401,131.437619947721));
#265420=CARTESIAN_POINT('Ctrl Pts',(203.060513880625,4.30241757323156,125.27919601562));
#265421=CARTESIAN_POINT('Ctrl Pts',(202.782066256812,-2.32291566837452,
124.198128435325));
#265422=CARTESIAN_POINT('Ctrl Pts',(202.503618632999,-6.81360289295739,
129.18786549711));
#265423=CARTESIAN_POINT('Ctrl Pts',(202.225171009186,-5.0429219211382,135.663082604955));
#265424=CARTESIAN_POINT('Ctrl Pts',(201.946723385373,1.36195793536179,137.673371567868));
#265425=CARTESIAN_POINT('Ctrl Pts',(201.66827576156,6.51526498482727,133.371375037445));
#265426=CARTESIAN_POINT('Ctrl Pts',(201.389828137747,5.6813618015098,126.710417660699));
#265427=CARTESIAN_POINT('Ctrl Pts',(201.111380513935,-0.373435327379839,
123.811593861123));
#265428=CARTESIAN_POINT('Ctrl Pts',(200.832932890122,-6.08506363376988,
127.338781095048));
#265429=CARTESIAN_POINT('Ctrl Pts',(200.554485266309,-6.20481573259303,
134.050666607207));
#265430=CARTESIAN_POINT('Ctrl Pts',(200.276037642496,-0.622645295272457,
137.779355505743));
#265431=CARTESIAN_POINT('Ctrl Pts',(199.997590018683,5.53170575049466,135.098364849491));
#265432=CARTESIAN_POINT('Ctrl Pts',(199.71914239487,6.60268945040398,128.471394077867));
#265433=CARTESIAN_POINT('Ctrl Pts',(199.440694771057,1.60612410470526,123.988305584475));
#265434=CARTESIAN_POINT('Ctrl Pts',(199.162247147244,-4.86639082969376,
125.768838683693));
#265435=CARTESIAN_POINT('Ctrl Pts',(198.883799523432,-6.86693032801245,
132.176770441218));
#265436=CARTESIAN_POINT('Ctrl Pts',(198.605351899619,-2.5570963230842,137.323524616753));
#265437=CARTESIAN_POINT('Ctrl Pts',(198.326904275806,4.10258428165832,136.479485555902));
#265438=CARTESIAN_POINT('Ctrl Pts',(198.048456651993,6.99219035394115,130.420283921986));
#265439=CARTESIAN_POINT('Ctrl Pts',(197.77000902818,3.45631507844086,124.714030008118));
#265440=CARTESIAN_POINT('Ctrl Pts',(197.491561404367,-3.25574490376804,
124.604492395141));
#265441=CARTESIAN_POINT('Ctrl Pts',(197.213113780554,-6.97593437139489,
130.192330798173));
#265442=CARTESIAN_POINT('Ctrl Pts',(196.934666156741,-4.28558094504976,
136.342594705906));
#265443=CARTESIAN_POINT('Ctrl Pts',(196.656218532928,2.3430120075278,137.403492044232));
#265444=CARTESIAN_POINT('Ctrl Pts',(196.377770909115,6.81849138768721,132.400109986944));
#265445=CARTESIAN_POINT('Ctrl Pts',(196.099323285303,5.02811028438465,125.930312215887));
#265446=CARTESIAN_POINT('Ctrl Pts',(195.82087566149,-1.38285853342424,123.939526815472));
#265447=CARTESIAN_POINT('Ctrl Pts',(195.542428037677,-6.5230479154113,128.257188313404));
#265448=CARTESIAN_POINT('Ctrl Pts',(195.263980413864,-5.66887493174189,
134.915576722577));
#265449=CARTESIAN_POINT('Ctrl Pts',(194.985532790051,0.394717174261835,
137.795958375315));
#265450=CARTESIAN_POINT('Ctrl Pts',(194.707085166238,6.09558348012494,134.251403247221));
#265451=CARTESIAN_POINT('Ctrl Pts',(194.428637542425,6.19490635356113,127.539184339867));
#265452=CARTESIAN_POINT('Ctrl Pts',(194.150189918612,0.601412926074683,
123.827502918989));
#265453=CARTESIAN_POINT('Ctrl Pts',(193.871742294799,-5.54474959981957,
126.527212884656));
#265454=CARTESIAN_POINT('Ctrl Pts',(193.593294670987,-6.59555811955654,
133.157412666584));
#265455=CARTESIAN_POINT('Ctrl Pts',(193.314847047174,-1.58537093834796,
137.625272568447));
#265456=CARTESIAN_POINT('Ctrl Pts',(193.036399423361,4.88169468552635,135.825047607524));
#265457=CARTESIAN_POINT('Ctrl Pts',(192.757951799548,6.86272137744547,129.411056577024));
#265458=CARTESIAN_POINT('Ctrl Pts',(192.479504175735,2.53724238606986,124.277443893095));
#265459=CARTESIAN_POINT('Ctrl Pts',(192.201056551922,-4.11983840692253,
125.141748821346));
#265460=CARTESIAN_POINT('Ctrl Pts',(191.922608928109,-6.99098896924831,
131.209717356357));
#265461=CARTESIAN_POINT('Ctrl Pts',(191.644161304296,-3.43776219763276,
136.905182851196));
#265462=CARTESIAN_POINT('Ctrl Pts',(191.365713680483,3.27460008958736,136.994290755064));
#265463=CARTESIAN_POINT('Ctrl Pts',(191.08726605667,6.9777648675845,131.395155257469));
#265464=CARTESIAN_POINT('Ctrl Pts',(190.808818432858,4.26870461503614,125.253108347726));
#265465=CARTESIAN_POINT('Ctrl Pts',(190.530370809044,-2.36308664091672,
124.212391080215));
#265466=CARTESIAN_POINT('Ctrl Pts',(190.251923185232,-6.82331671706736,
129.229371781915));
#265467=CARTESIAN_POINT('Ctrl Pts',(189.973475561419,-5.01325206778612,
135.693690281095));
#265468=CARTESIAN_POINT('Ctrl Pts',(189.695027937606,1.40374632081163,137.664953676525));
#265469=CARTESIAN_POINT('Ctrl Pts',(189.416580313793,6.53077041740369,133.331667209374));
#265470=CARTESIAN_POINT('Ctrl Pts',(189.13813268998,5.65633554627347,126.675909450142));
#265471=CARTESIAN_POINT('Ctrl Pts',(188.859685066167,-0.41599536452862,
123.81399662772));
#265472=CARTESIAN_POINT('Ctrl Pts',(188.581237442354,-6.10604685783229,
127.375886813701));
#265473=CARTESIAN_POINT('Ctrl Pts',(188.302789818542,-6.18493958576042,
134.088376935175));
#265474=CARTESIAN_POINT('Ctrl Pts',(188.024342194729,-0.580174985471077,
137.783016493883));
#265475=CARTESIAN_POINT('Ctrl Pts',(187.745894570916,5.55774208334242,135.064612228548));
#265476=CARTESIAN_POINT('Ctrl Pts',(187.467446947103,6.58836568835925,128.431244857581));
#265477=CARTESIAN_POINT('Ctrl Pts',(187.18899932329,1.56460308533104,123.97865493689));
#265478=CARTESIAN_POINT('Ctrl Pts',(186.910551699478,-4.89695331800637,
125.798555082479));
#265479=CARTESIAN_POINT('Ctrl Pts',(186.632104075664,-6.85844885156509,
132.218545967617));
#265480=CARTESIAN_POINT('Ctrl Pts',(186.353656451852,-2.51736494438869,
137.338969602853));
#265481=CARTESIAN_POINT('Ctrl Pts',(186.075208828038,4.13705436656654,136.454406814005));
#265482=CARTESIAN_POINT('Ctrl Pts',(185.796761204226,6.98972282098866,130.377727590732));
#265483=CARTESIAN_POINT('Ctrl Pts',(185.518313580413,3.41917746986535,124.693103276936));
#265484=CARTESIAN_POINT('Ctrl Pts',(185.2398659566,-3.29342493995873,124.62442590766));
#265485=CARTESIAN_POINT('Ctrl Pts',(184.961418332787,-6.97953072271363,
130.234806630193));
#265486=CARTESIAN_POINT('Ctrl Pts',(184.682970708974,-4.25178874032612,
136.368579642862));
#265487=CARTESIAN_POINT('Ctrl Pts',(184.404523085161,2.38313938299372,137.389107198495));
#265488=CARTESIAN_POINT('Ctrl Pts',(184.126075461348,6.82807883617355,132.358574329007));
#265489=CARTESIAN_POINT('Ctrl Pts',(183.847627837535,4.99834740910532,125.899794986266));
#265490=CARTESIAN_POINT('Ctrl Pts',(183.569180213722,-1.42462110408482,
123.948071857337));
#265491=CARTESIAN_POINT('Ctrl Pts',(183.290732589909,-6.53843241923107,
128.296943150732));
#265492=CARTESIAN_POINT('Ctrl Pts',(183.012284966097,-5.64374376128527,
134.950008601993));
#265493=CARTESIAN_POINT('Ctrl Pts',(182.733837342284,0.437269701071178,
137.793426081729));
#265494=CARTESIAN_POINT('Ctrl Pts',(182.455389718471,6.11645366995566,134.214233834728));
#265495=CARTESIAN_POINT('Ctrl Pts',(182.176942094658,6.17491552152431,127.501534682722));
#265496=CARTESIAN_POINT('Ctrl Pts',(181.898494470845,0.558931670205695,
123.82397121282));
#265497=CARTESIAN_POINT('Ctrl Pts',(181.620046847032,-5.57068308070185,
126.561044594899));
#265498=CARTESIAN_POINT('Ctrl Pts',(181.341599223219,-6.58111222344223,
133.197518104296));
#265499=CARTESIAN_POINT('Ctrl Pts',(181.063151599407,-1.54382073804491,
137.634796795631));
#265500=CARTESIAN_POINT('Ctrl Pts',(180.784703975594,4.91216658577983,135.795238324681));
#265501=CARTESIAN_POINT('Ctrl Pts',(180.506256351781,6.85411278995147,129.369307058824));
#265502=CARTESIAN_POINT('Ctrl Pts',(180.227808727968,2.49746418218255,124.262119907186));
#265503=CARTESIAN_POINT('Ctrl Pts',(179.949361104155,-4.15423200110403,
125.16693236216));
#265504=CARTESIAN_POINT('Ctrl Pts',(179.670913480342,-6.98839192089168,
131.252265980172));
#265505=CARTESIAN_POINT('Ctrl Pts',(179.392465856529,-3.40056106730489,
136.925996451342));
#265506=CARTESIAN_POINT('Ctrl Pts',(179.114018232716,3.31221928049139,136.974242649806));
#265507=CARTESIAN_POINT('Ctrl Pts',(178.835570608904,6.98123192042358,131.352668676138));
#265508=CARTESIAN_POINT('Ctrl Pts',(178.55712298509,4.23483347762603,125.227226382977));
#265509=CARTESIAN_POINT('Ctrl Pts',(178.278675361277,-2.40317004799311,
124.22689799325));
#265510=CARTESIAN_POINT('Ctrl Pts',(178.000227737465,-6.83277770089014,
129.270936428355));
#265511=CARTESIAN_POINT('Ctrl Pts',(177.721780113652,-4.98339644641697,
135.724116781409));
#265512=CARTESIAN_POINT('Ctrl Pts',(177.443332489839,1.44548268986267,137.65628156334));
#265513=CARTESIAN_POINT('Ctrl Pts',(177.164884866026,6.54603384991367,133.291865731052));
#265514=CARTESIAN_POINT('Ctrl Pts',(176.886437242213,5.63109969342586,126.64155422085));
#265515=CARTESIAN_POINT('Ctrl Pts',(176.6079896184,-0.458539986806858,123.816658424832));
#265516=CARTESIAN_POINT('Ctrl Pts',(176.329541994587,-6.12680382008778,
127.413119575705));
#265517=CARTESIAN_POINT('Ctrl Pts',(176.051094370774,-6.16483425371434,
134.125965572714));
#265518=CARTESIAN_POINT('Ctrl Pts',(175.772646746962,-0.537683177073775,
137.786418885364));
#265519=CARTESIAN_POINT('Ctrl Pts',(175.494199123148,5.58357247201413,135.030701742416));
#265520=CARTESIAN_POINT('Ctrl Pts',(175.215751499336,6.57379779200069,128.391183573973));
#265521=CARTESIAN_POINT('Ctrl Pts',(174.937303875523,1.5230240890144,123.969257218339));
#265522=CARTESIAN_POINT('Ctrl Pts',(174.65885625171,-4.92733434791298,125.82845697323));
#265523=CARTESIAN_POINT('Ctrl Pts',(174.380408627897,-6.84971323277332,
132.260269090858));
#265524=CARTESIAN_POINT('Ctrl Pts',(174.101961004084,-2.4775402838095,137.354172446613));
#265525=CARTESIAN_POINT('Ctrl Pts',(173.823513380271,4.1713711514037,136.429118707571));
#265526=CARTESIAN_POINT('Ctrl Pts',(173.545065756458,6.98699628128659,130.335187068521));
#265527=CARTESIAN_POINT('Ctrl Pts',(173.266618132645,3.38191316241135,124.672403000642));
#265528=CARTESIAN_POINT('Ctrl Pts',(172.988170508833,-3.33098293707706,
124.644588419932));
#265529=CARTESIAN_POINT('Ctrl Pts',(172.709722885019,-6.98286844495469,
130.277303567246));
#265530=CARTESIAN_POINT('Ctrl Pts',(172.431275261207,-4.21783898400718,
136.394358395635));
#265531=CARTESIAN_POINT('Ctrl Pts',(172.152827637394,2.42317845035331,137.374478352552));
#265532=CARTESIAN_POINT('Ctrl Pts',(171.874380013581,6.83741326768756,132.316981079111));
#265533=CARTESIAN_POINT('Ctrl Pts',(171.595932389768,4.96839931822471,125.869459497128));
#265534=CARTESIAN_POINT('Ctrl Pts',(171.317484765955,-1.46633088488636,
123.956870961504));
#265535=CARTESIAN_POINT('Ctrl Pts',(171.039037142142,-6.55357463903296,
128.336790901335));
#265536=CARTESIAN_POINT('Ctrl Pts',(170.760589518329,-5.61840345982816,
134.984286862899));
#265537=CARTESIAN_POINT('Ctrl Pts',(170.482141894517,0.479806024690783,
137.79063480575));
#265538=CARTESIAN_POINT('Ctrl Pts',(170.203694270703,6.13709721234627,134.176938068128));
#265539=CARTESIAN_POINT('Ctrl Pts',(169.925246646891,6.15469587572206,127.464007413007));
#265540=CARTESIAN_POINT('Ctrl Pts',(169.646799023078,0.51642970291829,123.820698167548));
#265541=CARTESIAN_POINT('Ctrl Pts',(169.368351399265,-5.59641013787386,
126.595033542778));
#265542=CARTESIAN_POINT('Ctrl Pts',(169.089903775452,-6.56642246179436,
133.237534862678));
#265543=CARTESIAN_POINT('Ctrl Pts',(168.811456151639,-1.50221333089678,
137.644067918489));
#265544=CARTESIAN_POINT('Ctrl Pts',(168.533008527826,4.94245646389391,135.76524410303));
#265545=CARTESIAN_POINT('Ctrl Pts',(168.254560904013,6.84525022078748,129.32761071706));
#265546=CARTESIAN_POINT('Ctrl Pts',(167.976113280201,2.45759343384159,124.247038346411));
#265547=CARTESIAN_POINT('Ctrl Pts',(167.697665656387,-4.1884716586909,125.192324799951));
#265548=CARTESIAN_POINT('Ctrl Pts',(167.419218032575,-6.98553591510243,
131.294798006688));
#265549=CARTESIAN_POINT('Ctrl Pts',(167.140770408762,-3.36323392793624,
136.946583212019));
#265550=CARTESIAN_POINT('Ctrl Pts',(166.862322784949,3.34971573589186,136.953965917302));
#265551=CARTESIAN_POINT('Ctrl Pts',(166.583875161136,6.98444028114645,131.310161777048));
#265552=CARTESIAN_POINT('Ctrl Pts',(166.305427537323,4.20080541690416,125.20155108099));
#265553=CARTESIAN_POINT('Ctrl Pts',(166.02697991351,-2.44316440471955,124.241648636582));
#265554=CARTESIAN_POINT('Ctrl Pts',(165.748532289697,-6.84198549362249,
129.312557896394));
#265555=CARTESIAN_POINT('Ctrl Pts',(165.470084665885,-4.95335616345982,
135.754360978348));
#265556=CARTESIAN_POINT('Ctrl Pts',(165.191637042072,1.48716549602113,137.647355549705));
#265557=CARTESIAN_POINT('Ctrl Pts',(164.913189418259,6.56105471673207,133.251972077313));
#265558=CARTESIAN_POINT('Ctrl Pts',(164.634741794446,5.60565517810829,126.60735324588));
#265559=CARTESIAN_POINT('Ctrl Pts',(164.356294170633,-0.501067617717217,
123.819579153818));
#265560=CARTESIAN_POINT('Ctrl Pts',(164.07784654682,-6.1473337513746,127.450478001396));
#265561=CARTESIAN_POINT('Ctrl Pts',(163.799398923007,-6.14450048146789,
134.163431126959));
#265562=CARTESIAN_POINT('Ctrl Pts',(163.520951299194,-0.495171444628521,
137.789562554107));
#265563=CARTESIAN_POINT('Ctrl Pts',(163.242503675381,5.60919595935461,134.996634647659));
#265564=CARTESIAN_POINT('Ctrl Pts',(162.964056051569,6.55898630114736,128.351211711527));
#265565=CARTESIAN_POINT('Ctrl Pts',(162.685608427755,1.48138865648,123.960112777059));
#265566=CARTESIAN_POINT('Ctrl Pts',(162.407160803943,-4.95753279363329,
125.85854324792));
#265567=CARTESIAN_POINT('Ctrl Pts',(162.12871318013,-6.84072379533872,132.301938264875));
#265568=CARTESIAN_POINT('Ctrl Pts',(161.850265556317,-2.4376238170639,137.369132584688));
#265569=CARTESIAN_POINT('Ctrl Pts',(161.571817932504,4.20553336454888,136.403622173655));
#265570=CARTESIAN_POINT('Ctrl Pts',(161.293370308691,6.98401083586784,130.292663931709));
#265571=CARTESIAN_POINT('Ctrl Pts',(161.014922684878,3.34452353692138,124.651929946293));
#265572=CARTESIAN_POINT('Ctrl Pts',(160.736475061065,-3.36841750339773,
124.664979184829));
#265573=CARTESIAN_POINT('Ctrl Pts',(160.458027437253,-6.98594741443756,
130.319820034592));
#265574=CARTESIAN_POINT('Ctrl Pts',(160.179579813439,-4.18373293411359,
136.419930008985));
#265575=CARTESIAN_POINT('Ctrl Pts',(159.901132189627,2.46312772594441,137.35960604848));
#265576=CARTESIAN_POINT('Ctrl Pts',(159.622684565814,6.84649433633851,132.275331778507));
#265577=CARTESIAN_POINT('Ctrl Pts',(159.344236942001,4.93826712148011,125.839306872565));
#265578=CARTESIAN_POINT('Ctrl Pts',(159.065789318188,-1.50798633025781,
123.965923801919));
#265579=CARTESIAN_POINT('Ctrl Pts',(158.787341694375,-6.56847401371661,
128.376730088641));
#265580=CARTESIAN_POINT('Ctrl Pts',(158.508894070562,-5.59285496636459,
135.018410235101));
#265581=CARTESIAN_POINT('Ctrl Pts',(158.230446446749,0.522324568921774,
137.787584650814));
#265582=CARTESIAN_POINT('Ctrl Pts',(157.951998822937,6.15751334234277,134.139517329431));
#265583=CARTESIAN_POINT('Ctrl Pts',(157.673551199123,6.13424816540071,127.426603921307));
#265584=CARTESIAN_POINT('Ctrl Pts',(157.395103575311,0.473908599138188,
123.817683904457));
#265585=CARTESIAN_POINT('Ctrl Pts',(157.116655951498,-5.62192981801017,
126.62917846882));
#265586=CARTESIAN_POINT('Ctrl Pts',(156.838208327685,-6.55148937894732,
133.277461458893));
#265587=CARTESIAN_POINT('Ctrl Pts',(156.559760703872,-1.46055025868114,
137.653085593479));
#265588=CARTESIAN_POINT('Ctrl Pts',(156.281313080059,4.97256319746619,135.735066054016));
#265589=CARTESIAN_POINT('Ctrl Pts',(156.002865456246,6.83613399835919,129.285969096806));
#265590=CARTESIAN_POINT('Ctrl Pts',(155.724417832433,2.4176316184721,124.232199769625));
#265591=CARTESIAN_POINT('Ctrl Pts',(155.44597020862,-4.2225561109203,125.217925193794));
#265592=CARTESIAN_POINT('Ctrl Pts',(155.167522584808,-6.98242105771092,
131.337311859867));
#265593=CARTESIAN_POINT('Ctrl Pts',(154.889074960995,-3.3257821626974,136.96694237038));
#265594=CARTESIAN_POINT('Ctrl Pts',(154.610627337182,3.38708806634394,136.933461308912));
#265595=CARTESIAN_POINT('Ctrl Pts',(154.332179713369,6.98738983086623,131.267636135312));
#265596=CARTESIAN_POINT('Ctrl Pts',(154.053732089556,4.1666216937926,125.17608339317));
#265597=CARTESIAN_POINT('Ctrl Pts',(153.775284465743,-2.48306822909056,
124.256642463619));
#265598=CARTESIAN_POINT('Ctrl Pts',(153.49683684193,-6.85093975406627,129.354234643731));
#265599=CARTESIAN_POINT('Ctrl Pts',(153.218389218117,-4.92313233206838,
135.784421751204));
#265600=CARTESIAN_POINT('Ctrl Pts',(152.939941594304,1.52879319471521,137.638175966376));
#265601=CARTESIAN_POINT('Ctrl Pts',(152.661493970491,6.57583246125511,133.21198772643));
#265602=CARTESIAN_POINT('Ctrl Pts',(152.383046346679,5.58000294317656,126.573307792561));
#265603=CARTESIAN_POINT('Ctrl Pts',(152.104598722866,-0.543576681382813,
123.822758706449));
#265604=CARTESIAN_POINT('Ctrl Pts',(151.826151099053,-6.16763589094857,
127.487960706439));
#265605=CARTESIAN_POINT('Ctrl Pts',(151.54770347524,-6.12393902249645,134.200772209611));
#265606=CARTESIAN_POINT('Ctrl Pts',(151.269255851427,-0.452641363423277,
137.792447383624));
#265607=CARTESIAN_POINT('Ctrl Pts',(150.990808227614,5.63461159587598,134.962412206646));
#265608=CARTESIAN_POINT('Ctrl Pts',(150.712360603801,6.54393176464461,128.311330751416));
#265609=CARTESIAN_POINT('Ctrl Pts',(150.433912979988,1.4396983305442,123.951221951899));
#265610=CARTESIAN_POINT('Ctrl Pts',(150.155465356176,-4.98754753615285,
125.888812791691));
#265611=CARTESIAN_POINT('Ctrl Pts',(149.877017732362,-6.83148087236823,
132.343551945603));
#265612=CARTESIAN_POINT('Ctrl Pts',(149.59857010855,-2.39761702327129,137.383849462723));
#265613=CARTESIAN_POINT('Ctrl Pts',(149.320122484737,4.23953974010866,136.377918157044));
#265614=CARTESIAN_POINT('Ctrl Pts',(149.041674860924,6.98076659535922,130.250159756006));
#265615=CARTESIAN_POINT('Ctrl Pts',(148.763227237111,3.30700997888175,124.631684872525));
#265616=CARTESIAN_POINT('Ctrl Pts',(148.484779613298,-3.40572725176907,
124.685597446761));
#265617=CARTESIAN_POINT('Ctrl Pts',(148.206331989485,-6.98876751706998,
130.362354456768));
#265618=CARTESIAN_POINT('Ctrl Pts',(147.927884365672,-4.14947185445744,
136.445293535346));
#265619=CARTESIAN_POINT('Ctrl Pts',(147.649436741859,2.50298572943186,137.344490837378));
#265620=CARTESIAN_POINT('Ctrl Pts',(147.370989118047,6.85532170562399,132.233627970525));
#265621=CARTESIAN_POINT('Ctrl Pts',(147.092541494233,4.90795193543132,125.809338229895));
#265622=CARTESIAN_POINT('Ctrl Pts',(146.814093870421,-1.54958589664124,
123.975230043125));
#265623=CARTESIAN_POINT('Ctrl Pts',(146.535646246608,-6.58312999118006,
128.41675923269));
#265624=CARTESIAN_POINT('Ctrl Pts',(146.257198622795,-5.56709922760349,
135.052377454143));
#265625=CARTESIAN_POINT('Ctrl Pts',(145.978750998982,0.564823758223794,
137.784275729942));
#265626=CARTESIAN_POINT('Ctrl Pts',(145.700303375169,6.17770130341801,134.101973005276));
#265627=CARTESIAN_POINT('Ctrl Pts',(145.421855751356,6.11357314825767,127.389325593625));
#265628=CARTESIAN_POINT('Ctrl Pts',(145.143408127543,0.431369934500661,
123.81492853524));
#265629=CARTESIAN_POINT('Ctrl Pts',(144.864960503731,-5.64724117546963,
126.663478107772));
#265630=CARTESIAN_POINT('Ctrl Pts',(144.586512879918,-6.53631352825206,
133.317296413447));
#265631=CARTESIAN_POINT('Ctrl Pts',(144.308065256105,-1.41883306523854,
137.661849486446));
#265632=CARTESIAN_POINT('Ctrl Pts',(144.029617632292,5.00248567088053,135.704705295899));
#265633=CARTESIAN_POINT('Ctrl Pts',(143.751170008479,6.82676446047164,129.244383741109));
#265634=CARTESIAN_POINT('Ctrl Pts',(143.472722384666,2.37758021687388,124.217604726676));
#265635=CARTESIAN_POINT('Ctrl Pts',(143.194274760853,-4.25648409478009,
125.243732595056));
#265636=CARTESIAN_POINT('Ctrl Pts',(142.91582713704,-6.97904746413934,131.379805964341));
#265637=CARTESIAN_POINT('Ctrl Pts',(142.637379513228,-3.28820715937746,
136.987073172008));
#265638=CARTESIAN_POINT('Ctrl Pts',(142.358931889414,3.42433488700229,136.912729584442));
#265639=CARTESIAN_POINT('Ctrl Pts',(142.080484265602,6.99008046028611,131.225093326731));
#265640=CARTESIAN_POINT('Ctrl Pts',(141.802036641788,4.13228357498186,125.150824263232));
#265641=CARTESIAN_POINT('Ctrl Pts',(141.523589017976,-2.52288004245522,
124.271878918761));
#265642=CARTESIAN_POINT('Ctrl Pts',(141.245141394163,-6.859640150418,129.395965126019));
#265643=CARTESIAN_POINT('Ctrl Pts',(140.96669377035,-4.89272607219785,135.814297986063));
#265644=CARTESIAN_POINT('Ctrl Pts',(140.688246146537,1.57036424341533,137.628743153505));
#265645=CARTESIAN_POINT('Ctrl Pts',(140.409798522724,6.59036653588803,133.17191416004));
#265646=CARTESIAN_POINT('Ctrl Pts',(140.131350898911,5.55414393918375,126.539419122461));
#265647=CARTESIAN_POINT('Ctrl Pts',(139.852903275098,-0.586065602614643,
123.826196964908));
#265648=CARTESIAN_POINT('Ctrl Pts',(139.574455651286,-6.18770948650656,
127.525566301902));
#265649=CARTESIAN_POINT('Ctrl Pts',(139.296008027473,-6.10315063871238,
134.237987436982));
#265650=CARTESIAN_POINT('Ctrl Pts',(139.01756040366,-0.410094509425858,
137.795073267016));
#265651=CARTESIAN_POINT('Ctrl Pts',(138.739112779847,5.65981843979252,134.928035687503));
#265652=CARTESIAN_POINT('Ctrl Pts',(138.460665156034,6.52863474034383,128.271542171445));
#265653=CARTESIAN_POINT('Ctrl Pts',(138.182217532221,1.39795465605713,123.942585072312));
#265654=CARTESIAN_POINT('Ctrl Pts',(137.903769908408,-5.01737746326431,
125.919264482896));
#265655=CARTESIAN_POINT('Ctrl Pts',(137.625322284595,-6.82198480636163,
132.385108591028));
#265656=CARTESIAN_POINT('Ctrl Pts',(137.346874660782,-2.35752138489827,
137.39832253538));
#265657=CARTESIAN_POINT('Ctrl Pts',(137.06842703697,4.27338901796432,136.352007610208));
#265658=CARTESIAN_POINT('Ctrl Pts',(136.789979413157,6.9772636799772,130.20767611642));
#265659=CARTESIAN_POINT('Ctrl Pts',(136.511531789344,3.26937387837121,124.611668529527));
#265660=CARTESIAN_POINT('Ctrl Pts',(136.233084165531,-3.44291079966457,
124.706442441713));
#265661=CARTESIAN_POINT('Ctrl Pts',(135.954636541718,-6.99132864835187,
130.404905257644));
#265662=CARTESIAN_POINT('Ctrl Pts',(135.676188917905,-4.1150570145959,136.470448034864));
#265663=CARTESIAN_POINT('Ctrl Pts',(135.397741294092,2.54275098386259,137.329133279345));
#265664=CARTESIAN_POINT('Ctrl Pts',(135.11929367028,6.8638950484427,132.191871200516));
#265665=CARTESIAN_POINT('Ctrl Pts',(134.840846046466,4.87745488341857,125.779554679616));
#265666=CARTESIAN_POINT('Ctrl Pts',(134.562398422654,-1.59112804254939,
123.984789340275));
#265667=CARTESIAN_POINT('Ctrl Pts',(134.283950798841,-6.59754202834077,
128.456876850186));
#265668=CARTESIAN_POINT('Ctrl Pts',(134.005503175028,-5.54113719793324,
135.086187261361));
#265669=CARTESIAN_POINT('Ctrl Pts',(133.727055551215,0.607302017773813,
137.780708165749));
#265670=CARTESIAN_POINT('Ctrl Pts',(133.448607927402,6.19766034749954,134.064306486881));
#265671=CARTESIAN_POINT('Ctrl Pts',(133.170160303589,6.09267159041341,127.352173811322));
#265672=CARTESIAN_POINT('Ctrl Pts',(132.891712679776,0.388815285291658,
123.812432161999));
#265673=CARTESIAN_POINT('Ctrl Pts',(132.613265055963,-5.67234327233058,
126.697931188648));
#265674=CARTESIAN_POINT('Ctrl Pts',(132.334817432151,-6.52089547205522,
133.357038250242));
#265675=CARTESIAN_POINT('Ctrl Pts',(132.056369808337,-1.37706329641493,
137.670359272641));
#265676=CARTESIAN_POINT('Ctrl Pts',(131.777922184525,5.0322227753486,135.674162953708));
#265677=CARTESIAN_POINT('Ctrl Pts',(131.499474560712,6.81714195431646,129.20285619093));
#265678=CARTESIAN_POINT('Ctrl Pts',(131.221026936899,2.33744071316646,124.203253758389));
#265679=CARTESIAN_POINT('Ctrl Pts',(130.942579313086,-4.29025435305649,
125.269746047434));
#265680=CARTESIAN_POINT('Ctrl Pts',(130.664131689273,-6.97541525939744,
131.422278745477));
#265681=CARTESIAN_POINT('Ctrl Pts',(130.38568406546,-3.25051031033198,137.006974870947));
#265682=CARTESIAN_POINT('Ctrl Pts',(130.107236441647,3.46145481767177,136.891771512113));
#265683=CARTESIAN_POINT('Ctrl Pts',(129.828788817834,6.99251206970404,131.182534927744));
#265684=CARTESIAN_POINT('Ctrl Pts',(129.550341194022,4.09779233288376,125.125774627163));
#265685=CARTESIAN_POINT('Ctrl Pts',(129.271893570209,-2.5625983695722,124.287357437414));
#265686=CARTESIAN_POINT('Ctrl Pts',(128.993445946396,-6.86808636028122,
129.43774779692));
#265687=CARTESIAN_POINT('Ctrl Pts',(128.714998322583,-4.86213851056362,
135.84398857585));
#265688=CARTESIAN_POINT('Ctrl Pts',(128.43655069877,1.61187710169066,137.61905746063));
#265689=CARTESIAN_POINT('Ctrl Pts',(128.158103074957,6.60465640206541,133.131752863082));
#265690=CARTESIAN_POINT('Ctrl Pts',(127.879655451144,5.52807912434469,126.505688491336));
#265691=CARTESIAN_POINT('Ctrl Pts',(127.601207827331,-0.628532806970051,
123.829893801787));
#265692=CARTESIAN_POINT('Ctrl Pts',(127.322760203518,-6.20755379421381,
127.563293394292));
#265693=CARTESIAN_POINT('Ctrl Pts',(127.044312579706,-6.08213610043705,
134.275075430049));
#265694=CARTESIAN_POINT('Ctrl Pts',(126.765864955893,-0.367532459225645,
137.797440106979));
#265695=CARTESIAN_POINT('Ctrl Pts',(126.48741733208,5.68481555705546,134.893506364063));
#265696=CARTESIAN_POINT('Ctrl Pts',(126.208969708267,6.51309579508176,128.231847445991));
#265697=CARTESIAN_POINT('Ctrl Pts',(125.930522084454,1.35615917984635,123.934202458341));
#265698=CARTESIAN_POINT('Ctrl Pts',(125.652074460641,-5.04702146960864,
125.949897193134));
#265699=CARTESIAN_POINT('Ctrl Pts',(125.373626836828,-6.81223594919939,
132.426606661257));
#265700=CARTESIAN_POINT('Ctrl Pts',(125.095179213015,-2.3173383877032,137.412551266352));
#265701=CARTESIAN_POINT('Ctrl Pts',(124.816731589202,4.3070799438184,136.325891493273));
#265702=CARTESIAN_POINT('Ctrl Pts',(124.538283965389,6.97350221952356,130.165214587198));
#265703=CARTESIAN_POINT('Ctrl Pts',(124.259836341577,3.2316166300094,124.591881659011));
#265704=CARTESIAN_POINT('Ctrl Pts',(123.981388717764,-3.47996676923432,
124.727513397266));
#265705=CARTESIAN_POINT('Ctrl Pts',(123.702941093951,-6.99363071337966,
130.447470860486));
#265706=CARTESIAN_POINT('Ctrl Pts',(123.424493470138,-4.08048968978323,
136.495392575427));
#265707=CARTESIAN_POINT('Ctrl Pts',(123.146045846325,2.58242201572056,137.313533943462));
#265708=CARTESIAN_POINT('Ctrl Pts',(122.867598222512,6.87221404710605,132.150063015792));
#265709=CARTESIAN_POINT('Ctrl Pts',(122.589150598699,4.84677709552158,125.749957325369));
#265710=CARTESIAN_POINT('Ctrl Pts',(122.310702974886,-1.63261122862275,
123.994601339147));
#265711=CARTESIAN_POINT('Ctrl Pts',(122.032255351073,-6.6117095911554,128.497081454556));
#265712=CARTESIAN_POINT('Ctrl Pts',(121.753807727261,-5.51496983938628,
135.119838403918));
#265713=CARTESIAN_POINT('Ctrl Pts',(121.475360103447,0.649757773524084,
137.776882090432));
#265714=CARTESIAN_POINT('Ctrl Pts',(121.196912479635,6.21738973499768,134.026519169992));
#265715=CARTESIAN_POINT('Ctrl Pts',(120.918464855822,6.07154426638285,127.315149951069));
#265716=CARTESIAN_POINT('Ctrl Pts',(120.640017232009,0.346246228389124,
123.810194877238));
#265717=CARTESIAN_POINT('Ctrl Pts',(120.361569608196,-5.69723517842559,
126.732536434776));
#265718=CARTESIAN_POINT('Ctrl Pts',(120.083121984383,-6.50523578167861,
133.396685496627));
#265719=CARTESIAN_POINT('Ctrl Pts',(119.80467436057,-1.3352425000044,137.678614636731));
#265720=CARTESIAN_POINT('Ctrl Pts',(119.526226736757,5.06177340895125,135.6434401592));
#265721=CARTESIAN_POINT('Ctrl Pts',(119.247779112945,6.8072668364591,129.161387985085));
#265722=CARTESIAN_POINT('Ctrl Pts',(118.969331489131,2.29721459473369,124.189147396544));
#265723=CARTESIAN_POINT('Ctrl Pts',(118.690883865319,-4.32386563438011,
125.29596458699));
#265724=CARTESIAN_POINT('Ctrl Pts',(118.412436241506,-6.97152457807781,
131.464728629428));
#265725=CARTESIAN_POINT('Ctrl Pts',(118.133988617693,-3.21269301243169,
137.026646729736));
#265726=CARTESIAN_POINT('Ctrl Pts',(117.85554099388,3.49844648286018,136.870587868534));
#265727=CARTESIAN_POINT('Ctrl Pts',(117.577093370067,6.99468456901571,131.139962515369));
#265728=CARTESIAN_POINT('Ctrl Pts',(117.298645746254,4.06314924558364,125.100935413187));
#265729=CARTESIAN_POINT('Ctrl Pts',(117.020198122441,-2.60222173866402,
124.303077446017));
#265730=CARTESIAN_POINT('Ctrl Pts',(116.741750498628,-6.8762780706787,129.479581108162));
#265731=CARTESIAN_POINT('Ctrl Pts',(116.463302874816,-4.83137078059878,
135.873492420371));
#265732=CARTESIAN_POINT('Ctrl Pts',(116.184855251003,1.65333023126747,137.609119246659));
#265733=CARTESIAN_POINT('Ctrl Pts',(115.90640762719,6.61870153027093,133.09150532375));
#265734=CARTESIAN_POINT('Ctrl Pts',(115.627960003377,5.5018094645007,126.472117149089));
#265735=CARTESIAN_POINT('Ctrl Pts',(115.349512379564,-0.670976720811003,
123.833849080098));
#265736=CARTESIAN_POINT('Ctrl Pts',(115.071064755751,-6.22716807873245,
127.601140585621));
#265737=CARTESIAN_POINT('Ctrl Pts',(114.792617131938,-6.06089618637186,
134.312034814502));
#265738=CARTESIAN_POINT('Ctrl Pts',(114.514169508125,-0.324956789974863,
137.79954781581));
#265739=CARTESIAN_POINT('Ctrl Pts',(114.235721884312,5.70960202138734,134.858825515823));
#265740=CARTESIAN_POINT('Ctrl Pts',(113.957274260499,6.4973155046598,128.192248045959));
#265741=CARTESIAN_POINT('Ctrl Pts',(113.678826636687,1.31431345065849,123.926074420608));
#265742=CARTESIAN_POINT('Ctrl Pts',(113.400379012874,-5.07647845671644,
125.980709787299));
#265743=CARTESIAN_POINT('Ctrl Pts',(113.121931389061,-6.80223466212876,
132.468044618562));
#265744=CARTESIAN_POINT('Ctrl Pts',(112.843483765248,-2.27706952068197,
137.42653512839));
#265745=CARTESIAN_POINT('Ctrl Pts',(112.565036141435,4.34061126924124,136.299570773982));
#265746=CARTESIAN_POINT('Ctrl Pts',(112.286588517622,6.96948235338073,130.122776741767));
#265747=CARTESIAN_POINT('Ctrl Pts',(112.008140893809,3.1937396329048,124.572324994188));
#265748=CARTESIAN_POINT('Ctrl Pts',(111.729693269996,-3.51689378735575,
124.748809532627));
#265749=CARTESIAN_POINT('Ctrl Pts',(111.451245646184,-6.99567362684944,
130.490049688009));
#265750=CARTESIAN_POINT('Ctrl Pts',(111.172798022371,-4.0457711609245,136.52012623271));
#265751=CARTESIAN_POINT('Ctrl Pts',(110.894350398558,2.62199735498092,137.297693407768));
#265752=CARTESIAN_POINT('Ctrl Pts',(110.615902774745,6.88027839335069,132.108204965571));
#265753=CARTESIAN_POINT('Ctrl Pts',(110.337455150932,4.81591970851693,125.720547263895));
#265754=CARTESIAN_POINT('Ctrl Pts',(110.059007527119,-1.67403391768677,
124.004665676154));
#265755=CARTESIAN_POINT('Ctrl Pts',(109.780559903306,-6.62563215463966,
128.537371556004));
#265756=CARTESIAN_POINT('Ctrl Pts',(109.502112279493,-5.48859812160383,
135.153329634858));
#265757=CARTESIAN_POINT('Ctrl Pts',(109.22366465568,0.692189452261082,137.772797645767));
#265758=CARTESIAN_POINT('Ctrl Pts',(108.945217031867,6.23688873483282,133.988612454835));
#265759=CARTESIAN_POINT('Ctrl Pts',(108.666769408055,6.05019195904657,127.278255384801));
#265760=CARTESIAN_POINT('Ctrl Pts',(108.388321784241,0.303664341205276,
123.808216763862));
#265761=CARTESIAN_POINT('Ctrl Pts',(108.109874160429,-5.72191597137591,
126.767292563848));
#265762=CARTESIAN_POINT('Ctrl Pts',(107.831426536616,-6.48933503739778,
133.436236683461));
#265763=CARTESIAN_POINT('Ctrl Pts',(107.552978912803,-1.29337222569216,
137.68661527281));
#265764=CARTESIAN_POINT('Ctrl Pts',(107.27453128899,5.09113647667873,135.612538050821));
#265765=CARTESIAN_POINT('Ctrl Pts',(106.996083665177,6.79713947282576,129.119980660195));
#265766=CARTESIAN_POINT('Ctrl Pts',(106.717636041364,2.25690335216928,124.175286163858));
#265767=CARTESIAN_POINT('Ctrl Pts',(106.439188417551,-4.35731669327239,
125.322387242187));
#265768=CARTESIAN_POINT('Ctrl Pts',(106.160740793739,-6.96737556435125,
131.5071540432));
#265769=CARTESIAN_POINT('Ctrl Pts',(105.882293169926,-3.17475666701035,
137.046088019424));
#265770=CARTESIAN_POINT('Ctrl Pts',(105.603845546113,3.53530851182771,136.849179438675));
#265771=CARTESIAN_POINT('Ctrl Pts',(105.3253979223,6.99659787771835,131.097377667143));
#265772=CARTESIAN_POINT('Ctrl Pts',(105.046950298487,4.02835559679407,125.076307541727));
#265773=CARTESIAN_POINT('Ctrl Pts',(104.768502674674,-2.64174868147234,
124.319038362058));
#265774=CARTESIAN_POINT('Ctrl Pts',(104.490055050861,-6.88421497806359,
129.521463509594));
#265775=CARTESIAN_POINT('Ctrl Pts',(104.211607427049,-4.80042402241278,
135.902808426348));
#265776=CARTESIAN_POINT('Ctrl Pts',(103.933159803235,1.69472209608453,137.598928879852));
#265777=CARTESIAN_POINT('Ctrl Pts',(103.654712179423,6.63250140005722,133.051173033428));
#265778=CARTESIAN_POINT('Ctrl Pts',(103.37626455561,5.47533593308374,126.438706339714));
#265779=CARTESIAN_POINT('Ctrl Pts',(103.097816931797,-0.713395771362793,
123.838062653278));
#265780=CARTESIAN_POINT('Ctrl Pts',(102.819369307984,-6.24655161324796,
127.639106473447));
#265781=CARTESIAN_POINT('Ctrl Pts',(102.540921684171,-6.03943168356949,
134.348864220799));
#265782=CARTESIAN_POINT('Ctrl Pts',(102.262474060358,-0.282369079330704,
137.801396315408));
#265783=CARTESIAN_POINT('Ctrl Pts',(101.984026436545,5.73417691431645,134.823994427897));
#265784=CARTESIAN_POINT('Ctrl Pts',(101.705578812732,6.48129445382252,128.15274543872));
#265785=CARTESIAN_POINT('Ctrl Pts',(101.427131188919,1.27241901910234,123.9182012603));
#265786=CARTESIAN_POINT('Ctrl Pts',(101.148683565106,-5.1057473330482,126.01170112362));
#265787=CARTESIAN_POINT('Ctrl Pts',(100.870235941294,-6.7919813157512,132.509420927444));
#265788=CARTESIAN_POINT('Ctrl Pts',(100.591788317481,-2.23671627601227,
137.440273603317));
#265789=CARTESIAN_POINT('Ctrl Pts',(100.313340693668,4.37398175171709,136.273046427655));
#265790=CARTESIAN_POINT('Ctrl Pts',(100.034893069855,6.96520423050629,130.080364152676));
#265791=CARTESIAN_POINT('Ctrl Pts',(99.7564454460421,3.15574429060373,124.552999259737));
#265792=CARTESIAN_POINT('Ctrl Pts',(99.4779978222292,-3.55369048568456,
124.770330058661));
#265793=CARTESIAN_POINT('Ctrl Pts',(99.1995501984162,-6.99745731306031,
130.532640162439));
#265794=CARTESIAN_POINT('Ctrl Pts',(98.9211025746034,-4.01090271452764,
136.544648090195));
#265795=CARTESIAN_POINT('Ctrl Pts',(98.6426549507905,2.66147553516503,137.281612259238));
#265796=CARTESIAN_POINT('Ctrl Pts',(98.3642073269776,6.88808778834931,132.066298600918));
#265797=CARTESIAN_POINT('Ctrl Pts',(98.0857597031646,4.78488386583629,125.691325584995));
#265798=CARTESIAN_POINT('Ctrl Pts',(97.8073120793519,-1.71539457480834,
124.014981978356));
#265799=CARTESIAN_POINT('Ctrl Pts',(97.5288644555388,-6.63930920288774,
128.577745661565));
#265800=CARTESIAN_POINT('Ctrl Pts',(97.2504168317261,-5.46202302179963,
135.186659713151));
#265801=CARTESIAN_POINT('Ctrl Pts',(96.9719692079131,0.734595481663425,
137.768454983106));
#265802=CARTESIAN_POINT('Ctrl Pts',(96.6935215841003,6.25615662446226,133.950587746053));
#265803=CARTESIAN_POINT('Ctrl Pts',(96.4150739602873,6.0286154596223,127.24149147966));
#265804=CARTESIAN_POINT('Ctrl Pts',(96.1366263364746,0.26107120162757,123.806497895168));
#265805=CARTESIAN_POINT('Ctrl Pts',(95.8581787126614,-5.74638473662552,
126.80219828796));
#265806=CARTESIAN_POINT('Ctrl Pts',(95.5797310888487,-6.47319382842077,
133.47569034516));
#265807=CARTESIAN_POINT('Ctrl Pts',(95.3012834650358,-1.25145402499642,
137.694360884412));
#265808=CARTESIAN_POINT('Ctrl Pts',(95.0228358412229,5.12031089047184,135.581457773658));
#265809=CARTESIAN_POINT('Ctrl Pts',(94.7443882174101,6.78676023868958,129.078635750625));
#265810=CARTESIAN_POINT('Ctrl Pts',(94.465940593597,2.21650847922131,124.161670573963));
#265811=CARTESIAN_POINT('Ctrl Pts',(94.1874929697842,-4.39060629019222,
125.349013033923));
#265812=CARTESIAN_POINT('Ctrl Pts',(93.9090453459715,-6.96296837196094,
131.549553414704));
#265813=CARTESIAN_POINT('Ctrl Pts',(93.6305977221583,-3.13670267981308,
137.065298019608));
#265814=CARTESIAN_POINT('Ctrl Pts',(93.3521500983456,3.5720395386382,136.82754701583));
#265815=CARTESIAN_POINT('Ctrl Pts',(93.0737024745325,6.99825192491364,131.054781961061));
#265816=CARTESIAN_POINT('Ctrl Pts',(92.7952548507199,3.99341267580637,125.051891925383));
#265817=CARTESIAN_POINT('Ctrl Pts',(92.5168072269068,-2.68117773331193,
124.335239594101));
#265818=CARTESIAN_POINT('Ctrl Pts',(92.238359603094,-6.89189678833074,129.563393449252));
#265819=CARTESIAN_POINT('Ctrl Pts',(91.959911979281,-4.7692993827493,135.931935507467));
#265820=CARTESIAN_POINT('Ctrl Pts',(91.6814643554683,1.73605116235111,137.588486737821));
#265821=CARTESIAN_POINT('Ctrl Pts',(91.4030167316553,6.6460555000649,133.010757486647));
#265822=CARTESIAN_POINT('Ctrl Pts',(91.1245691078424,5.44865951108031,126.405457301267));
#265823=CARTESIAN_POINT('Ctrl Pts',(90.8461214840295,-0.755788386771977,
123.84253436519));
#265824=CARTESIAN_POINT('Ctrl Pts',(90.5676738602166,-6.26570367949625,
127.677189650927));
#265825=CARTESIAN_POINT('Ctrl Pts',(90.2892262364038,-6.01774338740505,
134.38556228421));
#265826=CARTESIAN_POINT('Ctrl Pts',(90.0107786125907,-0.239770905396614,
137.802985537273));
#265827=CARTESIAN_POINT('Ctrl Pts',(89.7323309887781,5.75853932521132,134.78901439096));
#265828=CARTESIAN_POINT('Ctrl Pts',(89.453883364965,6.46503323623579,128.113341088056));
#265829=CARTESIAN_POINT('Ctrl Pts',(89.1754357411521,1.23047743759138,123.910583269158));
#265830=CARTESIAN_POINT('Ctrl Pts',(88.8969881173393,-5.13482701403487,
126.042870053701));
#265831=CARTESIAN_POINT('Ctrl Pts',(88.6185404935264,-6.78147629000823,
132.550734054689));
#265832=CARTESIAN_POINT('Ctrl Pts',(88.3400928697134,-2.19628014899849,
137.453766182047));
#265833=CARTESIAN_POINT('Ctrl Pts',(88.0616452459006,4.4071901546906,136.246319437167));
#265834=CARTESIAN_POINT('Ctrl Pts',(87.7831976220877,6.96066800942769,130.037978391542));
#265835=CARTESIAN_POINT('Ctrl Pts',(87.5047499982748,3.1176320110373,124.533905171779));
#265836=CARTESIAN_POINT('Ctrl Pts',(87.2263023744621,-3.59035550070555,
124.792074177916));
#265837=CARTESIAN_POINT('Ctrl Pts',(86.9478547506488,-6.99898170591706,
130.57524070557));
#265838=CARTESIAN_POINT('Ctrl Pts',(86.6694071268362,-3.97588564265574,
136.568957239218));
#265839=CARTESIAN_POINT('Ctrl Pts',(86.3909595030232,2.70085509339449,137.265291093768));
#265840=CARTESIAN_POINT('Ctrl Pts',(86.1125118792103,6.89564194272181,132.024345474689));
#265841=CARTESIAN_POINT('Ctrl Pts',(85.8340642553976,4.75367071752436,125.662293371487));
#265842=CARTESIAN_POINT('Ctrl Pts',(85.5556166315845,-1.75669166735309,
124.025549863481));
#265843=CARTESIAN_POINT('Ctrl Pts',(85.2771690077717,-6.65274022909182,
128.618202275162));
#265844=CARTESIAN_POINT('Ctrl Pts',(84.9987213839588,-5.4352455247236,135.21982740374));
#265845=CARTESIAN_POINT('Ctrl Pts',(84.7202737601459,0.776974290360158,
137.763854263368));
#265846=CARTESIAN_POINT('Ctrl Pts',(84.4418261363329,6.27519268990729,133.912446452669));
#265847=CARTESIAN_POINT('Ctrl Pts',(84.1633785125202,6.00681556763514,127.204859597945));
#265848=CARTESIAN_POINT('Ctrl Pts',(83.8849308887072,0.218468387960617,
123.805038334852));
#265849=CARTESIAN_POINT('Ctrl Pts',(83.6064832648944,-5.77064056747553,
126.837252313669));
#265850=CARTESIAN_POINT('Ctrl Pts',(83.3280356410814,-6.45681275286598,
133.515045019753));
#265851=CARTESIAN_POINT('Ctrl Pts',(83.0495880172686,-1.20948945121144,
137.701851184522));
#265852=CARTESIAN_POINT('Ctrl Pts',(82.7711403934555,5.14929556926191,135.550200479404));
#265853=CARTESIAN_POINT('Ctrl Pts',(82.4926927696429,6.77612951865689,129.037354788424));
#265854=CARTESIAN_POINT('Ctrl Pts',(82.2142451458298,2.17603147273656,124.148301131391));
#265855=CARTESIAN_POINT('Ctrl Pts',(81.9357975220171,-4.42373319158141,
125.375840975569));
#265856=CARTESIAN_POINT('Ctrl Pts',(81.6573498982041,-6.95830316421689,
131.591925172815));
#265857=CARTESIAN_POINT('Ctrl Pts',(81.3789022743912,-3.09853246094448,
137.084276018453));
#265858=CARTESIAN_POINT('Ctrl Pts',(81.1004546505783,3.60863820220999,136.805691401599));
#265859=CARTESIAN_POINT('Ctrl Pts',(80.8220070267654,6.99964664931016,131.012176975526));
#265860=CARTESIAN_POINT('Ctrl Pts',(80.5435594029525,3.95832177744353,125.02768946888));
#265861=CARTESIAN_POINT('Ctrl Pts',(80.2651117791397,-2.72050743312451,
124.351680541802));
#265862=CARTESIAN_POINT('Ctrl Pts',(79.9866641553267,-6.89932321682792,
129.605369373404));
#265863=CARTESIAN_POINT('Ctrl Pts',(79.7082165315139,-4.73799801494326,
135.960872584412));
#265864=CARTESIAN_POINT('Ctrl Pts',(79.4297689077009,1.77731589860328,137.577793207502));
#265865=CARTESIAN_POINT('Ctrl Pts',(79.1513212838881,6.65936332804202,132.970260181018));
#265866=CARTESIAN_POINT('Ctrl Pts',(78.8728736600752,5.42178118699497,126.372371265798));
#265867=CARTESIAN_POINT('Ctrl Pts',(78.5944260362623,-0.798152996164653,
123.847264050135));
#265868=CARTESIAN_POINT('Ctrl Pts',(78.3159784124494,-6.28462356779051,
127.715388706879));
#265869=CARTESIAN_POINT('Ctrl Pts',(78.0375307886365,-5.99583210154638,
134.422127644877));
#265870=CARTESIAN_POINT('Ctrl Pts',(77.7590831648237,-0.197163846663491,
137.804315422519));
#265871=CARTESIAN_POINT('Ctrl Pts',(77.4806355410107,5.78268835131386,134.753886701214));
#265872=CARTESIAN_POINT('Ctrl Pts',(77.2021879171979,6.44853245446487,128.07403645411));
#265873=CARTESIAN_POINT('Ctrl Pts',(76.9237402933849,1.18849026028645,123.903220729472));
#265874=CARTESIAN_POINT('Ctrl Pts',(76.6452926695721,-5.16371642211823,
126.074215422566));
#265875=CARTESIAN_POINT('Ctrl Pts',(76.3668450457591,-6.77071997416741,
132.591982469425));
#265876=CARTESIAN_POINT('Ctrl Pts',(76.0883974219463,-2.15576263801617,
137.467012364608));
#265877=CARTESIAN_POINT('Ctrl Pts',(75.8099497981334,4.44023524761227,136.219390792892));
#265878=CARTESIAN_POINT('Ctrl Pts',(75.5315021743204,6.95587385823614,129.995621028982));
#265879=CARTESIAN_POINT('Ctrl Pts',(75.2530545505077,3.0794042064702,124.515043437855));
#265880=CARTESIAN_POINT('Ctrl Pts',(74.9746069266946,-3.62688747378295,
124.814041084656));
#265881=CARTESIAN_POINT('Ctrl Pts',(74.6961593028819,-7.0002467489329,130.617849738824));
#265882=CARTESIAN_POINT('Ctrl Pts',(74.4177116790688,-3.94072124287924,
136.593052778991));
#265883=CARTESIAN_POINT('Ctrl Pts',(74.1392640552561,2.74013457044532,137.248730516143));
#265884=CARTESIAN_POINT('Ctrl Pts',(73.860816431443,6.90294057654623,131.982347141473));
#265885=CARTESIAN_POINT('Ctrl Pts',(73.5823688076304,4.72228142019582,125.633451699173));
#265886=CARTESIAN_POINT('Ctrl Pts',(73.3039211838172,-1.79792366504193,
124.036368939932));
#265887=CARTESIAN_POINT('Ctrl Pts',(73.0254735600045,-6.66592473556012,
128.658739897661));
#265888=CARTESIAN_POINT('Ctrl Pts',(72.7470259361915,-5.40826662262595,
135.252831477583));
#265889=CARTESIAN_POINT('Ctrl Pts',(72.4685783123786,0.819324307988826,
137.758995657032));
#265890=CARTESIAN_POINT('Ctrl Pts',(72.1901306885658,6.2939962257795,133.87418998802));
#265891=CARTESIAN_POINT('Ctrl Pts',(71.9116830647529,5.98479309088811,127.168361097063));
#265892=CARTESIAN_POINT('Ctrl Pts',(71.63323544094,0.17585747886725,123.803838136996));
#265893=CARTESIAN_POINT('Ctrl Pts',(71.3547878171271,-5.79468256511725,
126.872453342036));
#265894=CARTESIAN_POINT('Ctrl Pts',(71.0763401933142,-6.44019241774003,
133.554299248939));
#265895=CARTESIAN_POINT('Ctrl Pts',(70.7978925695013,-1.16748005934989,
137.709085895581));
#265896=CARTESIAN_POINT('Ctrl Pts',(70.5194449456884,5.17808943901089,135.518767326308));
#265897=CARTESIAN_POINT('Ctrl Pts',(70.2409973218756,6.76524770665308,128.996139303274));
#265898=CARTESIAN_POINT('Ctrl Pts',(69.9625496980626,2.1354738326052,124.135178331551));
#265899=CARTESIAN_POINT('Ctrl Pts',(69.6841020742497,-4.45669616991057,
125.402870073008));
#265900=CARTESIAN_POINT('Ctrl Pts',(69.4056544504369,-6.95338011399016,
131.634267747431));
#265901=CARTESIAN_POINT('Ctrl Pts',(69.1272068266238,-3.06024742481583,
137.103021312725));
#265902=CARTESIAN_POINT('Ctrl Pts',(68.8487592028112,3.64510314636624,136.783613405848));
#265903=CARTESIAN_POINT('Ctrl Pts',(68.5703115789981,7.00078199922599,130.969564289278));
#265904=CARTESIAN_POINT('Ctrl Pts',(68.2918639551854,3.92308420201135,125.003701069051));
#265905=CARTESIAN_POINT('Ctrl Pts',(68.0134163313723,-2.75973632353393,
124.368360595937));
#265906=CARTESIAN_POINT('Ctrl Pts',(67.7349687075595,-6.90649398836592,
129.647389726619));
#265907=CARTESIAN_POINT('Ctrl Pts',(67.4565210837467,-4.70652107887851,
135.98961858491));
#265908=CARTESIAN_POINT('Ctrl Pts',(67.1780734599337,1.81851477576126,137.566848685147));
#265909=CARTESIAN_POINT('Ctrl Pts',(66.8996258361208,6.67242439086218,132.929682617185));
#265910=CARTESIAN_POINT('Ctrl Pts',(66.6211782123079,5.39470195681365,126.339449459324));
#265911=CARTESIAN_POINT('Ctrl Pts',(66.3427305884951,-0.840488029704522,
123.852251532852));
#265912=CARTESIAN_POINT('Ctrl Pts',(66.0642829646821,-6.30331057704718,
127.753702225821));
#265913=CARTESIAN_POINT('Ctrl Pts',(65.7858353408693,-5.97369863792435,
134.458558947856));
#265914=CARTESIAN_POINT('Ctrl Pts',(65.5073877170563,-0.154549481951222,
137.805385921867));
#265915=CARTESIAN_POINT('Ctrl Pts',(65.2289400932435,5.80662309777304,134.718612660325));
#265916=CARTESIAN_POINT('Ctrl Pts',(64.9504924694306,6.43179271995227,128.03483299333));
#265917=CARTESIAN_POINT('Ctrl Pts',(64.6720448456177,1.14645904303803,123.896113914062));
#265918=CARTESIAN_POINT('Ctrl Pts',(64.3935972218049,-5.19241448679041,
126.1057360687));
#265919=CARTESIAN_POINT('Ctrl Pts',(64.1151495979918,-6.75971276680813,
132.633164643176));
#265920=CARTESIAN_POINT('Ctrl Pts',(63.8367019741791,-2.11516524445634,
137.480011660159));
#265921=CARTESIAN_POINT('Ctrl Pts',(63.5582543503661,4.47311580598391,136.192261492683));
#265922=CARTESIAN_POINT('Ctrl Pts',(63.2798067265533,6.95082195458075,129.953293634565));
#265923=CARTESIAN_POINT('Ctrl Pts',(63.0013591027403,3.041062293448,124.496414756892));
#265924=CARTESIAN_POINT('Ctrl Pts',(62.7229114789275,-3.66328505121137,
124.836229964889));
#265925=CARTESIAN_POINT('Ctrl Pts',(62.4444638551145,-7.00125239523119,
130.660465683307));
#265926=CARTESIAN_POINT('Ctrl Pts',(62.1660162313017,-3.90541081822766,
136.616933816649));
#265927=CARTESIAN_POINT('Ctrl Pts',(61.8875686074887,2.77931251080179,137.231931140021));
#265928=CARTESIAN_POINT('Ctrl Pts',(61.609120983676,6.909983419369,131.940305157533));
#265929=CARTESIAN_POINT('Ctrl Pts',(61.3306733598629,4.69071713699276,125.604801636791));
#265930=CARTESIAN_POINT('Ctrl Pts',(61.0522257360502,-1.83908904000824,
124.047438806804));
#265931=CARTESIAN_POINT('Ctrl Pts',(60.7737781122372,-6.67886223373588,
128.699357026925));
#265932=CARTESIAN_POINT('Ctrl Pts',(60.4953304884244,-5.38108731521968,
135.285670711703));
#265933=CARTESIAN_POINT('Ctrl Pts',(60.2168828646114,0.861643965253713,
137.753879344138));
#265934=CARTESIAN_POINT('Ctrl Pts',(59.9384352407986,6.31256653530686,133.835819769716));
#265935=CARTESIAN_POINT('Ctrl Pts',(59.6599876169856,5.96254884543232,127.131997329482));
#265936=CARTESIAN_POINT('Ctrl Pts',(59.3815399931728,0.133240053310041,
123.802897346075));
#265937=CARTESIAN_POINT('Ctrl Pts',(59.1030923693598,-5.81850983866561,
126.907800068673));
#265938=CARTESIAN_POINT('Ctrl Pts',(58.824644745547,-6.42333343891552,133.593451578138));
#265939=CARTESIAN_POINT('Ctrl Pts',(58.5461971217341,-1.12542740608588,
137.716064749505));
#265940=CARTESIAN_POINT('Ctrl Pts',(58.2677494979212,5.20669143275151,135.487159479138));
#265941=CARTESIAN_POINT('Ctrl Pts',(57.9893018741083,6.75411520590753,128.954990822428));
#265942=CARTESIAN_POINT('Ctrl Pts',(57.7108542502954,2.09483706170563,124.122302660713));
#265943=CARTESIAN_POINT('Ctrl Pts',(57.4324066264825,-4.48949400372376,
125.430099324666));
#265944=CARTESIAN_POINT('Ctrl Pts',(57.1539590026696,-6.94819940370625,
131.676579569534));
#265945=CARTESIAN_POINT('Ctrl Pts',(56.8755113788568,-3.02184899009409,
137.121533207807));
#265946=CARTESIAN_POINT('Ctrl Pts',(56.5970637550437,3.68143301988451,136.761313846687));
#265947=CARTESIAN_POINT('Ctrl Pts',(56.318616131231,7.00165793259049,130.926945481348));
#265948=CARTESIAN_POINT('Ctrl Pts',(56.040168507418,3.88770125525153,124.979927614796));
#265949=CARTESIAN_POINT('Ctrl Pts',(55.7617208836052,-2.79886295089852,
124.385279138419));
#265950=CARTESIAN_POINT('Ctrl Pts',(55.4832732597923,-6.91340883722955,
129.689452951814));
#265951=CARTESIAN_POINT('Ctrl Pts',(55.2048256359794,-4.67486974094423,
136.018172443767));
#265952=CARTESIAN_POINT('Ctrl Pts',(54.9263780121665,1.85964626718557,137.555653576309));
#265953=CARTESIAN_POINT('Ctrl Pts',(54.6479303883536,6.68523820454244,132.889026298762));
#265954=CARTESIAN_POINT('Ctrl Pts',(54.3694827645407,5.36742282396772,126.306693101776));
#265955=CARTESIAN_POINT('Ctrl Pts',(54.0910351407278,-0.882791918651148,
123.857496628527));
#265956=CARTESIAN_POINT('Ctrl Pts',(53.8125875169149,-6.32176401481248,
127.792128788032));
#265957=CARTESIAN_POINT('Ctrl Pts',(53.534139893102,-5.95134381670231,134.494854843172));
#265958=CARTESIAN_POINT('Ctrl Pts',(53.2556922692892,-0.111929390351441,
137.806196995646));
#265959=CARTESIAN_POINT('Ctrl Pts',(52.9772446454762,5.83034267767769,134.683193575387));
#265960=CARTESIAN_POINT('Ctrl Pts',(52.6987970216634,6.41481465299549,127.995732158415));
#265961=CARTESIAN_POINT('Ctrl Pts',(52.4203493978505,1.10438534332797,123.889263086274));
#265962=CARTESIAN_POINT('Ctrl Pts',(52.1419017740376,-5.22092014463445,
126.137430824095));
#265963=CARTESIAN_POINT('Ctrl Pts',(51.8634541502246,-6.74845507580631,
132.674279049921));
#265964=CARTESIAN_POINT('Ctrl Pts',(51.5850065264118,-2.07448947267055,
137.492763587005));
#265965=CARTESIAN_POINT('Ctrl Pts',(51.3065589025989,4.50583061140446,136.164932541826));
#265966=CARTESIAN_POINT('Ctrl Pts',(51.028111278786,6.94551248566166,129.910997776748));
#265967=CARTESIAN_POINT('Ctrl Pts',(50.7496636549731,3.00260769274395,124.478019819181));
#265968=CARTESIAN_POINT('Ctrl Pts',(50.4712160311602,-3.69954688426507,
124.858639996399));
#265969=CARTESIAN_POINT('Ctrl Pts',(50.1927684073473,-7.00199860754717,
130.70308695987));
#265970=CARTESIAN_POINT('Ctrl Pts',(49.9143207835345,-3.86995567714208,
136.640599467269));
#265971=CARTESIAN_POINT('Ctrl Pts',(49.6358731597215,2.81838746271124,137.214893587909));
#265972=CARTESIAN_POINT('Ctrl Pts',(49.3574255359087,6.91677021021505,131.89822108075));
#265973=CARTESIAN_POINT('Ctrl Pts',(49.0789779120958,4.65897903754105,125.576344245977));
#265974=CARTESIAN_POINT('Ctrl Pts',(48.8005302882828,-1.88018626685394,
124.058759053897));
#265975=CARTESIAN_POINT('Ctrl Pts',(48.5220826644701,-6.69155224421552,
128.740052157871));
#265976=CARTESIAN_POINT('Ctrl Pts',(48.243635040657,-5.35370860964396,135.318343889229));
#265977=CARTESIAN_POINT('Ctrl Pts',(47.9651874168443,0.903931693984841,
137.748505514272));
#265978=CARTESIAN_POINT('Ctrl Pts',(47.6867397930313,6.33090293035988,133.797337219578));
#265979=CARTESIAN_POINT('Ctrl Pts',(47.4082921692184,5.94008365553619,127.095769642671));
#265980=CARTESIAN_POINT('Ctrl Pts',(47.1298445454056,0.0906176904940206,
123.80221599695));
#265981=CARTESIAN_POINT('Ctrl Pts',(46.8513969215926,-5.84212150519187,
126.943291183793));
#265982=CARTESIAN_POINT('Ctrl Pts',(46.5729492977799,-6.40623644110861,
133.632500556544));
#265983=CARTESIAN_POINT('Ctrl Pts',(46.2945016739667,-1.08333304969514,
137.722787487691));
#265984=CARTESIAN_POINT('Ctrl Pts',(46.016054050154,5.23510049062639,135.455378109134));
#265985=CARTESIAN_POINT('Ctrl Pts',(45.737606426341,6.7427324289391,128.913910870662));
#265986=CARTESIAN_POINT('Ctrl Pts',(45.4591588025282,2.0541226658487,124.10967459599));
#265987=CARTESIAN_POINT('Ctrl Pts',(45.1807111787153,-4.5221254776858,125.457527721552));
#265988=CARTESIAN_POINT('Ctrl Pts',(44.9022635549024,-6.94276122533821,
131.718859071242));
#265989=CARTESIAN_POINT('Ctrl Pts',(44.6238159310895,-2.98333857964632,
137.139811017737));
#265990=CARTESIAN_POINT('Ctrl Pts',(44.3453683072766,3.71762647654865,136.738793550433));
#265991=CARTESIAN_POINT('Ctrl Pts',(44.0669206834637,7.00227441694529,130.88432213099));
#265992=CARTESIAN_POINT('Ctrl Pts',(43.7884730596509,3.85217424829189,124.956369987047));
#265993=CARTESIAN_POINT('Ctrl Pts',(43.5100254358379,-2.8378858653675,124.402435542326));
#265994=CARTESIAN_POINT('Ctrl Pts',(43.2315778120251,-6.92006750718621,
129.731557490323));
#265995=CARTESIAN_POINT('Ctrl Pts',(42.9531301882121,-4.64304517399252,
136.04653310291));
#265996=CARTESIAN_POINT('Ctrl Pts',(42.6746825643993,1.90070884873357,137.544208295828));
#265997=CARTESIAN_POINT('Ctrl Pts',(42.3962349405864,6.69780429426274,132.848292732287));
#265998=CARTESIAN_POINT('Ctrl Pts',(42.1177873167735,5.33994479929498,126.274103406951));
#265999=CARTESIAN_POINT('Ctrl Pts',(41.8393396929606,-0.925063095418803,
123.862999142802));
#266000=CARTESIAN_POINT('Ctrl Pts',(41.5608920691476,-6.33998319728738,
127.8306669696));
#266001=CARTESIAN_POINT('Ctrl Pts',(41.2824444453348,-5.92876846624656,
134.531013985867));
#266002=CARTESIAN_POINT('Ctrl Pts',(41.0039968215219,-0.069305151166692,
137.806748613804));
#266003=CARTESIAN_POINT('Ctrl Pts',(40.725549197709,5.85384621209049,134.647630758868));
#266004=CARTESIAN_POINT('Ctrl Pts',(40.4471015738961,6.39759888272248,127.956735398261));
#266005=CARTESIAN_POINT('Ctrl Pts',(40.1686539500832,1.06227072021291,123.882668499967));
#266006=CARTESIAN_POINT('Ctrl Pts',(39.8902063262704,-5.24923233936253,
126.169298514289));
#266007=CARTESIAN_POINT('Ctrl Pts',(39.6117587024575,-6.73694731831984,
132.715324166149));
#266008=CARTESIAN_POINT('Ctrl Pts',(39.3333110786445,-2.03373682991476,
137.505267672621));
#266009=CARTESIAN_POINT('Ctrl Pts',(39.0548634548317,4.53837845161457,136.137404953004));
#266010=CARTESIAN_POINT('Ctrl Pts',(38.7764158310188,6.9399456482232,129.86873502282));
#266011=CARTESIAN_POINT('Ctrl Pts',(38.4979682072059,2.96404182930761,124.459859306355));
#266012=CARTESIAN_POINT('Ctrl Pts',(38.219520583393,-3.73567162924815,124.881270348773));
#266013=CARTESIAN_POINT('Ctrl Pts',(37.9410729595801,-7.00248535822977,
130.745711989165));
#266014=CARTESIAN_POINT('Ctrl Pts',(37.6626253357672,-3.83435713342598,
136.664048853912));
#266015=CARTESIAN_POINT('Ctrl Pts',(37.3841777119543,2.8573579782368,137.197618491141));
#266016=CARTESIAN_POINT('Ctrl Pts',(37.1057300881414,6.92330069759731,131.856096470565));
#266017=CARTESIAN_POINT('Ctrl Pts',(36.8272824643285,4.62706829790778,125.548080581235));
#266018=CARTESIAN_POINT('Ctrl Pts',(36.5488348405156,-1.92121382270608,
124.070329261737));
#266019=CARTESIAN_POINT('Ctrl Pts',(36.2703872167028,-6.70399429676593,
128.780823782526));
#266020=CARTESIAN_POINT('Ctrl Pts',(35.9919395928899,-5.32613152042688,
135.350849799446));
#266021=CARTESIAN_POINT('Ctrl Pts',(35.7134919690769,0.946185927194629,
137.742874366562));
#266022=CARTESIAN_POINT('Ctrl Pts',(35.4350443452641,6.34900473147662,133.758743763591));
#266023=CARTESIAN_POINT('Ctrl Pts',(35.1565967214512,5.91739835365575,127.059679379064));
#266024=CARTESIAN_POINT('Ctrl Pts',(34.8781490976383,0.0479919698059151,
123.80179411487));
#266025=CARTESIAN_POINT('Ctrl Pts',(34.5997014738253,-5.8655166897575,126.978925372262));
#266026=CARTESIAN_POINT('Ctrl Pts',(34.3212538500126,-6.38890205785425,
133.671444737187));
#266027=CARTESIAN_POINT('Ctrl Pts',(34.0428062261996,-1.04119854999986,
137.729253861025));
#266028=CARTESIAN_POINT('Ctrl Pts',(33.7643586023867,5.26331555992738,135.423424393967));
#266029=CARTESIAN_POINT('Ctrl Pts',(33.4859109785738,6.73109979754094,128.872900970206));
#266030=CARTESIAN_POINT('Ctrl Pts',(33.207463354761,2.01333215372067,124.097294605319));
#266031=CARTESIAN_POINT('Ctrl Pts',(32.9290157309481,-4.55458938262534,
125.485154247296));
#266032=CARTESIAN_POINT('Ctrl Pts',(32.6505681071352,-6.93706578039975,
131.761104685873));
#266033=CARTESIAN_POINT('Ctrl Pts',(32.3721204833222,-2.94471762049033,
137.157854065221));
#266034=CARTESIAN_POINT('Ctrl Pts',(32.0936728595094,3.75368217519627,136.716053351584));
#266035=CARTESIAN_POINT('Ctrl Pts',(31.8152252356965,7.00263142944649,130.84169581763));
#266036=CARTESIAN_POINT('Ctrl Pts',(31.5367776118836,3.8165044975991,124.933029058741));
#266037=CARTESIAN_POINT('Ctrl Pts',(31.2583299880707,-2.87680362093211,
124.41982917192));
#266038=CARTESIAN_POINT('Ctrl Pts',(30.9798823642578,-6.92646975149653,
129.773701781947));
#266039=CARTESIAN_POINT('Ctrl Pts',(30.7014347404449,-4.6110485572945,136.074699511423));
#266040=CARTESIAN_POINT('Ctrl Pts',(30.422987116632,1.94170099881587,137.532513267813));
#266041=CARTESIAN_POINT('Ctrl Pts',(30.1445394928192,6.71012219438185,132.807483427156));
#266042=CARTESIAN_POINT('Ctrl Pts',(29.8660918690062,5.31226890100394,126.241681582474));
#266043=CARTESIAN_POINT('Ctrl Pts',(29.5876442451933,-0.967299993633269,
123.868758871779));
#266044=CARTESIAN_POINT('Ctrl Pts',(29.3091966213805,-6.35796744935336,
127.869315342481));
#266045=CARTESIAN_POINT('Ctrl Pts',(29.0307489975676,-5.90597342309497,
134.567035036052));
#266046=CARTESIAN_POINT('Ctrl Pts',(28.7523013737546,-0.026678343854083,
137.807040755898));
#266047=CARTESIAN_POINT('Ctrl Pts',(28.4738537499418,5.87713283007914,134.611925528561));
#266048=CARTESIAN_POINT('Ctrl Pts',(28.1954061261289,6.38014604707014,127.917844157905));
#266049=CARTESIAN_POINT('Ctrl Pts',(27.916958502316,1.02011673426565,123.876330399509));
#266050=CARTESIAN_POINT('Ctrl Pts',(27.6385108785031,-5.27735002185588,
126.201337958415));
#266051=CARTESIAN_POINT('Ctrl Pts',(27.3600632546902,-6.72518992077305,
132.756298470923));
#266052=CARTESIAN_POINT('Ctrl Pts',(27.0816156308773,-1.99290882629253,
137.51752345366));
#266053=CARTESIAN_POINT('Ctrl Pts',(26.8031680070644,4.57075812054227,136.109679746264));
#266054=CARTESIAN_POINT('Ctrl Pts',(26.5247203832516,6.93412164854658,129.826506938842));
#266055=CARTESIAN_POINT('Ctrl Pts',(26.2462727594386,2.92536613221128,124.441933891359));
#266056=CARTESIAN_POINT('Ctrl Pts',(25.9678251356258,-3.7716579475455,124.904120183435));
#266057=CARTESIAN_POINT('Ctrl Pts',(25.6893775118128,-7.00271262924226,
130.788339191706));
#266058=CARTESIAN_POINT('Ctrl Pts',(25.410929888,-3.79861650619593,136.687281107654));
#266059=CARTESIAN_POINT('Ctrl Pts',(25.1324822641871,2.89622261331168,137.180106489852));
#266060=CARTESIAN_POINT('Ctrl Pts',(24.8540346403742,6.92957463952618,131.813932887921));
#266061=CARTESIAN_POINT('Ctrl Pts',(24.5755870165613,4.59498610055721,125.520011689881));
#266062=CARTESIAN_POINT('Ctrl Pts',(24.2971393927484,-1.96217018727317,
124.082149001586));
#266063=CARTESIAN_POINT('Ctrl Pts',(24.0186917689355,-6.71618793034234,
128.821670390082));
#266064=CARTESIAN_POINT('Ctrl Pts',(23.7402441451226,-5.29835706944761,
135.383187237832));
#266065=CARTESIAN_POINT('Ctrl Pts',(23.4617965213097,0.988405099136929,
137.736986109674));
#266066=CARTESIAN_POINT('Ctrl Pts',(23.1833488974968,6.36687126788796,133.720040831851));
#266067=CARTESIAN_POINT('Ctrl Pts',(22.9049012736839,5.89449378040337,127.023727875996));
#266068=CARTESIAN_POINT('Ctrl Pts',(22.6264536498711,0.00536447075796404,
123.801631715467));
#266069=CARTESIAN_POINT('Ctrl Pts',(22.3480060260581,-5.88869452544514,
127.01470131364));
#266070=CARTESIAN_POINT('Ctrl Pts',(22.0695584022453,-6.3713309314846,133.710282676972));
#266071=CARTESIAN_POINT('Ctrl Pts',(21.7911107784324,-0.999025468309402,
137.735463629893));
#266072=CARTESIAN_POINT('Ctrl Pts',(21.5126631546195,5.29133559513472,135.391299517692));
#266073=CARTESIAN_POINT('Ctrl Pts',(21.2342155308066,6.71921774276442,128.831962640697));
#266074=CARTESIAN_POINT('Ctrl Pts',(20.9557679069937,1.97246703682929,124.085163147446));
#266075=CARTESIAN_POINT('Ctrl Pts',(20.6773202831809,-4.58688451558038,
125.51297787819));
#266076=CARTESIAN_POINT('Ctrl Pts',(20.3988726593679,-6.93111327993769,
131.803314848003));
#266077=CARTESIAN_POINT('Ctrl Pts',(20.120425035555,-2.90598754374001,137.175661681671));
#266078=CARTESIAN_POINT('Ctrl Pts',(19.8419774117421,3.78959877977074,136.693094092787));
#266079=CARTESIAN_POINT('Ctrl Pts',(19.5635297879293,7.00272895686486,130.799068120799));
#266080=CARTESIAN_POINT('Ctrl Pts',(19.2850821641163,3.78069332492835,124.909905694786));
#266081=CARTESIAN_POINT('Ctrl Pts',(19.0066345403035,-2.91561477548059,
124.437459382677));
#266082=CARTESIAN_POINT('Ctrl Pts',(18.7281869164906,-6.932615332923,129.815884265012));
#266083=CARTESIAN_POINT('Ctrl Pts',(18.4497392926777,-4.57888107649638,
136.102670625591));
#266084=CARTESIAN_POINT('Ctrl Pts',(18.1712916688647,1.98262119845391,137.520568925627));
#266085=CARTESIAN_POINT('Ctrl Pts',(17.892844045052,6.72219144845534,132.766599895572));
#266086=CARTESIAN_POINT('Ctrl Pts',(17.614396421239,5.28439615463518,126.209428829746));
#266087=CARTESIAN_POINT('Ctrl Pts',(17.3359487974261,-1.00950104819076,
123.87477560203));
#266088=CARTESIAN_POINT('Ctrl Pts',(17.0575011736132,-6.37571610459714,
127.908072474542));
#266089=CARTESIAN_POINT('Ctrl Pts',(16.7790535498004,-5.88295953192644,
134.602916658952));
#266090=CARTESIAN_POINT('Ctrl Pts',(16.5006059259874,0.0159494520341194,
137.807073411106));
#266091=CARTESIAN_POINT('Ctrl Pts',(16.2221583021745,5.90020166874948,134.576079207535));
#266092=CARTESIAN_POINT('Ctrl Pts',(15.9437106783617,6.3624567927597,127.879059878479));
#266093=CARTESIAN_POINT('Ctrl Pts',(15.6652630545488,0.977924947517885,
123.870249019757));
#266094=CARTESIAN_POINT('Ctrl Pts',(15.3868154307359,-5.3052721502032,126.233547969238));
#266095=CARTESIAN_POINT('Ctrl Pts',(15.108367806923,-6.71318331884074,132.797200445919));
#266096=CARTESIAN_POINT('Ctrl Pts',(14.8299201831101,-1.95200697470083,
137.529530475982));
#266097=CARTESIAN_POINT('Ctrl Pts',(14.5514725592972,4.6029684183469,136.081757948972));
#266098=CARTESIAN_POINT('Ctrl Pts',(14.2730249354843,6.92804070244224,129.784315089592));
#266099=CARTESIAN_POINT('Ctrl Pts',(13.9945773116714,2.88658203459712,124.424244238425));
#266100=CARTESIAN_POINT('Ctrl Pts',(13.7161296878585,-3.80750450567058,
124.927188653676));
#266101=CARTESIAN_POINT('Ctrl Pts',(13.4376820640456,-7.00268041216303,
130.830966987928));
#266102=CARTESIAN_POINT('Ctrl Pts',(13.1592344402328,-3.7627351198343,136.710295367612));
#266103=CARTESIAN_POINT('Ctrl Pts',(12.8807868164199,2.93497992779253,137.162358232954));
#266104=CARTESIAN_POINT('Ctrl Pts',(12.602339192607,6.93559180351842,131.771731895206));
#266105=CARTESIAN_POINT('Ctrl Pts',(12.323891568794,4.56273363430679,125.49213861202));
#266106=CARTESIAN_POINT('Ctrl Pts',(12.0454439449812,-2.00305384290271,
124.094217835458));
#266107=CARTESIAN_POINT('Ctrl Pts',(11.7669963211683,-6.72813269310505,
128.862590466954));
#266108=CARTESIAN_POINT('Ctrl Pts',(11.4885486973554,-5.27038628589867,
135.415355006116));
#266109=CARTESIAN_POINT('Ctrl Pts',(11.2101010735425,1.03058764536478,137.730840961799));
#266110=CARTESIAN_POINT('Ctrl Pts',(10.9316534497296,6.38450187754329,133.681229858508));
#266111=CARTESIAN_POINT('Ctrl Pts',(10.6532058259167,5.87137078451608,126.987916465666));
#266112=CARTESIAN_POINT('Ctrl Pts',(10.3747582021038,-0.0372632270726686,
123.801728804758));
#266113=CARTESIAN_POINT('Ctrl Pts',(10.0963105782909,-5.91165415339157,
127.050617682238));
#266114=CARTESIAN_POINT('Ctrl Pts',(9.81786295447806,-6.35352371310424,
133.749012936746));
#266115=CARTESIAN_POINT('Ctrl Pts',(9.53941533066515,-0.956815367363035,
137.741416564191));
#266116=CARTESIAN_POINT('Ctrl Pts',(9.26096770685226,5.31915955795546,135.35900467071));
#266117=CARTESIAN_POINT('Ctrl Pts',(8.98252008303941,6.70708670490366,128.791097399121));
#266118=CARTESIAN_POINT('Ctrl Pts',(8.70407245922646,1.93152882944647,124.073280671906));
#266119=CARTESIAN_POINT('Ctrl Pts',(8.42562483541358,-4.61900967984285,
125.540997583217));
#266120=CARTESIAN_POINT('Ctrl Pts',(8.14717721160073,-6.92490394452403,
131.845487993513));
#266121=CARTESIAN_POINT('Ctrl Pts',(7.86872958778781,-2.86714978455288,
137.193233207215));
#266122=CARTESIAN_POINT('Ctrl Pts',(7.59028196397491,3.82537495936868,136.669916624805));
#266123=CARTESIAN_POINT('Ctrl Pts',(7.31183434016203,7.00256699558648,130.756440620084));
#266124=CARTESIAN_POINT('Ctrl Pts',(7.03338671634916,3.7447420572761,124.887000752025));
#266125=CARTESIAN_POINT('Ctrl Pts',(6.75493909253623,-2.95431789085107,
124.455325521299));
#266126=CARTESIAN_POINT('Ctrl Pts',(6.47649146872337,-6.9385040237388,129.858103376433));
#266127=CARTESIAN_POINT('Ctrl Pts',(6.19804384491048,-4.54654392357636,
136.130445408932));
#266128=CARTESIAN_POINT('Ctrl Pts',(5.91959622109758,2.02346793133434,137.508375711873));
#266129=CARTESIAN_POINT('Ctrl Pts',(5.64114859728465,6.73401160925262,132.725643652489));
#266130=CARTESIAN_POINT('Ctrl Pts',(5.36270097347181,5.25632759302358,126.177346343905));
#266131=CARTESIAN_POINT('Ctrl Pts',(5.08425334965889,-1.05166469531565,
123.881049110601));
#266132=CARTESIAN_POINT('Ctrl Pts',(4.80580572584599,-6.39322850533622,
127.946936929627));
#266133=CARTESIAN_POINT('Ctrl Pts',(4.5273581020331,-5.85972764552883,134.638657524961));
#266134=CARTESIAN_POINT('Ctrl Pts',(4.24891047822024,0.0585766569097649,
137.806846578216));
#266135=CARTESIAN_POINT('Ctrl Pts',(3.97046285440732,5.92305187327717,134.54009312409));
#266136=CARTESIAN_POINT('Ctrl Pts',(3.69201523059441,6.34453177527304,127.840383997147));
#266137=CARTESIAN_POINT('Ctrl Pts',(3.41356760678156,0.935696923401329,
123.864424586062));
#266138=CARTESIAN_POINT('Ctrl Pts',(3.13511998296867,-5.33299768974021,
126.265927353204));
#266139=CARTESIAN_POINT('Ctrl Pts',(2.85667235915575,-6.70092795743158,
132.838028575505));
#266140=CARTESIAN_POINT('Ctrl Pts',(2.57822473534285,-1.91103279077285,
137.541288294661));
#266141=CARTESIAN_POINT('Ctrl Pts',(2.29977711153,4.63500815146407,136.053640595781));
#266142=CARTESIAN_POINT('Ctrl Pts',(2.02132948771708,6.92170303524179,129.742161038504));
#266143=CARTESIAN_POINT('Ctrl Pts',(1.74288186390418,2.84769097362441,124.40679100305));
#266144=CARTESIAN_POINT('Ctrl Pts',(1.46443424009131,-3.84320997531586,
124.950474904685));
#266145=CARTESIAN_POINT('Ctrl Pts',(1.18598661627842,-7.00238870818588,
130.873593798241));
#266146=CARTESIAN_POINT('Ctrl Pts',(0.907538992465495,-3.72671430393905,
136.733090780986));
#266147=CARTESIAN_POINT('Ctrl Pts',(0.629091368652655,2.97362848551254,
137.144374378117));
#266148=CARTESIAN_POINT('Ctrl Pts',(0.350643744839755,6.94135196660579,
131.729495056193));
#266149=CARTESIAN_POINT('Ctrl Pts',(0.0721961210268491,4.53031209428387,
125.4644623805));
#266150=CARTESIAN_POINT('Ctrl Pts',(-0.206251502786054,-2.04386327463549,
124.106535316138));
#266151=CARTESIAN_POINT('Ctrl Pts',(-0.484699126598912,-6.73982814243653,
128.903582496833));
#266152=CARTESIAN_POINT('Ctrl Pts',(-0.763146750411823,-5.24222020624778,
135.447351912307));
#266153=CARTESIAN_POINT('Ctrl Pts',(-1.04159437422473,1.07273200278813,
137.724439150648));
#266154=CARTESIAN_POINT('Ctrl Pts',(-1.32004199803759,6.40189590713365,
133.642312281717));
#266155=CARTESIAN_POINT('Ctrl Pts',(-1.59848962185049,5.84803022282516,
126.952246475077));
#266156=CARTESIAN_POINT('Ctrl Pts',(-1.87693724566341,-0.0798895441007186,
123.802085379146));
#266157=CARTESIAN_POINT('Ctrl Pts',(-2.1553848694763,-5.93439472281934,
127.08667314716));
#266158=CARTESIAN_POINT('Ctrl Pts',(-2.43383249328916,-6.33548106256618,
133.787634081347));
#266159=CARTESIAN_POINT('Ctrl Pts',(-2.71228011710207,-0.914569811271147,
137.747112443329));
#266160=CARTESIAN_POINT('Ctrl Pts',(-2.99072774091498,5.34678641736288,
135.326541049718));
#266161=CARTESIAN_POINT('Ctrl Pts',(-3.26917536472784,6.6947071334783,128.750306759754));
#266162=CARTESIAN_POINT('Ctrl Pts',(-3.54762298854074,1.89051904855254,
124.061647619009));
#266163=CARTESIAN_POINT('Ctrl Pts',(-3.82607061235365,-4.65096368500298,
125.569212324096));
#266164=CARTESIAN_POINT('Ctrl Pts',(-4.10451823616654,-6.91843800424817,
131.887622559669));
#266165=CARTESIAN_POINT('Ctrl Pts',(-4.38296585997939,-2.82820578207579,
137.210567990736));
#266166=CARTESIAN_POINT('Ctrl Pts',(-4.66141348379231,3.86100938829084,
136.646521806489));
#266167=CARTESIAN_POINT('Ctrl Pts',(-4.93986110760522,7.00214555161287,
130.713814895061));
#266168=CARTESIAN_POINT('Ctrl Pts',(-5.21830873141809,3.70865202682979,
124.864315079211));
#266169=CARTESIAN_POINT('Ctrl Pts',(-5.49675635523098,-2.99291153288594,
124.473426925751));
#266170=CARTESIAN_POINT('Ctrl Pts',(-5.77520397904388,-6.9441356057364,
129.900357551763));
#266171=CARTESIAN_POINT('Ctrl Pts',(-6.05365160285679,-4.51403829679898,
136.158022832244));
#266172=CARTESIAN_POINT('Ctrl Pts',(-6.33209922666964,2.06423968386644,
137.495934078373));
#266173=CARTESIAN_POINT('Ctrl Pts',(-6.61054685048256,6.74558223877327,
132.684616215558));
#266174=CARTESIAN_POINT('Ctrl Pts',(-6.88899447429547,5.22806425626005,
126.145435313781));
#266175=CARTESIAN_POINT('Ctrl Pts',(-7.16744209810832,-1.09378937261818,
123.887579165027));
#266176=CARTESIAN_POINT('Ctrl Pts',(-7.44588972192122,-6.41050400264194,
127.985907267597));
#266177=CARTESIAN_POINT('Ctrl Pts',(-7.72433734573414,-5.8362786247684,
134.674256309687));
#266178=CARTESIAN_POINT('Ctrl Pts',(-8.002784969547,0.101201691205851,137.806360265633));
#266179=CARTESIAN_POINT('Ctrl Pts',(-8.28123259335988,5.94568259693924,
134.503968611703));
#266180=CARTESIAN_POINT('Ctrl Pts',(-8.55968021717279,6.32637165882838,
127.80181794706));
#266181=CARTESIAN_POINT('Ctrl Pts',(-8.8381278409857,0.893434226691435,
123.858857314246));
#266182=CARTESIAN_POINT('Ctrl Pts',(-9.11657546479855,-5.3605256130866,
126.298474910485));
#266183=CARTESIAN_POINT('Ctrl Pts',(-9.39502308861147,-6.68842429067269,
132.878781346775));
#266184=CARTESIAN_POINT('Ctrl Pts',(-9.67347071242438,-1.86998779282204,
137.552796474009));
#266185=CARTESIAN_POINT('Ctrl Pts',(-9.95191833623725,4.66687613264966,
136.025328728591));
#266186=CARTESIAN_POINT('Ctrl Pts',(-10.2303659600501,6.91510888178999,
129.700046347612));
#266187=CARTESIAN_POINT('Ctrl Pts',(-10.508813583863,2.80869439041515,124.389574831969));
#266188=CARTESIAN_POINT('Ctrl Pts',(-10.787261207676,-3.87877303340228,
124.973978073582));
#266189=CARTESIAN_POINT('Ctrl Pts',(-11.0657088314888,-7.00183752812002,
130.916218043094));
#266190=CARTESIAN_POINT('Ctrl Pts',(-11.3441564553017,-3.69055539327479,
136.755666503084));
#266191=CARTESIAN_POINT('Ctrl Pts',(-11.6226040791146,3.01216685433575,
137.126155591738));
#266192=CARTESIAN_POINT('Ctrl Pts',(-11.9010517029275,6.94685491534338,
131.687223935982));
#266193=CARTESIAN_POINT('Ctrl Pts',(-12.1794993267404,4.49772268187999,
125.436984020872));
#266194=CARTESIAN_POINT('Ctrl Pts',(-12.4579469505533,-2.08459697026297,
124.119100987199));
#266195=CARTESIAN_POINT('Ctrl Pts',(-12.7363945743662,-6.75127384495765,
128.944644960744));
#266196=CARTESIAN_POINT('Ctrl Pts',(-13.0148421981791,-5.21385987419926,
135.479176770748));
#266197=CARTESIAN_POINT('Ctrl Pts',(-13.2932898219919,1.11483660973293,
137.717780913442));
#266198=CARTESIAN_POINT('Ctrl Pts',(-13.5717374458049,6.41905271211686,
133.603289543584));
#266199=CARTESIAN_POINT('Ctrl Pts',(-13.8501850696177,5.82447296022373,
126.916719225995));
#266200=CARTESIAN_POINT('Ctrl Pts',(-14.1286326934306,-0.122512900792341,
123.802701425419));
#266201=CARTESIAN_POINT('Ctrl Pts',(-14.4070803172435,-5.95691539106803,
127.122866372359));
#266202=CARTESIAN_POINT('Ctrl Pts',(-14.6855279410564,-6.31720364844761,
133.826144679651));
#266203=CARTESIAN_POINT('Ctrl Pts',(-14.9639755648693,-0.872290365458834,
137.752551056246));
#266204=CARTESIAN_POINT('Ctrl Pts',(-15.2424231886822,5.37421514963333,
135.293909857666));
#266205=CARTESIAN_POINT('Ctrl Pts',(-15.5208708124951,6.68207948721813,
128.709592234107));
#266206=CARTESIAN_POINT('Ctrl Pts',(-15.799318436308,1.84943921378025,124.050264419823));
#266207=CARTESIAN_POINT('Ctrl Pts',(-16.0777660601209,-4.68274534699314,
125.59762105532));
#266208=CARTESIAN_POINT('Ctrl Pts',(-16.3562136839338,-6.91171569870797,
131.929716985153));
#266209=CARTESIAN_POINT('Ctrl Pts',(-16.6346613077467,-2.78915697939336,
137.227665389888));
#266210=CARTESIAN_POINT('Ctrl Pts',(-16.9131089315595,3.89650074609022,
136.622910504741));
#266211=CARTESIAN_POINT('Ctrl Pts',(-17.1915565553724,7.00146464056082,
130.671192525245));
#266212=CARTESIAN_POINT('Ctrl Pts',(-17.4700041791854,3.67242457091876,
124.841849516969));
#266213=CARTESIAN_POINT('Ctrl Pts',(-17.7484518029982,-3.0313942714833,
124.491762925279));
#266214=CARTESIAN_POINT('Ctrl Pts',(-18.0268994268111,-6.94950987023543,
129.942645225261));
#266215=CARTESIAN_POINT('Ctrl Pts',(-18.305347050624,-4.48136540067248,
136.185401873632));
#266216=CARTESIAN_POINT('Ctrl Pts',(-18.5837946744369,2.10493494523792,
137.483244486159));
#266217=CARTESIAN_POINT('Ctrl Pts',(-18.8622422982498,6.75690290826339,
132.643519105064));
#266218=CARTESIAN_POINT('Ctrl Pts',(-19.1406899220627,5.19960719165284,
126.113696921846));
#266219=CARTESIAN_POINT('Ctrl Pts',(-19.4191375458756,-1.1358735191536,
123.894365523333));
#266220=CARTESIAN_POINT('Ctrl Pts',(-19.6975851696885,-6.42754195636435,
128.024982044393));
#266221=CARTESIAN_POINT('Ctrl Pts',(-19.9760327935014,-5.81261333855723,
134.709711694007));
#266222=CARTESIAN_POINT('Ctrl Pts',(-20.2544804173143,0.143822975436045,
137.805614491377));
#266223=CARTESIAN_POINT('Ctrl Pts',(-20.5329280411272,5.96809300114641,
134.467707008981));
#266224=CARTESIAN_POINT('Ctrl Pts',(-20.81137566494,6.30797711635522,127.763363157294));
#266225=CARTESIAN_POINT('Ctrl Pts',(-21.089823288753,0.851138423447451,
123.853547410611));
#266226=CARTESIAN_POINT('Ctrl Pts',(-21.3682709125658,-5.38785490018508,
126.331189435016));
#266227=CARTESIAN_POINT('Ctrl Pts',(-21.6467185363787,-6.67567278189203,
132.919457249623));
#266228=CARTESIAN_POINT('Ctrl Pts',(-21.9251661601916,-1.82887350178604,
137.564054587584));
#266229=CARTESIAN_POINT('Ctrl Pts',(-22.2036137840045,4.69857118102365,
135.996823396506));
#266230=CARTESIAN_POINT('Ctrl Pts',(-22.4820614078173,6.90825848643574,
129.657972577492));
#266231=CARTESIAN_POINT('Ctrl Pts',(-22.7605090316303,2.76959373000234,
124.372596363135));
#266232=CARTESIAN_POINT('Ctrl Pts',(-23.0389566554432,-3.91419236212754,
124.997697289448));
#266233=CARTESIAN_POINT('Ctrl Pts',(-23.3174042792561,-7.0010268923895,
130.958838143028));
#266234=CARTESIAN_POINT('Ctrl Pts',(-23.5958519030689,-3.65425972772349,
136.778021697354));
#266235=CARTESIAN_POINT('Ctrl Pts',(-23.8742995268818,3.05059360620828,
137.107702548922));
#266236=CARTESIAN_POINT('Ctrl Pts',(-24.1527471506948,6.95210044581739,
131.644920100946));
#266237=CARTESIAN_POINT('Ctrl Pts',(-24.4311947745076,4.4649666047081,125.409704551357));
#266238=CARTESIAN_POINT('Ctrl Pts',(-24.7096423983205,-2.12525342038311,
124.131914383013));
#266239=CARTESIAN_POINT('Ctrl Pts',(-24.9880900221334,-6.76246937654364,
128.985776337104));
#266240=CARTESIAN_POINT('Ctrl Pts',(-25.2665376459463,-5.18530634065569,
135.510828402156));
#266241=CARTESIAN_POINT('Ctrl Pts',(-25.5449852697592,1.15689990599717,
137.710866496904));
#266242=CARTESIAN_POINT('Ctrl Pts',(-25.8234328935721,6.43597165674122,
133.564163090109));
#266243=CARTESIAN_POINT('Ctrl Pts',(-26.101880517385,5.8006998696348,126.881336034893));
#266244=CARTESIAN_POINT('Ctrl Pts',(-26.3803281411979,-0.165131717723356,
123.803576920747));
#266245=CARTESIAN_POINT('Ctrl Pts',(-26.6587757650107,-5.9792153236265,
127.15919601668));
#266246=CARTESIAN_POINT('Ctrl Pts',(-26.9372233888237,-6.29869214802456,
133.864543304637));
#266247=CARTESIAN_POINT('Ctrl Pts',(-27.2156710126366,-0.829978596605981,
137.75773220141));
#266248=CARTESIAN_POINT('Ctrl Pts',(-27.4941186364494,5.40144473838504,
135.261112303716));
#266249=CARTESIAN_POINT('Ctrl Pts',(-27.7725662602623,6.66920423404522,
128.668955330874));
#266250=CARTESIAN_POINT('Ctrl Pts',(-28.0510138840753,1.80829084735756,
124.039131496154));
#266251=CARTESIAN_POINT('Ctrl Pts',(-28.3294615078881,-4.71435348813263,
125.626222724194));
#266252=CARTESIAN_POINT('Ctrl Pts',(-28.607909131701,-6.9047372770006,131.971769710144));
#266253=CARTESIAN_POINT('Ctrl Pts',(-28.8863567555139,-2.75000482347336,
137.244524771118));
#266254=CARTESIAN_POINT('Ctrl Pts',(-29.1648043793268,3.93184771762154,
136.599083594488));
#266255=CARTESIAN_POINT('Ctrl Pts',(-29.4432520031397,7.00052428766157,
130.628575090021));
#266256=CARTESIAN_POINT('Ctrl Pts',(-29.7216996269525,3.63606103196502,
124.819604897767));
#266257=CARTESIAN_POINT('Ctrl Pts',(-30.0001472507655,-3.06976468065099,
124.510332840438));
#266258=CARTESIAN_POINT('Ctrl Pts',(-30.2785948745783,-6.95462661809053,
129.984964829937));
#266259=CARTESIAN_POINT('Ctrl Pts',(-30.5570424983912,-4.44852644590303,
136.212581518559));
#266260=CARTESIAN_POINT('Ctrl Pts',(-30.8354901222041,2.14555220747066,
137.470307405446));
#266261=CARTESIAN_POINT('Ctrl Pts',(-31.113937746017,6.7679731982313,132.602353843876));
#266262=CARTESIAN_POINT('Ctrl Pts',(-31.3923853698299,5.17095745368924,
126.082132344179));
#266263=CARTESIAN_POINT('Ctrl Pts',(-31.6708329936428,-1.17791557547805,
123.901407934047));
#266264=CARTESIAN_POINT('Ctrl Pts',(-31.9492806174558,-6.44434173515584,
128.064159812084));
#266265=CARTESIAN_POINT('Ctrl Pts',(-32.2277282412685,-5.78873266382121,
134.745022364106));
#266266=CARTESIAN_POINT('Ctrl Pts',(-32.5061758650815,0.186438930252996,
137.804609283086));
#266267=CARTESIAN_POINT('Ctrl Pts',(-32.7846234888944,5.99028225547263,
134.431309659613));
#266268=CARTESIAN_POINT('Ctrl Pts',(-33.0630711127073,6.28934882947028,
127.725021052809));
#266269=CARTESIAN_POINT('Ctrl Pts',(-33.3415187365202,0.808811080956172,
123.848495071916));
#266270=CARTESIAN_POINT('Ctrl Pts',(-33.619966360333,-5.41498453833882,
126.364069714552));
#266271=CARTESIAN_POINT('Ctrl Pts',(-33.898413984146,-6.66267390360147,
132.960054776787));
#266272=CARTESIAN_POINT('Ctrl Pts',(-34.1768616079588,-1.78769144116968,
137.575062218212));
#266273=CARTESIAN_POINT('Ctrl Pts',(-34.4553092317717,4.73009212211488,
135.968125655805));
#266274=CARTESIAN_POINT('Ctrl Pts',(-34.7337568555846,6.90115210302259,
129.615941287202));
#266275=CARTESIAN_POINT('Ctrl Pts',(-35.0122044793975,2.73039044127535,
124.355856225691));
#266276=CARTESIAN_POINT('Ctrl Pts',(-35.2906521032104,-3.94946664901538,
125.02163167336));
#266277=CARTESIAN_POINT('Ctrl Pts',(-35.5690997270233,-6.99995683103299,
131.00145251874));
#266278=CARTESIAN_POINT('Ctrl Pts',(-35.8475473508362,-3.61782865223385,
136.800155535415));
#266279=CARTESIAN_POINT('Ctrl Pts',(-36.125994974649,3.08890731721304,137.089015933453));
#266280=CARTESIAN_POINT('Ctrl Pts',(-36.404442598462,6.95708836365274,131.60258511867));
#266281=CARTESIAN_POINT('Ctrl Pts',(-36.6828902222748,4.43204507655667,
125.382624982808));
#266282=CARTESIAN_POINT('Ctrl Pts',(-36.9613378460878,-2.16583111845593,
124.144975028777));
#266283=CARTESIAN_POINT('Ctrl Pts',(-37.2397854699006,-6.7734143223399,
129.026975101771));
#266284=CARTESIAN_POINT('Ctrl Pts',(-37.5182330937135,-5.15656066367905,
135.54230563367));
#266285=CARTESIAN_POINT('Ctrl Pts',(-37.7966807175264,1.19892033290996,
137.703696157251));
#266286=CARTESIAN_POINT('Ctrl Pts',(-38.0751283413393,6.45265211406898,
133.524934371139));
#266287=CARTESIAN_POINT('Ctrl Pts',(-38.3535759651522,5.77671183197903,
126.846098212911));
#266288=CARTESIAN_POINT('Ctrl Pts',(-38.6320235889651,-0.207744415637528,
123.80471183269));
#266289=CARTESIAN_POINT('Ctrl Pts',(-38.910471212778,-6.00129369416227,
127.195660733917));
#266290=CARTESIAN_POINT('Ctrl Pts',(-39.1889188365908,-6.27994724724761,
133.902828533427));
#266291=CARTESIAN_POINT('Ctrl Pts',(-39.4673664604039,-0.787636072591,137.762655686833));
#266292=CARTESIAN_POINT('Ctrl Pts',(-39.7458140842166,5.42847417461558,
135.228149603194));
#266293=CARTESIAN_POINT('Ctrl Pts',(-40.0242617080296,6.65608185105682,
128.628397555869));
#266294=CARTESIAN_POINT('Ctrl Pts',(-40.3027093318424,1.76707547405252,
124.028249260538));
#266295=CARTESIAN_POINT('Ctrl Pts',(-40.5811569556554,-4.7457869371699,
125.655016270872));
#266296=CARTESIAN_POINT('Ctrl Pts',(-40.8596045794682,-6.89750299771422,
132.013779176361));
#266297=CARTESIAN_POINT('Ctrl Pts',(-41.1380522032811,-2.7107507651133,
137.261145509698));
#266298=CARTESIAN_POINT('Ctrl Pts',(-41.416499827094,3.96704899308973,136.575041958643));
#266299=CARTESIAN_POINT('Ctrl Pts',(-41.694947450907,6.99932452776054,130.585964168594));
#266300=CARTESIAN_POINT('Ctrl Pts',(-41.9733950747197,3.59956275743227,
124.79758204589));
#266301=CARTESIAN_POINT('Ctrl Pts',(-42.2518426985328,-3.10802133855968,
124.529135983109));
#266302=CARTESIAN_POINT('Ctrl Pts',(-42.5302903223456,-6.95948565969872,
130.027314797628));
#266303=CARTESIAN_POINT('Ctrl Pts',(-42.8087379461585,-4.41552264935019,
136.23956075987));
#266304=CARTESIAN_POINT('Ctrl Pts',(-43.0871855699714,2.18608996547759,
137.457123315624));
#266305=CARTESIAN_POINT('Ctrl Pts',(-43.3656331937842,6.77879269846351,
132.561121957388));
#266306=CARTESIAN_POINT('Ctrl Pts',(-43.6440808175972,5.14211610399531,
126.050742750417));
#266307=CARTESIAN_POINT('Ctrl Pts',(-43.92252844141,-1.21991398370768,123.908706136214));
#266308=CARTESIAN_POINT('Ctrl Pts',(-44.200976065223,-6.46090271649442,
128.103439118922));
#266309=CARTESIAN_POINT('Ctrl Pts',(-44.4794236890358,-5.76463748546755,
134.780187011534));
#266310=CARTESIAN_POINT('Ctrl Pts',(-44.7578713128487,0.229047976506494,
137.803344678006));
#266311=CARTESIAN_POINT('Ctrl Pts',(-45.0363189366615,6.01224953768695,
134.394777912313));
#266312=CARTESIAN_POINT('Ctrl Pts',(-45.3147665604746,6.27048748845154,
127.686793054383));
#266313=CARTESIAN_POINT('Ctrl Pts',(-45.5932141842873,0.766453767672844,
123.843700485376));
#266314=CARTESIAN_POINT('Ctrl Pts',(-45.8716618081003,-5.44191352224889,
126.397114530699));
#266315=CARTESIAN_POINT('Ctrl Pts',(-46.1501094319132,-6.6494281374793,
133.000572423912));
#266316=CARTESIAN_POINT('Ctrl Pts',(-46.4285570557261,-1.74644313698983,
137.585818958004));
#266317=CARTESIAN_POINT('Ctrl Pts',(-46.7070046795389,4.76143778790304,
135.93923656989));
#266318=CARTESIAN_POINT('Ctrl Pts',(-46.9854523033519,6.89378999488032,
129.573954034227));
#266319=CARTESIAN_POINT('Ctrl Pts',(-47.2638999271647,2.69108597692664,
124.339355039948));
#266320=CARTESIAN_POINT('Ctrl Pts',(-47.5423475509777,-3.98459458696386,
125.045780338419));
#266321=CARTESIAN_POINT('Ctrl Pts',(-47.8207951747905,-6.998627383702,131.044059591139));
#266322=CARTESIAN_POINT('Ctrl Pts',(-48.0992427986034,-3.58126351677304,
136.822067197091));
#266323=CARTESIAN_POINT('Ctrl Pts',(-48.3776904224163,3.1271065676212,137.070096437769));
#266324=CARTESIAN_POINT('Ctrl Pts',(-48.6561380462292,6.9618184840203,131.560220557891));
#266325=CARTESIAN_POINT('Ctrl Pts',(-48.9345856700421,4.39895931734504,
125.355746318666));
#266326=CARTESIAN_POINT('Ctrl Pts',(-49.213033293855,-2.20632856086043,
124.158282440523));
#266327=CARTESIAN_POINT('Ctrl Pts',(-49.4914809176678,-6.78410827677761,
129.068239728113));
#266328=CARTESIAN_POINT('Ctrl Pts',(-49.7699285414808,-5.12762390845042,
135.573607298891));
#266329=CARTESIAN_POINT('Ctrl Pts',(-50.0483761652936,1.2408963333889,137.696270160183));
#266330=CARTESIAN_POINT('Ctrl Pts',(-50.3268237891066,6.46909346599971,
133.485604840309));
#266331=CARTESIAN_POINT('Ctrl Pts',(-50.6052714129194,5.7525097361419,126.811007065796));
#266332=CARTESIAN_POINT('Ctrl Pts',(-50.8837190367324,-0.250349415506305,
123.806106119193));
#266333=CARTESIAN_POINT('Ctrl Pts',(-51.1621666605453,-6.02314968455324,
127.232259172855));
#266334=CARTESIAN_POINT('Ctrl Pts',(-51.4406142843581,-6.26096964071598,
133.94099894735));
#266335=CARTESIAN_POINT('Ctrl Pts',(-51.719061908171,-0.745264362431691,
137.767321330073));
#266336=CARTESIAN_POINT('Ctrl Pts',(-51.997509531984,5.45530245673899,135.195022977544));
#266337=CARTESIAN_POINT('Ctrl Pts',(-52.2759571557968,6.64271282450778,
128.587920411975));
#266338=CARTESIAN_POINT('Ctrl Pts',(-52.5544047796097,1.72579462111621,
124.01761811622));
#266339=CARTESIAN_POINT('Ctrl Pts',(-52.8328524034226,-4.77704452932697,
125.684000628399));
#266340=CARTESIAN_POINT('Ctrl Pts',(-53.1113000272355,-6.89001312891767,
132.05574382713));
#266341=CARTESIAN_POINT('Ctrl Pts',(-53.3897476510484,-2.67139625888694,
137.277526989739));
#266342=CARTESIAN_POINT('Ctrl Pts',(-53.6681952748612,4.00210326809833,
136.550786488079));
#266343=CARTESIAN_POINT('Ctrl Pts',(-53.9466428986742,6.99786540531528,
130.543361339928));
#266344=CARTESIAN_POINT('Ctrl Pts',(-54.225090522487,3.56293109977782,124.775781777402));
#266345=CARTESIAN_POINT('Ctrl Pts',(-54.5035381462999,-3.14616282759469,
124.548171656537));
#266346=CARTESIAN_POINT('Ctrl Pts',(-54.7819857701128,-6.9640868150063,
130.069693559035));
#266347=CARTESIAN_POINT('Ctrl Pts',(-55.0604333939257,-4.382355233982,136.266338597842));
#266348=CARTESIAN_POINT('Ctrl Pts',(-55.3388810177386,2.22654671711671,
137.443692705233));
#266349=CARTESIAN_POINT('Ctrl Pts',(-55.6173286415515,6.78936100803939,
132.519824973462));
#266350=CARTESIAN_POINT('Ctrl Pts',(-55.8957762653644,5.11308421129812,
126.019529303714));
#266351=CARTESIAN_POINT('Ctrl Pts',(-56.1742238891773,-1.26186718757599,
123.916259859391));
#266352=CARTESIAN_POINT('Ctrl Pts',(-56.4526715129901,-6.47722428670686,
128.142818509401));
#266353=CARTESIAN_POINT('Ctrl Pts',(-56.7311191368031,-5.74032869635189,
134.815204333253));
#266354=CARTESIAN_POINT('Ctrl Pts',(-57.0095667606159,0.271648535303317,
137.801820722997));
#266355=CARTESIAN_POINT('Ctrl Pts',(-57.2880143844289,6.03399403378365,
134.358113120779));
#266356=CARTESIAN_POINT('Ctrl Pts',(-57.5664620082417,6.25139379221294,
127.64868057857));
#266357=CARTESIAN_POINT('Ctrl Pts',(-57.8449096320546,0.724068053163303,
123.839163828657));
#266358=CARTESIAN_POINT('Ctrl Pts',(-58.1233572558676,-5.46864085405239,
126.430322658971));
#266359=CARTESIAN_POINT('Ctrl Pts',(-58.4018048796803,-6.63593597435208,
133.0410086896));
#266360=CARTESIAN_POINT('Ctrl Pts',(-58.6802525034934,-1.705130117717,137.596324408362));
#266361=CARTESIAN_POINT('Ctrl Pts',(-58.9587001273061,4.79260701686295,
135.910157209259));
#266362=CARTESIAN_POINT('Ctrl Pts',(-59.2371477511191,6.88617243481463,
129.532012374421));
#266363=CARTESIAN_POINT('Ctrl Pts',(-59.515595374932,2.65168179339722,124.323093417365));
#266364=CARTESIAN_POINT('Ctrl Pts',(-59.7940429987449,-4.01957487429483,
125.070142389788));
#266365=CARTESIAN_POINT('Ctrl Pts',(-60.0724906225578,-6.99703859965941,
131.086657781405));
#266366=CARTESIAN_POINT('Ctrl Pts',(-60.3509382463707,-3.5445656762756,
136.843755870437));
#266367=CARTESIAN_POINT('Ctrl Pts',(-60.6293858701835,3.16518994194552,
137.050944762941));
#266368=CARTESIAN_POINT('Ctrl Pts',(-60.9078334939965,6.96629063164357,
131.517827988445));
#266369=CARTESIAN_POINT('Ctrl Pts',(-61.1862811178092,4.36571055307847,
125.32906955493));
#266370=CARTESIAN_POINT('Ctrl Pts',(-61.4647287416223,-2.24674424694855,
124.171836125139));
#266371=CARTESIAN_POINT('Ctrl Pts',(-61.743176365435,-6.79455084358828,
129.109568687053));
#266372=CARTESIAN_POINT('Ctrl Pts',(-62.0216239892481,-5.09849714723216,
135.60473223792));
#266373=CARTESIAN_POINT('Ctrl Pts',(-62.3000716130609,1.2828263519976,137.688588780872));
#266374=CARTESIAN_POINT('Ctrl Pts',(-62.5785192368738,6.48529510329292,
133.446175954988));
#266375=CARTESIAN_POINT('Ctrl Pts',(-62.8569668606868,5.72809447894126,
126.776063893867));
#266376=CARTESIAN_POINT('Ctrl Pts',(-63.1354144844995,-0.292945138585431,
123.80775972859));
#266377=CARTESIAN_POINT('Ctrl Pts',(-63.4138621083125,-6.04478248491762,
127.268989977326));
#266378=CARTESIAN_POINT('Ctrl Pts',(-63.6923097321254,-6.24176003165182,
133.979053131985));
#266379=CARTESIAN_POINT('Ctrl Pts',(-63.9707573559382,-0.702865036227365,
137.771728958244));
#266380=CARTESIAN_POINT('Ctrl Pts',(-64.2492049797512,5.48192859062395,
135.161733654286));
#266381=CARTESIAN_POINT('Ctrl Pts',(-64.527652603564,6.62909764979204,128.547525399088));
#266382=CARTESIAN_POINT('Ctrl Pts',(-64.806100227377,1.68444981822529,124.007238457143));
#266383=CARTESIAN_POINT('Ctrl Pts',(-65.0845478511898,-4.80812510634223,
125.713174722747));
#266384=CARTESIAN_POINT('Ctrl Pts',(-65.3629954750027,-6.88226794815085,
132.097662107432));
#266385=CARTESIAN_POINT('Ctrl Pts',(-65.6414430988157,-2.63194276308962,
137.29366860422));
#266386=CARTESIAN_POINT('Ctrl Pts',(-65.9198907226284,4.03700924369883,
136.526318081592));
#266387=CARTESIAN_POINT('Ctrl Pts',(-66.1983383464414,6.99614697439381,
130.500768182686));
#266388=CARTESIAN_POINT('Ctrl Pts',(-66.4767859702543,3.5261674164012,124.75420490012));
#266389=CARTESIAN_POINT('Ctrl Pts',(-66.7552335940671,-3.18418773440913,
124.567439155348));
#266390=CARTESIAN_POINT('Ctrl Pts',(-67.0336812178801,-6.96842991351606,
130.112099543802));
#266391=CARTESIAN_POINT('Ctrl Pts',(-67.3121288416929,-4.34902542882876,
136.292914040211));
#266392=CARTESIAN_POINT('Ctrl Pts',(-67.5905764655059,2.26692096324861,
137.43001607195));
#266393=CARTESIAN_POINT('Ctrl Pts',(-67.8690240893187,6.79967773534632,
132.478464422373));
#266394=CARTESIAN_POINT('Ctrl Pts',(-68.1474717131316,5.08386285138514,
125.988493160695));
#266395=CARTESIAN_POINT('Ctrl Pts',(-68.4259193369445,-1.30377363249137,
123.924068823677));
#266396=CARTESIAN_POINT('Ctrl Pts',(-68.7043669607574,-6.49330584099122,
128.182296524302));
#266397=CARTESIAN_POINT('Ctrl Pts',(-68.9828145845703,-5.71580719724563,
134.850073031684));
#266398=CARTESIAN_POINT('Ctrl Pts',(-69.2612622083832,0.314239028063776,
137.800037474531));
#266399=CARTESIAN_POINT('Ctrl Pts',(-69.5397098321961,6.05551493801243,
134.32131664364));
#266400=CARTESIAN_POINT('Ctrl Pts',(-69.818157456009,6.23206844827842,127.610685037641));
#266401=CARTESIAN_POINT('Ctrl Pts',(-70.0966050798218,0.681655508046095,
123.834885269867));
#266402=CARTESIAN_POINT('Ctrl Pts',(-70.3750527036349,-5.49516554335789,
126.463692868828));
#266403=CARTESIAN_POINT('Ctrl Pts',(-70.6535003274475,-6.62219791417695,
133.081362075471));
#266404=CARTESIAN_POINT('Ctrl Pts',(-70.9319479512606,-1.66375391422059,
137.606578180005));
#266405=CARTESIAN_POINT('Ctrl Pts',(-71.2103955750734,4.82359865400735,
135.880888651457));
#266406=CARTESIAN_POINT('Ctrl Pts',(-71.4888431988863,6.87829970509706,
129.490117861946));
#266407=CARTESIAN_POINT('Ctrl Pts',(-71.7672908226993,2.6121793508235,124.307071960521));
#266408=CARTESIAN_POINT('Ctrl Pts',(-72.045738446512,-4.05440621480077,
125.094716924722));
#266409=CARTESIAN_POINT('Ctrl Pts',(-72.3241860703251,-6.99519053777849,
131.129245511046));
#266410=CARTESIAN_POINT('Ctrl Pts',(-72.6026336941378,-3.5077364905931,
136.865220751771));
#266411=CARTESIAN_POINT('Ctrl Pts',(-72.8810813179508,3.20315602899298,
137.031561618638));
#266412=CARTESIAN_POINT('Ctrl Pts',(-73.1595289417638,6.97050464080582,
131.475408981201));
#266413=CARTESIAN_POINT('Ctrl Pts',(-73.4379765655765,4.33230001580124,
125.302595680118));
#266414=CARTESIAN_POINT('Ctrl Pts',(-73.7164241893894,-2.28707667910305,
124.18563558039));
#266415=CARTESIAN_POINT('Ctrl Pts',(-73.9948718132024,-6.80474163581863,
129.150960447132));
#266416=CARTESIAN_POINT('Ctrl Pts',(-74.2733194370152,-5.0691814593271,
135.635679297414));
#266417=CARTESIAN_POINT('Ctrl Pts',(-74.5517670608282,1.32470883500465,
137.680652303954));
#266418=CARTESIAN_POINT('Ctrl Pts',(-74.830214684641,6.5012564255912,133.406649176227));
#266419=CARTESIAN_POINT('Ctrl Pts',(-75.108662308454,5.70346696509291,126.741269991954));
#266420=CARTESIAN_POINT('Ctrl Pts',(-75.3871099322667,-0.335530006474783,
123.809672599606));
#266421=CARTESIAN_POINT('Ctrl Pts',(-75.6655575560798,-6.06619129364391,
127.305851786256));
#266422=CARTESIAN_POINT('Ctrl Pts',(-75.9440051798925,-6.22231913187452,
134.016989677222));
#266423=CARTESIAN_POINT('Ctrl Pts',(-76.2224528037055,-0.66043966510086,
137.775878408018));
#266424=CARTESIAN_POINT('Ctrl Pts',(-76.5009004275184,5.50835158962877,
135.128282866967));
#266425=CARTESIAN_POINT('Ctrl Pts',(-76.7793480513312,6.61523683142527,
128.507214014061));
#266426=CARTESIAN_POINT('Ctrl Pts',(-77.0577956751442,1.64304259742666,
123.997110667925));
#266427=CARTESIAN_POINT('Ctrl Pts',(-77.336243298957,-4.83902751651344,
125.742537472861));
#266428=CARTESIAN_POINT('Ctrl Pts',(-77.6146909227699,-6.87426774241415,
132.139532463972));
#266429=CARTESIAN_POINT('Ctrl Pts',(-77.8931385465828,-2.59239173968542,
137.309569755007));
#266430=CARTESIAN_POINT('Ctrl Pts',(-78.1715861703958,4.07176562643718,
136.501637645866));
#266431=CARTESIAN_POINT('Ctrl Pts',(-78.4500337942086,6.99416929867323,
130.458186275174));
#266432=CARTESIAN_POINT('Ctrl Pts',(-78.7284814180215,3.48927306959449,
124.732852213582));
#266433=CARTESIAN_POINT('Ctrl Pts',(-79.0069290418344,-3.22209464997582,
124.586937765577));
#266434=CARTESIAN_POINT('Ctrl Pts',(-79.2853766656473,-6.97251479429268,
130.154531180556));
#266435=CARTESIAN_POINT('Ctrl Pts',(-79.5638242894601,-4.3155344689392,
136.319286102215));
#266436=CARTESIAN_POINT('Ctrl Pts',(-79.8422719132732,2.30721120779087,
137.416093922569));
#266437=CARTESIAN_POINT('Ctrl Pts',(-80.1207195370859,6.80974249809405,
132.437041836753));
#266438=CARTESIAN_POINT('Ctrl Pts',(-80.3991671608989,5.0544531070646,125.957635471416));
#266439=CARTESIAN_POINT('Ctrl Pts',(-80.6776147847117,-1.34563176559565,
123.932132739704));
#266440=CARTESIAN_POINT('Ctrl Pts',(-80.9560624085247,-6.50914678343976,
128.221871700751));
#266441=CARTESIAN_POINT('Ctrl Pts',(-81.2345100323374,-5.69107389680138,
134.884791814753));
#266442=CARTESIAN_POINT('Ctrl Pts',(-81.5129576561506,0.356817876581242,
137.797994998686));
#266443=CARTESIAN_POINT('Ctrl Pts',(-81.7914052799631,6.07681145290804,
134.284389844403));
#266444=CARTESIAN_POINT('Ctrl Pts',(-82.0698529037763,6.21251217275584,
127.572807839535));
#266445=CARTESIAN_POINT('Ctrl Pts',(-82.348300527589,0.639217703933302,
123.830864967548));
#266446=CARTESIAN_POINT('Ctrl Pts',(-82.626748151402,-5.52148660728364,
126.497223923725));
#266447=CARTESIAN_POINT('Ctrl Pts',(-82.9051957752149,-6.60821446602265,
133.121631086217));
#266448=CARTESIAN_POINT('Ctrl Pts',(-83.1836433990278,-1.62231605971109,
137.616579892973));
#266449=CARTESIAN_POINT('Ctrl Pts',(-83.4620910228406,4.85441155092967,
135.851431981043));
#266450=CARTESIAN_POINT('Ctrl Pts',(-83.7405386466535,6.87017209745416,
129.448272049221));
#266451=CARTESIAN_POINT('Ctrl Pts',(-84.0189862704665,2.57258011298421,
124.291291263097));
#266452=CARTESIAN_POINT('Ctrl Pts',(-84.2974338942792,-4.08908731779306,
125.119503032603));
#266453=CARTESIAN_POINT('Ctrl Pts',(-84.5758815180923,-6.99308326653956,
131.171821201958));
#266454=CARTESIAN_POINT('Ctrl Pts',(-84.8543291419051,-3.47077732444568,
136.886461045702));
#266455=CARTESIAN_POINT('Ctrl Pts',(-85.132776765718,3.2410034219148,137.011947723114));
#266456=CARTESIAN_POINT('Ctrl Pts',(-85.4112243895309,6.97446035535538,
131.432965108015));
#266457=CARTESIAN_POINT('Ctrl Pts',(-85.6896720133437,4.29872894355427,
125.27632567523));
#266458=CARTESIAN_POINT('Ctrl Pts',(-85.9681196371569,-2.327324362789,124.19968029493));
#266459=CARTESIAN_POINT('Ctrl Pts',(-86.2465672609694,-6.81468027584547,
129.192413474561));
#266460=CARTESIAN_POINT('Ctrl Pts',(-86.5250148847825,-5.03967793103904,
135.666447330617));
#266461=CARTESIAN_POINT('Ctrl Pts',(-86.8034625085954,1.36654223043768,
137.672461023519));
#266462=CARTESIAN_POINT('Ctrl Pts',(-87.0819101324082,6.51697684144191,
133.367025968708));
#266463=CARTESIAN_POINT('Ctrl Pts',(-87.3603577562212,5.67862810717874,
126.706626649358));
#266464=CARTESIAN_POINT('Ctrl Pts',(-87.638805380034,-0.378102441176264,
123.811844661359));
#266465=CARTESIAN_POINT('Ctrl Pts',(-87.917253003847,-6.08737531742114,
127.342843233717));
#266466=CARTESIAN_POINT('Ctrl Pts',(-88.1957006276599,-6.20264766177327,
134.054807177307));
#266467=CARTESIAN_POINT('Ctrl Pts',(-88.4741482514726,-0.617989821139493,
137.779769525637));
#266468=CARTESIAN_POINT('Ctrl Pts',(-88.7525958752857,5.53457047463998,
135.094671855119));
#266469=CARTESIAN_POINT('Ctrl Pts',(-89.0310434990984,6.6011308830247,128.466987750645));
#266470=CARTESIAN_POINT('Ctrl Pts',(-89.3094911229114,1.60157449308101,
123.987235123859));
#266471=CARTESIAN_POINT('Ctrl Pts',(-89.5879387467241,-4.86975061474005,
125.772087790693));
#266472=CARTESIAN_POINT('Ctrl Pts',(-89.8663863705374,-6.8660128081587,
132.181353345229));
#266473=CARTESIAN_POINT('Ctrl Pts',(-90.1448339943499,-2.55274465425183,
137.325229852876));
#266474=CARTESIAN_POINT('Ctrl Pts',(-90.4232816181632,4.10637112840284,
136.476746095445));
#266475=CARTESIAN_POINT('Ctrl Pts',(-90.7017292419757,6.99193245143733,
130.415617195278));
#266476=CARTESIAN_POINT('Ctrl Pts',(-90.9801768657889,3.45224942649073,
124.711724509022));
#266477=CARTESIAN_POINT('Ctrl Pts',(-91.2586244896016,-3.2598821696406,
124.606666764696));
#266478=CARTESIAN_POINT('Ctrl Pts',(-91.5370721134145,-6.97634130596949,
130.196986896981));
#266479=CARTESIAN_POINT('Ctrl Pts',(-91.8155197372274,-4.28188359533257,
136.345453806627));
#266480=CARTESIAN_POINT('Ctrl Pts',(-92.0939673610402,2.34741595777304,
137.401926772977));
#266481=CARTESIAN_POINT('Ctrl Pts',(-92.3724149848533,6.81955492332935,
132.395558751529));
#266482=CARTESIAN_POINT('Ctrl Pts',(-92.650862608666,5.02485606812542,125.926957379319));
#266483=CARTESIAN_POINT('Ctrl Pts',(-92.929310232479,-1.38744003581995,
123.940451308663));
#266484=CARTESIAN_POINT('Ctrl Pts',(-93.2077578562919,-6.52474652706058,
128.261542572277));
#266485=CARTESIAN_POINT('Ctrl Pts',(-93.4862054801047,-5.66612971152105,
134.919359395943));
#266486=CARTESIAN_POINT('Ctrl Pts',(-93.7646531039176,0.39938350308132,
137.795693371147));
#266487=CARTESIAN_POINT('Ctrl Pts',(-94.0431007277306,6.09788278932073,
134.247334091402));
#266488=CARTESIAN_POINT('Ctrl Pts',(-94.3215483515434,6.19272569030992,
127.535050387806));
#266489=CARTESIAN_POINT('Ctrl Pts',(-94.5999959753563,0.596756213373149,
123.827103070676));
#266490=CARTESIAN_POINT('Ctrl Pts',(-94.8784435991693,-5.54760307049237,
126.530914581157));
#266491=CARTESIAN_POINT('Ctrl Pts',(-95.1568912229821,-6.59398614805128,
133.161814229653));
#266492=CARTESIAN_POINT('Ctrl Pts',(-95.4353388467949,-1.58081808968337,
137.626329176652));
#266493=CARTESIAN_POINT('Ctrl Pts',(-95.7137864706081,4.88504456584684,
135.821788289543));
#266494=CARTESIAN_POINT('Ctrl Pts',(-95.9922340944205,6.86178991305786,
129.406476486855));
#266495=CARTESIAN_POINT('Ctrl Pts',(-96.2706817182339,2.53288554724217,
124.275751909854));
#266496=CARTESIAN_POINT('Ctrl Pts',(-96.5491293420464,-4.12361689815126,
125.144499794972));
#266497=CARTESIAN_POINT('Ctrl Pts',(-96.8275769658595,-6.99071686402826,
131.214383276482));
#266498=CARTESIAN_POINT('Ctrl Pts',(-97.1060245896722,-3.4336895473684,
136.907475965166));
#266499=CARTESIAN_POINT('Ctrl Pts',(-97.3844722134854,3.27873071826322,
136.992103803166));
#266500=CARTESIAN_POINT('Ctrl Pts',(-97.6629198372979,6.9781576287114,131.390497941658));
#266501=CARTESIAN_POINT('Ctrl Pts',(-97.9413674611112,4.26499858032525,
125.250260513709));
#266502=CARTESIAN_POINT('Ctrl Pts',(-98.2198150849237,-2.36748580661544,
124.21396974833));
#266503=CARTESIAN_POINT('Ctrl Pts',(-98.498262708737,-6.82436639538843,
129.233926233285));
#266504=CARTESIAN_POINT('Ctrl Pts',(-98.7767103325495,-5.00998765563179,
135.69703519741));
#266505=CARTESIAN_POINT('Ctrl Pts',(-99.0551579563628,1.40832498814648,
137.664015243098));
#266506=CARTESIAN_POINT('Ctrl Pts',(-99.3336055801754,6.53245576831905,
133.327307800681));
#266507=CARTESIAN_POINT('Ctrl Pts',(-99.6120532039884,5.65357882561176,
126.672135149802));
#266508=CARTESIAN_POINT('Ctrl Pts',(-99.8905008278013,-0.420660865152761,
123.814275833361));
#266509=CARTESIAN_POINT('Ctrl Pts',(-100.168948451614,-6.10833377126732,
127.379962948978));
#266510=CARTESIAN_POINT('Ctrl Pts',(-100.447396075427,-6.18274635028192,
134.092504230901));
#266511=CARTESIAN_POINT('Ctrl Pts',(-100.72584369924,-0.575517077338011,
137.783402166914));
#266512=CARTESIAN_POINT('Ctrl Pts',(-101.004291323053,5.56058427410689,
135.060901864211));
#266513=CARTESIAN_POINT('Ctrl Pts',(-101.282738946866,6.58678032729173,
128.426848099441));
#266514=CARTESIAN_POINT('Ctrl Pts',(-101.561186570679,1.56004704180311,
123.977612190885));
#266515=CARTESIAN_POINT('Ctrl Pts',(-101.839634194492,-4.90029326256724,
125.801824581246));
#266516=CARTESIAN_POINT('Ctrl Pts',(-102.118081818304,-6.85750345127332,
132.223123201514));
#266517=CARTESIAN_POINT('Ctrl Pts',(-102.396529442117,-2.51300297592632,
137.340648317539));
#266518=CARTESIAN_POINT('Ctrl Pts',(-102.67497706593,4.14082446727623,136.451644352694));
#266519=CARTESIAN_POINT('Ctrl Pts',(-102.953424689743,6.98943651557314,
130.373062520413));
#266520=CARTESIAN_POINT('Ctrl Pts',(-103.231872313556,3.41509785901489,
124.690822569333));
#266521=CARTESIAN_POINT('Ctrl Pts',(-103.510319937369,-3.29754889317273,
124.626625421641));
#266522=CARTESIAN_POINT('Ctrl Pts',(-103.788767561182,-6.97990930675369,
130.239465119861));
#266523=CARTESIAN_POINT('Ctrl Pts',(-104.067215184995,-4.24807405495459,
136.371416183792));
#266524=CARTESIAN_POINT('Ctrl Pts',(-104.345662808808,2.38753372339306,
137.387515148146));
#266525=CARTESIAN_POINT('Ctrl Pts',(-104.62411043262,6.82911464744894,132.354016703874));
#266526=CARTESIAN_POINT('Ctrl Pts',(-104.902558056433,4.99507283129728,
125.896460021193));
#266527=CARTESIAN_POINT('Ctrl Pts',(-105.181005680246,-1.42919689394351,
123.949024222305));
#266528=CARTESIAN_POINT('Ctrl Pts',(-105.459453304059,-6.54010449379936,
128.301307668861));
#266529=CARTESIAN_POINT('Ctrl Pts',(-105.737900927872,-5.64097556572054,
134.953774494342));
#266530=CARTESIAN_POINT('Ctrl Pts',(-106.016348551685,0.441934330278796,
137.793132677202));
#266531=CARTESIAN_POINT('Ctrl Pts',(-106.294796175498,6.11872816644418,
134.210150757753));
#266532=CARTESIAN_POINT('Ctrl Pts',(-106.573243799311,6.17270973413615,
127.49741408157));
#266533=CARTESIAN_POINT('Ctrl Pts',(-106.851691423124,0.554272609792058,
123.823599718647));
#266534=CARTESIAN_POINT('Ctrl Pts',(-107.130139046936,-5.57351396522919,
126.564763592701));
#266535=CARTESIAN_POINT('Ctrl Pts',(-107.40858667075,-6.57951348749827,
133.201910016778));
#266536=CARTESIAN_POINT('Ctrl Pts',(-107.687034294562,-1.53926154185996,
137.635825669776));
#266537=CARTESIAN_POINT('Ctrl Pts',(-107.965481918375,4.91549656364115,
135.791958675416));
#266538=CARTESIAN_POINT('Ctrl Pts',(-108.243929542188,6.85315346251289,
129.364732723601));
#266539=CARTESIAN_POINT('Ctrl Pts',(-108.522377166001,2.49309712449469,
124.260454476607));
#266540=CARTESIAN_POINT('Ctrl Pts',(-108.800824789814,-4.15799367636883,
125.169706285567));
#266541=CARTESIAN_POINT('Ctrl Pts',(-109.079272413627,-6.98809141793296,
131.256930157466));
#266542=CARTESIAN_POINT('Ctrl Pts',(-109.35772003744,-3.39647453366164,
136.928264731447));
#266543=CARTESIAN_POINT('Ctrl Pts',(-109.636167661252,3.31633652003941,
136.97203059412));
#266544=CARTESIAN_POINT('Ctrl Pts',(-109.914615285065,6.98159632387027,
131.348009055767));
#266545=CARTESIAN_POINT('Ctrl Pts',(-110.193062908878,4.23111017600536,
125.22440116141));
#266546=CARTESIAN_POINT('Ctrl Pts',(-110.471510532691,-2.40755952238467,
124.228503411086));
#266547=CARTESIAN_POINT('Ctrl Pts',(-110.749958156504,-6.83379963552497,
129.275497185033));
#266548=CARTESIAN_POINT('Ctrl Pts',(-111.028405780317,-4.98011173328953,
135.727441764346));
#266549=CARTESIAN_POINT('Ctrl Pts',(-111.30685340413,1.45005555985492,137.655315275653));
#266550=CARTESIAN_POINT('Ctrl Pts',(-111.585301027943,6.54769263264538,
133.287496143919));
#266551=CARTESIAN_POINT('Ctrl Pts',(-111.863748651756,5.62832004860235,
126.63779677138));
#266552=CARTESIAN_POINT('Ctrl Pts',(-112.142196275568,-0.463203701385527,
123.816966025527));
#266553=CARTESIAN_POINT('Ctrl Pts',(-112.420643899382,-6.12906587855929,
127.417209556553));
#266554=CARTESIAN_POINT('Ctrl Pts',(-112.699091523194,-6.16261593485082,
134.130079441122));
#266555=CARTESIAN_POINT('Ctrl Pts',(-112.977539147007,-0.533023007539609,
137.786776197239));
#266556=CARTESIAN_POINT('Ctrl Pts',(-113.25598677082,5.58639202407863,135.026974145601));
#266557=CARTESIAN_POINT('Ctrl Pts',(-113.534434394633,6.57218569599142,
128.386796547837));
#266558=CARTESIAN_POINT('Ctrl Pts',(-113.812882018446,1.5184617824084,123.968242225583));
#266559=CARTESIAN_POINT('Ctrl Pts',(-114.091329642259,-4.93065432822552,
125.831746742611));
#266560=CARTESIAN_POINT('Ctrl Pts',(-114.369777266072,-6.84873998707567,
132.26484048503));
#266561=CARTESIAN_POINT('Ctrl Pts',(-114.648224889884,-2.4731681773514,
137.355824577657));
#266562=CARTESIAN_POINT('Ctrl Pts',(-114.926672513697,4.17512436637621,
136.426333347767));
#266563=CARTESIAN_POINT('Ctrl Pts',(-115.20512013751,6.98668158356849,130.330523827459));
#266564=CARTESIAN_POINT('Ctrl Pts',(-115.483567761323,3.377819743832,124.670147169045));
#266565=CARTESIAN_POINT('Ctrl Pts',(-115.762015385136,-3.33509342481799,
124.646812996834));
#266566=CARTESIAN_POINT('Ctrl Pts',(-116.040463008949,-6.98321866443162,
130.281964275151));
#266567=CARTESIAN_POINT('Ctrl Pts',(-116.318910632762,-4.21410710063033,
136.397172271667));
#266568=CARTESIAN_POINT('Ctrl Pts',(-116.597358256575,2.42756301807353,
137.372859582102));
#266569=CARTESIAN_POINT('Ctrl Pts',(-116.875805880388,6.83842131621399,
132.312417233142));
#266570=CARTESIAN_POINT('Ctrl Pts',(-117.154253504201,4.96510450020791,
125.866144527128));
#266571=CARTESIAN_POINT('Ctrl Pts',(-117.432701128013,-1.47090079265054,
123.957851162959));
#266572=CARTESIAN_POINT('Ctrl Pts',(-117.711148751826,-6.55522011456102,
128.341165516992));
#266573=CARTESIAN_POINT('Ctrl Pts',(-117.989596375639,-5.61561239149597,
134.988035834682));
#266574=CARTESIAN_POINT('Ctrl Pts',(-118.268043999452,0.484468781437156,
137.790313011739));
#266575=CARTESIAN_POINT('Ctrl Pts',(-118.546491623265,6.13934681184524,
134.172841221298));
#266576=CARTESIAN_POINT('Ctrl Pts',(-118.824939247078,6.15246504593319,
127.459900315453));
#266577=CARTESIAN_POINT('Ctrl Pts',(-119.103386870891,0.511768467435545,
123.820355041281));
#266578=CARTESIAN_POINT('Ctrl Pts',(-119.381834494704,-5.59921833135585,
126.598769704074));
#266579=CARTESIAN_POINT('Ctrl Pts',(-119.660282118516,-6.56479702065358,
133.241916961827));
#266580=CARTESIAN_POINT('Ctrl Pts',(-119.93872974233,-1.49764795613459,
137.645069020452));
#266581=CARTESIAN_POINT('Ctrl Pts',(-120.217177366142,4.94576641590264,
135.761944244007));
#266582=CARTESIAN_POINT('Ctrl Pts',(-120.495624989955,6.84426306584611,
129.323042306287));
#266583=CARTESIAN_POINT('Ctrl Pts',(-120.774072613768,2.45321631911644,
124.245399530209));
#266584=CARTESIAN_POINT('Ctrl Pts',(-121.052520237581,-4.19221637860163,
125.195121570349));
#266585=CARTESIAN_POINT('Ctrl Pts',(-121.330967861394,-6.98520702554029,
131.299460268319));
#266586=CARTESIAN_POINT('Ctrl Pts',(-121.609415485207,-3.35913366234199,
136.948826574209));
#266587=CARTESIAN_POINT('Ctrl Pts',(-121.88786310902,3.3538194337463,136.951728839794));
#266588=CARTESIAN_POINT('Ctrl Pts',(-122.166310732833,6.98477631340985,
131.305500024783));
#266589=CARTESIAN_POINT('Ctrl Pts',(-122.444758356646,4.19706498634193,
125.198748576561));
#266590=CARTESIAN_POINT('Ctrl Pts',(-122.723205980458,-2.44754402515043,
124.24328074465));
#266591=CARTESIAN_POINT('Ctrl Pts',(-123.001653604271,-6.84297964670285,
129.317124789377));
#266592=CARTESIAN_POINT('Ctrl Pts',(-123.280101228084,-4.95005127107555,
135.7576659047));
#266593=CARTESIAN_POINT('Ctrl Pts',(-123.558548851897,1.49173239922134,
137.646361443563));
#266594=CARTESIAN_POINT('Ctrl Pts',(-123.83699647571,6.5626868698133,133.247592473656));
#266595=CARTESIAN_POINT('Ctrl Pts',(-124.115444099523,5.60285271212367,
126.603612786514));
#266596=CARTESIAN_POINT('Ctrl Pts',(-124.393891723336,-0.505729373435472,
123.819915138168));
#266597=CARTESIAN_POINT('Ctrl Pts',(-124.672339347149,-6.14957087106115,
127.454581676257));
#266598=CARTESIAN_POINT('Ctrl Pts',(-124.950786970961,-6.14225716141998,
134.167531415611));
#266599=CARTESIAN_POINT('Ctrl Pts',(-125.229234594775,-0.490509186377616,
137.789891491587));
#266600=CARTESIAN_POINT('Ctrl Pts',(-125.507682218587,5.6119927682395,134.992889956494));
#266601=CARTESIAN_POINT('Ctrl Pts',(-125.786129842401,6.55734752993325,
128.346834579959));
#266602=CARTESIAN_POINT('Ctrl Pts',(-126.064577466213,1.47682025585389,
123.959125575163));
#266603=CARTESIAN_POINT('Ctrl Pts',(-126.343025090026,-4.9608326866744,
125.861853166013));
#266604=CARTESIAN_POINT('Ctrl Pts',(-126.621472713839,-6.8397227402992,
132.306503649927));
#266605=CARTESIAN_POINT('Ctrl Pts',(-126.899920337652,-2.43324173462049,
137.370758070868));
#266606=CARTESIAN_POINT('Ctrl Pts',(-127.178367961465,4.20926955470684,
136.400814018573));
#266607=CARTESIAN_POINT('Ctrl Pts',(-127.456815585278,6.98366775750873,
130.288002692701));
#266608=CARTESIAN_POINT('Ctrl Pts',(-127.73526320909,3.34041646229627,124.649699074291));
#266609=CARTESIAN_POINT('Ctrl Pts',(-128.013710832904,-3.37251437334987,
124.66722874222));
#266610=CARTESIAN_POINT('Ctrl Pts',(-128.292158456716,-6.9862692563739,
130.324482788031));
#266611=CARTESIAN_POINT('Ctrl Pts',(-128.570606080529,-4.17998399101771,
136.422721115849));
#266612=CARTESIAN_POINT('Ctrl Pts',(-128.849053704342,2.46750235851359,
137.357960617914));
#266613=CARTESIAN_POINT('Ctrl Pts',(-129.127501328155,6.84747458476236,
132.270761880817));
#266614=CARTESIAN_POINT('Ctrl Pts',(-129.405948951968,4.93495218534535,
125.836012020477));
#266615=CARTESIAN_POINT('Ctrl Pts',(-129.684396575781,-1.51255018658779,
123.966931803538));
#266616=CARTESIAN_POINT('Ctrl Pts',(-129.962844199593,-6.57009282923063,
128.381114639724));
#266617=CARTESIAN_POINT('Ctrl Pts',(-130.241291823406,-5.59004112868908,
135.022142147398));
#266618=CARTESIAN_POINT('Ctrl Pts',(-130.519739447219,0.52698528042665,
137.78723447924));
#266619=CARTESIAN_POINT('Ctrl Pts',(-130.798187071032,6.15973796149245,
134.135406864555));
#266620=CARTESIAN_POINT('Ctrl Pts',(-131.076634694845,6.13199237587537,
127.422510479544));
#266621=CARTESIAN_POINT('Ctrl Pts',(-131.355082318658,0.4692453613103,123.81736915881));
#266622=CARTESIAN_POINT('Ctrl Pts',(-131.633529942471,-5.62471521638866,
126.632931655165));
#266623=CARTESIAN_POINT('Ctrl Pts',(-131.911977566284,-6.54983729284086,
133.281833582332));
#266624=CARTESIAN_POINT('Ctrl Pts',(-132.190425190097,-1.45597887451291,
137.654058886162));
#266625=CARTESIAN_POINT('Ctrl Pts',(-132.46887281391,4.97585300097076,135.731746107516));
#266626=CARTESIAN_POINT('Ctrl Pts',(-132.747320437723,6.83511905249447,
129.281406779768));
#266627=CARTESIAN_POINT('Ctrl Pts',(-133.025768061535,2.4132446089053,124.230587628526));
#266628=CARTESIAN_POINT('Ctrl Pts',(-133.304215685348,-4.22628373671482,
125.220744707546));
#266629=CARTESIAN_POINT('Ctrl Pts',(-133.582663309161,-6.98206379373247,
131.341972033073));
#266630=CARTESIAN_POINT('Ctrl Pts',(-133.861110932974,-3.32166831708915,
136.969160731525));
#266631=CARTESIAN_POINT('Ctrl Pts',(-134.139558556787,3.39117807044069,
136.931199292478));
#266632=CARTESIAN_POINT('Ctrl Pts',(-134.4180061806,6.98769747949419,131.262972423894));
#266633=CARTESIAN_POINT('Ctrl Pts',(-134.696453804413,4.16286427289247,
125.173303709728));
#266634=CARTESIAN_POINT('Ctrl Pts',(-134.974901428226,-2.48743783327188,
124.25830120144));
#266635=CARTESIAN_POINT('Ctrl Pts',(-135.253349052039,-6.85190608875344,
129.358807503792));
#266636=CARTESIAN_POINT('Ctrl Pts',(-135.531796675851,-4.91980738289134,
135.787706498505));
#266637=CARTESIAN_POINT('Ctrl Pts',(-135.810244299665,1.53335396189511,
137.637154078616));
#266638=CARTESIAN_POINT('Ctrl Pts',(-136.088691923477,6.57743792420584,
133.207598268539));
#266639=CARTESIAN_POINT('Ctrl Pts',(-136.36713954729,5.57717775987727,126.569584461903));
#266640=CARTESIAN_POINT('Ctrl Pts',(-136.645587171103,-0.548236305497475,
123.823123062006));
#266641=CARTESIAN_POINT('Ctrl Pts',(-136.924034794916,-6.1698479889529,
127.492077923251));
#266642=CARTESIAN_POINT('Ctrl Pts',(-137.202482418729,-6.12167078439119,
134.204858766568));
#266643=CARTESIAN_POINT('Ctrl Pts',(-137.480930042542,-0.447977189217358,
137.792747934521));
#266644=CARTESIAN_POINT('Ctrl Pts',(-137.759377666354,5.63738555794455,
134.958650559891));
#266645=CARTESIAN_POINT('Ctrl Pts',(-138.037825290167,6.54226637895086,
128.306963676612));
#266646=CARTESIAN_POINT('Ctrl Pts',(-138.31627291398,1.43512400518173,123.950262577445));
#266647=CARTESIAN_POINT('Ctrl Pts',(-138.594720537793,-4.99082721964375,
125.892142735845));
#266648=CARTESIAN_POINT('Ctrl Pts',(-138.873168161606,-6.83045204508126,
132.348111152362));
#266649=CARTESIAN_POINT('Ctrl Pts',(-139.151615785419,-2.39322512722196,
137.385448243807));
#266650=CARTESIAN_POINT('Ctrl Pts',(-139.430063409232,4.24325876700673,
136.375087310741));
#266651=CARTESIAN_POINT('Ctrl Pts',(-139.708511033045,6.98039514907165,
130.245500691775));
#266652=CARTESIAN_POINT('Ctrl Pts',(-139.986958656858,3.30288940040013,
124.629479042785));
#266653=CARTESIAN_POINT('Ctrl Pts',(-140.26540628067,-3.40981035212143,
124.687871901284));
#266654=CARTESIAN_POINT('Ctrl Pts',(-140.543853904484,-6.98906096953965,
130.36701908296));
#266655=CARTESIAN_POINT('Ctrl Pts',(-140.822301528296,-4.1457059905611,
136.448061769617));
#266656=CARTESIAN_POINT('Ctrl Pts',(-141.100749152109,2.50735026474636,
137.342818807668));
#266657=CARTESIAN_POINT('Ctrl Pts',(-141.379196775922,6.85627411762182,
132.229052190456));
#266658=CARTESIAN_POINT('Ctrl Pts',(-141.657644399735,4.90461700401472,
125.80606361781));
#266659=CARTESIAN_POINT('Ctrl Pts',(-141.936092023548,-1.5541435324211,
123.976265807557));
#266660=CARTESIAN_POINT('Ctrl Pts',(-142.214539647361,-6.58472208669408,
128.421153556726));
#266661=CARTESIAN_POINT('Ctrl Pts',(-142.492987271174,-5.56426272485295,
135.056092168669));
#266662=CARTESIAN_POINT('Ctrl Pts',(-142.771434894987,0.569482251782813,
137.783897193782));
#266663=CARTESIAN_POINT('Ctrl Pts',(-143.0498825188,6.17990085978423,134.097849074668));
#266664=CARTESIAN_POINT('Ctrl Pts',(-143.328330142612,6.11129248258502,
127.385245959334));
#266665=CARTESIAN_POINT('Ctrl Pts',(-143.606777766425,0.426704867125613,
123.814642181877));
#266666=CARTESIAN_POINT('Ctrl Pts',(-143.885225390238,-5.65000367553061,
126.667248180088));
#266667=CARTESIAN_POINT('Ctrl Pts',(-144.163673014051,-6.53463485839856,
133.321658399163));
#266668=CARTESIAN_POINT('Ctrl Pts',(-144.442120637864,-1.4142558410586,
137.662794933783));
#266669=CARTESIAN_POINT('Ctrl Pts',(-144.720568261677,5.00575520397605,
135.701365384942));
#266670=CARTESIAN_POINT('Ctrl Pts',(-144.99901588549,6.82572176129271,129.239827686864));
#266671=CARTESIAN_POINT('Ctrl Pts',(-145.277463509303,2.37318347502772,
124.216019320419));
#266672=CARTESIAN_POINT('Ctrl Pts',(-145.555911133116,-4.26019448832994,
125.246574747685));
#266673=CARTESIAN_POINT('Ctrl Pts',(-145.834358756928,-6.97866183898313,
131.384463876438));
#266674=CARTESIAN_POINT('Ctrl Pts',(-146.112806380741,-3.28407988619528,
136.989266449907));
#266675=CARTESIAN_POINT('Ctrl Pts',(-146.391254004554,3.42841104578457,
136.910442712901));
#266676=CARTESIAN_POINT('Ctrl Pts',(-146.669701628367,6.99035971387901,
131.220427828976));
#266677=CARTESIAN_POINT('Ctrl Pts',(-146.94814925218,4.12850930297597,125.148067503779));
#266678=CARTESIAN_POINT('Ctrl Pts',(-147.226596875993,-2.52723946847004,
124.27356422487));
#266679=CARTESIAN_POINT('Ctrl Pts',(-147.505044499806,-6.86057863090408,
129.400543783708));
#266680=CARTESIAN_POINT('Ctrl Pts',(-147.783492123619,-4.88938118943532,
135.817562432597));
#266681=CARTESIAN_POINT('Ctrl Pts',(-148.061939747432,1.57491870557395,
137.627693521995));
#266682=CARTESIAN_POINT('Ctrl Pts',(-148.340387371245,6.5919452492172,133.167515010566));
#266683=CARTESIAN_POINT('Ctrl Pts',(-148.618834995057,5.55129614325799,
126.535713058481));
#266684=CARTESIAN_POINT('Ctrl Pts',(-148.89728261887,-0.590722922461593,
123.826589678167));
#266685=CARTESIAN_POINT('Ctrl Pts',(-149.175730242683,-6.18989648085842,
127.529696908099));
#266686=CARTESIAN_POINT('Ctrl Pts',(-149.454177866496,-6.10085756660025,
134.242060110815));
#266687=CARTESIAN_POINT('Ctrl Pts',(-149.732625490309,-0.405428592098244,
137.795345420191));
#266688=CARTESIAN_POINT('Ctrl Pts',(-150.011073114122,5.66256945225453,
134.924257224548));
#266689=CARTESIAN_POINT('Ctrl Pts',(-150.289520737935,6.52694280188189,
128.267185315226));
#266690=CARTESIAN_POINT('Ctrl Pts',(-150.567968361748,1.39337457546175,
123.94165356085));
#266691=CARTESIAN_POINT('Ctrl Pts',(-150.84641598556,-5.02063681567507,
125.922614329717));
#266692=CARTESIAN_POINT('Ctrl Pts',(-151.124863609373,-6.8209282449509,
132.389661450552));
#266693=CARTESIAN_POINT('Ctrl Pts',(-151.403311233186,-2.35311983798619,
137.399894552124));
#266694=CARTESIAN_POINT('Ctrl Pts',(-151.681758856999,4.2770907437925,136.349154177582));
#266695=CARTESIAN_POINT('Ctrl Pts',(-151.960206480812,6.97686387952531,
130.20301939961));
#266696=CARTESIAN_POINT('Ctrl Pts',(-152.238654104625,3.26523994872261,
124.609487823786));
#266697=CARTESIAN_POINT('Ctrl Pts',(-152.517101728438,-3.44697997911642,
124.708741709087));
#266698=CARTESIAN_POINT('Ctrl Pts',(-152.795549352251,-6.99159370048095,
130.40957158374));
#266699=CARTESIAN_POINT('Ctrl Pts',(-153.073996976064,-4.11127436944443,
136.473193293963));
#266700=CARTESIAN_POINT('Ctrl Pts',(-153.352444599876,2.54710526019297,
137.327434712448));
#266701=CARTESIAN_POINT('Ctrl Pts',(-153.63089222369,6.86481958872245,132.187289707623));
#266702=CARTESIAN_POINT('Ctrl Pts',(-153.909339847502,4.87410008029735,
125.776300428876));
#266703=CARTESIAN_POINT('Ctrl Pts',(-154.187787471315,-1.5956792888948,
123.98585282914));
#266704=CARTESIAN_POINT('Ctrl Pts',(-154.466235095128,-6.5991073448593,
128.461280784342));
#266705=CARTESIAN_POINT('Ctrl Pts',(-154.744682718941,-5.53827813521478,
135.089884640464));
#266706=CARTESIAN_POINT('Ctrl Pts',(-155.023130342754,0.611958120764675,
137.78030127903));
#266707=CARTESIAN_POINT('Ctrl Pts',(-155.301577966567,6.19983475957701,
134.060169243357));
#266708=CARTESIAN_POINT('Ctrl Pts',(-155.58002559038,6.0903661331043,127.348108135675));
#266709=CARTESIAN_POINT('Ctrl Pts',(-155.858473214192,0.38414856123516,
123.812174211531));
#266710=CARTESIAN_POINT('Ctrl Pts',(-156.136920838005,-5.67508277170857,
126.701718007236));
#266711=CARTESIAN_POINT('Ctrl Pts',(-156.415368461818,-6.51919028065846,
133.3613899366));
#266712=CARTESIAN_POINT('Ctrl Pts',(-156.693816085631,-1.37248040183399,
137.671276839599));
#266713=CARTESIAN_POINT('Ctrl Pts',(-156.972263709444,5.03547191688086,
135.670803202055));
#266714=CARTESIAN_POINT('Ctrl Pts',(-157.250711333257,6.81607154046107,
129.198306568304));
#266715=CARTESIAN_POINT('Ctrl Pts',(-157.52915895707,2.33303440196427,124.201695145721));
#266716=CARTESIAN_POINT('Ctrl Pts',(-157.807606580883,-4.29394737687161,
125.272610733624));
#266717=CARTESIAN_POINT('Ctrl Pts',(-158.086054204696,-6.97500128735293,
131.426934223863));
#266718=CARTESIAN_POINT('Ctrl Pts',(-158.364501828508,-3.2463697625135,
137.009142984327));
#266719=CARTESIAN_POINT('Ctrl Pts',(-158.642949452322,3.46551698009634,
136.889459870208));
#266720=CARTESIAN_POINT('Ctrl Pts',(-158.921397076134,6.99276291791392,
131.177867816534));
#266721=CARTESIAN_POINT('Ctrl Pts',(-159.199844699947,4.09400134962899,
125.123040893851));
#266722=CARTESIAN_POINT('Ctrl Pts',(-159.47829232376,-2.56694745588028,
124.289069249361));
#266723=CARTESIAN_POINT('Ctrl Pts',(-159.756739947573,-6.86899695179061,
129.442332082575));
#266724=CARTESIAN_POINT('Ctrl Pts',(-160.035187571386,-4.85877381816122,
135.84723260065));
#266725=CARTESIAN_POINT('Ctrl Pts',(-160.313635195198,1.61642509006095,
137.617980124263));
#266726=CARTESIAN_POINT('Ctrl Pts',(-160.592082819012,6.60620830727321,
133.12734418504));
#266727=CARTESIAN_POINT('Ctrl Pts',(-160.870530442824,5.52520882131862,
126.501999831362));
#266728=CARTESIAN_POINT('Ctrl Pts',(-161.148978066638,-0.633187649970563,
123.830314858198));
#266729=CARTESIAN_POINT('Ctrl Pts',(-161.42742569045,-6.20971560387352,
127.567437236815));
#266730=CARTESIAN_POINT('Ctrl Pts',(-161.705873314263,-6.07981827928859,
134.279134069845));
#266731=CARTESIAN_POINT('Ctrl Pts',(-161.984320938076,-0.362864971672915,
137.79768385235));
#266732=CARTESIAN_POINT('Ctrl Pts',(-162.262768561889,5.68754351797111,
134.889711224922));
#266733=CARTESIAN_POINT('Ctrl Pts',(-162.541216185702,6.5113773665471,128.227500969805));
#266734=CARTESIAN_POINT('Ctrl Pts',(-162.819663809515,1.35157351373451,
123.93329884439));
#266735=CARTESIAN_POINT('Ctrl Pts',(-163.098111433328,-5.05026037016286,
125.953266818493));
#266736=CARTESIAN_POINT('Ctrl Pts',(-163.376559057141,-6.81115169281603,
132.431153004838));
#266737=CARTESIAN_POINT('Ctrl Pts',(-163.655006680953,-2.31292735302948,
137.414096460505));
#266738=CARTESIAN_POINT('Ctrl Pts',(-163.933454304766,4.31076423140788,
136.323015580059));
#266739=CARTESIAN_POINT('Ctrl Pts',(-164.211901928579,6.97307407972212,
130.160560390364));
#266740=CARTESIAN_POINT('Ctrl Pts',(-164.490349552392,3.2274695023783,124.589726158078));
#266741=CARTESIAN_POINT('Ctrl Pts',(-164.768797176205,-3.4840218770001,
124.729837392289));
#266742=CARTESIAN_POINT('Ctrl Pts',(-165.047244800018,-6.99386735534677,
130.452138713572));
#266743=CARTESIAN_POINT('Ctrl Pts',(-165.325692423831,-4.07669040354407,
136.498114757629));
#266744=CARTESIAN_POINT('Ctrl Pts',(-165.604140047644,2.58676587171747,
137.31180890232));
#266745=CARTESIAN_POINT('Ctrl Pts',(-165.882587671457,6.87311068140868,
132.145475979844));
#266746=CARTESIAN_POINT('Ctrl Pts',(-166.161035295269,4.84340254500906,
125.746723556562));
#266747=CARTESIAN_POINT('Ctrl Pts',(-166.439482919082,-1.63715591688565,
123.995692513036));
#266748=CARTESIAN_POINT('Ctrl Pts',(-166.717930542895,-6.61324807067504,
128.501494835643));
#266749=CARTESIAN_POINT('Ctrl Pts',(-166.996378166708,-5.5120883226436,
135.12351831059));
#266750=CARTESIAN_POINT('Ctrl Pts',(-167.274825790521,0.654411313413328,
137.776446868231));
#266751=CARTESIAN_POINT('Ctrl Pts',(-167.553273414334,6.21953892221278,
134.022368766858));
#266752=CARTESIAN_POINT('Ctrl Pts',(-167.831721038147,6.06921410286677,
127.311098384725));
#266753=CARTESIAN_POINT('Ctrl Pts',(-168.11016866196,0.3415780205785,123.809965339223));
#266754=CARTESIAN_POINT('Ctrl Pts',(-168.388616285773,-5.69995157560742,
126.736339859314));
#266755=CARTESIAN_POINT('Ctrl Pts',(-168.667063909585,-6.50350413192509,
133.401026722375));
#266756=CARTESIAN_POINT('Ctrl Pts',(-168.945511533399,-1.33065410484337,
137.679504289309));
#266757=CARTESIAN_POINT('Ctrl Pts',(-169.223959157211,5.06500203852252,
135.640060691349));
#266758=CARTESIAN_POINT('Ctrl Pts',(-169.502406781024,6.80616874759175,
129.156844962666));
#266759=CARTESIAN_POINT('Ctrl Pts',(-169.780854404837,2.29279887745254,
124.18761563522));
#266760=CARTESIAN_POINT('Ctrl Pts',(-170.05930202865,-4.32754115161411,
125.298851700587));
#266761=CARTESIAN_POINT('Ctrl Pts',(-170.337749652463,-6.97108227448498,
131.469381501595));
#266762=CARTESIAN_POINT('Ctrl Pts',(-170.616197276276,-3.20853934340632,
137.028789598255));
#266763=CARTESIAN_POINT('Ctrl Pts',(-170.894644900089,3.50249449840198,
136.868251541923));
#266764=CARTESIAN_POINT('Ctrl Pts',(-171.173092523901,6.99490700254731,
131.135293963646));
#266765=CARTESIAN_POINT('Ctrl Pts',(-171.451540147715,4.05934169155642,
125.098224807315));
#266766=CARTESIAN_POINT('Ctrl Pts',(-171.729987771527,-2.60656032410858,
124.304815700371));
#266767=CARTESIAN_POINT('Ctrl Pts',(-172.00843539534,-6.87716073946864,
129.484170851909));
#266768=CARTESIAN_POINT('Ctrl Pts',(-172.286883019153,-4.82798640323697,
135.876715903229));
#266769=CARTESIAN_POINT('Ctrl Pts',(-172.565330642966,1.65787157732142,
137.608014245356));
#266770=CARTESIAN_POINT('Ctrl Pts',(-172.843778266779,6.62022656985093,
133.087087280501));
#266771=CARTESIAN_POINT('Ctrl Pts',(-173.122225890592,5.49891676073447,
126.468446029806));
#266772=CARTESIAN_POINT('Ctrl Pts',(-173.400673514405,-0.675628914478315,
123.834298464058));
#266773=CARTESIAN_POINT('Ctrl Pts',(-173.679121138218,-6.22930462359329,
127.605297510917));
#266774=CARTESIAN_POINT('Ctrl Pts',(-173.95756876203,-6.05855370207473,
134.316079269865));
#266775=CARTESIAN_POINT('Ctrl Pts',(-174.236016385844,-0.320287905152608,
137.799763144343));
#266776=CARTESIAN_POINT('Ctrl Pts',(-174.514464009656,5.71230682967103,
134.855013841124));
#266777=CARTESIAN_POINT('Ctrl Pts',(-174.792911633469,6.49557064972945,
128.187912110866));
#266778=CARTESIAN_POINT('Ctrl Pts',(-175.071359257282,1.30972236895365,
123.925198737649));
#266779=CARTESIAN_POINT('Ctrl Pts',(-175.349806881095,-5.07969678539539,
125.984099066334));
#266780=CARTESIAN_POINT('Ctrl Pts',(-175.628254504908,-6.80112275095037,
132.472584277733));
#266781=CARTESIAN_POINT('Ctrl Pts',(-175.906702128721,-2.27264916169912,
137.428053442694));
#266782=CARTESIAN_POINT('Ctrl Pts',(-176.185149752534,4.34427798206938,
136.296672486746));
#266783=CARTESIAN_POINT('Ctrl Pts',(-176.463597376347,6.96902589009458,
130.118125237372));
#266784=CARTESIAN_POINT('Ctrl Pts',(-176.742045000159,3.18957946096438,
124.570194777934));
#266785=CARTESIAN_POINT('Ctrl Pts',(-177.020492623972,-3.52093467317244,
124.751158169184));
#266786=CARTESIAN_POINT('Ctrl Pts',(-177.298940247785,-6.99588184988549,
130.494718895118));
#266787=CARTESIAN_POINT('Ctrl Pts',(-177.577387871598,-4.04195537438161,
136.522825237142));
#266788=CARTESIAN_POINT('Ctrl Pts',(-177.855835495411,2.62633062968132,
137.295941956302));
#266789=CARTESIAN_POINT('Ctrl Pts',(-178.134283119224,6.88114708845103,
132.103612556543));
#266790=CARTESIAN_POINT('Ctrl Pts',(-178.412730743037,4.81252553565828,
125.717334096849));
#266791=CARTESIAN_POINT('Ctrl Pts',(-178.69117836685,-1.67857187946192,
124.005784494632));
#266792=CARTESIAN_POINT('Ctrl Pts',(-178.969625990663,-6.62714374015151,
128.541794220484));
#266793=CARTESIAN_POINT('Ctrl Pts',(-179.248073614475,-5.48569425761253,
135.15699193274));
#266794=CARTESIAN_POINT('Ctrl Pts',(-179.526521238288,0.696840256609583,
137.772334104211));
#266795=CARTESIAN_POINT('Ctrl Pts',(-179.804968862101,6.23901261754625,
133.984449045885));
#266796=CARTESIAN_POINT('Ctrl Pts',(-180.083416485914,6.0478371756692,127.27421807789));
#266797=CARTESIAN_POINT('Ctrl Pts',(-180.361864109727,0.298994822622653,
123.808015646805));
#266798=CARTESIAN_POINT('Ctrl Pts',(-180.64031173354,-5.72460916570447,
126.771112453397));
#266799=CARTESIAN_POINT('Ctrl Pts',(-180.918759357353,-6.48757699345442,
133.440567287733));
#266800=CARTESIAN_POINT('Ctrl Pts',(-181.197206981166,-1.28877849997557,
137.687476978041));
#266801=CARTESIAN_POINT('Ctrl Pts',(-181.475654604978,5.094344474651,135.609138992));
#266802=CARTESIAN_POINT('Ctrl Pts',(-181.754102228792,6.79601374963652,
129.115444406326));
#266803=CARTESIAN_POINT('Ctrl Pts',(-182.032549852604,2.25247839243521,
124.173781310638));
#266804=CARTESIAN_POINT('Ctrl Pts',(-182.310997476417,-4.36097456772779,
125.32529667621));
#266805=CARTESIAN_POINT('Ctrl Pts',(-182.58944510023,-6.96690494559973,
131.511804136733));
#266806=CARTESIAN_POINT('Ctrl Pts',(-182.867892724043,-3.17059003069381,
137.048205563678));
#266807=CARTESIAN_POINT('Ctrl Pts',(-183.146340347856,3.53934223048593,
136.84681851393));
#266808=CARTESIAN_POINT('Ctrl Pts',(-183.424787971669,6.99679188832936,
131.092707847901));
#266809=CARTESIAN_POINT('Ctrl Pts',(-183.703235595482,4.02453161308464,
125.07362016374));
#266810=CARTESIAN_POINT('Ctrl Pts',(-183.981683219295,-2.64607660528548,
124.320802994409));
#266811=CARTESIAN_POINT('Ctrl Pts',(-184.260130843107,-6.88506969142675,
129.52605854136));
#266812=CARTESIAN_POINT('Ctrl Pts',(-184.53857846692,-4.79702008550057,
135.906011247817));
#266813=CARTESIAN_POINT('Ctrl Pts',(-184.817026090733,1.6992566315413,137.597796254561));
#266814=CARTESIAN_POINT('Ctrl Pts',(-185.095473714546,6.63399951749853,
133.046745788687));
#266815=CARTESIAN_POINT('Ctrl Pts',(-185.373921338359,5.47242093576752,
126.435052897159));
#266816=CARTESIAN_POINT('Ctrl Pts',(-185.652368962172,-0.718045143308166,
123.838540348135));
#266817=CARTESIAN_POINT('Ctrl Pts',(-185.930816585985,-6.24866281413942,
127.64327632748));
#266818=CARTESIAN_POINT('Ctrl Pts',(-186.209264209798,-6.03706462292539,
134.35289434186));
#266819=CARTESIAN_POINT('Ctrl Pts',(-186.487711833611,-0.277698970246197,
137.801583219124));
#266820=CARTESIAN_POINT('Ctrl Pts',(-186.766159457423,5.73685846974069,
134.820166358884));
#266821=CARTESIAN_POINT('Ctrl Pts',(-187.044607081237,6.47952323715255,
128.148420205389));
#266822=CARTESIAN_POINT('Ctrl Pts',(-187.323054705049,1.2678226919294,123.917353540782));
#266823=CARTESIAN_POINT('Ctrl Pts',(-187.601502328862,-5.10894497059535,
126.01510993074));
#266824=CARTESIAN_POINT('Ctrl Pts',(-187.879949952675,-6.79084179098006,
132.513953733987));
#266825=CARTESIAN_POINT('Ctrl Pts',(-188.158397576488,-2.23228675651833,
137.44176498151));
#266826=CARTESIAN_POINT('Ctrl Pts',(-188.436845200301,4.37763075391265,
136.270125873797));
#266827=CARTESIAN_POINT('Ctrl Pts',(-188.715292824114,6.96471946064982,
130.075715513085));
#266828=CARTESIAN_POINT('Ctrl Pts',(-188.993740447926,3.15157122851057,
124.550894407098));
#266829=CARTESIAN_POINT('Ctrl Pts',(-189.27218807174,-3.55771699981564,
124.772703249722));
#266830=CARTESIAN_POINT('Ctrl Pts',(-189.550635695553,-6.99763710944952,
130.53731055055));
#266831=CARTESIAN_POINT('Ctrl Pts',(-189.829083319365,-4.00707056907658,
136.547323816845));
#266832=CARTESIAN_POINT('Ctrl Pts',(-190.107530943179,2.66579806799723,
137.279834462351));
#266833=CARTESIAN_POINT('Ctrl Pts',(-190.385978566991,6.88892851205765,
132.061700988983));
#266834=CARTESIAN_POINT('Ctrl Pts',(-190.664426190804,4.78147019640398,
125.688133138775));
#266835=CARTESIAN_POINT('Ctrl Pts',(-190.942873814617,-1.71992564193992,
124.016128399968));
#266836=CARTESIAN_POINT('Ctrl Pts',(-191.22132143843,-6.64079383837953,
128.582177445553));
#266837=CARTESIAN_POINT('Ctrl Pts',(-191.499769062243,-5.45909691816341,
135.190304266535));
#266838=CARTESIAN_POINT('Ctrl Pts',(-191.778216686055,0.739243378134395,
137.767963139373));
#266839=CARTESIAN_POINT('Ctrl Pts',(-192.056664309869,6.25825512397307,
133.946411485565));
#266840=CARTESIAN_POINT('Ctrl Pts',(-192.335111933681,6.0262361436405,127.237468581785));
#266841=CARTESIAN_POINT('Ctrl Pts',(-192.613559557494,0.256400545303713,
123.806325206523));
#266842=CARTESIAN_POINT('Ctrl Pts',(-192.892007181307,-5.74905462830365,
126.806034500975));
#266843=CARTESIAN_POINT('Ctrl Pts',(-193.17045480512,-6.47140945543246,
133.480010167483));
#266844=CARTESIAN_POINT('Ctrl Pts',(-193.448902428933,-1.24685513894648,
137.695194610365));
#266845=CARTESIAN_POINT('Ctrl Pts',(-193.727350052746,5.12349813797151,
135.578039249819));
#266846=CARTESIAN_POINT('Ctrl Pts',(-194.005797676559,6.78560692289256,
129.074106433399));
#266847=CARTESIAN_POINT('Ctrl Pts',(-194.284245300372,2.2120744410027,124.160192684611));
#266848=CARTESIAN_POINT('Ctrl Pts',(-194.562692924184,-4.39424638632456,
125.35194468056));
#266849=CARTESIAN_POINT('Ctrl Pts',(-194.841140547997,-6.9624694554897,
131.554200557291));
#266850=CARTESIAN_POINT('Ctrl Pts',(-195.11958817181,-3.13252323060231,
137.067390161131));
#266851=CARTESIAN_POINT('Ctrl Pts',(-195.398035795623,3.57605881094196,
136.825161580438));
#266852=CARTESIAN_POINT('Ctrl Pts',(-195.676483419436,6.99841750541489,
131.050111047343));
#266853=CARTESIAN_POINT('Ctrl Pts',(-195.954931043249,3.98957240411393,
125.04922787486));
#266854=CARTESIAN_POINT('Ctrl Pts',(-196.233378667062,-2.68549483512068,
124.337030539057));
#266855=CARTESIAN_POINT('Ctrl Pts',(-196.511826290875,-6.89272351459547,
129.567993598765));
#266856=CARTESIAN_POINT('Ctrl Pts',(-196.790273914688,-4.76587601242081,
135.935117548864));
#266857=CARTESIAN_POINT('Ctrl Pts',(-197.0687215385,1.74057871918182,137.58732653051));
#266858=CARTESIAN_POINT('Ctrl Pts',(-197.347169162313,6.64752663985393,
133.006321204467));
#266859=CARTESIAN_POINT('Ctrl Pts',(-197.625616786126,5.44572232823074,
126.401821670817));
#266860=CARTESIAN_POINT('Ctrl Pts',(-197.904064409939,-0.760434764710735,
123.843040353244));
#266861=CARTESIAN_POINT('Ctrl Pts',(-198.182512033752,-6.26778945818702,
127.681372279183));
#266862=CARTESIAN_POINT('Ctrl Pts',(-198.460959657565,-6.01535183812634,
134.389577921633));
#266863=CARTESIAN_POINT('Ctrl Pts',(-198.739407281378,-0.235099745102313,
137.803144009248));
#266864=CARTESIAN_POINT('Ctrl Pts',(-199.017854905191,5.76119752841001,
134.785170069484));
#266865=CARTESIAN_POINT('Ctrl Pts',(-199.296302529004,6.46323572345932,
128.10902671676));
#266866=CARTESIAN_POINT('Ctrl Pts',(-199.574750152817,1.22587603526843,
123.909763544495));
#266867=CARTESIAN_POINT('Ctrl Pts',(-199.853197776629,-5.13800384196074,
126.04629826259));
#266868=CARTESIAN_POINT('Ctrl Pts',(-200.131645400443,-6.78030919386985,
132.555259840639));
#266869=CARTESIAN_POINT('Ctrl Pts',(-200.410093024255,-2.19184163313082,
137.455230568865));
#266870=CARTESIAN_POINT('Ctrl Pts',(-200.688540648069,4.41082131103843,
136.243376724908));
#266871=CARTESIAN_POINT('Ctrl Pts',(-200.96698827188,6.96015495096418,130.03333278901));
#266872=CARTESIAN_POINT('Ctrl Pts',(-201.245435895694,3.11344621342587,
124.531825760752));
#266873=CARTESIAN_POINT('Ctrl Pts',(-201.523883519507,-3.59436749394705,
124.794471835542));
#266874=CARTESIAN_POINT('Ctrl Pts',(-201.80233114332,-6.99913306899709,
130.579912101622));
#266875=CARTESIAN_POINT('Ctrl Pts',(-202.080778767133,-3.97203728029775,
136.571609588935));
#266876=CARTESIAN_POINT('Ctrl Pts',(-202.359226390945,2.705166724186,137.263487017335));
#266877=CARTESIAN_POINT('Ctrl Pts',(-202.637674014758,6.89645466388467,
132.019742830214));
#266878=CARTESIAN_POINT('Ctrl Pts',(-202.916121638571,4.75023767801316,
125.659121764391));
#266879=CARTESIAN_POINT('Ctrl Pts',(-203.194569262384,-1.76121567194074,
124.026723845744));
#266880=CARTESIAN_POINT('Ctrl Pts',(-203.473016886197,-6.65419785954973,
128.622643014438));
#266881=CARTESIAN_POINT('Ctrl Pts',(-203.75146451001,-5.43229728987039,
135.223454077576));
#266882=CARTESIAN_POINT('Ctrl Pts',(-204.029912133822,0.781619106723946,
137.763334135682));
#266883=CARTESIAN_POINT('Ctrl Pts',(-204.308359757636,6.27726572845484,
133.908257495395));
#266884=CARTESIAN_POINT('Ctrl Pts',(-204.586807381448,6.00441180721532,
127.200851258176));
#266885=CARTESIAN_POINT('Ctrl Pts',(-204.865255005262,0.213796766968775,
123.804894081017));
#266886=CARTESIAN_POINT('Ctrl Pts',(-205.143702629074,-5.77328705756903,
126.841104707996));
#266887=CARTESIAN_POINT('Ctrl Pts',(-205.422150252887,-6.4550021169537,
133.519353900054));
#266888=CARTESIAN_POINT('Ctrl Pts',(-205.7005978767,-1.20488557524167,137.702656900301));
#266889=CARTESIAN_POINT('Ctrl Pts',(-205.979045500513,5.15246194818434,
135.546762617222));
#266890=CARTESIAN_POINT('Ctrl Pts',(-206.257493124326,6.77494865298866,
129.032832575676));
#266891=CARTESIAN_POINT('Ctrl Pts',(-206.535940748139,2.17158852033829,
124.14685026067));
#266892=CARTESIAN_POINT('Ctrl Pts',(-206.814388371952,-4.42735537450605,
125.378794726189));
#266893=CARTESIAN_POINT('Ctrl Pts',(-207.092835995765,-6.9577759685135,
131.596569192254));
#266894=CARTESIAN_POINT('Ctrl Pts',(-207.371283619578,-3.09434035370993,
137.086342679721));
#266895=CARTESIAN_POINT('Ctrl Pts',(-207.64973124339,3.61264287922363,136.803281543952));
#266896=CARTESIAN_POINT('Ctrl Pts',(-207.928178867203,6.99978379356611,
131.007505140413));
#266897=CARTESIAN_POINT('Ctrl Pts',(-208.206626491016,3.95446536007061,
125.025048844539));
#266898=CARTESIAN_POINT('Ctrl Pts',(-208.485074114829,-2.72481355295718,
124.353497733001));
#266899=CARTESIAN_POINT('Ctrl Pts',(-208.763521738642,-6.90012192535954,
129.609974470206));
#266900=CARTESIAN_POINT('Ctrl Pts',(-209.041969362455,-4.73455533805275,
135.964033727826));
#266901=CARTESIAN_POINT('Ctrl Pts',(-209.320416986268,1.78183630903778,
137.576605461163));
#266902=CARTESIAN_POINT('Ctrl Pts',(-209.598864610081,6.66080743566547,
132.965815025787));
#266903=CARTESIAN_POINT('Ctrl Pts',(-209.877312233893,5.41882192745001,
126.368753582173));
#266904=CARTESIAN_POINT('Ctrl Pts',(-210.155759857706,-0.802796207923886,
123.847798312635));
#266905=CARTESIAN_POINT('Ctrl Pts',(-210.434207481519,-6.28668384699127,
127.719583954367));
#266906=CARTESIAN_POINT('Ctrl Pts',(-210.712655105332,-5.99341615225276,
134.42612864986));
#266907=CARTESIAN_POINT('Ctrl Pts',(-210.991102729145,-0.19249180825093,
137.804445456879));
#266908=CARTESIAN_POINT('Ctrl Pts',(-211.269550352958,5.78532310378624,
134.750026269725));
#266909=CARTESIAN_POINT('Ctrl Pts',(-211.547997976771,6.44670871218949,
128.069733104719));
#266910=CARTESIAN_POINT('Ctrl Pts',(-211.826445600584,1.18388395332015,
123.902429030038));
#266911=CARTESIAN_POINT('Ctrl Pts',(-212.104893224396,-5.16687232270428,
126.077662906191));
#266912=CARTESIAN_POINT('Ctrl Pts',(-212.38334084821,-6.76952534990887,
132.596501067076));
#266913=CARTESIAN_POINT('Ctrl Pts',(-212.661788472022,-2.15131529024619,
137.468449705789));
#266914=CARTESIAN_POINT('Ctrl Pts',(-212.940236095835,4.44384842355829,
136.216426031276));
#266915=CARTESIAN_POINT('Ctrl Pts',(-213.218683719648,6.95533253017721,
129.990978635656));
#266916=CARTESIAN_POINT('Ctrl Pts',(-213.497131343461,3.0752058284468,124.512989545492));
#266917=CARTESIAN_POINT('Ctrl Pts',(-213.775578967274,-3.63088479746918,
124.81646312));
#266918=CARTESIAN_POINT('Ctrl Pts',(-214.054026591087,-7.00036967309483,
130.622521969716));
#266919=CARTESIAN_POINT('Ctrl Pts',(-214.3324742149,-3.93685680621679,136.595681653493));
#266920=CARTESIAN_POINT('Ctrl Pts',(-214.610921838713,2.74443513942699,
137.246900227015));
#266921=CARTESIAN_POINT('Ctrl Pts',(-214.889369462525,6.90372526504794,
131.977739635008));
#266922=CARTESIAN_POINT('Ctrl Pts',(-215.167817086339,4.71882913781829,
125.630301048724));
#266923=CARTESIAN_POINT('Ctrl Pts',(-215.446264710151,-1.80244043944716,
124.037570439344));
#266924=CARTESIAN_POINT('Ctrl Pts',(-215.724712333964,-6.66735530697114,
128.66318942767));
#266925=CARTESIAN_POINT('Ctrl Pts',(-216.003159957777,-5.40529636580357,
135.256440137483));
#266926=CARTESIAN_POINT('Ctrl Pts',(-216.28160758159,0.823965872130078,
137.758447264668));
#266927=CARTESIAN_POINT('Ctrl Pts',(-216.560055205403,6.29604372654653,
133.869988489185));
#266928=CARTESIAN_POINT('Ctrl Pts',(-216.838502829216,5.98236497510254,
127.164367463932));
#266929=CARTESIAN_POINT('Ctrl Pts',(-217.116950453029,0.171185066315507,
123.803722323317));
#266930=CARTESIAN_POINT('Ctrl Pts',(-217.395398076842,-5.79730555555969,
126.876321774922));
#266931=CARTESIAN_POINT('Ctrl Pts',(-217.673845700654,-6.43835558599724,
133.558597027552));
#266932=CARTESIAN_POINT('Ctrl Pts',(-217.952293324468,-1.16287136405879,
137.709863571333));
#266933=CARTESIAN_POINT('Ctrl Pts',(-218.23074094828,5.18123483202488,135.515310253174));
#266934=CARTESIAN_POINT('Ctrl Pts',(-218.509188572093,6.76403933487094,
128.991624362576));
#266935=CARTESIAN_POINT('Ctrl Pts',(-218.787636195906,2.13102213066266,
124.133754533223));
#266936=CARTESIAN_POINT('Ctrl Pts',(-219.066083819719,-4.46030030540597,
125.405845818157));
#266937=CARTESIAN_POINT('Ctrl Pts',(-219.344531443532,-6.95282465859006,
131.638908471637));
#266938=CARTESIAN_POINT('Ctrl Pts',(-219.622979067345,-3.0560428148978,
137.105062417155));
#266939=CARTESIAN_POINT('Ctrl Pts',(-219.901426691158,3.6490930796943,136.781179215245));
#266940=CARTESIAN_POINT('Ctrl Pts',(-220.179874314971,7.00089070215466,
130.964891705888));
#266941=CARTESIAN_POINT('Ctrl Pts',(-220.458321938783,3.91921178185968,
125.001083968743));
#266942=CARTESIAN_POINT('Ctrl Pts',(-220.736769562596,-2.76403130182543,
124.370203966041));
#266943=CARTESIAN_POINT('Ctrl Pts',(-221.015217186409,-6.90726464956813,
129.651999600063));
#266944=CARTESIAN_POINT('Ctrl Pts',(-221.293664810222,-4.7030592229955,
135.992758713204));
#266945=CARTESIAN_POINT('Ctrl Pts',(-221.572112434035,1.82302787229404,
137.565633443793));
#266946=CARTESIAN_POINT('Ctrl Pts',(-221.850560057848,6.67384141280798,
132.925228753618));
#266947=CARTESIAN_POINT('Ctrl Pts',(-222.129007681661,5.39172073022998,
126.33584985658));
#266948=CARTESIAN_POINT('Ctrl Pts',(-222.407455305474,-0.845127903228338,
123.85281405));
#266949=CARTESIAN_POINT('Ctrl Pts',(-222.685902929286,-6.30534528041361,
127.757909937084));
#266950=CARTESIAN_POINT('Ctrl Pts',(-222.964350553099,-5.9712583781396,
134.462545172141));
#266951=CARTESIAN_POINT('Ctrl Pts',(-223.242798176912,-0.14987673854478,
137.805487513793));
#266952=CARTESIAN_POINT('Ctrl Pts',(-223.521245800725,5.80923430188729,
134.714736261875));
#266953=CARTESIAN_POINT('Ctrl Pts',(-223.799693424538,6.42994281575757,
128.030540825308));
#266954=CARTESIAN_POINT('Ctrl Pts',(-224.078141048351,1.1418480021166,123.895350269195));
#266955=CARTESIAN_POINT('Ctrl Pts',(-224.356588672164,-5.19554934309376,
126.109202699315));
#266956=CARTESIAN_POINT('Ctrl Pts',(-224.635036295977,-6.75849065869668,
132.637675885092));
#266957=CARTESIAN_POINT('Ctrl Pts',(-224.913483919789,-2.11070922958169,
137.481421902441));
#266958=CARTESIAN_POINT('Ctrl Pts',(-225.191931543603,4.47671086764076,
136.189274791569));
#266959=CARTESIAN_POINT('Ctrl Pts',(-225.470379167415,6.95025237698553,
129.948654622468));
#266960=CARTESIAN_POINT('Ctrl Pts',(-225.748826791228,3.03685149058481,
124.494386459301));
#266961=CARTESIAN_POINT('Ctrl Pts',(-226.027274415041,-3.66726755721984,
124.838676288203));
#266962=CARTESIAN_POINT('Ctrl Pts',(-226.305722038854,-7.00134687591997,
130.665138575908));
#266963=CARTESIAN_POINT('Ctrl Pts',(-226.584169662667,-3.9015304504591,
136.619539118521));
#266964=CARTESIAN_POINT('Ctrl Pts',(-226.86261728648,2.78360185861461,137.230074706019));
#266965=CARTESIAN_POINT('Ctrl Pts',(-227.141064910293,6.91074004613266,
131.935692959814));
#266966=CARTESIAN_POINT('Ctrl Pts',(-227.419512534106,4.68724573967455,
125.601672059739));
#266967=CARTESIAN_POINT('Ctrl Pts',(-227.697960157918,-1.8435984168596,
124.048667778841));
#266968=CARTESIAN_POINT('Ctrl Pts',(-227.976407781732,-6.68026569308986,
128.703815182788));
#266969=CARTESIAN_POINT('Ctrl Pts',(-228.254855405544,-5.37809514649209,
135.289261223946));
#266970=CARTESIAN_POINT('Ctrl Pts',(-228.533303029357,0.86628210517778,
137.753302707416));
#266971=CARTESIAN_POINT('Ctrl Pts',(-228.81175065317,6.31458842242258,133.831605885006));
#266972=CARTESIAN_POINT('Ctrl Pts',(-229.090198276983,5.96009646425557,
127.128018550972));
#266973=CARTESIAN_POINT('Ctrl Pts',(-229.368645900796,0.128567022336676,
123.802809976843));
#266974=CARTESIAN_POINT('Ctrl Pts',(-229.647093524609,-5.82110923226107,
126.911684396774));
#266975=CARTESIAN_POINT('Ctrl Pts',(-229.925541148421,-6.42147047940683,
133.597738095807));
#266976=CARTESIAN_POINT('Ctrl Pts',(-230.203988772235,-1.12081406224988,
137.716814356412));
#266977=CARTESIAN_POINT('Ctrl Pts',(-230.482436396047,5.20981572330331,
135.483683323156));
#266978=CARTESIAN_POINT('Ctrl Pts',(-230.76088401986,6.75287937278817,128.950483321085));
#266979=CARTESIAN_POINT('Ctrl Pts',(-231.039331643673,2.0903767751783,124.120905987538));
#266980=CARTESIAN_POINT('Ctrl Pts',(-231.317779267486,-4.49307995823781,
125.433096954076));
#266981=CARTESIAN_POINT('Ctrl Pts',(-231.596226891299,-6.94761570919197,
131.681216826544));
#266982=CARTESIAN_POINT('Ctrl Pts',(-231.874674515112,-3.01763203329532,
137.123548679767));
#266983=CARTESIAN_POINT('Ctrl Pts',(-232.153122138925,3.68540806167951,
136.758855413326));
#266984=CARTESIAN_POINT('Ctrl Pts',(-232.431569762738,7.00173819016367,
130.922272322824));
#266985=CARTESIAN_POINT('Ctrl Pts',(-232.71001738655,3.88381297581431,124.977334135496));
#266986=CARTESIAN_POINT('Ctrl Pts',(-232.988465010364,-2.80314662849731,
124.38714861912));
#266987=CARTESIAN_POINT('Ctrl Pts',(-233.266912634176,-6.914151422545,129.694067431082));
#266988=CARTESIAN_POINT('Ctrl Pts',(-233.545360257989,-4.67138883434919,
136.021291440583));
#266989=CARTESIAN_POINT('Ctrl Pts',(-233.823807881803,1.86415188258208,
137.554410884971));
#266990=CARTESIAN_POINT('Ctrl Pts',(-234.102255505615,6.68662808830262,
132.884563891901));
#266991=CARTESIAN_POINT('Ctrl Pts',(-234.380703129428,5.36441974081549,
126.303111713297));
#266992=CARTESIAN_POINT('Ctrl Pts',(-234.659150753241,-0.887428282007554,
123.858087379481));
#266993=CARTESIAN_POINT('Ctrl Pts',(-234.937598377053,-6.32377306694735,
127.796348807152));
#266994=CARTESIAN_POINT('Ctrl Pts',(-235.216046000867,-5.94887933685163,
134.498826139047));
#266995=CARTESIAN_POINT('Ctrl Pts',(-235.494493624679,-0.107256115101469,
137.806270141374));
#266996=CARTESIAN_POINT('Ctrl Pts',(-235.772941248493,5.83293023667497,
134.679301353618));
#266997=CARTESIAN_POINT('Ctrl Pts',(-236.051388872305,6.41293865542997,
127.991451330808));
#266998=CARTESIAN_POINT('Ctrl Pts',(-236.329836496118,1.09976973931543,
123.88852752427));
#266999=CARTESIAN_POINT('Ctrl Pts',(-236.608284119931,-5.22403384049169,
126.140916473241));
#267000=CARTESIAN_POINT('Ctrl Pts',(-236.886731743744,-6.7472055291277,
132.678782768935));
#267001=CARTESIAN_POINT('Ctrl Pts',(-237.165179367557,-2.07002495581049,
137.494146678133));
#267002=CARTESIAN_POINT('Ctrl Pts',(-237.44362699137,4.50940742555574,136.161924011888));
#267003=CARTESIAN_POINT('Ctrl Pts',(-237.722074615182,6.94491467963605,
129.906362317783));
#267004=CARTESIAN_POINT('Ctrl Pts',(-238.000522238996,2.99838462107406,
124.476017191522));
#267005=CARTESIAN_POINT('Ctrl Pts',(-238.278969862808,-3.70351442502255,
124.861110517033));
#267006=CARTESIAN_POINT('Ctrl Pts',(-238.557417486622,-7.00206464126185,
130.707760341024));
#267007=CARTESIAN_POINT('Ctrl Pts',(-238.835865110434,-3.86605952205578,
136.64318109997));
#267008=CARTESIAN_POINT('Ctrl Pts',(-239.114312734247,2.82266543041169,
137.213011077826));
#267009=CARTESIAN_POINT('Ctrl Pts',(-239.39276035806,6.91749874720356,131.893604362681));
#267010=CARTESIAN_POINT('Ctrl Pts',(-239.671207981873,4.655488653916,125.573235858291));
#267011=CARTESIAN_POINT('Ctrl Pts',(-239.949655605686,-1.88468807905538,
124.060015453022));
#267012=CARTESIAN_POINT('Ctrl Pts',(-240.228103229498,-6.69292853950653,
128.74451877439));
#267013=CARTESIAN_POINT('Ctrl Pts',(-240.506550853312,-5.35069463988719,
135.321916120768));
#267014=CARTESIAN_POINT('Ctrl Pts',(-240.784998477124,0.908566237823527,
137.747900654559));
#267015=CARTESIAN_POINT('Ctrl Pts',(-241.063446100938,6.33289912890243,
133.79311110514));
#267016=CARTESIAN_POINT('Ctrl Pts',(-241.34189372475,5.9376070998423,127.091805866219));
#267017=CARTESIAN_POINT('Ctrl Pts',(-241.620341348563,0.0859442142595387,
123.802157075403));
#267018=CARTESIAN_POINT('Ctrl Pts',(-241.898788972376,-5.84469720561911,
126.947191263173));
#267019=CARTESIAN_POINT('Ctrl Pts',(-242.177236596189,-6.40434742286629,
133.636775654432));
#267020=CARTESIAN_POINT('Ctrl Pts',(-242.455684220002,-1.07871522826414,
137.723508997977));
#267021=CARTESIAN_POINT('Ctrl Pts',(-242.734131843815,5.23820356294377,
135.451882999115));
#267022=CARTESIAN_POINT('Ctrl Pts',(-243.012579467628,6.74146918027728,
128.909410975699));
#267023=CARTESIAN_POINT('Ctrl Pts',(-243.29102709144,2.04965396001378,124.108305099723));
#267024=CARTESIAN_POINT('Ctrl Pts',(-243.569474715254,-4.52569311833944,
125.460547124147));
#267025=CARTESIAN_POINT('Ctrl Pts',(-243.847922339066,-6.94214931333881,
131.72349268922));
#267026=CARTESIAN_POINT('Ctrl Pts',(-244.12636996288,-2.9791094322281,137.141800782542));
#267027=CARTESIAN_POINT('Ctrl Pts',(-244.404817586691,3.72158647951367,
136.736310965414));
#267028=CARTESIAN_POINT('Ctrl Pts',(-244.683265210505,7.00232622618917,
130.879648570499));
#267029=CARTESIAN_POINT('Ctrl Pts',(-244.961712834317,3.84827025365086,
124.953800224859));
#267030=CARTESIAN_POINT('Ctrl Pts',(-245.240160458131,-2.84215808354001,
124.404331064352));
#267031=CARTESIAN_POINT('Ctrl Pts',(-245.518608081943,-6.92078198909823,
129.736176404423));
#267032=CARTESIAN_POINT('Ctrl Pts',(-245.797055705757,-4.63954534567172,
136.049630852671));
#267033=CARTESIAN_POINT('Ctrl Pts',(-246.075503329569,1.90520681603656,
137.542938200555));
#267034=CARTESIAN_POINT('Ctrl Pts',(-246.353950953382,6.69916698833444,
132.843821947487));
#267035=CARTESIAN_POINT('Ctrl Pts',(-246.632398577195,5.33691997085474,
126.270540365447));
#267036=CARTESIAN_POINT('Ctrl Pts',(-246.910846201008,-0.929695776805409,
123.86361810567));
#267037=CARTESIAN_POINT('Ctrl Pts',(-247.189293824821,-6.34196652374499,
127.834899140205));
#267038=CARTESIAN_POINT('Ctrl Pts',(-247.467741448634,-5.9262798576518,
134.534970206175));
#267039=CARTESIAN_POINT('Ctrl Pts',(-247.746189072447,-0.0646315172428821,
137.806793310625));
#267040=CARTESIAN_POINT('Ctrl Pts',(-248.024636696259,5.85641003008765,
134.643722858007));
#267041=CARTESIAN_POINT('Ctrl Pts',(-248.303084320073,6.39569686130214,
127.952466069697));
#267042=CARTESIAN_POINT('Ctrl Pts',(-248.581531943885,1.05765072414216,
123.881961048084));
#267043=CARTESIAN_POINT('Ctrl Pts',(-248.859979567699,-5.25232475939459,
126.172803052805));
#267044=CARTESIAN_POINT('Ctrl Pts',(-249.138427191511,-6.73567037937639,
132.719820195375));
#267045=CARTESIAN_POINT('Ctrl Pts',(-249.416874815324,-2.02926397650361,
137.506623561341));
#267046=CARTESIAN_POINT('Ctrl Pts',(-249.695322439137,4.54193688572079,
136.134374705723));
#267047=CARTESIAN_POINT('Ctrl Pts',(-249.97377006295,6.93931963591783,129.864103288757));
#267048=CARTESIAN_POINT('Ctrl Pts',(-250.252217686763,2.95980664532115,
124.457882422832));
#267049=CARTESIAN_POINT('Ctrl Pts',(-250.530665310576,-3.73962405773988,
124.883764975191));
#267050=CARTESIAN_POINT('Ctrl Pts',(-250.809112934388,-7.00252294251614,
130.750385685678));
#267051=CARTESIAN_POINT('Ctrl Pts',(-251.087560558202,-3.83044533540895,
136.666606721818));
#267052=CARTESIAN_POINT('Ctrl Pts',(-251.366008182014,2.86162440732935,
137.195709974661));
#267053=CARTESIAN_POINT('Ctrl Pts',(-251.644455805827,6.9240011177651,131.851475403357));
#267054=CARTESIAN_POINT('Ctrl Pts',(-251.92290342964,4.62355905740654,125.54499349784));
#267055=CARTESIAN_POINT('Ctrl Pts',(-252.201351053453,-1.92570790361727,
124.071613041873));
#267056=CARTESIAN_POINT('Ctrl Pts',(-252.479798677266,-6.70534337666252,
128.785298693283));
#267057=CARTESIAN_POINT('Ctrl Pts',(-252.758246301079,-5.3230958619522,
135.354403619622));
#267058=CARTESIAN_POINT('Ctrl Pts',(-253.036693924892,0.950816704398073,
137.74224130304));
#267059=CARTESIAN_POINT('Ctrl Pts',(-253.315141548704,6.35097516523885,
133.754505582129));
#267060=CARTESIAN_POINT('Ctrl Pts',(-253.593589172518,5.91489771943887,
127.055730740027));
#267061=CARTESIAN_POINT('Ctrl Pts',(-253.87203679633,0.0433182135112656,
123.801763664947));
#267062=CARTESIAN_POINT('Ctrl Pts',(-254.150484420143,-5.86806858651122,
126.982841017323));
#267063=CARTESIAN_POINT('Ctrl Pts',(-254.428932043956,-6.38698707931617,
133.675708334441));
#267064=CARTESIAN_POINT('Ctrl Pts',(-254.707379667769,-1.03657636838919,
137.729947101491));
#267065=CARTESIAN_POINT('Ctrl Pts',(-254.985827291582,5.26639719763008,
135.41991073597));
#267066=CARTESIAN_POINT('Ctrl Pts',(-255.264274915395,6.72980937160111,
128.868408326187));
#267067=CARTESIAN_POINT('Ctrl Pts',(-255.542722539208,2.00885483266244,
124.095953322692));
#267068=CARTESIAN_POINT('Ctrl Pts',(-255.821170163021,-4.5581378946222,
125.488193449449));
#267069=CARTESIAN_POINT('Ctrl Pts',(-256.099617786833,-6.93642696247006,
131.765738008466));
#267070=CARTESIAN_POINT('Ctrl Pts',(-256.378065410647,-2.94047400549736,
137.159811411449));
#267071=CARTESIAN_POINT('Ctrl Pts',(-256.656513034459,3.7576223973322,136.713559240208));
#267072=CARTESIAN_POINT('Ctrl Pts',(-256.934960658272,7.0026634652268,130.836998362911));
#267073=CARTESIAN_POINT('Ctrl Pts',(-257.213408282085,3.81256854888166,
124.930527794066));
#267074=CARTESIAN_POINT('Ctrl Pts',(-257.491855905898,-2.88103328591622,
124.421666290213));
#267075=CARTESIAN_POINT('Ctrl Pts',(-257.770303529711,-6.92721451599304,
129.778484277494));
#267076=CARTESIAN_POINT('Ctrl Pts',(-258.048751153524,-4.60741964202412,
136.077475067175));
#267077=CARTESIAN_POINT('Ctrl Pts',(-258.327198777336,1.94598288966397,
137.53178391186));
#267078=CARTESIAN_POINT('Ctrl Pts',(-258.60564640115,6.71185090883407,132.801931226644));
#267079=CARTESIAN_POINT('Ctrl Pts',(-258.884094024962,5.30847971878909,
126.240167716581));
#267080=CARTESIAN_POINT('Ctrl Pts',(-259.162541648776,-0.970525071554103,
123.86553674091));
#267081=CARTESIAN_POINT('Ctrl Pts',(-259.440989272588,-6.36258613651914,
127.881151058581));
#267082=CARTESIAN_POINT('Ctrl Pts',(-259.673028959099,-5.97575359986218,
133.442106215535));
#267083=CARTESIAN_POINT('Ctrl Pts',(-259.858689921174,-2.9628379271774,
136.206922793942));
#267084=CARTESIAN_POINT('Ctrl Pts',(-259.951535008647,-1.00384119663989,
136.721969923993));
#267085=CARTESIAN_POINT('Ctrl Pts',(-259.997972158816,-0.016740685831905,
136.724751058381));
#267086=CARTESIAN_POINT('Ctrl Pts',(210.384788400103,3.2437100417032,135.350446923363));
#267087=CARTESIAN_POINT('Ctrl Pts',(210.338370536501,4.00135710969089,134.809856772425));
#267088=CARTESIAN_POINT('Ctrl Pts',(210.245544735596,5.2274450014198,133.344996311945));
#267089=CARTESIAN_POINT('Ctrl Pts',(210.059903060087,6.03752477204218,129.574087134129));
#267090=CARTESIAN_POINT('Ctrl Pts',(209.827863373576,3.30140998082846,125.08375145776));
#267091=CARTESIAN_POINT('Ctrl Pts',(209.549415749763,-3.03864792542705,
124.935284604053));
#267092=CARTESIAN_POINT('Ctrl Pts',(209.27096812595,-6.57501826603042,130.18815040753));
#267093=CARTESIAN_POINT('Ctrl Pts',(208.992520502138,-4.0751627655632,136.003208990552));
#267094=CARTESIAN_POINT('Ctrl Pts',(208.714072878324,2.17267791003586,137.042921783734));
#267095=CARTESIAN_POINT('Ctrl Pts',(208.435625254512,6.42228832295553,132.348569225854));
#267096=CARTESIAN_POINT('Ctrl Pts',(208.157177630698,4.77100074356668,126.235763887068));
#267097=CARTESIAN_POINT('Ctrl Pts',(207.878730006886,-1.26506482749479,
124.320958291314));
#267098=CARTESIAN_POINT('Ctrl Pts',(207.600282383073,-6.13835327551471,
128.364250828182));
#267099=CARTESIAN_POINT('Ctrl Pts',(207.32183475926,-5.37092434612766,134.649796015418));
#267100=CARTESIAN_POINT('Ctrl Pts',(207.043387135447,0.332190207827403,
137.40162108792));
#267101=CARTESIAN_POINT('Ctrl Pts',(206.764939511634,5.73000189292936,134.090861108297));
#267102=CARTESIAN_POINT('Ctrl Pts',(206.486491887821,5.86224098722307,127.759980958474));
#267103=CARTESIAN_POINT('Ctrl Pts',(206.208044264008,0.607356820266201,
124.226729984437));
#267104=CARTESIAN_POINT('Ctrl Pts',(205.929596640195,-5.20565320191231,
126.738003936844));
#267105=CARTESIAN_POINT('Ctrl Pts',(205.651149016382,-6.23492509722864,
132.986059061584));
#267106=CARTESIAN_POINT('Ctrl Pts',(205.37270139257,-1.53460390898592,137.229240938669));
#267107=CARTESIAN_POINT('Ctrl Pts',(205.094253768756,4.57594250116295,135.568271122458));
#267108=CARTESIAN_POINT('Ctrl Pts',(204.815806144944,6.48142172411287,129.529500574057));
#267109=CARTESIAN_POINT('Ctrl Pts',(204.537358521131,2.43079079302514,124.662263970705));
#267110=CARTESIAN_POINT('Ctrl Pts',(204.258910897318,-3.85361800715474,
125.439314209572));
#267111=CARTESIAN_POINT('Ctrl Pts',(203.980463273505,-6.5967401814699,131.146579956944));
#267112=CARTESIAN_POINT('Ctrl Pts',(203.702015649692,-3.27778036432047,
136.539362872731));
#267113=CARTESIAN_POINT('Ctrl Pts',(203.42356802588,3.05329946149495,136.661958874297));
#267114=CARTESIAN_POINT('Ctrl Pts',(203.145120402066,6.5785462535266,131.40170824395));
#267115=CARTESIAN_POINT('Ctrl Pts',(202.866672778254,4.05843041346184,125.592524323598));
#267116=CARTESIAN_POINT('Ctrl Pts',(202.58822515444,-2.19118470860141,124.572763346851));
#267117=CARTESIAN_POINT('Ctrl Pts',(202.309777530628,-6.42720813017419,
129.279535830482));
#267118=CARTESIAN_POINT('Ctrl Pts',(202.031329906815,-4.75694126595338,
135.387547802118));
#267119=CARTESIAN_POINT('Ctrl Pts',(201.752882283002,1.28472223178851,137.283834652022));
#267120=CARTESIAN_POINT('Ctrl Pts',(201.474434659189,6.14578876089344,133.225801404307));
#267121=CARTESIAN_POINT('Ctrl Pts',(201.195987035376,5.35917565710019,126.94258236746));
#267122=CARTESIAN_POINT('Ctrl Pts',(200.917539411563,-0.352258065224466,
124.208148884143));
#267123=CARTESIAN_POINT('Ctrl Pts',(200.63909178775,-5.73998383440169,127.535311740963));
#267124=CARTESIAN_POINT('Ctrl Pts',(200.360644163938,-5.85294487354697,
133.866570813476));
#267125=CARTESIAN_POINT('Ctrl Pts',(200.082196540124,-0.587335506164227,
137.383808313225));
#267126=CARTESIAN_POINT('Ctrl Pts',(199.803748916312,5.2180064984534,134.854854804556));
#267127=CARTESIAN_POINT('Ctrl Pts',(199.525301292498,6.22825544477889,128.603695015683));
#267128=CARTESIAN_POINT('Ctrl Pts',(199.246853668687,1.51504190454761,124.374839406449));
#267129=CARTESIAN_POINT('Ctrl Pts',(198.968406044873,-4.5904211320519,126.054399690658));
#267130=CARTESIAN_POINT('Ctrl Pts',(198.689958421061,-6.47751140283473,
132.098942018204));
#267131=CARTESIAN_POINT('Ctrl Pts',(198.411510797247,-2.41208513843682,
136.95382728238));
#267132=CARTESIAN_POINT('Ctrl Pts',(198.133063173434,3.86992953127461,136.15765309974));
#267133=CARTESIAN_POINT('Ctrl Pts',(197.854615549622,6.59566801831256,130.442064648858));
#267134=CARTESIAN_POINT('Ctrl Pts',(197.576167925809,3.26030981281707,125.059408494076));
#267135=CARTESIAN_POINT('Ctrl Pts',(197.297720301996,-3.07111383566833,
124.956082684267));
#267136=CARTESIAN_POINT('Ctrl Pts',(197.019272678183,-6.58033390142619,
130.227038590899));
#267137=CARTESIAN_POINT('Ctrl Pts',(196.74082505437,-4.04254857895594,136.028525236289));
#267138=CARTESIAN_POINT('Ctrl Pts',(196.462377430557,2.21014139809766,137.029259811701));
#267139=CARTESIAN_POINT('Ctrl Pts',(196.183929806745,6.43181940170927,132.309616130935));
#267140=CARTESIAN_POINT('Ctrl Pts',(195.905482182931,4.74296958699597,126.206716169203));
#267141=CARTESIAN_POINT('Ctrl Pts',(195.627034559119,-1.30443757122094,
124.328826848098));
#267142=CARTESIAN_POINT('Ctrl Pts',(195.348586935305,-6.15313032680387,
128.401636713722));
#267143=CARTESIAN_POINT('Ctrl Pts',(195.070139311493,-5.34739690918169,
134.682432467391));
#267144=CARTESIAN_POINT('Ctrl Pts',(194.791691687679,0.372333033116476,
137.399469645412));
#267145=CARTESIAN_POINT('Ctrl Pts',(194.513244063867,5.74990710746052,134.055923815831));
#267146=CARTESIAN_POINT('Ctrl Pts',(194.234796440054,5.84359744862664,127.724350254736));
#267147=CARTESIAN_POINT('Ctrl Pts',(193.956348816241,0.567307210110782,
124.223155750211));
#267148=CARTESIAN_POINT('Ctrl Pts',(193.677901192428,-5.23031063999889,
126.769767009054));
#267149=CARTESIAN_POINT('Ctrl Pts',(193.399453568615,-6.22152852682933,
133.023972693263));
#267150=CARTESIAN_POINT('Ctrl Pts',(193.121005944802,-1.49546563606909,
137.238463313985));
#267151=CARTESIAN_POINT('Ctrl Pts',(192.84255832099,4.60485711668079,135.540327880088));
#267152=CARTESIAN_POINT('Ctrl Pts',(192.564110697177,6.47354113897745,129.490069896797));
#267153=CARTESIAN_POINT('Ctrl Pts',(192.285663073364,2.39335710461987,124.64758087922));
#267154=CARTESIAN_POINT('Ctrl Pts',(192.007215449551,-3.88620518688872,
125.462871665772));
#267155=CARTESIAN_POINT('Ctrl Pts',(191.728767825738,-6.59453476332446,
131.18672985278));
#267156=CARTESIAN_POINT('Ctrl Pts',(191.450320201925,-3.24280905319821,
136.559209392401));
#267157=CARTESIAN_POINT('Ctrl Pts',(191.171872578112,3.08889975678785,136.643264047941));
#267158=CARTESIAN_POINT('Ctrl Pts',(190.893424954299,6.58206059142805,131.361651697256));
#267159=CARTESIAN_POINT('Ctrl Pts',(190.614977330486,4.02662929408197,125.567916069518));
#267160=CARTESIAN_POINT('Ctrl Pts',(190.336529706674,-2.22907761274862,
124.586217166899));
#267161=CARTESIAN_POINT('Ctrl Pts',(190.05808208286,-6.43637108995848,129.318688322246));
#267162=CARTESIAN_POINT('Ctrl Pts',(189.779634459048,-4.72895396970476,
135.416419737866));
#267163=CARTESIAN_POINT('Ctrl Pts',(189.501186835235,1.32414082646293,137.275894133543));
#267164=CARTESIAN_POINT('Ctrl Pts',(189.222739211422,6.16041489098677,133.188345380025));
#267165=CARTESIAN_POINT('Ctrl Pts',(188.944291587609,5.33556862369218,126.910031093937));
#267166=CARTESIAN_POINT('Ctrl Pts',(188.665843963796,-0.392404551757433,
124.210415391489));
#267167=CARTESIAN_POINT('Ctrl Pts',(188.387396339983,-5.75977711417006,
127.570313219673));
#267168=CARTESIAN_POINT('Ctrl Pts',(188.10894871617,-5.83419588941534,133.902142614521));
#267169=CARTESIAN_POINT('Ctrl Pts',(187.830501092358,-0.547273658602122,
137.387261689231));
#267170=CARTESIAN_POINT('Ctrl Pts',(187.552053468544,5.24256632866185,134.823016271676));
#267171=CARTESIAN_POINT('Ctrl Pts',(187.273605844732,6.214743973489,128.565822630237));
#267172=CARTESIAN_POINT('Ctrl Pts',(186.995158220918,1.47587551380139,124.365736040492));
#267173=CARTESIAN_POINT('Ctrl Pts',(186.716710597106,-4.61925044254253,
126.082430892781));
#267174=CARTESIAN_POINT('Ctrl Pts',(186.438262973293,-6.46951090511933,
132.138348483055));
#267175=CARTESIAN_POINT('Ctrl Pts',(186.15981534948,-2.37460689906969,136.968396393875));
#267176=CARTESIAN_POINT('Ctrl Pts',(185.881367725667,3.90244484122886,136.133996556155));
#267177=CARTESIAN_POINT('Ctrl Pts',(185.602920101854,6.59334041746713,130.401921658061));
#267178=CARTESIAN_POINT('Ctrl Pts',(185.324472478041,3.22527825263932,125.039668503516));
#267179=CARTESIAN_POINT('Ctrl Pts',(185.046024854228,-3.10665706276191,
124.974885780916));
#267180=CARTESIAN_POINT('Ctrl Pts',(184.767577230416,-6.5837263061198,130.26710564752));
#267181=CARTESIAN_POINT('Ctrl Pts',(184.489129606603,-4.01067270706429,
136.05303658523));
#267182=CARTESIAN_POINT('Ctrl Pts',(184.21068198279,2.247993177529,137.015690720733));
#267183=CARTESIAN_POINT('Ctrl Pts',(183.932234358977,6.44086315254518,132.270435931769));
#267184=CARTESIAN_POINT('Ctrl Pts',(183.653786735164,4.71489454403,126.177929550814));
#267185=CARTESIAN_POINT('Ctrl Pts',(183.375339111351,-1.34383181504516,
124.33688730648));
#267186=CARTESIAN_POINT('Ctrl Pts',(183.096891487538,-6.16764238592767,
128.439137081397));
#267187=CARTESIAN_POINT('Ctrl Pts',(182.818443863726,-5.32369091022383,
134.71491173846));
#267188=CARTESIAN_POINT('Ctrl Pts',(182.539996239912,0.412472435216218,
137.397080956463));
#267189=CARTESIAN_POINT('Ctrl Pts',(182.2615486161,5.76959376309122,134.020862255314));
#267190=CARTESIAN_POINT('Ctrl Pts',(181.983100992287,5.82474028301032,127.688835683913));
#267191=CARTESIAN_POINT('Ctrl Pts',(181.704653368474,0.527235037225083,
124.219824324685));
#267192=CARTESIAN_POINT('Ctrl Pts',(181.426205744661,-5.25477345090652,
126.801680146133));
#267193=CARTESIAN_POINT('Ctrl Pts',(181.147758120848,-6.20790184760947,
133.061803779016));
#267194=CARTESIAN_POINT('Ctrl Pts',(180.869310497035,-1.45627171922457,
137.247447428754));
#267195=CARTESIAN_POINT('Ctrl Pts',(180.590862873222,4.63360097629919,135.5122090613));
#267196=CARTESIAN_POINT('Ctrl Pts',(180.31241524941,6.46542073859599,129.450687965235));
#267197=CARTESIAN_POINT('Ctrl Pts',(180.033967625596,2.35583469548556,124.633125906077));
#267198=CARTESIAN_POINT('Ctrl Pts',(179.755520001784,-3.91864834385308,
125.4866270652));
#267199=CARTESIAN_POINT('Ctrl Pts',(179.477072377971,-6.59208499180493,
131.226865573221));
#267200=CARTESIAN_POINT('Ctrl Pts',(179.198624754158,-3.20771757354326,
136.578842667508));
#267201=CARTESIAN_POINT('Ctrl Pts',(178.920177130345,3.12438558908937,136.62435285703));
#267202=CARTESIAN_POINT('Ctrl Pts',(178.641729506532,6.58533103007041,131.32157450091));
#267203=CARTESIAN_POINT('Ctrl Pts',(178.363281882719,3.99467896572256,125.5435018533));
#267204=CARTESIAN_POINT('Ctrl Pts',(178.084834258906,-2.26688791720775,
124.599901402811));
#267205=CARTESIAN_POINT('Ctrl Pts',(177.806386635093,-6.44529554785546,
129.357895865998));
#267206=CARTESIAN_POINT('Ctrl Pts',(177.527939011281,-4.70079144021631,
135.445120772143));
#267207=CARTESIAN_POINT('Ctrl Pts',(177.249491387467,1.36351035455298,137.26771380997));
#267208=CARTESIAN_POINT('Ctrl Pts',(176.971043763655,6.17481274467203,133.150801016333));
#267209=CARTESIAN_POINT('Ctrl Pts',(176.692596139842,5.31176387881016,126.877624126216));
#267210=CARTESIAN_POINT('Ctrl Pts',(176.414148516029,-0.432536497586617,
124.212926239906));
#267211=CARTESIAN_POINT('Ctrl Pts',(176.135700892216,-5.77935696328393,
127.605434537195));
#267212=CARTESIAN_POINT('Ctrl Pts',(175.857253268403,-5.81523071700703,
133.937599626117));
#267213=CARTESIAN_POINT('Ctrl Pts',(175.57880564459,-0.50719153161477,137.390471133416));
#267214=CARTESIAN_POINT('Ctrl Pts',(175.300358020777,5.2669318936477,134.791028826034));
#267215=CARTESIAN_POINT('Ctrl Pts',(175.021910396965,6.20100221257536,128.528033194638));
#267216=CARTESIAN_POINT('Ctrl Pts',(174.743462773151,1.43665443394553,124.356871260137));
#267217=CARTESIAN_POINT('Ctrl Pts',(174.465015149339,-4.64790858500931,
126.110637067746));
#267218=CARTESIAN_POINT('Ctrl Pts',(174.186567525525,-6.46127067729819,
132.177705516496));
#267219=CARTESIAN_POINT('Ctrl Pts',(173.908119901713,-2.33704066777073,
136.982737094758));
#267220=CARTESIAN_POINT('Ctrl Pts',(173.6296722779,3.93481554465429,136.11014252095));
#267221=CARTESIAN_POINT('Ctrl Pts',(173.351224654087,6.59076849796787,130.361793579788));
#267222=CARTESIAN_POINT('Ctrl Pts',(173.072777030274,3.1901271785899,125.020142125741));
#267223=CARTESIAN_POINT('Ctrl Pts',(172.794329406461,-3.14208517153551,
124.993904890899));
#267224=CARTESIAN_POINT('Ctrl Pts',(172.515881782648,-6.58687474841394,
130.30719261232));
#267225=CARTESIAN_POINT('Ctrl Pts',(172.237434158836,-3.97864821822065,
136.077353442554));
#267226=CARTESIAN_POINT('Ctrl Pts',(171.958986535022,2.28576165674636,137.001891466644));
#267227=CARTESIAN_POINT('Ctrl Pts',(171.68053891121,6.44966823482829,132.231201406644));
#267228=CARTESIAN_POINT('Ctrl Pts',(171.402091287397,4.68664478891289,126.149314366529));
#267229=CARTESIAN_POINT('Ctrl Pts',(171.123643663584,-1.38317626268716,
124.345187419464));
#267230=CARTESIAN_POINT('Ctrl Pts',(170.845196039771,-6.18192590079466,
128.476725093301));
#267231=CARTESIAN_POINT('Ctrl Pts',(170.566748415958,-5.29978763994156,
134.747246102621));
#267232=CARTESIAN_POINT('Ctrl Pts',(170.288300792145,0.452596552998033,
137.394447971839));
#267233=CARTESIAN_POINT('Ctrl Pts',(170.009853168332,5.78906662430322,133.985681506144));
#267234=CARTESIAN_POINT('Ctrl Pts',(169.73140554452,5.80566727950083,127.653436560012));
#267235=CARTESIAN_POINT('Ctrl Pts',(169.452957920706,0.487143327451347,
124.216736891574));
#267236=CARTESIAN_POINT('Ctrl Pts',(169.174510296894,-5.27904154425138,
126.833741604011));
#267237=CARTESIAN_POINT('Ctrl Pts',(168.896062673081,-6.19404513230377,
133.099551214382));
#267238=CARTESIAN_POINT('Ctrl Pts',(168.617615049268,-1.41702383969606,
137.256192792574));
#267239=CARTESIAN_POINT('Ctrl Pts',(168.339167425455,4.66217313612931,135.483915791456));
#267240=CARTESIAN_POINT('Ctrl Pts',(168.060719801642,6.45706075967145,129.411356194513));
#267241=CARTESIAN_POINT('Ctrl Pts',(167.782272177829,2.3182249900303,124.618899610305));
#267242=CARTESIAN_POINT('Ctrl Pts',(167.503824554016,-3.95094629386185,
125.510579515201));
#267243=CARTESIAN_POINT('Ctrl Pts',(167.225376930203,-6.58939094815179,
131.266985637585));
#267244=CARTESIAN_POINT('Ctrl Pts',(166.946929306391,-3.1725072307341,136.59826196706));
#267245=CARTESIAN_POINT('Ctrl Pts',(166.668481682578,3.15975564613386,136.605226004165));
#267246=CARTESIAN_POINT('Ctrl Pts',(166.390034058765,6.58835744684964,131.281478139015));
#267247=CARTESIAN_POINT('Ctrl Pts',(166.111586434952,3.96258061306513,125.519282580138));
#267248=CARTESIAN_POINT('Ctrl Pts',(165.833138811139,-2.30461422130139,
124.613815547242));
#267249=CARTESIAN_POINT('Ctrl Pts',(165.554691187326,-6.45398117295568,
129.397157009033));
#267250=CARTESIAN_POINT('Ctrl Pts',(165.276243563513,-4.67245472117232,
135.473649841348));
#267251=CARTESIAN_POINT('Ctrl Pts',(164.9977959397,1.40282935726546,137.259293984466));
#267252=CARTESIAN_POINT('Ctrl Pts',(164.719348315888,6.18898178840028,133.11316970443));
#267253=CARTESIAN_POINT('Ctrl Pts',(164.440900692075,5.2877623045642,126.845362665158));
#267254=CARTESIAN_POINT('Ctrl Pts',(164.162453068262,-0.472652415616787,
124.215681336348));
#267255=CARTESIAN_POINT('Ctrl Pts',(163.884005444449,-5.79872265620017,
127.640674392099));
#267256=CARTESIAN_POINT('Ctrl Pts',(163.605557820636,-5.79605005908598,
133.97294053439));
#267257=CARTESIAN_POINT('Ctrl Pts',(163.327110196823,-0.467090610458611,
137.393436526853));
#267258=CARTESIAN_POINT('Ctrl Pts',(163.04866257301,5.29110229053537,134.758893652935));
#267259=CARTESIAN_POINT('Ctrl Pts',(162.770214949197,6.18703067124424,128.49032810919));
#267260=CARTESIAN_POINT('Ctrl Pts',(162.491767325384,1.39738011833125,124.34824539387));
#267261=CARTESIAN_POINT('Ctrl Pts',(162.213319701571,-4.67639449751423,
126.139017170363));
#267262=CARTESIAN_POINT('Ctrl Pts',(161.934872077759,-6.45279102471594,
132.217011660137));
#267263=CARTESIAN_POINT('Ctrl Pts',(161.656424453946,-2.29938783657033,
136.996848853628));
#267264=CARTESIAN_POINT('Ctrl Pts',(161.377976830133,3.96704044204275,136.086091878046));
#267265=CARTESIAN_POINT('Ctrl Pts',(161.09952920632,6.58795235511813,130.321681900999));
#267266=CARTESIAN_POINT('Ctrl Pts',(160.821081582507,3.15485789320466,125.000830084311));
#267267=CARTESIAN_POINT('Ctrl Pts',(160.542633958694,-3.17739684918762,
125.013139309456));
#267268=CARTESIAN_POINT('Ctrl Pts',(160.264186334881,-6.58977911164196,
130.347297999864));
#267269=CARTESIAN_POINT('Ctrl Pts',(159.985738711068,-3.94647629910411,
136.10147490719));
#267270=CARTESIAN_POINT('Ctrl Pts',(159.707291087255,2.32344543622502,136.98786256077));
#267271=CARTESIAN_POINT('Ctrl Pts',(159.428843463442,6.45823432228318,132.191914009409));
#267272=CARTESIAN_POINT('Ctrl Pts',(159.15039583963,4.65822136844951,126.120871676696));
#267273=CARTESIAN_POINT('Ctrl Pts',(158.871948215817,-1.42246945622416,
124.353726879487));
#267274=CARTESIAN_POINT('Ctrl Pts',(158.593500592004,-6.19598034212407,
128.514399356595));
#267275=CARTESIAN_POINT('Ctrl Pts',(158.315052968191,-5.2756879840792,134.779434361708));
#267276=CARTESIAN_POINT('Ctrl Pts',(158.036605344378,0.49270389964821,137.391570789103));
#267277=CARTESIAN_POINT('Ctrl Pts',(157.758157720565,5.80832496952254,133.950382871961));
#267278=CARTESIAN_POINT('Ctrl Pts',(157.479710096752,5.78637914485521,127.618154194761));
#267279=CARTESIAN_POINT('Ctrl Pts',(157.201262472939,0.447033566402335,
124.213893565282));
#267280=CARTESIAN_POINT('Ctrl Pts',(156.922814849126,-5.3031140207705,126.865950194636));
#267281=CARTESIAN_POINT('Ctrl Pts',(156.644367225313,-6.17995889437779,
133.137213600617));
#267282=CARTESIAN_POINT('Ctrl Pts',(156.365919601501,-1.37772345182797,
137.264699081378));
#267283=CARTESIAN_POINT('Ctrl Pts',(156.087471977688,4.69057253741941,135.455449118975));
#267284=CARTESIAN_POINT('Ctrl Pts',(155.809024353875,6.44846151198586,129.372076042081));
#267285=CARTESIAN_POINT('Ctrl Pts',(155.530576730062,2.28052938189546,124.604902519066));
#267286=CARTESIAN_POINT('Ctrl Pts',(155.252129106249,-3.98309784010292,
125.534728128207));
#267287=CARTESIAN_POINT('Ctrl Pts',(154.973681482436,-6.58645273219382,
131.307088559209));
#267288=CARTESIAN_POINT('Ctrl Pts',(154.695233858623,-3.13717932950269,
136.617466571466));
#267289=CARTESIAN_POINT('Ctrl Pts',(154.41678623481,3.19500861727094,136.585884198101));
#267290=CARTESIAN_POINT('Ctrl Pts',(154.138338610998,6.59113972962085,131.241364097354));
#267291=CARTESIAN_POINT('Ctrl Pts',(153.859890987185,3.93033542552574,125.495259147487));
#267292=CARTESIAN_POINT('Ctrl Pts',(153.581443363372,-2.3422551270676,124.627959084596));
#267293=CARTESIAN_POINT('Ctrl Pts',(153.302995739559,-6.46242764341012,
129.436470296516));
#267294=CARTESIAN_POINT('Ctrl Pts',(153.024548115746,-4.64394486260028,
135.502005888322));
#267295=CARTESIAN_POINT('Ctrl Pts',(152.746100491933,1.44209637762021,137.250634969033));
#267296=CARTESIAN_POINT('Ctrl Pts',(152.46765286812,6.20292149713234,133.075452838754));
#267297=CARTESIAN_POINT('Ctrl Pts',(152.189205244307,5.26356479034146,126.813247906226));
#267298=CARTESIAN_POINT('Ctrl Pts',(151.910757620494,-0.512750819337957,
124.218680578724));
#267299=CARTESIAN_POINT('Ctrl Pts',(151.632309996682,-5.8178734753159,127.676031478561));
#267300=CARTESIAN_POINT('Ctrl Pts',(151.353862372869,-5.77665462639848,
134.008164029768));
#267301=CARTESIAN_POINT('Ctrl Pts',(151.075414749056,-0.4269723810881,137.39615775966));
#267302=CARTESIAN_POINT('Ctrl Pts',(150.796967125243,5.31507662368183,134.72661194316));
#267303=CARTESIAN_POINT('Ctrl Pts',(150.51851950143,6.17282986721635,128.452708771068));
#267304=CARTESIAN_POINT('Ctrl Pts',(150.240071877617,1.35805402228283,124.339858761329));
#267305=CARTESIAN_POINT('Ctrl Pts',(149.961624253804,-4.70470712450132,
126.167570148998));
#267306=CARTESIAN_POINT('Ctrl Pts',(149.683176629991,-6.44407226158927,
132.256265457474));
#267307=CARTESIAN_POINT('Ctrl Pts',(149.404729006178,-2.26164980070799,
137.010731147569));
#267308=CARTESIAN_POINT('Ctrl Pts',(149.126281382365,3.99911833928874,136.061845518646));
#267309=CARTESIAN_POINT('Ctrl Pts',(148.847833758553,6.58489209327119,130.281588108047));
#267310=CARTESIAN_POINT('Ctrl Pts',(148.56938613474,3.11947170339994,124.981733094838));
#267311=CARTESIAN_POINT('Ctrl Pts',(148.290938510927,-3.21259078723097,
125.032588323847));
#267312=CARTESIAN_POINT('Ctrl Pts',(148.012490887114,-6.59243928818165,
130.387420324031));
#267313=CARTESIAN_POINT('Ctrl Pts',(147.734043263301,-3.91415814185689,
136.125400085308));
#267314=CARTESIAN_POINT('Ctrl Pts',(147.455595639488,2.36104311957866,136.973604522958));
#267315=CARTESIAN_POINT('Ctrl Pts',(147.177148015675,6.46656109749016,132.152575195872));
#267316=CARTESIAN_POINT('Ctrl Pts',(146.898700391862,4.6296253358803,126.092602535266));
#267317=CARTESIAN_POINT('Ctrl Pts',(146.62025276805,-1.46170993963237,124.362505370115));
#267318=CARTESIAN_POINT('Ctrl Pts',(146.341805144237,-6.20980518912327,
128.552158475246));
#267319=CARTESIAN_POINT('Ctrl Pts',(146.063357520424,-5.2513928356585,134.811475322978));
#267320=CARTESIAN_POINT('Ctrl Pts',(145.784909896611,0.532792988974217,
137.388449514872));
#267321=CARTESIAN_POINT('Ctrl Pts',(145.506462272798,5.82736808512415,133.914967660766));
#267322=CARTESIAN_POINT('Ctrl Pts',(145.228014648985,5.76687659380242,127.582989895561));
#267323=CARTESIAN_POINT('Ctrl Pts',(144.949567025172,0.406907240360106,
124.211294451169));
#267324=CARTESIAN_POINT('Ctrl Pts',(144.671119401359,-5.32698998844935,
126.898304724507));
#267325=CARTESIAN_POINT('Ctrl Pts',(144.392671777546,-6.16564365580234,
133.174789542127));
#267326=CARTESIAN_POINT('Ctrl Pts',(144.114224153734,-1.33837201191069,
137.272965979966));
#267327=CARTESIAN_POINT('Ctrl Pts',(143.83577652992,4.71879812781917,135.426810098699));
#267328=CARTESIAN_POINT('Ctrl Pts',(143.557328906108,6.43962331418753,129.332848963481));
#267329=CARTESIAN_POINT('Ctrl Pts',(143.278881282295,2.24274926790569,124.591135151027));
#267330=CARTESIAN_POINT('Ctrl Pts',(143.000433658482,-4.01510179118866,
125.559072009383));
#267331=CARTESIAN_POINT('Ctrl Pts',(142.721986034669,-6.58327045280769,
131.347172852065));
#267332=CARTESIAN_POINT('Ctrl Pts',(142.443538410856,-3.10173517893752,
136.636455769093));
#267333=CARTESIAN_POINT('Ctrl Pts',(142.165090787043,3.23014319618891,136.566328155556));
#267334=CARTESIAN_POINT('Ctrl Pts',(141.886643163231,6.5936777752854,131.201233862367));
#267335=CARTESIAN_POINT('Ctrl Pts',(141.608195539417,3.89794459796173,125.471432445543));
#267336=CARTESIAN_POINT('Ctrl Pts',(141.329747915605,-2.37980923970876,
124.642331490782));
#267337=CARTESIAN_POINT('Ctrl Pts',(141.051300291792,-6.47063464623165,
129.475834271677));
#267338=CARTESIAN_POINT('Ctrl Pts',(140.772852667979,-4.61526292094352,
135.530187862324));
#267339=CARTESIAN_POINT('Ctrl Pts',(140.494405044166,1.48130996056343,137.241737084533));
#267340=CARTESIAN_POINT('Ctrl Pts',(140.215957420353,6.21663135432719,133.037651816923));
#267341=CARTESIAN_POINT('Ctrl Pts',(139.93750979654,5.23917223278974,126.781281039444));
#267342=CARTESIAN_POINT('Ctrl Pts',(139.659062172727,-0.552830222889001,
124.221923855894));
#267343=CARTESIAN_POINT('Ctrl Pts',(139.380614548914,-5.83680871099059,
127.711504486408));
#267344=CARTESIAN_POINT('Ctrl Pts',(139.102166925101,-5.75704513764935,
134.043268807033));
#267345=CARTESIAN_POINT('Ctrl Pts',(138.823719301288,-0.386838330098996,
137.398634730999));
#267346=CARTESIAN_POINT('Ctrl Pts',(138.545271677476,5.33885400470937,134.694184892919));
#267347=CARTESIAN_POINT('Ctrl Pts',(138.266824053663,6.15840032670771,128.41517657427));
#267348=CARTESIAN_POINT('Ctrl Pts',(137.98837642985,1.31867760304303,124.331711673279));
#267349=CARTESIAN_POINT('Ctrl Pts',(137.709928806037,-4.7328454168358,126.196294945608));
#267350=CARTESIAN_POINT('Ctrl Pts',(137.431481182224,-6.43511471099507,
132.295465453942));
#267351=CARTESIAN_POINT('Ctrl Pts',(137.153033558411,-2.22382795858067,
137.024383462168));
#267352=CARTESIAN_POINT('Ctrl Pts',(136.874585934598,4.03104804773404,136.037404341212));
#267353=CARTESIAN_POINT('Ctrl Pts',(136.596138310785,6.5815878258261,130.241513686623));
#267354=CARTESIAN_POINT('Ctrl Pts',(136.317690686972,3.08396992042408,124.96285186497));
#267355=CARTESIAN_POINT('Ctrl Pts',(136.03924306316,-3.24766568154122,125.052251213384));
#267356=CARTESIAN_POINT('Ctrl Pts',(135.760795439346,-6.5948551794591,130.427558098075));
#267357=CARTESIAN_POINT('Ctrl Pts',(135.482347815534,-3.88169494404043,
136.149128090351));
#267358=CARTESIAN_POINT('Ctrl Pts',(135.203900191721,2.3985533136112,136.959117881544));
#267359=CARTESIAN_POINT('Ctrl Pts',(134.925452567908,6.47464825189767,132.113186423748));
#267360=CARTESIAN_POINT('Ctrl Pts',(134.647004944095,4.60085775084163,126.064507989766));
#267361=CARTESIAN_POINT('Ctrl Pts',(134.368557320282,-1.50089625884118,
124.371522566057));
#267362=CARTESIAN_POINT('Ctrl Pts',(134.090109696469,-6.22339992950755,
128.590001050074));
#267363=CARTESIAN_POINT('Ctrl Pts',(133.811662072656,-5.22690309494509,
134.843367799137));
#267364=CARTESIAN_POINT('Ctrl Pts',(133.533214448844,0.572862335460145,
137.385084264805));
#267365=CARTESIAN_POINT('Ctrl Pts',(133.25476682503,5.84619526545829,133.879437184883));
#267366=CARTESIAN_POINT('Ctrl Pts',(132.976319201218,5.7471603490167,127.547944965438));
#267367=CARTESIAN_POINT('Ctrl Pts',(132.697871577405,0.366765836220533,
124.208939645549));
#267368=CARTESIAN_POINT('Ctrl Pts',(132.419423953592,-5.35066856255522,
126.930803994717));
#267369=CARTESIAN_POINT('Ctrl Pts',(132.140976329779,-6.15109994703373,
133.212277646521));
#267370=CARTESIAN_POINT('Ctrl Pts',(131.862528705966,-1.29897097812634,
137.280993182001));
#267371=CARTESIAN_POINT('Ctrl Pts',(131.584081082153,4.74684886141891,135.397999791857));
#267372=CARTESIAN_POINT('Ctrl Pts',(131.30563345834,6.43054649377913,129.293676412286));
#267373=CARTESIAN_POINT('Ctrl Pts',(131.027185834528,2.20488604801711,124.577598016342));
#267374=CARTESIAN_POINT('Ctrl Pts',(130.748738210715,-4.04695696120101,
125.583610256657));
#267375=CARTESIAN_POINT('Ctrl Pts',(130.470290586902,-6.57984422791396,
131.387237030814));
#267376=CARTESIAN_POINT('Ctrl Pts',(130.191842963089,-3.06617609243459,
136.65522885629));
#267377=CARTESIAN_POINT('Ctrl Pts',(129.913395339276,3.26515808096253,136.546558601182));
#267378=CARTESIAN_POINT('Ctrl Pts',(129.634947715463,6.59597148979528,131.161088921098));
#267379=CARTESIAN_POINT('Ctrl Pts',(129.35650009165,3.86540933062731,125.447803357213));
#267380=CARTESIAN_POINT('Ctrl Pts',(129.078052467837,-2.41727516764341,
124.656932233223));
#267381=CARTESIAN_POINT('Ctrl Pts',(128.799604844024,-6.47860187730669,
129.515247475871));
#267382=CARTESIAN_POINT('Ctrl Pts',(128.521157220212,-4.58640995902212,
135.558194719059));
#267383=CARTESIAN_POINT('Ctrl Pts',(128.242709596398,1.52046865302106,137.232600660681));
#267384=CARTESIAN_POINT('Ctrl Pts',(127.964261972586,6.23011085196111,132.999768039666));
#267385=CARTESIAN_POINT('Ctrl Pts',(127.685814348773,5.2145855357842,126.749463249355));
#267386=CARTESIAN_POINT('Ctrl Pts',(127.40736672496,-0.592889141112855,
124.225411047681));
#267387=CARTESIAN_POINT('Ctrl Pts',(127.128919101147,-5.85552766157182,
127.747092101177));
#267388=CARTESIAN_POINT('Ctrl Pts',(126.850471477334,-5.7372223194756,134.078253565364));
#267389=CARTESIAN_POINT('Ctrl Pts',(126.572023853521,-0.346689944673359,
137.400867349086));
#267390=CARTESIAN_POINT('Ctrl Pts',(126.293576229708,5.36243355253846,134.66161370381));
#267391=CARTESIAN_POINT('Ctrl Pts',(126.015128605896,6.14374258441013,128.377732909565));
#267392=CARTESIAN_POINT('Ctrl Pts',(125.736680982083,1.27925231971985,124.323804431618));
#267393=CARTESIAN_POINT('Ctrl Pts',(125.45823335827,-4.76080833184274,126.225190495787));
#267394=CARTESIAN_POINT('Ctrl Pts',(125.179785734457,-6.42591870485886,
132.334610196974));
#267395=CARTESIAN_POINT('Ctrl Pts',(124.901338110644,-2.1859237116904,137.037805291532));
#267396=CARTESIAN_POINT('Ctrl Pts',(124.622890486831,4.06282838421153,136.012769251418));
#267397=CARTESIAN_POINT('Ctrl Pts',(124.344442863018,6.5780396752237,130.201460121699));
#267398=CARTESIAN_POINT('Ctrl Pts',(124.065995239205,3.04835385980878,124.944187094356));
#267399=CARTESIAN_POINT('Ctrl Pts',(123.787547615392,-3.28262023240536,
125.07212724945));
#267400=CARTESIAN_POINT('Ctrl Pts',(123.509099991579,-6.59702669595264,
130.467709834674));
#267401=CARTESIAN_POINT('Ctrl Pts',(123.230652367767,-3.84908790859021,
136.17265804307));
#267402=CARTESIAN_POINT('Ctrl Pts',(122.952204743954,2.43597462836867,136.944403173336));
#267403=CARTESIAN_POINT('Ctrl Pts',(122.673757120141,6.48249548583303,132.073749152604));
#267404=CARTESIAN_POINT('Ctrl Pts',(122.395309496328,4.57191967932717,126.036589081248));
#267405=CARTESIAN_POINT('Ctrl Pts',(122.116861872515,-1.54002696178715,
124.380778133181));
#267406=CARTESIAN_POINT('Ctrl Pts',(121.838414248702,-6.23676405951882,
128.627925678811));
#267407=CARTESIAN_POINT('Ctrl Pts',(121.559966624889,-5.20221966941523,
134.8751106084));
#267408=CARTESIAN_POINT('Ctrl Pts',(121.281519001076,0.612910454321425,
137.381475163605));
#267409=CARTESIAN_POINT('Ctrl Pts',(121.003071377263,5.86480581287692,133.843792760907));
#267410=CARTESIAN_POINT('Ctrl Pts',(120.724623753451,5.72723114109079,127.513020702994));
#267411=CARTESIAN_POINT('Ctrl Pts',(120.446176129638,0.326610841437887,
124.206829235678));
#267412=CARTESIAN_POINT('Ctrl Pts',(120.167728505825,-5.3741488656698,126.963446800991));
#267413=CARTESIAN_POINT('Ctrl Pts',(119.889280882012,-6.13632830699453,
133.249676524665));
#267414=CARTESIAN_POINT('Ctrl Pts',(119.610833258199,-1.25952181049465,
137.288780390037));
#267415=CARTESIAN_POINT('Ctrl Pts',(119.332385634386,4.77472369878856,135.369019266025));
#267416=CARTESIAN_POINT('Ctrl Pts',(119.053938010573,6.42123138710552,129.254559840052));
#267417=CARTESIAN_POINT('Ctrl Pts',(118.77549038676,2.16694112526505,124.564291616636));
#267418=CARTESIAN_POINT('Ctrl Pts',(118.497042762948,-4.07866216973492,
125.608341960757));
#267419=CARTESIAN_POINT('Ctrl Pts',(118.218595139134,-6.57617418447253,
131.427279610862));
#267420=CARTESIAN_POINT('Ctrl Pts',(117.940147515322,-3.03050338764912,
136.673785137412));
#267421=CARTESIAN_POINT('Ctrl Pts',(117.661699891509,3.30005197410286,136.526576267552));
#267422=CARTESIAN_POINT('Ctrl Pts',(117.383252267696,6.59802078815589,131.120930761129));
#267423=CARTESIAN_POINT('Ctrl Pts',(117.104804643883,3.83273082912851,125.424372758082));
#267424=CARTESIAN_POINT('Ctrl Pts',(116.82635702007,-2.45465152255762,124.671760770883));
#267425=CARTESIAN_POINT('Ctrl Pts',(116.547909396257,-6.48632904140672,
129.554708448625));
#267426=CARTESIAN_POINT('Ctrl Pts',(116.269461772444,-4.55738704599302,
135.586025420722));
#267427=CARTESIAN_POINT('Ctrl Pts',(115.991014148631,1.55957100395386,137.223226036031));
#267428=CARTESIAN_POINT('Ctrl Pts',(115.712566524818,6.24335949054626,132.961802910777));
#267429=CARTESIAN_POINT('Ctrl Pts',(115.434118901006,5.18980561039392,126.717795714978));
#267430=CARTESIAN_POINT('Ctrl Pts',(115.155671277193,-0.632926089611396,
124.229142024863));
#267431=CARTESIAN_POINT('Ctrl Pts',(114.87722365338,-5.87402963342224,127.782793004156));
#267432=CARTESIAN_POINT('Ctrl Pts',(114.598776029567,-5.71718690641897,
134.113117008387));
#267433=CARTESIAN_POINT('Ctrl Pts',(114.320328405754,-0.306528712524212,
137.40285553119));
#267434=CARTESIAN_POINT('Ctrl Pts',(114.041880781941,5.38581439342023,134.628899582769));
#267435=CARTESIAN_POINT('Ctrl Pts',(113.763433158128,6.12885718347172,128.340379164441));
#267436=CARTESIAN_POINT('Ctrl Pts',(113.484985534315,1.23977963323159,124.316137329349));
#267437=CARTESIAN_POINT('Ctrl Pts',(113.206537910502,-4.78859483334625,
126.254255728798));
#267438=CARTESIAN_POINT('Ctrl Pts',(112.92809028669,-6.41648458394181,132.373698236044));
#267439=CARTESIAN_POINT('Ctrl Pts',(112.649642662877,-2.14793846459313,
137.050996138312));
#267440=CARTESIAN_POINT('Ctrl Pts',(112.371195039064,4.09445817108915,135.987941162125));
#267441=CARTESIAN_POINT('Ctrl Pts',(112.092747415251,6.57424777294209,130.161428897475));
#267442=CARTESIAN_POINT('Ctrl Pts',(111.814299791438,3.01262484132005,124.925739474628));
#267443=CARTESIAN_POINT('Ctrl Pts',(111.535852167625,-3.31745314456969,
125.092215695531));
#267444=CARTESIAN_POINT('Ctrl Pts',(111.257404543812,-6.59895375719588,
130.507874045991));
#267445=CARTESIAN_POINT('Ctrl Pts',(110.978956919999,-3.816338243772,136.195989071554));
#267446=CARTESIAN_POINT('Ctrl Pts',(110.700509296186,2.47330567719032,136.929460943594));
#267447=CARTESIAN_POINT('Ctrl Pts',(110.422061672374,6.49010250851429,132.0342648438));
#267448=CARTESIAN_POINT('Ctrl Pts',(110.143614048561,4.54281219364771,126.008846844259));
#267449=CARTESIAN_POINT('Ctrl Pts',(109.865166424748,-1.57910059846782,
124.390271728514));
#267450=CARTESIAN_POINT('Ctrl Pts',(109.586718800935,-6.24989708394428,
128.665930956147));
#267451=CARTESIAN_POINT('Ctrl Pts',(109.308271177122,-5.17734347372243,
134.906702574525));
#267452=CARTESIAN_POINT('Ctrl Pts',(109.029823553309,0.652935861560398,
137.377622345005));
#267453=CARTESIAN_POINT('Ctrl Pts',(108.751375929496,5.88319903775945,133.808035709655));
#267454=CARTESIAN_POINT('Ctrl Pts',(108.472928305683,5.70708970850866,127.478218402361));
#267455=CARTESIAN_POINT('Ctrl Pts',(108.19448068187,0.286443743970404,124.204963299759));
#267456=CARTESIAN_POINT('Ctrl Pts',(107.916033058058,-5.39743002772183,
126.996231933739));
#267457=CARTESIAN_POINT('Ctrl Pts',(107.637585434244,-6.12132928305326,
133.286984790727));
#267458=CARTESIAN_POINT('Ctrl Pts',(107.359137810432,-1.22002597081922,
137.296327315513));
#267459=CARTESIAN_POINT('Ctrl Pts',(107.080690186619,4.80242160701559,135.339869595089));
#267460=CARTESIAN_POINT('Ctrl Pts',(106.802242562806,6.41167833934146,129.215500696253));
#267461=CARTESIAN_POINT('Ctrl Pts',(106.523794938993,2.12891590571267,124.551216444981));
#267462=CARTESIAN_POINT('Ctrl Pts',(106.24534731518,-4.11021624194206,125.633266205238));
#267463=CARTESIAN_POINT('Ctrl Pts',(105.966899691367,-6.57226045847839,
131.467299108419));
#267464=CARTESIAN_POINT('Ctrl Pts',(105.688452067554,-2.99471838644612,
136.692123924851));
#267465=CARTESIAN_POINT('Ctrl Pts',(105.410004443742,3.33482358260376,136.506381895117));
#267466=CARTESIAN_POINT('Ctrl Pts',(105.131556819929,6.59982559442975,131.080760870538));
#267467=CARTESIAN_POINT('Ctrl Pts',(104.853109196116,3.79991030437941,125.401141516381));
#267468=CARTESIAN_POINT('Ctrl Pts',(104.574661572303,-2.49193691945696,
124.686816554284));
#267469=CARTESIAN_POINT('Ctrl Pts',(104.29621394849,-6.49381585219884,129.594215727701));
#267470=CARTESIAN_POINT('Ctrl Pts',(104.017766324677,-4.52819525731082,
135.613678936038));
#267471=CARTESIAN_POINT('Ctrl Pts',(103.739318700864,1.59861556440955,137.213613557961));
#267472=CARTESIAN_POINT('Ctrl Pts',(103.460871077051,6.25637677914949,132.923757837073));
#267473=CARTESIAN_POINT('Ctrl Pts',(103.182423453238,5.16483337484823,126.686279609768));
#267474=CARTESIAN_POINT('Ctrl Pts',(102.903975829425,-0.672939584800916,
124.233116649188));
#267475=CARTESIAN_POINT('Ctrl Pts',(102.625528205613,-5.89231394094447,
127.818605872432));
#267476=CARTESIAN_POINT('Ctrl Pts',(102.347080581799,-5.69693964089892,
134.147857844226));
#267477=CARTESIAN_POINT('Ctrl Pts',(102.068632957987,-0.266356121840884,
137.40459920364));
#267478=CARTESIAN_POINT('Ctrl Pts',(101.790185334174,5.40899566096888,134.59604374203));
#267479=CARTESIAN_POINT('Ctrl Pts',(101.511737710361,6.11374467547657,128.303116723058));
#267480=CARTESIAN_POINT('Ctrl Pts',(101.233290086548,1.20026100625305,124.308710650579));
#267481=CARTESIAN_POINT('Ctrl Pts',(100.954842462735,-4.81620389170723,
126.28348956762));
#267482=CARTESIAN_POINT('Ctrl Pts',(100.676394838922,-6.40681269782886,
132.412728122731));
#267483=CARTESIAN_POINT('Ctrl Pts',(100.397947215109,-2.10987362484612,
137.063955513716));
#267484=CARTESIAN_POINT('Ctrl Pts',(100.119499591297,4.12593623631335,135.962920993349));
#267485=CARTESIAN_POINT('Ctrl Pts',(99.8410519674839,6.5702122594916,130.121421497322));
#267486=CARTESIAN_POINT('Ctrl Pts',(99.5626043436712,2.97678418891005,124.907509689368));
#267487=CARTESIAN_POINT('Ctrl Pts',(99.2841567198582,-3.35216312728773,
125.112515807244));
#267488=CARTESIAN_POINT('Ctrl Pts',(99.0057090960455,-6.6006362917809,130.548049243728));
#267489=CARTESIAN_POINT('Ctrl Pts',(98.7272614722323,-3.78344716313679,
136.219120311263));
#267490=CARTESIAN_POINT('Ctrl Pts',(98.4488138484198,2.51054507676055,136.914291746006));
#267491=CARTESIAN_POINT('Ctrl Pts',(98.1703662246066,6.49746903806041,131.994734960442));
#267492=CARTESIAN_POINT('Ctrl Pts',(97.8919186007939,4.51353637239165,125.981282306795));
#267493=CARTESIAN_POINT('Ctrl Pts',(97.6134709769809,-1.61811572099509,
124.400003000271));
#267494=CARTESIAN_POINT('Ctrl Pts',(97.335023353168,-6.26279851613479,128.704015473778));
#267495=CARTESIAN_POINT('Ctrl Pts',(97.0565757293552,-5.15227542966332,
134.938142526861));
#267496=CARTESIAN_POINT('Ctrl Pts',(96.7781281055422,0.692937074020952,
137.373525951775));
#267497=CARTESIAN_POINT('Ctrl Pts',(96.4996804817294,5.90137425853808,133.772167356118));
#267498=CARTESIAN_POINT('Ctrl Pts',(96.2212328579164,5.6867367976186,127.443539353151));
#267499=CARTESIAN_POINT('Ctrl Pts',(95.9427852341037,0.246266032224636,
124.203341906934));
#267500=CARTESIAN_POINT('Ctrl Pts',(95.6643376102905,-5.42051118601915,
127.029158178097));
#267501=CARTESIAN_POINT('Ctrl Pts',(95.3858899864779,-6.10610343100435,
133.324201062238));
#267502=CARTESIAN_POINT('Ctrl Pts',(95.1074423626648,-1.18048492263276,
137.303633678775));
#267503=CARTESIAN_POINT('Ctrl Pts',(94.828994738852,4.82994155974394,135.3105518592));
#267504=CARTESIAN_POINT('Ctrl Pts',(94.5505471150391,6.40188770447863,129.176500428244));
#267505=CARTESIAN_POINT('Ctrl Pts',(94.2720994912261,2.09081179839861,124.538372985881));
#267506=CARTESIAN_POINT('Ctrl Pts',(93.9936518674133,-4.14161800857485,
125.658382066524));
#267507=CARTESIAN_POINT('Ctrl Pts',(93.7152042436005,-6.56810319495607,
131.507294040545));
#267508=CARTESIAN_POINT('Ctrl Pts',(93.4367566197874,-2.95882241485189,
136.710244539055));
#267509=CARTESIAN_POINT('Ctrl Pts',(93.1583089959747,3.36947161799043,136.485976232185));
#267510=CARTESIAN_POINT('Ctrl Pts',(92.8798613721617,6.60138584173913,131.040580737834));
#267511=CARTESIAN_POINT('Ctrl Pts',(92.6014137483489,3.76694897255651,125.37811049295));
#267512=CARTESIAN_POINT('Ctrl Pts',(92.3229661245359,-2.5291299767175,124.702099025532));
#267513=CARTESIAN_POINT('Ctrl Pts',(92.044518500723,-6.50106203225643,129.633767849141));
#267514=CARTESIAN_POINT('Ctrl Pts',(91.7660708769102,-4.49883567468812,
135.641154240296));
#267515=CARTESIAN_POINT('Ctrl Pts',(91.4876232530973,1.63760088757763,137.203763582666));
#267516=CARTESIAN_POINT('Ctrl Pts',(91.2091756292845,6.26916223541028,132.885634228324));
#267517=CARTESIAN_POINT('Ctrl Pts',(90.9307280054714,5.13966975450256,126.654916101563));
#267518=CARTESIAN_POINT('Ctrl Pts',(90.6522803816587,-0.71292814396669,
124.237334773374));
#267519=CARTESIAN_POINT('Ctrl Pts',(90.3738327578456,-5.91037990660673,
127.85452937895));
#267520=CARTESIAN_POINT('Ctrl Pts',(90.0953851340328,-5.67648127318543,
134.182474785545));
#267521=CARTESIAN_POINT('Ctrl Pts',(89.8169375102199,-0.226173661233629,
137.406098301819));
#267522=CARTESIAN_POINT('Ctrl Pts',(89.5384898864071,5.43197649619419,134.563047399079));
#267523=CARTESIAN_POINT('Ctrl Pts',(89.260042262594,6.09840562042418,128.265946966186));
#267524=CARTESIAN_POINT('Ctrl Pts',(88.9815946387814,1.1606979031614,124.301524670509));
#267525=CARTESIAN_POINT('Ctrl Pts',(88.7031470149683,-4.84363448386183,
126.312890928981));
#267526=CARTESIAN_POINT('Ctrl Pts',(88.4246993911556,-6.39690340491527,
132.45169841077));
#267527=CARTESIAN_POINT('Ctrl Pts',(88.1462517673426,-2.07173060295614,
137.076682937528));
#267528=CARTESIAN_POINT('Ctrl Pts',(87.8678041435297,4.15726141345302,135.937709672222));
#267529=CARTESIAN_POINT('Ctrl Pts',(87.5893565197169,6.5659332844097,130.081439403729));
#267530=CARTESIAN_POINT('Ctrl Pts',(87.3109088959039,2.94083323066708,124.889498414087));
#267531=CARTESIAN_POINT('Ctrl Pts',(87.032461272091,-3.38674889436835,125.133026832359));
#267532=CARTESIAN_POINT('Ctrl Pts',(86.7540136482781,-6.60207423736065,
130.588233939178));
#267533=CARTESIAN_POINT('Ctrl Pts',(86.4755660244652,-3.75041588547566,
136.242050905059));
#267534=CARTESIAN_POINT('Ctrl Pts',(86.1971184006524,2.54769144715974,136.898896142674));
#267535=CARTESIAN_POINT('Ctrl Pts',(85.9186707768394,6.50459480150186,131.955160967326));
#267536=CARTESIAN_POINT('Ctrl Pts',(85.6402231530266,4.48409330038545,125.953896490271));
#267537=CARTESIAN_POINT('Ctrl Pts',(85.3617755292137,-1.65707088364924,
124.409971587854));
#267538=CARTESIAN_POINT('Ctrl Pts',(85.0833279054008,-6.27546787802325,
128.742177820471));
#267539=CARTESIAN_POINT('Ctrl Pts',(84.8048802815879,-5.12701646614329,
134.969429300388));
#267540=CARTESIAN_POINT('Ctrl Pts',(84.526432657775,0.732912609443495,137.369186135708));
#267541=CARTESIAN_POINT('Ctrl Pts',(84.2479850339622,5.91933080172332,133.73618902941));
#267542=CARTESIAN_POINT('Ctrl Pts',(83.9695374101491,5.6661731626052,127.408984840408));
#267543=CARTESIAN_POINT('Ctrl Pts',(83.6910897863363,0.206079195000604,
124.201965117285));
#267544=CARTESIAN_POINT('Ctrl Pts',(83.4126421625234,-5.44339148528112,
127.062224313968));
#267545=CARTESIAN_POINT('Ctrl Pts',(83.1341945387106,-6.09065131504733,
133.361323960135));
#267546=CARTESIAN_POINT('Ctrl Pts',(82.8557469148977,-1.14090013114324,
137.310699209084));
#267547=CARTESIAN_POINT('Ctrl Pts',(82.5772992910847,4.85728253721157,135.281067144739));
#267548=CARTESIAN_POINT('Ctrl Pts',(82.2988516672719,6.39185984531258,129.137560481192));
#267549=CARTESIAN_POINT('Ctrl Pts',(82.0204040434589,2.05263021528453,124.52576171526));
#267550=CARTESIAN_POINT('Ctrl Pts',(81.7419564196462,-4.17286630602932,
125.683688613938));
#267551=CARTESIAN_POINT('Ctrl Pts',(81.4635087958331,-6.56370254795435,
131.547262925216));
#267552=CARTESIAN_POINT('Ctrl Pts',(81.1850611720204,-2.92281680300497,
136.728146308557));
#267553=CARTESIAN_POINT('Ctrl Pts',(80.9066135482074,3.40399479636718,136.465360034899));
#267554=CARTESIAN_POINT('Ctrl Pts',(80.6281659243945,6.60270147226842,131.000391851905));
#267555=CARTESIAN_POINT('Ctrl Pts',(80.3497183005816,3.73384805505426,125.355280541214));
#267556=CARTESIAN_POINT('Ctrl Pts',(80.0712706767688,-2.56622931613655,
124.717607618327));
#267557=CARTESIAN_POINT('Ctrl Pts',(79.7928230529558,-6.50806731306963,
129.673363347327));
#267558=CARTESIAN_POINT('Ctrl Pts',(79.514375429143,-4.46930938605503,135.668450315387));
#267559=CARTESIAN_POINT('Ctrl Pts',(79.23592780533,1.67652552884245,137.193676475141));
#267560=CARTESIAN_POINT('Ctrl Pts',(78.9574801815173,6.28171538555901,132.847433497217));
#267561=CARTESIAN_POINT('Ctrl Pts',(78.6790325577042,5.11431568180404,126.62370635255));
#267562=CARTESIAN_POINT('Ctrl Pts',(78.4005849338915,-0.752890285318027,
124.241796241119));
#267563=CARTESIAN_POINT('Ctrl Pts',(78.1221373100785,-5.92822686096799,
127.890562192549));
#267564=CARTESIAN_POINT('Ctrl Pts',(77.8436896862655,-5.65581256137084,
134.216966549603));
#267565=CARTESIAN_POINT('Ctrl Pts',(77.5652420624528,-0.185982819678218,
137.407352770183));
#267566=CARTESIAN_POINT('Ctrl Pts',(77.2867944386398,5.45475604753291,134.529911776607));
#267567=CARTESIAN_POINT('Ctrl Pts',(77.008346814827,6.08284058670873,128.228871271165));
#267568=CARTESIAN_POINT('Ctrl Pts',(76.729899191014,1.12109178998211,124.294579655415));
#267569=CARTESIAN_POINT('Ctrl Pts',(76.4514515672013,-4.8708855933594,126.342458723402));
#267570=CARTESIAN_POINT('Ctrl Pts',(76.1730039433881,-6.38675707239351,
132.4906076561));
#267571=CARTESIAN_POINT('Ctrl Pts',(75.8945563195755,-2.03351081232684,
137.089177938131));
#267572=CARTESIAN_POINT('Ctrl Pts',(75.6161086957625,4.18843254174224,135.912308132958));
#267573=CARTESIAN_POINT('Ctrl Pts',(75.3376610719495,6.56141100625526,130.041484098248));
#267574=CARTESIAN_POINT('Ctrl Pts',(75.0592134481368,2.90477329876725,124.871706316201));
#267575=CARTESIAN_POINT('Ctrl Pts',(74.7807658243238,-3.42120916422307,
125.153748010832));
#267576=CARTESIAN_POINT('Ctrl Pts',(74.5023182005109,-6.60326754065171,
130.628426643279));
#267577=CARTESIAN_POINT('Ctrl Pts',(74.223870576698,-3.71724563477466,136.264780003243));
#267578=CARTESIAN_POINT('Ctrl Pts',(73.9454229528852,2.58474341191554,136.883274704086));
#267579=CARTESIAN_POINT('Ctrl Pts',(73.6669753290721,6.51147953479087,131.915544330879));
#267580=CARTESIAN_POINT('Ctrl Pts',(73.3885277052595,4.45448406865298,125.926690409479));
#267581=CARTESIAN_POINT('Ctrl Pts',(73.1100800814464,-1.6959646429323,124.420177121874));
#267582=CARTESIAN_POINT('Ctrl Pts',(72.8316324576336,-6.28790470014163,
128.780416582107));
#267583=CARTESIAN_POINT('Ctrl Pts',(72.5531848338207,-5.1015675191428,135.000561735763));
#267584=CARTESIAN_POINT('Ctrl Pts',(72.2747372100078,0.772860986519783,
137.364603057617));
#267585=CARTESIAN_POINT('Ctrl Pts',(71.996289586195,5.93706800192887,133.700102062723));
#267586=CARTESIAN_POINT('Ctrl Pts',(71.7178419623819,5.64539956546153,127.374556144564));
#267587=CARTESIAN_POINT('Ctrl Pts',(71.4393943385692,0.165884721436248,
124.20083298183));
#267588=CARTESIAN_POINT('Ctrl Pts',(71.1609467147562,-5.46607007766984,
127.095429116077));
#267589=CARTESIAN_POINT('Ctrl Pts',(70.8824990909434,-6.07497350776591,
133.398352108815));
#267590=CARTESIAN_POINT('Ctrl Pts',(70.6040514671303,-1.10127306317963,
137.317523644624));
#267591=CARTESIAN_POINT('Ctrl Pts',(70.3256038433176,4.88444352628841,135.251416544269));
#267592=CARTESIAN_POINT('Ctrl Pts',(70.0471562195047,6.38159513342946,129.098682298033));
#267593=CARTESIAN_POINT('Ctrl Pts',(69.7687085956917,2.01437257120279,124.513383100429));
#267594=CARTESIAN_POINT('Ctrl Pts',(69.4902609718789,-4.20395997638847,
125.709184909736));
#267595=CARTESIAN_POINT('Ctrl Pts',(69.211813348066,-6.5590586805409,131.587204281367));
#267596=CARTESIAN_POINT('Ctrl Pts',(68.9333657242531,-2.88670288510633,
136.745828570004));
#267597=CARTESIAN_POINT('Ctrl Pts',(68.6549181004402,3.43839183846502,136.444534067195));
#267598=CARTESIAN_POINT('Ctrl Pts',(68.3764704766273,6.60377243726651,130.960195701968));
#267599=CARTESIAN_POINT('Ctrl Pts',(68.0980228528144,3.70060877843901,125.332652507142));
#267600=CARTESIAN_POINT('Ctrl Pts',(67.8195752290015,-2.6032335629848,124.733341757993));
#267601=CARTESIAN_POINT('Ctrl Pts',(67.5411276051886,-6.51483143505509,
129.713000755032));
#267602=CARTESIAN_POINT('Ctrl Pts',(67.2626799813758,-4.43961748551916,
135.695566149845));
#267603=CARTESIAN_POINT('Ctrl Pts',(66.9842323575627,1.71538804583728,137.183352609169));
#267604=CARTESIAN_POINT('Ctrl Pts',(66.7057847337499,6.29403576443417,132.809157059292));
#267605=CARTESIAN_POINT('Ctrl Pts',(66.4273371099371,5.08877209625689,126.592651519219));
#267606=CARTESIAN_POINT('Ctrl Pts',(66.1488894861241,-0.792824528042931,
124.246500887099));
#267607=CARTESIAN_POINT('Ctrl Pts',(65.8704418623113,-5.94585414270274,
127.92670297802));
#267608=CARTESIAN_POINT('Ctrl Pts',(65.5919942384984,-5.63493427134196,
134.251331858291));
#267609=CARTESIAN_POINT('Ctrl Pts',(65.3135466146855,-0.145785086460763,
137.408362562243));
#267610=CARTESIAN_POINT('Ctrl Pts',(65.0350989908726,5.47733347088038,134.496638102466));
#267611=CARTESIAN_POINT('Ctrl Pts',(64.7566513670597,6.06705015109826,128.191891011849));
#267612=CARTESIAN_POINT('Ctrl Pts',(64.4782037432468,1.0814441343344,124.28787586265));
#267613=CARTESIAN_POINT('Ctrl Pts',(64.199756119434,-4.89795621039988,126.37219185524));
#267614=CARTESIAN_POINT('Ctrl Pts',(63.921308495621,-6.37637407623982,132.529454416925));
#267615=CARTESIAN_POINT('Ctrl Pts',(63.6428608718081,-1.99521566920641,
137.101440052517));
#267616=CARTESIAN_POINT('Ctrl Pts',(63.3644132479953,4.21944846612332,135.886717316821));
#267617=CARTESIAN_POINT('Ctrl Pts',(63.0859656241823,6.556645592603,130.001557061437));
#267618=CARTESIAN_POINT('Ctrl Pts',(62.8075180003696,2.86860572942485,124.854134055001));
#267619=CARTESIAN_POINT('Ctrl Pts',(62.5290703765565,-3.4555426599142,125.174678574835));
#267620=CARTESIAN_POINT('Ctrl Pts',(62.2506227527437,-6.60421615743575,
130.66862586668));
#267621=CARTESIAN_POINT('Ctrl Pts',(61.9721751289308,-3.68393764016947,
136.287306763578));
#267622=CARTESIAN_POINT('Ctrl Pts',(61.6937275051179,2.62169959805353,136.867428009101));
#267623=CARTESIAN_POINT('Ctrl Pts',(61.415279881305,6.51812298281107,131.875886519111));
#267624=CARTESIAN_POINT('Ctrl Pts',(61.1368322574921,4.42470977437533,125.899665072552));
#267625=CARTESIAN_POINT('Ctrl Pts',(60.8583846336791,-1.73479555762186,
124.430619224162));
#267626=CARTESIAN_POINT('Ctrl Pts',(60.5799370098664,-6.30010852163892,
128.818730341733));
#267627=CARTESIAN_POINT('Ctrl Pts',(60.3014893860534,-5.07592953168175,
135.031538679362));
#267628=CARTESIAN_POINT('Ctrl Pts',(60.0230417622406,0.81278072494776,137.35977688733));
#267629=CARTESIAN_POINT('Ctrl Pts',(59.7445941384276,5.95458520189618,133.663907793273));
#267630=CARTESIAN_POINT('Ctrl Pts',(59.4661465146148,5.62441677596096,127.340254541386));
#267631=CARTESIAN_POINT('Ctrl Pts',(59.1876988908018,0.125684100952275,
124.199945542519));
#267632=CARTESIAN_POINT('Ctrl Pts',(58.909251266989,-5.48854612282181,127.128771354006));
#267633=CARTESIAN_POINT('Ctrl Pts',(58.6308036431761,-6.05907059010694,
133.435284136186));
#267634=CARTESIAN_POINT('Ctrl Pts',(58.3523560193632,-1.06160518713815,
137.324106732513));
#267635=CARTESIAN_POINT('Ctrl Pts',(58.0739083955504,4.91142352051418,135.221601156507));
#267636=CARTESIAN_POINT('Ctrl Pts',(57.7954607717374,6.37109394919177,129.059867319411));
#267637=CARTESIAN_POINT('Ctrl Pts',(57.5170131479246,1.97604028380464,124.501237600083));
#267638=CARTESIAN_POINT('Ctrl Pts',(57.2385655241116,-4.23489786746425,
125.734870009144));
#267639=CARTESIAN_POINT('Ctrl Pts',(56.9601179002987,-6.554171764796,131.627116628959));
#267640=CARTESIAN_POINT('Ctrl Pts',(56.6816702764859,-2.85048199937133,
136.76329066817));
#267641=CARTESIAN_POINT('Ctrl Pts',(56.4032226526729,3.47266146968847,136.423499100792));
#267642=CARTESIAN_POINT('Ctrl Pts',(56.1247750288601,6.60459869704857,130.919993777505));
#267643=CARTESIAN_POINT('Ctrl Pts',(55.8463274050471,3.66723237440476,125.310227229228));
#267644=CARTESIAN_POINT('Ctrl Pts',(55.5678797812343,-2.6401413460556,124.749300861495));
#267645=CARTESIAN_POINT('Ctrl Pts',(55.2894321574214,-6.5213541475661,129.752678603477));
#267646=CARTESIAN_POINT('Ctrl Pts',(55.0109845336085,-4.40976107332459,
135.722500738884));
#267647=CARTESIAN_POINT('Ctrl Pts',(54.7325369097956,1.75418699849736,137.172792367301));
#267648=CARTESIAN_POINT('Ctrl Pts',(54.4540892859827,6.30612291549916,132.770806332897));
#267649=CARTESIAN_POINT('Ctrl Pts',(54.1756416621698,5.06303994438864,126.561752752318));
#267650=CARTESIAN_POINT('Ctrl Pts',(53.897194038357,-0.832729392363195,
124.251448536985));
#267651=CARTESIAN_POINT('Ctrl Pts',(53.618746414544,-5.96326109862574,127.962950396153));
#267652=CARTESIAN_POINT('Ctrl Pts',(53.3402987907312,-5.61384717675129,
134.285569438194));
#267653=CARTESIAN_POINT('Ctrl Pts',(53.0618511669183,-0.105581951123662,
137.409127640582));
#267654=CARTESIAN_POINT('Ctrl Pts',(52.7834035431054,5.49970792962155,134.463227609627));
#267655=CARTESIAN_POINT('Ctrl Pts',(52.5049559192925,6.05103489871361,128.155007558556));
#267656=CARTESIAN_POINT('Ctrl Pts',(52.2265082954796,1.04175640537643,124.281413540623));
#267657=CARTESIAN_POINT('Ctrl Pts',(51.9480606716666,-4.9248453318719,126.402089222721));
#267658=CARTESIAN_POINT('Ctrl Pts',(51.6696130478539,-6.36575480119974,
132.568237253767));
#267659=CARTESIAN_POINT('Ctrl Pts',(51.3911654240409,-1.95684659263562,
137.113468826308));
#267660=CARTESIAN_POINT('Ctrl Pts',(51.112717800228,4.25030803728985,135.860938172086));
#267661=CARTESIAN_POINT('Ctrl Pts',(50.8342701764151,6.55163722003711,129.961659772806));
#267662=CARTESIAN_POINT('Ctrl Pts',(50.5558225526023,2.83233186284197,124.836782281636));
#267663=CARTESIAN_POINT('Ctrl Pts',(50.2773749287893,-3.48974810920128,
125.195817748775));
#267664=CARTESIAN_POINT('Ctrl Pts',(49.9989273049765,-6.60492005256131,
130.708830119782));
#267665=CARTESIAN_POINT('Ctrl Pts',(49.7204796811635,-3.65049313590031,
136.309630351328));
#267666=CARTESIAN_POINT('Ctrl Pts',(49.4420320573507,2.65855863614892,136.851356644924));
#267667=CARTESIAN_POINT('Ctrl Pts',(49.1635844335378,6.52452489938715,131.836189001557));
#267668=CARTESIAN_POINT('Ctrl Pts',(48.8851368097249,4.39477152084969,125.87282148092));
#267669=CARTESIAN_POINT('Ctrl Pts',(48.606689185912,-1.77356218882415,124.441297507781));
#267670=CARTESIAN_POINT('Ctrl Pts',(48.3282415620992,-6.31207889029818,
128.857117679619));
#267671=CARTESIAN_POINT('Ctrl Pts',(48.0497939382862,-5.05010345378512,
135.062358983324));
#267672=CARTESIAN_POINT('Ctrl Pts',(47.7713463144734,0.852670345487299,
137.354707803682));
#267673=CARTESIAN_POINT('Ctrl Pts',(47.4928986906604,5.97188175251911,133.627607562248));
#267674=CARTESIAN_POINT('Ctrl Pts',(47.2144510668476,5.60322557162828,127.306081301933));
#267675=CARTESIAN_POINT('Ctrl Pts',(46.9360034430346,0.0854788231980546,
124.199302832238));
#267676=CARTESIAN_POINT('Ctrl Pts',(46.6575558192218,-5.5108187878785,127.162249792247));
#267677=CARTESIAN_POINT('Ctrl Pts',(46.3791081954089,-6.04294315135938,
133.47211867372));
#267678=CARTESIAN_POINT('Ctrl Pts',(46.100660571596,-1.02189797292572,137.330448228811));
#267679=CARTESIAN_POINT('Ctrl Pts',(45.822212947783,4.93822152013526,135.191622086273));
#267680=CARTESIAN_POINT('Ctrl Pts',(45.5437653239702,6.36035668172477,129.02111698363));
#267681=CARTESIAN_POINT('Ctrl Pts',(45.2653177001572,1.9376347735074,124.489325664279));
#267682=CARTESIAN_POINT('Ctrl Pts',(44.9868700763445,-4.26567883284234,
125.76074296039));
#267683=CARTESIAN_POINT('Ctrl Pts',(44.7084224525315,-6.54904198180601,
131.666998489025));
#267684=CARTESIAN_POINT('Ctrl Pts',(44.4299748287186,-2.81415548797717,
136.780531955991));
#267685=CARTESIAN_POINT('Ctrl Pts',(44.1515272049057,3.50680242016433,136.402255915145));
#267686=CARTESIAN_POINT('Ctrl Pts',(43.8730795810928,6.60518022099696,130.879787568212));
#267687=CARTESIAN_POINT('Ctrl Pts',(43.59463195728,3.63372007972613,125.288005538446));
#267688=CARTESIAN_POINT('Ctrl Pts',(43.316184333467,-2.6769512977182,124.765484337463));
#267689=CARTESIAN_POINT('Ctrl Pts',(43.0377367096542,-6.52763520890084,
129.792395422388));
#267690=CARTESIAN_POINT('Ctrl Pts',(42.7592890858413,-4.37974125581177,
135.749253084432));
#267691=CARTESIAN_POINT('Ctrl Pts',(42.4808414620283,1.79292094911309,137.161996140853));
#267692=CARTESIAN_POINT('Ctrl Pts',(42.2023938382155,6.31797639086063,132.732382739134));
#267693=CARTESIAN_POINT('Ctrl Pts',(41.9239462144025,5.0371201797131,126.531011196811));
#267694=CARTESIAN_POINT('Ctrl Pts',(41.6454985905898,-0.872603399589798,
124.256639007436));
#267695=CARTESIAN_POINT('Ctrl Pts',(41.3670509667768,-5.98044708371573,
127.999303103786));
#267696=CARTESIAN_POINT('Ctrl Pts',(41.0886033429639,-5.592552058989,134.319678020622));
#267697=CARTESIAN_POINT('Ctrl Pts',(40.810155719151,-0.0653749034083074,
137.409647976851));
#267698=CARTESIAN_POINT('Ctrl Pts',(40.5317080953382,5.52187859466303,134.429681536124));
#267699=CARTESIAN_POINT('Ctrl Pts',(40.2532604715252,6.03479542300531,128.118222278014));
#267700=CARTESIAN_POINT('Ctrl Pts',(39.9748128477124,1.00203007375177,124.275192928799));
#267701=CARTESIAN_POINT('Ctrl Pts',(39.6963652238994,-4.95155196138904,
126.432149717987));
#267702=CARTESIAN_POINT('Ctrl Pts',(39.4179176000866,-6.35489964077443,
132.60695472951));
#267703=CARTESIAN_POINT('Ctrl Pts',(39.1394699762736,-1.91840500439501,
137.125263813774));
#267704=CARTESIAN_POINT('Ctrl Pts',(38.8610223524608,4.28101011172891,135.834971654011));
#267705=CARTESIAN_POINT('Ctrl Pts',(38.5825747286478,6.54638607414467,129.921793710766));
#267706=CARTESIAN_POINT('Ctrl Pts',(38.304127104835,2.79595304316033,124.819651639079));
#267707=CARTESIAN_POINT('Ctrl Pts',(38.0256794810221,-3.52382424458856,
125.217164749334));
#267708=CARTESIAN_POINT('Ctrl Pts',(37.7472318572093,-6.60537919994535,
130.749037912801));
#267709=CARTESIAN_POINT('Ctrl Pts',(37.4687842333963,-3.61691336126579,
136.331749939282));
#267710=CARTESIAN_POINT('Ctrl Pts',(37.1903366095834,2.69531916037638,136.835061207086));
#267711=CARTESIAN_POINT('Ctrl Pts',(36.9118889857706,6.53068504729366,131.796453249222));
#267712=CARTESIAN_POINT('Ctrl Pts',(36.6334413619576,4.36467041744916,125.846160629286));
#267713=CARTESIAN_POINT('Ctrl Pts',(36.3549937381448,-1.8122631000273,124.452211577043));
#267714=CARTESIAN_POINT('Ctrl Pts',(36.0765461143319,-6.32381536255287,
128.895577173308));
#267715=CARTESIAN_POINT('Ctrl Pts',(35.798098490519,-5.02409024244786,135.093021505591));
#267716=CARTESIAN_POINT('Ctrl Pts',(35.5196508667061,0.892528370013623,
137.34939599451));
#267717=CARTESIAN_POINT('Ctrl Pts',(35.2412032428932,5.98895701286753,133.591202714771));
#267718=CARTESIAN_POINT('Ctrl Pts',(34.9627556190803,5.58182673771145,127.272037692505));
#267719=CARTESIAN_POINT('Ctrl Pts',(34.6843079952674,0.0452703779943793,
124.198904874802));
#267720=CARTESIAN_POINT('Ctrl Pts',(34.4058603714545,-5.53288724751859,
127.195863190245));
#267721=CARTESIAN_POINT('Ctrl Pts',(34.1274127476417,-6.02659178913083,
133.508854356496));
#267722=CARTESIAN_POINT('Ctrl Pts',(33.8489651238287,-0.982152891908117,
137.336547898535));
#267723=CARTESIAN_POINT('Ctrl Pts',(33.5705175000158,4.96483653214189,135.161480444452));
#267724=CARTESIAN_POINT('Ctrl Pts',(33.292069876203,6.34938372890195,128.982432726597));
#267725=CARTESIAN_POINT('Ctrl Pts',(33.0136222523901,1.89915746344075,124.477647734417));
#267726=CARTESIAN_POINT('Ctrl Pts',(32.7351746285772,-4.29630173192265,
125.786802804744));
#267727=CARTESIAN_POINT('Ctrl Pts',(32.4567270047643,-6.543669521657,131.706848383727));
#267728=CARTESIAN_POINT('Ctrl Pts',(32.1782793809514,-2.77772469701646,
136.797551794587));
#267729=CARTESIAN_POINT('Ctrl Pts',(31.8998317571386,3.54081342478663,136.380805297429));
#267730=CARTESIAN_POINT('Ctrl Pts',(31.6213841333256,6.60551698756319,130.839578563946));
#267731=CARTESIAN_POINT('Ctrl Pts',(31.3429365095127,3.6000731362139,125.26598825823));
#267732=CARTESIAN_POINT('Ctrl Pts',(31.0644888856998,-2.71366205396602,
124.781891586214));
#267733=CARTESIAN_POINT('Ctrl Pts',(30.7860412618869,-6.53367438631237,
129.83214974004));
#267734=CARTESIAN_POINT('Ctrl Pts',(30.507593638074,-4.34955914537615,135.775822195171));
#267735=CARTESIAN_POINT('Ctrl Pts',(30.2291460142612,1.83158846238341,137.150964329883));
#267736=CARTESIAN_POINT('Ctrl Pts',(29.9506983904483,6.32959575128355,132.693887701803));
#267737=CARTESIAN_POINT('Ctrl Pts',(29.6722507666353,5.01101376269691,126.500427991838));
#267738=CARTESIAN_POINT('Ctrl Pts',(29.3938031428225,-0.912445072176531,
124.26207210612));
#267739=CARTESIAN_POINT('Ctrl Pts',(29.1153555190096,-5.99741146113971,
128.035759753857));
#267740=CARTESIAN_POINT('Ctrl Pts',(28.8369078951967,-5.57104970715349,
134.353656341672));
#267741=CARTESIAN_POINT('Ctrl Pts',(28.5584602713837,-0.0251654332018655,
137.409923551768));
#267742=CARTESIAN_POINT('Ctrl Pts',(28.280012647571,5.54384464446253,134.396001125022));
#267743=CARTESIAN_POINT('Ctrl Pts',(28.001565023758,6.0183323257333,128.081536533317));
#267744=CARTESIAN_POINT('Ctrl Pts',(27.7231173999451,0.962266611534229,
124.269214257685));
#267745=CARTESIAN_POINT('Ctrl Pts',(27.4446697761322,-4.97807510932732,
126.462372227135));
#267746=CARTESIAN_POINT('Ctrl Pts',(27.1662221523194,-6.34380899720599,
132.645605409466));
#267747=CARTESIAN_POINT('Ctrl Pts',(26.8877745285064,-1.87989232895117,
137.136824577849));
#267748=CARTESIAN_POINT('Ctrl Pts',(26.6093269046936,4.31155355176403,135.808818724794));
#267749=CARTESIAN_POINT('Ctrl Pts',(26.3308792808807,6.5408923495088,129.881960352566));
#267750=CARTESIAN_POINT('Ctrl Pts',(26.0524316570678,2.75947061841045,124.802742762115));
#267751=CARTESIAN_POINT('Ctrl Pts',(25.7739840332549,-3.55776980337282,
125.238718785491));
#267752=CARTESIAN_POINT('Ctrl Pts',(25.4955364094419,-6.60559358257403,
130.789247755823));
#267753=CARTESIAN_POINT('Ctrl Pts',(25.2170887856292,-3.58319956057628,
136.353664707793));
#267754=CARTESIAN_POINT('Ctrl Pts',(24.9386411618162,2.73197980856112,136.81854229942));
#267755=CARTESIAN_POINT('Ctrl Pts',(24.6601935380033,6.5366031982641,131.756680734531));
#267756=CARTESIAN_POINT('Ctrl Pts',(24.3817459141905,4.3344075795813,125.819683505575));
#267757=CARTESIAN_POINT('Ctrl Pts',(24.1032982903775,-1.85089685715453,
124.463361027524));
#267758=CARTESIAN_POINT('Ctrl Pts',(23.8248506665647,-6.33531750350378,
128.934107397669));
#267759=CARTESIAN_POINT('Ctrl Pts',(23.5464030427517,-4.99789086159903,
135.123525109951));
#267760=CARTESIAN_POINT('Ctrl Pts',(23.2679554189389,0.932353321572971,
137.343841656646));
#267761=CARTESIAN_POINT('Ctrl Pts',(22.9895077951259,6.00581035021119,133.554694599836));
#267762=CARTESIAN_POINT('Ctrl Pts',(22.7110601713131,5.56022106715229,127.238124974604));
#267763=CARTESIAN_POINT('Ctrl Pts',(22.4326125475002,0.00506025528043594,
124.198751684957));
#267764=CARTESIAN_POINT('Ctrl Pts',(22.1541649236873,-5.554750683987,127.229610302442));
#267765=CARTESIAN_POINT('Ctrl Pts',(21.8757172998744,-6.01001710932725,
133.545489823263));
#267766=CARTESIAN_POINT('Ctrl Pts',(21.5972696760615,-0.942371416853923,
137.342405515655));
#267767=CARTESIAN_POINT('Ctrl Pts',(21.3188220522486,4.99126757030501,135.131177347952));
#267768=CARTESIAN_POINT('Ctrl Pts',(21.0403744284357,6.33817549733007,128.943815981773));
#267769=CARTESIAN_POINT('Ctrl Pts',(20.7619268046228,1.86060977939589,124.466204243228));
#267770=CARTESIAN_POINT('Ctrl Pts',(20.48347918081,-4.32676542996233,125.813048576547));
#267771=CARTESIAN_POINT('Ctrl Pts',(20.205031556997,-6.5380545834274,131.746664836412));
#267772=CARTESIAN_POINT('Ctrl Pts',(19.9265839331841,-2.74119097644563,
136.814349553278));
#267773=CARTESIAN_POINT('Ctrl Pts',(19.6481363093713,3.57469322326559,136.359148042506));
#267774=CARTESIAN_POINT('Ctrl Pts',(19.3696886855584,6.60560898426828,130.799368254665));
#267775=CARTESIAN_POINT('Ctrl Pts',(19.0912410617455,3.56629279066743,125.244176204439));
#267776=CARTESIAN_POINT('Ctrl Pts',(18.8127934379326,-2.75027225446848,
124.798521999768));
#267777=CARTESIAN_POINT('Ctrl Pts',(18.5343458141197,-6.53947145601676,
129.871940083324));
#267778=CARTESIAN_POINT('Ctrl Pts',(18.2558981903068,-4.31921586042675,
135.802207086573));
#267779=CARTESIAN_POINT('Ctrl Pts',(17.9774505664939,1.87018810546999,137.139697343177));
#267780=CARTESIAN_POINT('Ctrl Pts',(17.6990029426811,6.34098056620813,132.65532264735));
#267781=CARTESIAN_POINT('Ctrl Pts',(17.4205553188681,4.98472166072295,126.470004270672));
#267782=CARTESIAN_POINT('Ctrl Pts',(17.1421076950552,-0.95225293377558,
124.26774763171));
#267783=CARTESIAN_POINT('Ctrl Pts',(16.8636600712423,-6.01415360227624,
128.072318995452));
#267784=CARTESIAN_POINT('Ctrl Pts',(16.5852124474295,-5.54934091802252,
134.387503142263));
#267785=CARTESIAN_POINT('Ctrl Pts',(16.3067648236166,0.0150449695187284,
137.409954355121));
#267786=CARTESIAN_POINT('Ctrl Pts',(16.0283171998036,5.56560526505998,134.362187624359));
#267787=CARTESIAN_POINT('Ctrl Pts',(15.7498695759908,6.00164621694371,128.044951683866));
#267788=CARTESIAN_POINT('Ctrl Pts',(15.4714219521779,0.922467492173741,
124.263477748823));
#267789=CARTESIAN_POINT('Ctrl Pts',(15.192974328365,-5.00441379286154,126.492755630261));
#267790=CARTESIAN_POINT('Ctrl Pts',(14.9145267045521,-6.33248328146239,
132.684187861418));
#267791=CARTESIAN_POINT('Ctrl Pts',(14.6360790807393,-1.84130999340576,
137.148150690142));
#267792=CARTESIAN_POINT('Ctrl Pts',(14.3576314569263,4.34193722559672,135.782480353541));
#267793=CARTESIAN_POINT('Ctrl Pts',(14.0791838331134,6.53515624970152,129.842161174248));
#267794=CARTESIAN_POINT('Ctrl Pts',(13.8007362093005,2.72288594046203,124.786056277307));
#267795=CARTESIAN_POINT('Ctrl Pts',(13.5222885854877,-3.59158352768866,
125.260479058552));
#267796=CARTESIAN_POINT('Ctrl Pts',(13.2438409616747,-6.60556319250329,
130.829458158858));
#267797=CARTESIAN_POINT('Ctrl Pts',(12.9653933378619,-3.54935298310934,
136.375373844801));
#267798=CARTESIAN_POINT('Ctrl Pts',(12.686945714049,2.76853922222938,136.801800534039));
#267799=CARTESIAN_POINT('Ctrl Pts',(12.4084980902361,6.5422791329992,131.716872931266));
#267800=CARTESIAN_POINT('Ctrl Pts',(12.1300504664232,4.30398412864651,125.793391090908));
#267801=CARTESIAN_POINT('Ctrl Pts',(11.8516028426103,-1.88946202861834,
124.474745446076));
#267802=CARTESIAN_POINT('Ctrl Pts',(11.5731552187974,-6.34658488693473,
128.972706924952));
#267803=CARTESIAN_POINT('Ctrl Pts',(11.2947075949845,-4.97150628206636,
135.153868666082));
#267804=CARTESIAN_POINT('Ctrl Pts',(11.0162599711716,0.972143724437105,
137.338044995907));
#267805=CARTESIAN_POINT('Ctrl Pts',(10.7378123473587,6.0224411400439,133.518084570262));
#267806=CARTESIAN_POINT('Ctrl Pts',(10.4593647235458,5.53840936055655,127.204344404875));
#267807=CARTESIAN_POINT('Ctrl Pts',(10.1809170997329,-0.0351500549433496,
124.198843268382));
#267808=CARTESIAN_POINT('Ctrl Pts',(9.90246947592002,-5.57640828712608,
127.263489878326));
#267809=CARTESIAN_POINT('Ctrl Pts',(9.62402185210712,-5.99321972612948,
133.582023716479));
#267810=CARTESIAN_POINT('Ctrl Pts',(9.34557422829421,-0.902555021880531,
137.348020863117));
#267811=CARTESIAN_POINT('Ctrl Pts',(9.06712660448133,5.01751365521256,135.100713919668));
#267812=CARTESIAN_POINT('Ctrl Pts',(8.78867898066847,6.32673240233446,128.905268180115));
#267813=CARTESIAN_POINT('Ctrl Pts',(8.51023135685555,1.82199314977141,124.454995614755));
#267814=CARTESIAN_POINT('Ctrl Pts',(8.23178373304265,-4.35706879811783,
125.839479303254));
#267815=CARTESIAN_POINT('Ctrl Pts',(7.9533361092298,-6.53219737518076,131.786446371669));
#267816=CARTESIAN_POINT('Ctrl Pts',(7.67488848541689,-2.70455568003535,
136.83092460962));
#267817=CARTESIAN_POINT('Ctrl Pts',(7.39644086160398,3.60844056017245,136.337284952891));
#267818=CARTESIAN_POINT('Ctrl Pts',(7.1179932377911,6.60545620770325,130.759158130379));
#267819=CARTESIAN_POINT('Ctrl Pts',(6.83954561397822,3.53238029483008,125.222570185327));
#267820=CARTESIAN_POINT('Ctrl Pts',(6.5610979901653,-2.78678054262086,124.815374961881));
#267821=CARTESIAN_POINT('Ctrl Pts',(6.28265036635242,-6.54502620320144,
129.911764977794));
#267822=CARTESIAN_POINT('Ctrl Pts',(6.00420274253956,-4.28871252534551,
135.828406780936));
#267823=CARTESIAN_POINT('Ctrl Pts',(5.72575511872663,1.90871844804856,137.128195598241));
#267824=CARTESIAN_POINT('Ctrl Pts',(5.44730749491374,6.35213041376593,132.616689004818));
#267825=CARTESIAN_POINT('Ctrl Pts',(5.16885987110085,4.95824484805471,126.439741160674));
#267826=CARTESIAN_POINT('Ctrl Pts',(4.89041224728798,-0.992025509291961,
124.273665373899));
#267827=CARTESIAN_POINT('Ctrl Pts',(4.61196462347505,-6.03067288673954,
128.108979473854));
#267828=CARTESIAN_POINT('Ctrl Pts',(4.33351699966218,-5.52742649602286,
134.421217168191));
#267829=CARTESIAN_POINT('Ctrl Pts',(4.05506937584931,0.0552548147426717,
137.409740385768));
#267830=CARTESIAN_POINT('Ctrl Pts',(3.77662175203639,5.58715965010757,134.328242287108));
#267831=CARTESIAN_POINT('Ctrl Pts',(3.49817412822347,5.98473771494644,128.008469085329));
#267832=CARTESIAN_POINT('Ctrl Pts',(3.21972650441063,0.882634190440881,
124.25798361478));
#267833=CARTESIAN_POINT('Ctrl Pts',(2.94127888059773,-5.03056703600248,
126.523298801495));
#267834=CARTESIAN_POINT('Ctrl Pts',(2.66283125678483,-6.32092291322184,
132.722700655682));
#267835=CARTESIAN_POINT('Ctrl Pts',(2.38438363297192,-1.80265942744139,
137.159241730961));
#267836=CARTESIAN_POINT('Ctrl Pts',(2.10593600915906,4.37216000734877,135.755957516231));
#267837=CARTESIAN_POINT('Ctrl Pts',(1.82748838534615,6.529177987276,129.802397650584));
#267838=CARTESIAN_POINT('Ctrl Pts',(1.54904076153325,2.68620036497402,124.769592802981));
#267839=CARTESIAN_POINT('Ctrl Pts',(1.27059313772038,-3.62526416455594,
125.282444762183));
#267840=CARTESIAN_POINT('Ctrl Pts',(0.992145513907496,-6.60528803085927,
130.869667631896));
#267841=CARTESIAN_POINT('Ctrl Pts',(0.713697890094564,-3.51537488306232,
136.396876545864));
#267842=CARTESIAN_POINT('Ctrl Pts',(0.435250266281723,2.80499604665836,
136.784836531317));
#267843=CARTESIAN_POINT('Ctrl Pts',(0.156802642468823,6.54771264117505,
131.677031314524));
#267844=CARTESIAN_POINT('Ctrl Pts',(-0.121644981344083,4.27340119199728,
125.767284359559));
#267845=CARTESIAN_POINT('Ctrl Pts',(-0.400092605156985,-1.92795718537184,
124.486364410847));
#267846=CARTESIAN_POINT('Ctrl Pts',(-0.678540228969845,-6.35761709532873,
129.011374324836));
#267847=CARTESIAN_POINT('Ctrl Pts',(-0.956987852782752,-4.94493748154019,
135.184051049593));
#267848=CARTESIAN_POINT('Ctrl Pts',(-1.23543547659566,1.01189810415772,
137.332006227089));
#267849=CARTESIAN_POINT('Ctrl Pts',(-1.51388310040852,6.03884876610542,
133.48137398265));
#267850=CARTESIAN_POINT('Ctrl Pts',(-1.79233072422142,5.51639242616521,
127.170697235071));
#267851=CARTESIAN_POINT('Ctrl Pts',(-2.07077834803434,-0.0753590626689394,
124.19917962168));
#267852=CARTESIAN_POINT('Ctrl Pts',(-2.34922597184723,-5.59785925440532,
127.297500662476));
#267853=CARTESIAN_POINT('Ctrl Pts',(-2.6276735956601,-5.97620026197078,
133.618454682368));
#267854=CARTESIAN_POINT('Ctrl Pts',(-2.906121219473,-0.862705182398668,
137.353393732843));
#267855=CARTESIAN_POINT('Ctrl Pts',(-3.18456884328591,5.04357381430661,
135.070091288433));
#267856=CARTESIAN_POINT('Ctrl Pts',(-3.46301646709877,6.31505486794284,
128.866790750024));
#267857=CARTESIAN_POINT('Ctrl Pts',(-3.74146409091167,1.78330900552073,
124.444022264336));
#267858=CARTESIAN_POINT('Ctrl Pts',(-4.01991171472458,-4.38721071348669,
125.866094005463));
#267859=CARTESIAN_POINT('Ctrl Pts',(-4.29835933853748,-6.52609811395827,
131.826191515377));
#267860=CARTESIAN_POINT('Ctrl Pts',(-4.57680696235032,-2.66782016531947,
136.847276349416));
#267861=CARTESIAN_POINT('Ctrl Pts',(-4.85525458616324,3.64205418498746,
136.31521683873));
#267862=CARTESIAN_POINT('Ctrl Pts',(-5.13370220997616,6.60505866352928,
130.718949681087));
#267863=CARTESIAN_POINT('Ctrl Pts',(-5.41214983378902,3.49833690534187,
125.201171001511));
#267864=CARTESIAN_POINT('Ctrl Pts',(-5.69059745760191,-2.82318556559566,
124.832449848059));
#267865=CARTESIAN_POINT('Ctrl Pts',(-5.96904508141481,-6.55033842203324,
129.951622947723));
#267866=CARTESIAN_POINT('Ctrl Pts',(-6.24749270522772,-4.2580502704442,
135.854420307421));
#267867=CARTESIAN_POINT('Ctrl Pts',(-6.52594032904057,1.9471780623631,137.116459521273));
#267868=CARTESIAN_POINT('Ctrl Pts',(-6.80438795285348,6.36304488079526,
132.577988205793));
#267869=CARTESIAN_POINT('Ctrl Pts',(-7.0828355766664,4.93158430580029,126.409639783256));
#267870=CARTESIAN_POINT('Ctrl Pts',(-7.36128320047925,-1.03176132493798,
124.279825113401));
#267871=CARTESIAN_POINT('Ctrl Pts',(-7.63973082429214,-6.04696870240127,
128.145739830595));
#267872=CARTESIAN_POINT('Ctrl Pts',(-7.91817844810507,-5.50530725320171,
134.454797170168));
#267873=CARTESIAN_POINT('Ctrl Pts',(-8.19662607191793,0.09546261247915,
137.40928165164));
#267874=CARTESIAN_POINT('Ctrl Pts',(-8.47507369573082,5.60850700089942,
134.294166371127));
#267875=CARTESIAN_POINT('Ctrl Pts',(-8.75352131954372,5.96760744629241,
127.972090089581));
#267876=CARTESIAN_POINT('Ctrl Pts',(-9.03196894335663,0.842768182373745,
124.252732059145));
#267877=CARTESIAN_POINT('Ctrl Pts',(-9.31041656716948,-5.05653386963193,
126.554000609049));
#267878=CARTESIAN_POINT('Ctrl Pts',(-9.5888641909824,-6.30912832085822,
132.76114236515));
#267879=CARTESIAN_POINT('Ctrl Pts',(-9.86731181479532,-1.76394206326903,
137.170097289323));
#267880=CARTESIAN_POINT('Ctrl Pts',(-10.1457594386081,4.40222077710389,
135.729251195677));
#267881=CARTESIAN_POINT('Ctrl Pts',(-10.424207062421,6.52295778375913,129.762671255026));
#267882=CARTESIAN_POINT('Ctrl Pts',(-10.7026546862339,2.64941525134336,
124.753352949195));
#267883=CARTESIAN_POINT('Ctrl Pts',(-10.9811023100469,-3.65881046592654,
125.304615082438));
#267884=CARTESIAN_POINT('Ctrl Pts',(-11.2595499338597,-6.60476810783814,
130.909874684957));
#267885=CARTESIAN_POINT('Ctrl Pts',(-11.5379975576726,-3.48126651950624,
136.418172014193));
#267886=CARTESIAN_POINT('Ctrl Pts',(-11.8164451814855,2.84134893092756,
136.767650919861));
#267887=CARTESIAN_POINT('Ctrl Pts',(-12.0948928052984,6.5529035214511,131.637157360647));
#267888=CARTESIAN_POINT('Ctrl Pts',(-12.3733404291112,4.2426599028951,125.741364278924));
#267889=CARTESIAN_POINT('Ctrl Pts',(-12.6517880529242,-1.96638090096281,
124.498217491291));
#267890=CARTESIAN_POINT('Ctrl Pts',(-12.9302356767371,-6.36841371988325,
129.050108164486));
#267891=CARTESIAN_POINT('Ctrl Pts',(-13.2086833005499,-4.91818544453708,
135.214071142064));
#267892=CARTESIAN_POINT('Ctrl Pts',(-13.4871309243628,1.05161498762227,
137.325725573964));
#267893=CARTESIAN_POINT('Ctrl Pts',(-13.7655785481758,6.05503262040511,
133.444564197323));
#267894=CARTESIAN_POINT('Ctrl Pts',(-14.0440261719886,5.49417107982388,
127.137184712));
#267895=CARTESIAN_POINT('Ctrl Pts',(-14.3224737958015,-0.115565277936756,
124.199760732389));
#267896=CARTESIAN_POINT('Ctrl Pts',(-14.6009214196144,-5.61910279095105,
127.331641394614));
#267897=CARTESIAN_POINT('Ctrl Pts',(-14.8793690434273,-5.95895934751375,
133.654781370965));
#267898=CARTESIAN_POINT('Ctrl Pts',(-15.1578166672402,-0.822823375059262,
137.358523925738));
#267899=CARTESIAN_POINT('Ctrl Pts',(-15.4362642910531,5.06944708191823,
135.039310588977));
#267900=CARTESIAN_POINT('Ctrl Pts',(-15.714711914866,6.3031433268707,128.828385117298));
#267901=CARTESIAN_POINT('Ctrl Pts',(-15.9931595386788,1.74455878009922,
124.433284598595));
#267902=CARTESIAN_POINT('Ctrl Pts',(-16.2716071624918,-4.41719005914895,
125.892891696959));
#267903=CARTESIAN_POINT('Ctrl Pts',(-16.5500547863046,-6.51975702577033,
131.865898794765));
#267904=CARTESIAN_POINT('Ctrl Pts',(-16.8285024101176,-2.63098579354628,
136.863404166748));
#267905=CARTESIAN_POINT('Ctrl Pts',(-17.1069500339304,3.67553285214529,
136.292944517765));
#267906=CARTESIAN_POINT('Ctrl Pts',(-17.3853976577434,6.60441636647752,
130.678744396729));
#267907=CARTESIAN_POINT('Ctrl Pts',(-17.6638452815562,3.46416388369313,
125.179979445948));
#267908=CARTESIAN_POINT('Ctrl Pts',(-17.9422929053691,-2.8594859743911,
124.849746025587));
#267909=CARTESIAN_POINT('Ctrl Pts',(-18.220740529182,-6.55540791566593,
129.991512516161));
#267910=CARTESIAN_POINT('Ctrl Pts',(-18.4991881529949,-4.22723023192423,
135.880246702087));
#267911=CARTESIAN_POINT('Ctrl Pts',(-18.7776357768078,1.98556552327847,
137.104489547159));
#267912=CARTESIAN_POINT('Ctrl Pts',(-19.0560834006207,6.37372356285652,
132.539221684343));
#267913=CARTESIAN_POINT('Ctrl Pts',(-19.3345310244336,4.90474102187576,
126.379701253833));
#267914=CARTESIAN_POINT('Ctrl Pts',(-19.6129786482465,-1.07145890828896,
124.286226621967));
#267915=CARTESIAN_POINT('Ctrl Pts',(-19.8914262720594,-6.06304044541393,
128.182598703507));
#267916=CARTESIAN_POINT('Ctrl Pts',(-20.1698738958722,-5.48298400919569,
134.488241903877));
#267917=CARTESIAN_POINT('Ctrl Pts',(-20.4483215196851,0.135666872813404,
137.408578169733));
#267918=CARTESIAN_POINT('Ctrl Pts',(-20.7267691434981,5.62964652640204,
134.25996113911));
#267919=CARTESIAN_POINT('Ctrl Pts',(-21.0052167673109,5.95025604574973,
127.935816044659));
#267920=CARTESIAN_POINT('Ctrl Pts',(-21.2836643911238,0.802870945221437,
124.247723276515));
#267921=CARTESIAN_POINT('Ctrl Pts',(-21.5621120149367,-5.08231333153929,
126.584859915257));
#267922=CARTESIAN_POINT('Ctrl Pts',(-21.8405596387496,-6.29709994142449,
132.79951156535));
#267923=CARTESIAN_POINT('Ctrl Pts',(-22.1190072625625,-1.725159335575,137.180716962973));
#267924=CARTESIAN_POINT('Ctrl Pts',(-22.3974548863754,4.43211842094896,
135.702362381491));
#267925=CARTESIAN_POINT('Ctrl Pts',(-22.6759025101882,6.51649586964294,
129.722983459651));
#267926=CARTESIAN_POINT('Ctrl Pts',(-22.9543501340012,2.61253196265622,
124.737337317723));
#267927=CARTESIAN_POINT('Ctrl Pts',(-23.232797757814,-3.6922211887298,125.326989197785));
#267928=CARTESIAN_POINT('Ctrl Pts',(-23.511245381627,-6.60400344270576,
130.950077828156));
#267929=CARTESIAN_POINT('Ctrl Pts',(-23.7896930054398,-3.4470291563393,
136.439259460675));
#267930=CARTESIAN_POINT('Ctrl Pts',(-24.0681406292527,2.87759652796706,
136.75024433649));
#267931=CARTESIAN_POINT('Ctrl Pts',(-24.3465882530656,6.55785158147733,
131.597252547181));
#267932=CARTESIAN_POINT('Ctrl Pts',(-24.6250358768785,4.21176140046998,
125.715631809479));
#267933=CARTESIAN_POINT('Ctrl Pts',(-24.9034835006914,-2.00473175158637,
124.510304248187));
#267934=CARTESIAN_POINT('Ctrl Pts',(-25.1819311245043,-6.3789743605254,
129.088907008606));
#267935=CARTESIAN_POINT('Ctrl Pts',(-25.4603787483172,-4.89125116236366,
135.24392783109));
#267936=CARTESIAN_POINT('Ctrl Pts',(-25.73882637213,1.09129290310671,137.319203269261));
#267937=CARTESIAN_POINT('Ctrl Pts',(-26.017273995943,6.07099210324431,133.407656578282));
#267938=CARTESIAN_POINT('Ctrl Pts',(-26.2957216197559,5.47174614495268,
127.103808077481));
#267939=CARTESIAN_POINT('Ctrl Pts',(-26.5741692435687,-0.155767210890682,
124.200586578976));
#267940=CARTESIAN_POINT('Ctrl Pts',(-26.8526168673816,-5.64013810957666,
127.365910809639));
#267941=CARTESIAN_POINT('Ctrl Pts',(-27.1310644911945,-5.94149762162655,
133.691002436174));
#267942=CARTESIAN_POINT('Ctrl Pts',(-27.4095121150075,-0.782911077696857,
137.363411251701));
#267943=CARTESIAN_POINT('Ctrl Pts',(-27.6879597388203,5.09513249930392,
135.008372961895));
#267944=CARTESIAN_POINT('Ctrl Pts',(-27.9664073626332,6.29099822050462,
128.79005270507));
#267945=CARTESIAN_POINT('Ctrl Pts',(-28.2448549864461,1.70574390941038,
124.422783015417));
#267946=CARTESIAN_POINT('Ctrl Pts',(-28.523302610259,-4.44700572420938,
125.919871384741));
#267947=CARTESIAN_POINT('Ctrl Pts',(-28.8017502340719,-6.51317434558802,
131.905566738465));
#267948=CARTESIAN_POINT('Ctrl Pts',(-29.0801978578848,-2.59405392962697,
136.879307463993));
#267949=CARTESIAN_POINT('Ctrl Pts',(-29.3586454816977,3.7088753210816,136.270468815306));
#267950=CARTESIAN_POINT('Ctrl Pts',(-29.6370931055106,6.6035293403484,130.638543767126));
#267951=CARTESIAN_POINT('Ctrl Pts',(-29.9155407293234,3.42986249617799,
125.158996303897));
#267952=CARTESIAN_POINT('Ctrl Pts',(-30.1939883531365,-2.89568042388203,
124.86726285355));
#267953=CARTESIAN_POINT('Ctrl Pts',(-30.4724359769491,-6.56023449624756,
130.031432204983));
#267954=CARTESIAN_POINT('Ctrl Pts',(-30.7508836007622,-4.19625355183344,
135.905885007927));
#267955=CARTESIAN_POINT('Ctrl Pts',(-31.029331224575,2.02387940833292,137.092286119451));
#267956=CARTESIAN_POINT('Ctrl Pts',(-31.3077788483879,6.38416606424714,
132.50039087698));
#267957=CARTESIAN_POINT('Ctrl Pts',(-31.5862264722008,4.8777159909692,126.349926681791));
#267958=CARTESIAN_POINT('Ctrl Pts',(-31.8646740960137,-1.11111678833609,
124.292869662384));
#267959=CARTESIAN_POINT('Ctrl Pts',(-32.1431217198266,-6.07888752023319,
128.219554726771));
#267960=CARTESIAN_POINT('Ctrl Pts',(-32.4215693436394,-5.46045759120085,
134.52155013001));
#267961=CARTESIAN_POINT('Ctrl Pts',(-32.7000169674524,0.175866105961793,
137.407629966116));
#267962=CARTESIAN_POINT('Ctrl Pts',(-32.9784645912652,5.65057744328232,
134.225627858545));
#267963=CARTESIAN_POINT('Ctrl Pts',(-33.2569122150782,5.93268415628106,
127.89964829471));
#267964=CARTESIAN_POINT('Ctrl Pts',(-33.535359838891,0.762943957391,124.242957452493));
#267965=CARTESIAN_POINT('Ctrl Pts',(-33.813807462704,-5.10790446645711,
126.615875576613));
#267966=CARTESIAN_POINT('Ctrl Pts',(-34.0922550865168,-6.28483822063666,
132.837806834499));
#267967=CARTESIAN_POINT('Ctrl Pts',(-34.3707027103298,-1.68631268146717,
137.191100358392));
#267968=CARTESIAN_POINT('Ctrl Pts',(-34.6491503341426,4.46185183101625,
135.675292070049));
#267969=CARTESIAN_POINT('Ctrl Pts',(-34.9275979579556,6.5097924843757,129.683335735103));
#267970=CARTESIAN_POINT('Ctrl Pts',(-35.2060455817684,2.57555186563646,
124.721546502031));
#267971=CARTESIAN_POINT('Ctrl Pts',(-35.4844932055813,-3.72549509491909,
125.349566279145));
#267972=CARTESIAN_POINT('Ctrl Pts',(-35.7629408293942,-6.60299406379731,
130.990275571749));
#267973=CARTESIAN_POINT('Ctrl Pts',(-36.0413884532071,-3.41266406223907,
136.460138103909));
#267974=CARTESIAN_POINT('Ctrl Pts',(-36.3198360770199,2.91373749460914,
136.73261742621));
#267975=CARTESIAN_POINT('Ctrl Pts',(-36.5982837008328,6.56255663790157,
131.557318352812));
#267976=CARTESIAN_POINT('Ctrl Pts',(-36.8767313246458,4.18070682967726,
125.690087904753));
#267977=CARTESIAN_POINT('Ctrl Pts',(-37.1551789484586,-2.04300831613737,
124.522624233657));
#267978=CARTESIAN_POINT('Ctrl Pts',(-37.4336265722715,-6.38929862592666,
129.12776941949));
#267979=CARTESIAN_POINT('Ctrl Pts',(-37.7120741960844,-4.86413563307991,
135.273620010322));
#267980=CARTESIAN_POINT('Ctrl Pts',(-37.9905218198973,1.13093038033133,
137.312439554669));
#267981=CARTESIAN_POINT('Ctrl Pts',(-38.2689694437102,6.0867266232385,133.370652493151));
#267982=CARTESIAN_POINT('Ctrl Pts',(-38.5474170675231,5.44911845251588,
127.070568568297));
#267983=CARTESIAN_POINT('Ctrl Pts',(-38.825864691336,-0.195963371833029,
124.201657130839));
#267984=CARTESIAN_POINT('Ctrl Pts',(-39.1043123151489,-5.66096443081045,
127.400307637685));
#267985=CARTESIAN_POINT('Ctrl Pts',(-39.3827599389617,-5.92381573136,133.727116535809));
#267986=CARTESIAN_POINT('Ctrl Pts',(-39.6612075627747,-0.742969769276543,
137.368055529631));
#267987=CARTESIAN_POINT('Ctrl Pts',(-39.9396551865875,5.12062911468111,
134.977279553588));
#267988=CARTESIAN_POINT('Ctrl Pts',(-40.2181028104005,6.27861999888597,
128.751794933764));
#267989=CARTESIAN_POINT('Ctrl Pts',(-40.4965504342133,1.66686583175366,
124.412517903944));
#267990=CARTESIAN_POINT('Ctrl Pts',(-40.7749980580263,-4.47665660383728,
125.947032069068));
#267991=CARTESIAN_POINT('Ctrl Pts',(-41.0534456818391,-6.5063503173351,
131.945193876568));
#267992=CARTESIAN_POINT('Ctrl Pts',(-41.3318933056519,-2.55702594208532,
136.894985651848));
#267993=CARTESIAN_POINT('Ctrl Pts',(-41.6103409294649,3.74208035627896,
136.247790564197));
#267994=CARTESIAN_POINT('Ctrl Pts',(-41.8887885532778,6.60239761801125,
130.598349281928));
#267995=CARTESIAN_POINT('Ctrl Pts',(-42.1672361770906,3.39543401384647,
125.138222352896));
#267996=CARTESIAN_POINT('Ctrl Pts',(-42.4456838009036,-2.93176757287012,
124.884999682853));
#267997=CARTESIAN_POINT('Ctrl Pts',(-42.7241314247165,-6.56481798492739,
130.071380534953));
#267998=CARTESIAN_POINT('Ctrl Pts',(-43.0025790485293,-4.16512137802412,
135.931334274905));
#267999=CARTESIAN_POINT('Ctrl Pts',(-43.2810266723423,2.06211829779186,
137.079849690351));
#268000=CARTESIAN_POINT('Ctrl Pts',(-43.5594742961552,6.39437199801655,
132.461497222591));
#268001=CARTESIAN_POINT('Ctrl Pts',(-43.837921919968,4.85051021450257,126.320317170437));
#268002=CARTESIAN_POINT('Ctrl Pts',(-44.116369543781,-1.150733495542,124.299753988494));
#268003=CARTESIAN_POINT('Ctrl Pts',(-44.3948171675938,-6.09450933963988,
128.256606530968));
#268004=CARTESIAN_POINT('Ctrl Pts',(-44.6732647914067,-5.43772883394191,
134.554720614319));
#268005=CARTESIAN_POINT('Ctrl Pts',(-44.9517124152196,0.216058822326645,
137.406437075925));
#268006=CARTESIAN_POINT('Ctrl Pts',(-45.2301600390324,5.67129897593744,
134.191167801664));
#268007=CARTESIAN_POINT('Ctrl Pts',(-45.5086076628454,5.91489242901924,
127.863588179946));
#268008=CARTESIAN_POINT('Ctrl Pts',(-45.7870552866582,0.722988698391639,
124.238434763679));
#268009=CARTESIAN_POINT('Ctrl Pts',(-46.0655029104712,-5.13330632609627,
126.647046443824));
#268010=CARTESIAN_POINT('Ctrl Pts',(-46.343950534284,-6.27234361285742,
132.876026753548));
#268011=CARTESIAN_POINT('Ctrl Pts',(-46.622398158097,-1.64740354042306,
137.201247090823));
#268012=CARTESIAN_POINT('Ctrl Pts',(-46.9008457819097,4.49141990552312,
135.64804126445));
#268013=CARTESIAN_POINT('Ctrl Pts',(-47.1792934057228,6.50284787635396,
129.643729550545));
#268014=CARTESIAN_POINT('Ctrl Pts',(-47.4577410295356,2.53847633059532,
124.705981087252));
#268015=CARTESIAN_POINT('Ctrl Pts',(-47.7361886533485,-3.75863095151733,
125.372345489915));
#268016=CARTESIAN_POINT('Ctrl Pts',(-48.0146362771614,-6.60174000851572,
131.030466426196));
#268017=CARTESIAN_POINT('Ctrl Pts',(-48.2930839009743,-3.37817251061699,
136.480807170229));
#268018=CARTESIAN_POINT('Ctrl Pts',(-48.5715315247872,2.94977049163681,
136.714770842195));
#268019=CARTESIAN_POINT('Ctrl Pts',(-48.8499791486,6.56701851637621,131.517356257317));
#268020=CARTESIAN_POINT('Ctrl Pts',(-49.128426772413,4.14949734125552,125.664733511282));
#268021=CARTESIAN_POINT('Ctrl Pts',(-49.4068743962258,-2.08120917626415,
124.535176991179));
#268022=CARTESIAN_POINT('Ctrl Pts',(-49.6853220200388,-6.39938613351776,
129.166693957078));
#268023=CARTESIAN_POINT('Ctrl Pts',(-49.9637696438516,-4.83683986146123,
135.303146579501));
#268024=CARTESIAN_POINT('Ctrl Pts',(-50.2422172676646,1.17052595051479,
137.305434680818));
#268025=CARTESIAN_POINT('Ctrl Pts',(-50.5206648914774,6.10223559733929,
133.333553313131));
#268026=CARTESIAN_POINT('Ctrl Pts',(-50.7991125152903,5.42628884099088,
127.03746741615));
#268027=CARTESIAN_POINT('Ctrl Pts',(-51.0775601391032,-0.236152271280866,
124.202972348307));
#268028=CARTESIAN_POINT('Ctrl Pts',(-51.3560077629162,-5.68158098292544,
127.434830604167));
#268029=CARTESIAN_POINT('Ctrl Pts',(-51.634455386729,-5.90591433192304,
133.763122331648));
#268030=CARTESIAN_POINT('Ctrl Pts',(-51.9129030105419,-0.703000929838195,
137.372456587432));
#268031=CARTESIAN_POINT('Ctrl Pts',(-52.1913506343548,5.14593598326309,
134.946031516236));
#268032=CARTESIAN_POINT('Ctrl Pts',(-52.4697982581677,6.26600912069438,
128.713613221033));
#268033=CARTESIAN_POINT('Ctrl Pts',(-52.7482458819806,1.62792598777083,
124.402489644555));
#268034=CARTESIAN_POINT('Ctrl Pts',(-53.0266935057934,-4.50614159930848,
125.97437274349));
#268035=CARTESIAN_POINT('Ctrl Pts',(-53.3051411296064,-6.49928519387843,
131.984778740675));
#268036=CARTESIAN_POINT('Ctrl Pts',(-53.5835887534191,-2.51990320300721,
136.910438149353));
#268037=CARTESIAN_POINT('Ctrl Pts',(-53.8620363772322,3.7751467273123,136.22491060479));
#268038=CARTESIAN_POINT('Ctrl Pts',(-54.140484001045,6.60102124140245,130.558162430556));
#268039=CARTESIAN_POINT('Ctrl Pts',(-54.418931624858,3.36087971245889,125.117658362733));
#268040=CARTESIAN_POINT('Ctrl Pts',(-54.6973792486707,-2.96774608413265,
124.902955856252));
#268041=CARTESIAN_POINT('Ctrl Pts',(-54.9758268724838,-6.56915821186243,
130.111356025769));
#268042=CARTESIAN_POINT('Ctrl Pts',(-55.2542744962966,-4.13383486411065,
135.956593559989));
#268043=CARTESIAN_POINT('Ctrl Pts',(-55.5327221201095,2.10028077469877,
137.067180720695));
#268044=CARTESIAN_POINT('Ctrl Pts',(-55.8111697439224,6.40434098598004,
132.422542162396));
#268045=CARTESIAN_POINT('Ctrl Pts',(-56.0896173677353,4.82312470059616,
126.29087381696));
#268046=CARTESIAN_POINT('Ctrl Pts',(-56.3680649915482,-1.19030756189505,
124.306879345194));
#268047=CARTESIAN_POINT('Ctrl Pts',(-56.646512615361,-6.10990532476174,
128.293752743129));
#268048=CARTESIAN_POINT('Ctrl Pts',(-56.924960239174,-5.41479857964128,
134.587752127659));
#268049=CARTESIAN_POINT('Ctrl Pts',(-57.2034078629868,0.256243532552689,
137.404999543363));
#268050=CARTESIAN_POINT('Ctrl Pts',(-57.4818554867998,5.69181035652338,
134.156582245398));
#268051=CARTESIAN_POINT('Ctrl Pts',(-57.7603031106126,5.89688152324325,
127.827637036585));
#268052=CARTESIAN_POINT('Ctrl Pts',(-58.0387507344255,0.683006648780185,
124.234155377662));
#268053=CARTESIAN_POINT('Ctrl Pts',(-58.3171983582384,-5.15851796918197,
126.67837136184));
#268054=CARTESIAN_POINT('Ctrl Pts',(-58.5956459820513,-6.25961658107885,
132.91416990625));
#268055=CARTESIAN_POINT('Ctrl Pts',(-58.8740936058642,-1.60843335423465,
137.211156784272));
#268056=CARTESIAN_POINT('Ctrl Pts',(-59.1525412296771,4.52082154881365,
135.620610974484));
#268057=CARTESIAN_POINT('Ctrl Pts',(-59.4309888534899,6.49566230291273,
129.604166373598));
#268058=CARTESIAN_POINT('Ctrl Pts',(-59.7094364773029,2.50130673138007,
124.69064165017));
#268059=CARTESIAN_POINT('Ctrl Pts',(-59.9878841011157,-3.79162753066369,
125.395325986002));
#268060=CARTESIAN_POINT('Ctrl Pts',(-60.2663317249287,-6.60024132333016,
131.070648902209));
#268061=CARTESIAN_POINT('Ctrl Pts',(-60.5447793487415,-3.34355577957023,
136.501265893734));
#268062=CARTESIAN_POINT('Ctrl Pts',(-60.8232269725544,2.98569418383416,
136.696705245755));
#268063=CARTESIAN_POINT('Ctrl Pts',(-61.1016745963673,6.57123705156454,
131.477367741508));
#268064=CARTESIAN_POINT('Ctrl Pts',(-61.3801222201802,4.11813409168408,
125.639569568584));
#268065=CARTESIAN_POINT('Ctrl Pts',(-61.6585698439931,-2.11933291641938,
124.547962055604));
#268066=CARTESIAN_POINT('Ctrl Pts',(-61.937017467806,-6.40923650950231,
129.205679179005));
#268067=CARTESIAN_POINT('Ctrl Pts',(-62.2154650916189,-4.80936485896274,
135.332506444514));
#268068=CARTESIAN_POINT('Ctrl Pts',(-62.4939127154318,1.21007814642843,
137.298188907278));
#268069=CARTESIAN_POINT('Ctrl Pts',(-62.7723603392447,6.1175184508558,133.296360412945));
#268070=CARTESIAN_POINT('Ctrl Pts',(-63.0508079630576,5.40325815633759,
127.004505847616));
#268071=CARTESIAN_POINT('Ctrl Pts',(-63.3292555868704,-0.276332420019459,
124.204532182646));
#268072=CARTESIAN_POINT('Ctrl Pts',(-63.6077032106833,-5.70198700196771,
127.469478429822));
#268073=CARTESIAN_POINT('Ctrl Pts',(-63.8861508344962,-5.8877940866586,
133.799018489484));
#268074=CARTESIAN_POINT('Ctrl Pts',(-64.1645984583092,-0.663006040441876,
137.376614262022));
#268075=CARTESIAN_POINT('Ctrl Pts',(-64.4430460821219,5.17105216729505,
134.914630007745));
#268076=CARTESIAN_POINT('Ctrl Pts',(-64.721493705935,6.25316605323042,128.675508981716));
#268077=CARTESIAN_POINT('Ctrl Pts',(-64.9999413297477,1.58892582039159,
124.392698608848));
#268078=CARTESIAN_POINT('Ctrl Pts',(-65.2783889535607,-4.53545961804555,
126.00189239489));
#268079=CARTESIAN_POINT('Ctrl Pts',(-65.5568365773735,-6.49197923701883,
132.024319863954));
#268080=CARTESIAN_POINT('Ctrl Pts',(-65.8352842011867,-2.48268708798906,
136.92566438391));
#268081=CARTESIAN_POINT('Ctrl Pts',(-66.1137318249993,3.80807320889562,
136.201829784909));
#268082=CARTESIAN_POINT('Ctrl Pts',(-66.3921794488124,6.59940026152389,
130.517984702147));
#268083=CARTESIAN_POINT('Ctrl Pts',(-66.6706270726251,3.3262008724376,125.097305095413));
#268084=CARTESIAN_POINT('Ctrl Pts',(-66.9490746964381,-3.00361462447264,
124.921130708376));
#268085=CARTESIAN_POINT('Ctrl Pts',(-67.227522320251,-6.57325501622426,
130.151357196124));
#268086=CARTESIAN_POINT('Ctrl Pts',(-67.5059699440638,-4.10239516942585,
135.981661927186));
#268087=CARTESIAN_POINT('Ctrl Pts',(-67.7844175678767,2.13836542492937,
137.054279679937));
#268088=CARTESIAN_POINT('Ctrl Pts',(-68.0628651916897,6.41407265873309,
132.383527139888));
#268089=CARTESIAN_POINT('Ctrl Pts',(-68.3413128155024,4.79556046403026,
126.261597712398));
#268090=CARTESIAN_POINT('Ctrl Pts',(-68.6197604393155,-1.22983752096341,
124.314245468451));
#268091=CARTESIAN_POINT('Ctrl Pts',(-68.8982080631282,-6.12507490509475,
128.330991986789));
#268092=CARTESIAN_POINT('Ctrl Pts',(-69.1766556869413,-5.39166767798822,
134.620643446035));
#268093=CARTESIAN_POINT('Ctrl Pts',(-69.455103310754,0.296418747580413,
137.403317421698));
#268094=CARTESIAN_POINT('Ctrl Pts',(-69.733550934567,5.7121108249834,134.121872471326));
#268095=CARTESIAN_POINT('Ctrl Pts',(-70.0119985583799,5.87865210635384,
127.791796196812));
#268096=CARTESIAN_POINT('Ctrl Pts',(-70.2904461821926,0.642999290106501,
124.230119453016));
#268097=CARTESIAN_POINT('Ctrl Pts',(-70.5688938060058,-5.18353846148724,
126.709849169906));
#268098=CARTESIAN_POINT('Ctrl Pts',(-70.8473414298183,-6.24665759690589,
132.95223487919));
#268099=CARTESIAN_POINT('Ctrl Pts',(-71.1257890536316,-1.56940356695681,
137.220829071533));
#268100=CARTESIAN_POINT('Ctrl Pts',(-71.4042366774442,4.55005567139915,
135.593002216589));
#268101=CARTESIAN_POINT('Ctrl Pts',(-71.6826843012574,6.48823603031619,
129.56464767029));
#268102=CARTESIAN_POINT('Ctrl Pts',(-71.9611319250699,2.46404444532374,
124.675528759193));
#268103=CARTESIAN_POINT('Ctrl Pts',(-72.2395795488831,-3.82448360965763,
125.418506915858));
#268104=CARTESIAN_POINT('Ctrl Pts',(-72.518027172696,-6.59849806377525,
131.110821510811));
#268105=CARTESIAN_POINT('Ctrl Pts',(-72.7964747965087,-3.30881515183405,
136.52151351632));
#268106=CARTESIAN_POINT('Ctrl Pts',(-73.0749224203217,3.02150724003593,
136.678421306317));
#268107=CARTESIAN_POINT('Ctrl Pts',(-73.3533700441346,6.57521208714753,
131.437354287172));
#268108=CARTESIAN_POINT('Ctrl Pts',(-73.6318176679474,4.08661824313884,
125.614597009117));
#268109=CARTESIAN_POINT('Ctrl Pts',(-73.9102652917603,-2.15737812391465,
124.56097895318));
#268110=CARTESIAN_POINT('Ctrl Pts',(-74.1887129155733,-6.41884938887091,
129.244723640663));
#268111=CARTESIAN_POINT('Ctrl Pts',(-74.4671605393861,-4.78171164368069,
135.361698517417));
#268112=CARTESIAN_POINT('Ctrl Pts',(-74.745608163199,1.24958550245192,137.290702502541));
#268113=CARTESIAN_POINT('Ctrl Pts',(-75.0240557870119,6.13257461747648,
133.25907517079));
#268114=CARTESIAN_POINT('Ctrl Pts',(-75.3025034108249,5.380027251966,126.971685084098));
#268115=CARTESIAN_POINT('Ctrl Pts',(-75.5809510346376,-0.31650232915867,
124.206336576053));
#268116=CARTESIAN_POINT('Ctrl Pts',(-75.8593986584506,-5.72218173178456,
127.504249830764));
#268117=CARTESIAN_POINT('Ctrl Pts',(-76.1378462822634,-5.86945566701928,
133.83480367917));
#268118=CARTESIAN_POINT('Ctrl Pts',(-76.4162939060764,-0.622986583113102,
137.380528399336));
#268119=CARTESIAN_POINT('Ctrl Pts',(-76.6947415298893,5.19597673608708,
134.88307619171));
#268120=CARTESIAN_POINT('Ctrl Pts',(-76.9731891537022,6.24009127239896,
128.637483627779));
#268121=CARTESIAN_POINT('Ctrl Pts',(-77.2516367775151,1.54986677478153,
124.383145159635));
#268122=CARTESIAN_POINT('Ctrl Pts',(-77.5300844013279,-4.56460957365852,
126.029590003516));
#268123=CARTESIAN_POINT('Ctrl Pts',(-77.8085320251407,-6.48443271748106,
132.063815781194));
#268124=CARTESIAN_POINT('Ctrl Pts',(-78.0869796489538,-2.44537897608793,
136.940663791305));
#268125=CARTESIAN_POINT('Ctrl Pts',(-78.3654272727665,3.84085858092573,
136.178548959823));
#268126=CARTESIAN_POINT('Ctrl Pts',(-78.6438748965796,6.5975347384416,130.477817585504));
#268127=CARTESIAN_POINT('Ctrl Pts',(-78.9223225203923,3.29139877882003,
125.077163305135));
#268128=CARTESIAN_POINT('Ctrl Pts',(-79.2007701442053,-3.03937186476788,
124.939523565746));
#268129=CARTESIAN_POINT('Ctrl Pts',(-79.4792177680182,-6.57710824620412,
130.191382563762));
#268130=CARTESIAN_POINT('Ctrl Pts',(-79.7576653918309,-4.07080345897965,
136.00653844758));
#268131=CARTESIAN_POINT('Ctrl Pts',(-80.036113015644,2.17637083724304,137.041147046131));
#268132=CARTESIAN_POINT('Ctrl Pts',(-80.314560639457,6.42356665566488,132.344453600785));
#268133=CARTESIAN_POINT('Ctrl Pts',(-80.5930082632696,4.76781852620778,
126.232489941585));
#268134=CARTESIAN_POINT('Ctrl Pts',(-80.8714558870828,-1.26932190795047,
124.321852085313));
#268135=CARTESIAN_POINT('Ctrl Pts',(-81.1499035108954,-6.14001751852468,
128.368322882032));
#268136=CARTESIAN_POINT('Ctrl Pts',(-81.4283511347085,-5.36833698610627,
134.653393350648));
#268137=CARTESIAN_POINT('Ctrl Pts',(-81.7067987585213,0.336582978702201,
137.401390773263));
#268138=CARTESIAN_POINT('Ctrl Pts',(-81.9852463823341,5.73219962907597,
134.087039765632));
#268139=CARTESIAN_POINT('Ctrl Pts',(-82.2636940061471,5.86020485384888,
127.756066988721));
#268140=CARTESIAN_POINT('Ctrl Pts',(-82.54214162996,0.602968104857597,124.226327139294));
#268141=CARTESIAN_POINT('Ctrl Pts',(-82.8205892537728,-5.20836687586887,
126.741478701599));
#268142=CARTESIAN_POINT('Ctrl Pts',(-83.0990368775859,-6.23346714053832,
132.990220261861));
#268143=CARTESIAN_POINT('Ctrl Pts',(-83.3774845013985,-1.53031562485268,
137.230263594196));
#268144=CARTESIAN_POINT('Ctrl Pts',(-83.6559321252116,4.57912118999838,
135.56521601382));
#268145=CARTESIAN_POINT('Ctrl Pts',(-83.9343797490243,6.48056933374724,
129.525174905002));
#268146=CARTESIAN_POINT('Ctrl Pts',(-84.2128273728376,2.42669085319518,
124.660642974335));
#268147=CARTESIAN_POINT('Ctrl Pts',(-84.4912749966499,-3.85719797100462,
125.441887420503));
#268148=CARTESIAN_POINT('Ctrl Pts',(-84.7697226204634,-6.59651029444787,
131.150982763393));
#268149=CARTESIAN_POINT('Ctrl Pts',(-85.0481702442759,-3.27395191473627,
136.541549287701));
#268150=CARTESIAN_POINT('Ctrl Pts',(-85.326617868089,3.05720833317481,136.659919701402));
#268151=CARTESIAN_POINT('Ctrl Pts',(-85.6050654919017,6.57894347582879,
131.397317377022));
#268152=CARTESIAN_POINT('Ctrl Pts',(-85.8835131157147,4.05495096345227,
125.58981675825));
#268153=CARTESIAN_POINT('Ctrl Pts',(-86.1619607395276,-2.19534338896908,
124.574227201559));
#268154=CARTESIAN_POINT('Ctrl Pts',(-86.4404083633404,-6.42822441541511,
129.283825895241));
#268155=CARTESIAN_POINT('Ctrl Pts',(-86.7188559871533,-4.75388124031539,
135.390721716488));
#268156=CARTESIAN_POINT('Ctrl Pts',(-86.9973036109663,1.28904655462414,
137.282975744021));
#268157=CARTESIAN_POINT('Ctrl Pts',(-87.2757512347791,6.14740353928957,
133.221698968287));
#268158=CARTESIAN_POINT('Ctrl Pts',(-87.554198858592,5.35659698870609,126.939006341782));
#268159=CARTESIAN_POINT('Ctrl Pts',(-87.8326464824051,-0.356660510187587,
124.208385461669));
#268160=CARTESIAN_POINT('Ctrl Pts',(-88.1110941062178,-5.74216442405318,
127.539143518524));
#268161=CARTESIAN_POINT('Ctrl Pts',(-88.3895417300309,-5.85089975254147,
133.870476574676));
#268162=CARTESIAN_POINT('Ctrl Pts',(-88.6679893538435,-0.582944040787213,
137.384198854334));
#268163=CARTESIAN_POINT('Ctrl Pts',(-88.9464369776566,5.22070876605056,
134.851371237371));
#268164=CARTESIAN_POINT('Ctrl Pts',(-89.2248846014694,6.22678526269035,
128.599538568266));
#268165=CARTESIAN_POINT('Ctrl Pts',(-89.5033322252823,1.51075029828878,
124.373829650922));
#268166=CARTESIAN_POINT('Ctrl Pts',(-89.7817798490951,-4.59359038598471,
126.057464543021));
#268167=CARTESIAN_POINT('Ctrl Pts',(-90.0602274729082,-6.47664591490472,
132.103265028861));
#268168=CARTESIAN_POINT('Ctrl Pts',(-90.338675096721,-2.40798024976945,
136.955435815729));
#268169=CARTESIAN_POINT('Ctrl Pts',(-90.6171227205338,3.87350162852866,
136.155068992212));
#268170=CARTESIAN_POINT('Ctrl Pts',(-90.8955703443469,6.59542474128344,
130.437662569033));
#268171=CARTESIAN_POINT('Ctrl Pts',(-91.1740179681596,3.25647472121003,
125.057233738258));
#268172=CARTESIAN_POINT('Ctrl Pts',(-91.4524655919725,-3.07501648002118,
124.958133746811));
#268173=CARTESIAN_POINT('Ctrl Pts',(-91.7309132157855,-6.58071775901922,
130.231430645527));
#268174=CARTESIAN_POINT('Ctrl Pts',(-92.0093608395982,-4.03906090341396,
136.031222199361));
#268175=CARTESIAN_POINT('Ctrl Pts',(-92.2878084634112,2.21429560333469,
137.027783305909));
#268176=CARTESIAN_POINT('Ctrl Pts',(-92.5662560872241,6.4328226249721,132.305322992969));
#268177=CARTESIAN_POINT('Ctrl Pts',(-92.844703711037,4.73989991511645,126.203551583122));
#268178=CARTESIAN_POINT('Ctrl Pts',(-93.1231513348499,-1.30875925974737,
124.329698913911));
#268179=CARTESIAN_POINT('Ctrl Pts',(-93.4015989586628,-6.15473261134757,
128.40574404555));
#268180=CARTESIAN_POINT('Ctrl Pts',(-93.6800465824757,-5.34480736852315,
134.686000627937));
#268181=CARTESIAN_POINT('Ctrl Pts',(-93.9584942062885,0.37673473761816,
137.399219669449));
#268182=CARTESIAN_POINT('Ctrl Pts',(-94.2369418301014,5.75207602440345,
134.052085419056));
#268183=CARTESIAN_POINT('Ctrl Pts',(-94.5153894539144,5.84154044929785,
127.720450736271));
#268184=CARTESIAN_POINT('Ctrl Pts',(-94.7938370777271,0.56291457640357,
124.222778577022));
#268185=CARTESIAN_POINT('Ctrl Pts',(-95.0722847015402,-5.23300229230026,
126.773258784876));
#268186=CARTESIAN_POINT('Ctrl Pts',(-95.350732325353,-6.22004570075364,
133.028124646699));
#268187=CARTESIAN_POINT('Ctrl Pts',(-95.6291799491659,-1.49117097634027,
137.239460002661));
#268188=CARTESIAN_POINT('Ctrl Pts',(-95.9076275729788,4.60801702757804,
135.537253395802));
#268189=CARTESIAN_POINT('Ctrl Pts',(-96.1860751967916,6.47266249729856,
129.48574954041));
#268190=CARTESIAN_POINT('Ctrl Pts',(-96.4645228206046,2.38924733914408,
124.645984847192));
#268191=CARTESIAN_POINT('Ctrl Pts',(-96.7429704444176,-3.88976940246256,
125.465466633565));
#268192=CARTESIAN_POINT('Ctrl Pts',(-97.0214180682302,-6.59427808900543,
131.191131171763));
#268193=CARTESIAN_POINT('Ctrl Pts',(-97.2998656920433,-3.23896736014657,
136.561372465446));
#268194=CARTESIAN_POINT('Ctrl Pts',(-97.5783133158561,3.09279614033489,
136.641201116591));
#268195=CARTESIAN_POINT('Ctrl Pts',(-97.856760939669,6.58243107933991,131.357258494642));
#268196=CARTESIAN_POINT('Ctrl Pts',(-98.135208563482,4.02313342606635,125.565229734223));
#268197=CARTESIAN_POINT('Ctrl Pts',(-98.4136561872948,-2.2332273047675,
124.587706309824));
#268198=CARTESIAN_POINT('Ctrl Pts',(-98.6921038111079,-6.43736124173946,
129.322984493793));
#268199=CARTESIAN_POINT('Ctrl Pts',(-98.9705514349205,-4.72587468013238,
135.419574966262));
#268200=CARTESIAN_POINT('Ctrl Pts',(-99.2489990587337,1.32845984070286,
137.275008918035));
#268201=CARTESIAN_POINT('Ctrl Pts',(-99.5274466825463,6.16200466680371,
133.184233190419));
#268202=CARTESIAN_POINT('Ctrl Pts',(-99.8058943063594,5.3329682347749,126.906470831589));
#268203=CARTESIAN_POINT('Ctrl Pts',(-100.084341930172,-0.396805475030165,
124.210678763569));
#268204=CARTESIAN_POINT('Ctrl Pts',(-100.362789553985,-5.76193433830736,
127.574158200105));
#268205=CARTESIAN_POINT('Ctrl Pts',(-100.641237177798,-5.83212703082168,
133.906035854126));
#268206=CARTESIAN_POINT('Ctrl Pts',(-100.919684801611,-0.542879897255484,
137.387625491007));
#268207=CARTESIAN_POINT('Ctrl Pts',(-101.198132425424,5.24524734073077,
134.819516319564));
#268208=CARTESIAN_POINT('Ctrl Pts',(-101.476580049237,6.21324851716398,
128.561675209245));
#268209=CARTESIAN_POINT('Ctrl Pts',(-101.75502767305,1.47157784038775,124.3647524279));
#268210=CARTESIAN_POINT('Ctrl Pts',(-102.033475296863,-4.62240098113028,
126.085514980508));
#268211=CARTESIAN_POINT('Ctrl Pts',(-102.311922920676,-6.4686191178319,
132.142666145147));
#268212=CARTESIAN_POINT('Ctrl Pts',(-102.590370544489,-2.3704922948573,
136.969979909799));
#268213=CARTESIAN_POINT('Ctrl Pts',(-102.868818168302,3.90600114210426,
136.131390752135));
#268214=CARTESIAN_POINT('Ctrl Pts',(-103.147265792114,6.59307034823604,
130.397521140692));
#268215=CARTESIAN_POINT('Ctrl Pts',(-103.425713415927,3.22142999373166,
125.037517133282));
#268216=CARTESIAN_POINT('Ctrl Pts',(-103.70416103974,-3.11054714940797,
124.976960561963));
#268217=CARTESIAN_POINT('Ctrl Pts',(-103.982608663553,-6.58408342091771,
130.271499957422));
#268218=CARTESIAN_POINT('Ctrl Pts',(-104.261056287366,-4.00716867896111,
136.055712267864));
#268219=CARTESIAN_POINT('Ctrl Pts',(-104.539503911179,2.25213831788793,
137.014188954471));
#268220=CARTESIAN_POINT('Ctrl Pts',(-104.817951534992,6.44184022367115,
132.266136766442));
#268221=CARTESIAN_POINT('Ctrl Pts',(-105.096399158805,4.71180566529118,
126.17478370933));
#268222=CARTESIAN_POINT('Ctrl Pts',(-105.374846782618,-1.34814811498862,
124.337785663482));
#268223=CARTESIAN_POINT('Ctrl Pts',(-105.65329440643,-6.16921963829011,
128.443254090687));
#268224=CARTESIAN_POINT('Ctrl Pts',(-105.931742030243,-5.32107969713743,
134.718464069627));
#268225=CARTESIAN_POINT('Ctrl Pts',(-106.210189654056,0.416872536489867,
137.396804190707));
#268226=CARTESIAN_POINT('Ctrl Pts',(-106.488637277869,5.77173927443855,
134.017010726842));
#268227=CARTESIAN_POINT('Ctrl Pts',(-106.767084901682,5.82265958431723,
127.684948759235));
#268228=CARTESIAN_POINT('Ctrl Pts',(-107.045532525495,0.52284018894291,
124.219473897692));
#268229=CARTESIAN_POINT('Ctrl Pts',(-107.323980149308,-5.25744379790729,
126.805188242113));
#268230=CARTESIAN_POINT('Ctrl Pts',(-107.602427773121,-6.20639377488812,
133.065946629143));
#268231=CARTESIAN_POINT('Ctrl Pts',(-107.880875396933,-1.45197107193893,
137.248417956151));
#268232=CARTESIAN_POINT('Ctrl Pts',(-108.159323020746,4.63674211339212,
135.509115398702));
#268233=CARTESIAN_POINT('Ctrl Pts',(-108.437770644559,6.46451581396073,
129.446373037437));
#268234=CARTESIAN_POINT('Ctrl Pts',(-108.716218268372,2.35171529065418,
124.631554920928));
#268235=CARTESIAN_POINT('Ctrl Pts',(-108.994665892185,-3.92219669708481,
125.489243681306));
#268236=CARTESIAN_POINT('Ctrl Pts',(-109.273113515998,-6.59180153016358,
131.231265248209));
#268237=CARTESIAN_POINT('Ctrl Pts',(-109.551561139811,-3.20386278442967,
136.580982315001));
#268238=CARTESIAN_POINT('Ctrl Pts',(-109.830008763624,3.12826934279688,
136.622266245509));
#268239=CARTESIAN_POINT('Ctrl Pts',(-110.108456387437,6.5856747684467,131.317179124427));
#268240=CARTESIAN_POINT('Ctrl Pts',(-110.38690401125,3.99116680999183,125.540836848117));
#268241=CARTESIAN_POINT('Ctrl Pts',(-110.665351635062,-2.27102846750687,
124.601415778499));
#268242=CARTESIAN_POINT('Ctrl Pts',(-110.943799258875,-6.44625952927566,
129.362197985281));
#268243=CARTESIAN_POINT('Ctrl Pts',(-111.222246882688,-4.69769300092514,
135.448257197571));
#268244=CARTESIAN_POINT('Ctrl Pts',(-111.500694506501,1.36782390021364,
137.266802319797));
#268245=CARTESIAN_POINT('Ctrl Pts',(-111.779142130314,6.17637745896884,
133.1466792255));
#268246=CARTESIAN_POINT('Ctrl Pts',(-112.057589754127,5.30914186574463,
126.874079759138));
#268247=CARTESIAN_POINT('Ctrl Pts',(-112.33603737794,-0.436935736099303,
124.213216396775));
#268248=CARTESIAN_POINT('Ctrl Pts',(-112.614485001753,-5.78149074196569,
127.609292578024));
#268249=CARTESIAN_POINT('Ctrl Pts',(-112.892932625565,-5.81313819748998,
133.94148019986));
#268250=CARTESIAN_POINT('Ctrl Pts',(-113.171380249379,-0.502795637109545,
137.390808182378));
#268251=CARTESIAN_POINT('Ctrl Pts',(-113.449827873191,5.26959155084185,
134.787512618686));
#268252=CARTESIAN_POINT('Ctrl Pts',(-113.728275497004,6.19948153742887,
128.523894953756));
#268253=CARTESIAN_POINT('Ctrl Pts',(-114.006723120817,1.43235085262869,
124.355913826926));
#268254=CARTESIAN_POINT('Ctrl Pts',(-114.28517074463,-4.65104029150761,
126.113740276555));
#268255=CARTESIAN_POINT('Ctrl Pts',(-114.563618368443,-6.46035262369882,
132.182017670029));
#268256=CARTESIAN_POINT('Ctrl Pts',(-114.842065992256,-2.33291650048142,
136.984295534578));
#268257=CARTESIAN_POINT('Ctrl Pts',(-115.120513616069,3.93835591737112,
136.107515116997));
#268258=CARTESIAN_POINT('Ctrl Pts',(-115.398961239881,6.59047164654225,
130.357394787938));
#268259=CARTESIAN_POINT('Ctrl Pts',(-115.677408863695,3.18626589498021,
125.018014220813));
#268260=CARTESIAN_POINT('Ctrl Pts',(-115.955856487507,-3.14596255632626,
124.996003313566));
#268261=CARTESIAN_POINT('Ctrl Pts',(-116.23430411132,-6.58720510718372,
130.311589014666));
#268262=CARTESIAN_POINT('Ctrl Pts',(-116.512751735133,-3.97512796739924,
136.0800077456));
#268263=CARTESIAN_POINT('Ctrl Pts',(-116.791199358946,2.28989757862811,
137.00036449556));
#268264=CARTESIAN_POINT('Ctrl Pts',(-117.069646982759,6.45061911761184,
132.226896373261));
#268265=CARTESIAN_POINT('Ctrl Pts',(-117.348094606572,4.68353681777373,
126.146187386213));
#268266=CARTESIAN_POINT('Ctrl Pts',(-117.626542230384,-1.38748701410568,
124.346112034364));
#268267=CARTESIAN_POINT('Ctrl Pts',(-117.904989854198,-6.18347806253024,
128.480851627495));
#268268=CARTESIAN_POINT('Ctrl Pts',(-118.18343747801,-5.29715485118671,
134.750782472776));
#268269=CARTESIAN_POINT('Ctrl Pts',(-118.461885101824,0.45699488799644,
137.394144426544));
#268270=CARTESIAN_POINT('Ctrl Pts',(-118.740332725636,5.79118865055225,
133.981816988697));
#268271=CARTESIAN_POINT('Ctrl Pts',(-119.018780349449,5.80356295854445,
127.649562373154));
#268272=CARTESIAN_POINT('Ctrl Pts',(-119.297227973262,0.482746427446748,
124.216413223762));
#268273=CARTESIAN_POINT('Ctrl Pts',(-119.575675597075,-5.28169048700048,
126.837265890154));
#268274=CARTESIAN_POINT('Ctrl Pts',(-119.854123220888,-6.19251186881905,
133.103684807684));
#268275=CARTESIAN_POINT('Ctrl Pts',(-120.132570844701,-1.41271736421608,
137.257137122728));
#268276=CARTESIAN_POINT('Ctrl Pts',(-120.411018468513,4.66529538302207,
135.480803065184));
#268277=CARTESIAN_POINT('Ctrl Pts',(-120.689466092327,6.45612958561205,
129.407046855192));
#268278=CARTESIAN_POINT('Ctrl Pts',(-120.967913716139,2.31409609848935,
124.61735373025));
#268279=CARTESIAN_POINT('Ctrl Pts',(-121.246361339953,-3.95447865326606,
125.51321768266));
#268280=CARTESIAN_POINT('Ctrl Pts',(-121.524808963765,-6.5890807096919,
131.271383505546));
#268281=CARTESIAN_POINT('Ctrl Pts',(-121.803256587578,-3.16863948839908,
136.600378109714));
#268282=CARTESIAN_POINT('Ctrl Pts',(-122.081704211391,3.16362662608795,
136.603115789794));
#268283=CARTESIAN_POINT('Ctrl Pts',(-122.360151835204,6.58867442295306,
131.277080751534));
#268284=CARTESIAN_POINT('Ctrl Pts',(-122.638599459017,3.9590522997634,125.51663900382));
#268285=CARTESIAN_POINT('Ctrl Pts',(-122.91704708283,-2.30874547645122,
124.615355099576));
#268286=CARTESIAN_POINT('Ctrl Pts',(-123.195494706643,-6.45491894829438,
129.401464916637));
#268287=CARTESIAN_POINT('Ctrl Pts',(-123.473942330455,-4.66933724697619,
135.476767347585));
#268288=CARTESIAN_POINT('Ctrl Pts',(-123.752389954268,1.40713727450679,
137.258356253404));
#268289=CARTESIAN_POINT('Ctrl Pts',(-124.030837578081,6.19052138319586,
133.109038465103));
#268290=CARTESIAN_POINT('Ctrl Pts',(-124.309285201894,5.28511876451003,
126.841834324687));
#268291=CARTESIAN_POINT('Ctrl Pts',(-124.587732825707,-0.477049806354697,
124.215998267256));
#268292=CARTESIAN_POINT('Ctrl Pts',(-124.86618044952,-5.80083291035842,
127.644545350364));
#268293=CARTESIAN_POINT('Ctrl Pts',(-125.144628073333,-5.79393395618462,
133.976808298475));
#268294=CARTESIAN_POINT('Ctrl Pts',(-125.423075697146,-0.462692745686338,
137.393746810514));
#268295=CARTESIAN_POINT('Ctrl Pts',(-125.701523320958,5.2937404943001,134.755361320645));
#268296=CARTESIAN_POINT('Ctrl Pts',(-125.979970944772,6.18548483362552,
128.486199201761));
#268297=CARTESIAN_POINT('Ctrl Pts',(-126.258418568584,1.39307078858202,
124.34731417552));
#268298=CARTESIAN_POINT('Ctrl Pts',(-126.536866192397,-4.67950725587653,
126.142139385264));
#268299=CARTESIAN_POINT('Ctrl Pts',(-126.81531381621,-6.45184673882346,
132.221318145323));
#268300=CARTESIAN_POINT('Ctrl Pts',(-127.093761440023,-2.29525425902701,
136.998382159598));
#268301=CARTESIAN_POINT('Ctrl Pts',(-127.372209063836,3.97056475541062,
136.083442971518));
#268302=CARTESIAN_POINT('Ctrl Pts',(-127.650656687649,6.58762873249828,
130.317284997668));
#268303=CARTESIAN_POINT('Ctrl Pts',(-127.929104311462,3.15098372797424,
124.998725723536));
#268304=CARTESIAN_POINT('Ctrl Pts',(-128.207551935275,-3.18126138844507,
125.015261295985));
#268305=CARTESIAN_POINT('Ctrl Pts',(-128.485999559087,-6.59008270214206,
130.351696331743));
#268306=CARTESIAN_POINT('Ctrl Pts',(-128.764447182901,-3.94293995600869,
136.104107732291));
#268307=CARTESIAN_POINT('Ctrl Pts',(-129.042894806713,2.32757198637139,
136.986310441447));
#268308=CARTESIAN_POINT('Ctrl Pts',(-129.321342430526,6.45915898148892,
132.187603267495));
#268309=CARTESIAN_POINT('Ctrl Pts',(-129.599790054339,4.6550944200771,126.117763673416));
#268310=CARTESIAN_POINT('Ctrl Pts',(-129.878237678152,-1.42677449938118,
124.354677718024));
#268311=CARTESIAN_POINT('Ctrl Pts',(-130.156685301965,-6.19750735571679,
128.518535262782));
#268312=CARTESIAN_POINT('Ctrl Pts',(-130.435132925778,-5.27303371721495,
134.782954639811));
#268313=CARTESIAN_POINT('Ctrl Pts',(-130.713580549591,0.497100305389368,
137.391240475519));
#268314=CARTESIAN_POINT('Ctrl Pts',(-130.992028173403,5.81042343204081,
133.946505508738));
#268315=CARTESIAN_POINT('Ctrl Pts',(-131.270475797217,5.78425127961196,
127.614292889281));
#268316=CARTESIAN_POINT('Ctrl Pts',(-131.548923421029,0.442634777604211,
124.213596668645));
#268317=CARTESIAN_POINT('Ctrl Pts',(-131.827371044842,-5.30574146111081,
126.869490540348));
#268318=CARTESIAN_POINT('Ctrl Pts',(-132.105818668655,-6.17840049694519,
133.141337783923));
#268319=CARTESIAN_POINT('Ctrl Pts',(-132.384266292468,-1.37341130773126,
137.265617179298));
#268320=CARTESIAN_POINT('Ctrl Pts',(-132.662713916281,4.69367577841589,
135.45231744437));
#268321=CARTESIAN_POINT('Ctrl Pts',(-132.941161540094,6.44750412300737,
129.367772450924));
#268322=CARTESIAN_POINT('Ctrl Pts',(-133.219609163907,2.27639115664257,
124.603381801387));
#268323=CARTESIAN_POINT('Ctrl Pts',(-133.49805678772,-3.98661407478655,
125.537387749261));
#268324=CARTESIAN_POINT('Ctrl Pts',(-133.776504411532,-6.58611572841139,
131.311484457178));
#268325=CARTESIAN_POINT('Ctrl Pts',(-134.054952035345,-3.13329877726696,
136.619559130867));
#268326=CARTESIAN_POINT('Ctrl Pts',(-134.333399659158,3.19886668003099,
136.583750459073));
#268327=CARTESIAN_POINT('Ctrl Pts',(-134.611847282971,6.59142993170542,
131.236964861823));
#268328=CARTESIAN_POINT('Ctrl Pts',(-134.890294906784,3.92679108539655,
125.492637097993));
#268329=CARTESIAN_POINT('Ctrl Pts',(-135.168742530597,-2.34637693398254,
124.629523756529));
#268330=CARTESIAN_POINT('Ctrl Pts',(-135.44719015441,-6.46333917791768,
129.440783832808));
#268331=CARTESIAN_POINT('Ctrl Pts',(-135.725637778223,-4.64080846901838,
135.505104359849));
#268332=CARTESIAN_POINT('Ctrl Pts',(-136.004085402036,1.44639850681073,
137.24967103183));
#268333=CARTESIAN_POINT('Ctrl Pts',(-136.282533025848,6.20443591537649,
133.07131230402));
#268334=CARTESIAN_POINT('Ctrl Pts',(-136.560980649661,5.26089982125598,
126.809735723105));
#268335=CARTESIAN_POINT('Ctrl Pts',(-136.839428273474,-0.517146199354053,
124.219024271924));
#268336=CARTESIAN_POINT('Ctrl Pts',(-137.117875897287,-5.81996012675442,
127.679915210822));
#268337=CARTESIAN_POINT('Ctrl Pts',(-137.3963235211,-5.77451501852576,134.012018840873));
#268338=CARTESIAN_POINT('Ctrl Pts',(-137.674771144913,-0.422572709013315,
137.396441266521));
#268339=CARTESIAN_POINT('Ctrl Pts',(-137.953218768726,5.31769327625758,
134.723063616821));
#268340=CARTESIAN_POINT('Ctrl Pts',(-138.231666392539,6.17125892440694,
128.448589350091));
#268341=CARTESIAN_POINT('Ctrl Pts',(-138.510114016352,1.35373910378499,
124.338953792345));
#268342=CARTESIAN_POINT('Ctrl Pts',(-138.788561640165,-4.70780081938319,
126.170711254294));
#268343=CARTESIAN_POINT('Ctrl Pts',(-139.067009263977,-6.44310177839452,
132.260566114734));
#268344=CARTESIAN_POINT('Ctrl Pts',(-139.34545688779,-2.25750696608163,
137.012239262869));
#268345=CARTESIAN_POINT('Ctrl Pts',(-139.623904511603,4.00262646271346,
136.059175207703));
#268346=CARTESIAN_POINT('Ctrl Pts',(-139.902352135416,6.5845417114487,130.277193256163));
#268347=CARTESIAN_POINT('Ctrl Pts',(-140.180799759229,3.11558480010749,
124.979652356196));
#268348=CARTESIAN_POINT('Ctrl Pts',(-140.459247383042,-3.21644233775325,
125.034733795609));
#268349=CARTESIAN_POINT('Ctrl Pts',(-140.737695006855,-6.59271609916233,
130.391820422461));
#268350=CARTESIAN_POINT('Ctrl Pts',(-141.016142630668,-3.91060583752806,
136.128011334905));
#268351=CARTESIAN_POINT('Ctrl Pts',(-141.294590254481,2.36516014507876,
136.97202731291));
#268352=CARTESIAN_POINT('Ctrl Pts',(-141.573037878293,6.46745949885459,
132.148258905163));
#268353=CARTESIAN_POINT('Ctrl Pts',(-141.851485502106,4.62647952614482,
126.089513624195));
#268354=CARTESIAN_POINT('Ctrl Pts',(-142.129933125919,-1.4660091150024,
124.363482397054));
#268355=CARTESIAN_POINT('Ctrl Pts',(-142.408380749732,-6.21130699798892,
128.556303600169));
#268356=CARTESIAN_POINT('Ctrl Pts',(-142.686828373545,-5.24871718904012,
134.814979378581));
#268357=CARTESIAN_POINT('Ctrl Pts',(-142.965275997358,0.537187302547703,
137.388092445238));
#268358=CARTESIAN_POINT('Ctrl Pts',(-143.243723621171,5.82944290615228,
133.911077595444));
#268359=CARTESIAN_POINT('Ctrl Pts',(-143.522171244983,5.76472526312116,
127.579141614542));
#268360=CARTESIAN_POINT('Ctrl Pts',(-143.800618868797,0.402506725767204,
124.21102433671));
#268361=CARTESIAN_POINT('Ctrl Pts',(-144.079066492609,-5.32959582902011,
126.901860998601));
#268362=CARTESIAN_POINT('Ctrl Pts',(-144.357514116423,-6.1640601821688,
133.178904162615));
#268363=CARTESIAN_POINT('Ctrl Pts',(-144.635961740235,-1.33405435898536,
137.27385781163));
#268364=CARTESIAN_POINT('Ctrl Pts',(-144.914409364048,4.72188224792766,
135.423659591808));
#268365=CARTESIAN_POINT('Ctrl Pts',(-145.192856987861,6.43863974576633,
129.328551279958));
#268366=CARTESIAN_POINT('Ctrl Pts',(-145.471304611674,2.23860186228433,
124.589639652074));
#268367=CARTESIAN_POINT('Ctrl Pts',(-145.749752235487,-4.01860177085642,
125.56175298548));
#268368=CARTESIAN_POINT('Ctrl Pts',(-146.0281998593,-6.58290669619051,131.35156661715));
#268369=CARTESIAN_POINT('Ctrl Pts',(-146.306647483113,-3.09784196059638,
136.638524667701));
#268370=CARTESIAN_POINT('Ctrl Pts',(-146.585095106925,3.2339881987928,136.564170970937));
#268371=CARTESIAN_POINT('Ctrl Pts',(-146.863542730738,6.59394119259793,
131.196832941802));
#268372=CARTESIAN_POINT('Ctrl Pts',(-147.141990354551,3.89438436234147,
125.468832020033));
#268373=CARTESIAN_POINT('Ctrl Pts',(-147.420437978364,-2.38392144565404,
124.643921224334));
#268374=CARTESIAN_POINT('Ctrl Pts',(-147.698885602177,-6.47151990613084,
129.480153276819));
#268375=CARTESIAN_POINT('Ctrl Pts',(-147.97733322599,-4.61210772419611,
135.533267184325));
#268376=CARTESIAN_POINT('Ctrl Pts',(-148.255780849803,1.48560614228611,
137.240746976909));
#268377=CARTESIAN_POINT('Ctrl Pts',(-148.534228473616,6.21812053990256,
133.033502140209));
#268378=CARTESIAN_POINT('Ctrl Pts',(-148.812676097428,5.23648593342438,
126.777785143819));
#268379=CARTESIAN_POINT('Ctrl Pts',(-149.091123721242,-0.557223429310831,
124.222294298654));
#268380=CARTESIAN_POINT('Ctrl Pts',(-149.369571345054,-5.83887168238761,
127.715400848752));
#268381=CARTESIAN_POINT('Ctrl Pts',(-149.648018968867,-5.75488210408933,
134.047110522317));
#268382=CARTESIAN_POINT('Ctrl Pts',(-149.92646659268,-0.382437013753756,
137.398891450554));
#268383=CARTESIAN_POINT('Ctrl Pts',(-150.204914216493,5.34144900913504,
134.690620704017));
#268384=CARTESIAN_POINT('Ctrl Pts',(-150.483361840306,6.15680433691945,
128.411066792389));
#268385=CARTESIAN_POINT('Ctrl Pts',(-150.761809464119,1.31435725568762,
124.330832987197));
#268386=CARTESIAN_POINT('Ctrl Pts',(-151.040257087932,-4.73591993359918,
126.199454824906));
#268387=CARTESIAN_POINT('Ctrl Pts',(-151.318704711745,-6.43411806645975,
132.299760123916));
#268388=CARTESIAN_POINT('Ctrl Pts',(-151.597152335558,-2.21967602038541,
137.025866330917));
#268389=CARTESIAN_POINT('Ctrl Pts',(-151.87559995937,4.03453985122072,136.034712724799));
#268390=CARTESIAN_POINT('Ctrl Pts',(-152.154047583183,6.58121069778455,
130.237121049039));
#268391=CARTESIAN_POINT('Ctrl Pts',(-152.432495206996,3.08007042310019,
124.960794825562));
#268392=CARTESIAN_POINT('Ctrl Pts',(-152.710942830809,-3.25150410060774,
125.054420090877));
#268393=CARTESIAN_POINT('Ctrl Pts',(-152.989390454622,-6.59510520066311,
130.431959800007));
#268394=CARTESIAN_POINT('Ctrl Pts',(-153.267838078435,-3.87812681010997,
136.151717667683));
#268395=CARTESIAN_POINT('Ctrl Pts',(-153.546285702248,2.40266066190714,
136.957515639215));
#268396=CARTESIAN_POINT('Ctrl Pts',(-153.824733326061,6.47552036213011,
132.108864744186));
#268397=CARTESIAN_POINT('Ctrl Pts',(-154.103180949873,4.59769319631231,
126.061438285362));
#268398=CARTESIAN_POINT('Ctrl Pts',(-154.381628573686,-1.50518940711724,
124.372525745196));
#268399=CARTESIAN_POINT('Ctrl Pts',(-154.660076197499,-6.22487647799626,
128.594155240135));
#268400=CARTESIAN_POINT('Ctrl Pts',(-154.938523821312,-5.22420616771914,
134.846855502398));
#268401=CARTESIAN_POINT('Ctrl Pts',(-155.216971445125,0.577254394032953,
137.384700452354));
#268402=CARTESIAN_POINT('Ctrl Pts',(-155.495419068938,5.84824636811312,
133.87553456161));
#268403=CARTESIAN_POINT('Ctrl Pts',(-155.773866692751,5.74498563261573,
127.544109851479));
#268404=CARTESIAN_POINT('Ctrl Pts',(-156.052314316564,0.362363758895462,
124.208696323275));
#268405=CARTESIAN_POINT('Ctrl Pts',(-156.330761940377,-5.353252706796,126.934376065411));
#268406=CARTESIAN_POINT('Ctrl Pts',(-156.60920956419,-6.14949145587554,
133.216382551721));
#268407=CARTESIAN_POINT('Ctrl Pts',(-156.887657188002,-1.29464797636456,
137.281858714364));
#268408=CARTESIAN_POINT('Ctrl Pts',(-157.166104811815,4.74991374635575,
135.394830569423));
#268409=CARTESIAN_POINT('Ctrl Pts',(-157.444552435628,6.42953678236183,
129.28938479565));
#268410=CARTESIAN_POINT('Ctrl Pts',(-157.723000059441,2.20072961571137,
124.576127791533));
#268411=CARTESIAN_POINT('Ctrl Pts',(-158.001447683254,-4.05044055615985,
125.586312488451));
#268412=CARTESIAN_POINT('Ctrl Pts',(-158.279895307067,-6.57945373194114,
131.391628500203));
#268413=CARTESIAN_POINT('Ctrl Pts',(-158.55834293088,-3.06227035225273,
136.657274017441));
#268414=CARTESIAN_POINT('Ctrl Pts',(-158.836790554693,3.2689898809326,136.54437805091));
#268415=CARTESIAN_POINT('Ctrl Pts',(-159.115238178505,6.59620811257463,
131.156686478575));
#268416=CARTESIAN_POINT('Ctrl Pts',(-159.393685802319,3.86183333144169,
125.445224652049));
#268417=CARTESIAN_POINT('Ctrl Pts',(-159.672133426131,-2.42137762023968,
124.658546969484));
#268418=CARTESIAN_POINT('Ctrl Pts',(-159.950581049944,-6.47946082979399,
129.519571789819));
#268419=CARTESIAN_POINT('Ctrl Pts',(-160.229028673757,-4.58323607602601,
135.56125477743));
#268420=CARTESIAN_POINT('Ctrl Pts',(-160.50747629757,1.52475872807955,137.231584419323));
#268421=CARTESIAN_POINT('Ctrl Pts',(-160.785923921383,6.23157474968534,
132.99560937474));
#268422=CARTESIAN_POINT('Ctrl Pts',(-161.064371545196,5.2118780056808,126.745983770767));
#268423=CARTESIAN_POINT('Ctrl Pts',(-161.342819169009,-0.597280011148509,
124.225808226271));
#268424=CARTESIAN_POINT('Ctrl Pts',(-161.621266792821,-5.85756687648338,
127.751000949223));
#268425=CARTESIAN_POINT('Ctrl Pts',(-161.899714416635,-5.73503594038016,
134.08208204247));
#268426=CARTESIAN_POINT('Ctrl Pts',(-162.178162040447,-0.342287147149402,
137.401097271823));
#268427=CARTESIAN_POINT('Ctrl Pts',(-162.45660966426,5.36500681265522,134.658033784415));
#268428=CARTESIAN_POINT('Ctrl Pts',(-162.735057288073,6.14212160678308,
128.373632919072));
#268429=CARTESIAN_POINT('Ctrl Pts',(-163.013504911886,1.27492670359879,
124.322952060995));
#268430=CARTESIAN_POINT('Ctrl Pts',(-163.291952535699,-4.76386355656041,
126.228369031995));
#268431=CARTESIAN_POINT('Ctrl Pts',(-163.570400159512,-6.42489593591386,
132.338898720518));
#268432=CARTESIAN_POINT('Ctrl Pts',(-163.848847783325,-2.18176282377798,
137.039262858781));
#268433=CARTESIAN_POINT('Ctrl Pts',(-164.127295407138,4.06630373837012,
136.010056429275));
#268434=CARTESIAN_POINT('Ctrl Pts',(-164.405743030951,6.57763581493773,
130.197069861187));
#268435=CARTESIAN_POINT('Ctrl Pts',(-164.684190654763,3.04444191295097,
124.942153830408));
#268436=CARTESIAN_POINT('Ctrl Pts',(-164.962638278576,-3.28644537778151,
125.074319452304));
#268437=CARTESIAN_POINT('Ctrl Pts',(-165.241085902389,-6.59724991811553,
130.472112977002));
#268438=CARTESIAN_POINT('Ctrl Pts',(-165.519533526202,-3.84550407727676,
136.175225852179));
#268439=CARTESIAN_POINT('Ctrl Pts',(-165.797981150015,2.44007214726114,
136.942775958099));
#268440=CARTESIAN_POINT('Ctrl Pts',(-166.076428773828,6.48334127261722,
132.069422244329));
#268441=CARTESIAN_POINT('Ctrl Pts',(-166.354876397641,4.56873649726763,
126.03353869726));
#268442=CARTESIAN_POINT('Ctrl Pts',(-166.633324021454,-1.54431392388507,
124.381807427344));
#268443=CARTESIAN_POINT('Ctrl Pts',(-166.911771645267,-6.23821529291649,
128.632088780075));
#268444=CARTESIAN_POINT('Ctrl Pts',(-167.19021926908,-5.19950156151742,
134.878581830081));
#268445=CARTESIAN_POINT('Ctrl Pts',(-167.468666892892,0.617300095144361,
137.381064622557));
#268446=CARTESIAN_POINT('Ctrl Pts',(-167.747114516705,5.86683312115408,
133.839877724298));
#268447=CARTESIAN_POINT('Ctrl Pts',(-168.025562140518,5.72503311955499,
127.509198898206));
#268448=CARTESIAN_POINT('Ctrl Pts',(-168.304009764331,0.32220736450136,
124.206612714607));
#268449=CARTESIAN_POINT('Ctrl Pts',(-168.582457388144,-5.37671121782417,
126.967034535923));
#268450=CARTESIAN_POINT('Ctrl Pts',(-168.860905011957,-6.1346948579149,
133.253771562468));
#268451=CARTESIAN_POINT('Ctrl Pts',(-169.13935263577,-1.25519362008691,
137.289619591024));
#268452=CARTESIAN_POINT('Ctrl Pts',(-169.417800259582,4.77776923498369,
135.365831445486));
#268453=CARTESIAN_POINT('Ctrl Pts',(-169.696247883396,6.42019557010726,
129.250274449328));
#268454=CARTESIAN_POINT('Ctrl Pts',(-169.974695507208,2.16277582029264,
124.562846720449));
#268455=CARTESIAN_POINT('Ctrl Pts',(-170.253143131021,-4.08212925089891,
125.611065348116));
#268456=CARTESIAN_POINT('Ctrl Pts',(-170.531590754834,-6.57575696361412,
131.431668621828));
#268457=CARTESIAN_POINT('Ctrl Pts',(-170.810038378647,-3.02658527035502,
136.675806485322));
#268458=CARTESIAN_POINT('Ctrl Pts',(-171.08848600246,3.30387042945021,136.524372432426));
#268459=CARTESIAN_POINT('Ctrl Pts',(-171.366933626273,6.59823060763395,
131.116526959784));
#268460=CARTESIAN_POINT('Ctrl Pts',(-171.645381250086,3.82913919888762,
125.421815868818));
#268461=CARTESIAN_POINT('Ctrl Pts',(-171.923828873899,-2.45874406978715,
124.673400450021));
#268462=CARTESIAN_POINT('Ctrl Pts',(-172.202276497711,-6.48716165465291,
129.559037911142));
#268463=CARTESIAN_POINT('Ctrl Pts',(-172.480724121525,-4.55419459435809,
135.589066102071));
#268464=CARTESIAN_POINT('Ctrl Pts',(-172.759171745337,1.5638548133772,137.222183698596));
#268465=CARTESIAN_POINT('Ctrl Pts',(-173.03761936915,6.24479804617409,132.957635411742));
#268466=CARTESIAN_POINT('Ctrl Pts',(-173.316066992963,5.18707694988104,
126.714332782362));
#268467=CARTESIAN_POINT('Ctrl Pts',(-173.594514616776,-0.637314460555731,
124.229565924566));
#268468=CARTESIAN_POINT('Ctrl Pts',(-173.872962240589,-5.8760450162844,
127.786714193059));
#268469=CARTESIAN_POINT('Ctrl Pts',(-174.151409864401,-5.71497726280517,
134.11693210545));
#268470=CARTESIAN_POINT('Ctrl Pts',(-174.429857488215,-0.302124596968923,
137.403058648589));
#268471=CARTESIAN_POINT('Ctrl Pts',(-174.708305112027,5.38836581387496,
134.625304065538));
#268472=CARTESIAN_POINT('Ctrl Pts',(-174.98675273584,6.1272112780718,128.336289117263));
#268473=CARTESIAN_POINT('Ctrl Pts',(-175.265200359654,1.2354489086321,124.315311305772));
#268474=CARTESIAN_POINT('Ctrl Pts',(-175.543647983466,-4.79163065280562,
126.257452804136));
#268475=CARTESIAN_POINT('Ctrl Pts',(-175.822095607279,-6.41543572848632,
132.377980454247));
#268476=CARTESIAN_POINT('Ctrl Pts',(-176.100543231092,-2.14376878114676,
137.05242835005));
#268477=CARTESIAN_POINT('Ctrl Pts',(-176.378990854905,4.09791694713909,
135.985207234778));
#268478=CARTESIAN_POINT('Ctrl Pts',(-176.657438478718,6.57381719537689,
130.157041176716));
#268479=CARTESIAN_POINT('Ctrl Pts',(-176.93588610253,3.00870058988678,124.923730061481));
#268480=CARTESIAN_POINT('Ctrl Pts',(-177.214333726344,-3.32126487451375,
125.094431142515));
#268481=CARTESIAN_POINT('Ctrl Pts',(-177.492781350156,-6.59915017204588,
130.512278465557));
#268482=CARTESIAN_POINT('Ctrl Pts',(-177.771228973969,-3.81273884787578,
136.198535017289));
#268483=CARTESIAN_POINT('Ctrl Pts',(-178.049676597782,2.47739321484437,
136.927808815745));
#268484=CARTESIAN_POINT('Ctrl Pts',(-178.328124221595,6.49092194050925,
132.029932867148));
#268485=CARTESIAN_POINT('Ctrl Pts',(-178.606571845408,4.53961050201187,
126.005815893719));
#268486=CARTESIAN_POINT('Ctrl Pts',(-178.885019469221,-1.58338121553252,
124.391327099562));
#268487=CARTESIAN_POINT('Ctrl Pts',(-179.163467093034,-6.25132294847495,
128.670102814346));
#268488=CARTESIAN_POINT('Ctrl Pts',(-179.441914716847,-5.1746042858732,
134.910157185999));
#268489=CARTESIAN_POINT('Ctrl Pts',(-179.72036234066,0.657322921973241,
137.377185090575));
#268490=CARTESIAN_POINT('Ctrl Pts',(-179.998809964472,5.88520247653593,
133.804108404782));
#268491=CARTESIAN_POINT('Ctrl Pts',(-180.277257588285,5.70486846328706,
127.474410048364));
#268492=CARTESIAN_POINT('Ctrl Pts',(-180.555705212098,0.282039030594865,
124.204773587913));
#268493=CARTESIAN_POINT('Ctrl Pts',(-180.834152835911,-5.39997049284089,
126.999835199963));
#268494=CARTESIAN_POINT('Ctrl Pts',(-181.112600459724,-6.11967093658025,
133.291069809391));
#268495=CARTESIAN_POINT('Ctrl Pts',(-181.391048083537,-1.21569275214809,
137.297140154028));
#268496=CARTESIAN_POINT('Ctrl Pts',(-181.669495707349,4.8054476816156,135.336663294571));
#268497=CARTESIAN_POINT('Ctrl Pts',(-181.947943331163,6.41061645514481,
129.21122169024));
#268498=CARTESIAN_POINT('Ctrl Pts',(-182.226390954976,2.12474188242055,
124.549796930959));
#268499=CARTESIAN_POINT('Ctrl Pts',(-182.504838578788,-4.11366668083735,
125.636010647245));
#268500=CARTESIAN_POINT('Ctrl Pts',(-182.783286202602,-6.5718165281946,
131.471685498325));
#268501=CARTESIAN_POINT('Ctrl Pts',(-183.061733826414,-2.99078803722709,
136.694121384618));
#268502=CARTESIAN_POINT('Ctrl Pts',(-183.340181450227,3.33862855183402,
136.5041548568));
#268503=CARTESIAN_POINT('Ctrl Pts',(-183.61862907404,6.60000860283161,131.076355873553));
#268504=CARTESIAN_POINT('Ctrl Pts',(-183.897076697853,3.79630317617236,
125.398606537762));
#268505=CARTESIAN_POINT('Ctrl Pts',(-184.175524321666,-2.49601940966891,
124.68848111554));
#268506=CARTESIAN_POINT('Ctrl Pts',(-184.453971945479,-6.49462209535141,
129.598550178357));
#268507=CARTESIAN_POINT('Ctrl Pts',(-184.732419569291,-4.52498435533419,
135.616700127691));
#268508=CARTESIAN_POINT('Ctrl Pts',(-185.010867193105,1.60289294946002,
137.212545163075));
#268509=CARTESIAN_POINT('Ctrl Pts',(-185.289314816917,6.25778993937471,
132.919581658354));
#268510=CARTESIAN_POINT('Ctrl Pts',(-185.56776244073,5.16208368503734,126.682833351442));
#268511=CARTESIAN_POINT('Ctrl Pts',(-185.846210064543,-0.677325294041226,
124.233567254297));
#268512=CARTESIAN_POINT('Ctrl Pts',(-186.124657688356,-5.89430541707644,
127.822539256894));
#268513=CARTESIAN_POINT('Ctrl Pts',(-186.403105312169,-5.69470681464601,
134.151659419877));
#268514=CARTESIAN_POINT('Ctrl Pts',(-186.681552935982,-0.261950851450417,
137.404775508174));
#268515=CARTESIAN_POINT('Ctrl Pts',(-186.960000559794,5.41152514721792,
134.592432760195));
#268516=CARTESIAN_POINT('Ctrl Pts',(-187.238448183608,6.11207390329327,
128.299036770752));
#268517=CARTESIAN_POINT('Ctrl Pts',(-187.51689580742,1.19592533365239,124.307911004657));
#268518=CARTESIAN_POINT('Ctrl Pts',(-187.795343431234,-4.81922019341476,
126.286705063617));
#268519=CARTESIAN_POINT('Ctrl Pts',(-188.073791055046,-6.40573779472858,
132.417003876913));
#268520=CARTESIAN_POINT('Ctrl Pts',(-188.352238678859,-2.10569530037498,
137.065362316871));
#268521=CARTESIAN_POINT('Ctrl Pts',(-188.630686302672,4.12937830608858,
135.960166062105));
#268522=CARTESIAN_POINT('Ctrl Pts',(-188.909133926485,6.56975498060235,
130.117036478904));
#268523=CARTESIAN_POINT('Ctrl Pts',(-189.187581550298,2.97284777831579,
124.905524201484));
#268524=CARTESIAN_POINT('Ctrl Pts',(-189.466029174111,-3.35596130055467,
125.114754416262));
#268525=CARTESIAN_POINT('Ctrl Pts',(-189.744476797923,-6.60080589203976,
130.552454777323));
#268526=CARTESIAN_POINT('Ctrl Pts',(-190.022924421737,-3.77983233603489,
136.221644299282));
#268527=CARTESIAN_POINT('Ctrl Pts',(-190.301372045549,2.5146224817104,136.912614766765));
#268528=CARTESIAN_POINT('Ctrl Pts',(-190.579819669362,6.49826208490189,
131.990398075938));
#268529=CARTESIAN_POINT('Ctrl Pts',(-190.858267293175,4.51031628981952,
125.978270902017));
#268530=CARTESIAN_POINT('Ctrl Pts',(-191.136714916988,-1.62238983440674,
124.401084409096));
#268531=CARTESIAN_POINT('Ctrl Pts',(-191.415162540801,-6.26419895896261,
128.708195934325));
#268532=CARTESIAN_POINT('Ctrl Pts',(-191.693610164614,-5.14951526336424,
134.941580400114));
#268533=CARTESIAN_POINT('Ctrl Pts',(-191.972057788427,0.697321391460013,
137.373062000163));
#268534=CARTESIAN_POINT('Ctrl Pts',(-192.25050541224,5.90335375357599,133.768227928508));
#268535=CARTESIAN_POINT('Ctrl Pts',(-192.528953036052,5.68449241101982,
127.439744591064));
#268536=CARTESIAN_POINT('Ctrl Pts',(-192.807400659866,0.241860245628379,
124.203179011344));
#268537=CARTESIAN_POINT('Ctrl Pts',(-193.085848283678,-5.42302966996514,
127.032776842093));
#268538=CARTESIAN_POINT('Ctrl Pts',(-193.364295907491,-6.10442024858855,
133.32827591039));
#268539=CARTESIAN_POINT('Ctrl Pts',(-193.642743531304,-1.17614683626724,
137.304420124699));
#268540=CARTESIAN_POINT('Ctrl Pts',(-193.921191155117,4.83294806061645,
135.307327197512));
#268541=CARTESIAN_POINT('Ctrl Pts',(-194.19963877893,6.40079979243214,129.172227965502));
#268542=CARTESIAN_POINT('Ctrl Pts',(-194.478086402743,2.08662921145659,
124.536978906625));
#268543=CARTESIAN_POINT('Ctrl Pts',(-194.756534026555,-4.14505167734362,
125.661147461485));
#268544=CARTESIAN_POINT('Ctrl Pts',(-195.034981650369,-6.5676325716969,
131.511677646851));
#268545=CARTESIAN_POINT('Ctrl Pts',(-195.313429274181,-2.95487997934909,
136.712218036662));
#268546=CARTESIAN_POINT('Ctrl Pts',(-195.591876897994,3.3732629601091,136.483726073203));
#268547=CARTESIAN_POINT('Ctrl Pts',(-195.870324521807,6.60154203228333,
131.03617470844));
#268548=CARTESIAN_POINT('Ctrl Pts',(-196.14877214562,3.76332648004682,125.375597518911));
#268549=CARTESIAN_POINT('Ctrl Pts',(-196.427219769433,-2.53320225863353,
124.703788407225));
#268550=CARTESIAN_POINT('Ctrl Pts',(-196.705667393246,-6.50184187543975,
129.63810712732));
#268551=CARTESIAN_POINT('Ctrl Pts',(-196.984115017059,-4.49560644135098,
135.644155830301));
#268552=CARTESIAN_POINT('Ctrl Pts',(-197.262562640871,1.64187168975517,
137.202669169918));
#268553=CARTESIAN_POINT('Ctrl Pts',(-197.541010264685,6.27054994786743,
132.881449524674));
#268554=CARTESIAN_POINT('Ctrl Pts',(-197.819457888497,5.13689913728475,
126.651486645231));
#268555=CARTESIAN_POINT('Ctrl Pts',(-198.097905512311,-0.717311028988463,
124.237812067191));
#268556=CARTESIAN_POINT('Ctrl Pts',(-198.376353136123,-5.91234740221361,
127.858474813215));
#268557=CARTESIAN_POINT('Ctrl Pts',(-198.654800759936,-5.67422534703162,
134.186262698915));
#268558=CARTESIAN_POINT('Ctrl Pts',(-198.933248383749,-0.221767399246752,
137.406247786956));
#268559=CARTESIAN_POINT('Ctrl Pts',(-199.211696007562,5.43448395450644,
134.559421086446));
#268560=CARTESIAN_POINT('Ctrl Pts',(-199.490143631375,6.09671004336861,
128.261877259937));
#268561=CARTESIAN_POINT('Ctrl Pts',(-199.768591255188,1.15635744321901,
124.300751431872));
#268562=CARTESIAN_POINT('Ctrl Pts',(-200.047038879001,-4.84663115604747,
126.316124726487));
#268563=CARTESIAN_POINT('Ctrl Pts',(-200.325486502814,-6.39580249400115,
132.455967542492));
#268564=CARTESIAN_POINT('Ctrl Pts',(-200.603934126626,-2.06754379228947,
137.078064279972));
#268565=CARTESIAN_POINT('Ctrl Pts',(-200.882381750439,4.16068664940635,
135.934933839164));
#268566=CARTESIAN_POINT('Ctrl Pts',(-201.160829374253,6.56544932114097,
130.077057250143));
#268567=CARTESIAN_POINT('Ctrl Pts',(-201.439276998065,2.9368848067771,124.887536925038));
#268568=CARTESIAN_POINT('Ctrl Pts',(-201.717724621878,-3.39053337021544,
125.13528852046));
#268569=CARTESIAN_POINT('Ctrl Pts',(-201.996172245691,-6.60221701674386,
130.592640423553));
#268570=CARTESIAN_POINT('Ctrl Pts',(-202.274619869504,-3.74678576111652,
136.244552841837));
#268571=CARTESIAN_POINT('Ctrl Pts',(-202.553067493317,2.55175856831618,
136.897194374181));
#268572=CARTESIAN_POINT('Ctrl Pts',(-202.83151511713,6.50536143380309,131.950819335672));
#268573=CARTESIAN_POINT('Ctrl Pts',(-203.109962740942,4.48085494619837,
125.950904742844));
#268574=CARTESIAN_POINT('Ctrl Pts',(-203.388410364755,-1.66133833502902,
124.411078994385));
#268575=CARTESIAN_POINT('Ctrl Pts',(-203.666857988568,-6.27684284725421,
128.746366728457));
#268576=CARTESIAN_POINT('Ctrl Pts',(-203.945305612381,-5.12423542367342,
134.97285030803));
#268577=CARTESIAN_POINT('Ctrl Pts',(-204.223753236194,0.737294021446153,
137.368695504108));
#268578=CARTESIAN_POINT('Ctrl Pts',(-204.502200860007,5.9212862796718,133.732237625041));
#268579=CARTESIAN_POINT('Ctrl Pts',(-204.78064848382,5.66390571779574,127.405203810847));
#268580=CARTESIAN_POINT('Ctrl Pts',(-205.059096107633,0.20167249844203,
124.201829043986));
#268581=CARTESIAN_POINT('Ctrl Pts',(-205.337543731446,-5.44588789473034,
127.065858241646));
#268582=CARTESIAN_POINT('Ctrl Pts',(-205.615991355258,-6.08894335906002,
133.36538848678));
#268583=CARTESIAN_POINT('Ctrl Pts',(-205.894438979071,-1.13655733783284,
137.311459233274));
#268584=CARTESIAN_POINT('Ctrl Pts',(-206.172886602884,4.86026935294961,
135.277824241371));
#268585=CARTESIAN_POINT('Ctrl Pts',(-206.451334226697,6.39074594572923,
129.133294720038));
#268586=CARTESIAN_POINT('Ctrl Pts',(-206.72978185051,2.04843921967989,124.524393122426));
#268587=CARTESIAN_POINT('Ctrl Pts',(-207.008229474323,-4.17628307743617,
125.686474859378));
#268588=CARTESIAN_POINT('Ctrl Pts',(-207.286677098136,-6.56320524915893,
131.551643585487));
#268589=CARTESIAN_POINT('Ctrl Pts',(-207.565124721949,-2.9188624273063,
136.730095770877));
#268590=CARTESIAN_POINT('Ctrl Pts',(-207.843572345762,3.40777237088467,
136.463086838631));
#268591=CARTESIAN_POINT('Ctrl Pts',(-208.122019969575,6.60283083916734,
130.995984953369));
#268592=CARTESIAN_POINT('Ctrl Pts',(-208.400467593387,3.73021033247459,
125.352789664874));
#268593=CARTESIAN_POINT('Ctrl Pts',(-208.678915217201,-2.57029123885685,
124.719321757855));
#268594=CARTESIAN_POINT('Ctrl Pts',(-208.957362841013,-6.50882072738636,
129.677707292235));
#268595=CARTESIAN_POINT('Ctrl Pts',(-209.235810464827,-4.4660619410178,
135.671432192519));
#268596=CARTESIAN_POINT('Ctrl Pts',(-209.514258088639,1.68078958989102,
137.192556085085));
#268597=CARTESIAN_POINT('Ctrl Pts',(-209.792705712452,6.28307759882623,
132.8432404237));
#268598=CARTESIAN_POINT('Ctrl Pts',(-210.071153336265,5.11152423984512,
126.620293825292));
#268599=CARTESIAN_POINT('Ctrl Pts',(-210.349600960078,-0.757270183712145,
124.242300205957));
#268600=CARTESIAN_POINT('Ctrl Pts',(-210.62804858389,-5.93017030314353,
127.894519530418));
#268601=CARTESIAN_POINT('Ctrl Pts',(-210.906496207704,-5.65353361891029,
134.220740660327));
#268602=CARTESIAN_POINT('Ctrl Pts',(-211.184943831516,-0.181575729370575,
137.407475430382));
#268603=CARTESIAN_POINT('Ctrl Pts',(-211.463391455329,5.4572413849935,134.52627026755));
#268604=CARTESIAN_POINT('Ctrl Pts',(-211.741839079142,6.08112026761121,
128.224811961777));
#268605=CARTESIAN_POINT('Ctrl Pts',(-212.020286702955,1.11674670353533,
124.293832852717));
#268606=CARTESIAN_POINT('Ctrl Pts',(-212.298734326768,-4.87386252498038,
126.345710702588));
#268607=CARTESIAN_POINT('Ctrl Pts',(-212.577181950581,-6.38563019446009,
132.494870007167));
#268608=CARTESIAN_POINT('Ctrl Pts',(-212.855629574394,-2.02931567060901,
137.090533768676));
#268609=CARTESIAN_POINT('Ctrl Pts',(-213.134077198207,4.19184081695006,
135.909511500946));
#268610=CARTESIAN_POINT('Ctrl Pts',(-213.412524822019,6.56090037654053,
130.037104971874));
#268611=CARTESIAN_POINT('Ctrl Pts',(-213.690972445832,2.90081300789186,
124.869768898671));
#268612=CARTESIAN_POINT('Ctrl Pts',(-213.969420069645,-3.42497980241531,
125.156032694208));
#268613=CARTESIAN_POINT('Ctrl Pts',(-214.247867693459,-6.60338349386843,
130.632833915152));
#268614=CARTESIAN_POINT('Ctrl Pts',(-214.52631531727,-3.71360034767391,
136.267259796069));
#268615=CARTESIAN_POINT('Ctrl Pts',(-214.804762941084,2.58880009856982,
136.881548209402));
#268616=CARTESIAN_POINT('Ctrl Pts',(-215.083210564897,6.51221972414398,
131.911198112957));
#268617=CARTESIAN_POINT('Ctrl Pts',(-215.36165818871,4.45122756284936,125.923718430264));
#268618=CARTESIAN_POINT('Ctrl Pts',(-215.640105812523,-1.70022527414834,
124.421310485075));
#268619=CARTESIAN_POINT('Ctrl Pts',(-215.918553436335,-6.28925414482577,
128.784613782311));
#268620=CARTESIAN_POINT('Ctrl Pts',(-216.197001060149,-5.09876570355457,
135.003965751026));
#268621=CARTESIAN_POINT('Ctrl Pts',(-216.475448683961,0.77723933073121,
137.364085764208));
#268622=CARTESIAN_POINT('Ctrl Pts',(-216.753896307774,5.93899939032692,
133.696138828015));
#268623=CARTESIAN_POINT('Ctrl Pts',(-217.032343931587,5.64310914646246,
127.370788987637));
#268624=CARTESIAN_POINT('Ctrl Pts',(-217.3107915554,0.161477278206604,124.200723735865));
#268625=CARTESIAN_POINT('Ctrl Pts',(-217.589239179213,-5.46854432011718,
127.099078172778));
#268626=CARTESIAN_POINT('Ctrl Pts',(-217.867686803026,-6.07324084149572,
133.402406163341));
#268627=CARTESIAN_POINT('Ctrl Pts',(-218.146134426838,-1.09692572384833,
137.318257218917));
#268628=CARTESIAN_POINT('Ctrl Pts',(-218.424582050652,4.88741054621452,
135.24815551939));
#268629=CARTESIAN_POINT('Ctrl Pts',(-218.703029674464,6.38045528758512,
129.094423396537));
#268630=CARTESIAN_POINT('Ctrl Pts',(-218.981477298277,2.01017332223456,
124.512040044732));
#268631=CARTESIAN_POINT('Ctrl Pts',(-219.25992492209,-4.20735972382344,
125.711991902411));
#268632=CARTESIAN_POINT('Ctrl Pts',(-219.538372545903,-6.55853472463687,
131.591581833275));
#268633=CARTESIAN_POINT('Ctrl Pts',(-219.816820169716,-2.8827367157428,
136.747753924796));
#268634=CARTESIAN_POINT('Ctrl Pts',(-220.095267793529,3.44215550540127,
136.442237917877));
#268635=CARTESIAN_POINT('Ctrl Pts',(-220.373715417342,6.60387497572639,
130.955788097589));
#268636=CARTESIAN_POINT('Ctrl Pts',(-220.652163041155,3.69695596058723,
125.330183820803));
#268637=CARTESIAN_POINT('Ctrl Pts',(-220.930610664968,-2.60728497599312,
124.735080591838));
#268638=CARTESIAN_POINT('Ctrl Pts',(-221.20905828878,-6.51555839258729,
129.717349205704));
#268639=CARTESIAN_POINT('Ctrl Pts',(-221.487505912593,-4.43635194911701,
135.698528203611));
#268640=CARTESIAN_POINT('Ctrl Pts',(-221.765953536406,1.71964520775051,
137.182206283321));
#268641=CARTESIAN_POINT('Ctrl Pts',(-222.044401160219,6.295372428034,132.804955771283));
#268642=CARTESIAN_POINT('Ctrl Pts',(-222.322848784032,5.08595993299503,
126.589256047487));
#268643=CARTESIAN_POINT('Ctrl Pts',(-222.601296407845,-0.797201277510683,
124.247031504286));
#268644=CARTESIAN_POINT('Ctrl Pts',(-222.879744031658,-5.94777345943203,
127.930672072853));
#268645=CARTESIAN_POINT('Ctrl Pts',(-223.158191655471,-5.63263239702162,
134.255092026522));
#268646=CARTESIAN_POINT('Ctrl Pts',(-223.436639279283,-0.141377331138957,
137.40845839296));
#268647=CARTESIAN_POINT('Ctrl Pts',(-223.715086903097,5.47979659539413,
134.492981531924));
#268648=CARTESIAN_POINT('Ctrl Pts',(-223.993534526909,6.06530515370598,
128.187842249741));
#268649=CARTESIAN_POINT('Ctrl Pts',(-224.271982150722,1.07709458239186,
124.287155523561));
#268650=CARTESIAN_POINT('Ctrl Pts',(-224.550429774535,-4.90091329114502,
126.375461895601));
#268651=CARTESIAN_POINT('Ctrl Pts',(-224.828877398348,-6.37522127304402,
132.533709829396));
#268652=CARTESIAN_POINT('Ctrl Pts',(-225.107325022161,-1.99101235188949,
137.102770320923));
#268653=CARTESIAN_POINT('Ctrl Pts',(-225.385772645974,4.22283965429091,
135.883899989486));
#268654=CARTESIAN_POINT('Ctrl Pts',(-225.664220269787,6.55610831536389,
129.997181124546));
#268655=CARTESIAN_POINT('Ctrl Pts',(-225.9426678936,2.86463371831382,124.852220780782));
#268656=CARTESIAN_POINT('Ctrl Pts',(-226.221115517412,-3.45929932072906,
125.176986168825));
#268657=CARTESIAN_POINT('Ctrl Pts',(-226.499563141226,-6.60430528018926,
130.673033762736));
#268658=CARTESIAN_POINT('Ctrl Pts',(-226.778010765038,-3.68027732540471,
136.289764320562));
#268659=CARTESIAN_POINT('Ctrl Pts',(-227.056458388851,2.62574569988376,
136.865676852203));
#268660=CARTESIAN_POINT('Ctrl Pts',(-227.334906012664,6.51883670178814,
131.871535875972));
#268661=CARTESIAN_POINT('Ctrl Pts',(-227.613353636477,4.42143523762624,
125.896712971676));
#268662=CARTESIAN_POINT('Ctrl Pts',(-227.89180126029,-1.73904921079426,
124.431778502036));
#268663=CARTESIAN_POINT('Ctrl Pts',(-228.170248884103,-6.30143239177224,
128.822935678624));
#268664=CARTESIAN_POINT('Ctrl Pts',(-228.448696507916,-5.07310704679746,
135.034925576111));
#268665=CARTESIAN_POINT('Ctrl Pts',(-228.727144131728,0.81715583912702,
137.359232951281));
#268666=CARTESIAN_POINT('Ctrl Pts',(-229.005591755541,5.95649242917557,
133.659932875084));
#268667=CARTESIAN_POINT('Ctrl Pts',(-229.284039379354,5.62210346764449,
127.336501396687));
#268668=CARTESIAN_POINT('Ctrl Pts',(-229.562487003167,0.121276074371264,
124.199863127936));
#268669=CARTESIAN_POINT('Ctrl Pts',(-229.84093462698,-5.4909981065832,127.132435404515));
#268670=CARTESIAN_POINT('Ctrl Pts',(-230.119382250793,-6.0573132777586,
133.439327568368));
#268671=CARTESIAN_POINT('Ctrl Pts',(-230.397829874606,-1.05725346287773,
137.324813829725));
#268672=CARTESIAN_POINT('Ctrl Pts',(-230.676277498418,4.91437063468431,
135.218322130955));
#268673=CARTESIAN_POINT('Ctrl Pts',(-230.954725122232,6.3699281993239,129.055615435388));
#268674=CARTESIAN_POINT('Ctrl Pts',(-231.233172746044,1.97183293707754,
124.49992013129));
#268675=CARTESIAN_POINT('Ctrl Pts',(-231.511620369858,-4.23828046494889,
125.73769764504));
#268676=CARTESIAN_POINT('Ctrl Pts',(-231.79006799367,-6.55362117119865,
131.631490910294));
#268677=CARTESIAN_POINT('Ctrl Pts',(-232.068515617483,-2.84650418331021,
136.765191844092));
#268678=CARTESIAN_POINT('Ctrl Pts',(-232.346963241296,3.47641108958031,
136.421180083507));
#268679=CARTESIAN_POINT('Ctrl Pts',(-232.625410865109,6.60467440326965,
130.915585630608));
#268680=CARTESIAN_POINT('Ctrl Pts',(-232.903858488922,3.66356459663667,
125.307780824367));
#268681=CARTESIAN_POINT('Ctrl Pts',(-233.182306112735,-2.64418209922576,
124.751064325225));
#268682=CARTESIAN_POINT('Ctrl Pts',(-233.460753736548,-6.52205462137589,
129.75703139878));
#268683=CARTESIAN_POINT('Ctrl Pts',(-233.73920136036,-4.40647756656326,
135.725442859523));
#268684=CARTESIAN_POINT('Ctrl Pts',(-234.017648984174,1.75843710352442,
137.17162014814));
#268685=CARTESIAN_POINT('Ctrl Pts',(-234.296096607986,6.30743397990132,
132.766596986079));
#268686=CARTESIAN_POINT('Ctrl Pts',(-234.574544231799,5.06020716402928,
126.558374461932));
#268687=CARTESIAN_POINT('Ctrl Pts',(-234.852991855612,-0.837102830722735,
124.252005786856));
#268688=CARTESIAN_POINT('Ctrl Pts',(-235.131439479425,-5.96515621878728,
127.966931100874));
#268689=CARTESIAN_POINT('Ctrl Pts',(-235.409887103238,-5.6115224558684,
134.289315524594));
#268690=CARTESIAN_POINT('Ctrl Pts',(-235.688334727051,-0.101173694118813,
137.409196638266));
#268691=CARTESIAN_POINT('Ctrl Pts',(-235.966782350864,5.50214874991674,
134.459556113093));
#268692=CARTESIAN_POINT('Ctrl Pts',(-236.245229974676,6.04926528768773,
128.150969493757));
#268693=CARTESIAN_POINT('Ctrl Pts',(-236.52367759849,1.03740254911254,124.280719691838));
#268694=CARTESIAN_POINT('Ctrl Pts',(-236.802125222302,-4.92778245216537,
126.405377203086));
#268695=CARTESIAN_POINT('Ctrl Pts',(-237.080572846115,-6.36457611545918,
132.572485569954));
#268696=CARTESIAN_POINT('Ctrl Pts',(-237.359020469928,-1.95263525547508,
137.114773483282));
#268697=CARTESIAN_POINT('Ctrl Pts',(-237.637468093741,4.25368201275546,
135.858100253825));
#268698=CARTESIAN_POINT('Ctrl Pts',(-237.915915717553,6.55107331518259,
129.957287187551));
#268699=CARTESIAN_POINT('Ctrl Pts',(-238.194363341367,2.8283482786799,124.834893221623));
#268700=CARTESIAN_POINT('Ctrl Pts',(-238.47281096518,-3.49349065343433,
125.198148167872));
#268701=CARTESIAN_POINT('Ctrl Pts',(-238.751258588993,-6.60498234154917,
130.713238476685));
#268702=CARTESIAN_POINT('Ctrl Pts',(-239.029706212805,-3.64681792910581,
136.312065581403));
#268703=CARTESIAN_POINT('Ctrl Pts',(-239.308153836619,2.66259400322518,
136.8495808907));
#268704=CARTESIAN_POINT('Ctrl Pts',(-239.586601460431,6.52521212154101,
131.831834094415));
#268705=CARTESIAN_POINT('Ctrl Pts',(-239.865049084244,4.39147907449425,
125.869889367774));
#268706=CARTESIAN_POINT('Ctrl Pts',(-240.143496708057,-1.77780870633274,
124.44248265737));
#268707=CARTESIAN_POINT('Ctrl Pts',(-240.42194433187,-6.31337713682396,
128.861330997368));
#268708=CARTESIAN_POINT('Ctrl Pts',(-240.700391955683,-5.04726040419313,
135.065728636055));
#268709=CARTESIAN_POINT('Ctrl Pts',(-240.978839579496,0.857042067512721,
137.354137245149));
#268710=CARTESIAN_POINT('Ctrl Pts',(-241.257287203309,5.97376474800676,
133.623621107872));
#268711=CARTESIAN_POINT('Ctrl Pts',(-241.535734827122,5.60088945971499,
127.302342308534));
#268712=CARTESIAN_POINT('Ctrl Pts',(-241.814182450934,0.0810703766063902,
124.199247252091));
#268713=CARTESIAN_POINT('Ctrl Pts',(-242.092630074747,-5.51324842209508,
127.165928700792));
#268714=CARTESIAN_POINT('Ctrl Pts',(-242.37107769856,-6.04116125805038,
133.476151333726));
#268715=CARTESIAN_POINT('Ctrl Pts',(-242.649525322373,-1.01754202499167,
137.331128822742));
#268716=CARTESIAN_POINT('Ctrl Pts',(-242.927972946186,4.94114861934255,
135.188325181553));
#268717=CARTESIAN_POINT('Ctrl Pts',(-243.206420569999,6.35916507103108,
129.016872274634));
#268718=CARTESIAN_POINT('Ctrl Pts',(-243.484868193812,1.93341948492588,
124.488033831209));
#268719=CARTESIAN_POINT('Ctrl Pts',(-243.763315817625,-4.26904415503308,
125.763591134728));
#268720=CARTESIAN_POINT('Ctrl Pts',(-244.041763441437,-6.54846477091785,
131.671369337695));
#268721=CARTESIAN_POINT('Ctrl Pts',(-244.320211065251,-2.8101661726183,
136.782408882594));
#268722=CARTESIAN_POINT('Ctrl Pts',(-244.598658689063,3.51053785406796,
136.399914115825));
#268723=CARTESIAN_POINT('Ctrl Pts',(-244.877106312876,6.60522909217403,
130.875379042142));
#268724=CARTESIAN_POINT('Ctrl Pts',(-245.155553936689,3.6300374779527,125.285581505715));
#268725=CARTESIAN_POINT('Ctrl Pts',(-245.434001560502,-2.68098124131831,
124.767272365732));
#268726=CARTESIAN_POINT('Ctrl Pts',(-245.712449184315,-6.528309173032,129.796752401026));
#268727=CARTESIAN_POINT('Ctrl Pts',(-245.990896808128,-4.37643990036281,
135.752175162922));
#268728=CARTESIAN_POINT('Ctrl Pts',(-246.269344431941,1.79716383976481,
137.160798071814));
#268729=CARTESIAN_POINT('Ctrl Pts',(-246.547792055753,6.31926180748295,
132.728165489484));
#268730=CARTESIAN_POINT('Ctrl Pts',(-246.826239679567,5.03426688722615,
126.527650212955));
#268731=CARTESIAN_POINT('Ctrl Pts',(-247.104687303379,-0.876973364781528,
124.257222869343));
#268732=CARTESIAN_POINT('Ctrl Pts',(-247.383134927193,-5.98231793708558,
128.003295270889));
#268733=CARTESIAN_POINT('Ctrl Pts',(-247.661582551005,-5.59020457768662,
134.32340988638));
#268734=CARTESIAN_POINT('Ctrl Pts',(-247.940030174818,-0.0609663080697638,
137.409690138946));
#268735=CARTESIAN_POINT('Ctrl Pts',(-248.218477798631,5.524297020294,134.425995249648));
#268736=CARTESIAN_POINT('Ctrl Pts',(-248.496925422444,6.03300126391963,
128.114195060156));
#268737=CARTESIAN_POINT('Ctrl Pts',(-248.775373046256,0.997672074500306,
124.274525596028));
#268738=CARTESIAN_POINT('Ctrl Pts',(-249.05382067007,-4.95446901239483,
126.435455516518));
#268739=CARTESIAN_POINT('Ctrl Pts',(-249.332268293882,-6.35369511616563,
132.611195791991));
#268740=CARTESIAN_POINT('Ctrl Pts',(-249.610715917695,-1.91418580344349,
137.126542810973));
#268741=CARTESIAN_POINT('Ctrl Pts',(-249.889163541508,4.28436674946925,
135.832113249982));
#268742=CARTESIAN_POINT('Ctrl Pts',(-250.167611165321,6.54579556256923,
129.917424639176));
#268743=CARTESIAN_POINT('Ctrl Pts',(-250.446058789134,2.79195803356287,
124.817786863269));
#268744=CARTESIAN_POINT('Ctrl Pts',(-250.724506412947,-3.52755253356211,
125.219517907192));
#268745=CARTESIAN_POINT('Ctrl Pts',(-251.00295403676,-6.60541465285253,
130.75344656718));
#268746=CARTESIAN_POINT('Ctrl Pts',(-251.281401660573,-3.61322339864049,
136.334162752248));
#268747=CARTESIAN_POINT('Ctrl Pts',(-251.559849284386,2.6993436431913,136.83326092127));
#268748=CARTESIAN_POINT('Ctrl Pts',(-251.838296908198,6.53134574711249,
131.792094239578));
#268749=CARTESIAN_POINT('Ctrl Pts',(-252.116744532012,4.3613601835781,125.843248612281));
#268750=CARTESIAN_POINT('Ctrl Pts',(-252.395192155824,-1.81650232468185,
124.453422554885));
#268751=CARTESIAN_POINT('Ctrl Pts',(-252.673639779637,-6.32508793705065,
128.899798314935));
#268752=CARTESIAN_POINT('Ctrl Pts',(-252.95208740345,-5.02122673409033,
135.096373791053));
#268753=CARTESIAN_POINT('Ctrl Pts',(-253.230535027263,0.896896539007115,
137.348798831588));
#268754=CARTESIAN_POINT('Ctrl Pts',(-253.508982651076,5.99081570467794,
133.587204877683));
#268755=CARTESIAN_POINT('Ctrl Pts',(-253.787430274889,5.57946791275175,
127.26831297809));
#268756=CARTESIAN_POINT('Ctrl Pts',(-254.065877898701,0.0408616672245685,
124.198876151673));
#268757=CARTESIAN_POINT('Ctrl Pts',(-254.344325522515,-5.53529442795169,
127.199556781751));
#268758=CARTESIAN_POINT('Ctrl Pts',(-254.622773146327,-6.0247854077167,
133.512876168065));
#268759=CARTESIAN_POINT('Ctrl Pts',(-254.90122077014,-0.977792831057213,
137.337201825807));
#268760=CARTESIAN_POINT('Ctrl Pts',(-255.179668393953,4.96774341227684,
135.158166043599));
#268761=CARTESIAN_POINT('Ctrl Pts',(-255.458116017766,6.34816648213513,
128.97819485735));
#268762=CARTESIAN_POINT('Ctrl Pts',(-255.736563641579,1.89493404819936,
124.476382515012));
#268763=CARTESIAN_POINT('Ctrl Pts',(-256.015011265392,-4.29964901022966,
125.789669655819));
#268764=CARTESIAN_POINT('Ctrl Pts',(-256.293458889205,-6.54306693065544,
131.711218953762));
#268765=CARTESIAN_POINT('Ctrl Pts',(-256.571906513018,-2.77372173452912,
136.799398141047));
#268766=CARTESIAN_POINT('Ctrl Pts',(-256.85035413683,3.54453019961847,136.378452625405));
#268767=CARTESIAN_POINT('Ctrl Pts',(-257.128801760644,6.60554720661629,
130.835147498674));
#268768=CARTESIAN_POINT('Ctrl Pts',(-257.407249384456,3.5963603924579,125.263628838565));
#268769=CARTESIAN_POINT('Ctrl Pts',(-257.685697008269,-2.71765185753996,
124.783624522784));
#268770=CARTESIAN_POINT('Ctrl Pts',(-257.964144632082,-6.53437691572335,
129.836661023534));
#268771=CARTESIAN_POINT('Ctrl Pts',(-258.242592255895,-4.34613602341029,
135.778440351053));
#268772=CARTESIAN_POINT('Ctrl Pts',(-258.521039879708,1.83562753012831,
137.150276335207));
#268773=CARTESIAN_POINT('Ctrl Pts',(-258.799487503521,6.33122643152078,
132.688650362788));
#268774=CARTESIAN_POINT('Ctrl Pts',(-259.077935127334,5.00743946241547,
126.498999976245));
#268775=CARTESIAN_POINT('Ctrl Pts',(-259.356382751147,-0.915487258132909,
124.259032700089));
#268776=CARTESIAN_POINT('Ctrl Pts',(-259.634830374959,-6.00176822571329,
128.046924274587));
#268777=CARTESIAN_POINT('Ctrl Pts',(-259.86687006147,-5.63687269779404,
133.292521465648));
#268778=CARTESIAN_POINT('Ctrl Pts',(-260.052531023546,-2.79481741349804,
135.900547185714));
#268779=CARTESIAN_POINT('Ctrl Pts',(-260.145376111017,-0.946914048523564,
136.386386345067));
#268780=CARTESIAN_POINT('Ctrl Pts',(-260.191813261187,-0.0157913329746497,
136.389009763222));
#268781=CARTESIAN_POINT('Ctrl Pts',(210.190947297731,3.04870273111253,135.077142573452));
#268782=CARTESIAN_POINT('Ctrl Pts',(210.144529434129,3.76080111712433,134.569051946243));
#268783=CARTESIAN_POINT('Ctrl Pts',(210.051703633225,4.91317831978039,133.192256847685));
#268784=CARTESIAN_POINT('Ctrl Pts',(209.866061957716,5.67455722768035,129.648049455111));
#268785=CARTESIAN_POINT('Ctrl Pts',(209.634022271206,3.10293383059235,125.427666478792));
#268786=CARTESIAN_POINT('Ctrl Pts',(209.355574647392,-2.85596866243967,
125.28812524467));
#268787=CARTESIAN_POINT('Ctrl Pts',(209.07712702358,-6.17973736462657,130.225196103446));
#268788=CARTESIAN_POINT('Ctrl Pts',(208.798679399767,-3.83016968018938,
135.690661498217));
#268789=CARTESIAN_POINT('Ctrl Pts',(208.520231775954,2.04205955310628,136.667868212554));
#268790=CARTESIAN_POINT('Ctrl Pts',(208.241784152142,6.03618933210081,132.255733564264));
#268791=CARTESIAN_POINT('Ctrl Pts',(207.963336528328,4.48417485225333,126.510421532214));
#268792=CARTESIAN_POINT('Ctrl Pts',(207.684888904515,-1.18901089957204,
124.710731370568));
#268793=CARTESIAN_POINT('Ctrl Pts',(207.406441280703,-5.76932406256156,
128.510946815645));
#268794=CARTESIAN_POINT('Ctrl Pts',(207.12799365689,-5.04803188696711,134.418613818075));
#268795=CARTESIAN_POINT('Ctrl Pts',(206.849546033077,0.312219397189005,
137.005003016302));
#268796=CARTESIAN_POINT('Ctrl Pts',(206.571098409264,5.38552219392035,133.893281295751));
#268797=CARTESIAN_POINT('Ctrl Pts',(206.292650785451,5.50981125882569,127.943004805273));
#268798=CARTESIAN_POINT('Ctrl Pts',(206.014203161638,0.570843377758803,
124.622167937696));
#268799=CARTESIAN_POINT('Ctrl Pts',(205.735755537825,-4.89269661278007,
126.982467612715));
#268800=CARTESIAN_POINT('Ctrl Pts',(205.457307914013,-5.86009012142741,
132.854898402769));
#268801=CARTESIAN_POINT('Ctrl Pts',(205.178860290199,-1.44234566848361,
136.842986120511));
#268802=CARTESIAN_POINT('Ctrl Pts',(204.900412666387,4.30084323855829,135.281871486376));
#268803=CARTESIAN_POINT('Ctrl Pts',(204.621965042573,6.09176771588946,129.606143376667));
#268804=CARTESIAN_POINT('Ctrl Pts',(204.343517418761,2.28465505058828,125.031518229909));
#268805=CARTESIAN_POINT('Ctrl Pts',(204.065069794948,-3.62194388278553,
125.761853295313));
#268806=CARTESIAN_POINT('Ctrl Pts',(203.786622171135,-6.20015338889199,
131.126006208945));
#268807=CARTESIAN_POINT('Ctrl Pts',(203.508174547322,-3.08072479357708,
136.194582558939));
#268808=CARTESIAN_POINT('Ctrl Pts',(203.229726923509,2.86973936865286,136.309808260363));
#268809=CARTESIAN_POINT('Ctrl Pts',(202.951279299696,6.1830532544492,131.365796540178));
#268810=CARTESIAN_POINT('Ctrl Pts',(202.672831675884,3.81444325369211,125.905852631576));
#268811=CARTESIAN_POINT('Ctrl Pts',(202.39438405207,-2.05945374882828,124.947398258377));
#268812=CARTESIAN_POINT('Ctrl Pts',(202.115936428258,-6.04081336739099,
129.371206163854));
#268813=CARTESIAN_POINT('Ctrl Pts',(201.837488804444,-4.47096061076856,
135.112012999282));
#268814=CARTESIAN_POINT('Ctrl Pts',(201.559041180632,1.20748652821524,136.894297736177));
#268815=CARTESIAN_POINT('Ctrl Pts',(201.280593556819,5.77631253695961,133.08022777117));
#268816=CARTESIAN_POINT('Ctrl Pts',(201.002145933006,5.03698951269057,127.174747074221));
#268817=CARTESIAN_POINT('Ctrl Pts',(200.723698309193,-0.331080803069094,
124.604703907164));
#268818=CARTESIAN_POINT('Ctrl Pts',(200.44525068538,-5.39490403503349,127.731842386878));
#268819=CARTESIAN_POINT('Ctrl Pts',(200.166803061567,-5.50107401450091,
133.682475019745));
#268820=CARTESIAN_POINT('Ctrl Pts',(199.888355437754,-0.552025717056,136.988261120707));
#268821=CARTESIAN_POINT('Ctrl Pts',(199.609907813942,4.90430724641216,134.611344759621));
#268822=CARTESIAN_POINT('Ctrl Pts',(199.331460190128,5.85382143915379,128.735995953499));
#268823=CARTESIAN_POINT('Ctrl Pts',(199.053012566316,1.42395970438994,124.761373228423));
#268824=CARTESIAN_POINT('Ctrl Pts',(198.774564942502,-4.31445143441004,
126.339960697623));
#268825=CARTESIAN_POINT('Ctrl Pts',(198.49611731869,-6.088092477657,132.02111359519));
#268826=CARTESIAN_POINT('Ctrl Pts',(198.217669694877,-2.26707395378944,
136.584129948007));
#268827=CARTESIAN_POINT('Ctrl Pts',(197.939222071064,3.6372747808909,135.835820643578));
#268828=CARTESIAN_POINT('Ctrl Pts',(197.660774447251,6.19914568268399,130.46384537573));
#268829=CARTESIAN_POINT('Ctrl Pts',(197.382326823438,3.06430454719326,125.404786980035));
#268830=CARTESIAN_POINT('Ctrl Pts',(197.103879199626,-2.88648276756863,
125.307672973393));
#268831=CARTESIAN_POINT('Ctrl Pts',(196.825431575812,-6.1847334314575,130.261746383626));
#268832=CARTESIAN_POINT('Ctrl Pts',(196.546983952,-3.79951621286212,135.71445576667));
#268833=CARTESIAN_POINT('Ctrl Pts',(196.268536328187,2.07727078866752,136.65502757917));
#268834=CARTESIAN_POINT('Ctrl Pts',(195.990088704374,6.04514741573133,132.219122274927));
#268835=CARTESIAN_POINT('Ctrl Pts',(195.711641080561,4.45782888960729,126.483120122517));
#268836=CARTESIAN_POINT('Ctrl Pts',(195.433193456748,-1.22601660901765,
124.718126880723));
#268837=CARTESIAN_POINT('Ctrl Pts',(195.154745832935,-5.78321273819644,
128.54608511404));
#268838=CARTESIAN_POINT('Ctrl Pts',(194.876298209123,-5.02591888662151,
134.449288212205));
#268839=CARTESIAN_POINT('Ctrl Pts',(194.597850585309,0.349948891971121,
137.002980915508));
#268840=CARTESIAN_POINT('Ctrl Pts',(194.319402961497,5.40423073479611,133.860444384439));
#268841=CARTESIAN_POINT('Ctrl Pts',(194.040955337684,5.49228854369214,127.909516169605));
#268842=CARTESIAN_POINT('Ctrl Pts',(193.762507713871,0.533201494146887,
124.618808581434));
#268843=CARTESIAN_POINT('Ctrl Pts',(193.484060090058,-4.91587168017823,
127.012321133451));
#268844=CARTESIAN_POINT('Ctrl Pts',(193.205612466245,-5.84749893410212,
132.890532719942));
#268845=CARTESIAN_POINT('Ctrl Pts',(192.927164842432,-1.40556033379022,
136.851654059523));
#268846=CARTESIAN_POINT('Ctrl Pts',(192.648717218619,4.32801954783523,135.255608152653));
#268847=CARTESIAN_POINT('Ctrl Pts',(192.370269594806,6.08436090050943,129.569083216569));
#268848=CARTESIAN_POINT('Ctrl Pts',(192.091821970994,2.24947182316989,125.017717865345));
#268849=CARTESIAN_POINT('Ctrl Pts',(191.81337434718,-3.65257196685492,125.783994510198));
#268850=CARTESIAN_POINT('Ctrl Pts',(191.534926723368,-6.19808055740059,
131.163742349203));
#268851=CARTESIAN_POINT('Ctrl Pts',(191.256479099555,-3.04785590876364,
136.213235933607));
#268852=CARTESIAN_POINT('Ctrl Pts',(190.978031475742,2.90319942398833,136.292237340818));
#268853=CARTESIAN_POINT('Ctrl Pts',(190.699583851929,6.18635631527163,131.328148137043));
#268854=CARTESIAN_POINT('Ctrl Pts',(190.421136228116,3.7845539731278,125.882723791311));
#268855=CARTESIAN_POINT('Ctrl Pts',(190.142688604304,-2.09506858458051,
124.960043253581));
#268856=CARTESIAN_POINT('Ctrl Pts',(189.86424098049,-6.04942546284962,129.408004862578));
#268857=CARTESIAN_POINT('Ctrl Pts',(189.585793356678,-4.44465587162338,
135.139149194637));
#268858=CARTESIAN_POINT('Ctrl Pts',(189.307345732864,1.24453533211424,136.886834590562));
#268859=CARTESIAN_POINT('Ctrl Pts',(189.028898109051,5.79005936456987,133.045023550676));
#268860=CARTESIAN_POINT('Ctrl Pts',(188.750450485239,5.01480170111087,127.144152737732));
#268861=CARTESIAN_POINT('Ctrl Pts',(188.472002861426,-0.368813738986236,
124.606834155258));
#268862=CARTESIAN_POINT('Ctrl Pts',(188.193555237613,-5.41350737050784,
127.764739625646));
#268863=CARTESIAN_POINT('Ctrl Pts',(187.9151076138,-5.48345219307025,133.715908293866));
#268864=CARTESIAN_POINT('Ctrl Pts',(187.636659989987,-0.51437233173317,
136.991506884579));
#268865=CARTESIAN_POINT('Ctrl Pts',(187.358212366174,4.92739057398128,134.581420314804));
#268866=CARTESIAN_POINT('Ctrl Pts',(187.079764742362,5.84112225861874,128.700400402891));
#268867=CARTESIAN_POINT('Ctrl Pts',(186.801317118548,1.38714794227173,124.752817144095));
#268868=CARTESIAN_POINT('Ctrl Pts',(186.522869494736,-4.34154756707868,
126.366306703083));
#268869=CARTESIAN_POINT('Ctrl Pts',(186.244421870923,-6.08057295867359,
132.058150998494));
#268870=CARTESIAN_POINT('Ctrl Pts',(185.96597424711,-2.23184885375068,136.597823184897));
#268871=CARTESIAN_POINT('Ctrl Pts',(185.687526623297,3.66783531589119,135.813586298303));
#268872=CARTESIAN_POINT('Ctrl Pts',(185.409078999484,6.19695801394562,130.42611572539));
#268873=CARTESIAN_POINT('Ctrl Pts',(185.130631375671,3.03137903541329,125.386233730096));
#268874=CARTESIAN_POINT('Ctrl Pts',(184.852183751858,-2.9198891855651,125.325345654173));
#268875=CARTESIAN_POINT('Ctrl Pts',(184.573736128045,-6.18792188952598,
130.299404664846));
#268876=CARTESIAN_POINT('Ctrl Pts',(184.295288504232,-3.76955667380246,
135.737493527599));
#268877=CARTESIAN_POINT('Ctrl Pts',(184.01684088042,2.11284697206427,136.642274242971));
#268878=CARTESIAN_POINT('Ctrl Pts',(183.738393256607,6.05364746891681,132.182297534532));
#268879=CARTESIAN_POINT('Ctrl Pts',(183.459945632794,4.43144167895468,126.456064115361));
#268880=CARTESIAN_POINT('Ctrl Pts',(183.181498008981,-1.2630425260055,124.725702755623));
#268881=CARTESIAN_POINT('Ctrl Pts',(182.903050385168,-5.79685235262429,
128.581331012064));
#268882=CARTESIAN_POINT('Ctrl Pts',(182.624602761355,-5.00363805916239,
134.479814874928));
#268883=CARTESIAN_POINT('Ctrl Pts',(182.346155137542,0.387675169361259,
137.000735831198));
#268884=CARTESIAN_POINT('Ctrl Pts',(182.06770751373,5.42273385622678,133.827490675898));
#268885=CARTESIAN_POINT('Ctrl Pts',(181.789259889916,5.47456504449634,127.876136685104));
#268886=CARTESIAN_POINT('Ctrl Pts',(181.510812266103,0.495538404244469,
124.615677436551));
#268887=CARTESIAN_POINT('Ctrl Pts',(181.232364642291,-4.93886382111119,
127.042315697369));
#268888=CARTESIAN_POINT('Ctrl Pts',(180.953917018477,-5.83469147177671,
132.926089453735));
#268889=CARTESIAN_POINT('Ctrl Pts',(180.675469394665,-1.36872270040423,
136.860098061879));
#268890=CARTESIAN_POINT('Ctrl Pts',(180.397021770852,4.35503536681857,135.229179797918));
#268891=CARTESIAN_POINT('Ctrl Pts',(180.118574147039,6.07672868724052,129.532068871648));
#268892=CARTESIAN_POINT('Ctrl Pts',(179.840126523226,2.21420520878857,125.004131904969));
#268893=CARTESIAN_POINT('Ctrl Pts',(179.561678899413,-3.68306468660213,
125.80632176824));
#268894=CARTESIAN_POINT('Ctrl Pts',(179.2832312756,-6.19577806271818,131.20146516627));
#268895=CARTESIAN_POINT('Ctrl Pts',(179.004783651788,-3.01487407978163,
136.231688883676));
#268896=CARTESIAN_POINT('Ctrl Pts',(178.726336027974,2.93655189768736,136.274463064253));
#268897=CARTESIAN_POINT('Ctrl Pts',(178.447888404162,6.18943013971724,131.290480325685));
#268898=CARTESIAN_POINT('Ctrl Pts',(178.169440780348,3.75452445381909,125.859777323623));
#268899=CARTESIAN_POINT('Ctrl Pts',(177.890993156536,-2.13060578642238,
124.972904812372));
#268900=CARTESIAN_POINT('Ctrl Pts',(177.612545532723,-6.05781339482078,
129.44485530364));
#268901=CARTESIAN_POINT('Ctrl Pts',(177.33409790891,-4.41818643401566,135.166124762878));
#268902=CARTESIAN_POINT('Ctrl Pts',(177.055650285097,1.28153801924328,136.879146056599));
#268903=CARTESIAN_POINT('Ctrl Pts',(176.777202661284,5.80359163943039,133.009736301615));
#268904=CARTESIAN_POINT('Ctrl Pts',(176.498755037472,4.99242806419446,127.113694031581));
#268905=CARTESIAN_POINT('Ctrl Pts',(176.220307413658,-0.406533008366379,
124.60919405498));
#268906=CARTESIAN_POINT('Ctrl Pts',(175.941859789846,-5.43191010648008,
127.797749498684));
#268907=CARTESIAN_POINT('Ctrl Pts',(175.663412166033,-5.46562718029972,
133.749233679521));
#268908=CARTESIAN_POINT('Ctrl Pts',(175.38496454222,-0.476699886155768,
136.994523381468));
#268909=CARTESIAN_POINT('Ctrl Pts',(175.106516918407,4.95029131528126,134.551355909651));
#268910=CARTESIAN_POINT('Ctrl Pts',(174.828069294595,5.82820663315002,128.664882815304));
#268911=CARTESIAN_POINT('Ctrl Pts',(174.549621670781,1.35028477887665,124.744485301934));
#268912=CARTESIAN_POINT('Ctrl Pts',(174.271174046969,-4.36848282210566,
126.392817162263));
#268913=CARTESIAN_POINT('Ctrl Pts',(173.992726423155,-6.07282812182305,
132.095141942134));
#268914=CARTESIAN_POINT('Ctrl Pts',(173.714278799343,-2.19654105173196,
136.611301742902));
#268915=CARTESIAN_POINT('Ctrl Pts',(173.435831175529,3.69825993790488,135.791166334329));
#268916=CARTESIAN_POINT('Ctrl Pts',(173.157383551717,6.19454071464915,130.388400091055));
#268917=CARTESIAN_POINT('Ctrl Pts',(172.878935927904,2.99834119476844,125.367881250842));
#268918=CARTESIAN_POINT('Ctrl Pts',(172.600488304091,-2.95318740599396,
125.343221361866));
#268919=CARTESIAN_POINT('Ctrl Pts',(172.322040680278,-6.1908810518732,130.337081657394));
#268920=CARTESIAN_POINT('Ctrl Pts',(172.043593056465,-3.7394574524341,135.760348489473));
#268921=CARTESIAN_POINT('Ctrl Pts',(171.765145432652,2.14834486313941,136.629304580736));
#268922=CARTESIAN_POINT('Ctrl Pts',(171.486697808839,6.06192320196904,132.145421734178));
#268923=CARTESIAN_POINT('Ctrl Pts',(171.208250185027,4.40489025960108,126.42916923593));
#268924=CARTESIAN_POINT('Ctrl Pts',(170.929802561213,-1.30002164048796,
124.733503877423));
#268925=CARTESIAN_POINT('Ctrl Pts',(170.651354937401,-5.81027716255637,
128.616659285268));
#268926=CARTESIAN_POINT('Ctrl Pts',(170.372907313588,-4.98117182005496,
134.510205342342));
#268927=CARTESIAN_POINT('Ctrl Pts',(170.094459689775,0.42538708130529,136.998261137926));
#268928=CARTESIAN_POINT('Ctrl Pts',(169.816012065962,5.44103603626017,133.794424944161));
#268929=CARTESIAN_POINT('Ctrl Pts',(169.537564442149,5.45663868327959,127.842865707018));
#268930=CARTESIAN_POINT('Ctrl Pts',(169.259116818336,0.457856951984399,
124.612775615598));
#268931=CARTESIAN_POINT('Ctrl Pts',(168.980669194523,-4.9616729506289,127.072449665244));
#268932=CARTESIAN_POINT('Ctrl Pts',(168.702221570711,-5.82166780281318,
132.961567566087));
#268933=CARTESIAN_POINT('Ctrl Pts',(168.423773946897,-1.33183434849535,
136.868317666657));
#268934=CARTESIAN_POINT('Ctrl Pts',(168.145326323085,4.38188980836473,135.202587479883));
#268935=CARTESIAN_POINT('Ctrl Pts',(167.866878699272,6.06887129855542,129.495101671966));
#268936=CARTESIAN_POINT('Ctrl Pts',(167.588431075459,2.17885654621902,124.9907608742));
#268937=CARTESIAN_POINT('Ctrl Pts',(167.309983451646,-3.71342092903282,
125.82883423045));
#268938=CARTESIAN_POINT('Ctrl Pts',(167.031535827833,-6.19324598120115,
131.239173268482));
#268939=CARTESIAN_POINT('Ctrl Pts',(166.75308820402,-2.98178053353198,136.249940722101));
#268940=CARTESIAN_POINT('Ctrl Pts',(166.474640580207,2.96979555637586,136.25648609103));
#268941=CARTESIAN_POINT('Ctrl Pts',(166.196192956395,6.19227461255283,131.252794500981));
#268942=CARTESIAN_POINT('Ctrl Pts',(165.917745332582,3.7243558092261,125.837014079288));
#268943=CARTESIAN_POINT('Ctrl Pts',(165.639297708769,-2.16606403788322,
124.985982457902));
#268944=CARTESIAN_POINT('Ctrl Pts',(165.360850084956,-6.06597685228888,
129.481756121673));
#268945=CARTESIAN_POINT('Ctrl Pts',(165.082402461143,-4.39155327888481,
135.192938704347));
#268946=CARTESIAN_POINT('Ctrl Pts',(164.80395483733,1.31849321850979,136.871232419228));
#268947=CARTESIAN_POINT('Ctrl Pts',(164.525507213517,5.81690886006848,132.974367331546));
#268948=CARTESIAN_POINT('Ctrl Pts',(164.247059589704,4.96986943102014,127.083372084437));
#268949=CARTESIAN_POINT('Ctrl Pts',(163.968611965891,-0.444237213516358,
124.611783518878));
#268950=CARTESIAN_POINT('Ctrl Pts',(163.690164342078,-5.45011156102575,
127.830870782803));
#268951=CARTESIAN_POINT('Ctrl Pts',(163.411716718265,-5.44759963670407,
133.782449941821));
#268952=CARTESIAN_POINT('Ctrl Pts',(163.133269094453,-0.439009776288703,
136.9973104996));
#268953=CARTESIAN_POINT('Ctrl Pts',(162.85482147064,4.97300862171615,134.52115265821));
#268954=CARTESIAN_POINT('Ctrl Pts',(162.576373846827,5.81507504134112,128.629444506854));
#268955=CARTESIAN_POINT('Ctrl Pts',(162.297926223014,1.31337158018249,124.736378010682));
#268956=CARTESIAN_POINT('Ctrl Pts',(162.019478599201,-4.39525620139515,
126.419491092807));
#268957=CARTESIAN_POINT('Ctrl Pts',(161.741030975388,-6.06485825409316,
132.132085055398));
#268958=CARTESIAN_POINT('Ctrl Pts',(161.462583351575,-2.16115185607673,
136.624565122567));
#268959=CARTESIAN_POINT('Ctrl Pts',(161.184135727762,3.72854751953661,135.768561582436));
#268960=CARTESIAN_POINT('Ctrl Pts',(160.905688103949,6.19189387436843,130.350699870288));
#268961=CARTESIAN_POINT('Ctrl Pts',(160.627240480137,2.96519224948793,125.349730222329));
#268962=CARTESIAN_POINT('Ctrl Pts',(160.348792856324,-2.9863761949775,125.361299434083));
#268963=CARTESIAN_POINT('Ctrl Pts',(160.070345232511,-6.19361080884636,
130.374775965136));
#268964=CARTESIAN_POINT('Ctrl Pts',(159.791897608698,-3.70921966409463,
135.783019805394));
#268965=CARTESIAN_POINT('Ctrl Pts',(159.513449984885,2.18376314650564,136.616119073061));
#268966=CARTESIAN_POINT('Ctrl Pts',(159.235002361072,6.06997430822783,132.108496240312));
#268967=CARTESIAN_POINT('Ctrl Pts',(158.956554737259,4.37817561541891,126.402436480826));
#268968=CARTESIAN_POINT('Ctrl Pts',(158.678107113446,-1.3369525821905,124.741529957054));
#268969=CARTESIAN_POINT('Ctrl Pts',(158.399659489633,-5.82348667053154,
128.652068624549));
#268970=CARTESIAN_POINT('Ctrl Pts',(158.121211865821,-4.95852100179383,
134.540458488317));
#268971=CARTESIAN_POINT('Ctrl Pts',(157.842764242008,0.463083230374652,
136.995556927392));
#268972=CARTESIAN_POINT('Ctrl Pts',(157.564316618195,5.45913659670229,133.761248414491));
#268973=CARTESIAN_POINT('Ctrl Pts',(157.285868994382,5.43851012430973,127.809704468215));
#268974=CARTESIAN_POINT('Ctrl Pts',(157.007421370569,0.420158533666468,
124.610103226106));
#268975=CARTESIAN_POINT('Ctrl Pts',(156.728973746756,-4.98429822353081,
127.102721920452));
#268976=CARTESIAN_POINT('Ctrl Pts',(156.450526122943,-5.80842840980828,
132.996965742341));
#268977=CARTESIAN_POINT('Ctrl Pts',(156.172078499131,-1.2948966449748,136.876312569277));
#268978=CARTESIAN_POINT('Ctrl Pts',(155.893630875317,4.40858187737264,135.175832183934));
#268979=CARTESIAN_POINT('Ctrl Pts',(155.615183251505,6.06078902561252,129.458182987356));
#268980=CARTESIAN_POINT('Ctrl Pts',(155.336735627692,2.14342714531882,124.977605268507));
#268981=CARTESIAN_POINT('Ctrl Pts',(155.058288003879,-3.74363956928552,
125.85153106262));
#268982=CARTESIAN_POINT('Ctrl Pts',(154.779840380066,-6.19048440667673,
131.276865258552));
#268983=CARTESIAN_POINT('Ctrl Pts',(154.501392756253,-2.94857649630798,
136.267990772552));
#268984=CARTESIAN_POINT('Ctrl Pts',(154.22294513244,3.00292916819795,136.238307087292));
#268985=CARTESIAN_POINT('Ctrl Pts',(153.944497508627,6.19488962837548,131.215092059396));
#268986=CARTESIAN_POINT('Ctrl Pts',(153.666049884815,3.69404915725887,125.814434901805));
#268987=CARTESIAN_POINT('Ctrl Pts',(153.387602261001,-2.20144202504465,
124.999275705575));
#268988=CARTESIAN_POINT('Ctrl Pts',(153.109154637189,-6.07391553275397,
129.518705949301));
#268989=CARTESIAN_POINT('Ctrl Pts',(152.830707013376,-4.36475739313218,
135.219590025439));
#268990=CARTESIAN_POINT('Ctrl Pts',(152.552259389563,1.3553995605252,136.863093971691));
#268991=CARTESIAN_POINT('Ctrl Pts',(152.27381176575,5.83001053300956,132.93891795108));
#268992=CARTESIAN_POINT('Ctrl Pts',(151.995364141937,4.94712663750637,127.053188019893));
#268993=CARTESIAN_POINT('Ctrl Pts',(151.716916518124,-0.481924957293099,
124.614602450997));
#268994=CARTESIAN_POINT('Ctrl Pts',(151.438468894311,-5.46811105968323,
127.864102250682));
#268995=CARTESIAN_POINT('Ctrl Pts',(151.160021270498,-5.4293702303005,133.815555849925));
#268996=CARTESIAN_POINT('Ctrl Pts',(150.881573646685,-0.40130339875292,
136.999868135696));
#268997=CARTESIAN_POINT('Ctrl Pts',(150.603126022873,4.99554165148768,134.490811679673));
#268998=CARTESIAN_POINT('Ctrl Pts',(150.324678399059,5.80172796978809,128.59408679072));
#268999=CARTESIAN_POINT('Ctrl Pts',(150.046230775247,1.27640971402146,124.728495570759));
#269000=CARTESIAN_POINT('Ctrl Pts',(149.767783151434,-4.42186671284978,
126.446327506304));
#269001=CARTESIAN_POINT('Ctrl Pts',(149.489335527621,-6.05666365081033,
132.168978969345));
#269002=CARTESIAN_POINT('Ctrl Pts',(149.210887903808,-2.12568257814469,
136.637612832414));
#269003=CARTESIAN_POINT('Ctrl Pts',(148.932440279995,3.75869693846883,135.74577288025));
#269004=CARTESIAN_POINT('Ctrl Pts',(148.653992656183,6.18901759118317,130.313016460088));
#269005=CARTESIAN_POINT('Ctrl Pts',(148.375545032369,2.93193342791814,125.331781317152));
#269006=CARTESIAN_POINT('Ctrl Pts',(148.097097408557,-3.01945432269288,
125.379579200934));
#269007=CARTESIAN_POINT('Ctrl Pts',(147.818649784743,-6.19611105929333,
130.412486191295));
#269008=CARTESIAN_POINT('Ctrl Pts',(147.540202160931,-3.67884442925635,
135.805506635269));
#269009=CARTESIAN_POINT('Ctrl Pts',(147.261754537118,2.21910050972548,136.602718208539));
#269010=CARTESIAN_POINT('Ctrl Pts',(146.983306913305,6.07780048935632,132.071522421221));
#269011=CARTESIAN_POINT('Ctrl Pts',(146.704859289492,4.35129873632927,126.375866840638));
#269012=CARTESIAN_POINT('Ctrl Pts',(146.426411665679,-1.37383398262348,
124.749780697104));
#269013=CARTESIAN_POINT('Ctrl Pts',(146.147964041867,-5.83648038706648,
128.687557717801));
#269014=CARTESIAN_POINT('Ctrl Pts',(145.869516418053,-4.93568644371351,
134.570573191811));
#269015=CARTESIAN_POINT('Ctrl Pts',(145.591068794241,0.500762219724632,
136.992623299802));
#269016=CARTESIAN_POINT('Ctrl Pts',(145.312621170428,5.47703486683029,133.727962316256));
#269017=CARTESIAN_POINT('Ctrl Pts',(145.034173546615,5.42018003934715,127.776654197497));
#269018=CARTESIAN_POINT('Ctrl Pts',(144.755725922802,0.382444546219556,
124.607660367099));
#269019=CARTESIAN_POINT('Ctrl Pts',(144.477278298989,-5.00673880142907,
127.133131341243));
#269020=CARTESIAN_POINT('Ctrl Pts',(144.198830675176,-5.79497378335261,
133.032282670807));
#269021=CARTESIAN_POINT('Ctrl Pts',(143.920383051363,-1.25791095858285,
136.884082473484));
#269022=CARTESIAN_POINT('Ctrl Pts',(143.64193542755,4.43511058475782,135.148914901497));
#269023=CARTESIAN_POINT('Ctrl Pts',(143.363487803737,6.05248216790344,129.421314185853));
#269024=CARTESIAN_POINT('Ctrl Pts',(143.085040179924,2.10791831893749,124.964665575378));
#269025=CARTESIAN_POINT('Ctrl Pts',(142.806592556112,-3.77371948759721,
125.87441142371));
#269026=CARTESIAN_POINT('Ctrl Pts',(142.528144932299,-6.18749344147606,
131.314539739788));
#269027=CARTESIAN_POINT('Ctrl Pts',(142.249697308486,-2.91526319849757,
136.285838366179));
#269028=CARTESIAN_POINT('Ctrl Pts',(141.971249684673,3.03595150537554,136.219926726669));
#269029=CARTESIAN_POINT('Ctrl Pts',(141.69280206086,6.19727509028471,131.177374398005));
#269030=CARTESIAN_POINT('Ctrl Pts',(141.414354437047,3.6636056209416,125.792040627854));
#269031=CARTESIAN_POINT('Ctrl Pts',(141.135906813234,-2.23673843696229,
125.012784062803));
#269032=CARTESIAN_POINT('Ctrl Pts',(140.857459189421,-6.0816291420453,129.555703417335));
#269033=CARTESIAN_POINT('Ctrl Pts',(140.579011565609,-4.33779976968917,
135.246077738584));
#269034=CARTESIAN_POINT('Ctrl Pts',(140.300563941795,1.39225567771152,136.854731015561));
#269035=CARTESIAN_POINT('Ctrl Pts',(140.022116317983,5.84289617276637,132.903389473806));
#269036=CARTESIAN_POINT('Ctrl Pts',(139.74366869417,4.92420052639575,127.023142956427));
#269037=CARTESIAN_POINT('Ctrl Pts',(139.465221070357,-0.519594843163371,
124.617650746882));
#269038=CARTESIAN_POINT('Ctrl Pts',(139.186773446544,-5.48590793547459,
127.897442670915));
#269039=CARTESIAN_POINT('Ctrl Pts',(138.908325822731,-5.41093963658633,
133.848550177083));
#269040=CARTESIAN_POINT('Ctrl Pts',(138.629878198918,-0.363582150772119,
137.002196194983));
#269041=CARTESIAN_POINT('Ctrl Pts',(138.351430575105,5.0178895696262,134.460334098336));
#269042=CARTESIAN_POINT('Ctrl Pts',(138.072982951292,5.78816591307159,128.558810977095));
#269043=CARTESIAN_POINT('Ctrl Pts',(137.79453532748,1.23940055002892,124.720838274248));
#269044=CARTESIAN_POINT('Ctrl Pts',(137.516087703667,-4.44831337040726,
126.473325408321));
#269045=CARTESIAN_POINT('Ctrl Pts',(137.237640079854,-6.0482446156285,132.205822316857));
#269046=CARTESIAN_POINT('Ctrl Pts',(136.959192456041,-2.09013453226308,
136.650444388955));
#269047=CARTESIAN_POINT('Ctrl Pts',(136.680744832228,3.78870707750376,135.722801072215));
#269048=CARTESIAN_POINT('Ctrl Pts',(136.402297208415,6.18591197167502,130.275351256826));
#269049=CARTESIAN_POINT('Ctrl Pts',(136.123849584602,2.89856596247695,125.314035200413));
#269050=CARTESIAN_POINT('Ctrl Pts',(135.845401960789,-3.05242056341787,
125.398059985055));
#269051=CARTESIAN_POINT('Ctrl Pts',(135.566954336976,-6.19838171056633,
130.450210938505));
#269052=CARTESIAN_POINT('Ctrl Pts',(135.288506713164,-3.64833287348497,
135.827808145838));
#269053=CARTESIAN_POINT('Ctrl Pts',(135.01005908935,2.25435564335981,136.589102483743));
#269054=CARTESIAN_POINT('Ctrl Pts',(134.731611465538,6.08540145535266,132.034501646982));
#269055=CARTESIAN_POINT('Ctrl Pts',(134.453163841725,4.32426061826468,126.349461299917));
#269056=CARTESIAN_POINT('Ctrl Pts',(134.174716217912,-1.41066447513297,
124.75825579184));
#269057=CARTESIAN_POINT('Ctrl Pts',(133.896268594099,-5.84925783067434,
128.723125249964));
#269058=CARTESIAN_POINT('Ctrl Pts',(133.617820970286,-4.91266899195694,
134.600548336913));
#269059=CARTESIAN_POINT('Ctrl Pts',(133.339373346473,0.538422653146471,
136.989460363863));
#269060=CARTESIAN_POINT('Ctrl Pts',(133.06092572266,5.49473018341705,133.694567882885));
#269061=CARTESIAN_POINT('Ctrl Pts',(132.782478098847,5.40164910761999,127.743716119554));
#269062=CARTESIAN_POINT('Ctrl Pts',(132.504030475035,0.344716387149417,
124.605447129098));
#269063=CARTESIAN_POINT('Ctrl Pts',(132.225582851222,-5.02899385277987,
127.163676800786));
#269064=CARTESIAN_POINT('Ctrl Pts',(131.947135227409,-5.78130442201224,
133.067517042801));
#269065=CARTESIAN_POINT('Ctrl Pts',(131.668687603596,-1.22087865983776,
136.891627091362));
#269066=CARTESIAN_POINT('Ctrl Pts',(131.390239979783,4.46147494748924,135.121836630005));
#269067=CARTESIAN_POINT('Ctrl Pts',(131.11179235597,6.04395103324181,129.384496633644));
#269068=CARTESIAN_POINT('Ctrl Pts',(130.833344732157,2.07233138286776,124.951942274296));
#269069=CARTESIAN_POINT('Ctrl Pts',(130.554897108344,-3.80365956934553,
125.897474465882));
#269070=CARTESIAN_POINT('Ctrl Pts',(130.276449484532,-6.18427319643048,
131.35219531615));
#269071=CARTESIAN_POINT('Ctrl Pts',(129.998001860718,-2.88184187453723,
136.303482841632));
#269072=CARTESIAN_POINT('Ctrl Pts',(129.719554236906,3.0688613442533,136.201345690253));
#269073=CARTESIAN_POINT('Ctrl Pts',(129.441106613093,6.1994309098865,131.139642914452));
#269074=CARTESIAN_POINT('Ctrl Pts',(129.16265898928,3.63302632837089,125.769832087263));
#269075=CARTESIAN_POINT('Ctrl Pts',(128.884211365467,-2.27195196571463,
125.026507029031));
#269076=CARTESIAN_POINT('Ctrl Pts',(128.605763741654,-6.08911739433215,
129.592747154821));
#269077=CARTESIAN_POINT('Ctrl Pts',(128.327316117841,-4.31068140748063,
135.272400862266));
#269078=CARTESIAN_POINT('Ctrl Pts',(128.048868494028,1.42906020435147,136.846143860731));
#269079=CARTESIAN_POINT('Ctrl Pts',(127.770420870216,5.85556530185681,132.867783216248));
#269080=CARTESIAN_POINT('Ctrl Pts',(127.491973246402,4.9010919472237,126.993238007373));
#269081=CARTESIAN_POINT('Ctrl Pts',(127.21352562259,-0.557245475255655,
124.620928293575));
#269082=CARTESIAN_POINT('Ctrl Pts',(126.935077998777,-5.50350152892981,
127.930890808061));
#269083=CARTESIAN_POINT('Ctrl Pts',(126.656630374964,-5.39230853851415,
133.881431700678));
#269084=CARTESIAN_POINT('Ctrl Pts',(126.378182751151,-0.325847430121078,
137.004294591193));
#269085=CARTESIAN_POINT('Ctrl Pts',(126.099735127338,5.04005154802147,134.429721043558));
#269086=CARTESIAN_POINT('Ctrl Pts',(125.821287503525,5.77438937373851,128.523618373138));
#269087=CARTESIAN_POINT('Ctrl Pts',(125.542839879712,1.20234545959337,124.713406404895));
#269088=CARTESIAN_POINT('Ctrl Pts',(125.264392255899,-4.47459519407686,
126.50048379844));
#269089=CARTESIAN_POINT('Ctrl Pts',(124.985944632086,-6.03960146051831,
132.24261373269));
#269090=CARTESIAN_POINT('Ctrl Pts',(124.707497008274,-2.05450903567761,
136.663059316712));
#269091=CARTESIAN_POINT('Ctrl Pts',(124.429049384461,3.81857682460466,135.69964700956));
#269092=CARTESIAN_POINT('Ctrl Pts',(124.150601760648,6.18257713092382,130.237705656202));
#269093=CARTESIAN_POINT('Ctrl Pts',(123.872154136835,2.86509108960817,125.296492529702));
#269094=CARTESIAN_POINT('Ctrl Pts',(123.593706513022,-3.08527369557641,
125.416741101634));
#269095=CARTESIAN_POINT('Ctrl Pts',(123.315258889209,-6.20042267852561,
130.487948808862));
#269096=CARTESIAN_POINT('Ctrl Pts',(123.036811265396,-3.61768612739718,
135.849923510712));
#269097=CARTESIAN_POINT('Ctrl Pts',(122.758363641583,2.28952724101679,136.575272403211));
#269098=CARTESIAN_POINT('Ctrl Pts',(122.47991601777,6.09277692456002,131.997435289415));
#269099=CARTESIAN_POINT('Ctrl Pts',(122.201468393958,4.29706226313277,126.323220837128));
#269100=CARTESIAN_POINT('Ctrl Pts',(121.923020770144,-1.44744269495155,
124.766954927214));
#269101=CARTESIAN_POINT('Ctrl Pts',(121.644573146332,-5.86181852788225,
128.758769903068));
#269102=CARTESIAN_POINT('Ctrl Pts',(121.366125522519,-4.88946949944416,
134.630382812884));
#269103=CARTESIAN_POINT('Ctrl Pts',(121.087677898706,0.576063135118759,
136.986068236777));
#269104=CARTESIAN_POINT('Ctrl Pts',(120.809230274893,5.51222189075617,133.661066351821));
#269105=CARTESIAN_POINT('Ctrl Pts',(120.53078265108,5.38291801579874,127.710891454918));
#269106=CARTESIAN_POINT('Ctrl Pts',(120.252335027267,0.306975454486648,
124.603463594118));
#269107=CARTESIAN_POINT('Ctrl Pts',(119.973887403454,-5.05106255291402,
127.194357167205));
#269108=CARTESIAN_POINT('Ctrl Pts',(119.695439779642,-5.76742083231046,
133.102667552701));
#269109=CARTESIAN_POINT('Ctrl Pts',(119.416992155829,-1.18380112098488,
136.898946143343));
#269110=CARTESIAN_POINT('Ctrl Pts',(119.138544532016,4.48767398862585,135.09459837285));
#269111=CARTESIAN_POINT('Ctrl Pts',(118.860096908203,6.03519593775195,129.347731695017));
#269112=CARTESIAN_POINT('Ctrl Pts',(118.58164928439,2.0366676557964,124.939435836727));
#269113=CARTESIAN_POINT('Ctrl Pts',(118.303201660577,-3.83345870508974,
125.920719334523));
#269114=CARTESIAN_POINT('Ctrl Pts',(118.024754036764,-6.18082379086727,
131.389830592295));
#269115=CARTESIAN_POINT('Ctrl Pts',(117.746306412951,-2.84831376286653,
136.320923545089));
#269116=CARTESIAN_POINT('Ctrl Pts',(117.467858789138,3.10165746534553,136.18256466657));
#269117=CARTESIAN_POINT('Ctrl Pts',(117.189411165326,6.20135700729606,131.101899006891));
#269118=CARTESIAN_POINT('Ctrl Pts',(116.910963541513,3.60231241267338,125.747810102979));
#269119=CARTESIAN_POINT('Ctrl Pts',(116.6325159177,-2.30708130645123,125.040444095748));
#269120=CARTESIAN_POINT('Ctrl Pts',(116.354068293887,-6.09638001213474,
129.62983578909));
#269121=CARTESIAN_POINT('Ctrl Pts',(116.075620670074,-4.28340331138726,
135.298558421074));
#269122=CARTESIAN_POINT('Ctrl Pts',(115.797173046261,1.46581177664024,136.837332825402));
#269123=CARTESIAN_POINT('Ctrl Pts',(115.518725422448,5.86801745082159,132.832100497806));
#269124=CARTESIAN_POINT('Ctrl Pts',(115.240277798635,4.87780175628715,126.963474280869));
#269125=CARTESIAN_POINT('Ctrl Pts',(114.961830174822,-0.594875458411799,
124.624434969628));
#269126=CARTESIAN_POINT('Ctrl Pts',(114.68338255101,-5.52089118811201,127.964445422689));
#269127=CARTESIAN_POINT('Ctrl Pts',(114.404934927196,-5.37347762646609,
133.914199202272));
#269128=CARTESIAN_POINT('Ctrl Pts',(114.126487303384,-0.288100635073559,
137.006163246571));
#269129=CARTESIAN_POINT('Ctrl Pts',(113.848039679571,5.06202676545313,134.398973649715));
#269130=CARTESIAN_POINT('Ctrl Pts',(113.569592055758,5.76039886228364,128.488510282924));
#269131=CARTESIAN_POINT('Ctrl Pts',(113.291144431945,1.16524581580469,124.706200238089));
#269132=CARTESIAN_POINT('Ctrl Pts',(113.012696808132,-4.50071120997606,
126.527801670297));
#269133=CARTESIAN_POINT('Ctrl Pts',(112.734249184319,-6.03073450575487,
132.279351853526));
#269134=CARTESIAN_POINT('Ctrl Pts',(112.455801560506,-2.01880740850426,
136.675457148234));
#269135=CARTESIAN_POINT('Ctrl Pts',(112.177353936694,3.84830507293705,135.676311550269));
#269136=CARTESIAN_POINT('Ctrl Pts',(111.898906312881,6.17901319250346,130.200081053184));
#269137=CARTESIAN_POINT('Ctrl Pts',(111.620458689068,2.8315100497353,125.279153955068));
#269138=CARTESIAN_POINT('Ctrl Pts',(111.342011065255,-3.11801250178361,
125.435621858436));
#269139=CARTESIAN_POINT('Ctrl Pts',(111.063563441442,-6.20223388754234,
130.525698403974));
#269140=CARTESIAN_POINT('Ctrl Pts',(110.785115817629,-3.58690532661952,
135.871851910398));
#269141=CARTESIAN_POINT('Ctrl Pts',(110.506668193816,2.32461399939974,136.56122847942));
#269142=CARTESIAN_POINT('Ctrl Pts',(110.228220570003,6.09992662367788,131.960324722029));
#269143=CARTESIAN_POINT('Ctrl Pts',(109.94977294619,4.26970467877848,126.297146424621));
#269144=CARTESIAN_POINT('Ctrl Pts',(109.671325322378,-1.48416727924886,
124.775877780875));
#269145=CARTESIAN_POINT('Ctrl Pts',(109.392877698565,-5.8741620132489,128.794490356288));
#269146=CARTESIAN_POINT('Ctrl Pts',(109.114430074752,-4.86608882584101,
134.660075514194));
#269147=CARTESIAN_POINT('Ctrl Pts',(108.835982450939,0.61368227085971,136.982447044243));
#269148=CARTESIAN_POINT('Ctrl Pts',(108.557534827126,5.52950934068608,133.627458964475));
#269149=CARTESIAN_POINT('Ctrl Pts',(108.279087203313,5.36398745797076,127.67818141992));
#269150=CARTESIAN_POINT('Ctrl Pts',(108.0006395795,0.269223146735527,124.601709835656));
#269151=CARTESIAN_POINT('Ctrl Pts',(107.722191955687,-5.07294408406776,
127.225171303631));
#269152=CARTESIAN_POINT('Ctrl Pts',(107.443744331874,-5.75332352870873,
133.137732897993));
#269153=CARTESIAN_POINT('Ctrl Pts',(107.165296708062,-1.14667971594628,
136.906039358215));
#269154=CARTESIAN_POINT('Ctrl Pts',(106.886849084249,4.51370673735246,135.067201139359));
#269155=CARTESIAN_POINT('Ctrl Pts',(106.608401460436,6.02621720585718,129.31102073231));
#269156=CARTESIAN_POINT('Ctrl Pts',(106.329953836623,2.00092845925606,124.927146726103));
#269157=CARTESIAN_POINT('Ctrl Pts',(106.05150621281,-3.86311579061174,125.944145168289));
#269158=CARTESIAN_POINT('Ctrl Pts',(105.773058588997,-6.17714535260555,
131.427444173636));
#269159=CARTESIAN_POINT('Ctrl Pts',(105.494610965184,-2.81468010588189,
136.338159830278));
#269160=CARTESIAN_POINT('Ctrl Pts',(105.216163341371,3.13433865337982,136.163584351558));
#269161=CARTESIAN_POINT('Ctrl Pts',(104.937715717558,6.20305331114115,131.064144073934));
#269162=CARTESIAN_POINT('Ctrl Pts',(104.659268093745,3.57146501196475,125.725975491034));
#269163=CARTESIAN_POINT('Ctrl Pts',(104.380820469933,-2.34212515744159,
125.054594746511));
#269164=CARTESIAN_POINT('Ctrl Pts',(104.10237284612,-6.10341672633411,129.666967945808));
#269165=CARTESIAN_POINT('Ctrl Pts',(103.823925222307,-4.25596649220884,
135.324549445729));
#269166=CARTESIAN_POINT('Ctrl Pts',(103.545477598494,1.50250903273456,136.828298236068));
#269167=CARTESIAN_POINT('Ctrl Pts',(103.267029974681,5.88025215824177,132.796342640716));
#269168=CARTESIAN_POINT('Ctrl Pts',(102.988582350868,4.85433081661274,126.933852879821));
#269169=CARTESIAN_POINT('Ctrl Pts',(102.710134727055,-0.63248339823904,
124.628170645098));
#269170=CARTESIAN_POINT('Ctrl Pts',(102.431687103242,-5.53807626864099,
127.998105271418));
#269171=CARTESIAN_POINT('Ctrl Pts',(102.153239479429,-5.35444759822839,
133.946851467654));
#269172=CARTESIAN_POINT('Ctrl Pts',(101.874791855617,-0.250343164351048,
137.00780209187));
#269173=CARTESIAN_POINT('Ctrl Pts',(101.596344231803,5.0838144076213,134.368093056165));
#269174=CARTESIAN_POINT('Ctrl Pts',(101.317896607991,5.74619489713063,128.453488007394));
#269175=CARTESIAN_POINT('Ctrl Pts',(101.039448984178,1.12810299340375,124.69922004086));
#269176=CARTESIAN_POINT('Ctrl Pts',(100.761001360365,-4.52666045036627,
126.55527801162));
#269177=CARTESIAN_POINT('Ctrl Pts',(100.482553736552,-6.0216440799065,132.316035318018));
#269178=CARTESIAN_POINT('Ctrl Pts',(100.204106112739,-1.98303097367997,
136.687637424115));
#269179=CARTESIAN_POINT('Ctrl Pts',(99.9256584889259,3.87789072090961,135.652795559044));
#269180=CARTESIAN_POINT('Ctrl Pts',(99.6472108651132,6.17522028847693,130.162478841968));
#269181=CARTESIAN_POINT('Ctrl Pts',(99.3687632413001,2.79782408721636,125.262020118999));
#269182=CARTESIAN_POINT('Ctrl Pts',(99.0903156174874,-3.15063576889091,
125.454701555827));
#269183=CARTESIAN_POINT('Ctrl Pts',(98.8118679936743,-6.20381527050148,
130.563458325018));
#269184=CARTESIAN_POINT('Ctrl Pts',(98.5334203698616,-3.55599161174595,
135.89359253233));
#269185=CARTESIAN_POINT('Ctrl Pts',(98.2549727460486,2.35961461835606,136.546971232774));
#269186=CARTESIAN_POINT('Ctrl Pts',(97.9765251222358,6.10685028777152,131.923171319966));
#269187=CARTESIAN_POINT('Ctrl Pts',(97.6980774984228,4.24218887894701,126.271239028595));
#269188=CARTESIAN_POINT('Ctrl Pts',(97.4196298746099,-1.52083686718185,
124.785024022185));
#269189=CARTESIAN_POINT('Ctrl Pts',(97.141182250797,-5.88628782938184,128.830285285991));
#269190=CARTESIAN_POINT('Ctrl Pts',(96.8627346269842,-4.842527837527,134.689625340572));
#269191=CARTESIAN_POINT('Ctrl Pts',(96.5842870031713,0.651278666378471,
136.978596920444));
#269192=CARTESIAN_POINT('Ctrl Pts',(96.3058393793584,5.54659189261388,133.593746966183));
#269193=CARTESIAN_POINT('Ctrl Pts',(96.0273917555454,5.34485813561491,127.645587226641));
#269194=CARTESIAN_POINT('Ctrl Pts',(95.7489441317327,0.231460862821695,
124.6001859187));
#269195=CARTESIAN_POINT('Ctrl Pts',(95.4704965079195,-5.09463763541278,
127.256118068232));
#269196=CARTESIAN_POINT('Ctrl Pts',(95.192048884107,-5.73901303358793,133.172711779316));
#269197=CARTESIAN_POINT('Ctrl Pts',(94.9136012602939,-1.10951582026908,
136.912906473138));
#269198=CARTESIAN_POINT('Ctrl Pts',(94.635153636481,4.53957222901603,135.039645944743));
#269199=CARTESIAN_POINT('Ctrl Pts',(94.3567060126683,6.01701517026768,129.274365105863));
#269200=CARTESIAN_POINT('Ctrl Pts',(94.0782583888551,1.96511511757592,124.915075397801));
#269201=CARTESIAN_POINT('Ctrl Pts',(93.7998107650425,-3.89262972695748,
125.967751099126));
#269202=CARTESIAN_POINT('Ctrl Pts',(93.5213631412293,-6.17323801795121,
131.465034666385));
#269203=CARTESIAN_POINT('Ctrl Pts',(93.2429155174167,-2.7809421498907,136.355191058501));
#269204=CARTESIAN_POINT('Ctrl Pts',(92.9644678936037,3.16690369734264,136.14440544854));
#269205=CARTESIAN_POINT('Ctrl Pts',(92.6860202697908,6.20451975856463,131.026379514606));
#269206=CARTESIAN_POINT('Ctrl Pts',(92.4075726459779,3.54048526930663,125.704329060518));
#269207=CARTESIAN_POINT('Ctrl Pts',(92.129125022165,-2.37708222012305,125.068958456964));
#269208=CARTESIAN_POINT('Ctrl Pts',(91.850677398352,-6.1102272761821,129.70414224903));
#269209=CARTESIAN_POINT('Ctrl Pts',(91.5722297745392,-4.22837196662692,
135.350372973126));
#269210=CARTESIAN_POINT('Ctrl Pts',(91.2937821507264,1.53915061280415,136.819040427511));
#269211=CARTESIAN_POINT('Ctrl Pts',(91.0153345269133,5.89226897075567,132.76051097));
#269212=CARTESIAN_POINT('Ctrl Pts',(90.7368869031008,4.8306799979248,126.90437490186));
#269213=CARTESIAN_POINT('Ctrl Pts',(90.4584392792875,-0.670067901161403,
124.632135181558));
#269214=CARTESIAN_POINT('Ctrl Pts',(90.1799916554748,-5.5550561337172,128.031869106972));
#269215=CARTESIAN_POINT('Ctrl Pts',(89.9015440316619,-5.3352191589658,133.979387286881));
#269216=CARTESIAN_POINT('Ctrl Pts',(89.6230964078489,-0.212576417070642,
137.009211066365));
#269217=CARTESIAN_POINT('Ctrl Pts',(89.3446487840362,5.10541366717708,134.337080407198));
#269218=CARTESIAN_POINT('Ctrl Pts',(89.0662011602232,5.73177800461257,128.418552844315));
#269219=CARTESIAN_POINT('Ctrl Pts',(88.7877535364103,1.09091836873142,124.69246607186));
#269220=CARTESIAN_POINT('Ctrl Pts',(88.5093059125973,-4.5524419536888,126.58291180426));
#269221=CARTESIAN_POINT('Ctrl Pts',(88.2308582887847,-6.0123305198223,132.352662766849));
#269222=CARTESIAN_POINT('Ctrl Pts',(87.9524106649715,-1.94718105691378,
136.69959969301));
#269223=CARTESIAN_POINT('Ctrl Pts',(87.6739630411587,3.90733267221543,135.629099907278));
#269224=CARTESIAN_POINT('Ctrl Pts',(87.395515417346,6.17119855939173,130.124900415918));
#269225=CARTESIAN_POINT('Ctrl Pts',(87.1170677935327,2.76403445029686,125.245091656395));
#269226=CARTESIAN_POINT('Ctrl Pts',(86.8386201697203,-3.18314228803115,
125.473979486801));
#269227=CARTESIAN_POINT('Ctrl Pts',(86.5601725459069,-6.20516676880425,
130.601227172784));
#269228=CARTESIAN_POINT('Ctrl Pts',(86.2817249220945,-3.52494612829556,
135.915144570902));
#269229=CARTESIAN_POINT('Ctrl Pts',(86.0032772982812,2.394527800925,136.532501191579));
#269230=CARTESIAN_POINT('Ctrl Pts',(85.7248296744686,6.11354766028192,131.885976459962));
#269231=CARTESIAN_POINT('Ctrl Pts',(85.4463820506556,4.21451588324655,126.245499609054));
#269232=CARTESIAN_POINT('Ctrl Pts',(85.1679344268427,-1.55745009994542,
124.794393312227));
#269233=CARTESIAN_POINT('Ctrl Pts',(84.8894868030298,-5.89819552695468,
128.86615336578));
#269234=CARTESIAN_POINT('Ctrl Pts',(84.611039179217,-4.81878740756302,134.719031197036));
#269235=CARTESIAN_POINT('Ctrl Pts',(84.332591555404,0.68885092852684,136.974518008049));
#269236=CARTESIAN_POINT('Ctrl Pts',(84.0541439315912,5.56346891353935,133.559931606153));
#269237=CARTESIAN_POINT('Ctrl Pts',(83.7756963077782,5.32553075757526,127.613110082872));
#269238=CARTESIAN_POINT('Ctrl Pts',(83.4972486839655,0.193690002040587,
124.598891899719));
#269239=CARTESIAN_POINT('Ctrl Pts',(83.2188010601524,-5.11614240308669,
127.287196314267));
#269240=CARTESIAN_POINT('Ctrl Pts',(82.9403534363397,-5.72448987722869,
133.207602900518));
#269241=CARTESIAN_POINT('Ctrl Pts',(82.6619058125266,-1.07231081107503,
136.919547233648));
#269242=CARTESIAN_POINT('Ctrl Pts',(82.3834581887138,4.56526950516122,135.011933810073));
#269243=CARTESIAN_POINT('Ctrl Pts',(82.1050105649009,6.00759017196827,129.237766173961));
#269244=CARTESIAN_POINT('Ctrl Pts',(81.826562941088,1.92922895783247,124.903222299129));
#269245=CARTESIAN_POINT('Ctrl Pts',(81.5481153172751,-3.92199942047723,
125.991536252305));
#269246=CARTESIAN_POINT('Ctrl Pts',(81.2696676934623,-6.16910193169181,
131.502600677615));
#269247=CARTESIAN_POINT('Ctrl Pts',(80.9912200696492,-2.74710114506546,
136.372016598662));
#269248=CARTESIAN_POINT('Ctrl Pts',(80.7127724458365,3.19935139052435,136.125028668197));
#269249=CARTESIAN_POINT('Ctrl Pts',(80.4343248220235,6.20575629522666,130.988606728286));
#269250=CARTESIAN_POINT('Ctrl Pts',(80.1558771982107,3.50937433266497,125.682871613546));
#269251=CARTESIAN_POINT('Ctrl Pts',(79.8774295743978,-2.41195119914859,
125.083534694853));
#269252=CARTESIAN_POINT('Ctrl Pts',(79.5989819505849,-6.11681140931136,
129.741357321249));
#269253=CARTESIAN_POINT('Ctrl Pts',(79.320534326772,-4.20062075716678,135.376028046362));
#269254=CARTESIAN_POINT('Ctrl Pts',(79.0420867029591,1.57573515908161,136.809559742781));
#269255=CARTESIAN_POINT('Ctrl Pts',(78.7636390791462,5.90406744307602,132.724606813414));
#269256=CARTESIAN_POINT('Ctrl Pts',(78.4851914553333,4.80685017661309,126.875041439303));
#269257=CARTESIAN_POINT('Ctrl Pts',(78.2067438315204,-0.707627574471386,
124.636328432103));
#269258=CARTESIAN_POINT('Ctrl Pts',(77.9282962077074,-5.57183015414549,
128.065735678218));
#269259=CARTESIAN_POINT('Ctrl Pts',(77.6498485838947,-5.31579302119528,
134.011805454327));
#269260=CARTESIAN_POINT('Ctrl Pts',(77.3714009600817,-0.174801792692954,
137.010390117845));
#269261=CARTESIAN_POINT('Ctrl Pts',(77.0929533362689,5.12682374375196,134.305936852001));
#269262=CARTESIAN_POINT('Ctrl Pts',(76.814505712456,5.7171487189526,128.38370608822));
#269263=CARTESIAN_POINT('Ctrl Pts',(76.536058088643,1.05369331967776,124.68593858136));
#269264=CARTESIAN_POINT('Ctrl Pts',(76.2576104648302,-4.57805476460059,
126.610702024239));
#269265=CARTESIAN_POINT('Ctrl Pts',(75.9791628410172,-6.00279417061961,
132.389232842773));
#269266=CARTESIAN_POINT('Ctrl Pts',(75.7007152172044,-1.91125898663751,
136.711343511654));
#269267=CARTESIAN_POINT('Ctrl Pts',(75.4222675933915,3.93662983587222,135.605225473025));
#269268=CARTESIAN_POINT('Ctrl Pts',(75.1438199695785,6.16694815427437,130.087347167514));
#269269=CARTESIAN_POINT('Ctrl Pts',(74.8653723457658,2.73014239106432,125.228369194547));
#269270=CARTESIAN_POINT('Ctrl Pts',(74.5869247219528,-3.21553085466319,
125.493454937009));
#269271=CARTESIAN_POINT('Ctrl Pts',(74.3084770981399,-6.20628833237051,
130.639003547736));
#269272=CARTESIAN_POINT('Ctrl Pts',(74.0300294743271,-3.49377002667009,
135.936507227495));
#269273=CARTESIAN_POINT('Ctrl Pts',(73.7515818505141,2.42935225338577,136.517818892029));
#269274=CARTESIAN_POINT('Ctrl Pts',(73.4731342267013,6.1200184930355,131.848741520285));
#269275=CARTESIAN_POINT('Ctrl Pts',(73.1946866028884,4.18668671711015,126.219929119786));
#269276=CARTESIAN_POINT('Ctrl Pts',(72.9162389790755,-1.59400562082267,
124.803985303816));
#269277=CARTESIAN_POINT('Ctrl Pts',(72.6377913552626,-5.90988466472314,
128.902093266552));
#269278=CARTESIAN_POINT('Ctrl Pts',(72.3593437314497,-4.79486841565966,
134.748291993943));
#269279=CARTESIAN_POINT('Ctrl Pts',(72.0808961076369,0.726397665050741,
136.970210458201));
#269280=CARTESIAN_POINT('Ctrl Pts',(71.8024484838239,5.58013977807825,133.526014137426));
#269281=CARTESIAN_POINT('Ctrl Pts',(71.524000860011,5.30600604003494,127.580751192065));
#269282=CARTESIAN_POINT('Ctrl Pts',(71.2455532361981,0.155911964005252,
124.597827826664));
#269283=CARTESIAN_POINT('Ctrl Pts',(70.9671056123853,-5.13745759022245,
127.318404890117));
#269284=CARTESIAN_POINT('Ctrl Pts',(70.6886579885723,-5.70975459779179,
133.242404968692));
#269285=CARTESIAN_POINT('Ctrl Pts',(70.4102103647595,-1.03506606700937,
136.925961393668));
#269286=CARTESIAN_POINT('Ctrl Pts',(70.1317627409465,4.59079761356593,134.98406576223));
#269287=CARTESIAN_POINT('Ctrl Pts',(69.8533151171337,5.99794256020584,129.201225292793));
#269288=CARTESIAN_POINT('Ctrl Pts',(69.5748674933208,1.89327130980037,124.891587869307));
#269289=CARTESIAN_POINT('Ctrl Pts',(69.2964198695077,-3.95122378286636,
126.015499746463));
#269290=CARTESIAN_POINT('Ctrl Pts',(69.0179722456952,-6.16473724709165,
131.540140815303));
#269291=CARTESIAN_POINT('Ctrl Pts',(68.7395246218819,-2.71315834539685,
136.388635827283));
#269292=CARTESIAN_POINT('Ctrl Pts',(68.4610769980694,3.23168053056381,136.105454728543));
#269293=CARTESIAN_POINT('Ctrl Pts',(68.1826293742561,6.20676287530703,130.950827114659));
#269294=CARTESIAN_POINT('Ctrl Pts',(67.9041817504435,3.47813335486666,125.661603945233));
#269295=CARTESIAN_POINT('Ctrl Pts',(67.6257341266304,-2.44673080243567,
125.09832292005));
#269296=CARTESIAN_POINT('Ctrl Pts',(67.3472865028177,-6.12316888174425,
129.778611783445));
#269297=CARTESIAN_POINT('Ctrl Pts',(67.0688388790048,-4.17271389215982,
135.401513714782));
#269298=CARTESIAN_POINT('Ctrl Pts',(66.7903912551918,1.61226131591331,136.799856533191));
#269299=CARTESIAN_POINT('Ctrl Pts',(66.511943631379,5.91564713800617,132.688631501398));
#269300=CARTESIAN_POINT('Ctrl Pts',(66.233496007566,4.78284223570014,126.845853579115));
#269301=CARTESIAN_POINT('Ctrl Pts',(65.9550483837533,-0.745161026381345,
124.640750241348));
#269302=CARTESIAN_POINT('Ctrl Pts',(65.6766007599402,-5.58839770835831,
128.099703730218));
#269303=CARTESIAN_POINT('Ctrl Pts',(65.3981531361275,-5.2961699047596,134.044104768727));
#269304=CARTESIAN_POINT('Ctrl Pts',(65.1197055123145,-0.137020690970298,
137.011339202618));
#269305=CARTESIAN_POINT('Ctrl Pts',(64.8412578885016,5.14804384398771,134.274663544608));
#269306=CARTESIAN_POINT('Ctrl Pts',(64.5628102646887,5.70230758224426,128.348949030369));
#269307=CARTESIAN_POINT('Ctrl Pts',(64.2843626408759,1.01642922563077,124.679637811238));
#269308=CARTESIAN_POINT('Ctrl Pts',(64.0059150170629,-4.60349793400934,
126.638647641779));
#269309=CARTESIAN_POINT('Ctrl Pts',(63.72746739325,-5.9930353856715,132.425744190676));
#269310=CARTESIAN_POINT('Ctrl Pts',(63.4490197694371,-1.87526609395646,
136.722868444874));
#269311=CARTESIAN_POINT('Ctrl Pts',(63.1705721456243,3.96578112626272,135.581173140958));
#269312=CARTESIAN_POINT('Ctrl Pts',(62.8921245218114,6.16246923062527,130.049820488308));
#269313=CARTESIAN_POINT('Ctrl Pts',(62.6136768979985,2.69614916540168,125.211853353112));
#269314=CARTESIAN_POINT('Ctrl Pts',(62.3352292741856,-3.24780026861702,
125.513127184779));
#269315=CARTESIAN_POINT('Ctrl Pts',(62.0567816503727,-6.20717991964031,
130.676786050054));
#269316=CARTESIAN_POINT('Ctrl Pts',(61.7783340265599,-3.46246446211126,
135.957679710507));
#269317=CARTESIAN_POINT('Ctrl Pts',(61.4998864027468,2.46408668530527,136.502924878181));
#269318=CARTESIAN_POINT('Ctrl Pts',(61.2214387789342,6.12626254625314,131.81146788069));
#269319=CARTESIAN_POINT('Ctrl Pts',(60.942991155121,4.15870241175792,126.194528508313));
#269320=CARTESIAN_POINT('Ctrl Pts',(60.6645435313083,-1.63050207523548,
124.813799641521));
#269321=CARTESIAN_POINT('Ctrl Pts',(60.3860959074953,-5.92135480954196,
128.938103656541));
#269322=CARTESIAN_POINT('Ctrl Pts',(60.1076482836825,-4.77077174814381,
134.777406647022));
#269323=CARTESIAN_POINT('Ctrl Pts',(59.8292006598696,0.763917484641806,
136.965674430521));
#269324=CARTESIAN_POINT('Ctrl Pts',(59.5507530360567,5.59660386848551,133.491995816827));
#269325=CARTESIAN_POINT('Ctrl Pts',(59.2723054122438,5.28628470648961,127.548511753291));
#269326=CARTESIAN_POINT('Ctrl Pts',(58.9938577884309,0.11812814859451,124.596993738963));
#269327=CARTESIAN_POINT('Ctrl Pts',(58.715410164618,-5.15858240697801,127.34974263934));
#269328=CARTESIAN_POINT('Ctrl Pts',(58.4369625408051,-5.69480774129836,
133.277116694236));
#269329=CARTESIAN_POINT('Ctrl Pts',(58.1585149169922,-0.997782968190397,
136.932148715521));
#269330=CARTESIAN_POINT('Ctrl Pts',(57.8800672931793,4.61615560827684,134.956042833877));
#269331=CARTESIAN_POINT('Ctrl Pts',(57.6016196693665,5.98807269247603,129.164743816393));
#269332=CARTESIAN_POINT('Ctrl Pts',(57.3231720455535,1.85724350590365,124.880172539454));
#269333=CARTESIAN_POINT('Ctrl Pts',(57.0447244217407,-3.98030173120474,
126.039640693622));
#269334=CARTESIAN_POINT('Ctrl Pts',(56.7662767979277,-6.16014412588574,
131.577653688385));
#269335=CARTESIAN_POINT('Ctrl Pts',(56.4878291741149,-2.67911500864857,
136.405048128532));
#269336=CARTESIAN_POINT('Ctrl Pts',(56.209381550302,3.26388991949243,136.085684354897));
#269337=CARTESIAN_POINT('Ctrl Pts',(55.9309339264891,6.20753946150667,130.913042073662));
#269338=CARTESIAN_POINT('Ctrl Pts',(55.6524863026762,3.44676349355797,125.640526843659));
#269339=CARTESIAN_POINT('Ctrl Pts',(55.3740386788633,-2.48141974121268,
125.113322584571));
#269340=CARTESIAN_POINT('Ctrl Pts',(55.0955910550504,-6.12929945790263,
129.815904255142));
#269341=CARTESIAN_POINT('Ctrl Pts',(54.8171434312375,-4.14465240570495,
135.426829034002));
#269342=CARTESIAN_POINT('Ctrl Pts',(54.5386958074246,1.64872772980914,136.789931158292));
#269343=CARTESIAN_POINT('Ctrl Pts',(54.2602481836117,5.92700762645589,132.652586367033));
#269344=CARTESIAN_POINT('Ctrl Pts',(53.9818005597989,4.75865706480954,126.81681240286));
#269345=CARTESIAN_POINT('Ctrl Pts',(53.703352935986,-0.78266686607524,124.645400445441));
#269346=CARTESIAN_POINT('Ctrl Pts',(53.4249053121731,-5.604758182439,128.133772004274));
#269347=CARTESIAN_POINT('Ctrl Pts',(53.1464576883601,-5.27635053680027,
134.076284033214));
#269348=CARTESIAN_POINT('Ctrl Pts',(52.8680100645473,-0.0992345118958833,
137.012058285519));
#269349=CARTESIAN_POINT('Ctrl Pts',(52.5895624407343,5.1690731815654,134.243261643865));
#269350=CARTESIAN_POINT('Ctrl Pts',(52.3111148169216,5.68725514443172,128.314282958697));
#269351=CARTESIAN_POINT('Ctrl Pts',(52.0326671931086,0.979127467424884,
124.673563994973));
#269352=CARTESIAN_POINT('Ctrl Pts',(51.7542195692957,-4.62877051910935,
126.666747621346));
#269353=CARTESIAN_POINT('Ctrl Pts',(51.4757719454828,-5.98305452659317,
132.462195457613));
#269354=CARTESIAN_POINT('Ctrl Pts',(51.1973243216699,-1.83920371260068,
136.734174065611));
#269355=CARTESIAN_POINT('Ctrl Pts',(50.9188766978571,3.99478546317524,135.556943802347));
#269356=CARTESIAN_POINT('Ctrl Pts',(50.6404290740441,6.15776195441257,130.012321768865));
#269357=CARTESIAN_POINT('Ctrl Pts',(50.3619814502312,2.66205603294,125.195544744091));
#269358=CARTESIAN_POINT('Ctrl Pts',(50.0835338264184,-3.27994933413751,
125.532995501151));
#269359=CARTESIAN_POINT('Ctrl Pts',(49.8050862026055,-6.20784149757545,
130.714573279694));
#269360=CARTESIAN_POINT('Ctrl Pts',(49.5266385787925,-3.43103059465853,
135.978661235386));
#269361=CARTESIAN_POINT('Ctrl Pts',(49.2481909549797,2.4987298095866,136.487819701939));
#269362=CARTESIAN_POINT('Ctrl Pts',(48.9697433311668,6.13227958855924,131.774156922365));
#269363=CARTESIAN_POINT('Ctrl Pts',(48.6912957073539,4.13056400415832,126.169298715863));
#269364=CARTESIAN_POINT('Ctrl Pts',(48.412848083541,-1.66693811079436,124.823835961664));
#269365=CARTESIAN_POINT('Ctrl Pts',(48.1344004597282,-5.93260553638082,
128.974183201367));
#269366=CARTESIAN_POINT('Ctrl Pts',(47.8559528359152,-4.7464982979263,134.806374077418));
#269367=CARTESIAN_POINT('Ctrl Pts',(47.5775052121024,0.801408996989757,
136.960910093092));
#269368=CARTESIAN_POINT('Ctrl Pts',(47.2990575882894,5.61286057467834,133.457877904919));
#269369=CARTESIAN_POINT('Ctrl Pts',(47.0206099644766,5.26636748772036,127.516392961194));
#269370=CARTESIAN_POINT('Ctrl Pts',(46.7421623406636,0.0803399559020909,
124.596389667526));
#269371=CARTESIAN_POINT('Ctrl Pts',(46.4637147168508,-5.17951607056515,
127.381208400702));
#269372=CARTESIAN_POINT('Ctrl Pts',(46.1852670930379,-5.67964986161014,
133.311736790894));
#269373=CARTESIAN_POINT('Ctrl Pts',(45.9068194692249,-0.960462896156299,
136.938108969933));
#269374=CARTESIAN_POINT('Ctrl Pts',(45.6283718454121,4.64134254964412,134.927866063412));
#269375=CARTESIAN_POINT('Ctrl Pts',(45.3499242215992,5.97798093451044,129.128323096598));
#269376=CARTESIAN_POINT('Ctrl Pts',(45.0714765977863,1.82114688116607,124.868976732569));
#269377=CARTESIAN_POINT('Ctrl Pts',(44.7930289739735,-4.00923218799886,
126.063958199228));
#269378=CARTESIAN_POINT('Ctrl Pts',(44.5145813501605,-6.15532273827383,
131.615137906808));
#269379=CARTESIAN_POINT('Ctrl Pts',(44.2361337263477,-2.644972396308,136.421252894246));
#269380=CARTESIAN_POINT('Ctrl Pts',(43.9576861025347,3.29597836378001,136.065718279858));
#269381=CARTESIAN_POINT('Ctrl Pts',(43.6792384787219,6.20808602504863,130.875253005433));
#269382=CARTESIAN_POINT('Ctrl Pts',(43.4007908549089,3.41526591116036,125.619641089845));
#269383=CARTESIAN_POINT('Ctrl Pts',(43.1223432310961,-2.5160167300689,125.128533132602));
#269384=CARTESIAN_POINT('Ctrl Pts',(42.8438956072832,-6.13520291061547,
129.853233354452));
#269385=CARTESIAN_POINT('Ctrl Pts',(42.5654479834703,-4.11643733763101,
135.451973065955));
#269386=CARTESIAN_POINT('Ctrl Pts',(42.2870003596574,1.68513304949262,136.779783985877));
#269387=CARTESIAN_POINT('Ctrl Pts',(42.0085527358444,5.93814848745852,132.616472745983));
#269388=CARTESIAN_POINT('Ctrl Pts',(41.7301051120316,4.73429556013123,126.787918986671));
#269389=CARTESIAN_POINT('Ctrl Pts',(41.4516574882187,-0.820143703760798,
124.65027887207));
#269390=CARTESIAN_POINT('Ctrl Pts',(41.1732098644058,-5.62091097014408,
128.167939237972));
#269391=CARTESIAN_POINT('Ctrl Pts',(40.8947622405929,-5.25633565173145,
134.108342055376));
#269392=CARTESIAN_POINT('Ctrl Pts',(40.61631461678,-0.0614446556499193,
137.012547339898));
#269393=CARTESIAN_POINT('Ctrl Pts',(40.3378669929672,5.18991097723558,134.211732313379));
#269394=CARTESIAN_POINT('Ctrl Pts',(40.0594193691542,5.67199196328813,128.279709157768));
#269395=CARTESIAN_POINT('Ctrl Pts',(39.7809717453414,0.941789427290636,
124.66771735763));
#269396=CARTESIAN_POINT('Ctrl Pts',(39.5025241215285,-4.65387158341555,
126.695000921683));
#269397=CARTESIAN_POINT('Ctrl Pts',(39.2240764977156,-5.97285196322902,
132.49858529287));
#269398=CARTESIAN_POINT('Ctrl Pts',(38.9456288739027,-1.80307317887526,
136.745259954929));
#269399=CARTESIAN_POINT('Ctrl Pts',(38.6671812500898,4.02364177184326,135.532538355018));
#269400=CARTESIAN_POINT('Ctrl Pts',(38.3887336262769,6.15282650006613,129.974852398711));
#269401=CARTESIAN_POINT('Ctrl Pts',(38.110286002464,2.62786425701304,125.179443971804));
#269402=CARTESIAN_POINT('Ctrl Pts',(37.8318383786511,-3.31197685992897,
125.553059149895));
#269403=CARTESIAN_POINT('Ctrl Pts',(37.5533907548383,-6.20827304166094,
130.752363836438));
#269404=CARTESIAN_POINT('Ctrl Pts',(37.2749431310254,-3.3994695891056,135.999451024653));
#269405=CARTESIAN_POINT('Ctrl Pts',(36.9964955072125,2.53328034251594,136.47250392303));
#269406=CARTESIAN_POINT('Ctrl Pts',(36.7180478833995,6.13806939699002,131.73681002788));
#269407=CARTESIAN_POINT('Ctrl Pts',(36.4396002595867,4.10227253699055,126.144240677337));
#269408=CARTESIAN_POINT('Ctrl Pts',(36.1611526357737,-1.70331237734853,
124.834093892349));
#269409=CARTESIAN_POINT('Ctrl Pts',(35.8827050119609,-5.94363642833981,
129.01033056409));
#269410=CARTESIAN_POINT('Ctrl Pts',(35.604257388148,-4.72204896446884,134.835193211735));
#269411=CARTESIAN_POINT('Ctrl Pts',(35.3258097643351,0.838870812832614,
136.955917622458));
#269412=CARTESIAN_POINT('Ctrl Pts',(35.0473621405222,5.62890929425843,133.423661665951));
#269413=CARTESIAN_POINT('Ctrl Pts',(34.7689145167094,5.24625512176713,127.484396005948));
#269414=CARTESIAN_POINT('Ctrl Pts',(34.4904668928964,0.0425487861828518,
124.596015634733));
#269415=CARTESIAN_POINT('Ctrl Pts',(34.2120192690835,-5.20025780527969,
127.412801008228));
#269416=CARTESIAN_POINT('Ctrl Pts',(33.9335716452707,-5.66428152040741,
133.346263975806));
#269417=CARTESIAN_POINT('Ctrl Pts',(33.6551240214578,-0.923107233816384,
136.943841936043));
#269418=CARTESIAN_POINT('Ctrl Pts',(33.3766763976448,4.66635750435639,134.899536494936));
#269419=CARTESIAN_POINT('Ctrl Pts',(33.098228773832,5.96766766026296,129.091964482989));
#269420=CARTESIAN_POINT('Ctrl Pts',(32.8197811500191,1.78498277316083,124.858000863516));
#269421=CARTESIAN_POINT('Ctrl Pts',(32.5413335262063,-4.03801408121996,
126.08845136219));
#269422=CARTESIAN_POINT('Ctrl Pts',(32.2628859023933,-6.15027326291425,
131.65259208158));
#269423=CARTESIAN_POINT('Ctrl Pts',(31.9844382785804,-2.6107317735426,136.437249523951));
#269424=CARTESIAN_POINT('Ctrl Pts',(31.7059906547675,3.32794467437699,136.045557243275));
#269425=CARTESIAN_POINT('Ctrl Pts',(31.4275430309546,6.20840254567991,130.837461310262));
#269426=CARTESIAN_POINT('Ctrl Pts',(31.1490954071417,3.3836417748287,125.598947457719));
#269427=CARTESIAN_POINT('Ctrl Pts',(30.8706477833288,-2.55052048699994,
125.143954000505));
#269428=CARTESIAN_POINT('Ctrl Pts',(30.5922001595159,-6.14087902112821,
129.890597698133));
#269429=CARTESIAN_POINT('Ctrl Pts',(30.3137525357031,-4.08806973345779,
135.476944878919));
#269430=CARTESIAN_POINT('Ctrl Pts',(30.0353049118902,1.72147592595096,136.769415391952));
#269431=CARTESIAN_POINT('Ctrl Pts',(29.7568572880773,5.94906930818524,132.58029197645));
#269432=CARTESIAN_POINT('Ctrl Pts',(29.4784096642643,4.70975862438989,126.759174401203));
#269433=CARTESIAN_POINT('Ctrl Pts',(29.1999620404515,-0.857590150719802,
124.65538534046));
#269434=CARTESIAN_POINT('Ctrl Pts',(28.9215144166386,-5.63685547292606,
128.202204165235));
#269435=CARTESIAN_POINT('Ctrl Pts',(28.6430667928257,-5.23612599121204,
134.140277647291));
#269436=CARTESIAN_POINT('Ctrl Pts',(28.3646191690128,-0.0236525225496446,
137.012806347637));
#269437=CARTESIAN_POINT('Ctrl Pts',(28.0861715451999,5.2105564588459,134.180076721482));
#269438=CARTESIAN_POINT('Ctrl Pts',(27.807723921387,5.65651860439647,128.245228908728));
#269439=CARTESIAN_POINT('Ctrl Pts',(27.5292762975741,0.904416488802812,
124.662098115861));
#269440=CARTESIAN_POINT('Ctrl Pts',(27.2508286737613,-4.67880019679877,
126.723406495856));
#269441=CARTESIAN_POINT('Ctrl Pts',(26.9723810499484,-5.96242807363892,
132.53491234801));
#269442=CARTESIAN_POINT('Ctrl Pts',(26.6939334261354,-1.76687583160983,
136.756125702037));
#269443=CARTESIAN_POINT('Ctrl Pts',(26.4154858023226,4.05234898298581,135.507957703324));
#269444=CARTESIAN_POINT('Ctrl Pts',(26.1370381785097,6.14766305047102,129.937413766291));
#269445=CARTESIAN_POINT('Ctrl Pts',(25.8585905546968,2.59357510460964,125.163551632871));
#269446=CARTESIAN_POINT('Ctrl Pts',(25.5801429308839,-3.34388165920016,
125.573317387547));
#269447=CARTESIAN_POINT('Ctrl Pts',(25.301695307071,-6.2084745359058,130.790156319941));
#269448=CARTESIAN_POINT('Ctrl Pts',(25.0232476832582,-3.36778261495664,
136.020048307934));
#269449=CARTESIAN_POINT('Ctrl Pts',(24.7448000594452,2.56773700381057,136.456978108987));
#269450=CARTESIAN_POINT('Ctrl Pts',(24.4663524356323,6.14363175700203,131.69942858114));
#269451=CARTESIAN_POINT('Ctrl Pts',(24.1879048118195,4.07382905860539,126.11935532127));
#269452=CARTESIAN_POINT('Ctrl Pts',(23.9094571880065,-1.73962352703587,
124.844573053462));
#269453=CARTESIAN_POINT('Ctrl Pts',(23.6310095641937,-5.95444707666522,
129.046544405257));
#269454=CARTESIAN_POINT('Ctrl Pts',(23.3525619403807,-4.69742465375045,
134.863862982068));
#269455=CARTESIAN_POINT('Ctrl Pts',(23.0741143165679,0.876301544009003,
136.950697203617));
#269456=CARTESIAN_POINT('Ctrl Pts',(22.795666692755,5.64474943253441,133.389348367819));
#269457=CARTESIAN_POINT('Ctrl Pts',(22.5172190689421,5.22594835390121,127.452522073212));
#269458=CARTESIAN_POINT('Ctrl Pts',(22.2387714451292,0.0047560398029127,
124.595871654449));
#269459=CARTESIAN_POINT('Ctrl Pts',(21.9603238213163,-5.22080684252888,
127.444519291243));
#269460=CARTESIAN_POINT('Ctrl Pts',(21.6818761975034,-5.64870328716988,
133.380696969555));
#269461=CARTESIAN_POINT('Ctrl Pts',(21.4034285736905,-0.885717365398449,
136.949347401415));
#269462=CARTESIAN_POINT('Ctrl Pts',(21.1249809498776,4.69119954547528,134.871055178212));
#269463=CARTESIAN_POINT('Ctrl Pts',(20.8465333260648,5.95713325189572,129.055669322849));
#269464=CARTESIAN_POINT('Ctrl Pts',(20.5680857022518,1.74875252196249,124.847245339011));
#269465=CARTESIAN_POINT('Ctrl Pts',(20.289638078439,-4.06664634434428,126.113119274905));
#269466=CARTESIAN_POINT('Ctrl Pts',(20.011190454626,-6.14499588691713,131.690014824823));
#269467=CARTESIAN_POINT('Ctrl Pts',(19.7327428308132,-2.57639440915122,
136.453037424885));
#269468=CARTESIAN_POINT('Ctrl Pts',(19.4542952070003,3.35978766676044,136.025201992224));
#269469=CARTESIAN_POINT('Ctrl Pts',(19.1758475831874,6.20848901167171,130.799668388532));
#269470=CARTESIAN_POINT('Ctrl Pts',(18.8973999593745,3.3518922564065,125.578446714094));
#269471=CARTESIAN_POINT('Ctrl Pts',(18.6189523355616,-2.58492973345636,
125.159584616859));
#269472=CARTESIAN_POINT('Ctrl Pts',(18.3405047117487,-6.14632757911053,
129.927995901635));
#269473=CARTESIAN_POINT('Ctrl Pts',(18.0620570879358,-4.05955064435711,
135.501743547556));
#269474=CARTESIAN_POINT('Ctrl Pts',(17.7836094641229,1.75775501248606,136.758825760728));
#269475=CARTESIAN_POINT('Ctrl Pts',(17.5051618403101,5.95976968396092,132.544045399129));
#269476=CARTESIAN_POINT('Ctrl Pts',(17.2267142164972,4.68504716681072,126.730579711598));
#269477=CARTESIAN_POINT('Ctrl Pts',(16.9482665926842,-0.8950048193604,124.660719661391));
#269478=CARTESIAN_POINT('Ctrl Pts',(16.6698189688713,-5.65259109995534,
128.236565516362));
#269479=CARTESIAN_POINT('Ctrl Pts',(16.3913713450585,-5.21572230411858,
134.172089625574));
#269480=CARTESIAN_POINT('Ctrl Pts',(16.1129237212456,0.0141404870033325,
137.012835299135));
#269481=CARTESIAN_POINT('Ctrl Pts',(15.8344760974327,5.23100886137047,134.148296041183));
#269482=CARTESIAN_POINT('Ctrl Pts',(15.5560284736198,5.64083564112771,128.210843489254));
#269483=CARTESIAN_POINT('Ctrl Pts',(15.2775808498069,0.8670100368296,124.656706477888));
#269484=CARTESIAN_POINT('Ctrl Pts',(14.999133225994,-4.70355543551987,126.751963291284));
#269485=CARTESIAN_POINT('Ctrl Pts',(14.7206856021811,-5.95178324408404,
132.571175276918));
#269486=CARTESIAN_POINT('Ctrl Pts',(14.4422379783683,-1.73061301211068,
136.766770904302));
#269487=CARTESIAN_POINT('Ctrl Pts',(14.1637903545553,4.08090603284655,135.48320275811));
#269488=CARTESIAN_POINT('Ctrl Pts',(13.8853427307424,6.14227179696077,129.900007258904));
#269489=CARTESIAN_POINT('Ctrl Pts',(13.6068951069296,2.55918984632695,125.147868316191));
#269490=CARTESIAN_POINT('Ctrl Pts',(13.3284474831167,-3.37566254970675,
125.593769463429));
#269491=CARTESIAN_POINT('Ctrl Pts',(13.0499998593037,-6.20844597284355,
130.827949329789));
#269492=CARTESIAN_POINT('Ctrl Pts',(12.7715522354909,-3.33597084638438,
136.04045232199));
#269493=CARTESIAN_POINT('Ctrl Pts',(12.493104611678,2.60209851666622,136.441242835124));
#269494=CARTESIAN_POINT('Ctrl Pts',(12.2146569878651,6.14896646247997,131.662013967328));
#269495=CARTESIAN_POINT('Ctrl Pts',(11.9362093640522,4.04523462298623,126.094643569795));
#269496=CARTESIAN_POINT('Ctrl Pts',(11.6577617402393,-1.77587021433397,
124.855273056695));
#269497=CARTESIAN_POINT('Ctrl Pts',(11.3793141164265,-5.96503708076441,
129.08282338295));
#269498=CARTESIAN_POINT('Ctrl Pts',(11.1008664926135,-4.67262627823404,
134.892382326048));
#269499=CARTESIAN_POINT('Ctrl Pts',(10.8224188688007,0.913699803509421,
136.945249030013));
#269500=CARTESIAN_POINT('Ctrl Pts',(10.5439712449878,5.6603804025445,133.354939282016));
#269501=CARTESIAN_POINT('Ctrl Pts',(10.2655236211749,5.20544793659703,127.420772344084));
#269502=CARTESIAN_POINT('Ctrl Pts',(9.98707599736195,-0.0330368828140487,
124.595957732005));
#269503=CARTESIAN_POINT('Ctrl Pts',(9.70862837354909,-5.24116242086055,
127.476362074414));
#269504=CARTESIAN_POINT('Ctrl Pts',(9.43018074973619,-5.63291573915475,
133.415034496211));
#269505=CARTESIAN_POINT('Ctrl Pts',(9.15173312592329,-0.848294676398009,
136.954625162043));
#269506=CARTESIAN_POINT('Ctrl Pts',(8.87328550211039,4.71586775246963,134.842423168626));
#269507=CARTESIAN_POINT('Ctrl Pts',(8.59483787829755,5.94637809976527,129.019438961107));
#269508=CARTESIAN_POINT('Ctrl Pts',(8.3163902544846,1.71245747009635,124.836710557603));
#269509=CARTESIAN_POINT('Ctrl Pts',(8.03794263067172,-4.09512791639282,
126.137961023291));
#269510=CARTESIAN_POINT('Ctrl Pts',(7.75949500685887,-6.1394908058375,131.727404749824));
#269511=CARTESIAN_POINT('Ctrl Pts',(7.48104738304595,-2.54196157551782,
136.468616012024));
#269512=CARTESIAN_POINT('Ctrl Pts',(7.20259975923305,3.39150616097622,136.004653280976));
#269513=CARTESIAN_POINT('Ctrl Pts',(6.92415213542018,6.20834541982004,130.761875640674));
#269514=CARTESIAN_POINT('Ctrl Pts',(6.64570451160728,3.32001853238404,125.558139618628));
#269515=CARTESIAN_POINT('Ctrl Pts',(6.36725688779438,-2.61924319439064,
125.175424402463));
#269516=CARTESIAN_POINT('Ctrl Pts',(6.08880926398148,-6.15154838266407,
129.965426579154));
#269517=CARTESIAN_POINT('Ctrl Pts',(5.81036164016863,-4.03088112711464,
135.52636815294));
#269518=CARTESIAN_POINT('Ctrl Pts',(5.53191401635571,1.79396896476278,136.748015484609));
#269519=CARTESIAN_POINT('Ctrl Pts',(5.2534663925428,5.97024921827925,132.507734357147));
#269520=CARTESIAN_POINT('Ctrl Pts',(4.97501876872993,4.66016210308585,126.702135977443));
#269521=CARTESIAN_POINT('Ctrl Pts',(4.69657114491704,-0.932386323268277,
124.666281637197));
#269522=CARTESIAN_POINT('Ctrl Pts',(4.41812352110413,-5.66811726814286,
128.27102201808));
#269523=CARTESIAN_POINT('Ctrl Pts',(4.13967589729124,-5.19512534651691,
134.203776811419));
#269524=CARTESIAN_POINT('Ctrl Pts',(3.86122827347838,0.051932972575587,
137.012634193321));
#269525=CARTESIAN_POINT('Ctrl Pts',(3.58278064966546,5.25126742693796,134.116391450127));
#269526=CARTESIAN_POINT('Ctrl Pts',(3.30433302585255,5.62494365461986,128.176554173511));
#269527=CARTESIAN_POINT('Ctrl Pts',(3.02588540203969,0.829571457480427,
124.651542643499));
#269528=CARTESIAN_POINT('Ctrl Pts',(2.74743777822681,-4.72813638226476,
126.780670249786));
#269529=CARTESIAN_POINT('Ctrl Pts',(2.46899015441389,-5.9409178690121,132.607372735859));
#269530=CARTESIAN_POINT('Ctrl Pts',(2.19054253060099,-1.69428606410994,
136.77719516726));
#269531=CARTESIAN_POINT('Ctrl Pts',(1.91209490678813,4.10931186323347,135.458274436681));
#269532=CARTESIAN_POINT('Ctrl Pts',(1.63364728297522,6.13665293931019,129.862634262664));
#269533=CARTESIAN_POINT('Ctrl Pts',(1.35519965916232,2.52470975632363,125.132394602912));
#269534=CARTESIAN_POINT('Ctrl Pts',(1.07675203534945,-3.40731835379603,
125.614414619682));
#269535=CARTESIAN_POINT('Ctrl Pts',(0.798304411536565,-6.20818735353264,
130.86574146555));
#269536=CARTESIAN_POINT('Ctrl Pts',(0.519856787723634,-3.30403546218559,
136.060662310741));
#269537=CARTESIAN_POINT('Ctrl Pts',(0.241409163910791,2.63636360780418,
136.425298684517));
#269538=CARTESIAN_POINT('Ctrl Pts',(-0.0370384599021062,6.15407331574431,
131.624567572855));
#269539=CARTESIAN_POINT('Ctrl Pts',(-0.315486083715014,4.01649028971072,
126.070106338619));
#269540=CARTESIAN_POINT('Ctrl Pts',(-0.593933707527915,-1.81205109610819,
124.866193505555));
#269541=CARTESIAN_POINT('Ctrl Pts',(-0.872381331340776,-5.97540604822092,
129.119166152838));
#269542=CARTESIAN_POINT('Ctrl Pts',(-1.15082895515369,-4.6476547568326,
134.920750186879));
#269543=CARTESIAN_POINT('Ctrl Pts',(-1.42927657896659,0.951064205527318,
136.939573303531));
#269544=CARTESIAN_POINT('Ctrl Pts',(-1.70772420277945,5.67580162507719,
133.320435683583));
#269545=CARTESIAN_POINT('Ctrl Pts',(-1.98617182659235,5.18475462950527,
127.389147995065));
#269546=CARTESIAN_POINT('Ctrl Pts',(-2.26461945040527,-0.0708285812371651,
124.596273864213));
#269547=CARTESIAN_POINT('Ctrl Pts',(-2.54306707421816,-5.26132378599129,
127.508328177794));
#269548=CARTESIAN_POINT('Ctrl Pts',(-2.82151469803103,-5.61691946137538,
133.449275283389));
#269549=CARTESIAN_POINT('Ctrl Pts',(-3.09996232184393,-0.810840553526189,
136.959675022356));
#269550=CARTESIAN_POINT('Ctrl Pts',(-3.37840994565684,4.74036121125036,
134.813641527147));
#269551=CARTESIAN_POINT('Ctrl Pts',(-3.6568575694697,5.93540260240737,128.983274740293));
#269552=CARTESIAN_POINT('Ctrl Pts',(-3.9353051932826,1.6760989624889,124.826396909662));
#269553=CARTESIAN_POINT('Ctrl Pts',(-4.21375281709551,-4.12345774197041,
126.162975686831));
#269554=CARTESIAN_POINT('Ctrl Pts',(-4.49220044090841,-6.13375822366836,
131.764760471086));
#269555=CARTESIAN_POINT('Ctrl Pts',(-4.77064806472125,-2.50743454856317,
136.483984708096));
#269556=CARTESIAN_POINT('Ctrl Pts',(-5.04909568853418,3.4230989816841,135.983911870971));
#269557=CARTESIAN_POINT('Ctrl Pts',(-5.32754331234708,6.20797177544568,
130.724084467112));
#269558=CARTESIAN_POINT('Ctrl Pts',(-5.60599093615995,3.28802178385396,
125.538026923812));
#269559=CARTESIAN_POINT('Ctrl Pts',(-5.88443855997284,-2.65345959830539,
125.191472770368));
#269560=CARTESIAN_POINT('Ctrl Pts',(-6.16288618378574,-6.15654123833006,
130.002888343683));
#269561=CARTESIAN_POINT('Ctrl Pts',(-6.44133380759864,-4.00206224408943,
135.550817782599));
#269562=CARTESIAN_POINT('Ctrl Pts',(-6.71978143141151,1.83011644085978,
136.736984964173));
#269563=CARTESIAN_POINT('Ctrl Pts',(-6.9982290552244,5.98050752281724,132.471360196026));
#269564=CARTESIAN_POINT('Ctrl Pts',(-7.27667667903734,4.63510435534053,
126.673844252731));
#269565=CARTESIAN_POINT('Ctrl Pts',(-7.55512430285017,-0.969733277257762,
124.672071061776));
#269566=CARTESIAN_POINT('Ctrl Pts',(-7.83357192666308,-5.68343340216059,
128.305572393592));
#269567=CARTESIAN_POINT('Ctrl Pts',(-8.112019550476,-5.17433588163501,134.235338030648));
#269568=CARTESIAN_POINT('Ctrl Pts',(-8.39046717428886,0.0897235337524442,
137.012203037646));
#269569=CARTESIAN_POINT('Ctrl Pts',(-8.66891479810176,5.27133140485959,
134.084364130551));
#269570=CARTESIAN_POINT('Ctrl Pts',(-8.94736242191464,5.60884323375645,
128.142362232103));
#269571=CARTESIAN_POINT('Ctrl Pts',(-9.22581004572757,0.792102138056052,
124.646606804043));
#269572=CARTESIAN_POINT('Ctrl Pts',(-9.50425766954039,-4.75254212617725,
126.809526307613));
#269573=CARTESIAN_POINT('Ctrl Pts',(-9.78270529335335,-5.92983235104376,
132.643503383524));
#269574=CARTESIAN_POINT('Ctrl Pts',(-10.0611529171662,-1.65789633371603,
136.787398104638));
#269575=CARTESIAN_POINT('Ctrl Pts',(-10.3396005409791,4.13756542155812,
135.433173662763));
#269576=CARTESIAN_POINT('Ctrl Pts',(-10.618048164792,6.13080668572826,129.82529616244));
#269577=CARTESIAN_POINT('Ctrl Pts',(-10.8964957886049,2.49013611227157,
125.11713106642));
#269578=CARTESIAN_POINT('Ctrl Pts',(-11.1749434124178,-3.4388478984508,
125.635252091294));
#269579=CARTESIAN_POINT('Ctrl Pts',(-11.4533910362307,-6.20769868755626,
130.90353132682));
#269580=CARTESIAN_POINT('Ctrl Pts',(-11.7318386600436,-3.2719776457377,
136.080677525301));
#269581=CARTESIAN_POINT('Ctrl Pts',(-12.0102862838565,2.67053100751937,
136.409146247984));
#269582=CARTESIAN_POINT('Ctrl Pts',(-12.2887339076694,6.15895212755882,
131.587090785312));
#269583=CARTESIAN_POINT('Ctrl Pts',(-12.5671815314823,3.98759712391021,
126.045744536976));
#269584=CARTESIAN_POINT('Ctrl Pts',(-12.8456291552951,-1.84816483166266,
124.877333995382));
#269585=CARTESIAN_POINT('Ctrl Pts',(-13.1240767791081,-5.98555359480885,
129.155571368227));
#269586=CARTESIAN_POINT('Ctrl Pts',(-13.4025244029209,-4.62251101487491,
134.948965513381));
#269587=CARTESIAN_POINT('Ctrl Pts',(-13.6809720267338,0.988393365511613,
136.933670234486));
#269588=CARTESIAN_POINT('Ctrl Pts',(-13.9594196505467,5.69101252869335,
133.285838851062));
#269589=CARTESIAN_POINT('Ctrl Pts',(-14.2378672743596,5.16386919942402,
127.357650198006));
#269590=CARTESIAN_POINT('Ctrl Pts',(-14.5163148981725,-0.108617655081171,
124.59682003936));
#269591=CARTESIAN_POINT('Ctrl Pts',(-14.7947625219854,-5.28129019083405,
127.540416416869));
#269592=CARTESIAN_POINT('Ctrl Pts',(-15.0732101457983,-5.60071504657988,
133.483418062279));
#269593=CARTESIAN_POINT('Ctrl Pts',(-15.3516577696111,-0.77335638465969,
136.96449679523));
#269594=CARTESIAN_POINT('Ctrl Pts',(-15.6301053934241,4.76467901420313,
134.784711320289));
#269595=CARTESIAN_POINT('Ctrl Pts',(-15.908553017237,5.92420716652329,128.947178000488));
#269596=CARTESIAN_POINT('Ctrl Pts',(-16.1870006410499,1.63967834641818,
124.816304777366));
#269597=CARTESIAN_POINT('Ctrl Pts',(-16.4654482648627,-4.15163477130477,
126.188162338596));
#269598=CARTESIAN_POINT('Ctrl Pts',(-16.7438958886757,-6.12779835283271,
131.802080604377));
#269599=CARTESIAN_POINT('Ctrl Pts',(-17.0223435124885,-2.4728146076992,
136.499142943608));
#269600=CARTESIAN_POINT('Ctrl Pts',(-17.3007911363014,3.45456495820035,
135.96297853079));
#269601=CARTESIAN_POINT('Ctrl Pts',(-17.5792387601143,6.20736809239421,
130.686296268213));
#269602=CARTESIAN_POINT('Ctrl Pts',(-17.8576863839272,3.25590319646751,
125.518109374927));
#269603=CARTESIAN_POINT('Ctrl Pts',(-18.13613400774,-2.6875776772989,125.207729125896));
#269604=CARTESIAN_POINT('Ctrl Pts',(-18.414581631553,-6.16130596109642,
130.040379807061));
#269605=CARTESIAN_POINT('Ctrl Pts',(-18.6930292553659,-3.97309506317598,
135.575091530542));
#269606=CARTESIAN_POINT('Ctrl Pts',(-18.9714768791788,1.86619610131902,
136.72573460816));
#269607=CARTESIAN_POINT('Ctrl Pts',(-19.2499245029916,5.99054421744964,
132.434924263623));
#269608=CARTESIAN_POINT('Ctrl Pts',(-19.5283721268046,4.6098748520987,126.645705585822));
#269609=CARTESIAN_POINT('Ctrl Pts',(-19.8068197506174,-1.00704429742433,
124.678087720601));
#269610=CARTESIAN_POINT('Ctrl Pts',(-20.0852673744304,-5.6985389344635,
128.340215362621));
#269611=CARTESIAN_POINT('Ctrl Pts',(-20.3637149982432,-5.15335467983417,
134.266772113748));
#269612=CARTESIAN_POINT('Ctrl Pts',(-20.6421626220562,0.127510770190762,
137.011541848088));
#269613=CARTESIAN_POINT('Ctrl Pts',(-20.920610245869,5.29120005165768,134.05221526924));
#269614=CARTESIAN_POINT('Ctrl Pts',(-21.1990578696819,5.59253497514422,
128.108268932023));
#269615=CARTESIAN_POINT('Ctrl Pts',(-21.4775054934948,0.754603466995427,
124.64189914242));
#269616=CARTESIAN_POINT('Ctrl Pts',(-21.7559531173077,-4.77677176289349,
126.838530395495));
#269617=CARTESIAN_POINT('Ctrl Pts',(-22.0344007411205,-5.91852710095694,
132.679565881077));
#269618=CARTESIAN_POINT('Ctrl Pts',(-22.3128483649335,-1.62144516936395,
136.797379338361));
#269619=CARTESIAN_POINT('Ctrl Pts',(-22.5912959887463,4.16566566087426,
135.407901366475));
#269620=CARTESIAN_POINT('Ctrl Pts',(-22.8697436125593,6.12473325285015,
129.787994341809));
#269621=CARTESIAN_POINT('Ctrl Pts',(-23.1481912363721,2.45547019531011,
125.102078272311));
#269622=CARTESIAN_POINT('Ctrl Pts',(-23.426638860185,-3.47025001533206,
125.656281106122));
#269623=CARTESIAN_POINT('Ctrl Pts',(-23.7050864839979,-6.20697999302203,
130.941317513284));
#269624=CARTESIAN_POINT('Ctrl Pts',(-23.9835341078108,-3.23979858495512,
136.100497223997));
#269625=CARTESIAN_POINT('Ctrl Pts',(-24.2619817316237,2.70459944972584,
136.392786124057));
#269626=CARTESIAN_POINT('Ctrl Pts',(-24.5404293554366,6.16360271713728,
131.549584993415));
#269627=CARTESIAN_POINT('Ctrl Pts',(-24.8188769792495,3.95855619623184,
126.021559067602));
#269628=CARTESIAN_POINT('Ctrl Pts',(-25.0973246030624,-1.88421008278963,
124.88869411336));
#269629=CARTESIAN_POINT('Ctrl Pts',(-25.3757722268753,-5.99547934450715,
129.192037680109));
#269630=CARTESIAN_POINT('Ctrl Pts',(-25.6542198506882,-4.59719598407162,
134.977027260026));
#269631=CARTESIAN_POINT('Ctrl Pts',(-25.932667474501,1.02568590021626,136.92754004162));
#269632=CARTESIAN_POINT('Ctrl Pts',(-26.211115098314,5.7060125497474,133.251150066453));
#269633=CARTESIAN_POINT('Ctrl Pts',(-26.4895627221268,5.14279242027056,
127.326280120068));
#269634=CARTESIAN_POINT('Ctrl Pts',(-26.7680103459397,-0.146402704058008,
124.597596237205));
#269635=CARTESIAN_POINT('Ctrl Pts',(-27.0464579697526,-5.30106089552683,
127.572625602596));
#269636=CARTESIAN_POINT('Ctrl Pts',(-27.3249055935655,-5.58430309522854,
133.517461567711));
#269637=CARTESIAN_POINT('Ctrl Pts',(-27.6033532173784,-0.735843558787732,
136.969090301993));
#269638=CARTESIAN_POINT('Ctrl Pts',(-27.8818008411913,4.78882026022281,
134.755633620073));
#269639=CARTESIAN_POINT('Ctrl Pts',(-28.1602484650042,5.91279220696403,
128.911150079267));
#269640=CARTESIAN_POINT('Ctrl Pts',(-28.4386960888171,1.60319697146318,
124.806434534681));
#269641=CARTESIAN_POINT('Ctrl Pts',(-28.7171437126299,-4.17965796028613,
126.213520045287));
#269642=CARTESIAN_POINT('Ctrl Pts',(-28.9955913364429,-6.12161141417542,
131.839363766787));
#269643=CARTESIAN_POINT('Ctrl Pts',(-29.2740389602557,-2.43810303578058,
136.514090156867));
#269644=CARTESIAN_POINT('Ctrl Pts',(-29.5524865840687,3.48590292454168,
135.941854036124));
#269645=CARTESIAN_POINT('Ctrl Pts',(-29.8309342078815,6.20653439303521,
130.648512444231));
#269646=CARTESIAN_POINT('Ctrl Pts',(-30.1093818316944,3.22366396039099,
125.498387710026));
#269647=CARTESIAN_POINT('Ctrl Pts',(-30.3878294555073,-2.72159616711309,
125.224192866663));
#269648=CARTESIAN_POINT('Ctrl Pts',(-30.6662770793202,-6.16584237440457,
130.077899580028));
#269649=CARTESIAN_POINT('Ctrl Pts',(-30.9447247031331,-3.94398065776386,
135.599188497297));
#269650=CARTESIAN_POINT('Ctrl Pts',(-31.2231723269461,1.90220660919519,
136.714264833456));
#269651=CARTESIAN_POINT('Ctrl Pts',(-31.5016199507588,6.00035893026297,
132.398427910084));
#269652=CARTESIAN_POINT('Ctrl Pts',(-31.7800675745718,4.58447452824918,
126.617721019404));
#269653=CARTESIAN_POINT('Ctrl Pts',(-32.0585151983846,-1.04431800119413,
124.68433139072));
#269654=CARTESIAN_POINT('Ctrl Pts',(-32.3369628221976,-5.71343330531054,
128.374949641459));
#269655=CARTESIAN_POINT('Ctrl Pts',(-32.6154104460104,-5.1321825185805,
134.298077895915));
#269656=CARTESIAN_POINT('Ctrl Pts',(-32.8938580698234,0.165293281670594,
137.010650649146));
#269657=CARTESIAN_POINT('Ctrl Pts',(-33.1723056936362,5.31087263109202,
134.019946057479));
#269658=CARTESIAN_POINT('Ctrl Pts',(-33.4507533174492,5.57601948309184,
128.074275536613));
#269659=CARTESIAN_POINT('Ctrl Pts',(-33.729200941262,0.717076833825826,
124.637419833072));
#269660=CARTESIAN_POINT('Ctrl Pts',(-34.0076485650749,-4.80082439457541,
126.867681438675));
#269661=CARTESIAN_POINT('Ctrl Pts',(-34.2860961888878,-5.90700253767186,
132.715558892209));
#269662=CARTESIAN_POINT('Ctrl Pts',(-34.5645438127007,-1.58493392176466,
136.807138498572));
#269663=CARTESIAN_POINT('Ctrl Pts',(-34.8429914365135,4.19361153991761,
135.382458484293));
#269664=CARTESIAN_POINT('Ctrl Pts',(-35.1214390603265,6.11843286572883,
129.750730183006));
#269665=CARTESIAN_POINT('Ctrl Pts',(-35.3998866841394,2.42071328999757,
125.087236778371));
#269666=CARTESIAN_POINT('Ctrl Pts',(-35.6783343079523,-3.50152354082281,
125.677500884929));
#269667=CARTESIAN_POINT('Ctrl Pts',(-35.9567819317651,-6.20603129656164,
130.979098624759));
#269668=CARTESIAN_POINT('Ctrl Pts',(-36.2352295555781,-3.2074994722443,
136.120120672404));
#269669=CARTESIAN_POINT('Ctrl Pts',(-36.5136771793909,2.73856767200523,
136.376218918968));
#269670=CARTESIAN_POINT('Ctrl Pts',(-36.7921248032039,6.1680249121504,131.512051586954));
#269671=CARTESIAN_POINT('Ctrl Pts',(-37.0705724270167,3.92936858279784,
125.997550826698));
#269672=CARTESIAN_POINT('Ctrl Pts',(-37.3490200508296,-1.92018551381882,
124.900273438536));
#269673=CARTESIAN_POINT('Ctrl Pts',(-37.6274676746425,-6.00518292951342,
129.228563737208));
#269674=CARTESIAN_POINT('Ctrl Pts',(-37.9059152984554,-4.57171060248077,
135.004934386972));
#269675=CARTESIAN_POINT('Ctrl Pts',(-38.1843629222683,1.0629404277527,136.921182952087));
#269676=CARTESIAN_POINT('Ctrl Pts',(-38.4628105460811,5.72080113240803,
133.216370615161));
#269677=CARTESIAN_POINT('Ctrl Pts',(-38.7412581698941,5.12152507305273,
127.295038923683));
#269678=CARTESIAN_POINT('Ctrl Pts',(-39.0197057937069,-0.184182328028525,
124.598602428988));
#269679=CARTESIAN_POINT('Ctrl Pts',(-39.2981534175199,-5.32063516745863,
127.604954541453));
#269680=CARTESIAN_POINT('Ctrl Pts',(-39.5766010413327,-5.56768421547239,
133.55140453819));
#269681=CARTESIAN_POINT('Ctrl Pts',(-39.8550486651457,-0.698303465962086,
136.973455372429));
#269682=CARTESIAN_POINT('Ctrl Pts',(-40.1334962889585,4.81278405474664,
134.726409503982));
#269683=CARTESIAN_POINT('Ctrl Pts',(-40.4119439127715,5.90115814671511,
128.875192311658));
#269684=CARTESIAN_POINT('Ctrl Pts',(-40.6903915365843,1.56665618945481,
124.796786547352));
#269685=CARTESIAN_POINT('Ctrl Pts',(-40.9688391603973,-4.20752627050468,
126.239047867263));
#269686=CARTESIAN_POINT('Ctrl Pts',(-41.2472867842101,-6.11519763695597,
131.876608576776));
#269687=CARTESIAN_POINT('Ctrl Pts',(-41.5257344080229,-2.40330111905734,
136.528825793999));
#269688=CARTESIAN_POINT('Ctrl Pts',(-41.8041820318359,3.51711171946819,
135.920539169751));
#269689=CARTESIAN_POINT('Ctrl Pts',(-42.0826296556488,6.20547070826194,
130.610734395262));
#269690=CARTESIAN_POINT('Ctrl Pts',(-42.3610772794617,3.19130527026066,
125.478862659902));
#269691=CARTESIAN_POINT('Ctrl Pts',(-42.6395249032745,-2.75551380718057,
125.240863382598));
#269692=CARTESIAN_POINT('Ctrl Pts',(-42.9179725270875,-6.17015031015604,
130.115446272278));
#269693=CARTESIAN_POINT('Ctrl Pts',(-43.1964201509003,-3.91472010669807,
135.623107789941));
#269694=CARTESIAN_POINT('Ctrl Pts',(-43.4748677747133,1.93814663010615,
136.702576065077));
#269695=CARTESIAN_POINT('Ctrl Pts',(-43.7533153985261,6.00995129756958,
132.361872487794));
#269696=CARTESIAN_POINT('Ctrl Pts',(-44.031763022339,4.55890432500984,126.589891590455));
#269697=CARTESIAN_POINT('Ctrl Pts',(-44.3102106461518,-1.08155300737633,
124.690801840773));
#269698=CARTESIAN_POINT('Ctrl Pts',(-44.5886582699649,-5.72811596278534,
128.409773943013));
#269699=CARTESIAN_POINT('Ctrl Pts',(-44.8671058937777,-5.11082018241628,
134.329254217104));
#269700=CARTESIAN_POINT('Ctrl Pts',(-45.1455535175906,0.2030696681468,137.009529473845));
#269701=CARTESIAN_POINT('Ctrl Pts',(-45.4240011414034,5.33034841418793,
133.987557691017));
#269702=CARTESIAN_POINT('Ctrl Pts',(-45.7024487652165,5.55929736958694,
128.040383305508));
#269703=CARTESIAN_POINT('Ctrl Pts',(-45.9808963890292,0.679523629110432,
124.633169041983));
#269704=CARTESIAN_POINT('Ctrl Pts',(-46.2593440128422,-4.82469912994364,
126.896978356949));
#269705=CARTESIAN_POINT('Ctrl Pts',(-46.537791636655,-5.89525908823553,
132.751481083186));
#269706=CARTESIAN_POINT('Ctrl Pts',(-46.816239260468,-1.54836394385628,
136.816675223641));
#269707=CARTESIAN_POINT('Ctrl Pts',(-47.0946868842807,4.22140202314317,
135.35684595901));
#269708=CARTESIAN_POINT('Ctrl Pts',(-47.3731345080937,6.11190575782758,
129.713505066864));
#269709=CARTESIAN_POINT('Ctrl Pts',(-47.6515821319066,2.38586668426401,
125.072607134557));
#269710=CARTESIAN_POINT('Ctrl Pts',(-47.9300297557195,-3.53266731607082,
125.69891064141));
#269711=CARTESIAN_POINT('Ctrl Pts',(-48.2084773795324,-6.20485263332943,
131.016873261253));
#269712=CARTESIAN_POINT('Ctrl Pts',(-48.4869250033452,-3.17508150446096,
136.139547143367));
#269713=CARTESIAN_POINT('Ctrl Pts',(-48.7653726271582,2.77243441565242,
136.359445246621));
#269714=CARTESIAN_POINT('Ctrl Pts',(-49.043820250971,6.1722185487321,131.474491956744));
#269715=CARTESIAN_POINT('Ctrl Pts',(-49.322267874784,3.900035365166,125.973720703898));
#269716=CARTESIAN_POINT('Ctrl Pts',(-49.6007154985968,-1.95608979166789,
124.912071541833));
#269717=CARTESIAN_POINT('Ctrl Pts',(-49.8791631224098,-6.0146639902579,
129.265148186042));
#269718=CARTESIAN_POINT('Ctrl Pts',(-50.1576107462225,-4.54605581447205,
135.032685860113));
#269719=CARTESIAN_POINT('Ctrl Pts',(-50.4360583700356,1.10015556764067,
136.914599201455));
#269720=CARTESIAN_POINT('Ctrl Pts',(-50.7145059938484,5.73537772867887,
133.181501785951));
#269721=CARTESIAN_POINT('Ctrl Pts',(-50.9929536176612,5.10006794583985,
127.263927766504));
#269722=CARTESIAN_POINT('Ctrl Pts',(-51.2714012414742,-0.221955127055423,
124.599838577421));
#269723=CARTESIAN_POINT('Ctrl Pts',(-51.5498488652871,-5.34001228129766,
127.637402035479));
#269724=CARTESIAN_POINT('Ctrl Pts',(-51.8282964891,-5.5508590231301,133.585245715947));
#269725=CARTESIAN_POINT('Ctrl Pts',(-52.1067441129128,-0.660737497244709,
136.977591844792));
#269726=CARTESIAN_POINT('Ctrl Pts',(-52.3851917367258,4.8365695097872,134.697040054928));
#269727=CARTESIAN_POINT('Ctrl Pts',(-52.6636393605386,5.889305416881,128.83930603009));
#269728=CARTESIAN_POINT('Ctrl Pts',(-52.9420869843516,1.53005735442545,
124.78736117289));
#269729=CARTESIAN_POINT('Ctrl Pts',(-53.2205346081644,-4.23523866929,126.264744858582));
#269730=CARTESIAN_POINT('Ctrl Pts',(-53.4989822319774,-6.1085572588392,
131.913813654221));
#269731=CARTESIAN_POINT('Ctrl Pts',(-53.7774298557902,-2.36841014712749,
136.543349308967));
#269732=CARTESIAN_POINT('Ctrl Pts',(-54.0558774796031,3.54819018652628,
135.8990347215));
#269733=CARTESIAN_POINT('Ctrl Pts',(-54.334325103416,6.20417707748961,130.572963521183));
#269734=CARTESIAN_POINT('Ctrl Pts',(-54.6127727272289,3.15882832513996,
125.459534948064));
#269735=CARTESIAN_POINT('Ctrl Pts',(-54.8912203510417,-2.7893293406706,
125.257740055968));
#269736=CARTESIAN_POINT('Ctrl Pts',(-55.1696679748547,-6.17422960871856,
130.153018492501));
#269737=CARTESIAN_POINT('Ctrl Pts',(-55.4481155986676,-3.88531449423931,
135.646848522136));
#269738=CARTESIAN_POINT('Ctrl Pts',(-55.7265632224805,1.97401483228084,
136.690668736158));
#269739=CARTESIAN_POINT('Ctrl Pts',(-56.0050108462934,6.01932096392068,
132.32525935133));
#269740=CARTESIAN_POINT('Ctrl Pts',(-56.2834584701062,4.53316518989421,
126.562218330207));
#269741=CARTESIAN_POINT('Ctrl Pts',(-56.5619060939192,-1.11874793621411,
124.697498830995));
#269742=CARTESIAN_POINT('Ctrl Pts',(-56.840353717732,-5.74258636281662,
128.444686976857));
#269743=CARTESIAN_POINT('Ctrl Pts',(-57.118801341545,-5.08926846293066,
134.360299922064));
#269744=CARTESIAN_POINT('Ctrl Pts',(-57.3972489653578,0.240838529802063,
137.00817836373));
#269745=CARTESIAN_POINT('Ctrl Pts',(-57.6756965891708,5.34962667926312,
133.955051370017));
#269746=CARTESIAN_POINT('Ctrl Pts',(-57.9541442129836,5.54236925427356,
128.0065934946));
#269747=CARTESIAN_POINT('Ctrl Pts',(-58.2325918367966,0.641945244397073,
124.629146926667));
#269748=CARTESIAN_POINT('Ctrl Pts',(-58.5110394606094,-4.84839508431156,
126.92642006471));
#269749=CARTESIAN_POINT('Ctrl Pts',(-58.7894870844223,-5.88329718780563,
132.787331122898));
#269750=CARTESIAN_POINT('Ctrl Pts',(-59.0679347082352,-1.5117365907523,
136.825989160181));
#269751=CARTESIAN_POINT('Ctrl Pts',(-59.3463823320481,4.24903608076433,
135.331064739709));
#269752=CARTESIAN_POINT('Ctrl Pts',(-59.624829955861,6.10515217101086,129.676320372777));
#269753=CARTESIAN_POINT('Ctrl Pts',(-59.9032775796738,2.3509316693629,125.058189882977));
#269754=CARTESIAN_POINT('Ctrl Pts',(-60.1817252034868,-3.56368018703254,
125.720509582217));
#269755=CARTESIAN_POINT('Ctrl Pts',(-60.4601728272995,-6.20344404700091,
131.054640023013));
#269756=CARTESIAN_POINT('Ctrl Pts',(-60.7386204511126,-3.14254588286485,
136.158775917031));
#269757=CARTESIAN_POINT('Ctrl Pts',(-61.0170680749254,2.80619842572279,
136.342465728569));
#269758=CARTESIAN_POINT('Ctrl Pts',(-61.2955156987383,6.17618347148551,
131.436907494571));
#269759=CARTESIAN_POINT('Ctrl Pts',(-61.5739633225512,3.87055763028967,
125.950069582238));
#269760=CARTESIAN_POINT('Ctrl Pts',(-61.8524109463641,-1.9919215858902,
124.924087986069));
#269761=CARTESIAN_POINT('Ctrl Pts',(-62.130858570177,-6.02392217541635,
129.301789670958));
#269762=CARTESIAN_POINT('Ctrl Pts',(-62.4093061939898,-4.5202325706933,
135.060280651108));
#269763=CARTESIAN_POINT('Ctrl Pts',(-62.6877538178028,1.13732994085927,
136.907789033684));
#269764=CARTESIAN_POINT('Ctrl Pts',(-62.9662014416156,5.74974179841868,
133.146544870902));
#269765=CARTESIAN_POINT('Ctrl Pts',(-63.2446490654287,5.0784218337339,127.232947801366));
#269766=CARTESIAN_POINT('Ctrl Pts',(-63.5230966892413,-0.25971970145348,
124.601304636701));
#269767=CARTESIAN_POINT('Ctrl Pts',(-63.8015443130544,-5.3591915190178,
127.669966882319));
#269768=CARTESIAN_POINT('Ctrl Pts',(-64.0799919368672,-5.53382814166538,
133.618983846983));
#269769=CARTESIAN_POINT('Ctrl Pts',(-64.3584395606801,-0.623147044656387,
136.9814995658));
#269770=CARTESIAN_POINT('Ctrl Pts',(-64.636887184493,4.86017574396616,134.667526361205));
#269771=CARTESIAN_POINT('Ctrl Pts',(-64.9153348083059,5.8772344566688,128.803492564343));
#269772=CARTESIAN_POINT('Ctrl Pts',(-65.1937824321189,1.4934018225579,124.778158760555));
#269773=CARTESIAN_POINT('Ctrl Pts',(-65.4722300559316,-4.26279412974889,
126.290610067033));
#269774=CARTESIAN_POINT('Ctrl Pts',(-65.7506776797446,-6.10169052588679,
131.950977620477));
#269775=CARTESIAN_POINT('Ctrl Pts',(-66.0291253035574,-2.33343141288849,
136.5576601636));
#269776=CARTESIAN_POINT('Ctrl Pts',(-66.3075729273703,3.57913717409239,
135.877341488227));
#269777=CARTESIAN_POINT('Ctrl Pts',(-66.5860205511832,6.20265354865397,
130.535201221608));
#269778=CARTESIAN_POINT('Ctrl Pts',(-66.8644681749961,3.126234328474,125.440405290707));
#269779=CARTESIAN_POINT('Ctrl Pts',(-67.142915798809,-2.82304151453613,
125.274822261403));
#269780=CARTESIAN_POINT('Ctrl Pts',(-67.421363422622,-6.17808011893247,
130.190614848446));
#269781=CARTESIAN_POINT('Ctrl Pts',(-67.6998110464348,-3.85576491002292,
135.670409814162));
#269782=CARTESIAN_POINT('Ctrl Pts',(-67.9782586702478,2.00980988661012,
136.678543287925));
#269783=CARTESIAN_POINT('Ctrl Pts',(-68.2567062940606,6.02846758211988,
132.288589857404));
#269784=CARTESIAN_POINT('Ctrl Pts',(-68.5351539178734,4.50725807667536,
126.534702264101));
#269785=CARTESIAN_POINT('Ctrl Pts',(-68.8136015416864,-1.15590140943545,
124.704422113226));
#269786=CARTESIAN_POINT('Ctrl Pts',(-69.0920491654993,-5.75684396919829,
128.479687449276));
#269787=CARTESIAN_POINT('Ctrl Pts',(-69.3704967893121,-5.0675281587308,
134.391213860386));
#269788=CARTESIAN_POINT('Ctrl Pts',(-69.648944413125,0.278598467097045,
137.006597368867));
#269789=CARTESIAN_POINT('Ctrl Pts',(-69.9273920369379,5.36870671195437,
133.922428299012));
#269790=CARTESIAN_POINT('Ctrl Pts',(-70.2058396607509,5.52523576442926,
127.972907355982));
#269791=CARTESIAN_POINT('Ctrl Pts',(-70.4842872845636,0.604343072166899,
124.625353636165));
#269792=CARTESIAN_POINT('Ctrl Pts',(-70.7627349083767,-4.87191137961658,
126.956005470983));
#269793=CARTESIAN_POINT('Ctrl Pts',(-71.0411825321895,-5.87111727963483,
132.823107682909));
#269794=CARTESIAN_POINT('Ctrl Pts',(-71.3196301560023,-1.47505321969301,
136.835079963061));
#269795=CARTESIAN_POINT('Ctrl Pts',(-71.5980777798154,4.27651268879093,
135.305115781721));
#269796=CARTESIAN_POINT('Ctrl Pts',(-71.8765254036282,6.09817235553532,
129.639177478635));
#269797=CARTESIAN_POINT('Ctrl Pts',(-72.1549730274411,2.31590953982396,
125.043985557866));
#269798=CARTESIAN_POINT('Ctrl Pts',(-72.433420651254,-3.5945610045145,125.742296906994));
#269799=CARTESIAN_POINT('Ctrl Pts',(-72.7118682750669,-6.20180558977201,
131.092397510578));
#269800=CARTESIAN_POINT('Ctrl Pts',(-72.9903158988798,-3.109893813075,136.177806280867));
#269801=CARTESIAN_POINT('Ctrl Pts',(-73.2687635226926,2.8398584510789,136.325280993997));
#269802=CARTESIAN_POINT('Ctrl Pts',(-73.5472111465057,6.17991953348924,
131.399299593141));
#269803=CARTESIAN_POINT('Ctrl Pts',(-73.8256587703184,3.84093647047644,
125.926598338115));
#269804=CARTESIAN_POINT('Ctrl Pts',(-74.1041063941314,-2.02767956872624,
124.93632232597));
#269805=CARTESIAN_POINT('Ctrl Pts',(-74.3825540179442,-6.0329571419232,
129.338486834193));
#269806=CARTESIAN_POINT('Ctrl Pts',(-74.6610016417573,-4.49424182803428,
135.08771773742));
#269807=CARTESIAN_POINT('Ctrl Pts',(-74.9394492655699,1.17446216989917,
136.900752701129));
#269808=CARTESIAN_POINT('Ctrl Pts',(-75.217896889383,5.76389280936176,133.111501165354));
#269809=CARTESIAN_POINT('Ctrl Pts',(-75.4963445131958,5.05658753883907,
127.202100176243));
#269810=CARTESIAN_POINT('Ctrl Pts',(-75.7747921370087,-0.297474651842549,
124.603000552501));
#269811=CARTESIAN_POINT('Ctrl Pts',(-76.0532397608216,-5.37817216992523,
127.702647875272));
#269812=CARTESIAN_POINT('Ctrl Pts',(-76.3316873846344,-5.51659220216403,
133.65261768112));
#269813=CARTESIAN_POINT('Ctrl Pts',(-76.6101350084474,-0.585533501125347,
136.985178390654));
#269814=CARTESIAN_POINT('Ctrl Pts',(-76.8885826322602,4.8836018825454,134.637869516455));
#269815=CARTESIAN_POINT('Ctrl Pts',(-77.1670302560731,5.86494571337264,
128.767753241497));
#269816=CARTESIAN_POINT('Ctrl Pts',(-77.4454778798861,1.4566909521364,124.769179651345));
#269817=CARTESIAN_POINT('Ctrl Pts',(-77.7239255036988,-4.29019163080361,
126.316642534169));
#269818=CARTESIAN_POINT('Ctrl Pts',(-78.0023731275119,-6.09459769254796,
131.988099098418));
#269819=CARTESIAN_POINT('Ctrl Pts',(-78.2808207513247,-2.29836621249045,
136.571757827603));
#269820=CARTESIAN_POINT('Ctrl Pts',(-78.5592683751376,3.60995153541429,
135.855460273781));
#269821=CARTESIAN_POINT('Ctrl Pts',(-78.8377159989505,6.20090017820995,
130.497448895834));
#269822=CARTESIAN_POINT('Ctrl Pts',(-79.1161636227633,3.09352448804556,
125.421474396687));
#269823=CARTESIAN_POINT('Ctrl Pts',(-79.3946112465763,-2.85664907955992,
125.292109365916));
#269824=CARTESIAN_POINT('Ctrl Pts',(-79.6730588703891,-6.18170169811556,
130.228233946967));
#269825=CARTESIAN_POINT('Ctrl Pts',(-79.9515064942021,-3.8260724490201,
135.693790792945));
#269826=CARTESIAN_POINT('Ctrl Pts',(-80.2299541180149,2.04553046669522,
136.666200169693));
#269827=CARTESIAN_POINT('Ctrl Pts',(-80.5084017418279,6.03739081323573,
132.251865364817));
#269828=CARTESIAN_POINT('Ctrl Pts',(-80.7868493656406,4.48118394535095,
126.507344411756));
#269829=CARTESIAN_POINT('Ctrl Pts',(-81.0652969894537,-1.19301205030527,
124.711571430921));
#269830=CARTESIAN_POINT('Ctrl Pts',(-81.3437446132665,-5.77088825360962,
128.514774063314));
#269831=CARTESIAN_POINT('Ctrl Pts',(-81.6221922370794,-5.04560007541116,
134.421994886542));
#269832=CARTESIAN_POINT('Ctrl Pts',(-81.9006398608923,0.316348080823153,
137.00478654784));
#269833=CARTESIAN_POINT('Ctrl Pts',(-82.179087484705,5.38758780524389,133.889689686862));
#269834=CARTESIAN_POINT('Ctrl Pts',(-82.4575351085182,5.50789753494193,
127.939326137905));
#269835=CARTESIAN_POINT('Ctrl Pts',(-82.7359827323308,0.566718505781886,
124.621789311041));
#269836=CARTESIAN_POINT('Ctrl Pts',(-83.0144303561439,-4.89524714445407,
126.985733479472));
#269837=CARTESIAN_POINT('Ctrl Pts',(-83.2928779799568,-5.858719815054,132.858809437506));
#269838=CARTESIAN_POINT('Ctrl Pts',(-83.5713256037696,-1.43831518999427,
136.843947295418));
#269839=CARTESIAN_POINT('Ctrl Pts',(-83.8497732275826,4.30383082906709,
135.279000046597));
#269840=CARTESIAN_POINT('Ctrl Pts',(-84.1282208513953,6.09096657004034,
129.602077760783));
#269841=CARTESIAN_POINT('Ctrl Pts',(-84.4066684752085,2.28080159340614,
125.029994685571));
#269842=CARTESIAN_POINT('Ctrl Pts',(-84.685116099021,-3.6253086242162,125.764271808403));
#269843=CARTESIAN_POINT('Ctrl Pts',(-84.9635637228342,-6.19993732235617,
131.130144324829));
#269844=CARTESIAN_POINT('Ctrl Pts',(-85.242011346647,-3.07712650502686,
136.196637529698));
#269845=CARTESIAN_POINT('Ctrl Pts',(-85.5204589704598,2.87341324443482,
136.307891679689));
#269846=CARTESIAN_POINT('Ctrl Pts',(-85.7989065942728,6.18342659630218,
131.361669646028));
#269847=CARTESIAN_POINT('Ctrl Pts',(-86.0773542180856,3.81117298335027,
125.903307841269));
#269848=CARTESIAN_POINT('Ctrl Pts',(-86.3558018418987,-2.06336241514917,
124.948774108188));
#269849=CARTESIAN_POINT('Ctrl Pts',(-86.6342494657113,-6.04176855498474,
129.375238315919));
#269850=CARTESIAN_POINT('Ctrl Pts',(-86.9126970895244,-4.46808454959173,
135.114996102359));
#269851=CARTESIAN_POINT('Ctrl Pts',(-87.1911447133372,1.2115508788106,136.893490464523));
#269852=CARTESIAN_POINT('Ctrl Pts',(-87.4695923371502,5.77783023713722,
133.076371967865));
#269853=CARTESIAN_POINT('Ctrl Pts',(-87.7480399609628,5.03456587023344,
127.171386034204));
#269854=CARTESIAN_POINT('Ctrl Pts',(-88.026487584776,-0.33521857919891,
124.60492626198));
#269855=CARTESIAN_POINT('Ctrl Pts',(-88.3049352085887,-5.39695353068522,
127.735443803332));
#269856=CARTESIAN_POINT('Ctrl Pts',(-88.5833828324018,-5.49915184330967,
133.686145972045));
#269857=CARTESIAN_POINT('Ctrl Pts',(-88.8618304562145,-0.547898260434929,
136.988628183031));
#269858=CARTESIAN_POINT('Ctrl Pts',(-89.1402780800275,4.90684705746115,
134.608070619623));
#269859=CARTESIAN_POINT('Ctrl Pts',(-89.4187257038403,5.85243964235601,
128.732089385887));
#269860=CARTESIAN_POINT('Ctrl Pts',(-89.6971733276532,1.41992610349655,
124.760424177987));
#269861=CARTESIAN_POINT('Ctrl Pts',(-89.9756209514662,-4.31743015722937,
126.342841295349));
#269862=CARTESIAN_POINT('Ctrl Pts',(-90.254068575279,-6.08727902165076,
132.025176712493));
#269863=CARTESIAN_POINT('Ctrl Pts',(-90.5325161990919,-2.26321584528708,
136.585641778581));
#269864=CARTESIAN_POINT('Ctrl Pts',(-90.8109638229048,3.64063212865448,
135.833391888981));
#269865=CARTESIAN_POINT('Ctrl Pts',(-91.0894114467178,6.19891703112955,
130.459707942787));
#269866=CARTESIAN_POINT('Ctrl Pts',(-91.3678590705306,3.06070001592934,
125.402742967496));
#269867=CARTESIAN_POINT('Ctrl Pts',(-91.6463066943433,-2.89015079040179,
125.309600728926));
#269868=CARTESIAN_POINT('Ctrl Pts',(-91.9247543181566,-6.18509421206894,
130.265874394073));
#269869=CARTESIAN_POINT('Ctrl Pts',(-92.2032019419691,-3.79623821149537,
135.716990592095));
#269870=CARTESIAN_POINT('Ctrl Pts',(-92.4816495657822,2.08117524889636,
136.653639838841));
#269871=CARTESIAN_POINT('Ctrl Pts',(-92.7600971895951,6.04609032661485,
132.21508723441));
#269872=CARTESIAN_POINT('Ctrl Pts',(-93.0385448134079,4.45494376210749,
126.480145786926));
#269873=CARTESIAN_POINT('Ctrl Pts',(-93.3169924372209,-1.23007848367479,
124.718946519161));
#269874=CARTESIAN_POINT('Ctrl Pts',(-93.5954400610337,-5.78471869563455,
128.549945518824));
#269875=CARTESIAN_POINT('Ctrl Pts',(-93.8738876848466,-5.02348502552524,
134.45264185993));
#269876=CARTESIAN_POINT('Ctrl Pts',(-94.1523353086595,0.354085972155003,
137.002745967751));
#269877=CARTESIAN_POINT('Ctrl Pts',(-94.4307829324724,5.40626925948619,
133.85683674671));
#269878=CARTESIAN_POINT('Ctrl Pts',(-94.7092305562852,5.49035520828578,
127.905851084735));
#269879=CARTESIAN_POINT('Ctrl Pts',(-94.9876781800983,0.529072939433998,
124.618454083368));
#269880=CARTESIAN_POINT('Ctrl Pts',(-95.2661258039109,-4.91840151410816,
127.015602988595));
#269881=CARTESIAN_POINT('Ctrl Pts',(-95.5445734277241,-5.84610525345601,
132.894435063746));
#269882=CARTESIAN_POINT('Ctrl Pts',(-95.8230210515366,-1.40152386299717,
136.85259082867));
#269883=CARTESIAN_POINT('Ctrl Pts',(-96.10146867535,4.33098948930923,135.252718502061));
#269884=CARTESIAN_POINT('Ctrl Pts',(-96.3799162991623,6.08353508153927,
129.565022593965));
#269885=CARTESIAN_POINT('Ctrl Pts',(-96.6583639229758,2.245609131046,125.01621778453));
#269886=CARTESIAN_POINT('Ctrl Pts',(-96.9368115467883,-3.65592190677386,
125.786433472156));
#269887=CARTESIAN_POINT('Ctrl Pts',(-97.2152591706015,-6.19783931398261,
131.167879067045));
#269888=CARTESIAN_POINT('Ctrl Pts',(-97.493706794414,-3.04424517292474,
136.215268965725));
#269889=CARTESIAN_POINT('Ctrl Pts',(-97.7721544182274,2.90686156240656,
136.290298430015));
#269890=CARTESIAN_POINT('Ctrl Pts',(-98.0506020420397,6.18670452996842,
131.324019047625));
#269891=CARTESIAN_POINT('Ctrl Pts',(-98.3290496658531,3.78126827180747,
125.880198954735));
#269892=CARTESIAN_POINT('Ctrl Pts',(-98.6074972896656,-2.09896880291958,
124.961442871316));
#269893=CARTESIAN_POINT('Ctrl Pts',(-98.8859449134787,-6.05035608809047,
129.412042754299));
#269894=CARTESIAN_POINT('Ctrl Pts',(-99.1643925372916,-4.44176170463296,
135.142114735114));
#269895=CARTESIAN_POINT('Ctrl Pts',(-99.4428401611044,1.24859469325925,
136.886002592972));
#269896=CARTESIAN_POINT('Ctrl Pts',(-99.7212877849174,5.79155356528836,
133.041158580159));
#269897=CARTESIAN_POINT('Ctrl Pts',(-99.9997354087301,5.01235764393804,
127.140806513377));
#269898=CARTESIAN_POINT('Ctrl Pts',(-100.278183032543,-0.37295008490757,
124.607081693777));
#269899=CARTESIAN_POINT('Ctrl Pts',(-100.556630656356,-5.41553490534739,
127.768353451233));
#269900=CARTESIAN_POINT('Ctrl Pts',(-100.835078280169,-5.48150771136145,
133.719567477352));
#269901=CARTESIAN_POINT('Ctrl Pts',(-101.113525903981,-0.510242717172956,
136.9918488151));
#269902=CARTESIAN_POINT('Ctrl Pts',(-101.391973527794,4.92991040735466,
134.578130774917));
#269903=CARTESIAN_POINT('Ctrl Pts',(-101.670421151607,5.83971670703623,
128.696502319049));
#269904=CARTESIAN_POINT('Ctrl Pts',(-101.94886877542,1.38310863897239,124.751892664915));
#269905=CARTESIAN_POINT('Ctrl Pts',(-102.227316399233,-4.34450869969331,
126.36920537977));
#269906=CARTESIAN_POINT('Ctrl Pts',(-102.505764023046,-6.07973478439049,
132.062209088779));
#269907=CARTESIAN_POINT('Ctrl Pts',(-102.784211646859,-2.22798161378826,
136.599311502058));
#269908=CARTESIAN_POINT('Ctrl Pts',(-103.062659270672,3.6711778169323,135.811137151577));
#269909=CARTESIAN_POINT('Ctrl Pts',(-103.341106894485,6.19670418089893,
130.42197976097));
#269910=CARTESIAN_POINT('Ctrl Pts',(-103.619554518298,3.02776212844844,
125.384211697232));
#269911=CARTESIAN_POINT('Ctrl Pts',(-103.89800214211,-2.92354540564323,
125.327295702285));
#269912=CARTESIAN_POINT('Ctrl Pts',(-104.176449765923,-6.18825753508174,
130.303534794984));
#269913=CARTESIAN_POINT('Ctrl Pts',(-104.454897389736,-3.76626330296762,
135.740008351935));
#269914=CARTESIAN_POINT('Ctrl Pts',(-104.733345013549,2.1167429123828,136.640862760796));
#269915=CARTESIAN_POINT('Ctrl Pts',(-105.011792637362,6.05456579989334,
132.17825682901));
#269916=CARTESIAN_POINT('Ctrl Pts',(-105.290240261175,4.42853849928509,
126.453107397468));
#269917=CARTESIAN_POINT('Ctrl Pts',(-105.568687884988,-1.26709933603374,
124.726547104658));
#269918=CARTESIAN_POINT('Ctrl Pts',(-105.847135508801,-5.79833478278087,
128.585200512514));
#269919=CARTESIAN_POINT('Ctrl Pts',(-106.125583132613,-5.00118382855433,
134.483153644914));
#269920=CARTESIAN_POINT('Ctrl Pts',(-106.404030756427,0.391810742700936,
137.000475704212));
#269921=CARTESIAN_POINT('Ctrl Pts',(-106.682478380239,5.42475038243292,
133.823870695931));
#269922=CARTESIAN_POINT('Ctrl Pts',(-106.960926004052,5.47260943449832,
127.872483436902));
#269923=CARTESIAN_POINT('Ctrl Pts',(-107.239373627865,0.491407768093767,
124.615348076738));
#269924=CARTESIAN_POINT('Ctrl Pts',(-107.517821251678,-4.94137363058539,
127.045612891524));
#269925=CARTESIAN_POINT('Ctrl Pts',(-107.796268875491,-5.83327406227795,
132.929983241508));
#269926=CARTESIAN_POINT('Ctrl Pts',(-108.074716499304,-1.36468060201792,
136.861010242526));
#269927=CARTESIAN_POINT('Ctrl Pts',(-108.353164123117,4.3579876631431,135.22627212199));
#269928=CARTESIAN_POINT('Ctrl Pts',(-108.631611746929,6.07587816540856,
129.528013351273));
#269929=CARTESIAN_POINT('Ctrl Pts',(-108.910059370743,2.21033345681367,
125.00265536525));
#269930=CARTESIAN_POINT('Ctrl Pts',(-109.188506994555,-3.68639971780079,
125.808781077045));
#269931=CARTESIAN_POINT('Ctrl Pts',(-109.466954618368,-6.19551164239422,
131.205600338952));
#269932=CARTESIAN_POINT('Ctrl Pts',(-109.745402242181,-3.01125103519769,
136.233699898554));
#269933=CARTESIAN_POINT('Ctrl Pts',(-110.023849865994,2.94020216555433,
136.272501896897));
#269934=CARTESIAN_POINT('Ctrl Pts',(-110.302297489807,6.18975321302316,
131.286349193086));
#269935=CARTESIAN_POINT('Ctrl Pts',(-110.58074511362,3.75122344397827,125.857272534824));
#269936=CARTESIAN_POINT('Ctrl Pts',(-110.859192737433,-2.13449741262907,
124.974328145912));
#269937=CARTESIAN_POINT('Ctrl Pts',(-111.137640361246,-6.05871942302636,
129.44889878553));
#269938=CARTESIAN_POINT('Ctrl Pts',(-111.416087985058,-4.41527426856075,
135.169072630797));
#269939=CARTESIAN_POINT('Ctrl Pts',(-111.694535608871,1.28559224057236,
136.878289363941));
#269940=CARTESIAN_POINT('Ctrl Pts',(-111.972983232684,5.8050622852923,133.005862307081));
#269941=CARTESIAN_POINT('Ctrl Pts',(-112.251430856497,4.9899636828869,127.110362746893));
#269942=CARTESIAN_POINT('Ctrl Pts',(-112.52987848031,-0.410667770813077,
124.609466768025));
#269943=CARTESIAN_POINT('Ctrl Pts',(-112.808326104123,-5.43391560537209,
127.801375599495));
#269944=CARTESIAN_POINT('Ctrl Pts',(-113.086773727936,-5.46366046012913,
133.752880958598));
#269945=CARTESIAN_POINT('Ctrl Pts',(-113.365221351749,-0.472568266679477,
136.994840167519));
#269946=CARTESIAN_POINT('Ctrl Pts',(-113.643668975562,4.95279107760506,
134.548051091771));
#269947=CARTESIAN_POINT('Ctrl Pts',(-113.922116599375,5.8267773788663,128.660993359675));
#269948=CARTESIAN_POINT('Ctrl Pts',(-114.200564223187,1.34623992284899,
124.74358542827));
#269949=CARTESIAN_POINT('Ctrl Pts',(-114.479011847001,-4.37142625478972,
126.395733810498));
#269950=CARTESIAN_POINT('Ctrl Pts',(-114.757459470813,-6.07196526032194,
132.099194855029));
#269951=CARTESIAN_POINT('Ctrl Pts',(-115.035907094626,-2.19266482361144,
136.612766491501));
#269952=CARTESIAN_POINT('Ctrl Pts',(-115.314354718439,3.70158746836604,
135.788696886227));
#269953=CARTESIAN_POINT('Ctrl Pts',(-115.592802342252,6.19426170951602,
130.384265748418));
#269954=CARTESIAN_POINT('Ctrl Pts',(-115.871249966065,2.99471204612843,
125.36588127258));
#269955=CARTESIAN_POINT('Ctrl Pts',(-116.149697589878,-2.95683168783455,
125.345193630298));
#269956=CARTESIAN_POINT('Ctrl Pts',(-116.428145213691,-6.19119154993583,
130.34121375418));
#269957=CARTESIAN_POINT('Ctrl Pts',(-116.706592837503,-3.73614883416816,
135.762843219532));
#269958=CARTESIAN_POINT('Ctrl Pts',(-116.985040461316,2.1522321391827,136.627869409019));
#269959=CARTESIAN_POINT('Ctrl Pts',(-117.263488085129,6.06281691900968,
132.14137551338));
#269960=CARTESIAN_POINT('Ctrl Pts',(-117.541935708942,4.40196913533955,
126.426230245297));
#269961=CARTESIAN_POINT('Ctrl Pts',(-117.820383332755,-1.30407323556081,
124.73437290577));
#269962=CARTESIAN_POINT('Ctrl Pts',(-118.098830956568,-5.81173601049948,
128.620537737998));
#269963=CARTESIAN_POINT('Ctrl Pts',(-118.377278580381,-4.97869731087745,
134.51352911087));
#269964=CARTESIAN_POINT('Ctrl Pts',(-118.655726204194,0.429520994555717,
136.997975841351));
#269965=CARTESIAN_POINT('Ctrl Pts',(-118.934173828006,5.44303048925927,
133.790792756097));
#269966=CARTESIAN_POINT('Ctrl Pts',(-119.21262145182,5.45466087115571,127.839224430854));
#269967=CARTESIAN_POINT('Ctrl Pts',(-119.491069075632,0.453724387457947,
124.612471406243));
#269968=CARTESIAN_POINT('Ctrl Pts',(-119.769516699445,-4.96416264264509,
127.075762076232));
#269969=CARTESIAN_POINT('Ctrl Pts',(-120.047964323258,-5.82022671698453,
132.965452653541));
#269970=CARTESIAN_POINT('Ctrl Pts',(-120.326411947071,-1.32778677229758,
136.869205225004));
#269971=CARTESIAN_POINT('Ctrl Pts',(-120.604859570884,4.38482435014149,
135.199661886361));
#269972=CARTESIAN_POINT('Ctrl Pts',(-120.883307194697,6.06799610537801,
129.491051404098));
#269973=CARTESIAN_POINT('Ctrl Pts',(-121.16175481851,2.17497587786225,124.989307930291));
#269974=CARTESIAN_POINT('Ctrl Pts',(-121.440202442323,-3.71674092793051,
125.831313794972));
#269975=CARTESIAN_POINT('Ctrl Pts',(-121.718650066136,-6.19295439384353,
131.243306742772));
#269976=CARTESIAN_POINT('Ctrl Pts',(-121.997097689948,-2.97814531445616,
136.251929645219));
#269977=CARTESIAN_POINT('Ctrl Pts',(-122.275545313761,2.97343381842962,
136.254502739794));
#269978=CARTESIAN_POINT('Ctrl Pts',(-122.553992937574,6.19257253249627,
131.248661478285));
#269979=CARTESIAN_POINT('Ctrl Pts',(-122.832440561387,3.72103961318487,
125.83452943108));
#269980=CARTESIAN_POINT('Ctrl Pts',(-123.1108881852,-2.16994692775201,124.987429454503));
#269981=CARTESIAN_POINT('Ctrl Pts',(-123.389335809013,-6.06685824988591,
129.485805043896));
#269982=CARTESIAN_POINT('Ctrl Pts',(-123.667783432826,-4.38862322287681,
135.19586879047));
#269983=CARTESIAN_POINT('Ctrl Pts',(-123.946231056639,1.32254214979223,
136.870351063246));
#269984=CARTESIAN_POINT('Ctrl Pts',(-124.224678680451,5.81835589657845,
132.97048445655));
#269985=CARTESIAN_POINT('Ctrl Pts',(-124.503126304264,4.96738481689638,
127.080055862859));
#269986=CARTESIAN_POINT('Ctrl Pts',(-124.781573928077,-0.448370239273912,
124.612081396343));
#269987=CARTESIAN_POINT('Ctrl Pts',(-125.06002155189,-5.4520949496557,127.834509024472));
#269988=CARTESIAN_POINT('Ctrl Pts',(-125.338469175703,-5.44561075094924,
133.786085181339));
#269989=CARTESIAN_POINT('Ctrl Pts',(-125.616916799516,-0.434876304995071,
136.997602129441));
#269990=CARTESIAN_POINT('Ctrl Pts',(-125.895364423329,4.97548822036069,
134.517832684797));
#269991=CARTESIAN_POINT('Ctrl Pts',(-126.173812047142,5.8136221373178,128.625563823564));
#269992=CARTESIAN_POINT('Ctrl Pts',(-126.452259670955,1.30932132131015,
124.735502775877));
#269993=CARTESIAN_POINT('Ctrl Pts',(-126.730707294768,-4.39818182507867,
126.422425604514));
#269994=CARTESIAN_POINT('Ctrl Pts',(-127.00915491858,-6.0639707373477,132.136132640718));
#269995=CARTESIAN_POINT('Ctrl Pts',(-127.287602542393,-2.15726678343353,
136.626006248326));
#269996=CARTESIAN_POINT('Ctrl Pts',(-127.566050166206,3.73185995611441,
135.766071924465));
#269997=CARTESIAN_POINT('Ctrl Pts',(-127.844497790019,6.19158970748781,
130.346567302635));
#269998=CARTESIAN_POINT('Ctrl Pts',(-128.122945413832,2.96155099365221,
125.34775237278));
#269999=CARTESIAN_POINT('Ctrl Pts',(-128.401393037645,-2.99000840354028,
125.363293849751));
#270000=CARTESIAN_POINT('Ctrl Pts',(-128.679840661458,-6.19389614791022,
130.378909875453));
#270001=CARTESIAN_POINT('Ctrl Pts',(-128.958288285271,-3.70589592099968,
135.785494348734));
#270002=CARTESIAN_POINT('Ctrl Pts',(-129.236735909083,2.18764161422919,
136.614660264981));
#270003=CARTESIAN_POINT('Ctrl Pts',(-129.515183532897,6.07084337821547,
132.104444654172));
#270004=CARTESIAN_POINT('Ctrl Pts',(-129.793631156709,4.37523665480886,
126.399515326358));
#270005=CARTESIAN_POINT('Ctrl Pts',(-130.072078780522,-1.34099881217456,
124.742423632508));
#270006=CARTESIAN_POINT('Ctrl Pts',(-130.350526404335,-5.82492188220296,
128.655955885842));
#270007=CARTESIAN_POINT('Ctrl Pts',(-130.628974028148,-4.95602630574081,
134.543767132223));
#270008=CARTESIAN_POINT('Ctrl Pts',(-130.907421651961,0.467215330352083,
136.995246471799));
#270009=CARTESIAN_POINT('Ctrl Pts',(-131.185869275774,5.46110890258918,
133.757604152921));
#270010=CARTESIAN_POINT('Ctrl Pts',(-131.464316899587,5.43651018334856,
127.80607529902));
#270011=CARTESIAN_POINT('Ctrl Pts',(-131.742764523399,0.416024193898128,
124.60982417848));
#270012=CARTESIAN_POINT('Ctrl Pts',(-132.021212147213,-4.98676770583297,
127.106049425532));
#270013=CARTESIAN_POINT('Ctrl Pts',(-132.299659771025,-5.80696370104951,
133.000841985516));
#270014=CARTESIAN_POINT('Ctrl Pts',(-132.578107394838,-1.2908437409496,
136.877175472434));
#270015=CARTESIAN_POINT('Ctrl Pts',(-132.856555018651,4.41149855586104,
135.172888781227));
#270016=CARTESIAN_POINT('Ctrl Pts',(-133.135002642464,6.05988919352027,
129.454138122079));
#270017=CARTESIAN_POINT('Ctrl Pts',(-133.413450266277,2.13953770437982,
124.976175974248));
#270018=CARTESIAN_POINT('Ctrl Pts',(-133.69189789009,-3.74694441285829,
125.854030790976));
#270019=CARTESIAN_POINT('Ctrl Pts',(-133.970345513903,-6.19016766309031,
131.280996881284));
#270020=CARTESIAN_POINT('Ctrl Pts',(-134.248793137716,-2.94492923744478,
136.269957530209));
#270021=CARTESIAN_POINT('Ctrl Pts',(-134.527240761528,3.00655528962129,
136.236301625668));
#270022=CARTESIAN_POINT('Ctrl Pts',(-134.805688385342,6.19516238391663,
131.210957299752));
#270023=CARTESIAN_POINT('Ctrl Pts',(-135.084136009154,3.69071789790064,
125.811970486258));
#270024=CARTESIAN_POINT('Ctrl Pts',(-135.362583632967,-2.2053160346932,
125.000746311619));
#270025=CARTESIAN_POINT('Ctrl Pts',(-135.64103125678,-6.07477226708194,
129.522760161825));
#270026=CARTESIAN_POINT('Ctrl Pts',(-135.919478880593,-4.36180955514542,
135.222502221193));
#270027=CARTESIAN_POINT('Ctrl Pts',(-136.197926504406,1.35944305172635,
136.862187985044));
#270028=CARTESIAN_POINT('Ctrl Pts',(-136.476374128219,5.83143390654715,
132.935026339502));
#270029=CARTESIAN_POINT('Ctrl Pts',(-136.754821752032,4.9446218826347,127.049886984307));
#270030=CARTESIAN_POINT('Ctrl Pts',(-137.033269375845,-0.486056093210629,
124.614925481843));
#270031=CARTESIAN_POINT('Ctrl Pts',(-137.311716999657,-5.47007226455594,
127.867752498391));
#270032=CARTESIAN_POINT('Ctrl Pts',(-137.59016462347,-5.42735925266033,
133.819178915179));
#270033=CARTESIAN_POINT('Ctrl Pts',(-137.868612247283,-0.397168228809268,
137.000134598521));
#270034=CARTESIAN_POINT('Ctrl Pts',(-138.147059871096,4.99800099457058,
134.487476673751));
#270035=CARTESIAN_POINT('Ctrl Pts',(-138.425507494909,5.80025146986304,
128.590215023569));
#270036=CARTESIAN_POINT('Ctrl Pts',(-138.703955118722,1.27235420238826,
124.727645007244));
#270037=CARTESIAN_POINT('Ctrl Pts',(-138.982402742535,-4.42477441912264,
126.449279772744));
#270038=CARTESIAN_POINT('Ctrl Pts',(-139.260850366348,-6.05575151170779,
132.173021077107));
#270039=CARTESIAN_POINT('Ctrl Pts',(-139.539297990161,-2.12178880494131,
136.639030281933));
#270040=CARTESIAN_POINT('Ctrl Pts',(-139.817745613973,3.76199415842019,
135.743263104665));
#270041=CARTESIAN_POINT('Ctrl Pts',(-140.096193237787,6.18868827382574,
130.308885820552));
#270042=CARTESIAN_POINT('Ctrl Pts',(-140.374640861599,2.92828019981485,
125.329825669606));
#270043=CARTESIAN_POINT('Ctrl Pts',(-140.653088485412,-3.02307432338508,
125.381595689934));
#270044=CARTESIAN_POINT('Ctrl Pts',(-140.931536109225,-6.19637122878504,
130.416621761961));
#270045=CARTESIAN_POINT('Ctrl Pts',(-141.209983733038,-3.675505684495,135.807960900193));
#270046=CARTESIAN_POINT('Ctrl Pts',(-141.488431356851,2.22297002541115,
136.601235818153));
#270047=CARTESIAN_POINT('Ctrl Pts',(-141.766878980664,6.07864488008735,
132.06746561987));
#270048=CARTESIAN_POINT('Ctrl Pts',(-142.045326604476,4.34834204827492,
126.372963630579));
#270049=CARTESIAN_POINT('Ctrl Pts',(-142.32377422829,-1.3778746975837,124.750698986551));
#270050=CARTESIAN_POINT('Ctrl Pts',(-142.602221852102,-5.83789190928377,
128.691453643612));
#270051=CARTESIAN_POINT('Ctrl Pts',(-142.880669475915,-4.93317165322728,
134.573866588494));
#270052=CARTESIAN_POINT('Ctrl Pts',(-143.159117099728,0.504892353312588,
136.992287696695));
#270053=CARTESIAN_POINT('Ctrl Pts',(-143.437564723541,5.47898495252035,
133.72430611622));
#270054=CARTESIAN_POINT('Ctrl Pts',(-143.716012347354,5.4181580436573,127.77303726975));
#270055=CARTESIAN_POINT('Ctrl Pts',(-143.994459971167,0.378308584408798,
124.607406491544));
#270056=CARTESIAN_POINT('Ctrl Pts',(-144.27290759498,-5.00918798250961,
127.136473817112));
#270057=CARTESIAN_POINT('Ctrl Pts',(-144.551355218793,-5.79348550593904,
133.036149926065));
#270058=CARTESIAN_POINT('Ctrl Pts',(-144.829802842605,-1.2538528769121,
136.884920689477));
#270059=CARTESIAN_POINT('Ctrl Pts',(-145.108250466418,4.43800929187927,
135.145953798675));
#270060=CARTESIAN_POINT('Ctrl Pts',(-145.386698090231,6.05155773023994,
129.417274873051));
#270061=CARTESIAN_POINT('Ctrl Pts',(-145.665145714044,2.10402024954095,
124.963259983731));
#270062=CARTESIAN_POINT('Ctrl Pts',(-145.943593337857,-3.77700905338292,
125.876931223274));
#270063=CARTESIAN_POINT('Ctrl Pts',(-146.22204096167,-6.18715155339789,
131.318669357863));
#270064=CARTESIAN_POINT('Ctrl Pts',(-146.500488585483,-2.9116040349975,
136.287782885497));
#270065=CARTESIAN_POINT('Ctrl Pts',(-146.778936209295,3.03956535180104,
136.217899228972));
#270066=CARTESIAN_POINT('Ctrl Pts',(-147.057383833109,6.19752267131684,
131.173238054629));
#270067=CARTESIAN_POINT('Ctrl Pts',(-147.335831456921,3.66025942170698,
125.789596536289));
#270068=CARTESIAN_POINT('Ctrl Pts',(-147.614279080735,-2.24060342283806,
125.014278223797));
#270069=CARTESIAN_POINT('Ctrl Pts',(-147.892726704547,-6.08246118135759,
129.559762769929));
#270070=CARTESIAN_POINT('Ctrl Pts',(-148.17117432836,-4.33483425895693,
135.248971936054));
#270071=CARTESIAN_POINT('Ctrl Pts',(-148.449621952173,1.39629357899829,
136.853800431821));
#270072=CARTESIAN_POINT('Ctrl Pts',(-148.728069575986,5.84429583058792,
132.899489269852));
#270073=CARTESIAN_POINT('Ctrl Pts',(-149.006517199799,4.9216757235908,127.019857229157));
#270074=CARTESIAN_POINT('Ctrl Pts',(-149.284964823612,-0.52372393616008,
124.617998919139));
#270075=CARTESIAN_POINT('Ctrl Pts',(-149.563412447425,-5.48784688391679,
127.901104789406));
#270076=CARTESIAN_POINT('Ctrl Pts',(-149.841860071237,-5.40890664157841,
133.852160933818));
#270077=CARTESIAN_POINT('Ctrl Pts',(-150.12030769505,-0.359445435409253,
137.002437480918));
#270078=CARTESIAN_POINT('Ctrl Pts',(-150.398755318863,5.02032856601553,
134.456984183485));
#270079=CARTESIAN_POINT('Ctrl Pts',(-150.677202942676,5.78666587195703,
128.554948269553));
#270080=CARTESIAN_POINT('Ctrl Pts',(-150.955650566489,1.23533993591347,
124.720012413542));
#270081=CARTESIAN_POINT('Ctrl Pts',(-151.234098190302,-4.45120305152329,
126.476295320094));
#270082=CARTESIAN_POINT('Ctrl Pts',(-151.512545814115,-6.0473078879686,
132.209858797279));
#270083=CARTESIAN_POINT('Ctrl Pts',(-151.790993437928,-2.08623220278462,
136.651838109709));
#270084=CARTESIAN_POINT('Ctrl Pts',(-152.069441061741,3.79198895864895,
135.720271272016));
#270085=CARTESIAN_POINT('Ctrl Pts',(-152.347888685554,6.18555751604382,
130.27122269847));
#270086=CARTESIAN_POINT('Ctrl Pts',(-152.626336309366,2.89490089747778,
125.312101827337));
#270087=CARTESIAN_POINT('Ctrl Pts',(-152.904783933179,-3.05602822209906,
125.400098472666));
#270088=CARTESIAN_POINT('Ctrl Pts',(-153.183231556992,-6.19861670084527,
130.454348016274));
#270089=CARTESIAN_POINT('Ctrl Pts',(-153.461679180805,-3.64497925077551,
135.830242041403));
#270090=CARTESIAN_POINT('Ctrl Pts',(-153.740126804618,2.25821606362131,
136.587596565983));
#270091=CARTESIAN_POINT('Ctrl Pts',(-154.018574428431,6.08622113553776,
132.030439780749));
#270092=CARTESIAN_POINT('Ctrl Pts',(-154.297022052244,4.32128631232727,
126.346576141847));
#270093=CARTESIAN_POINT('Ctrl Pts',(-154.575469676057,-1.41469952533967,
124.759198661251));
#270094=CARTESIAN_POINT('Ctrl Pts',(-154.85391729987,-5.85064561113321,
128.727029695929));
#270095=CARTESIAN_POINT('Ctrl Pts',(-155.132364923682,-4.9101342002235,
134.603826364333));
#270096=CARTESIAN_POINT('Ctrl Pts',(-155.410812547495,0.542550667301237,
136.989099625678));
#270097=CARTESIAN_POINT('Ctrl Pts',(-155.689260171308,5.49665797664923,
133.690899879866));
#270098=CARTESIAN_POINT('Ctrl Pts',(-155.967707795121,5.39960513212718,
127.740111567281));
#270099=CARTESIAN_POINT('Ctrl Pts',(-156.246155418934,0.340578956555753,
124.605218435021));
#270100=CARTESIAN_POINT('Ctrl Pts',(-156.524603042747,-5.03142264188343,
127.167034123586));
#270101=CARTESIAN_POINT('Ctrl Pts',(-156.80305066656,-5.77979263109261,
133.071375166841));
#270102=CARTESIAN_POINT('Ctrl Pts',(-157.081498290373,-1.21681555089514,
136.89244058913));
#270103=CARTESIAN_POINT('Ctrl Pts',(-157.359945914186,4.46435557583064,
135.118857936792));
#270104=CARTESIAN_POINT('Ctrl Pts',(-157.638393537999,6.04300202426259,
129.380463022997));
#270105=CARTESIAN_POINT('Ctrl Pts',(-157.916841161811,2.06842482945845,
124.950560437346));
#270106=CARTESIAN_POINT('Ctrl Pts',(-158.195288785624,-3.80693373544809,
125.900014243279));
#270107=CARTESIAN_POINT('Ctrl Pts',(-158.473736409437,-6.18390617652933,
131.356322776543));
#270108=CARTESIAN_POINT('Ctrl Pts',(-158.75218403325,-2.87817094199197,
136.305405050556));
#270109=CARTESIAN_POINT('Ctrl Pts',(-159.030631657063,3.07246278176887,
136.199296231612));
#270110=CARTESIAN_POINT('Ctrl Pts',(-159.309079280876,6.19965330723533,
131.135505140616));
#270111=CARTESIAN_POINT('Ctrl Pts',(-159.587526904689,3.62966531325439,
125.767408410247));
#270112=CARTESIAN_POINT('Ctrl Pts',(-159.865974528502,-2.27580778459908,
125.028024689608));
#270113=CARTESIAN_POINT('Ctrl Pts',(-160.144422152314,-6.08992470779737,
129.596811497064));
#270114=CARTESIAN_POINT('Ctrl Pts',(-160.422869776128,-4.3076983338908,
135.275276954208));
#270115=CARTESIAN_POINT('Ctrl Pts',(-160.70131739994,1.43309236609815,136.845188714382));
#270116=CARTESIAN_POINT('Ctrl Pts',(-160.979765023753,5.85694119209746,
132.863874564441));
#270117=CARTESIAN_POINT('Ctrl Pts',(-161.258212647566,4.89854719004298,
126.989967710171));
#270118=CARTESIAN_POINT('Ctrl Pts',(-161.536660271379,-0.561372372326459,
124.621301594343));
#270119=CARTESIAN_POINT('Ctrl Pts',(-161.815107895192,-5.50541814909322,
127.934564661631));
#270120=CARTESIAN_POINT('Ctrl Pts',(-162.093555519005,-5.39025360147175,
133.885030015096));
#270121=CARTESIAN_POINT('Ctrl Pts',(-162.372003142818,-0.32170932262588,
137.004510691297));
#270122=CARTESIAN_POINT('Ctrl Pts',(-162.650450766631,5.04247010733932,
134.426356343909));
#270123=CARTESIAN_POINT('Ctrl Pts',(-162.928898390443,5.77286584701905,
128.519764868338));
#270124=CARTESIAN_POINT('Ctrl Pts',(-163.207346014257,1.19827989346308,
124.712605277602));
#270125=CARTESIAN_POINT('Ctrl Pts',(-163.485793638069,-4.47746674295796,
126.503471245498));
#270126=CARTESIAN_POINT('Ctrl Pts',(-163.764241261882,-6.03864017901171,
132.246644436198));
#270127=CARTESIAN_POINT('Ctrl Pts',(-164.042688885695,-2.05059829452646,
136.664429257056));
#270128=CARTESIAN_POINT('Ctrl Pts',(-164.321136509508,3.82184324533235,
135.697097278492));
#270129=CARTESIAN_POINT('Ctrl Pts',(-164.599584133321,6.18219755015336,
130.23357933201));
#270130=CARTESIAN_POINT('Ctrl Pts',(-164.878031757134,2.86141432352365,
125.294581502737));
#270131=CARTESIAN_POINT('Ctrl Pts',(-165.156479380946,-3.08886887856293,
125.418801512319));
#270132=CARTESIAN_POINT('Ctrl Pts',(-165.43492700476,-6.20063248088431,
130.492087240433));
#270133=CARTESIAN_POINT('Ctrl Pts',(-165.713374628572,-3.61431775100944,
135.85233694673));
#270134=CARTESIAN_POINT('Ctrl Pts',(-165.991822252385,2.2933784228048,136.573743013877));
#270135=CARTESIAN_POINT('Ctrl Pts',(-166.270269876198,6.09357186382579,
131.993368508814));
#270136=CARTESIAN_POINT('Ctrl Pts',(-166.548717500011,4.2940704495262,126.320353837957));
#270137=CARTESIAN_POINT('Ctrl Pts',(-166.827165123824,-1.45147193088449,
124.767922341652));
#270138=CARTESIAN_POINT('Ctrl Pts',(-167.105612747637,-5.86318251515793,
128.762682724506));
#270139=CARTESIAN_POINT('Ctrl Pts',(-167.38406037145,-4.88691480039125,
134.633645349573));
#270140=CARTESIAN_POINT('Ctrl Pts',(-167.662507995262,0.580188876875391,
136.985682376883));
#270141=CARTESIAN_POINT('Ctrl Pts',(-167.940955619076,5.51412732009539,
133.657386681736));
#270142=CARTESIAN_POINT('Ctrl Pts',(-168.219403242888,5.38085213624319,
127.707299411689));
#270143=CARTESIAN_POINT('Ctrl Pts',(-168.497850866701,0.302836708424229,
124.60326008999));
#270144=CARTESIAN_POINT('Ctrl Pts',(-168.776298490514,-5.05347086004094,
127.197729212531));
#270145=CARTESIAN_POINT('Ctrl Pts',(-169.054746114327,-5.7658855839047,
133.106516402559));
#270146=CARTESIAN_POINT('Ctrl Pts',(-169.33319373814,-1.17973313533045,
136.899734892741));
#270147=CARTESIAN_POINT('Ctrl Pts',(-169.611641361953,4.49053643144484,
135.091602199623));
#270148=CARTESIAN_POINT('Ctrl Pts',(-169.890088985766,6.03422239262278,
129.34370393599));
#270149=CARTESIAN_POINT('Ctrl Pts',(-170.168536609579,2.03275276313275,
124.938077805679));
#270150=CARTESIAN_POINT('Ctrl Pts',(-170.446984233392,-3.83671735018369,
125.923278995643));
#270151=CARTESIAN_POINT('Ctrl Pts',(-170.725431857205,-6.18043165274327,
131.393955742061));
#270152=CARTESIAN_POINT('Ctrl Pts',(-171.003879481017,-2.84463119730373,
136.32282337239));
#270153=CARTESIAN_POINT('Ctrl Pts',(-171.282327104831,3.10524636049842,
136.180493322929));
#270154=CARTESIAN_POINT('Ctrl Pts',(-171.560774728643,6.20155421272058,
131.097759955922));
#270155=CARTESIAN_POINT('Ctrl Pts',(-171.839222352457,3.59893670621881,
125.745406930321));
#270156=CARTESIAN_POINT('Ctrl Pts',(-172.117669976268,-2.31092781546573,
125.04198519967));
#270157=CARTESIAN_POINT('Ctrl Pts',(-172.396117600082,-6.09716256983718,
129.633904970377));
#270158=CARTESIAN_POINT('Ctrl Pts',(-172.674565223895,-4.2804027854792,
135.301416300912));
#270159=CARTESIAN_POINT('Ctrl Pts',(-172.953012847708,1.469838049433,136.836353151837));
#270160=CARTESIAN_POINT('Ctrl Pts',(-173.23146047152,5.86936952249723,132.828183542982));
#270161=CARTESIAN_POINT('Ctrl Pts',(-173.509908095334,4.8752371390276,126.960219534917));
#270162=CARTESIAN_POINT('Ctrl Pts',(-173.788355719146,-0.599000006633149,
124.624833385073));
#270163=CARTESIAN_POINT('Ctrl Pts',(-174.06680334296,-5.5227854089755,127.968130875202));
#270164=CARTESIAN_POINT('Ctrl Pts',(-174.345250966772,-5.37140082353563,
133.917784941036));
#270165=CARTESIAN_POINT('Ctrl Pts',(-174.623698590585,-0.283961288785237,
137.006354152836));
#270166=CARTESIAN_POINT('Ctrl Pts',(-174.902146214398,5.06442479807889,
134.39559428995));
#270167=CARTESIAN_POINT('Ctrl Pts',(-175.18059383821,5.75885190641417,128.484666123661));
#270168=CARTESIAN_POINT('Ctrl Pts',(-175.459041462024,1.16117544831056,
124.705423873895));
#270169=CARTESIAN_POINT('Ctrl Pts',(-175.737489085836,-4.50356452021585,
126.530806541938));
#270170=CARTESIAN_POINT('Ctrl Pts',(-176.01593670965,-6.02974870602229,
132.28337663076));
#270171=CARTESIAN_POINT('Ctrl Pts',(-176.294384333462,-2.01488840059438,
136.676803257405));
#270172=CARTESIAN_POINT('Ctrl Pts',(-176.572831957276,3.85155591220881,
135.67374198281));
#270173=CARTESIAN_POINT('Ctrl Pts',(-176.851279581088,6.17860850065921,
130.195957116059));
#270174=CARTESIAN_POINT('Ctrl Pts',(-177.129727204901,2.82782171880919,
125.277265345029));
#270175=CARTESIAN_POINT('Ctrl Pts',(-177.408174828714,-3.12159507585506,
125.437704115845));
#270176=CARTESIAN_POINT('Ctrl Pts',(-177.686622452527,-6.20241849420629,
130.529838035997));
#270177=CARTESIAN_POINT('Ctrl Pts',(-177.965070076339,-3.58352232136993,
135.874244797437));
#270178=CARTESIAN_POINT('Ctrl Pts',(-178.243517700153,2.32845580000743,
136.559675675186));
#270179=CARTESIAN_POINT('Ctrl Pts',(-178.521965323965,6.10069679256748,
131.956253177754));
#270180=CARTESIAN_POINT('Ctrl Pts',(-178.800412947778,4.26669546836545,
126.294297690589));
#270181=CARTESIAN_POINT('Ctrl Pts',(-179.078860571591,-1.48819055160311,
124.776869704492));
#270182=CARTESIAN_POINT('Ctrl Pts',(-179.357308195404,-5.8755021567984,
128.798411408209));
#270183=CARTESIAN_POINT('Ctrl Pts',(-179.635755819217,-4.86351431413387,
134.663322439258));
#270184=CARTESIAN_POINT('Ctrl Pts',(-179.91420344303,0.617805587336893,
136.982036076937));
#270185=CARTESIAN_POINT('Ctrl Pts',(-180.192651066843,5.53139233552561,
133.623767763677));
#270186=CARTESIAN_POINT('Ctrl Pts',(-180.471098690656,5.36189975090491,
127.674602018838));
#270187=CARTESIAN_POINT('Ctrl Pts',(-180.749546314469,0.265083238567079,
124.601531529021));
#270188=CARTESIAN_POINT('Ctrl Pts',(-181.027993938281,-5.07533181997731,
127.22855794653));
#270189=CARTESIAN_POINT('Ctrl Pts',(-181.306441562095,-5.75176487970607,
133.141572331048));
#270190=CARTESIAN_POINT('Ctrl Pts',(-181.584889185907,-1.14260700432061,
136.906803330016));
#270191=CARTESIAN_POINT('Ctrl Pts',(-181.86333680972,4.5165508885802,135.064187597142));
#270192=CARTESIAN_POINT('Ctrl Pts',(-182.141784433533,6.02521916065313,
129.306998974155));
#270193=CARTESIAN_POINT('Ctrl Pts',(-182.420232057346,1.99700537240587,
124.925812551278));
#270194=CARTESIAN_POINT('Ctrl Pts',(-182.698679681159,-3.86635879394691,
125.946724618282));
#270195=CARTESIAN_POINT('Ctrl Pts',(-182.977127304972,-6.17672811078948,
131.431566859916));
#270196=CARTESIAN_POINT('Ctrl Pts',(-183.255574928785,-2.81098604376035,
136.340037205557));
#270197=CARTESIAN_POINT('Ctrl Pts',(-183.534022552597,3.13791487318212,
136.161491199671));
#270198=CARTESIAN_POINT('Ctrl Pts',(-183.81247017641,6.20322531733387,131.060003899207));
#270199=CARTESIAN_POINT('Ctrl Pts',(-184.090917800223,3.56807473926006,
125.723592911784));
#270200=CARTESIAN_POINT('Ctrl Pts',(-184.369365424036,-2.34596221405232,
125.056159236672));
#270201=CARTESIAN_POINT('Ctrl Pts',(-184.647813047849,-6.10417449927606,
129.671041815353));
#270202=CARTESIAN_POINT('Ctrl Pts',(-184.926260671662,-4.25294862516783,
135.327389007565));
#270203=CARTESIAN_POINT('Ctrl Pts',(-185.204708295475,1.50652926737877,
136.827294071589));
#270204=CARTESIAN_POINT('Ctrl Pts',(-185.483155919288,5.88158036125089,
132.792417528021));
#270205=CARTESIAN_POINT('Ctrl Pts',(-185.761603543101,4.85174643430717,
126.930613805724));
#270206=CARTESIAN_POINT('Ctrl Pts',(-186.040051166913,-0.6366054447743,
124.628594160457));
#270207=CARTESIAN_POINT('Ctrl Pts',(-186.318498790727,-5.53994802001346,
128.001802186308));
#270208=CARTESIAN_POINT('Ctrl Pts',(-186.596946414539,-5.35234900636664,
133.950424497894));
#270209=CARTESIAN_POINT('Ctrl Pts',(-186.875394038353,-0.246202732654624,
137.007967797222));
#270210=CARTESIAN_POINT('Ctrl Pts',(-187.153841662165,5.08619182469514,
134.364699161505));
#270211=CARTESIAN_POINT('Ctrl Pts',(-187.432289285978,5.744624569434,128.449653336115));
#270212=CARTESIAN_POINT('Ctrl Pts',(-187.71073690979,1.12402797537536,124.698468468532));
#270213=CARTESIAN_POINT('Ctrl Pts',(-187.989184533604,-4.52949541623416,
126.558300196495));
#270214=CARTESIAN_POINT('Ctrl Pts',(-188.267632157416,-6.0206337984771,
132.32005401984));
#270215=CARTESIAN_POINT('Ctrl Pts',(-188.54607978123,-1.97910384423165,
136.688959652232));
#270216=CARTESIAN_POINT('Ctrl Pts',(-188.824527405043,3.88112585826452,
135.650206250412));
#270217=CARTESIAN_POINT('Ctrl Pts',(-189.102975028855,6.17479050055486,
130.158357444724));
#270218=CARTESIAN_POINT('Ctrl Pts',(-189.381422652668,2.79412432812102,
125.260153995869));
#270219=CARTESIAN_POINT('Ctrl Pts',(-189.659870276481,-3.15420560129371,
125.456805582802));
#270220=CARTESIAN_POINT('Ctrl Pts',(-189.938317900294,-6.20397467462999,
130.567599004095));
#270221=CARTESIAN_POINT('Ctrl Pts',(-190.216765524107,-3.55259410299321,
135.89596478172));
#270222=CARTESIAN_POINT('Ctrl Pts',(-190.49521314792,2.36344689542356,136.545395071179));
#270223=CARTESIAN_POINT('Ctrl Pts',(-190.773660771733,6.10759565774615,
131.919095162891));
#270224=CARTESIAN_POINT('Ctrl Pts',(-191.052108395545,4.23916238323504,
126.26840866526));
#270225=CARTESIAN_POINT('Ctrl Pts',(-191.330556019359,-1.52485402687357,
124.786040418225));
#270226=CARTESIAN_POINT('Ctrl Pts',(-191.609003643171,-5.88760407954571,
128.834214423098));
#270227=CARTESIAN_POINT('Ctrl Pts',(-191.887451266984,-4.83993360856504,
134.692856533694));
#270228=CARTESIAN_POINT('Ctrl Pts',(-192.165898890797,0.655399404785621,
136.978160860955));
#270229=CARTESIAN_POINT('Ctrl Pts',(-192.44434651461,5.54845238317892,133.59004437145));
#270230=CARTESIAN_POINT('Ctrl Pts',(-192.722794138423,5.34274867839911,
127.642020600343));
#270231=CARTESIAN_POINT('Ctrl Pts',(-193.001241762236,0.227319945953055,
124.600032816164));
#270232=CARTESIAN_POINT('Ctrl Pts',(-193.279689386049,-5.09700471162664,
127.259519183211));
#270233=CARTESIAN_POINT('Ctrl Pts',(-193.558137009861,-5.73743104174462,
133.176541653297));
#270234=CARTESIAN_POINT('Ctrl Pts',(-193.836584633675,-1.105438533588,136.913645639033));
#270235=CARTESIAN_POINT('Ctrl Pts',(-194.115032257487,4.5423979832614,135.036615145204));
#270236=CARTESIAN_POINT('Ctrl Pts',(-194.3934798813,6.01599266197172,129.270349497605));
#270237=CARTESIAN_POINT('Ctrl Pts',(-194.671927505113,1.96118398191049,
124.913765128639));
#270238=CARTESIAN_POINT('Ctrl Pts',(-194.950375128926,-3.89585696836267,
125.970350242409));
#270239=CARTESIAN_POINT('Ctrl Pts',(-195.228822752739,-6.17279568790409,
131.469154736412));
#270240=CARTESIAN_POINT('Ctrl Pts',(-195.507270376552,-2.77723672809589,
136.357045912194));
#270241=CARTESIAN_POINT('Ctrl Pts',(-195.785718000365,3.17046710927626,
136.142290565968));
#270242=CARTESIAN_POINT('Ctrl Pts',(-196.064165624178,6.20466655915177,
131.022238369536));
#270243=CARTESIAN_POINT('Ctrl Pts',(-196.342613247991,3.5370805559797,125.701967162963));
#270244=CARTESIAN_POINT('Ctrl Pts',(-196.621060871803,-2.38090968214636,
125.070546275391));
#270245=CARTESIAN_POINT('Ctrl Pts',(-196.899508495616,-6.11096023628406,
129.708220655875));
#270246=CARTESIAN_POINT('Ctrl Pts',(-197.177956119429,-4.22533687028115,
135.353194111738));
#270247=CARTESIAN_POINT('Ctrl Pts',(-197.456403743242,1.54316466032852,
136.818011809327));
#270248=CARTESIAN_POINT('Ctrl Pts',(-197.734851367055,5.89357325588093,
132.75657784488));
#270249=CARTESIAN_POINT('Ctrl Pts',(-198.013298990868,4.82807594633875,
126.901151619645));
#270250=CARTESIAN_POINT('Ctrl Pts',(-198.291746614681,-0.674187293266194,
124.632583781138));
#270251=CARTESIAN_POINT('Ctrl Pts',(-198.570194238494,-5.55690534624021,
128.035577347248));
#270252=CARTESIAN_POINT('Ctrl Pts',(-198.848641862306,-5.33309885593691,
133.982947476197));
#270253=CARTESIAN_POINT('Ctrl Pts',(-199.12708948612,-0.2084350533912,137.009351564664));
#270254=CARTESIAN_POINT('Ctrl Pts',(-199.405537109932,5.10777038060287,
134.333672103408));
#270255=CARTESIAN_POINT('Ctrl Pts',(-199.683984733745,5.7301843632779,128.414727803113));
#270256=CARTESIAN_POINT('Ctrl Pts',(-199.962432357558,1.08683885116959,
124.691739319248));
#270257=CARTESIAN_POINT('Ctrl Pts',(-200.240879981371,-4.5552584701342,
126.585951190383));
#270258=CARTESIAN_POINT('Ctrl Pts',(-200.519327605184,-6.01129579413245,
132.356675244344));
#270259=CARTESIAN_POINT('Ctrl Pts',(-200.797775228997,-1.94324595144814,
136.700897991079));
#270260=CARTESIAN_POINT('Ctrl Pts',(-201.076222852809,3.91055198777426,
135.626490953421));
#270261=CARTESIAN_POINT('Ctrl Pts',(-201.354670476623,6.17074369131775,
130.120781711275));
#270262=CARTESIAN_POINT('Ctrl Pts',(-201.633118100435,2.76032340012831,
125.243248089324));
#270263=CARTESIAN_POINT('Ctrl Pts',(-201.911565724248,-3.18669924648382,
125.476105205376));
#270264=CARTESIAN_POINT('Ctrl Pts',(-202.190013348061,-6.20530096449064,
130.605368745483));
#270265=CARTESIAN_POINT('Ctrl Pts',(-202.468460971874,-3.52153424193529,
135.91749609474));
#270266=CARTESIAN_POINT('Ctrl Pts',(-202.746908595687,2.39835041244635,
136.530901731028));
#270267=CARTESIAN_POINT('Ctrl Pts',(-203.0253562195,6.11426820372151,131.881895841131));
#270268=CARTESIAN_POINT('Ctrl Pts',(-203.303803843313,4.21147221438356,
126.242687721299));
#270269=CARTESIAN_POINT('Ctrl Pts',(-203.582251467125,-1.56146099811728,
124.795434143027));
#270270=CARTESIAN_POINT('Ctrl Pts',(-203.860699090939,-5.89948783495869,
128.870090442477));
#270271=CARTESIAN_POINT('Ctrl Pts',(-204.139146714752,-4.81617355747646,
134.722246538484));
#270272=CARTESIAN_POINT('Ctrl Pts',(-204.417594338564,0.69296893616836,
136.974056872534));
#270273=CARTESIAN_POINT('Ctrl Pts',(-204.696041962377,5.56530683088876,
133.556217754686));
#270274=CARTESIAN_POINT('Ctrl Pts',(-204.97448958619,5.32339962837619,127.60955636352));
#270275=CARTESIAN_POINT('Ctrl Pts',(-205.252937210003,0.18954822991528,
124.598764006957));
#270276=CARTESIAN_POINT('Ctrl Pts',(-205.531384833816,-5.11848873189165,
127.290611775294));
#270277=CARTESIAN_POINT('Ctrl Pts',(-205.809832457629,-5.72288460116635,
133.211423073505));
#270278=CARTESIAN_POINT('Ctrl Pts',(-206.088280081441,-1.06822910042401,
136.920261566246));
#270279=CARTESIAN_POINT('Ctrl Pts',(-206.366727705255,4.56807675771487,
135.00888586552));
#270280=CARTESIAN_POINT('Ctrl Pts',(-206.645175329067,6.00654323846982,
129.233756864401));
#270281=CARTESIAN_POINT('Ctrl Pts',(-206.92362295288,1.92528991902147,124.901935984182));
#270282=CARTESIAN_POINT('Ctrl Pts',(-207.202070576693,-3.92521078036628,
125.994154992568));
#270283=CARTESIAN_POINT('Ctrl Pts',(-207.480518200506,-6.16863452980439,
131.506717978718));
#270284=CARTESIAN_POINT('Ctrl Pts',(-207.758965824319,-2.74338450090264,
136.373848862034));
#270285=CARTESIAN_POINT('Ctrl Pts',(-208.037413448132,3.20290186254569,
136.12289213331));
#270286=CARTESIAN_POINT('Ctrl Pts',(-208.315861071945,6.20587788476857,
130.984464766326));
#270287=CARTESIAN_POINT('Ctrl Pts',(-208.594308695758,3.50595530487857,
125.680530485208));
#270288=CARTESIAN_POINT('Ctrl Pts',(-208.872756319571,-2.41576892475653,
125.085145782709));
#270289=CARTESIAN_POINT('Ctrl Pts',(-209.151203943383,-6.11751952941318,
129.745440114266));
#270290=CARTESIAN_POINT('Ctrl Pts',(-209.429651567197,-4.19756854398286,
135.378830657213));
#270291=CARTESIAN_POINT('Ctrl Pts',(-209.708099191009,1.57974287074426,
136.808506709009));
#270292=CARTESIAN_POINT('Ctrl Pts',(-209.986546814822,5.90534776198698,
132.720665821612));
#270293=CARTESIAN_POINT('Ctrl Pts',(-210.264994438635,4.80422655224024,
126.87183406841));
#270294=CARTESIAN_POINT('Ctrl Pts',(-210.543442062448,-0.711744159500396,
124.63680209928));
#270295=CARTESIAN_POINT('Ctrl Pts',(-210.821889686261,-5.57365675929581,
128.06945510647));
#270296=CARTESIAN_POINT('Ctrl Pts',(-211.100337310074,-5.31365108556781,
134.015352670796));
#270297=CARTESIAN_POINT('Ctrl Pts',(-211.378784933887,-0.170659650490228,
137.010505403884));
#270298=CARTESIAN_POINT('Ctrl Pts',(-211.657232557699,5.12915966620077,
134.302514265376));
#270299=CARTESIAN_POINT('Ctrl Pts',(-211.935680181513,5.71553182303293,
128.379890818834));
#270300=CARTESIAN_POINT('Ctrl Pts',(-212.214127805325,1.04960945375051,
124.685236675394));
#270301=CARTESIAN_POINT('Ctrl Pts',(-212.492575429138,-4.58085272725645,
126.613758498985));
#270302=CARTESIAN_POINT('Ctrl Pts',(-212.771023052951,-6.00173503901134,
132.393238947258));
#270303=CARTESIAN_POINT('Ctrl Pts',(-213.049470676764,-1.90731605097184,
136.712617831564));
#270304=CARTESIAN_POINT('Ctrl Pts',(-213.327918300577,3.93983321034183,
135.602596970618));
#270305=CARTESIAN_POINT('Ctrl Pts',(-213.60636592439,6.16646822290386,130.083231308093));
#270306=CARTESIAN_POINT('Ctrl Pts',(-213.884813548203,2.72642018733693,
125.226548251849));
#270307=CARTESIAN_POINT('Ctrl Pts',(-214.163261172015,-3.21907480736146,
125.495602268416));
#270308=CARTESIAN_POINT('Ctrl Pts',(-214.441708795829,-6.20639731464204,
130.643145860587));
#270309=CARTESIAN_POINT('Ctrl Pts',(-214.720156419641,-3.49034388913101,
135.938837938644));
#270310=CARTESIAN_POINT('Ctrl Pts',(-214.998604043455,2.43316505771265,
136.516196191791));
#270311=CARTESIAN_POINT('Ctrl Pts',(-215.277051667267,6.12071418324004,
131.844656590906));
#270312=CARTESIAN_POINT('Ctrl Pts',(-215.55549929108,4.18362598788043,126.217135811804));
#270313=CARTESIAN_POINT('Ctrl Pts',(-215.833946914893,-1.59801010884951,
124.805050530808));
#270314=CARTESIAN_POINT('Ctrl Pts',(-216.112394538706,-5.91115298268039,
128.90603813695));
#270315=CARTESIAN_POINT('Ctrl Pts',(-216.390842162519,-4.79223504130557,
134.75149136457));
#270316=CARTESIAN_POINT('Ctrl Pts',(-216.669289786332,0.730512789332353,
136.969724263749));
#270317=CARTESIAN_POINT('Ctrl Pts',(-216.947737410145,5.5819550541073,133.522289166845));
#270318=CARTESIAN_POINT('Ctrl Pts',(-217.226185033957,5.3038533178224,127.577210511344));
#270319=CARTESIAN_POINT('Ctrl Pts',(-217.50463265777,0.151769490097695,
124.597725148413));
#270320=CARTESIAN_POINT('Ctrl Pts',(-217.783080281583,-5.13978308467467,
127.321834570635));
#270321=CARTESIAN_POINT('Ctrl Pts',(-218.061527905396,-5.70812609699421,
133.24621529913));
#270322=CARTESIAN_POINT('Ctrl Pts',(-218.339975529209,-1.03098008363786,
136.9266508665));
#270323=CARTESIAN_POINT('Ctrl Pts',(-218.618423153022,4.59358626040416,
134.981000785606));
#270324=CARTESIAN_POINT('Ctrl Pts',(-218.896870776835,5.99687124029931,
129.197222430498));
#270325=CARTESIAN_POINT('Ctrl Pts',(-219.175318400648,1.88932451380644,
124.890325556239));
#270326=CARTESIAN_POINT('Ctrl Pts',(-219.45376602446,-3.95441914224089,
126.018137986666));
#270327=CARTESIAN_POINT('Ctrl Pts',(-219.732213648274,-6.16424479068368,
131.544255194914));
#270328=CARTESIAN_POINT('Ctrl Pts',(-220.010661272086,-2.70943061658779,
136.390445432439));
#270329=CARTESIAN_POINT('Ctrl Pts',(-220.289108895899,3.23521793110825,
136.103296620509));
#270330=CARTESIAN_POINT('Ctrl Pts',(-220.567556519712,6.20685924929812,
130.94668448929));
#270331=CARTESIAN_POINT('Ctrl Pts',(-220.846004143525,3.47470013931478,
125.659283672863));
#270332=CARTESIAN_POINT('Ctrl Pts',(-221.124451767337,-2.45053865016082,
125.099957217636));
#270333=CARTESIAN_POINT('Ctrl Pts',(-221.402899391151,-6.12385213560643,
129.782698811345));
#270334=CARTESIAN_POINT('Ctrl Pts',(-221.681347014963,-4.16964467523852,
135.404297694017));
#270335=CARTESIAN_POINT('Ctrl Pts',(-221.959794638777,1.61626254320698,
136.79877912285));
#270336=CARTESIAN_POINT('Ctrl Pts',(-222.238242262589,5.91690344326002,
132.684682788949));
#270337=CARTESIAN_POINT('Ctrl Pts',(-222.516689886402,4.7801991357601,126.842662238393));
#270338=CARTESIAN_POINT('Ctrl Pts',(-222.795137510215,-0.749274651793031,
124.64124895857));
#270339=CARTESIAN_POINT('Ctrl Pts',(-223.073585134028,-5.59020163845046,
128.103434208622));
#270340=CARTESIAN_POINT('Ctrl Pts',(-223.352032757841,-5.29400641590365,
134.047638880903));
#270341=CARTESIAN_POINT('Ctrl Pts',(-223.630480381654,-0.132877923733138,
137.011429272127));
#270342=CARTESIAN_POINT('Ctrl Pts',(-223.908928005467,5.15035888890098,
134.271226801972));
#270343=CARTESIAN_POINT('Ctrl Pts',(-224.187375629279,5.70066749165438,
128.345143674176));
#270344=CARTESIAN_POINT('Ctrl Pts',(-224.465823253093,1.01234116266713,
124.678960777928));
#270345=CARTESIAN_POINT('Ctrl Pts',(-224.744270876905,-4.60627723919628,
126.641721091889));
#270346=CARTESIAN_POINT('Ctrl Pts',(-225.022718500718,-5.99195188739136,
132.4297437737));
#270347=CARTESIAN_POINT('Ctrl Pts',(-225.301166124531,-1.87131547419729,
136.724118739406));
#270348=CARTESIAN_POINT('Ctrl Pts',(-225.579613748344,3.96896844094108,
135.578525187401));
#270349=CARTESIAN_POINT('Ctrl Pts',(-225.858061372157,6.16196425374224,
130.045707626623));
#270350=CARTESIAN_POINT('Ctrl Pts',(-226.13650899597,2.69241594604283,125.210055102262));
#270351=CARTESIAN_POINT('Ctrl Pts',(-226.414956619783,-3.25133108423828,
125.515296049447));
#270352=CARTESIAN_POINT('Ctrl Pts',(-226.693404243596,-6.20726368445854,
130.680928949564));
#270353=CARTESIAN_POINT('Ctrl Pts',(-226.971851867408,-3.45902420035033,
135.959989522602));
#270354=CARTESIAN_POINT('Ctrl Pts',(-227.250299491222,2.46788954115291,
136.501278998386));
#270355=CARTESIAN_POINT('Ctrl Pts',(-227.528747115034,6.12693335744362,
131.80737879213));
#270356=CARTESIAN_POINT('Ctrl Pts',(-227.807194738847,4.15562473557794,
126.191753883612));
#270357=CARTESIAN_POINT('Ctrl Pts',(-228.08564236266,-1.63450000472891,
124.81488922523));
#270358=CARTESIAN_POINT('Ctrl Pts',(-228.364089986473,-5.9225990904546,
128.942056174461));
#270359=CARTESIAN_POINT('Ctrl Pts',(-228.642537610286,-4.76811894710285,
134.780589928275));
#270360=CARTESIAN_POINT('Ctrl Pts',(-228.920985234099,0.768029573076269,
136.965163195147));
#270361=CARTESIAN_POINT('Ctrl Pts',(-229.199432857912,5.59839643592858,
133.48825986516));
#270362=CARTESIAN_POINT('Ctrl Pts',(-229.477880481725,5.28411047103341,
127.544984242401));
#270363=CARTESIAN_POINT('Ctrl Pts',(-229.756328105537,0.11398512640586,
124.59691627903));
#270364=CARTESIAN_POINT('Ctrl Pts',(-230.03477572935,-5.16088698090536,
127.353186412258));
#270365=CARTESIAN_POINT('Ctrl Pts',(-230.313223353163,-5.69315607611037,
133.280917040931));
#270366=CARTESIAN_POINT('Ctrl Pts',(-230.591670976976,-0.993692863505588,
136.932813303039));
#270367=CARTESIAN_POINT('Ctrl Pts',(-230.870118600789,4.6189255460653,134.952960938754));
#270368=CARTESIAN_POINT('Ctrl Pts',(-231.148566224602,5.98697702585963,
129.160747549691));
#270369=CARTESIAN_POINT('Ctrl Pts',(-231.427013848415,1.85328909897679,
124.878934275042));
#270370=CARTESIAN_POINT('Ctrl Pts',(-231.705461472227,-3.98348097165998,
126.042298336002));
#270371=CARTESIAN_POINT('Ctrl Pts',(-231.983909096041,-6.15962663320533,
131.581764994044));
#270372=CARTESIAN_POINT('Ctrl Pts',(-232.262356719853,-2.6753763333251,
136.406835008417));
#270373=CARTESIAN_POINT('Ctrl Pts',(-232.540804343666,3.26741411748112,
136.083504753687));
#270374=CARTESIAN_POINT('Ctrl Pts',(-232.819251967479,6.20761061637562,
130.90889893839));
#270375=CARTESIAN_POINT('Ctrl Pts',(-233.097699591292,3.44331621745904,
125.638227513236));
#270376=CARTESIAN_POINT('Ctrl Pts',(-233.376147215105,-2.48521756995422,
125.114980031328));
#270377=CARTESIAN_POINT('Ctrl Pts',(-233.654594838918,-6.12995782020675,
129.819995366479));
#270378=CARTESIAN_POINT('Ctrl Pts',(-233.933042462731,-4.14156629877734,
135.429594278462));
#270379=CARTESIAN_POINT('Ctrl Pts',(-234.211490086544,1.65272232446679,
136.788829411307));
#270380=CARTESIAN_POINT('Ctrl Pts',(-234.489937710357,5.92823987150001,
132.648630080257));
#270381=CARTESIAN_POINT('Ctrl Pts',(-234.768385334169,4.75599458724306,
126.813637210565));
#270382=CARTESIAN_POINT('Ctrl Pts',(-235.046832957982,-0.786777379437916,
124.64592419423));
#270383=CARTESIAN_POINT('Ctrl Pts',(-235.325280581795,-5.6065393706272,
128.137513394595));
#270384=CARTESIAN_POINT('Ctrl Pts',(-235.603728205608,-5.27416557488518,
134.079804910139));
#270385=CARTESIAN_POINT('Ctrl Pts',(-235.882175829421,-0.0950912731361558,
137.012123135159));
#270386=CARTESIAN_POINT('Ctrl Pts',(-236.160623453234,5.17136726315852,
134.239810872567));
#270387=CARTESIAN_POINT('Ctrl Pts',(-236.439071077047,5.68559191994549,
128.310487656705));
#270388=CARTESIAN_POINT('Ctrl Pts',(-236.71751870086,0.975035358909668,
124.672911859406));
#270389=CARTESIAN_POINT('Ctrl Pts',(-236.995966324673,-4.63153106383903,
126.669837932931));
#270390=CARTESIAN_POINT('Ctrl Pts',(-237.274413948486,-5.98194670179065,
132.466188370973));
#270391=CARTESIAN_POINT('Ctrl Pts',(-237.552861572298,-1.83524555513966,
136.735400288432));
#270392=CARTESIAN_POINT('Ctrl Pts',(-237.831309196112,3.99795659995517,
135.554276495761));
#270393=CARTESIAN_POINT('Ctrl Pts',(-238.109756819924,6.15723195072914,
130.008212057319));
#270394=CARTESIAN_POINT('Ctrl Pts',(-238.388204443737,2.65831193628575,
125.193769251723));
#270395=CARTESIAN_POINT('Ctrl Pts',(-238.66665206755,-3.28346688184612,
125.535185818711));
#270396=CARTESIAN_POINT('Ctrl Pts',(-238.945099691363,-6.20790004183648,
130.718716612347));
#270397=CARTESIAN_POINT('Ctrl Pts',(-239.223547315176,-3.42757633615586,
135.980950062836));
#270398=CARTESIAN_POINT('Ctrl Pts',(-239.501994938989,2.50252257603867,
136.486150703575));
#270399=CARTESIAN_POINT('Ctrl Pts',(-239.780442562802,6.13292549587844,
131.770063826148));
#270400=CARTESIAN_POINT('Ctrl Pts',(-240.058890186614,4.12746949507249,
126.166542877259));
#270401=CARTESIAN_POINT('Ctrl Pts',(-240.337337810428,-1.67092933361012,
124.824949861719));
#270402=CARTESIAN_POINT('Ctrl Pts',(-240.61578543424,-5.93382573414137,
128.978143220346));
#270403=CARTESIAN_POINT('Ctrl Pts',(-240.894233058053,-4.74382616849909,
134.80954115134));
#270404=CARTESIAN_POINT('Ctrl Pts',(-241.172680681866,0.805517897201924,
136.960373835741));
#270405=CARTESIAN_POINT('Ctrl Pts',(-241.451128305679,5.6146303671111,133.454131110603));
#270406=CARTESIAN_POINT('Ctrl Pts',(-241.729575929492,5.26417181958768,
127.512878750849));
#270407=CARTESIAN_POINT('Ctrl Pts',(-242.008023553305,0.0761965389532375,
124.596337428779));
#270408=CARTESIAN_POINT('Ctrl Pts',(-242.286471177117,-5.18179963857104,
127.384666138411));
#270409=CARTESIAN_POINT('Ctrl Pts',(-242.564918800931,-5.67797509323448,
133.315527013022));
#270410=CARTESIAN_POINT('Ctrl Pts',(-242.843366424743,-0.956368821719198,
136.938748647509));
#270411=CARTESIAN_POINT('Ctrl Pts',(-243.121814048556,4.64409367574132,
134.924767363992));
#270412=CARTESIAN_POINT('Ctrl Pts',(-243.400261672369,5.9768609617849,129.124333573571));
#270413=CARTESIAN_POINT('Ctrl Pts',(-243.678709296182,1.81718500983798,
124.867762562695));
#270414=CARTESIAN_POINT('Ctrl Pts',(-243.957156919995,-4.01239519172672,
126.066635145309));
#270415=CARTESIAN_POINT('Ctrl Pts',(-244.235604543808,-6.15478022849689,
131.619245986169));
#270416=CARTESIAN_POINT('Ctrl Pts',(-244.514052167621,-2.64122291300849,
136.423016982646));
#270417=CARTESIAN_POINT('Ctrl Pts',(-244.792499791433,3.29948922862226,
136.063517266237));
#270418=CARTESIAN_POINT('Ctrl Pts',(-245.070947415247,6.20813195815889,
130.871109513785));
#270419=CARTESIAN_POINT('Ctrl Pts',(-245.349395039059,3.41180470225455,
125.617362786572));
#270420=CARTESIAN_POINT('Ctrl Pts',(-245.627842662872,-2.51980439909662,
125.13021366711));
#270421=CARTESIAN_POINT('Ctrl Pts',(-245.906290286685,-6.13583635696575,
129.857328397629));
#270422=CARTESIAN_POINT('Ctrl Pts',(-246.184737910498,-4.1133344550539,
135.454719473173));
#270423=CARTESIAN_POINT('Ctrl Pts',(-246.463185534311,1.68912086349306,
136.778657943074));
#270424=CARTESIAN_POINT('Ctrl Pts',(-246.741633158124,5.93935662663147,
132.612509031482));
#270425=CARTESIAN_POINT('Ctrl Pts',(-247.020080781937,4.73161380359756,
126.784760060463));
#270426=CARTESIAN_POINT('Ctrl Pts',(-247.29852840575,-0.824250952757648,
124.650827633015));
#270427=CARTESIAN_POINT('Ctrl Pts',(-247.576976029562,-5.62266935042617,
128.171691401572));
#270428=CARTESIAN_POINT('Ctrl Pts',(-247.855423653376,-5.25412929772145,
134.111849566585));
#270429=CARTESIAN_POINT('Ctrl Pts',(-248.133871277188,-0.0573010988966442,
137.012586967267));
#270430=CARTESIAN_POINT('Ctrl Pts',(-248.412318901001,5.19218401050035,
134.208267641291));
#270431=CARTESIAN_POINT('Ctrl Pts',(-248.690766524814,5.67030566653712,
128.275924050614));
#270432=CARTESIAN_POINT('Ctrl Pts',(-248.969214148627,0.937693424858449,
124.667090143972));
#270433=CARTESIAN_POINT('Ctrl Pts',(-249.24766177244,-4.65661326539506,
126.698107980232));
#270434=CARTESIAN_POINT('Ctrl Pts',(-249.526109396252,-5.97171985295489,
132.502571388608));
#270435=CARTESIAN_POINT('Ctrl Pts',(-249.804557020066,-1.79910763038337,
136.746462060605));
#270436=CARTESIAN_POINT('Ctrl Pts',(-250.083004643878,4.02679661321771,
135.52985179424));
#270437=CARTESIAN_POINT('Ctrl Pts',(-250.361452267692,6.15227148922063,
129.970745989595));
#270438=CARTESIAN_POINT('Ctrl Pts',(-250.639899891504,2.62410942180459,
125.177691303707));
#270439=CARTESIAN_POINT('Ctrl Pts',(-250.918347515317,-3.31548100938434,
125.555270839195));
#270440=CARTESIAN_POINT('Ctrl Pts',(-251.19679513913,-6.20830636318893,
130.756507448682));
#270441=CARTESIAN_POINT('Ctrl Pts',(-251.475242762943,-3.39600146187203,
136.001718782677));
#270442=CARTESIAN_POINT('Ctrl Pts',(-251.753690386756,2.53706287905323,
136.47081186788));
#270443=CARTESIAN_POINT('Ctrl Pts',(-252.032138010569,6.13869037645988,
131.732713075798));
#270444=CARTESIAN_POINT('Ctrl Pts',(-252.310585634382,4.09916130974965,
126.141503726722));
#270445=CARTESIAN_POINT('Ctrl Pts',(-252.589033258195,-1.70729674574642,
124.835232067896));
#270446=CARTESIAN_POINT('Ctrl Pts',(-252.867480882007,-5.94483249743877,
129.014297936587));
#270447=CARTESIAN_POINT('Ctrl Pts',(-253.14592850582,-4.71935760622846,
134.838343962485));
#270448=CARTESIAN_POINT('Ctrl Pts',(-253.424376129633,0.842976373616159,
136.955356360136));
#270449=CARTESIAN_POINT('Ctrl Pts',(-253.702823753446,5.63065624411703,
133.419904173236));
#270450=CARTESIAN_POINT('Ctrl Pts',(-253.981271377259,5.24403810606461,
127.480895216153));
#270451=CARTESIAN_POINT('Ctrl Pts',(-254.259719001072,0.0384051209378723,
124.595988638398));
#270452=CARTESIAN_POINT('Ctrl Pts',(-254.538166624885,-5.20252026939218,
127.416272546179));
#270453=CARTESIAN_POINT('Ctrl Pts',(-254.816614248698,-5.66258373611722,
133.350044001689));
#270454=CARTESIAN_POINT('Ctrl Pts',(-255.095061872511,-0.919009293725241,
136.944456550123));
#270455=CARTESIAN_POINT('Ctrl Pts',(-255.373509496324,4.6690896269236,134.896421351226));
#270456=CARTESIAN_POINT('Ctrl Pts',(-255.651957120136,5.96652359266914,
129.087981388513));
#270457=CARTESIAN_POINT('Ctrl Pts',(-255.93040474395,1.78101326373629,124.856811707331));
#270458=CARTESIAN_POINT('Ctrl Pts',(-256.208852367762,-4.04116012583712,
126.091145862189));
#270459=CARTESIAN_POINT('Ctrl Pts',(-256.487299991575,-6.14970689884083,
131.656699899059));
#270460=CARTESIAN_POINT('Ctrl Pts',(-256.765747615388,-2.60696946356087,
136.438984870644));
#270461=CARTESIAN_POINT('Ctrl Pts',(-257.044195239201,3.33143800190474,
136.043346010603));
#270462=CARTESIAN_POINT('Ctrl Pts',(-257.322642863014,6.2084309480058,130.833296634437));
#270463=CARTESIAN_POINT('Ctrl Pts',(-257.601090486826,3.38015223603414,
125.596729883064));
#270464=CARTESIAN_POINT('Ctrl Pts',(-257.87953811064,-2.5542704291637,125.145582755354));
#270465=CARTESIAN_POINT('Ctrl Pts',(-258.157985734452,-6.14153931545366,
129.894837769574));
#270466=CARTESIAN_POINT('Ctrl Pts',(-258.436433358265,-4.08485240479644,
135.479405634932));
#270467=CARTESIAN_POINT('Ctrl Pts',(-258.714880982078,1.72527217059264,
136.768768758555));
#270468=CARTESIAN_POINT('Ctrl Pts',(-258.993328605892,5.95060195420752,
132.575369498931));
#270469=CARTESIAN_POINT('Ctrl Pts',(-259.271776229703,4.70639920604184,
126.75783223591));
#270470=CARTESIAN_POINT('Ctrl Pts',(-259.550223853517,-0.860449444711704,
124.652528659269));
#270471=CARTESIAN_POINT('Ctrl Pts',(-259.82867147733,-5.64095031490746,
128.212697490595));
#270472=CARTESIAN_POINT('Ctrl Pts',(-260.060711163841,-5.29799179572588,
133.142936715762));
#270473=CARTESIAN_POINT('Ctrl Pts',(-260.246372125917,-2.62679689981868,
135.594171577488));
#270474=CARTESIAN_POINT('Ctrl Pts',(-260.339217213388,-0.889986900407246,
136.05080276614));
#270475=CARTESIAN_POINT('Ctrl Pts',(-260.385654363559,-0.0148419801173944,
136.053268468065));
#270476=CARTESIAN_POINT('Ctrl Pts',(209.997106195361,2.85369542052185,134.803838223542));
#270477=CARTESIAN_POINT('Ctrl Pts',(209.950688331758,3.52024512455777,134.328247120061));
#270478=CARTESIAN_POINT('Ctrl Pts',(209.857862530854,4.598911638141,133.039517383424));
#270479=CARTESIAN_POINT('Ctrl Pts',(209.672220855345,5.31158968331849,129.722011776094));
#270480=CARTESIAN_POINT('Ctrl Pts',(209.440181168834,2.90445768035623,125.771581499823));
#270481=CARTESIAN_POINT('Ctrl Pts',(209.161733545021,-2.67328939945229,
125.640965885288));
#270482=CARTESIAN_POINT('Ctrl Pts',(208.883285921209,-5.78445646322271,
130.262241799363));
#270483=CARTESIAN_POINT('Ctrl Pts',(208.604838297395,-3.58517659481558,
135.378114005881));
#270484=CARTESIAN_POINT('Ctrl Pts',(208.326390673583,1.91144119617671,136.292814641374));
#270485=CARTESIAN_POINT('Ctrl Pts',(208.04794304977,5.65009034124608,132.162897902674));
#270486=CARTESIAN_POINT('Ctrl Pts',(207.769495425957,4.19734896093999,126.785079177362));
#270487=CARTESIAN_POINT('Ctrl Pts',(207.491047802144,-1.1129569716493,125.100504449821));
#270488=CARTESIAN_POINT('Ctrl Pts',(207.212600178331,-5.4002948496084,128.657642803108));
#270489=CARTESIAN_POINT('Ctrl Pts',(206.934152554519,-4.72513942780656,
134.187431620732));
#270490=CARTESIAN_POINT('Ctrl Pts',(206.655704930705,0.292248586550605,
136.608384944684));
#270491=CARTESIAN_POINT('Ctrl Pts',(206.377257306892,5.04104249491135,133.695701483205));
#270492=CARTESIAN_POINT('Ctrl Pts',(206.09880968308,5.15738153042831,128.12602865207));
#270493=CARTESIAN_POINT('Ctrl Pts',(205.820362059267,0.534329935251406,
125.017605890956));
#270494=CARTESIAN_POINT('Ctrl Pts',(205.541914435454,-4.57974002364783,
127.226931288585));
#270495=CARTESIAN_POINT('Ctrl Pts',(205.263466811641,-5.48525514562618,
132.723737743954));
#270496=CARTESIAN_POINT('Ctrl Pts',(204.985019187828,-1.35008742798131,
136.456731302353));
#270497=CARTESIAN_POINT('Ctrl Pts',(204.706571564015,4.02574397595362,134.995471850294));
#270498=CARTESIAN_POINT('Ctrl Pts',(204.428123940202,5.70211370766606,129.682786179275));
#270499=CARTESIAN_POINT('Ctrl Pts',(204.149676316389,2.13851930815143,125.40077248911));
#270500=CARTESIAN_POINT('Ctrl Pts',(203.871228692576,-3.39026975841633,
126.084392381055));
#270501=CARTESIAN_POINT('Ctrl Pts',(203.592781068764,-5.8035665963141,131.105432460946));
#270502=CARTESIAN_POINT('Ctrl Pts',(203.314333444951,-2.88366922283368,
135.849802245147));
#270503=CARTESIAN_POINT('Ctrl Pts',(203.035885821138,2.68617927581077,135.957657646429));
#270504=CARTESIAN_POINT('Ctrl Pts',(202.757438197325,5.78756025537181,131.329884836407));
#270505=CARTESIAN_POINT('Ctrl Pts',(202.478990573512,3.57045609392238,126.219180939555));
#270506=CARTESIAN_POINT('Ctrl Pts',(202.200542949699,-1.92772278905516,
125.322033169903));
#270507=CARTESIAN_POINT('Ctrl Pts',(201.922095325886,-5.6544186046078,129.462876497226));
#270508=CARTESIAN_POINT('Ctrl Pts',(201.643647702073,-4.18497995558374,
134.836478196445));
#270509=CARTESIAN_POINT('Ctrl Pts',(201.36520007826,1.13025082464198,136.504760820331));
#270510=CARTESIAN_POINT('Ctrl Pts',(201.086752454448,5.4068363130258,132.934654138033));
#270511=CARTESIAN_POINT('Ctrl Pts',(200.808304830635,4.71480336828096,127.406911780982));
#270512=CARTESIAN_POINT('Ctrl Pts',(200.529857206822,-0.309903540913717,
125.001258930184));
#270513=CARTESIAN_POINT('Ctrl Pts',(200.251409583008,-5.04982423566531,
127.928373032793));
#270514=CARTESIAN_POINT('Ctrl Pts',(199.972961959197,-5.14920315545485,
133.498379226012));
#270515=CARTESIAN_POINT('Ctrl Pts',(199.694514335383,-0.516715927947778,
136.59271392819));
#270516=CARTESIAN_POINT('Ctrl Pts',(199.416066711571,4.59060799437092,134.367834714685));
#270517=CARTESIAN_POINT('Ctrl Pts',(199.137619087757,5.47938743352869,128.868296891315));
#270518=CARTESIAN_POINT('Ctrl Pts',(198.859171463945,1.33287750423228,125.147907050397));
#270519=CARTESIAN_POINT('Ctrl Pts',(198.580723840131,-4.03848173676817,
126.625521704588));
#270520=CARTESIAN_POINT('Ctrl Pts',(198.302276216319,-5.69867355247927,
131.943285172176));
#270521=CARTESIAN_POINT('Ctrl Pts',(198.023828592506,-2.12206276914206,
136.214432613634));
#270522=CARTESIAN_POINT('Ctrl Pts',(197.745380968693,3.4046200305072,135.513988187415));
#270523=CARTESIAN_POINT('Ctrl Pts',(197.46693334488,5.80262334705539,130.485626102603));
#270524=CARTESIAN_POINT('Ctrl Pts',(197.188485721067,2.86829928156946,125.750165465994));
#270525=CARTESIAN_POINT('Ctrl Pts',(196.910038097254,-2.70185169946893,
125.65926326252));
#270526=CARTESIAN_POINT('Ctrl Pts',(196.631590473441,-5.78913296148881,
130.296454176353));
#270527=CARTESIAN_POINT('Ctrl Pts',(196.353142849628,-3.5564838467683,135.400386297052));
#270528=CARTESIAN_POINT('Ctrl Pts',(196.074695225815,1.94440017923737,136.280795346639));
#270529=CARTESIAN_POINT('Ctrl Pts',(195.796247602003,5.6584754297534,132.128628418917));
#270530=CARTESIAN_POINT('Ctrl Pts',(195.51779997819,4.17268819221861,126.759524075833));
#270531=CARTESIAN_POINT('Ctrl Pts',(195.239352354377,-1.14759564681435,
125.107426913349));
#270532=CARTESIAN_POINT('Ctrl Pts',(194.960904730564,-5.41329514958902,
128.690533514357));
#270533=CARTESIAN_POINT('Ctrl Pts',(194.682457106751,-4.70444086406131,
134.216143957018));
#270534=CARTESIAN_POINT('Ctrl Pts',(194.404009482938,0.327564750825761,
136.606492185605));
#270535=CARTESIAN_POINT('Ctrl Pts',(194.125561859125,5.0585543621317,133.664964953048));
#270536=CARTESIAN_POINT('Ctrl Pts',(193.847114235312,5.14097963875765,128.094682084473));
#270537=CARTESIAN_POINT('Ctrl Pts',(193.568666611499,0.499095778182989,
125.014461412655));
#270538=CARTESIAN_POINT('Ctrl Pts',(193.290218987687,-4.60143272035756,
127.254875257849));
#270539=CARTESIAN_POINT('Ctrl Pts',(193.011771363874,-5.4734693413749,132.757092746623));
#270540=CARTESIAN_POINT('Ctrl Pts',(192.733323740061,-1.31565503151135,
136.464844805061));
#270541=CARTESIAN_POINT('Ctrl Pts',(192.454876116248,4.05118197898966,134.970888425217));
#270542=CARTESIAN_POINT('Ctrl Pts',(192.176428492435,5.69518066204141,129.648096536341));
#270543=CARTESIAN_POINT('Ctrl Pts',(191.897980868622,2.1055865417199,125.38785485147));
#270544=CARTESIAN_POINT('Ctrl Pts',(191.619533244809,-3.4189387468211,126.105117354624));
#270545=CARTESIAN_POINT('Ctrl Pts',(191.341085620997,-5.80162635147675,
131.140754845624));
#270546=CARTESIAN_POINT('Ctrl Pts',(191.062637997183,-2.85290276432908,
135.867262474811));
#270547=CARTESIAN_POINT('Ctrl Pts',(190.784190373371,2.71749909118881,135.941210633695));
#270548=CARTESIAN_POINT('Ctrl Pts',(190.505742749557,5.79065203911519,131.29464457683));
#270549=CARTESIAN_POINT('Ctrl Pts',(190.227295125745,3.54247865217362,126.197531513104));
#270550=CARTESIAN_POINT('Ctrl Pts',(189.948847501932,-1.96105955641241,
125.333869340265));
#270551=CARTESIAN_POINT('Ctrl Pts',(189.670399878119,-5.66247983574075,
129.497321402909));
#270552=CARTESIAN_POINT('Ctrl Pts',(189.391952254306,-4.160357773542,134.861878651407));
#270553=CARTESIAN_POINT('Ctrl Pts',(189.113504630493,1.16492983776554,136.497775047581));
#270554=CARTESIAN_POINT('Ctrl Pts',(188.83505700668,5.41970383815296,132.901701721328));
#270555=CARTESIAN_POINT('Ctrl Pts',(188.556609382867,4.69403477852959,127.378274381527));
#270556=CARTESIAN_POINT('Ctrl Pts',(188.278161759054,-0.345222926215044,
125.003252919028));
#270557=CARTESIAN_POINT('Ctrl Pts',(187.999714135242,-5.0672376268456,127.959166031618));
#270558=CARTESIAN_POINT('Ctrl Pts',(187.721266511429,-5.13270849672517,
133.529673973213));
#270559=CARTESIAN_POINT('Ctrl Pts',(187.442818887616,-0.48147100486422,
136.595752079925));
#270560=CARTESIAN_POINT('Ctrl Pts',(187.164371263803,4.61221481930072,134.339824357932));
#270561=CARTESIAN_POINT('Ctrl Pts',(186.88592363999,5.4675005437485,128.834978175547));
#270562=CARTESIAN_POINT('Ctrl Pts',(186.607476016177,1.29842037074208,125.139898247696));
#270563=CARTESIAN_POINT('Ctrl Pts',(186.329028392364,-4.06384469161484,
126.650182513385));
#270564=CARTESIAN_POINT('Ctrl Pts',(186.050580768551,-5.69163501222784,
131.977953513933));
#270565=CARTESIAN_POINT('Ctrl Pts',(185.772133144738,-2.08909080843167,
136.227249975919));
#270566=CARTESIAN_POINT('Ctrl Pts',(185.493685520926,3.4332257905535,135.493176040453));
#270567=CARTESIAN_POINT('Ctrl Pts',(185.215237897112,5.80057561042411,130.450309792719));
#270568=CARTESIAN_POINT('Ctrl Pts',(184.9367902733,2.83747981818726,125.732798956676));
#270569=CARTESIAN_POINT('Ctrl Pts',(184.658342649487,-2.73312130836828,
125.675805527429));
#270570=CARTESIAN_POINT('Ctrl Pts',(184.379895025674,-5.79211747293216,
130.331703682172));
#270571=CARTESIAN_POINT('Ctrl Pts',(184.101447401861,-3.52844064054064,
135.421950469967));
#270572=CARTESIAN_POINT('Ctrl Pts',(183.822999778048,1.97770076659953,136.26885776521));
#270573=CARTESIAN_POINT('Ctrl Pts',(183.544552154236,5.66643178528845,132.094159137294));
#270574=CARTESIAN_POINT('Ctrl Pts',(183.266104530422,4.14798881387936,126.734198679909));
#270575=CARTESIAN_POINT('Ctrl Pts',(182.98765690661,-1.18225323696583,125.114518204765));
#270576=CARTESIAN_POINT('Ctrl Pts',(182.709209282797,-5.42606231932092,
128.72352494273));
#270577=CARTESIAN_POINT('Ctrl Pts',(182.430761658984,-4.68358520810093,
134.244718011395));
#270578=CARTESIAN_POINT('Ctrl Pts',(182.152314035171,0.362877903506298,
136.604390705933));
#270579=CARTESIAN_POINT('Ctrl Pts',(181.873866411358,5.07587394936235,133.634119096483));
#270580=CARTESIAN_POINT('Ctrl Pts',(181.595418787545,5.12438980598236,128.063437686296));
#270581=CARTESIAN_POINT('Ctrl Pts',(181.316971163732,0.463841771263853,
125.011530548415));
#270582=CARTESIAN_POINT('Ctrl Pts',(181.038523539919,-4.62295419131585,
127.282951248603));
#270583=CARTESIAN_POINT('Ctrl Pts',(180.760075916106,-5.46148109594396,
132.790375128456));
#270584=CARTESIAN_POINT('Ctrl Pts',(180.481628292294,-1.2811736815839,136.472748695004));
#270585=CARTESIAN_POINT('Ctrl Pts',(180.203180668481,4.07646975733793,134.946150534538));
#270586=CARTESIAN_POINT('Ctrl Pts',(179.924733044668,5.68803663588505,129.61344977806));
#270587=CARTESIAN_POINT('Ctrl Pts',(179.646285420855,2.07257572209157,125.37513790386));
#270588=CARTESIAN_POINT('Ctrl Pts',(179.367837797042,-3.44748102935117,
126.12601647128));
#270589=CARTESIAN_POINT('Ctrl Pts',(179.089390173229,-5.79947113363144,
131.176064759319));
#270590=CARTESIAN_POINT('Ctrl Pts',(178.810942549416,-2.82203058602,135.884535099843));
#270591=CARTESIAN_POINT('Ctrl Pts',(178.532494925603,2.74871820628535,135.924573271475));
#270592=CARTESIAN_POINT('Ctrl Pts',(178.254047301791,5.79352924936408,131.259386150458));
#270593=CARTESIAN_POINT('Ctrl Pts',(177.975599677977,3.51436994191561,126.176052793945));
#270594=CARTESIAN_POINT('Ctrl Pts',(177.697152054165,-1.99432365563702,
125.345908221933));
#270595=CARTESIAN_POINT('Ctrl Pts',(177.418704430351,-5.6703312417861,129.531814741282));
#270596=CARTESIAN_POINT('Ctrl Pts',(177.140256806539,-4.135581427815,134.887128753614));
#270597=CARTESIAN_POINT('Ctrl Pts',(176.861809182726,1.19956568393359,136.490578303229));
#270598=CARTESIAN_POINT('Ctrl Pts',(176.583361558913,5.43237053418876,132.868671586896));
#270599=CARTESIAN_POINT('Ctrl Pts',(176.3049139351,4.67309224957875,127.349763936946));
#270600=CARTESIAN_POINT('Ctrl Pts',(176.026466311287,-0.380529519146142,
125.005461870054));
#270601=CARTESIAN_POINT('Ctrl Pts',(175.748018687475,-5.08446324967622,
127.990064460173));
#270602=CARTESIAN_POINT('Ctrl Pts',(175.469571063661,-5.11602364359241,
133.560867732924));
#270603=CARTESIAN_POINT('Ctrl Pts',(175.191123439849,-0.446208240696769,
136.59857562952));
#270604=CARTESIAN_POINT('Ctrl Pts',(174.912675816035,4.63365073691483,134.311682993269));
#270605=CARTESIAN_POINT('Ctrl Pts',(174.634228192223,5.45541105372469,128.801732435971));
#270606=CARTESIAN_POINT('Ctrl Pts',(174.35578056841,1.26391512380778,125.132099343732));
#270607=CARTESIAN_POINT('Ctrl Pts',(174.077332944597,-4.089057059202,126.674997256779));
#270608=CARTESIAN_POINT('Ctrl Pts',(173.798885320784,-5.68438556634791,
132.012578367773));
#270609=CARTESIAN_POINT('Ctrl Pts',(173.520437696972,-2.0560414356932,136.239866391045));
#270610=CARTESIAN_POINT('Ctrl Pts',(173.241990073158,3.46170433115548,135.472190147709));
#270611=CARTESIAN_POINT('Ctrl Pts',(172.963542449346,5.79831293133042,130.41500660232));
#270612=CARTESIAN_POINT('Ctrl Pts',(172.685094825533,2.80655521094699,125.715620375941));
#270613=CARTESIAN_POINT('Ctrl Pts',(172.40664720172,-2.76428964045241,125.692537832834));
#270614=CARTESIAN_POINT('Ctrl Pts',(172.128199577907,-5.79488735533246,
130.366970702468));
#270615=CARTESIAN_POINT('Ctrl Pts',(171.849751954094,-3.50026668664755,
135.443343536393));
#270616=CARTESIAN_POINT('Ctrl Pts',(171.571304330281,2.01092806953244,136.256717694829));
#270617=CARTESIAN_POINT('Ctrl Pts',(171.292856706468,5.6741781691098,132.059642061713));
#270618=CARTESIAN_POINT('Ctrl Pts',(171.014409082656,4.12313573028927,126.709024105332));
#270619=CARTESIAN_POINT('Ctrl Pts',(170.735961458842,-1.21686701828875,
125.121820335384));
#270620=CARTESIAN_POINT('Ctrl Pts',(170.45751383503,-5.43862842431808,128.756593477234));
#270621=CARTESIAN_POINT('Ctrl Pts',(170.179066211217,-4.66255600016836,
134.273164582064));
#270622=CARTESIAN_POINT('Ctrl Pts',(169.900618587404,0.398177609612544,
136.602074304013));
#270623=CARTESIAN_POINT('Ctrl Pts',(169.62217096359,5.09300544821711,133.603168382178));
#270624=CARTESIAN_POINT('Ctrl Pts',(169.343723339778,5.10761008705837,128.032294854024));
#270625=CARTESIAN_POINT('Ctrl Pts',(169.065275715965,0.428570576517446,
125.008814339624));
#270626=CARTESIAN_POINT('Ctrl Pts',(168.786828092152,-4.64430435700642,
127.311157726477));
#270627=CARTESIAN_POINT('Ctrl Pts',(168.508380468339,-5.4492904733226,132.823583917792));
#270628=CARTESIAN_POINT('Ctrl Pts',(168.229932844526,-1.24664485729461,
136.480442540741));
#270629=CARTESIAN_POINT('Ctrl Pts',(167.951485220714,4.10160648060013,134.92125916831));
#270630=CARTESIAN_POINT('Ctrl Pts',(167.673037596901,5.6806818374394,129.578847149419));
#270631=CARTESIAN_POINT('Ctrl Pts',(167.394589973088,2.03948810240773,125.362622138095));
#270632=CARTESIAN_POINT('Ctrl Pts',(167.116142349275,-3.47589556420378,
126.147088945699));
#270633=CARTESIAN_POINT('Ctrl Pts',(166.837694725462,-5.79710101425052,
131.21136089938));
#270634=CARTESIAN_POINT('Ctrl Pts',(166.559247101649,-2.79105383632985,
135.901619477142));
#270635=CARTESIAN_POINT('Ctrl Pts',(166.280799477836,2.77983546661788,135.907746177893));
#270636=CARTESIAN_POINT('Ctrl Pts',(166.002351854023,5.79619177825601,131.224110862948));
#270637=CARTESIAN_POINT('Ctrl Pts',(165.72390423021,3.48613100538707,126.154745578436));
#270638=CARTESIAN_POINT('Ctrl Pts',(165.445456606397,-2.02751385446508,
125.358149368562));
#270639=CARTESIAN_POINT('Ctrl Pts',(165.167008982585,-5.67797253162207,
129.566355234311));
#270640=CARTESIAN_POINT('Ctrl Pts',(164.888561358772,-4.11065183659732,
134.912227567346));
#270641=CARTESIAN_POINT('Ctrl Pts',(164.610113734959,1.23415707975413,136.483170853989));
#270642=CARTESIAN_POINT('Ctrl Pts',(164.331666111146,5.44483593173667,132.835564958663));
#270643=CARTESIAN_POINT('Ctrl Pts',(164.053218487333,4.65197655747607,127.321381503715));
#270644=CARTESIAN_POINT('Ctrl Pts',(163.77477086352,-0.415822011415935,
125.007885701408));
#270645=CARTESIAN_POINT('Ctrl Pts',(163.496323239708,-5.10150046585131,
128.021067173507));
#270646=CARTESIAN_POINT('Ctrl Pts',(163.217875615894,-5.09914921432216,
133.591959349252));
#270647=CARTESIAN_POINT('Ctrl Pts',(162.939427992082,-0.41092894211879,
136.601184472346));
#270648=CARTESIAN_POINT('Ctrl Pts',(162.660980368268,4.65491495289691,134.283411663486));
#270649=CARTESIAN_POINT('Ctrl Pts',(162.382532744456,5.443119411438,128.768560904517));
#270650=CARTESIAN_POINT('Ctrl Pts',(162.104085120643,1.22936304203373,125.124510627495));
#270651=CARTESIAN_POINT('Ctrl Pts',(161.82563749683,-4.11411790527609,126.69996501525));
#270652=CARTESIAN_POINT('Ctrl Pts',(161.547189873017,-5.67692548347038,
132.04715845066));
#270653=CARTESIAN_POINT('Ctrl Pts',(161.268742249204,-2.02291587558315,
136.252281391507));
#270654=CARTESIAN_POINT('Ctrl Pts',(160.990294625391,3.49005459703047,135.451031286826));
#270655=CARTESIAN_POINT('Ctrl Pts',(160.711847001578,5.79583539361873,130.379717839577));
#270656=CARTESIAN_POINT('Ctrl Pts',(160.433399377766,2.77552660577121,125.698630360346));
#270657=CARTESIAN_POINT('Ctrl Pts',(160.154951753952,-2.79535554076737,
125.70945955871));
#270658=CARTESIAN_POINT('Ctrl Pts',(159.87650413014,-5.79744250605075,130.402253930408));
#270659=CARTESIAN_POINT('Ctrl Pts',(159.598056506327,-3.47196302908515,
135.4645647036));
#270660=CARTESIAN_POINT('Ctrl Pts',(159.319608882514,2.04408085678626,136.244375585352));
#270661=CARTESIAN_POINT('Ctrl Pts',(159.041161258701,5.68171429417248,132.025078471215));
#270662=CARTESIAN_POINT('Ctrl Pts',(158.762713634888,4.09812986238831,126.684001284956));
#270663=CARTESIAN_POINT('Ctrl Pts',(158.484266011075,-1.25143570815684,
125.129333034622));
#270664=CARTESIAN_POINT('Ctrl Pts',(158.205818387262,-5.450992998939,128.789737892503));
#270665=CARTESIAN_POINT('Ctrl Pts',(157.927370763449,-4.64135401950845,
134.301482614925));
#270666=CARTESIAN_POINT('Ctrl Pts',(157.648923139637,0.43346256110109,136.59954306568));
#270667=CARTESIAN_POINT('Ctrl Pts',(157.370475515823,5.10994822388206,133.572113957021));
#270668=CARTESIAN_POINT('Ctrl Pts',(157.092027892011,5.09064110376424,128.001254741669));
#270669=CARTESIAN_POINT('Ctrl Pts',(156.813580268198,0.39328350093061,125.006312886931));
#270670=CARTESIAN_POINT('Ctrl Pts',(156.535132644385,-4.66548242629113,
127.339493646268));
#270671=CARTESIAN_POINT('Ctrl Pts',(156.256685020572,-5.43689792523874,
132.856717884066));
#270672=CARTESIAN_POINT('Ctrl Pts',(155.978237396759,-1.21206983812162,
136.487926057176));
#270673=CARTESIAN_POINT('Ctrl Pts',(155.699789772946,4.12659121732586,134.896215248893));
#270674=CARTESIAN_POINT('Ctrl Pts',(155.421342149133,5.67311653923917,129.544289932631));
#270675=CARTESIAN_POINT('Ctrl Pts',(155.142894525321,2.0063249087422,125.350308017949));
#270676=CARTESIAN_POINT('Ctrl Pts',(154.864446901507,-3.50418129846815,
126.168333997033));
#270677=CARTESIAN_POINT('Ctrl Pts',(154.585999277695,-5.79451608115961,
131.246641957895));
#270678=CARTESIAN_POINT('Ctrl Pts',(154.307551653882,-2.75997366311328,
135.918514973638));
#270679=CARTESIAN_POINT('Ctrl Pts',(154.029104030069,2.81084971912495,135.890729976482));
#270680=CARTESIAN_POINT('Ctrl Pts',(153.750656406256,5.79863952713012,131.188820021437));
#270681=CARTESIAN_POINT('Ctrl Pts',(153.472208782443,3.457762888992,126.133610656121));
#270682=CARTESIAN_POINT('Ctrl Pts',(153.19376115863,-2.0606289230217,125.370592326552));
#270683=CARTESIAN_POINT('Ctrl Pts',(152.915313534817,-5.68540342209783,
129.600941602086));
#270684=CARTESIAN_POINT('Ctrl Pts',(152.636865911004,-4.08556992366409,
134.937174162558));
#270685=CARTESIAN_POINT('Ctrl Pts',(152.358418287191,1.26870274343019,136.475552974349));
#270686=CARTESIAN_POINT('Ctrl Pts',(152.079970663379,5.45709956888678,132.802383063404));
#270687=CARTESIAN_POINT('Ctrl Pts',(151.801523039566,4.63068848467127,127.293128133558));
#270688=CARTESIAN_POINT('Ctrl Pts',(151.523075415753,-0.451099095248245,
125.010524323271));
#270689=CARTESIAN_POINT('Ctrl Pts',(151.24462779194,-5.11834864405056,128.052173022803));
#270690=CARTESIAN_POINT('Ctrl Pts',(150.966180168127,-5.08208583420252,
133.622947670083));
#270691=CARTESIAN_POINT('Ctrl Pts',(150.687732544314,-0.375634416417742,
136.603578511732));
#270692=CARTESIAN_POINT('Ctrl Pts',(150.409284920501,4.67600667929353,134.255011416186));
#270693=CARTESIAN_POINT('Ctrl Pts',(150.130837296688,5.43062607235983,128.735464810371));
#270694=CARTESIAN_POINT('Ctrl Pts',(149.852389672876,1.19476540576009,125.117132380189));
#270695=CARTESIAN_POINT('Ctrl Pts',(149.573942049063,-4.13902630119825,
126.725084863609));
#270696=CARTESIAN_POINT('Ctrl Pts',(149.29549442525,-5.66925504003138,132.081692481218));
#270697=CARTESIAN_POINT('Ctrl Pts',(149.017046801437,-1.98971535558138,
136.264494517259));
#270698=CARTESIAN_POINT('Ctrl Pts',(148.738599177624,3.5182755376489,135.429700241853));
#270699=CARTESIAN_POINT('Ctrl Pts',(148.460151553811,5.79314308909515,130.344444812129));
#270700=CARTESIAN_POINT('Ctrl Pts',(148.181703929998,2.74439515243632,125.681829539465));
#270701=CARTESIAN_POINT('Ctrl Pts',(147.903256306185,-2.82631785815477,
125.726570078021));
#270702=CARTESIAN_POINT('Ctrl Pts',(147.624808682372,-5.79978283040501,
130.437552058559));
#270703=CARTESIAN_POINT('Ctrl Pts',(147.346361058559,-3.4435307166558,135.48561318523));
#270704=CARTESIAN_POINT('Ctrl Pts',(147.067913434747,2.07715789987228,136.23183189412));
#270705=CARTESIAN_POINT('Ctrl Pts',(146.789465810933,5.68903988122249,131.990469646568));
#270706=CARTESIAN_POINT('Ctrl Pts',(146.511018187121,4.07297213677825,126.65913114601));
#270707=CARTESIAN_POINT('Ctrl Pts',(146.232570563308,-1.2859580256146,125.137056024094));
#270708=CARTESIAN_POINT('Ctrl Pts',(145.954122939495,-5.46315558500969,
128.822956960357));
#270709=CARTESIAN_POINT('Ctrl Pts',(145.675675315682,-4.61998005176852,
134.329671060644));
#270710=CARTESIAN_POINT('Ctrl Pts',(145.397227691869,0.468731450475054,
136.596797084732));
#270711=CARTESIAN_POINT('Ctrl Pts',(145.118780068056,5.12670164853643,133.540956971746));
#270712=CARTESIAN_POINT('Ctrl Pts',(144.840332444244,5.07348348489189,127.970318499433));
#270713=CARTESIAN_POINT('Ctrl Pts',(144.56188482043,0.357981852079004,125.004026283029));
#270714=CARTESIAN_POINT('Ctrl Pts',(144.283437196618,-4.6864876144088,127.367957957979));
#270715=CARTESIAN_POINT('Ctrl Pts',(144.004989572805,-5.42430391090288,
132.889775799486));
#270716=CARTESIAN_POINT('Ctrl Pts',(143.726541948992,-1.17744990525502,
136.495198967004));
#270717=CARTESIAN_POINT('Ctrl Pts',(143.448094325179,4.15142304169647,134.871019704297));
#270718=CARTESIAN_POINT('Ctrl Pts',(143.169646701366,5.66534102161933,129.509779408224));
#270719=CARTESIAN_POINT('Ctrl Pts',(142.891199077553,1.9730873699693,125.338195999729));
#270720=CARTESIAN_POINT('Ctrl Pts',(142.61275145374,-3.53233718400576,126.189750838038));
#270721=CARTESIAN_POINT('Ctrl Pts',(142.334303829928,-5.79171643014443,
131.281906627513));
#270722=CARTESIAN_POINT('Ctrl Pts',(142.055856206114,-2.72879121805762,
135.935220963265));
#270723=CARTESIAN_POINT('Ctrl Pts',(141.777408582302,2.84175981456215,135.873525297782));
#270724=CARTESIAN_POINT('Ctrl Pts',(141.498960958489,5.80087240528401,131.153514933643));
#270725=CARTESIAN_POINT('Ctrl Pts',(141.220513334676,3.42926664392146,126.112648810165));
#270726=CARTESIAN_POINT('Ctrl Pts',(140.942065710863,-2.09366763421581,
125.383236634823));
#270727=CARTESIAN_POINT('Ctrl Pts',(140.66361808705,-5.69262363785895,129.635572562993));
#270728=CARTESIAN_POINT('Ctrl Pts',(140.385170463237,-4.06033661843482,
134.961967614844));
#270729=CARTESIAN_POINT('Ctrl Pts',(140.106722839424,1.30320139485961,136.467724946589));
#270730=CARTESIAN_POINT('Ctrl Pts',(139.828275215611,5.46916099120554,132.769127130691));
#270731=CARTESIAN_POINT('Ctrl Pts',(139.549827591798,4.60922882000175,127.26500487341));
#270732=CARTESIAN_POINT('Ctrl Pts',(139.271379967986,-0.486359463437733,
125.013377637868));
#270733=CARTESIAN_POINT('Ctrl Pts',(138.992932344173,-5.13500715995863,
128.083380855422));
#270734=CARTESIAN_POINT('Ctrl Pts',(138.71448472036,-5.06483413552331,133.653831547135));
#270735=CARTESIAN_POINT('Ctrl Pts',(138.436037096547,-0.340325971445257,
136.605757658967));
#270736=CARTESIAN_POINT('Ctrl Pts',(138.157589472734,4.69692513454305,134.226483303753));
#270737=CARTESIAN_POINT('Ctrl Pts',(137.879141848921,5.41793149943546,128.70244537992));
#270738=CARTESIAN_POINT('Ctrl Pts',(137.600694225109,1.16012349701482,125.109964875215));
#270739=CARTESIAN_POINT('Ctrl Pts',(137.322246601295,-4.16378132397874,
126.750355871033));
#270740=CARTESIAN_POINT('Ctrl Pts',(137.043798977483,-5.66137452026194,
132.116179179772));
#270741=CARTESIAN_POINT('Ctrl Pts',(136.765351353669,-1.95644110594549,
136.276505315742));
#270742=CARTESIAN_POINT('Ctrl Pts',(136.486903729857,3.54636610727348,135.408197803219));
#270743=CARTESIAN_POINT('Ctrl Pts',(136.208456106044,5.79023611752392,130.309188827029));
#270744=CARTESIAN_POINT('Ctrl Pts',(135.930008482231,2.71316200452982,125.665218535856));
#270745=CARTESIAN_POINT('Ctrl Pts',(135.651560858418,-2.85717544529452,
125.743868756725));
#270746=CARTESIAN_POINT('Ctrl Pts',(135.373113234605,-5.80190824167357,
130.472863778936));
#270747=CARTESIAN_POINT('Ctrl Pts',(135.094665610792,-3.41497080292952,
135.506488201326));
#270748=CARTESIAN_POINT('Ctrl Pts',(134.816217986979,2.11015797310843,136.219087085943));
#270749=CARTESIAN_POINT('Ctrl Pts',(134.537770363167,5.69615465880763,131.955816870215));
#270750=CARTESIAN_POINT('Ctrl Pts',(134.259322739353,4.04766348568775,126.634414610068));
#270751=CARTESIAN_POINT('Ctrl Pts',(133.980875115541,-1.32043269142476,
125.144989017623));
#270752=CARTESIAN_POINT('Ctrl Pts',(133.702427491728,-5.47511573184112,
128.856249449853));
#270753=CARTESIAN_POINT('Ctrl Pts',(133.423979867915,-4.59843488896879,
134.357728874689));
#270754=CARTESIAN_POINT('Ctrl Pts',(133.145532244102,0.503982970832797,
136.59383646292));
#270755=CARTESIAN_POINT('Ctrl Pts',(132.867084620289,5.14326510137581,133.509698580887));
#270756=CARTESIAN_POINT('Ctrl Pts',(132.588636996476,5.05613786622328,127.93948727367));
#270757=CARTESIAN_POINT('Ctrl Pts',(132.310189372663,0.322666938078297,
125.001954612649));
#270758=CARTESIAN_POINT('Ctrl Pts',(132.03174174885,-4.70731914300451,127.396549606854));
#270759=CARTESIAN_POINT('Ctrl Pts',(131.753294125038,-5.41150889699075,
132.92275643908));
#270760=CARTESIAN_POINT('Ctrl Pts',(131.474846501225,-1.14278634154918,
136.502261000723));
#270761=CARTESIAN_POINT('Ctrl Pts',(131.196398877412,4.17610103355955,134.845673468154));
#270762=CARTESIAN_POINT('Ctrl Pts',(130.917951253599,5.65735557270449,129.475316855001));
#270763=CARTESIAN_POINT('Ctrl Pts',(130.639503629786,1.93977671771839,125.326286532249));
#270764=CARTESIAN_POINT('Ctrl Pts',(130.361056005973,-3.56036217749005,
126.211338675105));
#270765=CARTESIAN_POINT('Ctrl Pts',(130.08260838216,-5.788702164947,131.317153601487));
#270766=CARTESIAN_POINT('Ctrl Pts',(129.804160758347,-2.69750765663984,
135.951736826975));
#270767=CARTESIAN_POINT('Ctrl Pts',(129.525713134534,2.87256460754407,135.856132779323));
#270768=CARTESIAN_POINT('Ctrl Pts',(129.247265510721,5.80289032997773,131.118196907806));
#270769=CARTESIAN_POINT('Ctrl Pts',(128.968817886909,3.40064332611445,126.091860817314));
#270770=CARTESIAN_POINT('Ctrl Pts',(128.690370263096,-2.12662876378584,
125.396081824838));
#270771=CARTESIAN_POINT('Ctrl Pts',(128.411922639283,-5.69963291135762,
129.670246833772));
#270772=CARTESIAN_POINT('Ctrl Pts',(128.13347501547,-4.03495285593914,134.986607005474));
#270773=CARTESIAN_POINT('Ctrl Pts',(127.855027391657,1.33765175568188,136.459687060782));
#270774=CARTESIAN_POINT('Ctrl Pts',(127.576579767844,5.48101975175251,132.73579839283));
#270775=CARTESIAN_POINT('Ctrl Pts',(127.298132144031,4.5875983586632,127.237012765392));
#270776=CARTESIAN_POINT('Ctrl Pts',(127.019684520218,-0.521601809398458,
125.016445539469));
#270777=CARTESIAN_POINT('Ctrl Pts',(126.741236896406,-5.15147539628782,
128.114689514947));
#270778=CARTESIAN_POINT('Ctrl Pts',(126.462789272592,-5.0473947575527,133.684609835992));
#270779=CARTESIAN_POINT('Ctrl Pts',(126.18434164878,-0.305004915568794,
136.607721833301));
#270780=CARTESIAN_POINT('Ctrl Pts',(125.905894024967,4.71766954350447,134.197828383304));
#270781=CARTESIAN_POINT('Ctrl Pts',(125.627446401154,5.40503616306688,128.669503836711));
#270782=CARTESIAN_POINT('Ctrl Pts',(125.348998777341,1.12543859946687,125.10300837817));
#270783=CARTESIAN_POINT('Ctrl Pts',(125.070551153528,-4.18838205631096,
126.775777101093));
#270784=CARTESIAN_POINT('Ctrl Pts',(124.792103529715,-5.65328421617778,
132.150617268407));
#270785=CARTESIAN_POINT('Ctrl Pts',(124.513655905902,-1.9230943596648,136.288313341892));
#270786=CARTESIAN_POINT('Ctrl Pts',(124.23520828209,3.57432526499779,135.386524767704));
#270787=CARTESIAN_POINT('Ctrl Pts',(123.956760658277,5.78711458662396,130.273951190703));
#270788=CARTESIAN_POINT('Ctrl Pts',(123.678313034464,2.68182831940755,125.648797965047));
#270789=CARTESIAN_POINT('Ctrl Pts',(123.399865410651,-2.88792715874745,
125.761354953818));
#270790=CARTESIAN_POINT('Ctrl Pts',(123.121417786838,-5.8038186610986,130.50818778305));
#270791=CARTESIAN_POINT('Ctrl Pts',(122.842970163025,-3.38628434620416,
135.527188978355));
#270792=CARTESIAN_POINT('Ctrl Pts',(122.564522539212,2.1430798536649,136.206141633086));
#270793=CARTESIAN_POINT('Ctrl Pts',(122.286074915399,5.703058363287,131.921121426228));
#270794=CARTESIAN_POINT('Ctrl Pts',(122.007627291586,4.02220484693838,126.609852593007));
#270795=CARTESIAN_POINT('Ctrl Pts',(121.729179667773,-1.35485842811595,
125.153131721247));
#270796=CARTESIAN_POINT('Ctrl Pts',(121.450732043961,-5.48687299624567,
128.889614127324));
#270797=CARTESIAN_POINT('Ctrl Pts',(121.172284420148,-4.57671932947311,
134.385655017367));
#270798=CARTESIAN_POINT('Ctrl Pts',(120.893836796335,0.539215815916097,
136.59066130995));
#270799=CARTESIAN_POINT('Ctrl Pts',(120.615389172522,5.15963796863542,133.478339942736));
#270800=CARTESIAN_POINT('Ctrl Pts',(120.336941548709,5.0386048905067,127.908762206842));
#270801=CARTESIAN_POINT('Ctrl Pts',(120.058493924896,0.287340067535411,
125.000097952557));
#270802=CARTESIAN_POINT('Ctrl Pts',(119.780046301083,-4.72797624015824,
127.42526753342));
#270803=CARTESIAN_POINT('Ctrl Pts',(119.50159867727,-5.39851335762638,132.955658580739));
#270804=CARTESIAN_POINT('Ctrl Pts',(119.223151053457,-1.10808043147514,
136.509111896649));
#270805=CARTESIAN_POINT('Ctrl Pts',(118.944703429644,4.20062427846316,134.820177479675));
#270806=CARTESIAN_POINT('Ctrl Pts',(118.666255805832,5.64916048839838,129.440903549983));
#270807=CARTESIAN_POINT('Ctrl Pts',(118.387808182019,1.90639418632776,125.314580056818));
#270808=CARTESIAN_POINT('Ctrl Pts',(118.109360558206,-3.58825524044456,
126.23309670829));
#270809=CARTESIAN_POINT('Ctrl Pts',(117.830912934393,-5.785473397262,131.352381573729));
#270810=CARTESIAN_POINT('Ctrl Pts',(117.55246531058,-2.66612413808396,135.968061952766));
#270811=CARTESIAN_POINT('Ctrl Pts',(117.274017686767,2.9032629565882,135.838553065588));
#270812=CARTESIAN_POINT('Ctrl Pts',(116.995570062954,5.80469322643624,131.082867252651));
#270813=CARTESIAN_POINT('Ctrl Pts',(116.717122439142,3.37189399621826,126.071247447876));
#270814=CARTESIAN_POINT('Ctrl Pts',(116.438674815328,-2.15951109034483,
125.409127420613));
#270815=CARTESIAN_POINT('Ctrl Pts',(116.160227191516,-5.70643098286277,
129.704963129555));
#270816=CARTESIAN_POINT('Ctrl Pts',(115.881779567703,-4.00941957678149,
135.011091421425));
#270817=CARTESIAN_POINT('Ctrl Pts',(115.60333194389,1.37205254932662,136.451439614773));
#270818=CARTESIAN_POINT('Ctrl Pts',(115.324884320077,5.49267541109693,132.702398084833));
#270819=CARTESIAN_POINT('Ctrl Pts',(115.046436696264,4.56579790218037,127.20915284676));
#270820=CARTESIAN_POINT('Ctrl Pts',(114.767989072451,-0.556824827212187,
125.019727914392));
#270821=CARTESIAN_POINT('Ctrl Pts',(114.489541448638,-5.1677527428018,128.146097841224));
#270822=CARTESIAN_POINT('Ctrl Pts',(114.211093824825,-5.02976834651319,
133.715281396157));
#270823=CARTESIAN_POINT('Ctrl Pts',(113.932646201012,-0.269672557622912,
136.60947096195));
#270824=CARTESIAN_POINT('Ctrl Pts',(113.6541985772,4.73823913748602,134.169047716661));
#270825=CARTESIAN_POINT('Ctrl Pts',(113.375750953387,5.39194054109557,128.636641401405));
#270826=CARTESIAN_POINT('Ctrl Pts',(113.097303329574,1.09071199837779,125.09626314683));
#270827=CARTESIAN_POINT('Ctrl Pts',(112.818855705761,-4.21282758660586,
126.801347611796));
#270828=CARTESIAN_POINT('Ctrl Pts',(112.540408081948,-5.64498442756793,
132.185005471008));
#270829=CARTESIAN_POINT('Ctrl Pts',(112.261960458135,-1.8896763524154,136.299918158156));
#270830=CARTESIAN_POINT('Ctrl Pts',(111.983512834322,3.60215197478495,135.364681938413));
#270831=CARTESIAN_POINT('Ctrl Pts',(111.705065210509,5.78377861206482,130.238733208892));
#270832=CARTESIAN_POINT('Ctrl Pts',(111.426617586696,2.65039525815055,125.632568435507));
#270833=CARTESIAN_POINT('Ctrl Pts',(111.148169962883,-2.91857185899754,
125.77902802134));
#270834=CARTESIAN_POINT('Ctrl Pts',(110.869722339071,-5.80551401788879,
130.543522761958));
#270835=CARTESIAN_POINT('Ctrl Pts',(110.591274715258,-3.35747240946702,
135.547714749242));
#270836=CARTESIAN_POINT('Ctrl Pts',(110.312827091445,2.17592232160915,136.192996015246));
#270837=CARTESIAN_POINT('Ctrl Pts',(110.034379467632,5.70975073884148,131.886384600257));
#270838=CARTESIAN_POINT('Ctrl Pts',(109.755931843819,3.99659716390926,126.585446004984));
#270839=CARTESIAN_POINT('Ctrl Pts',(109.477484220006,-1.38923396002991,
125.161483833236));
#270840=CARTESIAN_POINT('Ctrl Pts',(109.199036596193,-5.49842694255352,
128.923049756431));
#270841=CARTESIAN_POINT('Ctrl Pts',(108.92058897238,-4.55483417795961,134.413448453863));
#270842=CARTESIAN_POINT('Ctrl Pts',(108.642141348568,0.57442868015902,136.58727174348));
#270843=CARTESIAN_POINT('Ctrl Pts',(108.363693724754,5.17581964361271,133.446882219296));
#270844=CARTESIAN_POINT('Ctrl Pts',(108.085246100942,5.02088520743284,127.878144437479));
#270845=CARTESIAN_POINT('Ctrl Pts',(107.806798477129,0.252002549500665,
124.998456371553));
#270846=CARTESIAN_POINT('Ctrl Pts',(107.528350853316,-4.74845814041369,
127.454110673523));
#270847=CARTESIAN_POINT('Ctrl Pts',(107.249903229503,-5.38531777436419,
132.988481005259));
#270848=CARTESIAN_POINT('Ctrl Pts',(106.97145560569,-1.07333346107335,136.515751400918));
#270849=CARTESIAN_POINT('Ctrl Pts',(106.693007981877,4.22499186768932,134.794532683627));
#270850=CARTESIAN_POINT('Ctrl Pts',(106.414560358064,5.64075607237289,129.406540768369));
#270851=CARTESIAN_POINT('Ctrl Pts',(106.136112734251,1.87294101279944,125.303077007226));
#270852=CARTESIAN_POINT('Ctrl Pts',(105.857665110439,-3.61601533928142,
126.25502413134));
#270853=CARTESIAN_POINT('Ctrl Pts',(105.579217486626,-5.78203024673271,
131.387589238853));
#270854=CARTESIAN_POINT('Ctrl Pts',(105.300769862813,-2.63464182531766,
135.984195735705));
#270855=CARTESIAN_POINT('Ctrl Pts',(105.022322239,2.93385372415587,135.820786808));
#270856=CARTESIAN_POINT('Ctrl Pts',(104.743874615187,5.80628102785255,131.047527277329));
#270857=CARTESIAN_POINT('Ctrl Pts',(104.465426991374,3.34301971955009,126.050809465687));
#270858=CARTESIAN_POINT('Ctrl Pts',(104.186979367561,-2.19231339542621,
125.422372938737));
#270859=CARTESIAN_POINT('Ctrl Pts',(103.908531743748,-5.71301760046937,
129.739720163916));
#270860=CARTESIAN_POINT('Ctrl Pts',(103.630084119935,-3.98373772710686,
135.03541995542));
#270861=CARTESIAN_POINT('Ctrl Pts',(103.351636496123,1.40640250105958,136.442982914176));
#270862=CARTESIAN_POINT('Ctrl Pts',(103.07318887231,5.50412753733405,132.66892744436));
#270863=CARTESIAN_POINT('Ctrl Pts',(102.794741248497,4.54382825837723,127.181426149873));
#270864=CARTESIAN_POINT('Ctrl Pts',(102.516293624684,-0.592027211677165,
125.023224641008));
#270865=CARTESIAN_POINT('Ctrl Pts',(102.237846000871,-5.18383859633749,
128.177604670405));
#270866=CARTESIAN_POINT('Ctrl Pts',(101.959398377058,-5.01195555555783,
133.745845091081));
#270867=CARTESIAN_POINT('Ctrl Pts',(101.680950753245,-0.234330206861215,
136.611004980102));
#270868=CARTESIAN_POINT('Ctrl Pts',(101.402503129432,4.75863315427373,134.140142370299));
#270869=CARTESIAN_POINT('Ctrl Pts',(101.124055505619,5.37864511878468,128.603859291732));
#270870=CARTESIAN_POINT('Ctrl Pts',(100.845607881807,1.05594498055446,125.089729431141));
#270871=CARTESIAN_POINT('Ctrl Pts',(100.567160257994,-4.23711700902531,
126.827066455619));
#270872=CARTESIAN_POINT('Ctrl Pts',(100.288712634181,-5.63647546198416,
132.219342513305));
#270873=CARTESIAN_POINT('Ctrl Pts',(100.010265010368,-1.85618832251382,
136.311319334515));
#270874=CARTESIAN_POINT('Ctrl Pts',(99.731817386555,3.62984520550588,135.342670124737));
#270875=CARTESIAN_POINT('Ctrl Pts',(99.4533697627421,5.78022831746224,130.203536186614));
#270876=CARTESIAN_POINT('Ctrl Pts',(99.1749221389292,2.61886398552269,125.616530548629));
#270877=CARTESIAN_POINT('Ctrl Pts',(98.8964745151164,-2.9491084104941,125.796887304409));
#270878=CARTESIAN_POINT('Ctrl Pts',(98.6180268913035,-5.80699424922206,
130.578867406308));
#270879=CARTESIAN_POINT('Ctrl Pts',(98.3395792674906,-3.32853606035512,
135.568064753397));
#270880=CARTESIAN_POINT('Ctrl Pts',(98.0611316436778,2.20868415995158,136.179650719541));
#270881=CARTESIAN_POINT('Ctrl Pts',(97.7826840198649,5.71623153748262,131.851607679491));
#270882=CARTESIAN_POINT('Ctrl Pts',(97.5042363960519,3.97084138550236,126.561195750394));
#270883=CARTESIAN_POINT('Ctrl Pts',(97.2257887722391,-1.42355801336861,
125.170045044101));
#270884=CARTESIAN_POINT('Ctrl Pts',(96.9473411484261,-5.50977714262889,
128.956555098203));
#270885=CARTESIAN_POINT('Ctrl Pts',(96.6688935246133,-4.53278024539068,
134.441108154283));
#270886=CARTESIAN_POINT('Ctrl Pts',(96.3904459008004,0.609620258735999,
136.583667889112));
#270887=CARTESIAN_POINT('Ctrl Pts',(96.1119982769875,5.19180952668969,133.415326576248));
#270888=CARTESIAN_POINT('Ctrl Pts',(95.8335506531746,5.00297947361121,127.847635100131));
#270889=CARTESIAN_POINT('Ctrl Pts',(95.5551030293618,0.216655693418756,
124.997029930466));
#270890=CARTESIAN_POINT('Ctrl Pts',(95.2766554055487,-4.7687640848064,127.483077958369));
#270891=CARTESIAN_POINT('Ctrl Pts',(94.9982077817361,-5.37192263617151,
133.021222496396));
#270892=CARTESIAN_POINT('Ctrl Pts',(94.7197601579228,-1.03854671790542,
136.522179267501));
#270893=CARTESIAN_POINT('Ctrl Pts',(94.4413125341102,4.24920289828813,134.768740030285));
#270894=CARTESIAN_POINT('Ctrl Pts',(94.1628649102971,5.63214263605674,129.372229783482));
#270895=CARTESIAN_POINT('Ctrl Pts',(93.8844172864844,1.83941843675322,125.29177780972));
#270896=CARTESIAN_POINT('Ctrl Pts',(93.6059696626714,-3.6436414453401,126.277120131727));
#270897=CARTESIAN_POINT('Ctrl Pts',(93.3275220388585,-5.77837284094635,
131.422775292226));
#270898=CARTESIAN_POINT('Ctrl Pts',(93.0490744150458,-2.60306188492951,
136.000137577949));
#270899=CARTESIAN_POINT('Ctrl Pts',(92.7706267912327,2.96433577669487,135.802834664895));
#270900=CARTESIAN_POINT('Ctrl Pts',(92.49217916742,5.80765367539012,131.012178291378));
#270901=CARTESIAN_POINT('Ctrl Pts',(92.213731543607,3.31402156605677,126.030547628085));
#270902=CARTESIAN_POINT('Ctrl Pts',(91.9352839197941,-2.22503446352861,
125.435817888395));
#270903=CARTESIAN_POINT('Ctrl Pts',(91.6568362959812,-5.71939252010779,
129.77451664892));
#270904=CARTESIAN_POINT('Ctrl Pts',(91.3783886721684,-3.95790825856573,
135.059591705955));
#270905=CARTESIAN_POINT('Ctrl Pts',(91.0999410483554,1.44070033803066,136.434317272356));
#270906=CARTESIAN_POINT('Ctrl Pts',(90.8214934245425,5.51537570610103,132.635387711677));
#270907=CARTESIAN_POINT('Ctrl Pts',(90.5430458007297,4.52169024134706,127.153833702157));
#270908=CARTESIAN_POINT('Ctrl Pts',(90.2645981769166,-0.627207658356129,
125.026935589742));
#270909=CARTESIAN_POINT('Ctrl Pts',(89.9861505531037,-5.19973236082766,
128.209208834995));
#270910=CARTESIAN_POINT('Ctrl Pts',(89.707702929291,-4.99395704474619,133.776299788217));
#270911=CARTESIAN_POINT('Ctrl Pts',(89.4292553054779,-0.198979172907652,
136.61232383091));
#270912=CARTESIAN_POINT('Ctrl Pts',(89.1508076816652,4.77885083815996,134.111113415317));
#270913=CARTESIAN_POINT('Ctrl Pts',(88.8723600578521,5.36515038880097,128.571158722445));
#270914=CARTESIAN_POINT('Ctrl Pts',(88.5939124340396,1.02113883430145,125.08340747321));
#270915=CARTESIAN_POINT('Ctrl Pts',(88.3154648102263,-4.26124942351577,
126.85293267954));
#270916=CARTESIAN_POINT('Ctrl Pts',(88.0370171864138,-5.62775763472933,
132.253627122929));
#270917=CARTESIAN_POINT('Ctrl Pts',(87.7585695626006,-1.82263151087143,
136.322516448493));
#270918=CARTESIAN_POINT('Ctrl Pts',(87.480121938788,3.65740393097785,135.320490142334));
#270919=CARTESIAN_POINT('Ctrl Pts',(87.2016743149749,5.77646383437373,130.168361428106));
#270920=CARTESIAN_POINT('Ctrl Pts',(86.9232266911622,2.58723566992664,125.600684898703));
#270921=CARTESIAN_POINT('Ctrl Pts',(86.6447790673492,-2.97953568169397,
125.814932141244));
#270922=CARTESIAN_POINT('Ctrl Pts',(86.3663314435363,-5.80825930024783,
130.614220406392));
#270923=CARTESIAN_POINT('Ctrl Pts',(86.0878838197235,-3.29947637111547,
135.588238236744));
#270924=CARTESIAN_POINT('Ctrl Pts',(85.8094361959104,2.24136415469026,136.166106240484));
#270925=CARTESIAN_POINT('Ctrl Pts',(85.5309885720977,5.72250051906197,131.816791952599));
#270926=CARTESIAN_POINT('Ctrl Pts',(85.2525409482847,3.94493846610766,126.537102727838));
#270927=CARTESIAN_POINT('Ctrl Pts',(84.9740933244718,-1.45782931624159,
125.178815036599));
#270928=CARTESIAN_POINT('Ctrl Pts',(84.6956457006588,-5.52092317588609,
128.990128911089));
#270929=CARTESIAN_POINT('Ctrl Pts',(84.417198076846,-4.51055834898274,134.468633093685));
#270930=CARTESIAN_POINT('Ctrl Pts',(84.138750453033,0.644789247610192,136.579849880389));
#270931=CARTESIAN_POINT('Ctrl Pts',(83.8603028292202,5.20760702535536,133.383674182895));
#270932=CARTESIAN_POINT('Ctrl Pts',(83.5818552054073,4.98488835254533,127.817235325336));
#270933=CARTESIAN_POINT('Ctrl Pts',(83.3034075815944,0.181300809080568,
124.995818682153));
#270934=CARTESIAN_POINT('Ctrl Pts',(83.0249599577814,-4.78889332089225,
127.512168314565));
#270935=CARTESIAN_POINT('Ctrl Pts',(82.7465123339688,-5.35832843941005,
133.053881840899));
#270936=CARTESIAN_POINT('Ctrl Pts',(82.4680647101557,-1.00372149100682,
136.528395258211));
#270937=CARTESIAN_POINT('Ctrl Pts',(82.1896170863428,4.27325647311088,134.742800475408));
#270938=CARTESIAN_POINT('Ctrl Pts',(81.91116946253,5.62332049862395,129.337971866731));
#270939=CARTESIAN_POINT('Ctrl Pts',(81.632721838717,1.80582770038043,125.280682882997));
#270940=CARTESIAN_POINT('Ctrl Pts',(81.3542742149043,-3.67113253492515,
126.299383890674));
#270941=CARTESIAN_POINT('Ctrl Pts',(81.0758265910913,-5.77450131542928,
131.457938430015));
#270942=CARTESIAN_POINT('Ctrl Pts',(80.7973789672785,-2.57138548712596,
136.015886888767));
#270943=CARTESIAN_POINT('Ctrl Pts',(80.5189313434656,2.99470798468153,135.784697301496));
#270944=CARTESIAN_POINT('Ctrl Pts',(80.2404837196526,5.80881111818491,130.976821604667));
#270945=CARTESIAN_POINT('Ctrl Pts',(79.9620360958398,3.2849006102757,126.010462685879));
#270946=CARTESIAN_POINT('Ctrl Pts',(79.6835884720269,-2.25767308216064,
125.449461771377));
#270947=CARTESIAN_POINT('Ctrl Pts',(79.4051408482139,-5.72555550555307,
129.809351295171));
#270948=CARTESIAN_POINT('Ctrl Pts',(79.1266932244012,-3.93193212827854,
135.083605777338));
#270949=CARTESIAN_POINT('Ctrl Pts',(78.8482456005881,1.47494478932078,136.425443010422));
#270950=CARTESIAN_POINT('Ctrl Pts',(78.5697979767754,5.526419500593,132.601780129612));
#270951=CARTESIAN_POINT('Ctrl Pts',(78.2913503529625,4.49938467142216,127.126376526057));
#270952=CARTESIAN_POINT('Ctrl Pts',(78.0129027291494,-0.662364863624755,
125.030860623086));
#270953=CARTESIAN_POINT('Ctrl Pts',(77.7344551053368,-5.21543344732299,
128.240909163888));
#270954=CARTESIAN_POINT('Ctrl Pts',(77.4560074815235,-4.97577348101974,
133.806644359053));
#270955=CARTESIAN_POINT('Ctrl Pts',(77.1775598577108,-0.163620765707691,
136.613427465507));
#270956=CARTESIAN_POINT('Ctrl Pts',(76.8991122338979,4.79889143997102,134.081961927395));
#270957=CARTESIAN_POINT('Ctrl Pts',(76.620664610085,5.35145685119646,128.538540905275));
#270958=CARTESIAN_POINT('Ctrl Pts',(76.3422169862721,0.986294849373407,
125.077297507303));
#270959=CARTESIAN_POINT('Ctrl Pts',(76.0637693624593,-4.28522393584178,
126.878945325076));
#270960=CARTESIAN_POINT('Ctrl Pts',(75.7853217386464,-5.61883126884571,
132.287858029448));
#270961=CARTESIAN_POINT('Ctrl Pts',(75.5068741148335,-1.78900716094817,
136.333509085178));
#270962=CARTESIAN_POINT('Ctrl Pts',(75.2284264910206,3.68482713000219,135.298142813091));
#270963=CARTESIAN_POINT('Ctrl Pts',(74.9499788672077,5.77248530229349,130.133210236781));
#270964=CARTESIAN_POINT('Ctrl Pts',(74.6715312433948,2.55551148336137,125.585032072894));
#270965=CARTESIAN_POINT('Ctrl Pts',(74.3930836195819,-3.0098525451033,125.833161863185));
#270966=CARTESIAN_POINT('Ctrl Pts',(74.1146359957691,-5.80930912408932,
130.649580452192));
#270967=CARTESIAN_POINT('Ctrl Pts',(73.8361883719562,-3.27029441856551,
135.608234451746));
#270968=CARTESIAN_POINT('Ctrl Pts',(73.5577407481433,2.273961094856,136.152363079971));
#270969=CARTESIAN_POINT('Ctrl Pts',(73.2792931243304,5.72855745128013,131.781938709691));
#270970=CARTESIAN_POINT('Ctrl Pts',(73.0008455005175,3.91888936556733,126.513167830092));
#270971=CARTESIAN_POINT('Ctrl Pts',(72.7223978767045,-1.49204659871303,
125.187793485758));
#270972=CARTESIAN_POINT('Ctrl Pts',(72.4439502528918,-5.53186462930466,
129.023769950998));
#270973=CARTESIAN_POINT('Ctrl Pts',(72.1655026290786,-4.48816931217651,
134.496022252122));
#270974=CARTESIAN_POINT('Ctrl Pts',(71.8870550052659,0.679934343581693,
136.575817858786));
#270975=CARTESIAN_POINT('Ctrl Pts',(71.6086073814528,5.22321155422762,133.351926212129));
#270976=CARTESIAN_POINT('Ctrl Pts',(71.3301597576401,4.96661251460835,127.786946239566));
#270977=CARTESIAN_POINT('Ctrl Pts',(71.0517121338272,0.145939206574258,
124.994822671498));
#270978=CARTESIAN_POINT('Ctrl Pts',(70.7732645100143,-4.80884510277506,
127.541380664158));
#270979=CARTESIAN_POINT('Ctrl Pts',(70.4948168862015,-5.34453568781766,
133.086457828568));
#270980=CARTESIAN_POINT('Ctrl Pts',(70.2163692623885,-0.968859070839113,
136.534399142713));
#270981=CARTESIAN_POINT('Ctrl Pts',(69.9379216385757,4.29715170084345,134.716714980192));
#270982=CARTESIAN_POINT('Ctrl Pts',(69.6594740147628,5.61428998698222,129.303768287553));
#270983=CARTESIAN_POINT('Ctrl Pts',(69.3810263909498,1.77217004839796,125.269792638185));
#270984=CARTESIAN_POINT('Ctrl Pts',(69.102578767137,-3.69848758934425,126.321814583191));
#270985=CARTESIAN_POINT('Ctrl Pts',(68.8241311433241,-5.77041581364239,
131.493077349239));
#270986=CARTESIAN_POINT('Ctrl Pts',(68.5456835195112,-2.53961380568736,
136.031443084562));
#270987=CARTESIAN_POINT('Ctrl Pts',(68.2672358956983,3.02496922266262,135.76637538989));
#270988=CARTESIAN_POINT('Ctrl Pts',(67.9887882718854,5.80975331334755,130.94145852735));
#270989=CARTESIAN_POINT('Ctrl Pts',(67.7103406480725,3.25565793129432,125.990555383323));
#270990=CARTESIAN_POINT('Ctrl Pts',(67.4318930242597,-2.29022804188655,
125.463304082106));
#270991=CARTESIAN_POINT('Ctrl Pts',(67.1534454004468,-5.73150632843341,
129.844222811859));
#270992=CARTESIAN_POINT('Ctrl Pts',(66.8749977766338,-3.90581029880048,
135.107461279717));
#270993=CARTESIAN_POINT('Ctrl Pts',(66.5965501528209,1.50913458598933,136.416360457212));
#270994=CARTESIAN_POINT('Ctrl Pts',(66.3181025290079,5.53725851157817,132.568105943505));
#270995=CARTESIAN_POINT('Ctrl Pts',(66.0396549051952,4.47691237514338,127.09905563901));
#270996=CARTESIAN_POINT('Ctrl Pts',(65.7612072813823,-0.69749752471975,
125.034999595595));
#270997=CARTESIAN_POINT('Ctrl Pts',(65.4827596575694,-5.23094127401388,
128.272704482416));
#270998=CARTESIAN_POINT('Ctrl Pts',(65.2043120337565,-4.95740553817722,
133.836877679162));
#270999=CARTESIAN_POINT('Ctrl Pts',(64.9258644099437,-0.128256295479839,
136.614315842995));
#271000=CARTESIAN_POINT('Ctrl Pts',(64.6474167861306,4.81875421709505,134.05268898675));
#271001=CARTESIAN_POINT('Ctrl Pts',(64.3689691623179,5.33756501339024,128.506007048888));
#271002=CARTESIAN_POINT('Ctrl Pts',(64.0905215385049,0.951414316927145,
125.071399759827));
#271003=CARTESIAN_POINT('Ctrl Pts',(63.8120739146922,-4.30903965761881,
126.905103428319));
#271004=CARTESIAN_POINT('Ctrl Pts',(63.5336262908791,-5.60969669510319,
132.322033964426));
#271005=CARTESIAN_POINT('Ctrl Pts',(63.2551786670663,-1.75531651870651,
136.344296837232));
#271006=CARTESIAN_POINT('Ctrl Pts',(62.9767310432534,3.71211378640213,135.275628965096));
#271007=CARTESIAN_POINT('Ctrl Pts',(62.6982834194405,5.76829286864752,130.098083915181));
#271008=CARTESIAN_POINT('Ctrl Pts',(62.4198357956276,2.52369260137852,125.569572651222));
#271009=CARTESIAN_POINT('Ctrl Pts',(62.1413881718147,-3.04005787731984,
125.851575794724));
#271010=CARTESIAN_POINT('Ctrl Pts',(61.8629405480017,-5.81014368184488,
130.684946233427));
#271011=CARTESIAN_POINT('Ctrl Pts',(61.5844929241889,-3.24099128405306,
135.628052657436));
#271012=CARTESIAN_POINT('Ctrl Pts',(61.3060453003759,2.306473772557,136.138421747261));
#271013=CARTESIAN_POINT('Ctrl Pts',(61.0275976765631,5.73440210969521,131.747049242268));
#271014=CARTESIAN_POINT('Ctrl Pts',(60.7491500527502,3.89269504914048,126.489391944074));
#271015=CARTESIAN_POINT('Ctrl Pts',(60.4707024289374,-1.5262085928491,125.196980058879));
#271016=CARTESIAN_POINT('Ctrl Pts',(60.1922548051244,-5.54260109744501,
129.057476971348));
#271017=CARTESIAN_POINT('Ctrl Pts',(59.9138071813117,-4.46561396460588,
134.52327461468));
#271018=CARTESIAN_POINT('Ctrl Pts',(59.6353595574987,0.715054244335847,
136.571571973714));
#271019=CARTESIAN_POINT('Ctrl Pts',(59.3569119336859,5.23862253507484,133.320083840384));
#271020=CARTESIAN_POINT('Ctrl Pts',(59.0784643098728,4.94815263701827,127.756768965196));
#271021=CARTESIAN_POINT('Ctrl Pts',(58.80001668606,0.110572196236736,124.994041935407));
#271022=CARTESIAN_POINT('Ctrl Pts',(58.5215690622471,-4.82861869113419,
127.570713924673));
#271023=CARTESIAN_POINT('Ctrl Pts',(58.2431214384343,-5.3305448924898,133.118949252284));
#271024=CARTESIAN_POINT('Ctrl Pts',(57.9646738146213,-0.933960749242644,
136.54019069853));
#271025=CARTESIAN_POINT('Ctrl Pts',(57.6862261908085,4.32088769603949,134.690484511247));
#271026=CARTESIAN_POINT('Ctrl Pts',(57.4077785669955,5.6050514357603,129.269620313377));
#271027=CARTESIAN_POINT('Ctrl Pts',(57.1293309431827,1.73844672800264,125.259107478825));
#271028=CARTESIAN_POINT('Ctrl Pts',(56.8508833193697,-3.72570559494523,
126.3444113781));
#271029=CARTESIAN_POINT('Ctrl Pts',(56.5724356955568,-5.76611648697549,
131.528190747811));
#271030=CARTESIAN_POINT('Ctrl Pts',(56.293988071744,-2.50774801792579,136.046805588895));
#271031=CARTESIAN_POINT('Ctrl Pts',(56.0155404479311,3.05511836929639,135.747869609001));
#271032=CARTESIAN_POINT('Ctrl Pts',(55.7370928241181,5.81048022596477,130.906090369819));
#271033=CARTESIAN_POINT('Ctrl Pts',(55.4586452003054,3.22629461271119,125.97082645809));
#271034=CARTESIAN_POINT('Ctrl Pts',(55.1801975764924,-2.32269813636975,
125.477344307648));
#271035=CARTESIAN_POINT('Ctrl Pts',(54.9017499526795,-5.73724476823917,
129.879129906805));
#271036=CARTESIAN_POINT('Ctrl Pts',(54.6233023288666,-3.87954373808533,
135.131157329118));
#271037=CARTESIAN_POINT('Ctrl Pts',(54.3448547050537,1.54326846112093,136.407069949284));
#271038=CARTESIAN_POINT('Ctrl Pts',(54.0664070812409,5.54789233741261,132.534366401168));
#271039=CARTESIAN_POINT('Ctrl Pts',(53.7879594574279,4.45427418523046,127.071872053402));
#271040=CARTESIAN_POINT('Ctrl Pts',(53.5095118336151,-0.732604339787292,
125.039352353899));
#271041=CARTESIAN_POINT('Ctrl Pts',(53.2310642098022,-5.24625526625226,
128.304593612394));
#271042=CARTESIAN_POINT('Ctrl Pts',(52.9526165859893,-4.93885389684926,
133.866998628235));
#271043=CARTESIAN_POINT('Ctrl Pts',(52.6741689621764,-0.0928870726681018,
136.614988930455));
#271044=CARTESIAN_POINT('Ctrl Pts',(52.3957213383635,4.83843843350925,134.023295678104));
#271045=CARTESIAN_POINT('Ctrl Pts',(52.1172737145507,5.32347539014984,128.473558358838));
#271046=CARTESIAN_POINT('Ctrl Pts',(51.8388260907377,0.91649852947334,125.065714449322));
#271047=CARTESIAN_POINT('Ctrl Pts',(51.5603784669247,-4.33269570634681,
126.931406019971));
#271048=CARTESIAN_POINT('Ctrl Pts',(51.2819308431118,-5.6003542519866,132.356153661459));
#271049=CARTESIAN_POINT('Ctrl Pts',(51.0034832192991,-1.72156083256576,
136.354879304913));
#271050=CARTESIAN_POINT('Ctrl Pts',(50.7250355954861,3.73926288906064,135.252949432607));
#271051=CARTESIAN_POINT('Ctrl Pts',(50.4465879716733,5.76388668878802,130.062983764924));
#271052=CARTESIAN_POINT('Ctrl Pts',(50.1681403478604,2.49178020303801,125.554307206545));
#271053=CARTESIAN_POINT('Ctrl Pts',(49.8896927240475,-3.07015055907373,
125.870173253527));
#271054=CARTESIAN_POINT('Ctrl Pts',(49.6112451002346,-5.81076294258959,
130.720316439607));
#271055=CARTESIAN_POINT('Ctrl Pts',(49.3327974764216,-3.21156805341676,
135.647692119444));
#271056=CARTESIAN_POINT('Ctrl Pts',(49.0543498526089,2.33890098302428,136.124282758954));
#271057=CARTESIAN_POINT('Ctrl Pts',(48.7759022287959,5.74003427773134,131.712124843171));
#271058=CARTESIAN_POINT('Ctrl Pts',(48.497454604983,3.86635648746696,126.465775950806));
#271059=CARTESIAN_POINT('Ctrl Pts',(48.2190069811701,-1.56031403276457,
125.206374415548));
#271060=CARTESIAN_POINT('Ctrl Pts',(47.9405593573573,-5.55313218246346,
129.091248723115));
#271061=CARTESIAN_POINT('Ctrl Pts',(47.6621117335443,-4.44289314206747,
134.550389171513));
#271062=CARTESIAN_POINT('Ctrl Pts',(47.3836641097315,0.750147648492217,
136.567112382502));
#271063=CARTESIAN_POINT('Ctrl Pts',(47.1052164859186,5.25383939683757,133.288148247589));
#271064=CARTESIAN_POINT('Ctrl Pts',(46.8267688621057,4.92950940381243,127.726704620456));
#271065=CARTESIAN_POINT('Ctrl Pts',(46.5483212382927,0.0752010886061242,
124.993476502813));
#271066=CARTESIAN_POINT('Ctrl Pts',(46.2698736144798,-4.84821335325179,
127.600167009156));
#271067=CARTESIAN_POINT('Ctrl Pts',(45.991425990667,-5.31635657186091,133.151354908068));
#271068=CARTESIAN_POINT('Ctrl Pts',(45.7129783668541,-0.899027819386881,
136.545769711054));
#271069=CARTESIAN_POINT('Ctrl Pts',(45.4345307430412,4.344463579153,134.664110040551));
#271070=CARTESIAN_POINT('Ctrl Pts',(45.1560831192283,5.5956051872961,129.235529209567));
#271071=CARTESIAN_POINT('Ctrl Pts',(44.8776354954154,1.70465898882477,125.248627800858));
#271072=CARTESIAN_POINT('Ctrl Pts',(44.5991878716026,-3.7527855431554,126.367173438067));
#271073=CARTESIAN_POINT('Ctrl Pts',(44.3207402477896,-5.76160349474165,
131.563277324591));
#271074=CARTESIAN_POINT('Ctrl Pts',(44.0422926239769,-2.47578930463884,
136.0619738325));
#271075=CARTESIAN_POINT('Ctrl Pts',(43.7638450001637,3.08515430739569,135.72918064457));
#271076=CARTESIAN_POINT('Ctrl Pts',(43.485397376351,5.8109918291003,130.870718442656));
#271077=CARTESIAN_POINT('Ctrl Pts',(43.206949752538,3.19681174259461,125.951276641244));
#271078=CARTESIAN_POINT('Ctrl Pts',(42.9285021287252,-2.3550821624196,125.491581927739));
#271079=CARTESIAN_POINT('Ctrl Pts',(42.6500545049123,-5.74277061233009,
129.914071286517));
#271080=CARTESIAN_POINT('Ctrl Pts',(42.3716068810994,-3.85313341945026,
135.154693047476));
#271081=CARTESIAN_POINT('Ctrl Pts',(42.0931592572865,1.57734514987214,136.397571830902));
#271082=CARTESIAN_POINT('Ctrl Pts',(41.8147116334736,5.5583205840564,132.50056275283));
#271083=CARTESIAN_POINT('Ctrl Pts',(41.5362640096606,4.43147094054935,127.04482677653));
#271084=CARTESIAN_POINT('Ctrl Pts',(41.2578163858478,-0.767684007931795,
125.043918736703));
#271085=CARTESIAN_POINT('Ctrl Pts',(40.9793687620349,-5.26137485657243,
128.336575372158));
#271086=CARTESIAN_POINT('Ctrl Pts',(40.700921138222,-4.9201192444739,133.897006090131));
#271087=CARTESIAN_POINT('Ctrl Pts',(40.4224735144091,-0.0575144078915333,
136.615446702946));
#271088=CARTESIAN_POINT('Ctrl Pts',(40.1440258905964,4.85794335980812,133.993783090635));
#271089=CARTESIAN_POINT('Ctrl Pts',(39.8655782667833,5.30918850357096,128.441196037522));
#271090=CARTESIAN_POINT('Ctrl Pts',(39.5871306429705,0.8815487808295,125.060241786462));
#271091=CARTESIAN_POINT('Ctrl Pts',(39.3086830191576,-4.35619120544207,
126.957852125381));
#271092=CARTESIAN_POINT('Ctrl Pts',(39.0302353953447,-5.59080428568363,
132.39021585623));
#271093=CARTESIAN_POINT('Ctrl Pts',(38.7517877715318,-1.6877413533555,136.365256096082));
#271094=CARTESIAN_POINT('Ctrl Pts',(38.4733401477189,3.76627343195761,135.230105056025));
#271095=CARTESIAN_POINT('Ctrl Pts',(38.194892523906,5.7592669259876,130.027911086658));
#271096=CARTESIAN_POINT('Ctrl Pts',(37.9164449000932,2.45977547086574,125.539236304527));
#271097=CARTESIAN_POINT('Ctrl Pts',(37.6379972762802,-3.10012947526937,
125.888953550457));
#271098=CARTESIAN_POINT('Ctrl Pts',(37.3595496524674,-5.81116688337655,
130.755689760074));
#271099=CARTESIAN_POINT('Ctrl Pts',(37.0811020286545,-3.18202581694541,
135.667152110023));
#271100=CARTESIAN_POINT('Ctrl Pts',(36.8026544048415,2.3712415246555,136.109946638975));
#271101=CARTESIAN_POINT('Ctrl Pts',(36.5242067810287,5.74545374668639,131.677166806538));
#271102=CARTESIAN_POINT('Ctrl Pts',(36.2457591572158,3.83987465653194,126.442320725389));
#271103=CARTESIAN_POINT('Ctrl Pts',(35.9673115334029,-1.59436165466975,
125.215976207654));
#271104=CARTESIAN_POINT('Ctrl Pts',(35.6888639095901,-5.56345749412674,
129.125083954872));
#271105=CARTESIAN_POINT('Ctrl Pts',(35.4104162857771,-4.42000768648982,
134.57736491788));
#271106=CARTESIAN_POINT('Ctrl Pts',(35.1319686619643,0.785213255651605,
136.562439250406));
#271107=CARTESIAN_POINT('Ctrl Pts',(34.8535210381513,5.26886157564935,133.25612061713));
#271108=CARTESIAN_POINT('Ctrl Pts',(34.5750734143385,4.91068350582282,127.69675431939));
#271109=CARTESIAN_POINT('Ctrl Pts',(34.2966257905255,0.0398271943713243,
124.993126394665));
#271110=CARTESIAN_POINT('Ctrl Pts',(34.0181781667127,-4.86762836304081,
127.629738826211));
#271111=CARTESIAN_POINT('Ctrl Pts',(33.7397305428998,-5.30197125168398,
133.183673595116));
#271112=CARTESIAN_POINT('Ctrl Pts',(33.4612829190869,-0.864061575724654,
136.551135973552));
#271113=CARTESIAN_POINT('Ctrl Pts',(33.182835295274,4.36787847657091,134.637592545421));
#271114=CARTESIAN_POINT('Ctrl Pts',(32.9043876714611,5.58595159162396,129.201496239381));
#271115=CARTESIAN_POINT('Ctrl Pts',(32.6259400476482,1.67080808288091,125.238353992614));
#271116=CARTESIAN_POINT('Ctrl Pts',(32.3474924238352,-3.77972643051725,
126.390099919638));
#271117=CARTESIAN_POINT('Ctrl Pts',(32.0690448000224,-5.75687700417149,
131.598335779433));
#271118=CARTESIAN_POINT('Ctrl Pts',(31.7905971762095,-2.44373885006871,
136.076947253315));
#271119=CARTESIAN_POINT('Ctrl Pts',(31.5121495523967,3.11507592396733,135.71030918912));
#271120=CARTESIAN_POINT('Ctrl Pts',(31.2337019285837,5.81128810379662,130.835344056578));
#271121=CARTESIAN_POINT('Ctrl Pts',(30.9552543047708,3.16721041344351,125.931906657209));
#271122=CARTESIAN_POINT('Ctrl Pts',(30.676806680958,-2.38737892003384,125.506016414799));
#271123=CARTESIAN_POINT('Ctrl Pts',(30.398359057145,-5.74808365594406,129.949045656226));
#271124=CARTESIAN_POINT('Ctrl Pts',(30.1199114333322,-3.82658032153943,
135.178067562667));
#271125=CARTESIAN_POINT('Ctrl Pts',(29.8414638095193,1.61136338951851,136.387866454021));
#271126=CARTESIAN_POINT('Ctrl Pts',(29.5630161857064,5.56854286508694,132.466696251098));
#271127=CARTESIAN_POINT('Ctrl Pts',(29.2845685618935,4.40850348608286,127.017920810568));
#271128=CARTESIAN_POINT('Ctrl Pts',(29.0061209380806,-0.802735229263066,
125.048698574801));
#271129=CARTESIAN_POINT('Ctrl Pts',(28.7276733142678,-5.27629948471241,
128.368648576612));
#271130=CARTESIAN_POINT('Ctrl Pts',(28.4492256904548,-4.90120227527057,
133.926898952911));
#271131=CARTESIAN_POINT('Ctrl Pts',(28.170778066642,-0.0221396118974229,
136.615689143506));
#271132=CARTESIAN_POINT('Ctrl Pts',(27.892330442829,4.87726827322928,133.964152317942));
#271133=CARTESIAN_POINT('Ctrl Pts',(27.6138828190162,5.29470488305963,128.408921284139));
#271134=CARTESIAN_POINT('Ctrl Pts',(27.3354351952032,0.846566366071392,
125.054981974037));
#271135=CARTESIAN_POINT('Ctrl Pts',(27.0569875713904,-4.37952528427021,
126.984440764576));
#271136=CARTESIAN_POINT('Ctrl Pts',(26.7785399475775,-5.58104715007188,
132.424219286554));
#271137=CARTESIAN_POINT('Ctrl Pts',(26.5000923237646,-1.65385933426847,
136.375426826225));
#271138=CARTESIAN_POINT('Ctrl Pts',(26.2216446999517,3.79314441420758,135.207096681855));
#271139=CARTESIAN_POINT('Ctrl Pts',(25.9431970761388,5.75443375143326,129.992867180015));
#271140=CARTESIAN_POINT('Ctrl Pts',(25.6647494523259,2.42767959080881,125.524360503627));
#271141=CARTESIAN_POINT('Ctrl Pts',(25.3863018285131,-3.12999351502748,
125.907915989602));
#271142=CARTESIAN_POINT('Ctrl Pts',(25.1078542047001,-5.81135548923757,
130.791064884058));
#271143=CARTESIAN_POINT('Ctrl Pts',(24.8294065808873,-3.152365669337,135.686431908074));
#271144=CARTESIAN_POINT('Ctrl Pts',(24.5509589570743,2.40349419906,136.095413918554));
#271145=CARTESIAN_POINT('Ctrl Pts',(24.2725113332615,5.75066031573997,131.64217642775));
#271146=CARTESIAN_POINT('Ctrl Pts',(23.9940637094486,3.81325053762949,126.419027136963));
#271147=CARTESIAN_POINT('Ctrl Pts',(23.7156160856357,-1.62835019691723,
125.2257850794));
#271148=CARTESIAN_POINT('Ctrl Pts',(23.4371684618228,-5.57357664982666,
129.158981412844));
#271149=CARTESIAN_POINT('Ctrl Pts',(23.1587208380098,-4.39695844590187,
134.604200854185));
#271150=CARTESIAN_POINT('Ctrl Pts',(22.880273214197,0.820249766445046,136.557552750588));
#271151=CARTESIAN_POINT('Ctrl Pts',(22.6018255903841,5.28368851485763,133.224002135804));
#271152=CARTESIAN_POINT('Ctrl Pts',(22.3233779665712,4.89167564065013,127.666919171818));
#271153=CARTESIAN_POINT('Ctrl Pts',(22.0449303427584,0.00445182432539013,
124.992991623939));
#271154=CARTESIAN_POINT('Ctrl Pts',(21.7664827189454,-4.88686300107076,
127.659428280044));
#271155=CARTESIAN_POINT('Ctrl Pts',(21.4880350951325,-5.28738946501251,
133.215904115845));
#271156=CARTESIAN_POINT('Ctrl Pts',(21.2095874713197,-0.829063313942982,
136.556289287176));
#271157=CARTESIAN_POINT('Ctrl Pts',(20.9311398475068,4.39113152064558,134.610933008472));
#271158=CARTESIAN_POINT('Ctrl Pts',(20.6526922236938,5.57609100646137,129.167522663925));
#271159=CARTESIAN_POINT('Ctrl Pts',(20.374244599881,1.6368952645291,125.228286434793));
#271160=CARTESIAN_POINT('Ctrl Pts',(20.0957969760681,-3.80652725872624,
126.413189973261));
#271161=CARTESIAN_POINT('Ctrl Pts',(19.8173493522552,-5.75193719040684,
131.633364813234));
#271162=CARTESIAN_POINT('Ctrl Pts',(19.5389017284423,-2.41159784185683,
136.091725296493));
#271163=CARTESIAN_POINT('Ctrl Pts',(19.2604541046294,3.14488211025528,135.691255941942));
#271164=CARTESIAN_POINT('Ctrl Pts',(18.9820064808165,5.81136903907515,130.799968522399));
#271165=CARTESIAN_POINT('Ctrl Pts',(18.7035588570036,3.13749172214556,125.912717223747));
#271166=CARTESIAN_POINT('Ctrl Pts',(18.4251112331907,-2.41958721244422,
125.52064723395));
#271167=CARTESIAN_POINT('Ctrl Pts',(18.1466636093778,-5.75318370220431,
129.984051719947));
#271168=CARTESIAN_POINT('Ctrl Pts',(17.868215985565,-3.79988542828747,135.201280008538));
#271169=CARTESIAN_POINT('Ctrl Pts',(17.589768361752,1.64532191950215,136.377954178279));
#271170=CARTESIAN_POINT('Ctrl Pts',(17.3113207379392,5.57855880171371,132.432768150908));
#271171=CARTESIAN_POINT('Ctrl Pts',(17.0328731141263,4.38537267289848,126.991155152525));
#271172=CARTESIAN_POINT('Ctrl Pts',(16.7544254903134,-0.83775670494522,
125.053691691071));
#271173=CARTESIAN_POINT('Ctrl Pts',(16.4759778665005,-5.29102859763445,
128.400812037271));
#271174=CARTESIAN_POINT('Ctrl Pts',(16.1975302426876,-4.88210369021464,
133.956676108886));
#271175=CARTESIAN_POINT('Ctrl Pts',(15.9190826188747,0.013236004487936,
136.61571624315));
#271176=CARTESIAN_POINT('Ctrl Pts',(15.6406349950618,4.89641245768097,133.934404458007));
#271177=CARTESIAN_POINT('Ctrl Pts',(15.3621873712489,5.2800250653117,128.376735294641));
#271178=CARTESIAN_POINT('Ctrl Pts',(15.0837397474361,0.811552581485459,
125.049935206953));
#271179=CARTESIAN_POINT('Ctrl Pts',(14.8052921236231,-4.40269707817821,
127.011170952307));
#271180=CARTESIAN_POINT('Ctrl Pts',(14.5268444998103,-5.57108320670569,
132.458162692417));
#271181=CARTESIAN_POINT('Ctrl Pts',(14.2483968759974,-1.6199160308156,136.385391118461));
#271182=CARTESIAN_POINT('Ctrl Pts',(13.9699492521845,3.81987484009636,135.18392516268));
#271183=CARTESIAN_POINT('Ctrl Pts',(13.6915016283715,5.74938734422005,129.95785334356));
#271184=CARTESIAN_POINT('Ctrl Pts',(13.4130540045587,2.39549375219187,125.509680355073));
#271185=CARTESIAN_POINT('Ctrl Pts',(13.1346063807458,-3.15974157172482,
125.927059868305));
#271186=CARTESIAN_POINT('Ctrl Pts',(12.8561587569329,-5.81132875318382,
130.82644050072));
#271187=CARTESIAN_POINT('Ctrl Pts',(12.57771113312,-3.12258870965941,135.705530799178));
#271188=CARTESIAN_POINT('Ctrl Pts',(12.2992635093071,2.43565781110307,136.080685136208));
#271189=CARTESIAN_POINT('Ctrl Pts',(12.0208158854942,5.75565379196074,131.607155003388));
#271190=CARTESIAN_POINT('Ctrl Pts',(11.7423682616813,3.78648511732596,126.395896048684));
#271191=CARTESIAN_POINT('Ctrl Pts',(11.4639206378685,-1.66227840004959,
125.235800667314));
#271192=CARTESIAN_POINT('Ctrl Pts',(11.1854730140555,-5.58348927459409,
129.192939840948));
#271193=CARTESIAN_POINT('Ctrl Pts',(10.9070253902426,-4.37374627440173,
134.630895986013));
#271194=CARTESIAN_POINT('Ctrl Pts',(10.6285777664298,0.855255882581734,
136.552453064119));
#271195=CARTESIAN_POINT('Ctrl Pts',(10.3501301426169,5.29831966504511,133.19179399377));
#271196=CARTESIAN_POINT('Ctrl Pts',(10.071682518804,4.87248651263752,127.637200283293));
#271197=CARTESIAN_POINT('Ctrl Pts',(9.79323489499104,-0.0309237106847325,
124.993072195629));
#271198=CARTESIAN_POINT('Ctrl Pts',(9.51478727117816,-4.90591655459505,
127.689234270502));
#271199=CARTESIAN_POINT('Ctrl Pts',(9.23633964736526,-5.27261175218,133.248045275945));
#271200=CARTESIAN_POINT('Ctrl Pts',(8.95789202355236,-0.794034330915497,
136.561229460968));
#271201=CARTESIAN_POINT('Ctrl Pts',(8.67944439973947,4.41422184972672,134.584132417584));
#271202=CARTESIAN_POINT('Ctrl Pts',(8.40099677592661,5.56602379719609,129.1336097421));
#271203=CARTESIAN_POINT('Ctrl Pts',(8.12254915211368,1.60292179042129,125.218425500451));
#271204=CARTESIAN_POINT('Ctrl Pts',(7.84410152830078,-3.83318703466779,
126.436442743329));
#271205=CARTESIAN_POINT('Ctrl Pts',(7.56565390448795,-5.74678423649425,
131.668363127979));
#271206=CARTESIAN_POINT('Ctrl Pts',(7.28720628067502,-2.37936747100029,
136.106307414428));
#271207=CARTESIAN_POINT('Ctrl Pts',(7.00875865686212,3.17457176177998,135.672021609062));
#271208=CARTESIAN_POINT('Ctrl Pts',(6.73031103304925,5.81123463193681,130.764593150968));
#271209=CARTESIAN_POINT('Ctrl Pts',(6.45186340923634,3.10765676993803,125.89370905193));
#271210=CARTESIAN_POINT('Ctrl Pts',(6.17341578542346,-2.45170584616043,
125.535473843045));
#271211=CARTESIAN_POINT('Ctrl Pts',(5.89496816161054,-5.75807056212669,
130.019088180515));
#271212=CARTESIAN_POINT('Ctrl Pts',(5.61652053779771,-3.77304972888379,
135.224329524944));
#271213=CARTESIAN_POINT('Ctrl Pts',(5.33807291398477,1.67921948147701,136.367835370977));
#271214=CARTESIAN_POINT('Ctrl Pts',(5.05962529017187,5.58836802279258,132.398779709476));
#271215=CARTESIAN_POINT('Ctrl Pts',(4.781177666359,4.36207935811697,126.964530794212));
#271216=CARTESIAN_POINT('Ctrl Pts',(4.50273004254611,-0.872747137244579,
125.058897900495));
#271217=CARTESIAN_POINT('Ctrl Pts',(4.2242824187332,-5.30556164954619,128.433064562307));
#271218=CARTESIAN_POINT('Ctrl Pts',(3.94583479492031,-4.86282419701095,
133.986336454649));
#271219=CARTESIAN_POINT('Ctrl Pts',(3.66738717110745,0.0486111304084952,
136.615528000873));
#271220=CARTESIAN_POINT('Ctrl Pts',(3.38893954729453,4.91537520376836,133.904540613147));
#271221=CARTESIAN_POINT('Ctrl Pts',(3.11049192348162,5.26514959429328,128.344639261694));
#271222=CARTESIAN_POINT('Ctrl Pts',(2.83204429966877,0.776508724519974,
125.045101672218));
#271223=CARTESIAN_POINT('Ctrl Pts',(2.55359667585587,-4.42570572852705,
127.038041698076));
#271224=CARTESIAN_POINT('Ctrl Pts',(2.27514905204296,-5.56091282480238,
132.492044816037));
#271225=CARTESIAN_POINT('Ctrl Pts',(1.99670142823006,-1.58591270077849,
136.395148603559));
#271226=CARTESIAN_POINT('Ctrl Pts',(1.7182538044172,3.84646371911817,135.160591357131));
#271227=CARTESIAN_POINT('Ctrl Pts',(1.43980618060429,5.7441278913444,129.922870874744));
#271228=CARTESIAN_POINT('Ctrl Pts',(1.16135855679139,2.36321914767325,125.495196402842));
#271229=CARTESIAN_POINT('Ctrl Pts',(0.882910932978526,-3.18937254303613,
125.946384477181));
#271230=CARTESIAN_POINT('Ctrl Pts',(0.604463309165634,-5.81108667620601,
130.861815299204));
#271231=CARTESIAN_POINT('Ctrl Pts',(0.326015685352703,-3.09269604130886,
135.724448075619));
#271232=CARTESIAN_POINT('Ctrl Pts',(0.0475680615398608,2.46773116894999,
136.065760837718));
#271233=CARTESIAN_POINT('Ctrl Pts',(-0.230879562273037,5.76043399031358,
131.572103831187));
#271234=CARTESIAN_POINT('Ctrl Pts',(-0.509327186085944,3.75957938742415,
126.37292831768));
#271235=CARTESIAN_POINT('Ctrl Pts',(-0.787774809898847,-1.69614500684454,
125.246022600264));
#271236=CARTESIAN_POINT('Ctrl Pts',(-1.06622243371171,-5.59319500111311,
129.226957980841));
#271237=CARTESIAN_POINT('Ctrl Pts',(-1.34467005752462,-4.35037203212501,
134.657449324165));
#271238=CARTESIAN_POINT('Ctrl Pts',(-1.62311768133752,0.890230306896913,
136.547140379971));
#271239=CARTESIAN_POINT('Ctrl Pts',(-1.90156530515039,5.31275448404895,
133.159497384516));
#271240=CARTESIAN_POINT('Ctrl Pts',(-2.18001292896328,4.85311683284533,
127.607598755059));
#271241=CARTESIAN_POINT('Ctrl Pts',(-2.4584605527762,-0.0662980998053887,
124.993368106748));
#271242=CARTESIAN_POINT('Ctrl Pts',(-2.73690817658909,-4.92478831757726,
127.719155693111));
#271243=CARTESIAN_POINT('Ctrl Pts',(-3.01535580040196,-5.25763866077998,
133.280095884409));
#271244=CARTESIAN_POINT('Ctrl Pts',(-3.29380342421486,-0.758975924653704,
136.565956311869));
#271245=CARTESIAN_POINT('Ctrl Pts',(-3.57225104802777,4.43714860819409,
134.557191765862));
#271246=CARTESIAN_POINT('Ctrl Pts',(-3.85069867184063,5.55575033687191,
129.099758730564));
#271247=CARTESIAN_POINT('Ctrl Pts',(-4.12914629565353,1.56888891945708,
125.208771554989));
#271248=CARTESIAN_POINT('Ctrl Pts',(-4.40759391946644,-3.85970477045413,
126.459857368199));
#271249=CARTESIAN_POINT('Ctrl Pts',(-4.68604154327934,-5.74141833337845,
131.703329426794));
#271250=CARTESIAN_POINT('Ctrl Pts',(-4.96448916709218,-2.34704893180687,
136.120693066776));
#271251=CARTESIAN_POINT('Ctrl Pts',(-5.24293679090511,3.20414377838073,
135.652606903212));
#271252=CARTESIAN_POINT('Ctrl Pts',(-5.52138441471801,5.81088488736209,
130.729219253137));
#271253=CARTESIAN_POINT('Ctrl Pts',(-5.79983203853088,3.07770666236606,
125.874882846113));
#271254=CARTESIAN_POINT('Ctrl Pts',(-6.07827966234377,-2.48373363101511,
125.550495692676));
#271255=CARTESIAN_POINT('Ctrl Pts',(-6.35672728615668,-5.7627440546269,
130.054153739642));
#271256=CARTESIAN_POINT('Ctrl Pts',(-6.63517490996957,-3.74607421773465,
135.247215257776));
#271257=CARTESIAN_POINT('Ctrl Pts',(-6.91362253378244,1.71305481935644,
136.357510407073));
#271258=CARTESIAN_POINT('Ctrl Pts',(-7.19207015759534,5.59797016483923,
132.36473218626));
#271259=CARTESIAN_POINT('Ctrl Pts',(-7.47051778140826,4.33862440488076,
126.938048722207));
#271260=CARTESIAN_POINT('Ctrl Pts',(-7.74896540522111,-0.907705229577551,
125.064317010151));
#271261=CARTESIAN_POINT('Ctrl Pts',(-8.027413029034,-5.31989810191992,128.46540495659));
#271262=CARTESIAN_POINT('Ctrl Pts',(-8.30586065284694,-4.84336451006833,
134.015878891129));
#271263=CARTESIAN_POINT('Ctrl Pts',(-8.58430827665978,0.0839844550257475,
136.615124423653));
#271264=CARTESIAN_POINT('Ctrl Pts',(-8.86275590047269,4.93415580881975,
133.874561889976));
#271265=CARTESIAN_POINT('Ctrl Pts',(-9.14120352428557,5.25007902122049,
128.312634374625));
#271266=CARTESIAN_POINT('Ctrl Pts',(-9.4196511480985,0.741436093738357,
125.040481548942));
#271267=CARTESIAN_POINT('Ctrl Pts',(-9.69809877191133,-4.44855038272257,
127.065052006178));
#271268=CARTESIAN_POINT('Ctrl Pts',(-9.97654639572428,-5.5505363812293,
132.525864401898));
#271269=CARTESIAN_POINT('Ctrl Pts',(-10.2549940195371,-1.55185060416301,
136.404698919952));
#271270=CARTESIAN_POINT('Ctrl Pts',(-10.53344164335,3.87291006601234,135.137096129849));
#271271=CARTESIAN_POINT('Ctrl Pts',(-10.8118892671629,5.7386555876974,129.887921069854));
#271272=CARTESIAN_POINT('Ctrl Pts',(-11.0903368909758,2.33085697319978,
125.480909183646));
#271273=CARTESIAN_POINT('Ctrl Pts',(-11.3687845147887,-3.21888533097506,
125.965889100148));
#271274=CARTESIAN_POINT('Ctrl Pts',(-11.6472321386015,-5.81062926727439,
130.897187968684));
#271275=CARTESIAN_POINT('Ctrl Pts',(-11.9256797624145,-3.06268877196916,
135.743183036409));
#271276=CARTESIAN_POINT('Ctrl Pts',(-12.2041273862274,2.49971308411117,
136.050641576106));
#271277=CARTESIAN_POINT('Ctrl Pts',(-12.4825750100403,5.76500073366654,
131.537024209977));
#271278=CARTESIAN_POINT('Ctrl Pts',(-12.7610226338531,3.73253434492532,
126.350124795028));
#271279=CARTESIAN_POINT('Ctrl Pts',(-13.039470257666,-1.7299487623625,125.256450499474));
#271280=CARTESIAN_POINT('Ctrl Pts',(-13.3179178814789,-5.60269346973446,
129.261034571969));
#271281=CARTESIAN_POINT('Ctrl Pts',(-13.5963655052918,-4.32683658521273,
134.683859884699));
#271282=CARTESIAN_POINT('Ctrl Pts',(-13.8748131291047,0.925171743400955,
136.541614895008));
#271283=CARTESIAN_POINT('Ctrl Pts',(-14.1532607529176,5.3269924369816,133.127113504801));
#271284=CARTESIAN_POINT('Ctrl Pts',(-14.4317083767304,4.83356731902416,
127.578115684011));
#271285=CARTESIAN_POINT('Ctrl Pts',(-14.7101560005434,-0.101670032225581,
124.99387934633));
#271286=CARTESIAN_POINT('Ctrl Pts',(-14.9886036243562,-4.94347759071707,
127.749191439124));
#271287=CARTESIAN_POINT('Ctrl Pts',(-15.2670512481692,-5.24247074564602,
133.312054753593));
#271288=CARTESIAN_POINT('Ctrl Pts',(-15.545498871982,-0.723889394260118,
136.570469664722));
#271289=CARTESIAN_POINT('Ctrl Pts',(-15.823946495795,4.45991094648802,134.530112051601));
#271290=CARTESIAN_POINT('Ctrl Pts',(-16.1023941196078,5.54527100617588,
129.065970883678));
#271291=CARTESIAN_POINT('Ctrl Pts',(-16.3808417434207,1.53479791273714,
125.199324956138));
#271292=CARTESIAN_POINT('Ctrl Pts',(-16.6592893672336,-3.88607948346057,
126.483432980235));
#271293=CARTESIAN_POINT('Ctrl Pts',(-16.9377369910465,-5.73583967989507,
131.738262413989));
#271294=CARTESIAN_POINT('Ctrl Pts',(-17.2161846148594,-2.31464342185212,
136.134881720468));
#271295=CARTESIAN_POINT('Ctrl Pts',(-17.4946322386723,3.23359706425542,
135.633012543814));
#271296=CARTESIAN_POINT('Ctrl Pts',(-17.7730798624852,5.81031981831091,
130.693848139697));
#271297=CARTESIAN_POINT('Ctrl Pts',(-18.0515274862981,3.04764250924188,
125.856239303907));
#271298=CARTESIAN_POINT('Ctrl Pts',(-18.3299751101109,-2.51566938020671,
125.565712226204));
#271299=CARTESIAN_POINT('Ctrl Pts',(-18.6084227339239,-5.76720400652691,
130.089247097961));
#271300=CARTESIAN_POINT('Ctrl Pts',(-18.8868703577367,-3.71895989442774,
135.269936358996));
#271301=CARTESIAN_POINT('Ctrl Pts',(-19.1653179815497,1.74682667935956,
136.346979669161));
#271302=CARTESIAN_POINT('Ctrl Pts',(-19.4437656053625,5.60736487204277,
132.330626842902));
#271303=CARTESIAN_POINT('Ctrl Pts',(-19.7222132291754,4.31500868232164,
126.91170991781));
#271304=CARTESIAN_POINT('Ctrl Pts',(-20.0006608529883,-0.942629686559699,
125.069948819234));
#271305=CARTESIAN_POINT('Ctrl Pts',(-20.2791084768012,-5.33403742351306,
128.497832021735));
#271306=CARTESIAN_POINT('Ctrl Pts',(-20.5575561006141,-4.82372535047263,
134.045302323618));
#271307=CARTESIAN_POINT('Ctrl Pts',(-20.836003724427,0.119354667568119,
136.614505526443));
#271308=CARTESIAN_POINT('Ctrl Pts',(-21.1144513482399,4.95275357691331,
133.844469399368));
#271309=CARTESIAN_POINT('Ctrl Pts',(-21.3928989720528,5.23481390453873,
128.280721819388));
#271310=CARTESIAN_POINT('Ctrl Pts',(-21.6713465958657,0.706335988769417,
125.036075008324));
#271311=CARTESIAN_POINT('Ctrl Pts',(-21.9497942196786,-4.47123019424771,
127.092200875735));
#271312=CARTESIAN_POINT('Ctrl Pts',(-22.2282418434914,-5.53995426048939,
132.559620196804));
#271313=CARTESIAN_POINT('Ctrl Pts',(-22.5066894673044,-1.5177310031529,
136.41404171375));
#271314=CARTESIAN_POINT('Ctrl Pts',(-22.7851370911172,3.89921290079955,
135.11344035146));
#271315=CARTESIAN_POINT('Ctrl Pts',(-23.0635847149301,5.73297063605735,
129.853005223969));
#271316=CARTESIAN_POINT('Ctrl Pts',(-23.342032338743,2.298408427964,125.466819226899));
#271317=CARTESIAN_POINT('Ctrl Pts',(-23.6204799625559,-3.24827884193431,
125.985573014458));
#271318=CARTESIAN_POINT('Ctrl Pts',(-23.8989275863688,-5.80995654333829,
130.932557198412));
#271319=CARTESIAN_POINT('Ctrl Pts',(-24.1773752101816,-3.03256801357094,
135.761734987319));
#271320=CARTESIAN_POINT('Ctrl Pts',(-24.4558228339946,2.53160237148462,
136.035327911625));
#271321=CARTESIAN_POINT('Ctrl Pts',(-24.7342704578075,5.76935385279724,
131.501917439649));
#271322=CARTESIAN_POINT('Ctrl Pts',(-25.0127180816204,3.70535099199371,
126.327486325724));
#271323=CARTESIAN_POINT('Ctrl Pts',(-25.2911657054332,-1.76368841399288,
125.267083978533));
#271324=CARTESIAN_POINT('Ctrl Pts',(-25.5696133292462,-5.61198432848891,
129.295168351611));
#271325=CARTESIAN_POINT('Ctrl Pts',(-25.8480609530591,-4.30314080577957,
134.71012668896));
#271326=CARTESIAN_POINT('Ctrl Pts',(-26.1265085768719,0.960078897325804,
136.535876813977));
#271327=CARTESIAN_POINT('Ctrl Pts',(-26.4049562006848,5.3410329962505,133.094643554625));
#271328=CARTESIAN_POINT('Ctrl Pts',(-26.6834038244978,4.81383869558843,
127.548752162656));
#271329=CARTESIAN_POINT('Ctrl Pts',(-26.9618514483106,-0.137038197225328,
124.994605895435));
#271330=CARTESIAN_POINT('Ctrl Pts',(-27.2402990721235,-4.96198368147699,
127.779340395554));
#271331=CARTESIAN_POINT('Ctrl Pts',(-27.5187466959364,-5.22710856883054,
133.343920699249));
#271332=CARTESIAN_POINT('Ctrl Pts',(-27.7971943197493,-0.688776039878604,
136.574769352283));
#271333=CARTESIAN_POINT('Ctrl Pts',(-28.0756419435621,4.48250802114168,
134.502894278251));
#271334=CARTESIAN_POINT('Ctrl Pts',(-28.3540895673751,5.53458619342344,
129.032247453463));
#271335=CARTESIAN_POINT('Ctrl Pts',(-28.632537191188,1.50065003351598,125.190086053944));
#271336=CARTESIAN_POINT('Ctrl Pts',(-28.9109848150008,-3.91231019636288,
126.507168705834));
#271337=CARTESIAN_POINT('Ctrl Pts',(-29.1894324388138,-5.73004848276283,
131.773160795109));
#271338=CARTESIAN_POINT('Ctrl Pts',(-29.4678800626266,-2.28215214193419,
136.148872849742));
#271339=CARTESIAN_POINT('Ctrl Pts',(-29.7463276864396,3.26293052800175,
135.613239256942));
#271340=CARTESIAN_POINT('Ctrl Pts',(-30.0247753102524,5.80953944572202,
130.658481121338));
#271341=CARTESIAN_POINT('Ctrl Pts',(-30.3032229340653,3.01746542460398,
125.837779116156));
#271342=CARTESIAN_POINT('Ctrl Pts',(-30.5816705578782,-2.54751191034413,
125.581122879776));
#271343=CARTESIAN_POINT('Ctrl Pts',(-30.8601181816911,-5.77145025256159,
130.124366955075));
#271344=CARTESIAN_POINT('Ctrl Pts',(-31.138565805504,-3.69170776369427,
135.292491986665));
#271345=CARTESIAN_POINT('Ctrl Pts',(-31.4170134293169,1.78053381005746,
136.336243547461));
#271346=CARTESIAN_POINT('Ctrl Pts',(-31.6954610531298,5.6165517962788,132.296464943187));
#271347=CARTESIAN_POINT('Ctrl Pts',(-31.9739086769427,4.29123306552915,
126.885515357016));
#271348=CARTESIAN_POINT('Ctrl Pts',(-32.2523563007555,-0.977519214052166,
125.075793119056));
#271349=CARTESIAN_POINT('Ctrl Pts',(-32.5308039245685,-5.34797909038788,
128.530344556146));
#271350=CARTESIAN_POINT('Ctrl Pts',(-32.8092515483813,-4.80390744596015,
134.07460566182));
#271351=CARTESIAN_POINT('Ctrl Pts',(-33.0876991721943,0.154720457379397,
136.613671332177));
#271352=CARTESIAN_POINT('Ctrl Pts',(-33.3661467960071,4.9711678189017,133.814264256411));
#271353=CARTESIAN_POINT('Ctrl Pts',(-33.64459441982,5.21935480990263,128.248902778514));
#271354=CARTESIAN_POINT('Ctrl Pts',(-33.9230420436329,0.671209710260644,
125.031882213649));
#271355=CARTESIAN_POINT('Ctrl Pts',(-34.2014896674458,-4.49374432269368,
127.119487300736));
#271356=CARTESIAN_POINT('Ctrl Pts',(-34.4799372912587,-5.52916685470707,
132.59331094992));
#271357=CARTESIAN_POINT('Ctrl Pts',(-34.7583849150716,-1.48355516206214,
136.423176638752));
#271358=CARTESIAN_POINT('Ctrl Pts',(-35.0368325388844,3.92537124881898,
135.089624898536));
#271359=CARTESIAN_POINT('Ctrl Pts',(-35.3152801626974,5.72707324708195,
129.818124630907));
#271360=CARTESIAN_POINT('Ctrl Pts',(-35.5937277865103,2.26587471435868,
125.45292705471));
#271361=CARTESIAN_POINT('Ctrl Pts',(-35.8721754103231,-3.27755198672651,
126.005435490714));
#271362=CARTESIAN_POINT('Ctrl Pts',(-36.1506230341361,-5.80906852932597,
130.967921677768));
#271363=CARTESIAN_POINT('Ctrl Pts',(-36.4290706579489,-3.00233488224952,
135.780103240898));
#271364=CARTESIAN_POINT('Ctrl Pts',(-36.7075182817618,2.56339784940132,
136.019820411726));
#271365=CARTESIAN_POINT('Ctrl Pts',(-36.9859659055747,5.77349318639923,
131.466784821096));
#271366=CARTESIAN_POINT('Ctrl Pts',(-37.2644135293876,3.67803033591843,
126.305013748643));
#271367=CARTESIAN_POINT('Ctrl Pts',(-37.5428611532005,-1.79736271150026,
125.277922643415));
#271368=CARTESIAN_POINT('Ctrl Pts',(-37.8213087770133,-5.62106723310019,
129.329358054928));
#271369=CARTESIAN_POINT('Ctrl Pts',(-38.0997564008263,-4.27928557188161,
134.736248763623));
#271370=CARTESIAN_POINT('Ctrl Pts',(-38.3782040246392,0.994950475174061,
136.529926349506));
#271371=CARTESIAN_POINT('Ctrl Pts',(-38.656651648452,5.35487564157755,133.062088737171));
#271372=CARTESIAN_POINT('Ctrl Pts',(-38.9350992722649,4.79393169358958,
127.51950927907));
#271373=CARTESIAN_POINT('Ctrl Pts',(-39.2135468960779,-0.172401284224016,
124.995547727136));
#271374=CARTESIAN_POINT('Ctrl Pts',(-39.4919945198907,-4.98030590410683,
127.809601445221));
#271375=CARTESIAN_POINT('Ctrl Pts',(-39.7704421437036,-5.21155269958477,
133.375692540572));
#271376=CARTESIAN_POINT('Ctrl Pts',(-40.0488897675166,-0.65363716264763,
136.578855215227));
#271377=CARTESIAN_POINT('Ctrl Pts',(-40.3273373913294,4.50493899481217,
134.475539454375));
#271378=CARTESIAN_POINT('Ctrl Pts',(-40.6057850151423,5.52369629454426,
128.998589689552));
#271379=CARTESIAN_POINT('Ctrl Pts',(-40.8842326389552,1.46644654715595,
125.181055190758));
#271380=CARTESIAN_POINT('Ctrl Pts',(-41.1626802627681,-3.93839593717207,
126.531063665459));
#271381=CARTESIAN_POINT('Ctrl Pts',(-41.441127886581,-5.72404495657686,
131.808023276983));
#271382=CARTESIAN_POINT('Ctrl Pts',(-41.7195755103939,-2.24957629602936,
136.162665936149));
#271383=CARTESIAN_POINT('Ctrl Pts',(-41.9980231342068,3.29214308265742,
135.593287775304));
#271384=CARTESIAN_POINT('Ctrl Pts',(-42.2764707580197,5.80854379851262,
130.623119508596));
#271385=CARTESIAN_POINT('Ctrl Pts',(-42.5549183818325,2.98717652667487,
125.81950296691));
#271386=CARTESIAN_POINT('Ctrl Pts',(-42.8333660056454,-2.57926004149102,
125.596727082342));
#271387=CARTESIAN_POINT('Ctrl Pts',(-43.1118136294584,-5.7754826353847,
130.159512009603));
#271388=CARTESIAN_POINT('Ctrl Pts',(-43.3902612532712,-3.66431883537201,
135.314881304976));
#271389=CARTESIAN_POINT('Ctrl Pts',(-43.6687088770841,1.81417496242045,
136.325302439805));
#271390=CARTESIAN_POINT('Ctrl Pts',(-43.947156500897,5.62553059712261,132.262247752997));
#271391=CARTESIAN_POINT('Ctrl Pts',(-44.2256041247099,4.26729843551711,
126.859466010475));
#271392=CARTESIAN_POINT('Ctrl Pts',(-44.5040517485228,-1.01237251921066,
125.081849693053));
#271393=CARTESIAN_POINT('Ctrl Pts',(-44.7824993723357,-5.3617225859308,
128.562941355057));
#271394=CARTESIAN_POINT('Ctrl Pts',(-45.0609469961486,-4.78391153089065,
134.103787819889));
#271395=CARTESIAN_POINT('Ctrl Pts',(-45.3393946199614,0.190080513966956,
136.612621871764));
#271396=CARTESIAN_POINT('Ctrl Pts',(-45.6178422437743,4.98939785243841,
133.783947580368));
#271397=CARTESIAN_POINT('Ctrl Pts',(-45.8962898675873,5.20370231015464,
128.217178431071));
#271398=CARTESIAN_POINT('Ctrl Pts',(-46.1747374914001,0.636058559829223,
125.027903320286));
#271399=CARTESIAN_POINT('Ctrl Pts',(-46.453185115213,-4.51609193379101,
127.146910270074));
#271400=CARTESIAN_POINT('Ctrl Pts',(-46.7316327390259,-5.51817456361365,
132.626935412823));
#271401=CARTESIAN_POINT('Ctrl Pts',(-47.0100803628388,-1.4493243472895,
136.43210335646));
#271402=CARTESIAN_POINT('Ctrl Pts',(-47.2885279866517,3.95138414076325,
135.06565065357));
#271403=CARTESIAN_POINT('Ctrl Pts',(-47.5669756104645,5.72096363930122,
129.783280583183));
#271404=CARTESIAN_POINT('Ctrl Pts',(-47.8454232342775,2.23325703793269,
125.439233181862));
#271405=CARTESIAN_POINT('Ctrl Pts',(-48.1238708580903,-3.30670368062431,
126.025475792906));
#271406=CARTESIAN_POINT('Ctrl Pts',(-48.4023184819033,-5.80796525814313,
131.00328009631));
#271407=CARTESIAN_POINT('Ctrl Pts',(-48.6807661057162,-2.97199049830493,
135.798287116504));
#271408=CARTESIAN_POINT('Ctrl Pts',(-48.9592137295291,2.59509833966803,
136.004119651047));
#271409=CARTESIAN_POINT('Ctrl Pts',(-49.2376613533419,5.77741858108801,
131.431627656171));
#271410=CARTESIAN_POINT('Ctrl Pts',(-49.5161089771548,3.65057338907646,
126.282707896514));
#271411=CARTESIAN_POINT('Ctrl Pts',(-49.7945566009678,-1.8309704070716,
125.288966092489));
#271412=CARTESIAN_POINT('Ctrl Pts',(-50.0730042247805,-5.62994184699806,
129.363602415007));
#271413=CARTESIAN_POINT('Ctrl Pts',(-50.3514518485936,-4.25527176748286,
134.762225140725));
#271414=CARTESIAN_POINT('Ctrl Pts',(-50.6298994724063,1.02978518476655,
136.52376372209));
#271415=CARTESIAN_POINT('Ctrl Pts',(-50.9083470962193,5.36851986001845,
133.029450258773));
#271416=CARTESIAN_POINT('Ctrl Pts',(-51.1867947200322,4.77384705068883,
127.490388116857));
#271417=CARTESIAN_POINT('Ctrl Pts',(-51.465242343845,-0.207757982829986,
124.996704806535));
#271418=CARTESIAN_POINT('Ctrl Pts',(-51.743689967658,-4.99844357966987,
127.839973466791));
#271419=CARTESIAN_POINT('Ctrl Pts',(-52.0221375914708,-5.19580371433717,
133.407369100245));
#271420=CARTESIAN_POINT('Ctrl Pts',(-52.3005852152837,-0.618474064651215,
136.58272710215));
#271421=CARTESIAN_POINT('Ctrl Pts',(-52.5790328390967,4.52720303631132,
134.448048593619));
#271422=CARTESIAN_POINT('Ctrl Pts',(-52.8574804629095,5.51260171306762,
128.964998839148));
#271423=CARTESIAN_POINT('Ctrl Pts',(-53.1359280867224,1.43218872108006,
125.172232701224));
#271424=CARTESIAN_POINT('Ctrl Pts',(-53.4143757105353,-3.96433573927151,
126.555116973674));
#271425=CARTESIAN_POINT('Ctrl Pts',(-53.6928233343482,-5.71782932379997,
131.842848567767));
#271426=CARTESIAN_POINT('Ctrl Pts',(-53.9712709581611,-2.21691709124776,
136.176260468582));
#271427=CARTESIAN_POINT('Ctrl Pts',(-54.249718581974,3.32123364574025,135.573158838211));
#271428=CARTESIAN_POINT('Ctrl Pts',(-54.5281662057869,5.80733291357678,
130.58776461181));
#271429=CARTESIAN_POINT('Ctrl Pts',(-54.8066138295998,2.95677693782102,
125.801411533396));
#271430=CARTESIAN_POINT('Ctrl Pts',(-55.0850614534126,-2.61091259720856,
125.612524255684));
#271431=CARTESIAN_POINT('Ctrl Pts',(-55.3635090772256,-5.77930100557468,
130.194680959234));
#271432=CARTESIAN_POINT('Ctrl Pts',(-55.6419567010384,-3.63679412436797,
135.337103484283));
#271433=CARTESIAN_POINT('Ctrl Pts',(-55.9204043248514,1.8477488898629,136.314156751619));
#271434=CARTESIAN_POINT('Ctrl Pts',(-56.1988519486642,5.63430094186134,
132.227976540264));
#271435=CARTESIAN_POINT('Ctrl Pts',(-56.4772995724772,4.24320567919224,
126.833562843453));
#271436=CARTESIAN_POINT('Ctrl Pts',(-56.7557471962901,-1.04718831053316,
125.088118316796));
#271437=CARTESIAN_POINT('Ctrl Pts',(-57.0341948201028,-5.3752674008715,
128.595621210585));
#271438=CARTESIAN_POINT('Ctrl Pts',(-57.3126424439159,-4.76373834622006,
134.13284771647));
#271439=CARTESIAN_POINT('Ctrl Pts',(-57.5910900677287,0.225433527051438,
136.611357184097));
#271440=CARTESIAN_POINT('Ctrl Pts',(-57.8695376915416,5.00744300200284,
133.753520494635));
#271441=CARTESIAN_POINT('Ctrl Pts',(-58.1479853153544,5.18785698530388,
128.185549952615));
#271442=CARTESIAN_POINT('Ctrl Pts',(-58.4264329391674,0.600883840013963,
125.024138475672));
#271443=CARTESIAN_POINT('Ctrl Pts',(-58.7048805629802,-4.53827219944114,
127.174468767579));
#271444=CARTESIAN_POINT('Ctrl Pts',(-58.9833281867932,-5.5069777945324,
132.660492339548));
#271445=CARTESIAN_POINT('Ctrl Pts',(-59.261775810606,-1.41503982726995,
136.440821536091));
#271446=CARTESIAN_POINT('Ctrl Pts',(-59.540223434419,3.97725061271504,135.041518504932));
#271447=CARTESIAN_POINT('Ctrl Pts',(-59.8186710582318,5.71464203910897,
129.748474371954));
#271448=CARTESIAN_POINT('Ctrl Pts',(-60.0971186820448,2.20055660734573,
125.425738115783));
#271449=CARTESIAN_POINT('Ctrl Pts',(-60.3755663058576,-3.3357328434014,
126.045693178431));
#271450=CARTESIAN_POINT('Ctrl Pts',(-60.6540139296705,-5.80664677067165,
131.038631143817));
#271451=CARTESIAN_POINT('Ctrl Pts',(-60.9324615534834,-2.94153598615947,
135.816285940328));
#271452=CARTESIAN_POINT('Ctrl Pts',(-61.2109091772963,2.62670266761142,
135.988226211385));
#271453=CARTESIAN_POINT('Ctrl Pts',(-61.4893568011092,5.78112989140647,
131.396447247635));
#271454=CARTESIAN_POINT('Ctrl Pts',(-61.767804424922,3.62298116889529,126.260569595891));
#271455=CARTESIAN_POINT('Ctrl Pts',(-62.046252048735,-1.86451025536104,
125.300213916535));
#271456=CARTESIAN_POINT('Ctrl Pts',(-62.3246996725479,-5.63860784133039,
129.39790016291));
#271457=CARTESIAN_POINT('Ctrl Pts',(-62.6031472963608,-4.23110028242386,
134.788054857702));
#271458=CARTESIAN_POINT('Ctrl Pts',(-62.8815949201736,1.0645817352901,136.517389160091));
#271459=CARTESIAN_POINT('Ctrl Pts',(-63.1600425439866,5.38196514598156,
132.99672932886));
#271460=CARTESIAN_POINT('Ctrl Pts',(-63.4384901677994,4.75358551113023,
127.461389755115));
#271461=CARTESIAN_POINT('Ctrl Pts',(-63.7169377916123,-0.243106982887504,
124.998077090756));
#271462=CARTESIAN_POINT('Ctrl Pts',(-63.9953854154252,-5.0163960360679,
127.870455334816));
#271463=CARTESIAN_POINT('Ctrl Pts',(-64.2738330392381,-5.17986219667218,
133.438949204482));
#271464=CARTESIAN_POINT('Ctrl Pts',(-64.552280663051,-0.583288048870894,
136.586384869579));
#271465=CARTESIAN_POINT('Ctrl Pts',(-64.8307282868638,4.54929932063727,
134.420422714664));
#271466=CARTESIAN_POINT('Ctrl Pts',(-65.1091759106768,5.50130286010717,
128.93147614697));
#271467=CARTESIAN_POINT('Ctrl Pts',(-65.3876235344896,1.39787782472419,
125.16361891226));
#271468=CARTESIAN_POINT('Ctrl Pts',(-65.6660711583025,-3.99012864145221,
126.579327739175));
#271469=CARTESIAN_POINT('Ctrl Pts',(-65.9445187821156,-5.71140181475477,
131.877635376998));
#271470=CARTESIAN_POINT('Ctrl Pts',(-66.2229664059283,-2.18417573778792,
136.189655943291));
#271471=CARTESIAN_POINT('Ctrl Pts',(-66.5014140297413,3.35020113928917,
135.552853191544));
#271472=CARTESIAN_POINT('Ctrl Pts',(-66.7798616535541,5.80590683578406,
130.552417741069));
#271473=CARTESIAN_POINT('Ctrl Pts',(-67.0583092773671,2.92626778451039,
125.783505486001));
#271474=CARTESIAN_POINT('Ctrl Pts',(-67.3367569011799,-2.64246840459962,
125.628513814431));
#271475=CARTESIAN_POINT('Ctrl Pts',(-67.6152045249929,-5.78290522164069,
130.229872500769));
#271476=CARTESIAN_POINT('Ctrl Pts',(-67.8936521488056,-3.60913465062,135.359157701137));
#271477=CARTESIAN_POINT('Ctrl Pts',(-68.1720997726187,1.88125434829088,
136.302806895912));
#271478=CARTESIAN_POINT('Ctrl Pts',(-68.4505473964314,5.64286250550667,
132.193652574919));
#271479=CARTESIAN_POINT('Ctrl Pts',(-68.7289950202444,4.21895568932047,
126.807806815805));
#271480=CARTESIAN_POINT('Ctrl Pts',(-69.0074426440573,-1.08196529790749,
125.094598758));
#271481=CARTESIAN_POINT('Ctrl Pts',(-69.2858902678701,-5.38861303330182,
128.628382911763));
#271482=CARTESIAN_POINT('Ctrl Pts',(-69.564337891683,-4.74338863947339,
134.161784274737));
#271483=CARTESIAN_POINT('Ctrl Pts',(-69.8427855154959,0.260778186613682,
136.609877316035));
#271484=CARTESIAN_POINT('Ctrl Pts',(-70.1212331393089,5.02530259892534,
133.722984126697));
#271485=CARTESIAN_POINT('Ctrl Pts',(-70.3996807631217,5.17181942250469,
128.154018515153));
#271486=CARTESIAN_POINT('Ctrl Pts',(-70.6781283869345,0.5656868542273,125.020587819316));
#271487=CARTESIAN_POINT('Ctrl Pts',(-70.9565760107477,-4.56028429774593,
127.202161772061));
#271488=CARTESIAN_POINT('Ctrl Pts',(-71.2350236345604,-5.49557696236377,
132.693980486629));
#271489=CARTESIAN_POINT('Ctrl Pts',(-71.5134712583732,-1.38070287242923,
136.449330854589));
#271490=CARTESIAN_POINT('Ctrl Pts',(-71.7919188821862,4.00296970618273,
135.017229346852));
#271491=CARTESIAN_POINT('Ctrl Pts',(-72.0703665059991,5.70810868075446,
129.71370728698));
#271492=CARTESIAN_POINT('Ctrl Pts',(-72.348814129812,2.16777463432419,125.412442356538));
#271493=CARTESIAN_POINT('Ctrl Pts',(-72.6272617536249,-3.36463839937136,
126.06608689813));
#271494=CARTESIAN_POINT('Ctrl Pts',(-72.9057093774378,-5.80511311576878,
131.073973510343));
#271495=CARTESIAN_POINT('Ctrl Pts',(-73.1841570012506,-2.91097247431594,
135.834099045416));
#271496=CARTESIAN_POINT('Ctrl Pts',(-73.4626046250635,2.65820966212185,
135.972140681676));
#271497=CARTESIAN_POINT('Ctrl Pts',(-73.7410522488765,5.78462697983096,
131.361244899111));
#271498=CARTESIAN_POINT('Ctrl Pts',(-74.0194998726893,3.59525469781404,
126.238599667113));
#271499=CARTESIAN_POINT('Ctrl Pts',(-74.2979474965022,-1.89798101353784,
125.31166569876));
#271500=CARTESIAN_POINT('Ctrl Pts',(-74.5763951203151,-5.64706489497548,
129.432250027724));
#271501=CARTESIAN_POINT('Ctrl Pts',(-74.854842744128,-4.20677201238788,
134.813736957424));
#271502=CARTESIAN_POINT('Ctrl Pts',(-75.1332903679409,1.09933883734644,
136.510802899716));
#271503=CARTESIAN_POINT('Ctrl Pts',(-75.4117379917539,5.39521100124704,
132.963927159917));
#271504=CARTESIAN_POINT('Ctrl Pts',(-75.6901856155667,4.73314782571214,
127.432515268386));
#271505=CARTESIAN_POINT('Ctrl Pts',(-75.9686332393795,-0.278446974526432,
124.99966452895));
#271506=CARTESIAN_POINT('Ctrl Pts',(-76.2470808631926,-5.03416260806588,
127.901045919781));
#271507=CARTESIAN_POINT('Ctrl Pts',(-76.5255284870053,-5.16372873730878,
133.470431683069));
#271508=CARTESIAN_POINT('Ctrl Pts',(-76.8039761108183,-0.548080419137594,
136.589828381972));
#271509=CARTESIAN_POINT('Ctrl Pts',(-77.0824237346311,4.57122702900371,
134.392662841198));
#271510=CARTESIAN_POINT('Ctrl Pts',(-77.360871358444,5.48980015434633,128.898022855216));
#271511=CARTESIAN_POINT('Ctrl Pts',(-77.639318982257,1.36351512949127,125.155214143056));
#271512=CARTESIAN_POINT('Ctrl Pts',(-77.9177666060698,-4.0157736879487,
126.603695064822));
#271513=CARTESIAN_POINT('Ctrl Pts',(-78.1962142298826,-5.70476266761487,
131.91238241564));
#271514=CARTESIAN_POINT('Ctrl Pts',(-78.4746618536957,-2.15135344889296,
136.202851863901));
#271515=CARTESIAN_POINT('Ctrl Pts',(-78.7531094775085,3.37904448990285,
135.532371587738));
#271516=CARTESIAN_POINT('Ctrl Pts',(-79.0315571013213,5.8042656179783,130.517080206165));
#271517=CARTESIAN_POINT('Ctrl Pts',(-79.3100047251342,2.8956501972711,125.765785488239));
#271518=CARTESIAN_POINT('Ctrl Pts',(-79.5884523489472,-2.67392629435197,
125.644695166086));
#271519=CARTESIAN_POINT('Ctrl Pts',(-79.8668999727601,-5.78629515002701,
130.265085330171));
#271520=CARTESIAN_POINT('Ctrl Pts',(-80.1453475965729,-3.58134143906054,
135.38104313831));
#271521=CARTESIAN_POINT('Ctrl Pts',(-80.4237952203859,1.91469009614739,
136.291253293255));
#271522=CARTESIAN_POINT('Ctrl Pts',(-80.7022428441988,5.65121497080658,
132.15927712885));
#271523=CARTESIAN_POINT('Ctrl Pts',(-80.9806904680116,4.19454936449412,
126.782198881926));
#271524=CARTESIAN_POINT('Ctrl Pts',(-81.2591380918246,-1.11670219266007,
125.10129077653));
#271525=CARTESIAN_POINT('Ctrl Pts',(-81.5375857156372,-5.40175898869456,
128.661225244595));
#271526=CARTESIAN_POINT('Ctrl Pts',(-81.8160333394505,-4.72286316471603,
134.190596422436));
#271527=CARTESIAN_POINT('Ctrl Pts',(-82.0944809632629,0.296113182944105,
136.608182322418));
#271528=CARTESIAN_POINT('Ctrl Pts',(-82.3729285870762,5.04297598141181,
133.692339608092));
#271529=CARTESIAN_POINT('Ctrl Pts',(-82.6513762108889,5.15559021603496,
128.122585287091));
#271530=CARTESIAN_POINT('Ctrl Pts',(-82.9298238347018,0.530468906706182,
125.017251482786));
#271531=CARTESIAN_POINT('Ctrl Pts',(-83.2082714585147,-4.58212741303929,
127.229988257347));
#271532=CARTESIAN_POINT('Ctrl Pts',(-83.4867190823277,-5.48397248956967,
132.72739861315));
#271533=CARTESIAN_POINT('Ctrl Pts',(-83.7651667061405,-1.34631475513585,
136.45763099664));
#271534=CARTESIAN_POINT('Ctrl Pts',(-84.0436143299535,4.02854046813582,
134.992784079373));
#271535=CARTESIAN_POINT('Ctrl Pts',(-84.3220619537663,5.70136380633342,
129.678980616565));
#271536=CARTESIAN_POINT('Ctrl Pts',(-84.6005095775792,2.13491233361711,
125.399346396808));
#271537=CARTESIAN_POINT('Ctrl Pts',(-84.8789572013921,-3.39341927742779,
126.086656196302));
#271538=CARTESIAN_POINT('Ctrl Pts',(-85.1574048252049,-5.80336435026449,
131.109305886265));
#271539=CARTESIAN_POINT('Ctrl Pts',(-85.4358524490179,-2.88030109531746,
135.851725771696));
#271540=CARTESIAN_POINT('Ctrl Pts',(-85.7143000728307,2.68961815569484,
135.955863657977));
#271541=CARTESIAN_POINT('Ctrl Pts',(-85.9927476966438,5.78790971677558,
131.326021915035));
#271542=CARTESIAN_POINT('Ctrl Pts',(-86.2711953204564,3.56739500324825,
126.216798924288));
#271543=CARTESIAN_POINT('Ctrl Pts',(-86.5496429442695,-1.93138144132926,
125.323321014816));
#271544=CARTESIAN_POINT('Ctrl Pts',(-86.8280905680822,-5.65531269455438,
129.466650736599));
#271545=CARTESIAN_POINT('Ctrl Pts',(-87.1065381918953,-4.18228785886808,
134.83927048823));
#271546=CARTESIAN_POINT('Ctrl Pts',(-87.3849858157081,1.13405520299706,
136.504005185026));
#271547=CARTESIAN_POINT('Ctrl Pts',(-87.663433439521,5.40825693498488,132.931044967442));
#271548=CARTESIAN_POINT('Ctrl Pts',(-87.9418810633338,4.71253475176078,
127.403765726628));
#271549=CARTESIAN_POINT('Ctrl Pts',(-88.2203286871468,-0.313776648210234,
125.00146706229));
#271550=CARTESIAN_POINT('Ctrl Pts',(-88.4987763109598,-5.05174263731727,
127.931744088139));
#271551=CARTESIAN_POINT('Ctrl Pts',(-88.7772239347726,-5.14740393407785,
133.501815369412));
#271552=CARTESIAN_POINT('Ctrl Pts',(-89.0556715585855,-0.512852480082647,
136.593057511728));
#271553=CARTESIAN_POINT('Ctrl Pts',(-89.3341191823985,4.59298534887173,
134.364770001874));
#271554=CARTESIAN_POINT('Ctrl Pts',(-89.6125668062112,5.47809402202166,
128.864640203508));
#271555=CARTESIAN_POINT('Ctrl Pts',(-89.8910144300243,1.32910190870433,
125.147018705051));
#271556=CARTESIAN_POINT('Ctrl Pts',(-90.169462053837,-4.04126992847403,
126.628218047677));
#271557=CARTESIAN_POINT('Ctrl Pts',(-90.44790967765,-5.69791212839678,131.947088396125));
#271558=CARTESIAN_POINT('Ctrl Pts',(-90.7263573014627,-2.1184514408047,
136.215847741432));
#271559=CARTESIAN_POINT('Ctrl Pts',(-91.0048049252757,3.40776262878029,
135.511714785749));
#271560=CARTESIAN_POINT('Ctrl Pts',(-91.2832525490887,5.80240932097568,
130.48175331654));
#271561=CARTESIAN_POINT('Ctrl Pts',(-91.5617001729014,2.86492531064864,
125.748252196732));
#271562=CARTESIAN_POINT('Ctrl Pts',(-91.8401477967144,-2.70528510078237,
125.661067711041));
#271563=CARTESIAN_POINT('Ctrl Pts',(-92.1185954205271,-5.78947066511866,
130.30031814262));
#271564=CARTESIAN_POINT('Ctrl Pts',(-92.3970430443404,-3.55341551957677,
135.402758984829));
#271565=CARTESIAN_POINT('Ctrl Pts',(-92.6754906681528,1.94805489445803,
136.279496371773));
#271566=CARTESIAN_POINT('Ctrl Pts',(-92.9539382919661,5.6593580282576,132.124851475851));
#271567=CARTESIAN_POINT('Ctrl Pts',(-93.2323859157787,4.16998760909852,
126.75673999073));
#271568=CARTESIAN_POINT('Ctrl Pts',(-93.5108335395918,-1.15139770760221,
125.10819412441));
#271569=CARTESIAN_POINT('Ctrl Pts',(-93.7892811634045,-5.41470477992152,
128.694146992097));
#271570=CARTESIAN_POINT('Ctrl Pts',(-94.0677287872175,-4.70216268252734,
134.219283091922));
#271571=CARTESIAN_POINT('Ctrl Pts',(-94.3461764110305,0.331437206691851,
136.606272266052));
#271572=CARTESIAN_POINT('Ctrl Pts',(-94.6246240348431,5.0604624945689,133.661588074364));
#271573=CARTESIAN_POINT('Ctrl Pts',(-94.9030716586564,5.13916996727372,
128.0912514332));
#271574=CARTESIAN_POINT('Ctrl Pts',(-95.1815192824688,0.495231302464415,
125.014129589715));
#271575=CARTESIAN_POINT('Ctrl Pts',(-95.459966906282,-4.60380073591605,
127.257947192314));
#271576=CARTESIAN_POINT('Ctrl Pts',(-95.7384145300948,-5.47216480615837,
132.760745480792));
#271577=CARTESIAN_POINT('Ctrl Pts',(-96.0168621539077,-1.31187674965409,
136.465721654678));
#271578=CARTESIAN_POINT('Ctrl Pts',(-96.2953097777207,4.05396195104042,
134.96818360832));
#271579=CARTESIAN_POINT('Ctrl Pts',(-96.5737574015334,5.69440766577999,
129.64429564752));
#271580=CARTESIAN_POINT('Ctrl Pts',(-96.8522050253465,2.10197092294792,
125.386450721867));
#271581=CARTESIAN_POINT('Ctrl Pts',(-97.1306526491593,-3.42207441108517,
126.107400310748));
#271582=CARTESIAN_POINT('Ctrl Pts',(-97.4091002729722,-5.80140053895979,
131.144626962327));
#271583=CARTESIAN_POINT('Ctrl Pts',(-97.6875478967851,-2.8495229857029,
135.869165466005));
#271584=CARTESIAN_POINT('Ctrl Pts',(-97.965995520598,2.72092698447821,135.93939574344));
#271585=CARTESIAN_POINT('Ctrl Pts',(-98.2444431444108,5.79097798059694,
131.290779600608));
#271586=CARTESIAN_POINT('Ctrl Pts',(-98.5228907682237,3.53940311754856,
126.195168175249));
#271587=CARTESIAN_POINT('Ctrl Pts',(-98.8013383920368,-1.96471030107164,
125.33517943281));
#271588=CARTESIAN_POINT('Ctrl Pts',(-99.0797860158496,-5.6633509344415,
129.501101014807));
#271589=CARTESIAN_POINT('Ctrl Pts',(-99.3582336396624,-4.15764872913354,
134.864654503967));
#271590=CARTESIAN_POINT('Ctrl Pts',(-99.6366812634755,1.16872954581563,
136.496996267908));
#271591=CARTESIAN_POINT('Ctrl Pts',(-99.9151288872883,5.42110246377302,
132.898083969897));
#271592=CARTESIAN_POINT('Ctrl Pts',(-100.193576511101,4.69174705310118,
127.375142195163));
#271593=CARTESIAN_POINT('Ctrl Pts',(-100.472024134914,-0.34909469478497,
125.003484623986));
#271594=CARTESIAN_POINT('Ctrl Pts',(-100.750471758727,-5.06913547238742,
127.96254870236));
#271595=CARTESIAN_POINT('Ctrl Pts',(-101.02891938254,-5.13088839190121,
133.533099100579));
#271596=CARTESIAN_POINT('Ctrl Pts',(-101.307367006353,-0.47760553709043,
136.596072139193));
#271597=CARTESIAN_POINT('Ctrl Pts',(-101.585814630166,4.61457347397855,
134.33674523027));
#271598=CARTESIAN_POINT('Ctrl Pts',(-101.864262253979,5.46618489690847,
128.831329428852));
#271599=CARTESIAN_POINT('Ctrl Pts',(-102.142709877791,1.29463943755703,
125.139032901931));
#271600=CARTESIAN_POINT('Ctrl Pts',(-102.421157501604,-4.06661641825637,
126.652895779031));
#271601=CARTESIAN_POINT('Ctrl Pts',(-102.699605125417,-5.69085045094906,
131.981752032413));
#271602=CARTESIAN_POINT('Ctrl Pts',(-102.97805274923,-2.08547093271925,
136.228643094318));
#271603=CARTESIAN_POINT('Ctrl Pts',(-103.256500373043,3.43635449176034,
135.490883551018));
#271604=CARTESIAN_POINT('Ctrl Pts',(-103.534947996856,5.80033801356182,
130.446438381249));
#271605=CARTESIAN_POINT('Ctrl Pts',(-103.813395620669,2.83409426316523,
125.730906261181));
#271606=CARTESIAN_POINT('Ctrl Pts',(-104.091843244482,-2.73654366187847,
125.677630842606));
#271607=CARTESIAN_POINT('Ctrl Pts',(-104.370290868295,-5.79243164924577,
130.335569632546));
#271608=CARTESIAN_POINT('Ctrl Pts',(-104.648738492108,-3.52535792697413,
135.424304436005));
#271609=CARTESIAN_POINT('Ctrl Pts',(-104.92718611592,1.98134750687769,136.267536567122));
#271610=CARTESIAN_POINT('Ctrl Pts',(-105.205633739733,5.66729137611554,
132.090376891579));
#271611=CARTESIAN_POINT('Ctrl Pts',(-105.484081363546,4.14527133327901,
126.731431085605));
#271612=CARTESIAN_POINT('Ctrl Pts',(-105.762528987359,-1.18605055707886,
125.115308545834));
#271613=CARTESIAN_POINT('Ctrl Pts',(-106.040976611172,-5.42744992727162,
128.72714693434));
#271614=CARTESIAN_POINT('Ctrl Pts',(-106.319424234985,-4.68128795997122,
134.247843220201));
#271615=CARTESIAN_POINT('Ctrl Pts',(-106.597871858798,0.366748948912009,
136.604147217717));
#271616=CARTESIAN_POINT('Ctrl Pts',(-106.876319482611,5.07776149042729,
133.630730665021));
#271617=CARTESIAN_POINT('Ctrl Pts',(-107.154767106424,5.12255928467941,
128.060018114567));
#271618=CARTESIAN_POINT('Ctrl Pts',(-107.433214730236,0.45997534724462,
125.011222255784));
#271619=CARTESIAN_POINT('Ctrl Pts',(-107.711662354049,-4.62530346326349,
127.286037540936));
#271620=CARTESIAN_POINT('Ctrl Pts',(-107.990109977862,-5.46015434966779,
132.794019853873));
#271621=CARTESIAN_POINT('Ctrl Pts',(-108.268557601675,-1.2773901320969,
136.473602528901));
#271622=CARTESIAN_POINT('Ctrl Pts',(-108.547005225488,4.07923321289408,
134.943428845277));
#271623=CARTESIAN_POINT('Ctrl Pts',(-108.825452849301,5.6872405168564,129.609653665109));
#271624=CARTESIAN_POINT('Ctrl Pts',(-109.103900473114,2.06895162297316,
125.373755809571));
#271625=CARTESIAN_POINT('Ctrl Pts',(-109.382348096927,-3.45060273851677,
126.128318472786));
#271626=CARTESIAN_POINT('Ctrl Pts',(-109.66079572074,-5.79922175462486,
131.179935429694));
#271627=CARTESIAN_POINT('Ctrl Pts',(-109.939243344552,-2.81863928596571,
135.886417482107));
#271628=CARTESIAN_POINT('Ctrl Pts',(-110.217690968365,2.7521349883118,135.922737548286));
#271629=CARTESIAN_POINT('Ctrl Pts',(-110.496138592178,5.79383165759959,
131.255519261747));
#271630=CARTESIAN_POINT('Ctrl Pts',(-110.774586215991,3.51128007796473,
126.17370822153));
#271631=CARTESIAN_POINT('Ctrl Pts',(-111.053033839804,-1.99796635775128,
125.347240513325));
#271632=CARTESIAN_POINT('Ctrl Pts',(-111.331481463617,-5.67117931677705,
129.535599585778));
#271633=CARTESIAN_POINT('Ctrl Pts',(-111.60992908743,-4.13285553619637,
134.889888064022));
#271634=CARTESIAN_POINT('Ctrl Pts',(-111.888376711243,1.20336058093108,
136.489776408084));
#271635=CARTESIAN_POINT('Ctrl Pts',(-112.166824335056,5.43374711161577,
132.865045388662));
#271636=CARTESIAN_POINT('Ctrl Pts',(-112.445271958868,4.67078550002918,
127.34664573465));
#271637=CARTESIAN_POINT('Ctrl Pts',(-112.723719582681,-0.384399805526852,
125.005717139274));
#271638=CARTESIAN_POINT('Ctrl Pts',(-113.002167206494,-5.08634046877848,
127.993458620965));
#271639=CARTESIAN_POINT('Ctrl Pts',(-113.280614830307,-5.11418272276831,
133.564281717336));
#271640=CARTESIAN_POINT('Ctrl Pts',(-113.55906245412,-0.442340896249408,
136.598872152659));
#271641=CARTESIAN_POINT('Ctrl Pts',(-113.837510077933,4.63599060436829,
134.308589564856));
#271642=CARTESIAN_POINT('Ctrl Pts',(-114.115957701746,5.45407322030374,
128.798091765594));
#271643=CARTESIAN_POINT('Ctrl Pts',(-114.394405325558,1.26012899306928,
125.131257029612));
#271644=CARTESIAN_POINT('Ctrl Pts',(-114.672852949372,-4.09181221807183,
126.677727344441));
#271645=CARTESIAN_POINT('Ctrl Pts',(-114.951300573184,-5.68357789694507,
132.016372040028));
#271646=CARTESIAN_POINT('Ctrl Pts',(-115.229748196997,-2.05241314674147,
136.241237448422));
#271647=CARTESIAN_POINT('Ctrl Pts',(-115.50819582081,3.46481901936097,135.469878655457));
#271648=CARTESIAN_POINT('Ctrl Pts',(-115.786643444623,5.79805177248978,
130.411136708898));
#271649=CARTESIAN_POINT('Ctrl Pts',(-116.065091068436,2.80315819727665,
125.713748324348));
#271650=CARTESIAN_POINT('Ctrl Pts',(-116.343538692249,-2.76770081934284,
125.694383947029));
#271651=CARTESIAN_POINT('Ctrl Pts',(-116.621986316062,-5.79517799268792,
130.370838493694));
#271652=CARTESIAN_POINT('Ctrl Pts',(-116.900433939875,-3.49716970093708,
135.445678693465));
#271653=CARTESIAN_POINT('Ctrl Pts',(-117.178881563688,2.0145666997373,136.255374322477));
#271654=CARTESIAN_POINT('Ctrl Pts',(-117.4573291875,5.67501472040751,132.055854653499));
#271655=CARTESIAN_POINT('Ctrl Pts',(-117.735776811314,4.12040145290537,
126.706273104381));
#271656=CARTESIAN_POINT('Ctrl Pts',(-118.014224435126,-1.22065945701595,
125.122633777175));
#271657=CARTESIAN_POINT('Ctrl Pts',(-118.29267205894,-5.43999395846872,
128.760223848501));
#271658=CARTESIAN_POINT('Ctrl Pts',(-118.571119682752,-4.6602397705682,
134.276275748964));
#271659=CARTESIAN_POINT('Ctrl Pts',(-118.849567306565,0.402047101114997,
136.601807256156));
#271660=CARTESIAN_POINT('Ctrl Pts',(-119.128014930377,5.09487232796628,
133.599768523497));
#271661=CARTESIAN_POINT('Ctrl Pts',(-119.406462554191,5.10575878376697,
128.028886488555));
#271662=CARTESIAN_POINT('Ctrl Pts',(-119.684910178003,0.424702347469154,
125.008529588725));
#271663=CARTESIAN_POINT('Ctrl Pts',(-119.963357801817,-4.64663479828973,
127.314258262312));
#271664=CARTESIAN_POINT('Ctrl Pts',(-120.241805425629,-5.44794156515001,
132.827220499399));
#271665=CARTESIAN_POINT('Ctrl Pts',(-120.520253049442,-1.24285618037906,
136.48127332728));
#271666=CARTESIAN_POINT('Ctrl Pts',(-120.798700673255,4.10435331726091,
134.918520707537));
#271667=CARTESIAN_POINT('Ctrl Pts',(-121.077148297068,5.67986262514396,
129.575055953004));
#271668=CARTESIAN_POINT('Ctrl Pts',(-121.355595920881,2.03585565723516,
125.361262130332));
#271669=CARTESIAN_POINT('Ctrl Pts',(-121.634043544694,-3.47900320259493,
126.149409907283));
#271670=CARTESIAN_POINT('Ctrl Pts',(-121.912491168507,-5.79682807799514,
131.215229979999));
#271671=CARTESIAN_POINT('Ctrl Pts',(-122.19093879232,-2.78765114051323,
135.903481180724));
#271672=CARTESIAN_POINT('Ctrl Pts',(-122.469386416133,2.78324101077128,
135.905889689793));
#271673=CARTESIAN_POINT('Ctrl Pts',(-122.747834039945,5.79647064203949,
131.220242205036));
#271674=CARTESIAN_POINT('Ctrl Pts',(-123.026281663758,3.48302692660634,
126.152419858339));
#271675=CARTESIAN_POINT('Ctrl Pts',(-123.304729287571,-2.03114837905279,
125.359503809431));
#271676=CARTESIAN_POINT('Ctrl Pts',(-123.583176911384,-5.67879755147744,
129.570145171156));
#271677=CARTESIAN_POINT('Ctrl Pts',(-123.861624535197,-4.10790919877744,
134.914970233354));
#271678=CARTESIAN_POINT('Ctrl Pts',(-124.14007215901,1.23794702507767,136.482345873087));
#271679=CARTESIAN_POINT('Ctrl Pts',(-124.418519782823,5.44619040996103,
132.831930447996));
#271680=CARTESIAN_POINT('Ctrl Pts',(-124.696967406636,4.64965086928273,
127.318277401031));
#271681=CARTESIAN_POINT('Ctrl Pts',(-124.975415030448,-0.419690672193134,
125.00816452543));
#271682=CARTESIAN_POINT('Ctrl Pts',(-125.253862654262,-5.10335698895296,
128.024472698579));
#271683=CARTESIAN_POINT('Ctrl Pts',(-125.532310278074,-5.09728754571388,
133.595362064203));
#271684=CARTESIAN_POINT('Ctrl Pts',(-125.810757901887,-0.407059864303788,
136.601457448367));
#271685=CARTESIAN_POINT('Ctrl Pts',(-126.0892055257,4.65723594642128,134.280304048949));
#271686=CARTESIAN_POINT('Ctrl Pts',(-126.367653149513,5.44175944101008,
128.764928445366));
#271687=CARTESIAN_POINT('Ctrl Pts',(-126.646100773326,1.22557185403828,
125.123691376234));
#271688=CARTESIAN_POINT('Ctrl Pts',(-126.924548397139,-4.11685639428078,
126.702711823764));
#271689=CARTESIAN_POINT('Ctrl Pts',(-127.202996020952,-5.67609473587197,
132.050947136115));
#271690=CARTESIAN_POINT('Ctrl Pts',(-127.481443644765,-2.01927930784003,
136.253630337055));
#271691=CARTESIAN_POINT('Ctrl Pts',(-127.759891268577,3.4931551568182,135.44870087741));
#271692=CARTESIAN_POINT('Ctrl Pts',(-128.038338892391,5.79555068247735,
130.375849607603));
#271693=CARTESIAN_POINT('Ctrl Pts',(-128.316786516203,2.77211825933019,
125.696779022025));
#271694=CARTESIAN_POINT('Ctrl Pts',(-128.595234140016,-2.7987554186355,
125.711326403516));
#271695=CARTESIAN_POINT('Ctrl Pts',(-128.873681763829,-5.79770959367839,
130.406123419165));
#271696=CARTESIAN_POINT('Ctrl Pts',(-129.152129387642,-3.46885188599067,
135.466880965177));
#271697=CARTESIAN_POINT('Ctrl Pts',(-129.430577011455,2.04771124208698,
136.243010088514));
#271698=CARTESIAN_POINT('Ctrl Pts',(-129.709024635268,5.68252777494204,
132.021286040849));
#271699=CARTESIAN_POINT('Ctrl Pts',(-129.98747225908,4.09537888954061,126.681266979298));
#271700=CARTESIAN_POINT('Ctrl Pts',(-130.265919882893,-1.25522312496795,
125.130169546993));
#271701=CARTESIAN_POINT('Ctrl Pts',(-130.544367506706,-5.45233640868912,
128.793376508901));
#271702=CARTESIAN_POINT('Ctrl Pts',(-130.822815130519,-4.63901889426667,
134.304579624636));
#271703=CARTESIAN_POINT('Ctrl Pts',(-131.101262754332,0.437330355314798,
136.599252468079));
#271704=CARTESIAN_POINT('Ctrl Pts',(-131.379710378145,5.11179437313754,
133.568702797104));
#271705=CARTESIAN_POINT('Ctrl Pts',(-131.658158001958,5.08876908708517,
127.997857708758));
#271706=CARTESIAN_POINT('Ctrl Pts',(-131.936605625771,0.389413610192037,
125.006051688315));
#271707=CARTESIAN_POINT('Ctrl Pts',(-132.215053249584,-4.66779395055513,
127.342608310716));
#271708=CARTESIAN_POINT('Ctrl Pts',(-132.493500873397,-5.43552690515385,
132.860346187109));
#271709=CARTESIAN_POINT('Ctrl Pts',(-132.77194849721,-1.20827617416795,
136.488733765571));
#271710=CARTESIAN_POINT('Ctrl Pts',(-133.050396121022,4.12932133330617,
134.893460118082));
#271711=CARTESIAN_POINT('Ctrl Pts',(-133.328843744835,5.67227426403318,
129.540503793235));
#271712=CARTESIAN_POINT('Ctrl Pts',(-133.607291368648,2.00268425211708,
125.348970147109));
#271713=CARTESIAN_POINT('Ctrl Pts',(-133.885738992461,-3.50727475093002,
126.170673832692));
#271714=CARTESIAN_POINT('Ctrl Pts',(-134.164186616274,-5.79421959776922,
131.25050930539));
#271715=CARTESIAN_POINT('Ctrl Pts',(-134.442634240087,-2.75655969762259,
135.920355929551));
#271716=CARTESIAN_POINT('Ctrl Pts',(-134.7210818639,2.81424389921159,135.888852792264));
#271717=CARTESIAN_POINT('Ctrl Pts',(-134.999529487713,5.79889483612785,
131.18494973768));
#271718=CARTESIAN_POINT('Ctrl Pts',(-135.277977111526,3.45464471040472,
126.131303874523));
#271719=CARTESIAN_POINT('Ctrl Pts',(-135.556424735338,-2.06425513540386,
125.371968866708));
#271720=CARTESIAN_POINT('Ctrl Pts',(-135.834872359151,-5.68620535624619,
129.604736490841));
#271721=CARTESIAN_POINT('Ctrl Pts',(-136.113319982964,-4.08281064127246,
134.939900082537));
#271722=CARTESIAN_POINT('Ctrl Pts',(-136.391767606777,1.27248759664198,
136.474704938258));
#271723=CARTESIAN_POINT('Ctrl Pts',(-136.67021523059,5.45843189771781,132.798740374984));
#271724=CARTESIAN_POINT('Ctrl Pts',(-136.948662854403,4.62834394401342,
127.290038245509));
#271725=CARTESIAN_POINT('Ctrl Pts',(-137.227110478216,-0.454965987067202,
125.010826691762));
#271726=CARTESIAN_POINT('Ctrl Pts',(-137.505558102029,-5.12018440235748,
128.055589785961));
#271727=CARTESIAN_POINT('Ctrl Pts',(-137.784005725841,-5.0802034867949,
133.626338989485));
#271728=CARTESIAN_POINT('Ctrl Pts',(-138.062453349655,-0.371763748605222,
136.603827930521));
#271729=CARTESIAN_POINT('Ctrl Pts',(-138.340900973467,4.67830871288359,
134.251889730681));
#271730=CARTESIAN_POINT('Ctrl Pts',(-138.61934859728,5.42924401531914,128.731840697047));
#271731=CARTESIAN_POINT('Ctrl Pts',(-138.897796221093,1.19096930099152,
125.116336222143));
#271732=CARTESIAN_POINT('Ctrl Pts',(-139.176243844906,-4.14174801886209,
126.727848291193));
#271733=CARTESIAN_POINT('Ctrl Pts',(-139.454691468719,-5.66840124502105,
132.085476039479));
#271734=CARTESIAN_POINT('Ctrl Pts',(-139.733139092532,-1.98607064380098,
136.265821300996));
#271735=CARTESIAN_POINT('Ctrl Pts',(-140.011586716345,3.52136185412693,
135.427351001626));
#271736=CARTESIAN_POINT('Ctrl Pts',(-140.290034340158,5.79283483620279,
130.340578384942));
#271737=CARTESIAN_POINT('Ctrl Pts',(-140.56848196397,2.7409755995222,125.679998983016));
#271738=CARTESIAN_POINT('Ctrl Pts',(-140.846929587784,-2.82970630901691,
125.72845758426));
#271739=CARTESIAN_POINT('Ctrl Pts',(-141.125377211596,-5.80002635840773,
130.441423101462));
#271740=CARTESIAN_POINT('Ctrl Pts',(-141.403824835409,-3.44040553146196,
135.487910465481));
#271741=CARTESIAN_POINT('Ctrl Pts',(-141.682272459222,2.08077990574355,
136.230444323395));
#271742=CARTESIAN_POINT('Ctrl Pts',(-141.960720083035,5.68983026132012,
131.986672334579));
#271743=CARTESIAN_POINT('Ctrl Pts',(-142.239167706848,4.07020457040501,
126.656413636965));
#271744=CARTESIAN_POINT('Ctrl Pts',(-142.517615330661,-1.289740280165,125.137915576048));
#271745=CARTESIAN_POINT('Ctrl Pts',(-142.796062954474,-5.46447682057862,
128.826603687055));
#271746=CARTESIAN_POINT('Ctrl Pts',(-143.074510578287,-4.61762611741445,
134.332753798405));
#271747=CARTESIAN_POINT('Ctrl Pts',(-143.352958202099,0.472597404077474,
136.596482948152));
#271748=CARTESIAN_POINT('Ctrl Pts',(-143.631405825913,5.12852699888841,
133.537534636997));
#271749=CARTESIAN_POINT('Ctrl Pts',(-143.909853449725,5.07159082419343,
127.966932924958));
#271750=CARTESIAN_POINT('Ctrl Pts',(-144.188301073538,0.354110443050382,
125.003788646376));
#271751=CARTESIAN_POINT('Ctrl Pts',(-144.466748697351,-4.6887801359991,
127.371086635623));
#271752=CARTESIAN_POINT('Ctrl Pts',(-144.745196321164,-5.4229108297093,
132.893395689516));
#271753=CARTESIAN_POINT('Ctrl Pts',(-145.023643944977,-1.17365139483885,
136.495983567324));
#271754=CARTESIAN_POINT('Ctrl Pts',(-145.30209156879,4.15413633583088,134.868248005541));
#271755=CARTESIAN_POINT('Ctrl Pts',(-145.580539192603,5.66447571471356,
129.505998466145));
#271756=CARTESIAN_POINT('Ctrl Pts',(-145.858986816416,1.96943863679757,
125.336880315387));
#271757=CARTESIAN_POINT('Ctrl Pts',(-146.137434440228,-3.53541633590941,
126.192109461069));
#271758=CARTESIAN_POINT('Ctrl Pts',(-146.415882064041,-5.79139641060527,
131.285772098575));
#271759=CARTESIAN_POINT('Ctrl Pts',(-146.694329687854,-2.72536610939861,
135.937041103293));
#271760=CARTESIAN_POINT('Ctrl Pts',(-146.972777311667,2.84514250480927,
135.871627487008));
#271761=CARTESIAN_POINT('Ctrl Pts',(-147.25122493548,5.80110415003576,131.149643167454));
#271762=CARTESIAN_POINT('Ctrl Pts',(-147.529672559293,3.42613448107249,
126.110361052543));
#271763=CARTESIAN_POINT('Ctrl Pts',(-147.808120183106,-2.09728540002206,
125.38463522326));
#271764=CARTESIAN_POINT('Ctrl Pts',(-148.086567806919,-5.69340245658434,
129.639372263039));
#271765=CARTESIAN_POINT('Ctrl Pts',(-148.365015430732,-4.05756079371773,
134.964676687782));
#271766=CARTESIAN_POINT('Ctrl Pts',(-148.643463054544,1.30698101571045,
136.466853886735));
#271767=CARTESIAN_POINT('Ctrl Pts',(-148.921910678358,5.47047112127328,
132.765476399497));
#271768=CARTESIAN_POINT('Ctrl Pts',(-149.20035830217,4.60686551375719,127.261929314495));
#271769=CARTESIAN_POINT('Ctrl Pts',(-149.478805925983,-0.49022444300932,
125.013703539625));
#271770=CARTESIAN_POINT('Ctrl Pts',(-149.757253549796,-5.13682208544599,
128.086808730058));
#271771=CARTESIAN_POINT('Ctrl Pts',(-150.035701173609,-5.06293117906749,
133.657211345319));
#271772=CARTESIAN_POINT('Ctrl Pts',(-150.314148797422,-0.336453857064764,
136.605983511281));
#271773=CARTESIAN_POINT('Ctrl Pts',(-150.592596421235,4.69920812289605,
134.223347662954));
#271774=CARTESIAN_POINT('Ctrl Pts',(-150.871044045047,5.41652740699458,
128.698829746717));
#271775=CARTESIAN_POINT('Ctrl Pts',(-151.14949166886,1.15632261613933,125.109191839888));
#271776=CARTESIAN_POINT('Ctrl Pts',(-151.427939292673,-4.1664861694474,
126.753135815284));
#271777=CARTESIAN_POINT('Ctrl Pts',(-151.706386916486,-5.66049770947745,
132.119957470642));
#271778=CARTESIAN_POINT('Ctrl Pts',(-151.984834540299,-1.95278838518384,
136.277809888502));
#271779=CARTESIAN_POINT('Ctrl Pts',(-152.263282164112,3.54943806607717,
135.405829819234));
#271780=CARTESIAN_POINT('Ctrl Pts',(-152.541729787925,5.78990433430307,
130.3053243479));
#271781=CARTESIAN_POINT('Ctrl Pts',(-152.820177411738,2.70973137185537,
125.663408829112));
#271782=CARTESIAN_POINT('Ctrl Pts',(-153.09862503555,-2.86055234359039,
125.745776854456));
#271783=CARTESIAN_POINT('Ctrl Pts',(-153.377072659364,-5.80212820102742,
130.476736232542));
#271784=CARTESIAN_POINT('Ctrl Pts',(-153.655520283176,-3.41183169144105,
135.508766415124));
#271785=CARTESIAN_POINT('Ctrl Pts',(-153.933967906989,2.1137714653355,136.21767749275));
#271786=CARTESIAN_POINT('Ctrl Pts',(-154.212415530802,5.69692190894542,
131.952014817313));
#271787=CARTESIAN_POINT('Ctrl Pts',(-154.490863154615,4.04487942834225,
126.631713998332));
#271788=CARTESIAN_POINT('Ctrl Pts',(-154.769310778428,-1.32420964356211,
125.145871577308));
#271789=CARTESIAN_POINT('Ctrl Pts',(-155.047758402241,-5.47641474427016,
128.859904151722));
#271790=CARTESIAN_POINT('Ctrl Pts',(-155.326206026054,-4.59606223272787,
134.360797226267));
#271791=CARTESIAN_POINT('Ctrl Pts',(-155.604653649866,0.507846940569522,
136.593498799002));
#271792=CARTESIAN_POINT('Ctrl Pts',(-155.88310127368,5.14506958518534,133.50626519812));
#271793=CARTESIAN_POINT('Ctrl Pts',(-156.161548897493,5.05422463163864,
127.936113283085));
#271794=CARTESIAN_POINT('Ctrl Pts',(-156.439996521305,0.318794154216047,
125.001740546765));
#271795=CARTESIAN_POINT('Ctrl Pts',(-156.718444145118,-4.70959257697085,
127.399692181761));
#271796=CARTESIAN_POINT('Ctrl Pts',(-156.996891768931,-5.41009380630968,
132.926367781962));
#271797=CARTESIAN_POINT('Ctrl Pts',(-157.275339392744,-1.1389831254257,
136.503022463895));
#271798=CARTESIAN_POINT('Ctrl Pts',(-157.553787016557,4.17879740530553,
134.84288530416));
#271799=CARTESIAN_POINT('Ctrl Pts',(-157.83223464037,5.65646726616335,129.471541250343));
#271800=CARTESIAN_POINT('Ctrl Pts',(-158.110682264183,1.93612004320555,
125.324993083158));
#271801=CARTESIAN_POINT('Ctrl Pts',(-158.389129887996,-3.56342691473634,
126.213715998108));
#271802=CARTESIAN_POINT('Ctrl Pts',(-158.667577511808,-5.78835862111754,
131.321017052882));
#271803=CARTESIAN_POINT('Ctrl Pts',(-158.946025135621,-2.69407153173119,
135.95353608367));
#271804=CARTESIAN_POINT('Ctrl Pts',(-159.224472759434,2.87593568260513,
135.854214412314));
#271805=CARTESIAN_POINT('Ctrl Pts',(-159.502920383247,5.80309850189603,
131.114323802656));
#271806=CARTESIAN_POINT('Ctrl Pts',(-159.78136800706,3.39749729506709,126.089592168444));
#271807=CARTESIAN_POINT('Ctrl Pts',(-160.059815630873,-2.13023794895846,
125.39750240973));
#271808=CARTESIAN_POINT('Ctrl Pts',(-160.338263254686,-5.70038858580074,
129.674051204309));
#271809=CARTESIAN_POINT('Ctrl Pts',(-160.616710878499,-4.03216059175559,
134.989299130986));
#271810=CARTESIAN_POINT('Ctrl Pts',(-160.895158502312,1.34142600411673,
136.458793009441));
#271811=CARTESIAN_POINT('Ctrl Pts',(-161.173606126125,5.48230763450959,
132.732139754142));
#271812=CARTESIAN_POINT('Ctrl Pts',(-161.452053749937,4.58521637440516,
127.233951649575));
#271813=CARTESIAN_POINT('Ctrl Pts',(-161.730501373751,-0.525464733504406,
125.016794962416));
#271814=CARTESIAN_POINT('Ctrl Pts',(-162.008948997563,-5.15326942170307,
128.118128374039));
#271815=CARTESIAN_POINT('Ctrl Pts',(-162.287396621376,-5.04547126256333,
133.687977987722));
#271816=CARTESIAN_POINT('Ctrl Pts',(-162.565844245189,-0.301131498102361,
136.607924110772));
#271817=CARTESIAN_POINT('Ctrl Pts',(-162.844291869002,4.71993340202341,
134.194678903404));
#271818=CARTESIAN_POINT('Ctrl Pts',(-163.122739492814,5.40361008725504,
128.665896817606));
#271819=CARTESIAN_POINT('Ctrl Pts',(-163.401187116628,1.12163308332736,
125.102258494207));
#271820=CARTESIAN_POINT('Ctrl Pts',(-163.67963474044,-4.19106992935549,
126.778573459));
#271821=CARTESIAN_POINT('Ctrl Pts',(-163.958082364253,-5.65238442210956,
132.154390151878));
#271822=CARTESIAN_POINT('Ctrl Pts',(-164.236529988066,-1.91943376527495,
136.289595655332));
#271823=CARTESIAN_POINT('Ctrl Pts',(-164.514977611879,3.57738275229458,
135.384138127707));
#271824=CARTESIAN_POINT('Ctrl Pts',(-164.793425235692,5.78675928536899,
130.270088802833));
#271825=CARTESIAN_POINT('Ctrl Pts',(-165.071872859505,2.67838673409632,
125.647009175068));
#271826=CARTESIAN_POINT('Ctrl Pts',(-165.350320483318,-2.89129237934434,
125.763283572333));
#271827=CARTESIAN_POINT('Ctrl Pts',(-165.628768107131,-5.80401504365309,
130.512061503863));
#271828=CARTESIAN_POINT('Ctrl Pts',(-165.907215730944,-3.38313142474212,
135.52944804128));
#271829=CARTESIAN_POINT('Ctrl Pts',(-166.185663354757,2.14668469834846,
136.204710069657));
#271830=CARTESIAN_POINT('Ctrl Pts',(-166.464110978569,5.70380245503433,
131.917314773299));
#271831=CARTESIAN_POINT('Ctrl Pts',(-166.742558602383,4.01940440178476,
126.607168978656));
#271832=CARTESIAN_POINT('Ctrl Pts',(-167.021006226195,-1.3586299378839,
125.15403725596));
#271833=CARTESIAN_POINT('Ctrl Pts',(-167.299453850008,-5.48814973739939,
128.893276668938));
#271834=CARTESIAN_POINT('Ctrl Pts',(-167.577901473821,-4.57432803926507,
134.388708869063));
#271835=CARTESIAN_POINT('Ctrl Pts',(-167.856349097634,0.543077658606429,
136.590300131209));
#271836=CARTESIAN_POINT('Ctrl Pts',(-168.134796721447,5.16142151903669,
133.474895639175));
#271837=CARTESIAN_POINT('Ctrl Pts',(-168.413244345259,5.03667115293141,
127.905399925171));
#271838=CARTESIAN_POINT('Ctrl Pts',(-168.691691969073,0.283466052347084,
124.999907465374));
#271839=CARTESIAN_POINT('Ctrl Pts',(-168.970139592885,-4.7302305022577,
127.42842388914));
#271840=CARTESIAN_POINT('Ctrl Pts',(-169.248587216698,-5.39707630989451,
132.959261242652));
#271841=CARTESIAN_POINT('Ctrl Pts',(-169.527034840511,-1.10427265057399,
136.509850194457));
#271842=CARTESIAN_POINT('Ctrl Pts',(-169.805482464324,4.20330362790601,
134.81737295376));
#271843=CARTESIAN_POINT('Ctrl Pts',(-170.083930088137,5.6482492151383,129.437133422652));
#271844=CARTESIAN_POINT('Ctrl Pts',(-170.36237771195,1.90272970597286,125.313308890908));
#271845=CARTESIAN_POINT('Ctrl Pts',(-170.640825335763,-3.59130544946847,
126.235492643171));
#271846=CARTESIAN_POINT('Ctrl Pts',(-170.919272959575,-5.78510634187241,
131.356242862295));
#271847=CARTESIAN_POINT('Ctrl Pts',(-171.197720583389,-2.66267712425244,
135.969840259458));
#271848=CARTESIAN_POINT('Ctrl Pts',(-171.476168207202,2.90662229154664,
135.836614213432));
#271849=CARTESIAN_POINT('Ctrl Pts',(-171.754615831014,5.80487781780722,
131.07899295206));
#271850=CARTESIAN_POINT('Ctrl Pts',(-172.033063454828,3.36873421355001,
126.068997991823));
#271851=CARTESIAN_POINT('Ctrl Pts',(-172.31151107864,-2.16311156114431,
125.410569949319));
#271852=CARTESIAN_POINT('Ctrl Pts',(-172.589958702453,-5.70716348502144,
129.70877202961));
#271853=CARTESIAN_POINT('Ctrl Pts',(-172.868406326266,-4.00661097660031,
135.013766499754));
#271854=CARTESIAN_POINT('Ctrl Pts',(-173.146853950079,1.3758212854888,136.450522605077));
#271855=CARTESIAN_POINT('Ctrl Pts',(-173.425301573892,5.49394099882038,
132.698731674224));
#271856=CARTESIAN_POINT('Ctrl Pts',(-173.703749197705,4.56339732817417,
127.206106287473));
#271857=CARTESIAN_POINT('Ctrl Pts',(-173.982196821517,-0.560685552710569,
125.02010084558));
#271858=CARTESIAN_POINT('Ctrl Pts',(-174.260644445331,-5.1695258016666,
128.149547557344));
#271859=CARTESIAN_POINT('Ctrl Pts',(-174.539092069143,-5.02782438426607,
133.718637776622));
#271860=CARTESIAN_POINT('Ctrl Pts',(-174.817539692956,-0.265797980601551,
136.609649657082));
#271861=CARTESIAN_POINT('Ctrl Pts',(-175.095987316769,4.74048378228282,
134.165884514362));
#271862=CARTESIAN_POINT('Ctrl Pts',(-175.374434940582,5.39049253475655,
128.633043130058));
#271863=CARTESIAN_POINT('Ctrl Pts',(-175.652882564395,1.08690198798901,
125.095536442018));
#271864=CARTESIAN_POINT('Ctrl Pts',(-175.931330188208,-4.21549838762608,
126.80416027974));
#271865=CARTESIAN_POINT('Ctrl Pts',(-176.209777812021,-5.64406168355824,
132.188772807274));
#271866=CARTESIAN_POINT('Ctrl Pts',(-176.488225435833,-1.886008020042,136.301178164761));
#271867=CARTESIAN_POINT('Ctrl Pts',(-176.766673059646,3.60519487727851,
135.362276730843));
#271868=CARTESIAN_POINT('Ctrl Pts',(-177.045120683459,5.78339980594152,
130.234873055403));
#271869=CARTESIAN_POINT('Ctrl Pts',(-177.323568307272,2.64694284773159,
125.630800628577));
#271870=CARTESIAN_POINT('Ctrl Pts',(-177.602015931085,-2.92192527719638,
125.780977089175));
#271871=CARTESIAN_POINT('Ctrl Pts',(-177.880463554898,-5.80568681636668,
130.547397606436));
#271872=CARTESIAN_POINT('Ctrl Pts',(-178.158911178711,-3.35430579486411,
135.549954577584));
#271873=CARTESIAN_POINT('Ctrl Pts',(-178.437358802524,2.17951838517049,
136.191542534628));
#271874=CARTESIAN_POINT('Ctrl Pts',(-178.715806426336,5.71047164462571,
131.88257348836));
#271875=CARTESIAN_POINT('Ctrl Pts',(-178.99425405015,3.99378043471903,126.582779487459));
#271876=CARTESIAN_POINT('Ctrl Pts',(-179.272701673962,-1.39299988767372,
125.162412309422));
#271877=CARTESIAN_POINT('Ctrl Pts',(-179.551149297775,-5.49968136512185,
128.926720002072));
#271878=CARTESIAN_POINT('Ctrl Pts',(-179.829596921588,-4.55242434239454,
134.416487692516));
#271879=CARTESIAN_POINT('Ctrl Pts',(-180.108044545401,0.578288252700551,
136.5868870633));
#271880=CARTESIAN_POINT('Ctrl Pts',(-180.386492169214,5.17758219451528,
133.443427122574));
#271881=CARTESIAN_POINT('Ctrl Pts',(-180.664939793027,5.01893103852278,
127.874793989312));
#271882=CARTESIAN_POINT('Ctrl Pts',(-180.94338741684,0.248127446539293,
124.998289470128));
#271883=CARTESIAN_POINT('Ctrl Pts',(-181.221835040653,-4.75069314711374,
127.457280693096));
#271884=CARTESIAN_POINT('Ctrl Pts',(-181.500282664465,-5.38385882283189,
132.992074852706));
#271885=CARTESIAN_POINT('Ctrl Pts',(-181.778730288279,-1.06952125649312,
136.516466506004));
#271886=CARTESIAN_POINT('Ctrl Pts',(-182.057177912091,4.22765409554481,
134.791711899713));
#271887=CARTESIAN_POINT('Ctrl Pts',(-182.335625535904,5.63982186616143,
129.402776258069));
#271888=CARTESIAN_POINT('Ctrl Pts',(-182.614073159717,1.86926886239121,
125.301828171599));
#271889=CARTESIAN_POINT('Ctrl Pts',(-182.89252078353,-3.61905090705647,
126.257438589318));
#271890=CARTESIAN_POINT('Ctrl Pts',(-183.170968407343,-5.78163969338434,
131.391448221508));
#271891=CARTESIAN_POINT('Ctrl Pts',(-183.449416031155,-2.63118405029363,
135.985953026497));
#271892=CARTESIAN_POINT('Ctrl Pts',(-183.727863654969,2.93720119453022,
135.818827542541));
#271893=CARTESIAN_POINT('Ctrl Pts',(-184.006311278781,5.80644203183612,
131.04365192486));
#271894=CARTESIAN_POINT('Ctrl Pts',(-184.284758902595,3.33984630234777,
126.048579285806));
#271895=CARTESIAN_POINT('Ctrl Pts',(-184.563206526407,-2.19590501843575,
125.423837357804));
#271896=CARTESIAN_POINT('Ctrl Pts',(-184.84165415022,-5.71372690320071,
129.743533452349));
#271897=CARTESIAN_POINT('Ctrl Pts',(-185.120101774033,-3.98091289500146,
135.03807788744));
#271898=CARTESIAN_POINT('Ctrl Pts',(-185.398549397846,1.41016558529749,
136.442042980103));
#271899=CARTESIAN_POINT('Ctrl Pts',(-185.676997021659,5.50537078312707,
132.665253397689));
#271900=CARTESIAN_POINT('Ctrl Pts',(-185.955444645472,4.54140918357699,
127.178394260007));
#271901=CARTESIAN_POINT('Ctrl Pts',(-186.233892269285,-0.595885595507362,
125.023621066618));
#271902=CARTESIAN_POINT('Ctrl Pts',(-186.512339893098,-5.18559062295048,
128.181065115723));
#271903=CARTESIAN_POINT('Ctrl Pts',(-186.79078751691,-5.00999119808726,
133.749189575911));
#271904=CARTESIAN_POINT('Ctrl Pts',(-187.069235140724,-0.230454613858838,
136.611160086272));
#271905=CARTESIAN_POINT('Ctrl Pts',(-187.347682764536,4.76085850217237,
134.136965562817));
#271906=CARTESIAN_POINT('Ctrl Pts',(-187.626130388349,5.37717523557474,
128.600269901479));
#271907=CARTESIAN_POINT('Ctrl Pts',(-187.904578012162,1.05213061709833,
125.089025932407));
#271908=CARTESIAN_POINT('Ctrl Pts',(-188.183025635975,-4.23977063905356,
126.829895329374));
#271909=CARTESIAN_POINT('Ctrl Pts',(-188.461473259788,-5.63552980222562,
132.223104162766));
#271910=CARTESIAN_POINT('Ctrl Pts',(-188.739920883601,-1.85251238808831,
136.312556987595));
#271911=CARTESIAN_POINT('Ctrl Pts',(-189.018368507414,3.63287341044046,
135.340246438718));
#271912=CARTESIAN_POINT('Ctrl Pts',(-189.296816131227,5.77982602050738,
130.199678410544));
#271913=CARTESIAN_POINT('Ctrl Pts',(-189.575263755039,2.61540087792624,
125.614783790254));
#271914=CARTESIAN_POINT('Ctrl Pts',(-189.853711378852,-2.95244990203274,
125.798856749341));
#271915=CARTESIAN_POINT('Ctrl Pts',(-190.132159002665,-5.80714345722022,
130.582743230867));
#271916=CARTESIAN_POINT('Ctrl Pts',(-190.410606626478,-3.32535586995153,
135.570285264159));
#271917=CARTESIAN_POINT('Ctrl Pts',(-190.689054250291,2.21227130913674,
136.178175375592));
#271918=CARTESIAN_POINT('Ctrl Pts',(-190.967501874104,5.7169292305904,131.847792249846));
#271919=CARTESIAN_POINT('Ctrl Pts',(-191.245949497917,3.96800847665057,
126.558546428502));
#271920=CARTESIAN_POINT('Ctrl Pts',(-191.52439712173,-1.4273182193404,125.170996427354));
#271921=CARTESIAN_POINT('Ctrl Pts',(-191.802844745543,-5.51100920012879,
128.960232911869));
#271922=CARTESIAN_POINT('Ctrl Pts',(-192.081292369355,-4.53035195376586,
134.444132667273));
#271923=CARTESIAN_POINT('Ctrl Pts',(-192.359739993168,0.613477418111232,
136.583259721745));
#271924=CARTESIAN_POINT('Ctrl Pts',(-192.638187616981,5.19355101278185,
133.411860814392));
#271925=CARTESIAN_POINT('Ctrl Pts',(-192.916635240794,5.00100494577841,
127.844296609621));
#271926=CARTESIAN_POINT('Ctrl Pts',(-193.195082864607,0.21277964627773,
124.996886620986));
#271927=CARTESIAN_POINT('Ctrl Pts',(-193.47353048842,-4.77097975328813,
127.486261524329));
#271928=CARTESIAN_POINT('Ctrl Pts',(-193.751978112233,-5.3704418349007,
133.024807396204));
#271929=CARTESIAN_POINT('Ctrl Pts',(-194.030425736046,-1.03473023090876,
136.522871153366));
#271930=CARTESIAN_POINT('Ctrl Pts',(-194.308873359859,4.25184790590635,
134.765903092897));
#271931=CARTESIAN_POINT('Ctrl Pts',(-194.587320983671,5.63118553151129,
129.368471029708));
#271932=CARTESIAN_POINT('Ctrl Pts',(-194.865768607484,1.83573875236439,
125.290551350653));
#271933=CARTESIAN_POINT('Ctrl Pts',(-195.144216231297,-3.64666225938173,
126.279553023333));
#271934=CARTESIAN_POINT('Ctrl Pts',(-195.42266385511,-5.77795880411129,
131.426631825972));
#271935=CARTESIAN_POINT('Ctrl Pts',(-195.701111478923,-2.59959347684268,
136.001873787725));
#271936=CARTESIAN_POINT('Ctrl Pts',(-195.979559102736,2.96767125844341,
135.800855058734));
#271937=CARTESIAN_POINT('Ctrl Pts',(-196.258006726549,5.80779108602021,
131.008302030633));
#271938=CARTESIAN_POINT('Ctrl Pts',(-196.536454350362,3.31083463191258,
126.028336807015));
#271939=CARTESIAN_POINT('Ctrl Pts',(-196.814901974175,-2.22861710565919,
125.437304143558));
#271940=CARTESIAN_POINT('Ctrl Pts',(-197.093349597988,-5.72007859712835,
129.778334184429));
#271941=CARTESIAN_POINT('Ctrl Pts',(-197.3717972218,-3.95506729921131,135.062232393175));
#271942=CARTESIAN_POINT('Ctrl Pts',(-197.650244845613,1.44445763090186,
136.433354448736));
#271943=CARTESIAN_POINT('Ctrl Pts',(-197.928692469426,5.51659656389443,
132.631706165088));
#271944=CARTESIAN_POINT('Ctrl Pts',(-198.207140093239,4.51925275539276,
127.150816594059));
#271945=CARTESIAN_POINT('Ctrl Pts',(-198.485587717052,-0.631063557543924,
125.027355495085));
#271946=CARTESIAN_POINT('Ctrl Pts',(-198.764035340865,-5.2014632902668,
128.212679881281));
#271947=CARTESIAN_POINT('Ctrl Pts',(-199.042482964678,-4.99197236484219,
133.779632253479));
#271948=CARTESIAN_POINT('Ctrl Pts',(-199.320930588491,-0.19510270753564,
136.612455342372));
#271949=CARTESIAN_POINT('Ctrl Pts',(-199.599378212304,4.7810568066993,134.10792312037));
#271950=CARTESIAN_POINT('Ctrl Pts',(-199.877825836116,5.36365868318719,
128.56757834629));
#271951=CARTESIAN_POINT('Ctrl Pts',(-200.156273459929,1.01732025912016,
125.082727206624));
#271952=CARTESIAN_POINT('Ctrl Pts',(-200.434721083742,-4.26388578422093,
126.855777654281));
#271953=CARTESIAN_POINT('Ctrl Pts',(-200.713168707555,-5.62678909426374,
132.257382946195));
#271954=CARTESIAN_POINT('Ctrl Pts',(-200.991616331368,-1.8189481106068,
136.323731702186));
#271955=CARTESIAN_POINT('Ctrl Pts',(-201.270063955181,3.66041732614217,
135.318048067677));
#271956=CARTESIAN_POINT('Ctrl Pts',(-201.548511578994,5.77603806149454,
130.164506172408));
#271957=CARTESIAN_POINT('Ctrl Pts',(-201.826959202806,2.58376199347953,
125.59895925361));
#271958=CARTESIAN_POINT('Ctrl Pts',(-202.10540682662,-2.9828651227522,125.816921890294));
#271959=CARTESIAN_POINT('Ctrl Pts',(-202.383854450432,-5.80838491223743,
130.618097067413));
#271960=CARTESIAN_POINT('Ctrl Pts',(-202.662302074245,-3.29628272275406,
135.590439347642));
#271961=CARTESIAN_POINT('Ctrl Pts',(-202.940749698058,2.24494225657654,
136.164609087875));
#271962=CARTESIAN_POINT('Ctrl Pts',(-203.219197321871,5.72317497363993,
131.812972346589));
#271963=CARTESIAN_POINT('Ctrl Pts',(-203.497644945684,3.94208948256877,
126.534470699752));
#271964=CARTESIAN_POINT('Ctrl Pts',(-203.776092569497,-1.46158366120557,
125.179789291667));
#271965=CARTESIAN_POINT('Ctrl Pts',(-204.05454019331,-5.52213282266317,
128.993814156497));
#271966=CARTESIAN_POINT('Ctrl Pts',(-204.332987817123,-4.5081116912795,
134.471642768938));
#271967=CARTESIAN_POINT('Ctrl Pts',(-204.611435440935,0.648643850890564,
136.579418240959));
#271968=CARTESIAN_POINT('Ctrl Pts',(-204.889883064748,5.20932738210573,
133.380197884332));
#271969=CARTESIAN_POINT('Ctrl Pts',(-205.168330688562,4.98289353895661,
127.813908916192));
#271970=CARTESIAN_POINT('Ctrl Pts',(-205.446778312374,0.177423961388546,
124.995698969927));
#271971=CARTESIAN_POINT('Ctrl Pts',(-205.725225936187,-4.79108956905296,
127.515365308944));
#271972=CARTESIAN_POINT('Ctrl Pts',(-206.00367356,-5.35682584327266,133.057457660231));
#271973=CARTESIAN_POINT('Ctrl Pts',(-206.282121183813,-0.999900863015179,
136.529063899218));
#271974=CARTESIAN_POINT('Ctrl Pts',(-206.560568807626,4.27588416248015,
134.739947489669));
#271975=CARTESIAN_POINT('Ctrl Pts',(-206.839016431439,5.62234053121038,
129.334219008764));
#271976=CARTESIAN_POINT('Ctrl Pts',(-207.117464055252,1.80214061836306,
125.279478845937));
#271977=CARTESIAN_POINT('Ctrl Pts',(-207.395911679064,-3.67413848329639,
126.301835125757));
#271978=CARTESIAN_POINT('Ctrl Pts',(-207.674359302878,-5.77406381044983,
131.461792371951));
#271979=CARTESIAN_POINT('Ctrl Pts',(-207.95280692669,-2.56790657449899,
136.01760195319));
#271980=CARTESIAN_POINT('Ctrl Pts',(-208.231254550503,2.99803135420673,
135.782697427989));
#271981=CARTESIAN_POINT('Ctrl Pts',(-208.509702174316,5.8089249303698,130.972944579282));
#271982=CARTESIAN_POINT('Ctrl Pts',(-208.788149798129,3.28170027728254,
126.008271305542));
#271983=CARTESIAN_POINT('Ctrl Pts',(-209.066597421942,-2.2612466106562,
125.450969807563));
#271984=CARTESIAN_POINT('Ctrl Pts',(-209.345045045754,-5.72621833144002,
129.813172936296));
#271985=CARTESIAN_POINT('Ctrl Pts',(-209.623492669568,-3.92907514694791,
135.086229121905));
#271986=CARTESIAN_POINT('Ctrl Pts',(-209.90194029338,1.4786961515975,136.424457332932));
#271987=CARTESIAN_POINT('Ctrl Pts',(-210.180387917194,5.52761792514773,
132.598091219525));
#271988=CARTESIAN_POINT('Ctrl Pts',(-210.458835541006,4.49692886463537,
127.123374311529));
#271989=CARTESIAN_POINT('Ctrl Pts',(-210.73728316482,-0.666218135288655,
125.031303992602));
#271990=CARTESIAN_POINT('Ctrl Pts',(-211.015730788632,-5.21714321544808,
128.244390682522));
#271991=CARTESIAN_POINT('Ctrl Pts',(-211.294178412445,-4.97376855222533,
133.809964681263));
#271992=CARTESIAN_POINT('Ctrl Pts',(-211.572626036258,-0.159743571609885,
136.613535377387));
#271993=CARTESIAN_POINT('Ctrl Pts',(-211.851073660071,4.80107794740803,
134.0787582632));
#271994=CARTESIAN_POINT('Ctrl Pts',(-212.129521283884,5.34994337845465,
128.534969675892));
#271995=CARTESIAN_POINT('Ctrl Pts',(-212.407968907697,0.982472203965689,
125.076640498072));
#271996=CARTESIAN_POINT('Ctrl Pts',(-212.686416531509,-4.28784292953254,
126.881806295382));
#271997=CARTESIAN_POINT('Ctrl Pts',(-212.964864155322,-5.61783988356258,
132.291607887347));
#271998=CARTESIAN_POINT('Ctrl Pts',(-213.243311779135,-1.78531643133465,
136.334701894451));
#271999=CARTESIAN_POINT('Ctrl Pts',(-213.521759402948,3.68782560373359,
135.295682440288));
#272000=CARTESIAN_POINT('Ctrl Pts',(-213.800207026761,5.77203606926717,
130.129357644311));
#272001=CARTESIAN_POINT('Ctrl Pts',(-214.078654650574,2.55202736678199,
125.583327605028));
#272002=CARTESIAN_POINT('Ctrl Pts',(-214.357102274386,-3.0131698123076,
125.835171842623));
#272003=CARTESIAN_POINT('Ctrl Pts',(-214.6355498982,-5.80941113541564,130.653457806023));
#272004=CARTESIAN_POINT('Ctrl Pts',(-214.913997522012,-3.26708743058812,
135.610416081219));
#272005=CARTESIAN_POINT('Ctrl Pts',(-215.192445145826,2.27753001685547,
136.15084417418));
#272006=CARTESIAN_POINT('Ctrl Pts',(-215.470892769638,5.72920864233609,
131.778115068854));
#272007=CARTESIAN_POINT('Ctrl Pts',(-215.749340393451,3.9160244129115,126.510553193344));
#272008=CARTESIAN_POINT('Ctrl Pts',(-216.027788017264,-1.49579494355069,
125.18879057654));
#272009=CARTESIAN_POINT('Ctrl Pts',(-216.306235641077,-5.53305182053502,
129.02746249159));
#272010=CARTESIAN_POINT('Ctrl Pts',(-216.58468326489,-4.48570437905656,
134.499016978113));
#272011=CARTESIAN_POINT('Ctrl Pts',(-216.863130888703,0.683786247933482,
136.57536276329));
#272012=CARTESIAN_POINT('Ctrl Pts',(-217.141578512516,5.2249107178877,133.348439505674));
#272013=CARTESIAN_POINT('Ctrl Pts',(-217.420026136328,4.96459748918233,
127.78363203505));
#272014=CARTESIAN_POINT('Ctrl Pts',(-217.698473760142,0.142061701988793,
124.994726560962));
#272015=CARTESIAN_POINT('Ctrl Pts',(-217.976921383954,-4.81102184923216,
127.544590968491));
#272016=CARTESIAN_POINT('Ctrl Pts',(-218.255369007768,-5.34301135249269,
133.090024434919));
#272017=CARTESIAN_POINT('Ctrl Pts',(-218.53381663158,-0.965034443427401,
136.535044514085));
#272018=CARTESIAN_POINT('Ctrl Pts',(-218.812264255394,4.29976197459382,
134.713846051821));
#272019=CARTESIAN_POINT('Ctrl Pts',(-219.090711879206,5.61328719301349,
129.300021464458));
#272020=CARTESIAN_POINT('Ctrl Pts',(-219.369159503019,1.76847570537835,
125.268611067748));
#272021=CARTESIAN_POINT('Ctrl Pts',(-219.647607126831,-3.70147856065836,
126.324284070919));
#272022=CARTESIAN_POINT('Ctrl Pts',(-219.926054750645,-5.76995485673049,
131.496928556552));
#272023=CARTESIAN_POINT('Ctrl Pts',(-220.204502374457,-2.5361245174328,
136.033136940081));
#272024=CARTESIAN_POINT('Ctrl Pts',(-220.48294999827,3.02828035681523,135.764355323142));
#272025=CARTESIAN_POINT('Ctrl Pts',(-220.761397622083,5.80984352286985,
130.937580880991));
#272026=CARTESIAN_POINT('Ctrl Pts',(-221.039845245896,3.25244431804234,
125.988383524923));
#272027=CARTESIAN_POINT('Ctrl Pts',(-221.318292869709,-2.29379232432851,
125.464833843433));
#272028=CARTESIAN_POINT('Ctrl Pts',(-221.596740493522,-5.73214587862558,
129.848048416986));
#272029=CARTESIAN_POINT('Ctrl Pts',(-221.875188117335,-3.90293740136003,
135.110067184424));
#272030=CARTESIAN_POINT('Ctrl Pts',(-222.153635741148,1.51287987866345,
136.415351962378));
#272031=CARTESIAN_POINT('Ctrl Pts',(-222.432083364961,5.53843445848603,
132.564409806615));
#272032=CARTESIAN_POINT('Ctrl Pts',(-222.710530988774,4.47443833852516,
127.0960684293));
#272033=CARTESIAN_POINT('Ctrl Pts',(-222.988978612586,-0.701348026075381,
125.035466412855));
#272034=CARTESIAN_POINT('Ctrl Pts',(-223.267426236399,-5.23262981746888,
128.27619634439));
#272035=CARTESIAN_POINT('Ctrl Pts',(-223.545873860212,-4.95538043478568,
133.840185735283));
#272036=CARTESIAN_POINT('Ctrl Pts',(-223.824321484025,-0.124378516327312,
136.614400151295));
#272037=CARTESIAN_POINT('Ctrl Pts',(-224.102769107838,4.82092118240782,
134.049472072021));
#272038=CARTESIAN_POINT('Ctrl Pts',(-224.381216731651,5.33602982960279,
128.502445098609));
#272039=CARTESIAN_POINT('Ctrl Pts',(-224.659664355464,0.947587742942381,
125.070766032295));
#272040=CARTESIAN_POINT('Ctrl Pts',(-224.938111979277,-4.31164118724753,
126.907980288176));
#272041=CARTESIAN_POINT('Ctrl Pts',(-225.216559603089,-5.60868250173869,
132.325777718005));
#272042=CARTESIAN_POINT('Ctrl Pts',(-225.495007226903,-1.75161859650508,
136.345467157888));
#272043=CARTESIAN_POINT('Ctrl Pts',(-225.773454850715,3.71509722759125,
135.273150385318));
#272044=CARTESIAN_POINT('Ctrl Pts',(-226.051902474528,5.7678201921206,130.0942341287));
#272045=CARTESIAN_POINT('Ctrl Pts',(-226.330350098341,2.52019817377184,
125.567889423742));
#272046=CARTESIAN_POINT('Ctrl Pts',(-226.608797722154,-3.04336284774751,
125.853605930069));
#272047=CARTESIAN_POINT('Ctrl Pts',(-226.887245345967,-5.81022208872781,
130.688824136393));
#272048=CARTESIAN_POINT('Ctrl Pts',(-227.16569296978,-3.23777107529596,
135.630214724643));
#272049=CARTESIAN_POINT('Ctrl Pts',(-227.444140593593,2.31003338242206,
136.13688114457));
#272050=CARTESIAN_POINT('Ctrl Pts',(-227.722588217406,5.73503001309909,
131.74322170829));
#272051=CARTESIAN_POINT('Ctrl Pts',(-228.001035841218,3.88981423352964,
126.486794795549));
#272052=CARTESIAN_POINT('Ctrl Pts',(-228.279483465031,-1.52995079866356,
125.197999948425));
#272053=CARTESIAN_POINT('Ctrl Pts',(-228.557931088844,-5.54376578913698,
129.061176670297));
#272054=CARTESIAN_POINT('Ctrl Pts',(-228.836378712657,-4.46313084740822,
134.526254280438));
#272055=CARTESIAN_POINT('Ctrl Pts',(-229.11482633647,0.718903307025501,
136.571093439014));
#272056=CARTESIAN_POINT('Ctrl Pts',(-229.393273960283,5.24030044268158,
133.316586855238));
#272057=CARTESIAN_POINT('Ctrl Pts',(-229.671721584096,4.94611747442232,
127.753467088116));
#272058=CARTESIAN_POINT('Ctrl Pts',(-229.950169207909,0.106694178440453,
124.993969430123));
#272059=CARTESIAN_POINT('Ctrl Pts',(-230.228616831722,-4.83077585522751,
127.57393742));
#272060=CARTESIAN_POINT('Ctrl Pts',(-230.507064455534,-5.32899887446215,
133.122506513493));
#272061=CARTESIAN_POINT('Ctrl Pts',(-230.785512079348,-0.930132264133436,
136.540812776352));
#272062=CARTESIAN_POINT('Ctrl Pts',(-231.06395970316,4.3234804574463,134.687599746553));
#272063=CARTESIAN_POINT('Ctrl Pts',(-231.342407326973,5.60402585239536,
129.265879663993));
#272064=CARTESIAN_POINT('Ctrl Pts',(-231.620854950786,1.73474526087603,
125.257948418793));
#272065=CARTESIAN_POINT('Ctrl Pts',(-231.899302574599,-3.72868147837107,
126.346899026965));
#272066=CARTESIAN_POINT('Ctrl Pts',(-232.177750198412,-5.76563209521201,
131.532039077795));
#272067=CARTESIAN_POINT('Ctrl Pts',(-232.456197822225,-2.50424848333998,
136.048478172742));
#272068=CARTESIAN_POINT('Ctrl Pts',(-232.734645446038,3.05841714538193,
135.745829423867));
#272069=CARTESIAN_POINT('Ctrl Pts',(-233.01309306985,5.81054682948159,130.902212246173));
#272070=CARTESIAN_POINT('Ctrl Pts',(-233.291540693664,3.22306783828139,
125.968674202107));
#272071=CARTESIAN_POINT('Ctrl Pts',(-233.569988317476,-2.32625304068266,
125.478895737432));
#272072=CARTESIAN_POINT('Ctrl Pts',(-233.84843594129,-5.73786101903762,
129.882959334177));
#272073=CARTESIAN_POINT('Ctrl Pts',(-234.126883565102,-3.87665503099142,
135.133745697402));
#272074=CARTESIAN_POINT('Ctrl Pts',(-234.405331188915,1.54700754540913,
136.406038674476));
#272075=CARTESIAN_POINT('Ctrl Pts',(-234.683778812728,5.54904576309872,
132.530663174436));
#272076=CARTESIAN_POINT('Ctrl Pts',(-234.962226436541,4.45178201045685,
127.0688999592));
#272077=CARTESIAN_POINT('Ctrl Pts',(-235.240674060353,-0.736451928153096,
125.039842601604));
#272078=CARTESIAN_POINT('Ctrl Pts',(-235.519121684167,-5.24792252246713,
128.308095688315));
#272079=CARTESIAN_POINT('Ctrl Pts',(-235.797569307979,-4.93680869390195,
133.870294295687));
#272080=CARTESIAN_POINT('Ctrl Pts',(-236.076016931792,-0.0890088521534987,
136.61504963205));
#272081=CARTESIAN_POINT('Ctrl Pts',(-236.354464555605,4.8405857764003,134.020065632043));
#272082=CARTESIAN_POINT('Ctrl Pts',(-236.632912179418,5.32191855220324,
128.470005819654));
#272083=CARTESIAN_POINT('Ctrl Pts',(-236.911359803231,0.912668168706789,
125.065104026974));
#272084=CARTESIAN_POINT('Ctrl Pts',(-237.189807427044,-4.33527967551271,
126.934298662776));
#272085=CARTESIAN_POINT('Ctrl Pts',(-237.468255050857,-5.59931728812211,
132.359891171993));
#272086=CARTESIAN_POINT('Ctrl Pts',(-237.74670267467,-1.71785585480426,
136.356027093583));
#272087=CARTESIAN_POINT('Ctrl Pts',(-238.025150298482,3.7422311871549,135.250452737698));
#272088=CARTESIAN_POINT('Ctrl Pts',(-238.303597922296,5.76339058627568,
130.059136927086));
#272089=CARTESIAN_POINT('Ctrl Pts',(-238.582045546108,2.48827559389159,
125.552645281824));
#272090=CARTESIAN_POINT('Ctrl Pts',(-238.860493169922,-3.07344311025789,
125.87222346955));
#272091=CARTESIAN_POINT('Ctrl Pts',(-239.138940793734,-5.81081774212379,
130.724194748009));
#272092=CARTESIAN_POINT('Ctrl Pts',(-239.417388417547,-3.20833474320591,
135.649834544268));
#272093=CARTESIAN_POINT('Ctrl Pts',(-239.69583604136,2.34245114885216,136.12272051645));
#272094=CARTESIAN_POINT('Ctrl Pts',(-239.974283665173,5.7406388702159,131.708293557882));
#272095=CARTESIAN_POINT('Ctrl Pts',(-240.252731288985,3.86345991565072,
126.463196386742));
#272096=CARTESIAN_POINT('Ctrl Pts',(-240.531178912799,-1.56404996088748,
125.207417066067));
#272097=CARTESIAN_POINT('Ctrl Pts',(-240.809626536611,-5.5542743314588,
129.094955443325));
#272098=CARTESIAN_POINT('Ctrl Pts',(-241.088074160425,-4.44039193280503,
134.553353666625));
#272099=CARTESIAN_POINT('Ctrl Pts',(-241.366521784237,0.753993726891117,
136.566610426332));
#272100=CARTESIAN_POINT('Ctrl Pts',(-241.64496940805,5.25549598621542,133.284641113335));
#272101=CARTESIAN_POINT('Ctrl Pts',(-241.923417031863,4.92745417946037,
127.723415193164));
#272102=CARTESIAN_POINT('Ctrl Pts',(-242.201864655676,0.071322701300089,
124.993427605467));
#272103=CARTESIAN_POINT('Ctrl Pts',(-242.480312279489,-4.85035085504701,
127.603403576029));
#272104=CARTESIAN_POINT('Ctrl Pts',(-242.758759903302,-5.31478892841856,
133.154902692318));
#272105=CARTESIAN_POINT('Ctrl Pts',(-243.037207527115,-0.895195618446729,
136.546368472274));
#272106=CARTESIAN_POINT('Ctrl Pts',(-243.315655150928,4.34703873214009,
134.661209546432));
#272107=CARTESIAN_POINT('Ctrl Pts',(-243.59410277474,5.59455685253872,129.231794872506));
#272108=CARTESIAN_POINT('Ctrl Pts',(-243.872550398553,1.7009505347501,125.247491294183));
#272109=CARTESIAN_POINT('Ctrl Pts',(-244.150998022366,-3.75574622842035,
126.36967915589));
#272110=CARTESIAN_POINT('Ctrl Pts',(-244.429445646179,-5.76109568607594,
131.567122634643));
#272111=CARTESIAN_POINT('Ctrl Pts',(-244.707893269992,-2.47227965339868,
136.063625082699));
#272112=CARTESIAN_POINT('Ctrl Pts',(-244.986340893805,3.08844060317656,
135.727120416648));
#272113=CARTESIAN_POINT('Ctrl Pts',(-245.264788517618,5.81103482414375,
130.866839985428));
#272114=CARTESIAN_POINT('Ctrl Pts',(-245.543236141431,3.1935719265564,125.949144067427));
#272115=CARTESIAN_POINT('Ctrl Pts',(-245.821683765243,-2.35862755687492,
125.49315496849));
#272116=CARTESIAN_POINT('Ctrl Pts',(-246.100131389057,-5.74336354089951,
129.917904394232));
#272117=CARTESIAN_POINT('Ctrl Pts',(-246.378579012869,-3.85022900974501,
135.157263783424));
#272118=CARTESIAN_POINT('Ctrl Pts',(-246.657026636682,1.58107788722132,
136.396517814333));
#272119=CARTESIAN_POINT('Ctrl Pts',(-246.935474260495,5.55945144577998,
132.496852573479));
#272120=CARTESIAN_POINT('Ctrl Pts',(-247.213921884308,4.42896071996899,
127.04186990797));
#272121=CARTESIAN_POINT('Ctrl Pts',(-247.492369508121,-0.77152854073377,
125.044432396689));
#272122=CARTESIAN_POINT('Ctrl Pts',(-247.770817131934,-5.26302076376676,
128.340087532256));
#272123=CARTESIAN_POINT('Ctrl Pts',(-248.049264755747,-4.91805401775627,
133.90028924679));
#272124=CARTESIAN_POINT('Ctrl Pts',(-248.32771237956,-0.0536358897235281,
136.615483795589));
#272125=CARTESIAN_POINT('Ctrl Pts',(-248.606160003372,4.86007100070672,
133.990540032933));
#272126=CARTESIAN_POINT('Ctrl Pts',(-248.884607627186,5.30761006915461,
128.437653041073));
#272127=CARTESIAN_POINT('Ctrl Pts',(-249.163055250998,0.877714775216597,
125.059654691916));
#272128=CARTESIAN_POINT('Ctrl Pts',(-249.441502874812,-4.35875751839529,
126.960760443945));
#272129=CARTESIAN_POINT('Ctrl Pts',(-249.719950498624,-5.58974458974414,
132.393946985223));
#272130=CARTESIAN_POINT('Ctrl Pts',(-249.998398122437,-1.68402945732324,
136.366381310236));
#272131=CARTESIAN_POINT('Ctrl Pts',(-250.27684574625,3.76922647696617,135.227590338499));
#272132=CARTESIAN_POINT('Ctrl Pts',(-250.555293370063,5.75874741587205,
130.024067340013));
#272133=CARTESIAN_POINT('Ctrl Pts',(-250.833740993876,2.45626081004631,
125.537595744144));
#272134=CARTESIAN_POINT('Ctrl Pts',(-251.112188617689,-3.10340948520656,
125.891023771197));
#272135=CARTESIAN_POINT('Ctrl Pts',(-251.390636241501,-5.81119807352532,
130.759568330183));
#272136=CARTESIAN_POINT('Ctrl Pts',(-251.669083865314,-3.17877952510356,
135.669274813107));
#272137=CARTESIAN_POINT('Ctrl Pts',(-251.947531489127,2.37478211491517,
136.10836281449));
#272138=CARTESIAN_POINT('Ctrl Pts',(-252.22597911294,5.74603500580729,131.673331912019));
#272139=CARTESIAN_POINT('Ctrl Pts',(-252.504426736753,3.83696243592119,
126.439758841162));
#272140=CARTESIAN_POINT('Ctrl Pts',(-252.782874360566,-1.59809116681098,
125.217041580908));
#272141=CARTESIAN_POINT('Ctrl Pts',(-253.061321984379,-5.5645770578269,
129.128797558239));
#272142=CARTESIAN_POINT('Ctrl Pts',(-253.339769608192,-4.41748847836656,
134.580314133917));
#272143=CARTESIAN_POINT('Ctrl Pts',(-253.618217232004,0.789056208225191,
136.561913888683));
#272144=CARTESIAN_POINT('Ctrl Pts',(-253.896664855818,5.27049678355612,
133.252603468789));
#272145=CARTESIAN_POINT('Ctrl Pts',(-254.17511247963,4.90860829937749,127.693477454216));
#272146=CARTESIAN_POINT('Ctrl Pts',(-254.453560103444,0.0359485746511809,
124.993101125124));
#272147=CARTESIAN_POINT('Ctrl Pts',(-254.732007727256,-4.86974611083267,
127.632988310607));
#272148=CARTESIAN_POINT('Ctrl Pts',(-255.010455351069,-5.30038206451776,
133.187211835313));
#272149=CARTESIAN_POINT('Ctrl Pts',(-255.288902974882,-0.860225756393269,
136.55171127444));
#272150=CARTESIAN_POINT('Ctrl Pts',(-255.567350598695,4.37043584157037,
134.634676658854));
#272151=CARTESIAN_POINT('Ctrl Pts',(-255.845798222508,5.58488070320316,
129.197767919676));
#272152=CARTESIAN_POINT('Ctrl Pts',(-256.12424584632,1.66709247927321,125.23724089965));
#272153=CARTESIAN_POINT('Ctrl Pts',(-256.402693470134,-3.78267124144458,
126.39262206856));
#272154=CARTESIAN_POINT('Ctrl Pts',(-256.681141093946,-5.75634686702621,
131.602180844355));
#272155=CARTESIAN_POINT('Ctrl Pts',(-256.95958871776,-2.44021719259262,
136.078571600242));
#272156=CARTESIAN_POINT('Ctrl Pts',(-257.238036341572,3.118345804191,135.708239395799));
#272157=CARTESIAN_POINT('Ctrl Pts',(-257.516483965385,5.81131468939531,
130.8314457702));
#272158=CARTESIAN_POINT('Ctrl Pts',(-257.794931589198,3.16394407961038,
125.929830927563));
#272159=CARTESIAN_POINT('Ctrl Pts',(-258.073379213011,-2.39088900078744,
125.507540987923));
#272160=CARTESIAN_POINT('Ctrl Pts',(-258.351826836824,-5.74870171518396,
129.953014515613));
#272161=CARTESIAN_POINT('Ctrl Pts',(-258.630274460636,-3.82356878618261,
135.180370918811));
#272162=CARTESIAN_POINT('Ctrl Pts',(-258.908722084449,1.61491681105698,
136.387261181902));
#272163=CARTESIAN_POINT('Ctrl Pts',(-259.187169708263,5.56997747689423,
132.462088635074));
#272164=CARTESIAN_POINT('Ctrl Pts',(-259.465617332075,4.40535894966821,
127.016664495574));
#272165=CARTESIAN_POINT('Ctrl Pts',(-259.744064955888,-0.805411631290512,
125.046024618449));
#272166=CARTESIAN_POINT('Ctrl Pts',(-260.022512579701,-5.28013240410161,
128.378470706602));
#272167=CARTESIAN_POINT('Ctrl Pts',(-260.254552266212,-4.95911089365773,
132.993351965875));
#272168=CARTESIAN_POINT('Ctrl Pts',(-260.440213228287,-2.45877638613931,
135.28779596926));
#272169=CARTESIAN_POINT('Ctrl Pts',(-260.53305831576,-0.833059752290926,
135.715219187214));
#272170=CARTESIAN_POINT('Ctrl Pts',(-260.579495465929,-0.013892627260139,
135.717527172907));
#272171=CARTESIAN_POINT('Ctrl Pts',(-207.299567498839,-3.90840034609179,
135.243902605347));
#272172=CARTESIAN_POINT('Ctrl Pts',(-207.309485839119,-3.91568439033028,
135.211326968109));
#272173=CARTESIAN_POINT('Ctrl Pts',(-207.319294625375,-3.92298020337359,
135.178719366898));
#272174=CARTESIAN_POINT('Ctrl Pts',(-207.373488585912,-3.96376374076592,
134.996347972705));
#272175=CARTESIAN_POINT('Ctrl Pts',(-207.415719149759,-3.99734042662899,
134.845804617557));
#272176=CARTESIAN_POINT('Ctrl Pts',(-207.499376031093,-4.06628914634799,
134.528884546366));
#272177=CARTESIAN_POINT('Ctrl Pts',(-207.540351370784,-4.10153445023782,
134.36234850031));
#272178=CARTESIAN_POINT('Ctrl Pts',(-207.656874908577,-4.20404560328433,
133.851628215195));
#272179=CARTESIAN_POINT('Ctrl Pts',(-207.723530466945,-4.26603286108595,
133.504762588803));
#272180=CARTESIAN_POINT('Ctrl Pts',(-207.778274395763,-4.31466228417799,
133.153864562742));
#272181=CARTESIAN_POINT('Ctrl Pts',(-178.531763843762,1.96089658445146,
125.231307795101));
#272182=CARTESIAN_POINT('Ctrl Pts',(-178.570801079156,1.56843596370832,
125.131935448447));
#272183=CARTESIAN_POINT('Ctrl Pts',(-178.601759745776,1.16805303801507,
125.056039372548));
#272184=CARTESIAN_POINT('Ctrl Pts',(-178.625335154052,0.72444720086025,
124.99874952163));
#272185=CARTESIAN_POINT('Ctrl Pts',(-178.627404925171,0.683646809442433,
124.993728200571));
#272186=CARTESIAN_POINT('Ctrl Pts',(-178.629486211621,0.64054918726823,
124.988685854593));
#272187=CARTESIAN_POINT('Ctrl Pts',(-178.629595291271,0.638284118533388,
124.988421607827));
#272188=CARTESIAN_POINT('Ctrl Pts',(-178.629744702131,0.635172831973636,
124.988059686924));
#272189=CARTESIAN_POINT('Ctrl Pts',(-178.629785292499,0.634326701253174,
124.987961366993));
#272190=CARTESIAN_POINT('Ctrl Pts',(-178.629858681012,0.632795262003021,
124.987783607086));
#272191=CARTESIAN_POINT('Ctrl Pts',(-178.629891493623,0.632109958282007,
124.987704131074));
#272192=CARTESIAN_POINT('Ctrl Pts',(-178.62994393397,0.631013785865012,
124.98757711741));
#272193=CARTESIAN_POINT('Ctrl Pts',(-178.62996357934,0.630602923758097,
124.98752953583));
#272194=CARTESIAN_POINT('Ctrl Pts',(-178.629994326891,0.629959541468569,
124.98745506556));
#272195=CARTESIAN_POINT('Ctrl Pts',(-178.630005435777,0.629727024217423,
124.987428160163));
#272196=CARTESIAN_POINT('Ctrl Pts',(-178.630026130574,0.629293740909809,
124.987378038377));
#272197=CARTESIAN_POINT('Ctrl Pts',(-178.630035717301,0.629092974966084,
124.987354819958));
#272198=CARTESIAN_POINT('Ctrl Pts',(-178.630056886341,0.628649540099313,
124.987303550298));
#272199=CARTESIAN_POINT('Ctrl Pts',(-178.630068467602,0.628406869994507,
124.98727550168));
#272200=CARTESIAN_POINT('Ctrl Pts',(-178.630101658504,0.627711187230269,
124.987195117429));
#272201=CARTESIAN_POINT('Ctrl Pts',(-178.630123259547,0.627258171775908,
124.987142803207));
#272202=CARTESIAN_POINT('Ctrl Pts',(-178.630259381619,0.624401810565511,
124.986813142828));
#272203=CARTESIAN_POINT('Ctrl Pts',(-178.630373575472,0.621998354980397,
124.986536611421));
#272204=CARTESIAN_POINT('Ctrl Pts',(-178.630705048662,0.615000656884468,
124.985733983766));
#272205=CARTESIAN_POINT('Ctrl Pts',(-178.630921427308,0.610406113059156,
124.985210129304));
#272206=CARTESIAN_POINT('Ctrl Pts',(-178.636268568232,0.496200348966026,
124.972266679728));
#272207=CARTESIAN_POINT('Ctrl Pts',(-178.64069439242,0.386339611214377,
124.961599087318));
#272208=CARTESIAN_POINT('Ctrl Pts',(-178.65506927048,-0.0414682925157202,
124.927025558109));
#272209=CARTESIAN_POINT('Ctrl Pts',(-178.659656383999,-0.360982716739327,
124.916125069186));
#272210=CARTESIAN_POINT('Ctrl Pts',(-178.657730373057,-0.680012995379148,
124.92072784072));
#272211=CARTESIAN_POINT('',(-177.476367722506,-5.64337912711117,130.804360617576));
#272212=CARTESIAN_POINT('Ctrl Pts',(-177.476367722506,-5.64337912711113,
130.804360617586));
#272213=CARTESIAN_POINT('Ctrl Pts',(-177.476367722506,-5.66278702247985,
131.040394557583));
#272214=CARTESIAN_POINT('Ctrl Pts',(-177.481821319387,-5.65742368675511,
131.284442682447));
#272215=CARTESIAN_POINT('Ctrl Pts',(-177.494362458831,-5.6215507189005,
131.5448204376));
#272216=CARTESIAN_POINT('Ctrl Pts',(-177.494712937718,-5.6205398291972,
131.551991505204));
#272217=CARTESIAN_POINT('Ctrl Pts',(-177.495082378428,-5.61946569039355,
131.55944266065));
#272218=CARTESIAN_POINT('Ctrl Pts',(-177.495096443372,-5.61942478425224,
131.559726172768));
#272219=CARTESIAN_POINT('Ctrl Pts',(-177.495125486698,-5.6193402891457,
131.560311279265));
#272220=CARTESIAN_POINT('Ctrl Pts',(-177.495140466066,-5.6192966956462,
131.560612872408));
#272221=CARTESIAN_POINT('Ctrl Pts',(-177.495163361027,-5.61923004398011,
131.561073561054));
#272222=CARTESIAN_POINT('Ctrl Pts',(-177.495171270364,-5.61920701437734,
131.561232661122));
#272223=CARTESIAN_POINT('Ctrl Pts',(-177.495185587491,-5.61916532000669,
131.561520565902));
#272224=CARTESIAN_POINT('Ctrl Pts',(-177.495191994478,-5.61914665895088,
131.561649371792));
#272225=CARTESIAN_POINT('Ctrl Pts',(-177.495205667846,-5.61910682818089,
131.561924190531));
#272226=CARTESIAN_POINT('Ctrl Pts',(-177.495212934609,-5.61908565661172,
131.562070201652));
#272227=CARTESIAN_POINT('Ctrl Pts',(-177.495232530402,-5.61902855560728,
131.562463826025));
#272228=CARTESIAN_POINT('Ctrl Pts',(-177.495244863336,-5.61899260850394,
131.562711438321));
#272229=CARTESIAN_POINT('Ctrl Pts',(-177.495303923655,-5.61882041779216,
131.563896629399));
#272230=CARTESIAN_POINT('Ctrl Pts',(-177.495350729054,-5.6186838181541,
131.564834152763));
#272231=CARTESIAN_POINT('Ctrl Pts',(-177.500236184812,-5.60441144589133,
131.662509836507));
#272232=CARTESIAN_POINT('Ctrl Pts',(-177.505963587261,-5.58621592287407,
131.758520867681));
#272233=CARTESIAN_POINT('Ctrl Pts',(-177.527820287702,-5.51277087162531,
132.075255600853));
#272234=CARTESIAN_POINT('Ctrl Pts',(-177.547590315895,-5.44069144148586,
132.290973448603));
#272235=CARTESIAN_POINT('Ctrl Pts',(-177.609386990917,-5.20268998524819,
132.843250606157));
#272236=CARTESIAN_POINT('Ctrl Pts',(-177.657311288753,-5.00712947277706,
133.165027679615));
#272237=CARTESIAN_POINT('Ctrl Pts',(-177.779852173243,-4.46943606900208,
133.857655628443));
#272238=CARTESIAN_POINT('Ctrl Pts',(-177.858334959518,-4.09801820021662,
134.208982373595));
#272239=CARTESIAN_POINT('Ctrl Pts',(-178.033565929287,-3.13626912879633,
134.909021435998));
#272240=CARTESIAN_POINT('Ctrl Pts',(-178.123833995731,-2.5229730614002,
135.204982366882));
#272241=CARTESIAN_POINT('Ctrl Pts',(-178.219857087681,-1.56463168596343,
135.50774809867));
#272242=CARTESIAN_POINT('Ctrl Pts',(-178.244990796156,-1.25482479666693,
135.583862452928));
#272243=CARTESIAN_POINT('Ctrl Pts',(-178.266053397623,-0.911313259705867,
135.646805482782));
#272244=CARTESIAN_POINT('Ctrl Pts',(-178.267880485167,-0.880555601331235,
135.652254596537));
#272245=CARTESIAN_POINT('Ctrl Pts',(-178.269729479139,-0.848389479458237,
135.657759390394));
#272246=CARTESIAN_POINT('Ctrl Pts',(-178.269808415561,-0.847014208584358,
135.657994379534));
#272247=CARTESIAN_POINT('Ctrl Pts',(-178.269900842308,-0.84540149531386,
135.658269506422));
#272248=CARTESIAN_POINT('Ctrl Pts',(-178.26991444318,-0.845164118492042,
135.658309991603));
#272249=CARTESIAN_POINT('Ctrl Pts',(-178.269945205294,-0.844627086959365,
135.658401558698));
#272250=CARTESIAN_POINT('Ctrl Pts',(-178.26996236452,-0.844327431044021,
135.658452634283));
#272251=CARTESIAN_POINT('Ctrl Pts',(-178.270036338938,-0.843035175886533,
135.658672820216));
#272252=CARTESIAN_POINT('Ctrl Pts',(-178.270093100188,-0.842042544645915,
135.65884176107));
#272253=CARTESIAN_POINT('Ctrl Pts',(-178.270171301912,-0.840673485715273,
135.659074502599));
#272254=CARTESIAN_POINT('Ctrl Pts',(-178.270192793215,-0.840297088128566,
135.659138462936));
#272255=CARTESIAN_POINT('Ctrl Pts',(-178.270228585886,-0.839669959618898,
135.65924498328));
#272256=CARTESIAN_POINT('Ctrl Pts',(-178.270242892027,-0.839419231083232,
135.659287558272));
#272257=CARTESIAN_POINT('Ctrl Pts',(-178.270270866443,-0.838928818979041,
135.659370808756));
#272258=CARTESIAN_POINT('Ctrl Pts',(-178.270284535031,-0.838689135834364,
135.659411485233));
#272259=CARTESIAN_POINT('Ctrl Pts',(-178.270316659246,-0.838125679795843,
135.659507082639));
#272260=CARTESIAN_POINT('Ctrl Pts',(-178.270335112011,-0.837801905327044,
135.659561994584));
#272261=CARTESIAN_POINT('Ctrl Pts',(-178.27039519559,-0.836747298356631,
135.659740788603));
#272262=CARTESIAN_POINT('Ctrl Pts',(-178.270436800547,-0.836016450446397,
135.659864589485));
#272263=CARTESIAN_POINT('Ctrl Pts',(-178.271388514283,-0.819284919468759,
135.662696415416));
#272264=CARTESIAN_POINT('Ctrl Pts',(-178.272283232261,-0.803275074011935,
135.665356129665));
#272265=CARTESIAN_POINT('Ctrl Pts',(-178.278448654202,-0.690946895868277,
135.683667854268));
#272266=CARTESIAN_POINT('Ctrl Pts',(-178.283175569697,-0.594299441116708,
135.69762350265));
#272267=CARTESIAN_POINT('Ctrl Pts',(-178.29762587154,-0.257144687268308,
135.740133838043));
#272268=CARTESIAN_POINT('Ctrl Pts',(-178.304395271029,-0.0150406824488884,
135.759773395935));
#272269=CARTESIAN_POINT('Ctrl Pts',(-178.311724226144,0.565295564888802,
135.781048775607));
#272270=CARTESIAN_POINT('Ctrl Pts',(-178.308758158221,0.904892298835856,
135.772540046965));
#272271=CARTESIAN_POINT('Ctrl Pts',(-178.284936729491,1.67857512639212,
135.702974800853));
#272272=CARTESIAN_POINT('Ctrl Pts',(-178.2591473322,2.10490618035434,135.627638776919));
#272273=CARTESIAN_POINT('Ctrl Pts',(-178.194644860972,2.84130200828785,
135.429071105338));
#272274=CARTESIAN_POINT('Ctrl Pts',(-178.161544567716,3.14862850841257,
135.324747060875));
#272275=CARTESIAN_POINT('Ctrl Pts',(-178.08287528526,3.78466764810847,135.063692269719));
#272276=CARTESIAN_POINT('Ctrl Pts',(-178.035971305646,4.11310941484443,
134.901002070262));
#272277=CARTESIAN_POINT('Ctrl Pts',(-177.986855337731,4.42643889577882,
134.716028699704));
#272278=CARTESIAN_POINT('Ctrl Pts',(-177.724568368167,-4.0763856389639,
128.064914591592));
#272279=CARTESIAN_POINT('Ctrl Pts',(-177.691585751546,-4.29769346073786,
128.245438695333));
#272280=CARTESIAN_POINT('Ctrl Pts',(-177.658565300108,-4.50476052182415,
128.444579006132));
#272281=CARTESIAN_POINT('Ctrl Pts',(-177.591983415667,-4.91024198597078,
128.913284039984));
#272282=CARTESIAN_POINT('Ctrl Pts',(-177.559170578233,-5.10202391398061,
129.189936967786));
#272283=CARTESIAN_POINT('Ctrl Pts',(-177.511016994937,-5.38947078045,129.745095435989));
#272284=CARTESIAN_POINT('Ctrl Pts',(-177.494082314589,-5.49376686443764,
130.017086379215));
#272285=CARTESIAN_POINT('Ctrl Pts',(-177.479282123345,-5.60168409655279,
130.464069607833));
#272286=CARTESIAN_POINT('Ctrl Pts',(-177.476367722506,-5.6292128072582,
130.63207340011));
#272287=CARTESIAN_POINT('Ctrl Pts',(-177.476367722506,-5.64337912711113,
130.804360617586));
#272288=CARTESIAN_POINT('Ctrl Pts',(-207.34813506021,-2.42719411321803,
126.52758245404));
#272289=CARTESIAN_POINT('Ctrl Pts',(-207.275406626519,-2.16786091358167,
126.278797702914));
#272290=CARTESIAN_POINT('Ctrl Pts',(-207.201807943886,-1.87211081777635,
126.052281281209));
#272291=CARTESIAN_POINT('Ctrl Pts',(-207.11237315121,-1.37178070646407,
125.790031492887));
#272292=CARTESIAN_POINT('Ctrl Pts',(-207.084971087936,-1.18086676444924,
125.712744191699));
#272293=CARTESIAN_POINT('Ctrl Pts',(-207.063270754911,-0.944940672522864,
125.65220001207));
#272294=CARTESIAN_POINT('Ctrl Pts',(-207.060199958288,-0.907909035294405,
125.643661607663));
#272295=CARTESIAN_POINT('Ctrl Pts',(-207.05651245521,-0.857669349578529,
125.633430886317));
#272296=CARTESIAN_POINT('Ctrl Pts',(-207.055601249506,-0.844672757306036,
125.630905093974));
#272297=CARTESIAN_POINT('Ctrl Pts',(-207.053869199003,-0.818733203357481,
125.626107588021));
#272298=CARTESIAN_POINT('Ctrl Pts',(-207.053047813369,-0.805792534069772,
125.623834345885));
#272299=CARTESIAN_POINT('Ctrl Pts',(-207.052056959923,-0.789313017632923,
125.621093920067));
#272300=CARTESIAN_POINT('Ctrl Pts',(-207.051848658496,-0.785795645827727,
125.620517927937));
#272301=CARTESIAN_POINT('Ctrl Pts',(-207.051309755514,-0.77655390024144,
125.619028033472));
#272302=CARTESIAN_POINT('Ctrl Pts',(-207.050984267124,-0.770827036641165,
125.61812844047));
#272303=CARTESIAN_POINT('Ctrl Pts',(-207.050558971052,-0.763143325302232,
125.616953324576));
#272304=CARTESIAN_POINT('Ctrl Pts',(-207.050451847101,-0.761190106292071,
125.616657364513));
#272305=CARTESIAN_POINT('Ctrl Pts',(-207.050281269822,-0.758050935866936,
125.616186141554));
#272306=CARTESIAN_POINT('Ctrl Pts',(-207.050217207391,-0.756865277556876,
125.616009178234));
#272307=CARTESIAN_POINT('Ctrl Pts',(-207.050140480006,-0.755437087963941,
125.615797241911));
#272308=CARTESIAN_POINT('Ctrl Pts',(-207.050127474191,-0.755194716525449,
125.615761317682));
#272309=CARTESIAN_POINT('Ctrl Pts',(-207.050104551004,-0.754767027640041,
125.615698000761));
#272310=CARTESIAN_POINT('Ctrl Pts',(-207.050094627378,-0.754581711618658,
125.61567059062));
#272311=CARTESIAN_POINT('Ctrl Pts',(-207.050079247226,-0.754294241125006,
125.615628109336));
#272312=CARTESIAN_POINT('Ctrl Pts',(-207.050073784885,-0.754192093897613,
125.615613021962));
#272313=CARTESIAN_POINT('Ctrl Pts',(-207.050065117715,-0.754029935148036,
125.615589082738));
#272314=CARTESIAN_POINT('Ctrl Pts',(-207.050061910961,-0.7539699207954,
125.615580225526));
#272315=CARTESIAN_POINT('Ctrl Pts',(-207.050055915098,-0.753857675590644,
125.615563664704));
#272316=CARTESIAN_POINT('Ctrl Pts',(-207.050053125904,-0.753805447395421,
125.615555960854));
#272317=CARTESIAN_POINT('Ctrl Pts',(-207.050046939125,-0.753689569362406,
125.615538872798));
#272318=CARTESIAN_POINT('Ctrl Pts',(-207.050043542009,-0.753625921891587,
125.6155294899));
#272319=CARTESIAN_POINT('Ctrl Pts',(-207.050033723883,-0.753441915123111,
125.615502372131));
#272320=CARTESIAN_POINT('Ctrl Pts',(-207.050027305447,-0.753321553335802,
125.615484644445));
#272321=CARTESIAN_POINT('Ctrl Pts',(-207.049984956323,-0.752526935601,125.615367677068));
#272322=CARTESIAN_POINT('Ctrl Pts',(-207.049949137064,-0.751852627823885,
125.615268748258));
#272323=CARTESIAN_POINT('Ctrl Pts',(-207.049848735386,-0.74995628909578,
125.614991458904));
#272324=CARTESIAN_POINT('Ctrl Pts',(-207.049784416123,-0.748734138025705,
125.614813832405));
#272325=CARTESIAN_POINT('Ctrl Pts',(-207.046900286426,-0.693599268926534,
125.606849368149));
#272326=CARTESIAN_POINT('Ctrl Pts',(-207.04482234318,-0.63943866282689,
125.601129670294));
#272327=CARTESIAN_POINT('Ctrl Pts',(-207.040659911464,-0.464929010650244,
125.589677856696));
#272328=CARTESIAN_POINT('Ctrl Pts',(-207.041642634753,-0.345181292398407,
125.592365210721));
#272329=CARTESIAN_POINT('Ctrl Pts',(-207.053450498118,-0.0530637227305841,
125.624908849078));
#272330=CARTESIAN_POINT('Ctrl Pts',(-207.068272476064,0.114378418145951,
125.665776031825));
#272331=CARTESIAN_POINT('Ctrl Pts',(-207.109163444678,0.432031775628351,
125.78146128078));
#272332=CARTESIAN_POINT('Ctrl Pts',(-207.134520331742,0.580945678162572,
125.854273005136));
#272333=CARTESIAN_POINT('Ctrl Pts',(-207.162924005066,0.722039655879066,
125.938592129034));
#272334=CARTESIAN_POINT('Origin',(210.,0.,130.804360617566));
#272335=CARTESIAN_POINT('',(-207.850862027148,5.62578014279778,132.627039335973));
#272336=CARTESIAN_POINT('Ctrl Pts',(-207.850956227665,5.62869451042201,
132.628018664143));
#272337=CARTESIAN_POINT('Ctrl Pts',(-207.832561498011,5.57924092088534,
132.78065646182));
#272338=CARTESIAN_POINT('Ctrl Pts',(-207.812041489125,5.52351902058675,
132.931423281303));
#272339=CARTESIAN_POINT('Ctrl Pts',(-207.709624216109,5.24091110965318,
133.6098729297));
#272340=CARTESIAN_POINT('Ctrl Pts',(-207.605250752705,4.94131457183235,
134.105628873409));
#272341=CARTESIAN_POINT('Ctrl Pts',(-207.496674502688,4.59187829781674,
134.535658549994));
#272342=CARTESIAN_POINT('',(-207.955976777759,5.91281439438548,130.433367747241));
#272343=CARTESIAN_POINT('Ctrl Pts',(-207.955976777759,5.91281439438548,
130.433367747241));
#272344=CARTESIAN_POINT('Ctrl Pts',(-207.947415967503,5.92542666017732,
130.614125802698));
#272345=CARTESIAN_POINT('Ctrl Pts',(-207.912377717299,5.94123870869834,
131.355802411338));
#272346=CARTESIAN_POINT('Ctrl Pts',(-207.877339467095,5.80436545607685,
132.093047857022));
#272347=CARTESIAN_POINT('Ctrl Pts',(-207.850862027148,5.62578014279735,
132.627039335975));
#272348=CARTESIAN_POINT('Ctrl Pts',(-207.794849275159,5.47606313559233,
128.563676994761));
#272349=CARTESIAN_POINT('Ctrl Pts',(-207.883928897283,5.72131300358244,
129.163049323563));
#272350=CARTESIAN_POINT('Ctrl Pts',(-207.940709210396,5.86582931839541,
129.807281383254));
#272351=CARTESIAN_POINT('Ctrl Pts',(-207.955943877287,5.9051406252583,130.43389502075));
#272352=CARTESIAN_POINT('Ctrl Pts',(210.578629502474,3.43871735229388,135.623751273273));
#272353=CARTESIAN_POINT('Ctrl Pts',(210.532211638871,4.24191310225744,135.050661598608));
#272354=CARTESIAN_POINT('Ctrl Pts',(210.439385837966,5.5417116830592,133.497735776206));
#272355=CARTESIAN_POINT('Ctrl Pts',(210.253744162458,6.40049231640402,129.500124813146));
#272356=CARTESIAN_POINT('Ctrl Pts',(210.021704475947,3.49988613106459,124.739836436729));
#272357=CARTESIAN_POINT('Ctrl Pts',(209.743256852134,-3.22132718841443,
124.582443963435));
#272358=CARTESIAN_POINT('Ctrl Pts',(209.464809228321,-6.97029916743427,
130.151104711613));
#272359=CARTESIAN_POINT('Ctrl Pts',(209.186361604508,-4.320155850937,136.315756482887));
#272360=CARTESIAN_POINT('Ctrl Pts',(208.907913980696,2.30329626696544,137.417975354914));
#272361=CARTESIAN_POINT('Ctrl Pts',(208.629466356883,6.80838731381026,132.441404887444));
#272362=CARTESIAN_POINT('Ctrl Pts',(208.35101873307,5.05782663488002,125.961106241921));
#272363=CARTESIAN_POINT('Ctrl Pts',(208.072571109257,-1.34111875541754,
123.931185212061));
#272364=CARTESIAN_POINT('Ctrl Pts',(207.794123485444,-6.50738248846785,
128.217554840719));
#272365=CARTESIAN_POINT('Ctrl Pts',(207.515675861631,-5.69381680528821,
134.880978212762));
#272366=CARTESIAN_POINT('Ctrl Pts',(207.237228237818,0.352161018465804,
137.798239159538));
#272367=CARTESIAN_POINT('Ctrl Pts',(206.958780614005,6.07448159193836,134.288440920842));
#272368=CARTESIAN_POINT('Ctrl Pts',(206.680332990192,6.21467071562046,127.576957111676));
#272369=CARTESIAN_POINT('Ctrl Pts',(206.40188536638,0.643870262773591,123.831292031177));
#272370=CARTESIAN_POINT('Ctrl Pts',(206.123437742567,-5.51860979104455,
126.493540260974));
#272371=CARTESIAN_POINT('Ctrl Pts',(205.844990118754,-6.60976007302988,
133.117219720399));
#272372=CARTESIAN_POINT('Ctrl Pts',(205.566542494941,-1.62686214948821,
137.615495756827));
#272373=CARTESIAN_POINT('Ctrl Pts',(205.288094871128,4.8510417637676,135.85467075854));
#272374=CARTESIAN_POINT('Ctrl Pts',(205.009647247315,6.87107573233629,129.452857771449));
#272375=CARTESIAN_POINT('Ctrl Pts',(204.731199623502,2.57692653546199,124.293009711503));
#272376=CARTESIAN_POINT('Ctrl Pts',(204.452751999689,-4.08529213152394,
125.116775123829));
#272377=CARTESIAN_POINT('Ctrl Pts',(204.174304375876,-6.9933269740478,131.167153704944));
#272378=CARTESIAN_POINT('Ctrl Pts',(203.895856752063,-3.47483593506387,
136.884143186524));
#272379=CARTESIAN_POINT('Ctrl Pts',(203.617409128251,3.23685955433703,137.014109488232));
#272380=CARTESIAN_POINT('Ctrl Pts',(203.338961504438,6.97403925260401,131.437619947721));
#272381=CARTESIAN_POINT('Ctrl Pts',(203.060513880625,4.30241757323156,125.27919601562));
#272382=CARTESIAN_POINT('Ctrl Pts',(202.782066256812,-2.32291566837452,
124.198128435325));
#272383=CARTESIAN_POINT('Ctrl Pts',(202.503618632999,-6.81360289295739,
129.18786549711));
#272384=CARTESIAN_POINT('Ctrl Pts',(202.225171009186,-5.0429219211382,135.663082604955));
#272385=CARTESIAN_POINT('Ctrl Pts',(201.946723385373,1.36195793536179,137.673371567868));
#272386=CARTESIAN_POINT('Ctrl Pts',(201.66827576156,6.51526498482727,133.371375037445));
#272387=CARTESIAN_POINT('Ctrl Pts',(201.389828137747,5.6813618015098,126.710417660699));
#272388=CARTESIAN_POINT('Ctrl Pts',(201.111380513935,-0.373435327379839,
123.811593861123));
#272389=CARTESIAN_POINT('Ctrl Pts',(200.832932890122,-6.08506363376988,
127.338781095048));
#272390=CARTESIAN_POINT('Ctrl Pts',(200.554485266309,-6.20481573259303,
134.050666607207));
#272391=CARTESIAN_POINT('Ctrl Pts',(200.276037642496,-0.622645295272457,
137.779355505743));
#272392=CARTESIAN_POINT('Ctrl Pts',(199.997590018683,5.53170575049466,135.098364849491));
#272393=CARTESIAN_POINT('Ctrl Pts',(199.71914239487,6.60268945040398,128.471394077867));
#272394=CARTESIAN_POINT('Ctrl Pts',(199.440694771057,1.60612410470526,123.988305584475));
#272395=CARTESIAN_POINT('Ctrl Pts',(199.162247147244,-4.86639082969376,
125.768838683693));
#272396=CARTESIAN_POINT('Ctrl Pts',(198.883799523432,-6.86693032801245,
132.176770441218));
#272397=CARTESIAN_POINT('Ctrl Pts',(198.605351899619,-2.5570963230842,137.323524616753));
#272398=CARTESIAN_POINT('Ctrl Pts',(198.326904275806,4.10258428165832,136.479485555902));
#272399=CARTESIAN_POINT('Ctrl Pts',(198.048456651993,6.99219035394115,130.420283921986));
#272400=CARTESIAN_POINT('Ctrl Pts',(197.77000902818,3.45631507844086,124.714030008118));
#272401=CARTESIAN_POINT('Ctrl Pts',(197.491561404367,-3.25574490376804,
124.604492395141));
#272402=CARTESIAN_POINT('Ctrl Pts',(197.213113780554,-6.97593437139489,
130.192330798173));
#272403=CARTESIAN_POINT('Ctrl Pts',(196.934666156741,-4.28558094504976,
136.342594705906));
#272404=CARTESIAN_POINT('Ctrl Pts',(196.656218532928,2.3430120075278,137.403492044232));
#272405=CARTESIAN_POINT('Ctrl Pts',(196.377770909115,6.81849138768721,132.400109986944));
#272406=CARTESIAN_POINT('Ctrl Pts',(196.099323285303,5.02811028438465,125.930312215887));
#272407=CARTESIAN_POINT('Ctrl Pts',(195.82087566149,-1.38285853342424,123.939526815472));
#272408=CARTESIAN_POINT('Ctrl Pts',(195.542428037677,-6.5230479154113,128.257188313404));
#272409=CARTESIAN_POINT('Ctrl Pts',(195.263980413864,-5.66887493174189,
134.915576722577));
#272410=CARTESIAN_POINT('Ctrl Pts',(194.985532790051,0.394717174261835,
137.795958375315));
#272411=CARTESIAN_POINT('Ctrl Pts',(194.707085166238,6.09558348012494,134.251403247221));
#272412=CARTESIAN_POINT('Ctrl Pts',(194.428637542425,6.19490635356113,127.539184339867));
#272413=CARTESIAN_POINT('Ctrl Pts',(194.150189918612,0.601412926074683,
123.827502918989));
#272414=CARTESIAN_POINT('Ctrl Pts',(193.871742294799,-5.54474959981957,
126.527212884656));
#272415=CARTESIAN_POINT('Ctrl Pts',(193.593294670987,-6.59555811955654,
133.157412666584));
#272416=CARTESIAN_POINT('Ctrl Pts',(193.314847047174,-1.58537093834796,
137.625272568447));
#272417=CARTESIAN_POINT('Ctrl Pts',(193.036399423361,4.88169468552635,135.825047607524));
#272418=CARTESIAN_POINT('Ctrl Pts',(192.757951799548,6.86272137744547,129.411056577024));
#272419=CARTESIAN_POINT('Ctrl Pts',(192.479504175735,2.53724238606986,124.277443893095));
#272420=CARTESIAN_POINT('Ctrl Pts',(192.201056551922,-4.11983840692253,
125.141748821346));
#272421=CARTESIAN_POINT('Ctrl Pts',(191.922608928109,-6.99098896924831,
131.209717356357));
#272422=CARTESIAN_POINT('Ctrl Pts',(191.644161304296,-3.43776219763276,
136.905182851196));
#272423=CARTESIAN_POINT('Ctrl Pts',(191.365713680483,3.27460008958736,136.994290755064));
#272424=CARTESIAN_POINT('Ctrl Pts',(191.08726605667,6.9777648675845,131.395155257469));
#272425=CARTESIAN_POINT('Ctrl Pts',(190.808818432858,4.26870461503614,125.253108347726));
#272426=CARTESIAN_POINT('Ctrl Pts',(190.530370809044,-2.36308664091672,
124.212391080215));
#272427=CARTESIAN_POINT('Ctrl Pts',(190.251923185232,-6.82331671706736,
129.229371781915));
#272428=CARTESIAN_POINT('Ctrl Pts',(189.973475561419,-5.01325206778612,
135.693690281095));
#272429=CARTESIAN_POINT('Ctrl Pts',(189.695027937606,1.40374632081163,137.664953676525));
#272430=CARTESIAN_POINT('Ctrl Pts',(189.416580313793,6.53077041740369,133.331667209374));
#272431=CARTESIAN_POINT('Ctrl Pts',(189.13813268998,5.65633554627347,126.675909450142));
#272432=CARTESIAN_POINT('Ctrl Pts',(188.859685066167,-0.41599536452862,
123.81399662772));
#272433=CARTESIAN_POINT('Ctrl Pts',(188.581237442354,-6.10604685783229,
127.375886813701));
#272434=CARTESIAN_POINT('Ctrl Pts',(188.302789818542,-6.18493958576042,
134.088376935175));
#272435=CARTESIAN_POINT('Ctrl Pts',(188.024342194729,-0.580174985471077,
137.783016493883));
#272436=CARTESIAN_POINT('Ctrl Pts',(187.745894570916,5.55774208334242,135.064612228548));
#272437=CARTESIAN_POINT('Ctrl Pts',(187.467446947103,6.58836568835925,128.431244857581));
#272438=CARTESIAN_POINT('Ctrl Pts',(187.18899932329,1.56460308533104,123.97865493689));
#272439=CARTESIAN_POINT('Ctrl Pts',(186.910551699478,-4.89695331800637,
125.798555082479));
#272440=CARTESIAN_POINT('Ctrl Pts',(186.632104075664,-6.85844885156509,
132.218545967617));
#272441=CARTESIAN_POINT('Ctrl Pts',(186.353656451852,-2.51736494438869,
137.338969602853));
#272442=CARTESIAN_POINT('Ctrl Pts',(186.075208828038,4.13705436656654,136.454406814005));
#272443=CARTESIAN_POINT('Ctrl Pts',(185.796761204226,6.98972282098866,130.377727590732));
#272444=CARTESIAN_POINT('Ctrl Pts',(185.518313580413,3.41917746986535,124.693103276936));
#272445=CARTESIAN_POINT('Ctrl Pts',(185.2398659566,-3.29342493995873,124.62442590766));
#272446=CARTESIAN_POINT('Ctrl Pts',(184.961418332787,-6.97953072271363,
130.234806630193));
#272447=CARTESIAN_POINT('Ctrl Pts',(184.682970708974,-4.25178874032612,
136.368579642862));
#272448=CARTESIAN_POINT('Ctrl Pts',(184.404523085161,2.38313938299372,137.389107198495));
#272449=CARTESIAN_POINT('Ctrl Pts',(184.126075461348,6.82807883617355,132.358574329007));
#272450=CARTESIAN_POINT('Ctrl Pts',(183.847627837535,4.99834740910532,125.899794986266));
#272451=CARTESIAN_POINT('Ctrl Pts',(183.569180213722,-1.42462110408482,
123.948071857337));
#272452=CARTESIAN_POINT('Ctrl Pts',(183.290732589909,-6.53843241923107,
128.296943150732));
#272453=CARTESIAN_POINT('Ctrl Pts',(183.012284966097,-5.64374376128527,
134.950008601993));
#272454=CARTESIAN_POINT('Ctrl Pts',(182.733837342284,0.437269701071178,
137.793426081729));
#272455=CARTESIAN_POINT('Ctrl Pts',(182.455389718471,6.11645366995566,134.214233834728));
#272456=CARTESIAN_POINT('Ctrl Pts',(182.176942094658,6.17491552152431,127.501534682722));
#272457=CARTESIAN_POINT('Ctrl Pts',(181.898494470845,0.558931670205695,
123.82397121282));
#272458=CARTESIAN_POINT('Ctrl Pts',(181.620046847032,-5.57068308070185,
126.561044594899));
#272459=CARTESIAN_POINT('Ctrl Pts',(181.341599223219,-6.58111222344223,
133.197518104296));
#272460=CARTESIAN_POINT('Ctrl Pts',(181.063151599407,-1.54382073804491,
137.634796795631));
#272461=CARTESIAN_POINT('Ctrl Pts',(180.784703975594,4.91216658577983,135.795238324681));
#272462=CARTESIAN_POINT('Ctrl Pts',(180.506256351781,6.85411278995147,129.369307058824));
#272463=CARTESIAN_POINT('Ctrl Pts',(180.227808727968,2.49746418218255,124.262119907186));
#272464=CARTESIAN_POINT('Ctrl Pts',(179.949361104155,-4.15423200110403,
125.16693236216));
#272465=CARTESIAN_POINT('Ctrl Pts',(179.670913480342,-6.98839192089168,
131.252265980172));
#272466=CARTESIAN_POINT('Ctrl Pts',(179.392465856529,-3.40056106730489,
136.925996451342));
#272467=CARTESIAN_POINT('Ctrl Pts',(179.114018232716,3.31221928049139,136.974242649806));
#272468=CARTESIAN_POINT('Ctrl Pts',(178.835570608904,6.98123192042358,131.352668676138));
#272469=CARTESIAN_POINT('Ctrl Pts',(178.55712298509,4.23483347762603,125.227226382977));
#272470=CARTESIAN_POINT('Ctrl Pts',(178.278675361277,-2.40317004799311,
124.22689799325));
#272471=CARTESIAN_POINT('Ctrl Pts',(178.000227737465,-6.83277770089014,
129.270936428355));
#272472=CARTESIAN_POINT('Ctrl Pts',(177.721780113652,-4.98339644641697,
135.724116781409));
#272473=CARTESIAN_POINT('Ctrl Pts',(177.443332489839,1.44548268986267,137.65628156334));
#272474=CARTESIAN_POINT('Ctrl Pts',(177.164884866026,6.54603384991367,133.291865731052));
#272475=CARTESIAN_POINT('Ctrl Pts',(176.886437242213,5.63109969342586,126.64155422085));
#272476=CARTESIAN_POINT('Ctrl Pts',(176.6079896184,-0.458539986806858,123.816658424832));
#272477=CARTESIAN_POINT('Ctrl Pts',(176.329541994587,-6.12680382008778,
127.413119575705));
#272478=CARTESIAN_POINT('Ctrl Pts',(176.051094370774,-6.16483425371434,
134.125965572714));
#272479=CARTESIAN_POINT('Ctrl Pts',(175.772646746962,-0.537683177073775,
137.786418885364));
#272480=CARTESIAN_POINT('Ctrl Pts',(175.494199123148,5.58357247201413,135.030701742416));
#272481=CARTESIAN_POINT('Ctrl Pts',(175.215751499336,6.57379779200069,128.391183573973));
#272482=CARTESIAN_POINT('Ctrl Pts',(174.937303875523,1.5230240890144,123.969257218339));
#272483=CARTESIAN_POINT('Ctrl Pts',(174.65885625171,-4.92733434791298,125.82845697323));
#272484=CARTESIAN_POINT('Ctrl Pts',(174.380408627897,-6.84971323277332,
132.260269090858));
#272485=CARTESIAN_POINT('Ctrl Pts',(174.101961004084,-2.4775402838095,137.354172446613));
#272486=CARTESIAN_POINT('Ctrl Pts',(173.823513380271,4.1713711514037,136.429118707571));
#272487=CARTESIAN_POINT('Ctrl Pts',(173.545065756458,6.98699628128659,130.335187068521));
#272488=CARTESIAN_POINT('Ctrl Pts',(173.266618132645,3.38191316241135,124.672403000642));
#272489=CARTESIAN_POINT('Ctrl Pts',(172.988170508833,-3.33098293707706,
124.644588419932));
#272490=CARTESIAN_POINT('Ctrl Pts',(172.709722885019,-6.98286844495469,
130.277303567246));
#272491=CARTESIAN_POINT('Ctrl Pts',(172.431275261207,-4.21783898400718,
136.394358395635));
#272492=CARTESIAN_POINT('Ctrl Pts',(172.152827637394,2.42317845035331,137.374478352552));
#272493=CARTESIAN_POINT('Ctrl Pts',(171.874380013581,6.83741326768756,132.316981079111));
#272494=CARTESIAN_POINT('Ctrl Pts',(171.595932389768,4.96839931822471,125.869459497128));
#272495=CARTESIAN_POINT('Ctrl Pts',(171.317484765955,-1.46633088488636,
123.956870961504));
#272496=CARTESIAN_POINT('Ctrl Pts',(171.039037142142,-6.55357463903296,
128.336790901335));
#272497=CARTESIAN_POINT('Ctrl Pts',(170.760589518329,-5.61840345982816,
134.984286862899));
#272498=CARTESIAN_POINT('Ctrl Pts',(170.482141894517,0.479806024690783,
137.79063480575));
#272499=CARTESIAN_POINT('Ctrl Pts',(170.203694270703,6.13709721234627,134.176938068128));
#272500=CARTESIAN_POINT('Ctrl Pts',(169.925246646891,6.15469587572206,127.464007413007));
#272501=CARTESIAN_POINT('Ctrl Pts',(169.646799023078,0.51642970291829,123.820698167548));
#272502=CARTESIAN_POINT('Ctrl Pts',(169.368351399265,-5.59641013787386,
126.595033542778));
#272503=CARTESIAN_POINT('Ctrl Pts',(169.089903775452,-6.56642246179436,
133.237534862678));
#272504=CARTESIAN_POINT('Ctrl Pts',(168.811456151639,-1.50221333089678,
137.644067918489));
#272505=CARTESIAN_POINT('Ctrl Pts',(168.533008527826,4.94245646389391,135.76524410303));
#272506=CARTESIAN_POINT('Ctrl Pts',(168.254560904013,6.84525022078748,129.32761071706));
#272507=CARTESIAN_POINT('Ctrl Pts',(167.976113280201,2.45759343384159,124.247038346411));
#272508=CARTESIAN_POINT('Ctrl Pts',(167.697665656387,-4.1884716586909,125.192324799951));
#272509=CARTESIAN_POINT('Ctrl Pts',(167.419218032575,-6.98553591510243,
131.294798006688));
#272510=CARTESIAN_POINT('Ctrl Pts',(167.140770408762,-3.36323392793624,
136.946583212019));
#272511=CARTESIAN_POINT('Ctrl Pts',(166.862322784949,3.34971573589186,136.953965917302));
#272512=CARTESIAN_POINT('Ctrl Pts',(166.583875161136,6.98444028114645,131.310161777048));
#272513=CARTESIAN_POINT('Ctrl Pts',(166.305427537323,4.20080541690416,125.20155108099));
#272514=CARTESIAN_POINT('Ctrl Pts',(166.02697991351,-2.44316440471955,124.241648636582));
#272515=CARTESIAN_POINT('Ctrl Pts',(165.748532289697,-6.84198549362249,
129.312557896394));
#272516=CARTESIAN_POINT('Ctrl Pts',(165.470084665885,-4.95335616345982,
135.754360978348));
#272517=CARTESIAN_POINT('Ctrl Pts',(165.191637042072,1.48716549602113,137.647355549705));
#272518=CARTESIAN_POINT('Ctrl Pts',(164.913189418259,6.56105471673207,133.251972077313));
#272519=CARTESIAN_POINT('Ctrl Pts',(164.634741794446,5.60565517810829,126.60735324588));
#272520=CARTESIAN_POINT('Ctrl Pts',(164.356294170633,-0.501067617717217,
123.819579153818));
#272521=CARTESIAN_POINT('Ctrl Pts',(164.07784654682,-6.1473337513746,127.450478001396));
#272522=CARTESIAN_POINT('Ctrl Pts',(163.799398923007,-6.14450048146789,
134.163431126959));
#272523=CARTESIAN_POINT('Ctrl Pts',(163.520951299194,-0.495171444628521,
137.789562554107));
#272524=CARTESIAN_POINT('Ctrl Pts',(163.242503675381,5.60919595935461,134.996634647659));
#272525=CARTESIAN_POINT('Ctrl Pts',(162.964056051569,6.55898630114736,128.351211711527));
#272526=CARTESIAN_POINT('Ctrl Pts',(162.685608427755,1.48138865648,123.960112777059));
#272527=CARTESIAN_POINT('Ctrl Pts',(162.407160803943,-4.95753279363329,
125.85854324792));
#272528=CARTESIAN_POINT('Ctrl Pts',(162.12871318013,-6.84072379533872,132.301938264875));
#272529=CARTESIAN_POINT('Ctrl Pts',(161.850265556317,-2.4376238170639,137.369132584688));
#272530=CARTESIAN_POINT('Ctrl Pts',(161.571817932504,4.20553336454888,136.403622173655));
#272531=CARTESIAN_POINT('Ctrl Pts',(161.293370308691,6.98401083586784,130.292663931709));
#272532=CARTESIAN_POINT('Ctrl Pts',(161.014922684878,3.34452353692138,124.651929946293));
#272533=CARTESIAN_POINT('Ctrl Pts',(160.736475061065,-3.36841750339773,
124.664979184829));
#272534=CARTESIAN_POINT('Ctrl Pts',(160.458027437253,-6.98594741443756,
130.319820034592));
#272535=CARTESIAN_POINT('Ctrl Pts',(160.179579813439,-4.18373293411359,
136.419930008985));
#272536=CARTESIAN_POINT('Ctrl Pts',(159.901132189627,2.46312772594441,137.35960604848));
#272537=CARTESIAN_POINT('Ctrl Pts',(159.622684565814,6.84649433633851,132.275331778507));
#272538=CARTESIAN_POINT('Ctrl Pts',(159.344236942001,4.93826712148011,125.839306872565));
#272539=CARTESIAN_POINT('Ctrl Pts',(159.065789318188,-1.50798633025781,
123.965923801919));
#272540=CARTESIAN_POINT('Ctrl Pts',(158.787341694375,-6.56847401371661,
128.376730088641));
#272541=CARTESIAN_POINT('Ctrl Pts',(158.508894070562,-5.59285496636459,
135.018410235101));
#272542=CARTESIAN_POINT('Ctrl Pts',(158.230446446749,0.522324568921774,
137.787584650814));
#272543=CARTESIAN_POINT('Ctrl Pts',(157.951998822937,6.15751334234277,134.139517329431));
#272544=CARTESIAN_POINT('Ctrl Pts',(157.673551199123,6.13424816540071,127.426603921307));
#272545=CARTESIAN_POINT('Ctrl Pts',(157.395103575311,0.473908599138188,
123.817683904457));
#272546=CARTESIAN_POINT('Ctrl Pts',(157.116655951498,-5.62192981801017,
126.62917846882));
#272547=CARTESIAN_POINT('Ctrl Pts',(156.838208327685,-6.55148937894732,
133.277461458893));
#272548=CARTESIAN_POINT('Ctrl Pts',(156.559760703872,-1.46055025868114,
137.653085593479));
#272549=CARTESIAN_POINT('Ctrl Pts',(156.281313080059,4.97256319746619,135.735066054016));
#272550=CARTESIAN_POINT('Ctrl Pts',(156.002865456246,6.83613399835919,129.285969096806));
#272551=CARTESIAN_POINT('Ctrl Pts',(155.724417832433,2.4176316184721,124.232199769625));
#272552=CARTESIAN_POINT('Ctrl Pts',(155.44597020862,-4.2225561109203,125.217925193794));
#272553=CARTESIAN_POINT('Ctrl Pts',(155.167522584808,-6.98242105771092,
131.337311859867));
#272554=CARTESIAN_POINT('Ctrl Pts',(154.889074960995,-3.3257821626974,136.96694237038));
#272555=CARTESIAN_POINT('Ctrl Pts',(154.610627337182,3.38708806634394,136.933461308912));
#272556=CARTESIAN_POINT('Ctrl Pts',(154.332179713369,6.98738983086623,131.267636135312));
#272557=CARTESIAN_POINT('Ctrl Pts',(154.053732089556,4.1666216937926,125.17608339317));
#272558=CARTESIAN_POINT('Ctrl Pts',(153.775284465743,-2.48306822909056,
124.256642463619));
#272559=CARTESIAN_POINT('Ctrl Pts',(153.49683684193,-6.85093975406627,129.354234643731));
#272560=CARTESIAN_POINT('Ctrl Pts',(153.218389218117,-4.92313233206838,
135.784421751204));
#272561=CARTESIAN_POINT('Ctrl Pts',(152.939941594304,1.52879319471521,137.638175966376));
#272562=CARTESIAN_POINT('Ctrl Pts',(152.661493970491,6.57583246125511,133.21198772643));
#272563=CARTESIAN_POINT('Ctrl Pts',(152.383046346679,5.58000294317656,126.573307792561));
#272564=CARTESIAN_POINT('Ctrl Pts',(152.104598722866,-0.543576681382813,
123.822758706449));
#272565=CARTESIAN_POINT('Ctrl Pts',(151.826151099053,-6.16763589094857,
127.487960706439));
#272566=CARTESIAN_POINT('Ctrl Pts',(151.54770347524,-6.12393902249645,134.200772209611));
#272567=CARTESIAN_POINT('Ctrl Pts',(151.269255851427,-0.452641363423277,
137.792447383624));
#272568=CARTESIAN_POINT('Ctrl Pts',(150.990808227614,5.63461159587598,134.962412206646));
#272569=CARTESIAN_POINT('Ctrl Pts',(150.712360603801,6.54393176464461,128.311330751416));
#272570=CARTESIAN_POINT('Ctrl Pts',(150.433912979988,1.4396983305442,123.951221951899));
#272571=CARTESIAN_POINT('Ctrl Pts',(150.155465356176,-4.98754753615285,
125.888812791691));
#272572=CARTESIAN_POINT('Ctrl Pts',(149.877017732362,-6.83148087236823,
132.343551945603));
#272573=CARTESIAN_POINT('Ctrl Pts',(149.59857010855,-2.39761702327129,137.383849462723));
#272574=CARTESIAN_POINT('Ctrl Pts',(149.320122484737,4.23953974010866,136.377918157044));
#272575=CARTESIAN_POINT('Ctrl Pts',(149.041674860924,6.98076659535922,130.250159756006));
#272576=CARTESIAN_POINT('Ctrl Pts',(148.763227237111,3.30700997888175,124.631684872525));
#272577=CARTESIAN_POINT('Ctrl Pts',(148.484779613298,-3.40572725176907,
124.685597446761));
#272578=CARTESIAN_POINT('Ctrl Pts',(148.206331989485,-6.98876751706998,
130.362354456768));
#272579=CARTESIAN_POINT('Ctrl Pts',(147.927884365672,-4.14947185445744,
136.445293535346));
#272580=CARTESIAN_POINT('Ctrl Pts',(147.649436741859,2.50298572943186,137.344490837378));
#272581=CARTESIAN_POINT('Ctrl Pts',(147.370989118047,6.85532170562399,132.233627970525));
#272582=CARTESIAN_POINT('Ctrl Pts',(147.092541494233,4.90795193543132,125.809338229895));
#272583=CARTESIAN_POINT('Ctrl Pts',(146.814093870421,-1.54958589664124,
123.975230043125));
#272584=CARTESIAN_POINT('Ctrl Pts',(146.535646246608,-6.58312999118006,
128.41675923269));
#272585=CARTESIAN_POINT('Ctrl Pts',(146.257198622795,-5.56709922760349,
135.052377454143));
#272586=CARTESIAN_POINT('Ctrl Pts',(145.978750998982,0.564823758223794,
137.784275729942));
#272587=CARTESIAN_POINT('Ctrl Pts',(145.700303375169,6.17770130341801,134.101973005276));
#272588=CARTESIAN_POINT('Ctrl Pts',(145.421855751356,6.11357314825767,127.389325593625));
#272589=CARTESIAN_POINT('Ctrl Pts',(145.143408127543,0.431369934500661,
123.81492853524));
#272590=CARTESIAN_POINT('Ctrl Pts',(144.864960503731,-5.64724117546963,
126.663478107772));
#272591=CARTESIAN_POINT('Ctrl Pts',(144.586512879918,-6.53631352825206,
133.317296413447));
#272592=CARTESIAN_POINT('Ctrl Pts',(144.308065256105,-1.41883306523854,
137.661849486446));
#272593=CARTESIAN_POINT('Ctrl Pts',(144.029617632292,5.00248567088053,135.704705295899));
#272594=CARTESIAN_POINT('Ctrl Pts',(143.751170008479,6.82676446047164,129.244383741109));
#272595=CARTESIAN_POINT('Ctrl Pts',(143.472722384666,2.37758021687388,124.217604726676));
#272596=CARTESIAN_POINT('Ctrl Pts',(143.194274760853,-4.25648409478009,
125.243732595056));
#272597=CARTESIAN_POINT('Ctrl Pts',(142.91582713704,-6.97904746413934,131.379805964341));
#272598=CARTESIAN_POINT('Ctrl Pts',(142.637379513228,-3.28820715937746,
136.987073172008));
#272599=CARTESIAN_POINT('Ctrl Pts',(142.358931889414,3.42433488700229,136.912729584442));
#272600=CARTESIAN_POINT('Ctrl Pts',(142.080484265602,6.99008046028611,131.225093326731));
#272601=CARTESIAN_POINT('Ctrl Pts',(141.802036641788,4.13228357498186,125.150824263232));
#272602=CARTESIAN_POINT('Ctrl Pts',(141.523589017976,-2.52288004245522,
124.271878918761));
#272603=CARTESIAN_POINT('Ctrl Pts',(141.245141394163,-6.859640150418,129.395965126019));
#272604=CARTESIAN_POINT('Ctrl Pts',(140.96669377035,-4.89272607219785,135.814297986063));
#272605=CARTESIAN_POINT('Ctrl Pts',(140.688246146537,1.57036424341533,137.628743153505));
#272606=CARTESIAN_POINT('Ctrl Pts',(140.409798522724,6.59036653588803,133.17191416004));
#272607=CARTESIAN_POINT('Ctrl Pts',(140.131350898911,5.55414393918375,126.539419122461));
#272608=CARTESIAN_POINT('Ctrl Pts',(139.852903275098,-0.586065602614643,
123.826196964908));
#272609=CARTESIAN_POINT('Ctrl Pts',(139.574455651286,-6.18770948650656,
127.525566301902));
#272610=CARTESIAN_POINT('Ctrl Pts',(139.296008027473,-6.10315063871238,
134.237987436982));
#272611=CARTESIAN_POINT('Ctrl Pts',(139.01756040366,-0.410094509425858,
137.795073267016));
#272612=CARTESIAN_POINT('Ctrl Pts',(138.739112779847,5.65981843979252,134.928035687503));
#272613=CARTESIAN_POINT('Ctrl Pts',(138.460665156034,6.52863474034383,128.271542171445));
#272614=CARTESIAN_POINT('Ctrl Pts',(138.182217532221,1.39795465605713,123.942585072312));
#272615=CARTESIAN_POINT('Ctrl Pts',(137.903769908408,-5.01737746326431,
125.919264482896));
#272616=CARTESIAN_POINT('Ctrl Pts',(137.625322284595,-6.82198480636163,
132.385108591028));
#272617=CARTESIAN_POINT('Ctrl Pts',(137.346874660782,-2.35752138489827,
137.39832253538));
#272618=CARTESIAN_POINT('Ctrl Pts',(137.06842703697,4.27338901796432,136.352007610208));
#272619=CARTESIAN_POINT('Ctrl Pts',(136.789979413157,6.9772636799772,130.20767611642));
#272620=CARTESIAN_POINT('Ctrl Pts',(136.511531789344,3.26937387837121,124.611668529527));
#272621=CARTESIAN_POINT('Ctrl Pts',(136.233084165531,-3.44291079966457,
124.706442441713));
#272622=CARTESIAN_POINT('Ctrl Pts',(135.954636541718,-6.99132864835187,
130.404905257644));
#272623=CARTESIAN_POINT('Ctrl Pts',(135.676188917905,-4.1150570145959,136.470448034864));
#272624=CARTESIAN_POINT('Ctrl Pts',(135.397741294092,2.54275098386259,137.329133279345));
#272625=CARTESIAN_POINT('Ctrl Pts',(135.11929367028,6.8638950484427,132.191871200516));
#272626=CARTESIAN_POINT('Ctrl Pts',(134.840846046466,4.87745488341857,125.779554679616));
#272627=CARTESIAN_POINT('Ctrl Pts',(134.562398422654,-1.59112804254939,
123.984789340275));
#272628=CARTESIAN_POINT('Ctrl Pts',(134.283950798841,-6.59754202834077,
128.456876850186));
#272629=CARTESIAN_POINT('Ctrl Pts',(134.005503175028,-5.54113719793324,
135.086187261361));
#272630=CARTESIAN_POINT('Ctrl Pts',(133.727055551215,0.607302017773813,
137.780708165749));
#272631=CARTESIAN_POINT('Ctrl Pts',(133.448607927402,6.19766034749954,134.064306486881));
#272632=CARTESIAN_POINT('Ctrl Pts',(133.170160303589,6.09267159041341,127.352173811322));
#272633=CARTESIAN_POINT('Ctrl Pts',(132.891712679776,0.388815285291658,
123.812432161999));
#272634=CARTESIAN_POINT('Ctrl Pts',(132.613265055963,-5.67234327233058,
126.697931188648));
#272635=CARTESIAN_POINT('Ctrl Pts',(132.334817432151,-6.52089547205522,
133.357038250242));
#272636=CARTESIAN_POINT('Ctrl Pts',(132.056369808337,-1.37706329641493,
137.670359272641));
#272637=CARTESIAN_POINT('Ctrl Pts',(131.777922184525,5.0322227753486,135.674162953708));
#272638=CARTESIAN_POINT('Ctrl Pts',(131.499474560712,6.81714195431646,129.20285619093));
#272639=CARTESIAN_POINT('Ctrl Pts',(131.221026936899,2.33744071316646,124.203253758389));
#272640=CARTESIAN_POINT('Ctrl Pts',(130.942579313086,-4.29025435305649,
125.269746047434));
#272641=CARTESIAN_POINT('Ctrl Pts',(130.664131689273,-6.97541525939744,
131.422278745477));
#272642=CARTESIAN_POINT('Ctrl Pts',(130.38568406546,-3.25051031033198,137.006974870947));
#272643=CARTESIAN_POINT('Ctrl Pts',(130.107236441647,3.46145481767177,136.891771512113));
#272644=CARTESIAN_POINT('Ctrl Pts',(129.828788817834,6.99251206970404,131.182534927744));
#272645=CARTESIAN_POINT('Ctrl Pts',(129.550341194022,4.09779233288376,125.125774627163));
#272646=CARTESIAN_POINT('Ctrl Pts',(129.271893570209,-2.5625983695722,124.287357437414));
#272647=CARTESIAN_POINT('Ctrl Pts',(128.993445946396,-6.86808636028122,
129.43774779692));
#272648=CARTESIAN_POINT('Ctrl Pts',(128.714998322583,-4.86213851056362,
135.84398857585));
#272649=CARTESIAN_POINT('Ctrl Pts',(128.43655069877,1.61187710169066,137.61905746063));
#272650=CARTESIAN_POINT('Ctrl Pts',(128.158103074957,6.60465640206541,133.131752863082));
#272651=CARTESIAN_POINT('Ctrl Pts',(127.879655451144,5.52807912434469,126.505688491336));
#272652=CARTESIAN_POINT('Ctrl Pts',(127.601207827331,-0.628532806970051,
123.829893801787));
#272653=CARTESIAN_POINT('Ctrl Pts',(127.322760203518,-6.20755379421381,
127.563293394292));
#272654=CARTESIAN_POINT('Ctrl Pts',(127.044312579706,-6.08213610043705,
134.275075430049));
#272655=CARTESIAN_POINT('Ctrl Pts',(126.765864955893,-0.367532459225645,
137.797440106979));
#272656=CARTESIAN_POINT('Ctrl Pts',(126.48741733208,5.68481555705546,134.893506364063));
#272657=CARTESIAN_POINT('Ctrl Pts',(126.208969708267,6.51309579508176,128.231847445991));
#272658=CARTESIAN_POINT('Ctrl Pts',(125.930522084454,1.35615917984635,123.934202458341));
#272659=CARTESIAN_POINT('Ctrl Pts',(125.652074460641,-5.04702146960864,
125.949897193134));
#272660=CARTESIAN_POINT('Ctrl Pts',(125.373626836828,-6.81223594919939,
132.426606661257));
#272661=CARTESIAN_POINT('Ctrl Pts',(125.095179213015,-2.3173383877032,137.412551266352));
#272662=CARTESIAN_POINT('Ctrl Pts',(124.816731589202,4.3070799438184,136.325891493273));
#272663=CARTESIAN_POINT('Ctrl Pts',(124.538283965389,6.97350221952356,130.165214587198));
#272664=CARTESIAN_POINT('Ctrl Pts',(124.259836341577,3.2316166300094,124.591881659011));
#272665=CARTESIAN_POINT('Ctrl Pts',(123.981388717764,-3.47996676923432,
124.727513397266));
#272666=CARTESIAN_POINT('Ctrl Pts',(123.702941093951,-6.99363071337966,
130.447470860486));
#272667=CARTESIAN_POINT('Ctrl Pts',(123.424493470138,-4.08048968978323,
136.495392575427));
#272668=CARTESIAN_POINT('Ctrl Pts',(123.146045846325,2.58242201572056,137.313533943462));
#272669=CARTESIAN_POINT('Ctrl Pts',(122.867598222512,6.87221404710605,132.150063015792));
#272670=CARTESIAN_POINT('Ctrl Pts',(122.589150598699,4.84677709552158,125.749957325369));
#272671=CARTESIAN_POINT('Ctrl Pts',(122.310702974886,-1.63261122862275,
123.994601339147));
#272672=CARTESIAN_POINT('Ctrl Pts',(122.032255351073,-6.6117095911554,128.497081454556));
#272673=CARTESIAN_POINT('Ctrl Pts',(121.753807727261,-5.51496983938628,
135.119838403918));
#272674=CARTESIAN_POINT('Ctrl Pts',(121.475360103447,0.649757773524084,
137.776882090432));
#272675=CARTESIAN_POINT('Ctrl Pts',(121.196912479635,6.21738973499768,134.026519169992));
#272676=CARTESIAN_POINT('Ctrl Pts',(120.918464855822,6.07154426638285,127.315149951069));
#272677=CARTESIAN_POINT('Ctrl Pts',(120.640017232009,0.346246228389124,
123.810194877238));
#272678=CARTESIAN_POINT('Ctrl Pts',(120.361569608196,-5.69723517842559,
126.732536434776));
#272679=CARTESIAN_POINT('Ctrl Pts',(120.083121984383,-6.50523578167861,
133.396685496627));
#272680=CARTESIAN_POINT('Ctrl Pts',(119.80467436057,-1.3352425000044,137.678614636731));
#272681=CARTESIAN_POINT('Ctrl Pts',(119.526226736757,5.06177340895125,135.6434401592));
#272682=CARTESIAN_POINT('Ctrl Pts',(119.247779112945,6.8072668364591,129.161387985085));
#272683=CARTESIAN_POINT('Ctrl Pts',(118.969331489131,2.29721459473369,124.189147396544));
#272684=CARTESIAN_POINT('Ctrl Pts',(118.690883865319,-4.32386563438011,
125.29596458699));
#272685=CARTESIAN_POINT('Ctrl Pts',(118.412436241506,-6.97152457807781,
131.464728629428));
#272686=CARTESIAN_POINT('Ctrl Pts',(118.133988617693,-3.21269301243169,
137.026646729736));
#272687=CARTESIAN_POINT('Ctrl Pts',(117.85554099388,3.49844648286018,136.870587868534));
#272688=CARTESIAN_POINT('Ctrl Pts',(117.577093370067,6.99468456901571,131.139962515369));
#272689=CARTESIAN_POINT('Ctrl Pts',(117.298645746254,4.06314924558364,125.100935413187));
#272690=CARTESIAN_POINT('Ctrl Pts',(117.020198122441,-2.60222173866402,
124.303077446017));
#272691=CARTESIAN_POINT('Ctrl Pts',(116.741750498628,-6.8762780706787,129.479581108162));
#272692=CARTESIAN_POINT('Ctrl Pts',(116.463302874816,-4.83137078059878,
135.873492420371));
#272693=CARTESIAN_POINT('Ctrl Pts',(116.184855251003,1.65333023126747,137.609119246659));
#272694=CARTESIAN_POINT('Ctrl Pts',(115.90640762719,6.61870153027093,133.09150532375));
#272695=CARTESIAN_POINT('Ctrl Pts',(115.627960003377,5.5018094645007,126.472117149089));
#272696=CARTESIAN_POINT('Ctrl Pts',(115.349512379564,-0.670976720811003,
123.833849080098));
#272697=CARTESIAN_POINT('Ctrl Pts',(115.071064755751,-6.22716807873245,
127.601140585621));
#272698=CARTESIAN_POINT('Ctrl Pts',(114.792617131938,-6.06089618637186,
134.312034814502));
#272699=CARTESIAN_POINT('Ctrl Pts',(114.514169508125,-0.324956789974863,
137.79954781581));
#272700=CARTESIAN_POINT('Ctrl Pts',(114.235721884312,5.70960202138734,134.858825515823));
#272701=CARTESIAN_POINT('Ctrl Pts',(113.957274260499,6.4973155046598,128.192248045959));
#272702=CARTESIAN_POINT('Ctrl Pts',(113.678826636687,1.31431345065849,123.926074420608));
#272703=CARTESIAN_POINT('Ctrl Pts',(113.400379012874,-5.07647845671644,
125.980709787299));
#272704=CARTESIAN_POINT('Ctrl Pts',(113.121931389061,-6.80223466212876,
132.468044618562));
#272705=CARTESIAN_POINT('Ctrl Pts',(112.843483765248,-2.27706952068197,
137.42653512839));
#272706=CARTESIAN_POINT('Ctrl Pts',(112.565036141435,4.34061126924124,136.299570773982));
#272707=CARTESIAN_POINT('Ctrl Pts',(112.286588517622,6.96948235338073,130.122776741767));
#272708=CARTESIAN_POINT('Ctrl Pts',(112.008140893809,3.1937396329048,124.572324994188));
#272709=CARTESIAN_POINT('Ctrl Pts',(111.729693269996,-3.51689378735575,
124.748809532627));
#272710=CARTESIAN_POINT('Ctrl Pts',(111.451245646184,-6.99567362684944,
130.490049688009));
#272711=CARTESIAN_POINT('Ctrl Pts',(111.172798022371,-4.0457711609245,136.52012623271));
#272712=CARTESIAN_POINT('Ctrl Pts',(110.894350398558,2.62199735498092,137.297693407768));
#272713=CARTESIAN_POINT('Ctrl Pts',(110.615902774745,6.88027839335069,132.108204965571));
#272714=CARTESIAN_POINT('Ctrl Pts',(110.337455150932,4.81591970851693,125.720547263895));
#272715=CARTESIAN_POINT('Ctrl Pts',(110.059007527119,-1.67403391768677,
124.004665676154));
#272716=CARTESIAN_POINT('Ctrl Pts',(109.780559903306,-6.62563215463966,
128.537371556004));
#272717=CARTESIAN_POINT('Ctrl Pts',(109.502112279493,-5.48859812160383,
135.153329634858));
#272718=CARTESIAN_POINT('Ctrl Pts',(109.22366465568,0.692189452261082,137.772797645767));
#272719=CARTESIAN_POINT('Ctrl Pts',(108.945217031867,6.23688873483282,133.988612454835));
#272720=CARTESIAN_POINT('Ctrl Pts',(108.666769408055,6.05019195904657,127.278255384801));
#272721=CARTESIAN_POINT('Ctrl Pts',(108.388321784241,0.303664341205276,
123.808216763862));
#272722=CARTESIAN_POINT('Ctrl Pts',(108.109874160429,-5.72191597137591,
126.767292563848));
#272723=CARTESIAN_POINT('Ctrl Pts',(107.831426536616,-6.48933503739778,
133.436236683461));
#272724=CARTESIAN_POINT('Ctrl Pts',(107.552978912803,-1.29337222569216,
137.68661527281));
#272725=CARTESIAN_POINT('Ctrl Pts',(107.27453128899,5.09113647667873,135.612538050821));
#272726=CARTESIAN_POINT('Ctrl Pts',(106.996083665177,6.79713947282576,129.119980660195));
#272727=CARTESIAN_POINT('Ctrl Pts',(106.717636041364,2.25690335216928,124.175286163858));
#272728=CARTESIAN_POINT('Ctrl Pts',(106.439188417551,-4.35731669327239,
125.322387242187));
#272729=CARTESIAN_POINT('Ctrl Pts',(106.160740793739,-6.96737556435125,
131.5071540432));
#272730=CARTESIAN_POINT('Ctrl Pts',(105.882293169926,-3.17475666701035,
137.046088019424));
#272731=CARTESIAN_POINT('Ctrl Pts',(105.603845546113,3.53530851182771,136.849179438675));
#272732=CARTESIAN_POINT('Ctrl Pts',(105.3253979223,6.99659787771835,131.097377667143));
#272733=CARTESIAN_POINT('Ctrl Pts',(105.046950298487,4.02835559679407,125.076307541727));
#272734=CARTESIAN_POINT('Ctrl Pts',(104.768502674674,-2.64174868147234,
124.319038362058));
#272735=CARTESIAN_POINT('Ctrl Pts',(104.490055050861,-6.88421497806359,
129.521463509594));
#272736=CARTESIAN_POINT('Ctrl Pts',(104.211607427049,-4.80042402241278,
135.902808426348));
#272737=CARTESIAN_POINT('Ctrl Pts',(103.933159803235,1.69472209608453,137.598928879852));
#272738=CARTESIAN_POINT('Ctrl Pts',(103.654712179423,6.63250140005722,133.051173033428));
#272739=CARTESIAN_POINT('Ctrl Pts',(103.37626455561,5.47533593308374,126.438706339714));
#272740=CARTESIAN_POINT('Ctrl Pts',(103.097816931797,-0.713395771362793,
123.838062653278));
#272741=CARTESIAN_POINT('Ctrl Pts',(102.819369307984,-6.24655161324796,
127.639106473447));
#272742=CARTESIAN_POINT('Ctrl Pts',(102.540921684171,-6.03943168356949,
134.348864220799));
#272743=CARTESIAN_POINT('Ctrl Pts',(102.262474060358,-0.282369079330704,
137.801396315408));
#272744=CARTESIAN_POINT('Ctrl Pts',(101.984026436545,5.73417691431645,134.823994427897));
#272745=CARTESIAN_POINT('Ctrl Pts',(101.705578812732,6.48129445382252,128.15274543872));
#272746=CARTESIAN_POINT('Ctrl Pts',(101.427131188919,1.27241901910234,123.9182012603));
#272747=CARTESIAN_POINT('Ctrl Pts',(101.148683565106,-5.1057473330482,126.01170112362));
#272748=CARTESIAN_POINT('Ctrl Pts',(100.870235941294,-6.7919813157512,132.509420927444));
#272749=CARTESIAN_POINT('Ctrl Pts',(100.591788317481,-2.23671627601227,
137.440273603317));
#272750=CARTESIAN_POINT('Ctrl Pts',(100.313340693668,4.37398175171709,136.273046427655));
#272751=CARTESIAN_POINT('Ctrl Pts',(100.034893069855,6.96520423050629,130.080364152676));
#272752=CARTESIAN_POINT('Ctrl Pts',(99.7564454460421,3.15574429060373,124.552999259737));
#272753=CARTESIAN_POINT('Ctrl Pts',(99.4779978222292,-3.55369048568456,
124.770330058661));
#272754=CARTESIAN_POINT('Ctrl Pts',(99.1995501984162,-6.99745731306031,
130.532640162439));
#272755=CARTESIAN_POINT('Ctrl Pts',(98.9211025746034,-4.01090271452764,
136.544648090195));
#272756=CARTESIAN_POINT('Ctrl Pts',(98.6426549507905,2.66147553516503,137.281612259238));
#272757=CARTESIAN_POINT('Ctrl Pts',(98.3642073269776,6.88808778834931,132.066298600918));
#272758=CARTESIAN_POINT('Ctrl Pts',(98.0857597031646,4.78488386583629,125.691325584995));
#272759=CARTESIAN_POINT('Ctrl Pts',(97.8073120793519,-1.71539457480834,
124.014981978356));
#272760=CARTESIAN_POINT('Ctrl Pts',(97.5288644555388,-6.63930920288774,
128.577745661565));
#272761=CARTESIAN_POINT('Ctrl Pts',(97.2504168317261,-5.46202302179963,
135.186659713151));
#272762=CARTESIAN_POINT('Ctrl Pts',(96.9719692079131,0.734595481663425,
137.768454983106));
#272763=CARTESIAN_POINT('Ctrl Pts',(96.6935215841003,6.25615662446226,133.950587746053));
#272764=CARTESIAN_POINT('Ctrl Pts',(96.4150739602873,6.0286154596223,127.24149147966));
#272765=CARTESIAN_POINT('Ctrl Pts',(96.1366263364746,0.26107120162757,123.806497895168));
#272766=CARTESIAN_POINT('Ctrl Pts',(95.8581787126614,-5.74638473662552,
126.80219828796));
#272767=CARTESIAN_POINT('Ctrl Pts',(95.5797310888487,-6.47319382842077,
133.47569034516));
#272768=CARTESIAN_POINT('Ctrl Pts',(95.3012834650358,-1.25145402499642,
137.694360884412));
#272769=CARTESIAN_POINT('Ctrl Pts',(95.0228358412229,5.12031089047184,135.581457773658));
#272770=CARTESIAN_POINT('Ctrl Pts',(94.7443882174101,6.78676023868958,129.078635750625));
#272771=CARTESIAN_POINT('Ctrl Pts',(94.465940593597,2.21650847922131,124.161670573963));
#272772=CARTESIAN_POINT('Ctrl Pts',(94.1874929697842,-4.39060629019222,
125.349013033923));
#272773=CARTESIAN_POINT('Ctrl Pts',(93.9090453459715,-6.96296837196094,
131.549553414704));
#272774=CARTESIAN_POINT('Ctrl Pts',(93.6305977221583,-3.13670267981308,
137.065298019608));
#272775=CARTESIAN_POINT('Ctrl Pts',(93.3521500983456,3.5720395386382,136.82754701583));
#272776=CARTESIAN_POINT('Ctrl Pts',(93.0737024745325,6.99825192491364,131.054781961061));
#272777=CARTESIAN_POINT('Ctrl Pts',(92.7952548507199,3.99341267580637,125.051891925383));
#272778=CARTESIAN_POINT('Ctrl Pts',(92.5168072269068,-2.68117773331193,
124.335239594101));
#272779=CARTESIAN_POINT('Ctrl Pts',(92.238359603094,-6.89189678833074,129.563393449252));
#272780=CARTESIAN_POINT('Ctrl Pts',(91.959911979281,-4.7692993827493,135.931935507467));
#272781=CARTESIAN_POINT('Ctrl Pts',(91.6814643554683,1.73605116235111,137.588486737821));
#272782=CARTESIAN_POINT('Ctrl Pts',(91.4030167316553,6.6460555000649,133.010757486647));
#272783=CARTESIAN_POINT('Ctrl Pts',(91.1245691078424,5.44865951108031,126.405457301267));
#272784=CARTESIAN_POINT('Ctrl Pts',(90.8461214840295,-0.755788386771977,
123.84253436519));
#272785=CARTESIAN_POINT('Ctrl Pts',(90.5676738602166,-6.26570367949625,
127.677189650927));
#272786=CARTESIAN_POINT('Ctrl Pts',(90.2892262364038,-6.01774338740505,
134.38556228421));
#272787=CARTESIAN_POINT('Ctrl Pts',(90.0107786125907,-0.239770905396614,
137.802985537273));
#272788=CARTESIAN_POINT('Ctrl Pts',(89.7323309887781,5.75853932521132,134.78901439096));
#272789=CARTESIAN_POINT('Ctrl Pts',(89.453883364965,6.46503323623579,128.113341088056));
#272790=CARTESIAN_POINT('Ctrl Pts',(89.1754357411521,1.23047743759138,123.910583269158));
#272791=CARTESIAN_POINT('Ctrl Pts',(88.8969881173393,-5.13482701403487,
126.042870053701));
#272792=CARTESIAN_POINT('Ctrl Pts',(88.6185404935264,-6.78147629000823,
132.550734054689));
#272793=CARTESIAN_POINT('Ctrl Pts',(88.3400928697134,-2.19628014899849,
137.453766182047));
#272794=CARTESIAN_POINT('Ctrl Pts',(88.0616452459006,4.4071901546906,136.246319437167));
#272795=CARTESIAN_POINT('Ctrl Pts',(87.7831976220877,6.96066800942769,130.037978391542));
#272796=CARTESIAN_POINT('Ctrl Pts',(87.5047499982748,3.1176320110373,124.533905171779));
#272797=CARTESIAN_POINT('Ctrl Pts',(87.2263023744621,-3.59035550070555,
124.792074177916));
#272798=CARTESIAN_POINT('Ctrl Pts',(86.9478547506488,-6.99898170591706,
130.57524070557));
#272799=CARTESIAN_POINT('Ctrl Pts',(86.6694071268362,-3.97588564265574,
136.568957239218));
#272800=CARTESIAN_POINT('Ctrl Pts',(86.3909595030232,2.70085509339449,137.265291093768));
#272801=CARTESIAN_POINT('Ctrl Pts',(86.1125118792103,6.89564194272181,132.024345474689));
#272802=CARTESIAN_POINT('Ctrl Pts',(85.8340642553976,4.75367071752436,125.662293371487));
#272803=CARTESIAN_POINT('Ctrl Pts',(85.5556166315845,-1.75669166735309,
124.025549863481));
#272804=CARTESIAN_POINT('Ctrl Pts',(85.2771690077717,-6.65274022909182,
128.618202275162));
#272805=CARTESIAN_POINT('Ctrl Pts',(84.9987213839588,-5.4352455247236,135.21982740374));
#272806=CARTESIAN_POINT('Ctrl Pts',(84.7202737601459,0.776974290360158,
137.763854263368));
#272807=CARTESIAN_POINT('Ctrl Pts',(84.4418261363329,6.27519268990729,133.912446452669));
#272808=CARTESIAN_POINT('Ctrl Pts',(84.1633785125202,6.00681556763514,127.204859597945));
#272809=CARTESIAN_POINT('Ctrl Pts',(83.8849308887072,0.218468387960617,
123.805038334852));
#272810=CARTESIAN_POINT('Ctrl Pts',(83.6064832648944,-5.77064056747553,
126.837252313669));
#272811=CARTESIAN_POINT('Ctrl Pts',(83.3280356410814,-6.45681275286598,
133.515045019753));
#272812=CARTESIAN_POINT('Ctrl Pts',(83.0495880172686,-1.20948945121144,
137.701851184522));
#272813=CARTESIAN_POINT('Ctrl Pts',(82.7711403934555,5.14929556926191,135.550200479404));
#272814=CARTESIAN_POINT('Ctrl Pts',(82.4926927696429,6.77612951865689,129.037354788424));
#272815=CARTESIAN_POINT('Ctrl Pts',(82.2142451458298,2.17603147273656,124.148301131391));
#272816=CARTESIAN_POINT('Ctrl Pts',(81.9357975220171,-4.42373319158141,
125.375840975569));
#272817=CARTESIAN_POINT('Ctrl Pts',(81.6573498982041,-6.95830316421689,
131.591925172815));
#272818=CARTESIAN_POINT('Ctrl Pts',(81.3789022743912,-3.09853246094448,
137.084276018453));
#272819=CARTESIAN_POINT('Ctrl Pts',(81.1004546505783,3.60863820220999,136.805691401599));
#272820=CARTESIAN_POINT('Ctrl Pts',(80.8220070267654,6.99964664931016,131.012176975526));
#272821=CARTESIAN_POINT('Ctrl Pts',(80.5435594029525,3.95832177744353,125.02768946888));
#272822=CARTESIAN_POINT('Ctrl Pts',(80.2651117791397,-2.72050743312451,
124.351680541802));
#272823=CARTESIAN_POINT('Ctrl Pts',(79.9866641553267,-6.89932321682792,
129.605369373404));
#272824=CARTESIAN_POINT('Ctrl Pts',(79.7082165315139,-4.73799801494326,
135.960872584412));
#272825=CARTESIAN_POINT('Ctrl Pts',(79.4297689077009,1.77731589860328,137.577793207502));
#272826=CARTESIAN_POINT('Ctrl Pts',(79.1513212838881,6.65936332804202,132.970260181018));
#272827=CARTESIAN_POINT('Ctrl Pts',(78.8728736600752,5.42178118699497,126.372371265798));
#272828=CARTESIAN_POINT('Ctrl Pts',(78.5944260362623,-0.798152996164653,
123.847264050135));
#272829=CARTESIAN_POINT('Ctrl Pts',(78.3159784124494,-6.28462356779051,
127.715388706879));
#272830=CARTESIAN_POINT('Ctrl Pts',(78.0375307886365,-5.99583210154638,
134.422127644877));
#272831=CARTESIAN_POINT('Ctrl Pts',(77.7590831648237,-0.197163846663491,
137.804315422519));
#272832=CARTESIAN_POINT('Ctrl Pts',(77.4806355410107,5.78268835131386,134.753886701214));
#272833=CARTESIAN_POINT('Ctrl Pts',(77.2021879171979,6.44853245446487,128.07403645411));
#272834=CARTESIAN_POINT('Ctrl Pts',(76.9237402933849,1.18849026028645,123.903220729472));
#272835=CARTESIAN_POINT('Ctrl Pts',(76.6452926695721,-5.16371642211823,
126.074215422566));
#272836=CARTESIAN_POINT('Ctrl Pts',(76.3668450457591,-6.77071997416741,
132.591982469425));
#272837=CARTESIAN_POINT('Ctrl Pts',(76.0883974219463,-2.15576263801617,
137.467012364608));
#272838=CARTESIAN_POINT('Ctrl Pts',(75.8099497981334,4.44023524761227,136.219390792892));
#272839=CARTESIAN_POINT('Ctrl Pts',(75.5315021743204,6.95587385823614,129.995621028982));
#272840=CARTESIAN_POINT('Ctrl Pts',(75.2530545505077,3.0794042064702,124.515043437855));
#272841=CARTESIAN_POINT('Ctrl Pts',(74.9746069266946,-3.62688747378295,
124.814041084656));
#272842=CARTESIAN_POINT('Ctrl Pts',(74.6961593028819,-7.0002467489329,130.617849738824));
#272843=CARTESIAN_POINT('Ctrl Pts',(74.4177116790688,-3.94072124287924,
136.593052778991));
#272844=CARTESIAN_POINT('Ctrl Pts',(74.1392640552561,2.74013457044532,137.248730516143));
#272845=CARTESIAN_POINT('Ctrl Pts',(73.860816431443,6.90294057654623,131.982347141473));
#272846=CARTESIAN_POINT('Ctrl Pts',(73.5823688076304,4.72228142019582,125.633451699173));
#272847=CARTESIAN_POINT('Ctrl Pts',(73.3039211838172,-1.79792366504193,
124.036368939932));
#272848=CARTESIAN_POINT('Ctrl Pts',(73.0254735600045,-6.66592473556012,
128.658739897661));
#272849=CARTESIAN_POINT('Ctrl Pts',(72.7470259361915,-5.40826662262595,
135.252831477583));
#272850=CARTESIAN_POINT('Ctrl Pts',(72.4685783123786,0.819324307988826,
137.758995657032));
#272851=CARTESIAN_POINT('Ctrl Pts',(72.1901306885658,6.2939962257795,133.87418998802));
#272852=CARTESIAN_POINT('Ctrl Pts',(71.9116830647529,5.98479309088811,127.168361097063));
#272853=CARTESIAN_POINT('Ctrl Pts',(71.63323544094,0.17585747886725,123.803838136996));
#272854=CARTESIAN_POINT('Ctrl Pts',(71.3547878171271,-5.79468256511725,
126.872453342036));
#272855=CARTESIAN_POINT('Ctrl Pts',(71.0763401933142,-6.44019241774003,
133.554299248939));
#272856=CARTESIAN_POINT('Ctrl Pts',(70.7978925695013,-1.16748005934989,
137.709085895581));
#272857=CARTESIAN_POINT('Ctrl Pts',(70.5194449456884,5.17808943901089,135.518767326308));
#272858=CARTESIAN_POINT('Ctrl Pts',(70.2409973218756,6.76524770665308,128.996139303274));
#272859=CARTESIAN_POINT('Ctrl Pts',(69.9625496980626,2.1354738326052,124.135178331551));
#272860=CARTESIAN_POINT('Ctrl Pts',(69.6841020742497,-4.45669616991057,
125.402870073008));
#272861=CARTESIAN_POINT('Ctrl Pts',(69.4056544504369,-6.95338011399016,
131.634267747431));
#272862=CARTESIAN_POINT('Ctrl Pts',(69.1272068266238,-3.06024742481583,
137.103021312725));
#272863=CARTESIAN_POINT('Ctrl Pts',(68.8487592028112,3.64510314636624,136.783613405848));
#272864=CARTESIAN_POINT('Ctrl Pts',(68.5703115789981,7.00078199922599,130.969564289278));
#272865=CARTESIAN_POINT('Ctrl Pts',(68.2918639551854,3.92308420201135,125.003701069051));
#272866=CARTESIAN_POINT('Ctrl Pts',(68.0134163313723,-2.75973632353393,
124.368360595937));
#272867=CARTESIAN_POINT('Ctrl Pts',(67.7349687075595,-6.90649398836592,
129.647389726619));
#272868=CARTESIAN_POINT('Ctrl Pts',(67.4565210837467,-4.70652107887851,
135.98961858491));
#272869=CARTESIAN_POINT('Ctrl Pts',(67.1780734599337,1.81851477576126,137.566848685147));
#272870=CARTESIAN_POINT('Ctrl Pts',(66.8996258361208,6.67242439086218,132.929682617185));
#272871=CARTESIAN_POINT('Ctrl Pts',(66.6211782123079,5.39470195681365,126.339449459324));
#272872=CARTESIAN_POINT('Ctrl Pts',(66.3427305884951,-0.840488029704522,
123.852251532852));
#272873=CARTESIAN_POINT('Ctrl Pts',(66.0642829646821,-6.30331057704718,
127.753702225821));
#272874=CARTESIAN_POINT('Ctrl Pts',(65.7858353408693,-5.97369863792435,
134.458558947856));
#272875=CARTESIAN_POINT('Ctrl Pts',(65.5073877170563,-0.154549481951222,
137.805385921867));
#272876=CARTESIAN_POINT('Ctrl Pts',(65.2289400932435,5.80662309777304,134.718612660325));
#272877=CARTESIAN_POINT('Ctrl Pts',(64.9504924694306,6.43179271995227,128.03483299333));
#272878=CARTESIAN_POINT('Ctrl Pts',(64.6720448456177,1.14645904303803,123.896113914062));
#272879=CARTESIAN_POINT('Ctrl Pts',(64.3935972218049,-5.19241448679041,
126.1057360687));
#272880=CARTESIAN_POINT('Ctrl Pts',(64.1151495979918,-6.75971276680813,
132.633164643176));
#272881=CARTESIAN_POINT('Ctrl Pts',(63.8367019741791,-2.11516524445634,
137.480011660159));
#272882=CARTESIAN_POINT('Ctrl Pts',(63.5582543503661,4.47311580598391,136.192261492683));
#272883=CARTESIAN_POINT('Ctrl Pts',(63.2798067265533,6.95082195458075,129.953293634565));
#272884=CARTESIAN_POINT('Ctrl Pts',(63.0013591027403,3.041062293448,124.496414756892));
#272885=CARTESIAN_POINT('Ctrl Pts',(62.7229114789275,-3.66328505121137,
124.836229964889));
#272886=CARTESIAN_POINT('Ctrl Pts',(62.4444638551145,-7.00125239523119,
130.660465683307));
#272887=CARTESIAN_POINT('Ctrl Pts',(62.1660162313017,-3.90541081822766,
136.616933816649));
#272888=CARTESIAN_POINT('Ctrl Pts',(61.8875686074887,2.77931251080179,137.231931140021));
#272889=CARTESIAN_POINT('Ctrl Pts',(61.609120983676,6.909983419369,131.940305157533));
#272890=CARTESIAN_POINT('Ctrl Pts',(61.3306733598629,4.69071713699276,125.604801636791));
#272891=CARTESIAN_POINT('Ctrl Pts',(61.0522257360502,-1.83908904000824,
124.047438806804));
#272892=CARTESIAN_POINT('Ctrl Pts',(60.7737781122372,-6.67886223373588,
128.699357026925));
#272893=CARTESIAN_POINT('Ctrl Pts',(60.4953304884244,-5.38108731521968,
135.285670711703));
#272894=CARTESIAN_POINT('Ctrl Pts',(60.2168828646114,0.861643965253713,
137.753879344138));
#272895=CARTESIAN_POINT('Ctrl Pts',(59.9384352407986,6.31256653530686,133.835819769716));
#272896=CARTESIAN_POINT('Ctrl Pts',(59.6599876169856,5.96254884543232,127.131997329482));
#272897=CARTESIAN_POINT('Ctrl Pts',(59.3815399931728,0.133240053310041,
123.802897346075));
#272898=CARTESIAN_POINT('Ctrl Pts',(59.1030923693598,-5.81850983866561,
126.907800068673));
#272899=CARTESIAN_POINT('Ctrl Pts',(58.824644745547,-6.42333343891552,133.593451578138));
#272900=CARTESIAN_POINT('Ctrl Pts',(58.5461971217341,-1.12542740608588,
137.716064749505));
#272901=CARTESIAN_POINT('Ctrl Pts',(58.2677494979212,5.20669143275151,135.487159479138));
#272902=CARTESIAN_POINT('Ctrl Pts',(57.9893018741083,6.75411520590753,128.954990822428));
#272903=CARTESIAN_POINT('Ctrl Pts',(57.7108542502954,2.09483706170563,124.122302660713));
#272904=CARTESIAN_POINT('Ctrl Pts',(57.4324066264825,-4.48949400372376,
125.430099324666));
#272905=CARTESIAN_POINT('Ctrl Pts',(57.1539590026696,-6.94819940370625,
131.676579569534));
#272906=CARTESIAN_POINT('Ctrl Pts',(56.8755113788568,-3.02184899009409,
137.121533207807));
#272907=CARTESIAN_POINT('Ctrl Pts',(56.5970637550437,3.68143301988451,136.761313846687));
#272908=CARTESIAN_POINT('Ctrl Pts',(56.318616131231,7.00165793259049,130.926945481348));
#272909=CARTESIAN_POINT('Ctrl Pts',(56.040168507418,3.88770125525153,124.979927614796));
#272910=CARTESIAN_POINT('Ctrl Pts',(55.7617208836052,-2.79886295089852,
124.385279138419));
#272911=CARTESIAN_POINT('Ctrl Pts',(55.4832732597923,-6.91340883722955,
129.689452951814));
#272912=CARTESIAN_POINT('Ctrl Pts',(55.2048256359794,-4.67486974094423,
136.018172443767));
#272913=CARTESIAN_POINT('Ctrl Pts',(54.9263780121665,1.85964626718557,137.555653576309));
#272914=CARTESIAN_POINT('Ctrl Pts',(54.6479303883536,6.68523820454244,132.889026298762));
#272915=CARTESIAN_POINT('Ctrl Pts',(54.3694827645407,5.36742282396772,126.306693101776));
#272916=CARTESIAN_POINT('Ctrl Pts',(54.0910351407278,-0.882791918651148,
123.857496628527));
#272917=CARTESIAN_POINT('Ctrl Pts',(53.8125875169149,-6.32176401481248,
127.792128788032));
#272918=CARTESIAN_POINT('Ctrl Pts',(53.534139893102,-5.95134381670231,134.494854843172));
#272919=CARTESIAN_POINT('Ctrl Pts',(53.2556922692892,-0.111929390351441,
137.806196995646));
#272920=CARTESIAN_POINT('Ctrl Pts',(52.9772446454762,5.83034267767769,134.683193575387));
#272921=CARTESIAN_POINT('Ctrl Pts',(52.6987970216634,6.41481465299549,127.995732158415));
#272922=CARTESIAN_POINT('Ctrl Pts',(52.4203493978505,1.10438534332797,123.889263086274));
#272923=CARTESIAN_POINT('Ctrl Pts',(52.1419017740376,-5.22092014463445,
126.137430824095));
#272924=CARTESIAN_POINT('Ctrl Pts',(51.8634541502246,-6.74845507580631,
132.674279049921));
#272925=CARTESIAN_POINT('Ctrl Pts',(51.5850065264118,-2.07448947267055,
137.492763587005));
#272926=CARTESIAN_POINT('Ctrl Pts',(51.3065589025989,4.50583061140446,136.164932541826));
#272927=CARTESIAN_POINT('Ctrl Pts',(51.028111278786,6.94551248566166,129.910997776748));
#272928=CARTESIAN_POINT('Ctrl Pts',(50.7496636549731,3.00260769274395,124.478019819181));
#272929=CARTESIAN_POINT('Ctrl Pts',(50.4712160311602,-3.69954688426507,
124.858639996399));
#272930=CARTESIAN_POINT('Ctrl Pts',(50.1927684073473,-7.00199860754717,
130.70308695987));
#272931=CARTESIAN_POINT('Ctrl Pts',(49.9143207835345,-3.86995567714208,
136.640599467269));
#272932=CARTESIAN_POINT('Ctrl Pts',(49.6358731597215,2.81838746271124,137.214893587909));
#272933=CARTESIAN_POINT('Ctrl Pts',(49.3574255359087,6.91677021021505,131.89822108075));
#272934=CARTESIAN_POINT('Ctrl Pts',(49.0789779120958,4.65897903754105,125.576344245977));
#272935=CARTESIAN_POINT('Ctrl Pts',(48.8005302882828,-1.88018626685394,
124.058759053897));
#272936=CARTESIAN_POINT('Ctrl Pts',(48.5220826644701,-6.69155224421552,
128.740052157871));
#272937=CARTESIAN_POINT('Ctrl Pts',(48.243635040657,-5.35370860964396,135.318343889229));
#272938=CARTESIAN_POINT('Ctrl Pts',(47.9651874168443,0.903931693984841,
137.748505514272));
#272939=CARTESIAN_POINT('Ctrl Pts',(47.6867397930313,6.33090293035988,133.797337219578));
#272940=CARTESIAN_POINT('Ctrl Pts',(47.4082921692184,5.94008365553619,127.095769642671));
#272941=CARTESIAN_POINT('Ctrl Pts',(47.1298445454056,0.0906176904940206,
123.80221599695));
#272942=CARTESIAN_POINT('Ctrl Pts',(46.8513969215926,-5.84212150519187,
126.943291183793));
#272943=CARTESIAN_POINT('Ctrl Pts',(46.5729492977799,-6.40623644110861,
133.632500556544));
#272944=CARTESIAN_POINT('Ctrl Pts',(46.2945016739667,-1.08333304969514,
137.722787487691));
#272945=CARTESIAN_POINT('Ctrl Pts',(46.016054050154,5.23510049062639,135.455378109134));
#272946=CARTESIAN_POINT('Ctrl Pts',(45.737606426341,6.7427324289391,128.913910870662));
#272947=CARTESIAN_POINT('Ctrl Pts',(45.4591588025282,2.0541226658487,124.10967459599));
#272948=CARTESIAN_POINT('Ctrl Pts',(45.1807111787153,-4.5221254776858,125.457527721552));
#272949=CARTESIAN_POINT('Ctrl Pts',(44.9022635549024,-6.94276122533821,
131.718859071242));
#272950=CARTESIAN_POINT('Ctrl Pts',(44.6238159310895,-2.98333857964632,
137.139811017737));
#272951=CARTESIAN_POINT('Ctrl Pts',(44.3453683072766,3.71762647654865,136.738793550433));
#272952=CARTESIAN_POINT('Ctrl Pts',(44.0669206834637,7.00227441694529,130.88432213099));
#272953=CARTESIAN_POINT('Ctrl Pts',(43.7884730596509,3.85217424829189,124.956369987047));
#272954=CARTESIAN_POINT('Ctrl Pts',(43.5100254358379,-2.8378858653675,124.402435542326));
#272955=CARTESIAN_POINT('Ctrl Pts',(43.2315778120251,-6.92006750718621,
129.731557490323));
#272956=CARTESIAN_POINT('Ctrl Pts',(42.9531301882121,-4.64304517399252,
136.04653310291));
#272957=CARTESIAN_POINT('Ctrl Pts',(42.6746825643993,1.90070884873357,137.544208295828));
#272958=CARTESIAN_POINT('Ctrl Pts',(42.3962349405864,6.69780429426274,132.848292732287));
#272959=CARTESIAN_POINT('Ctrl Pts',(42.1177873167735,5.33994479929498,126.274103406951));
#272960=CARTESIAN_POINT('Ctrl Pts',(41.8393396929606,-0.925063095418803,
123.862999142802));
#272961=CARTESIAN_POINT('Ctrl Pts',(41.5608920691476,-6.33998319728738,
127.8306669696));
#272962=CARTESIAN_POINT('Ctrl Pts',(41.2824444453348,-5.92876846624656,
134.531013985867));
#272963=CARTESIAN_POINT('Ctrl Pts',(41.0039968215219,-0.069305151166692,
137.806748613804));
#272964=CARTESIAN_POINT('Ctrl Pts',(40.725549197709,5.85384621209049,134.647630758868));
#272965=CARTESIAN_POINT('Ctrl Pts',(40.4471015738961,6.39759888272248,127.956735398261));
#272966=CARTESIAN_POINT('Ctrl Pts',(40.1686539500832,1.06227072021291,123.882668499967));
#272967=CARTESIAN_POINT('Ctrl Pts',(39.8902063262704,-5.24923233936253,
126.169298514289));
#272968=CARTESIAN_POINT('Ctrl Pts',(39.6117587024575,-6.73694731831984,
132.715324166149));
#272969=CARTESIAN_POINT('Ctrl Pts',(39.3333110786445,-2.03373682991476,
137.505267672621));
#272970=CARTESIAN_POINT('Ctrl Pts',(39.0548634548317,4.53837845161457,136.137404953004));
#272971=CARTESIAN_POINT('Ctrl Pts',(38.7764158310188,6.9399456482232,129.86873502282));
#272972=CARTESIAN_POINT('Ctrl Pts',(38.4979682072059,2.96404182930761,124.459859306355));
#272973=CARTESIAN_POINT('Ctrl Pts',(38.219520583393,-3.73567162924815,124.881270348773));
#272974=CARTESIAN_POINT('Ctrl Pts',(37.9410729595801,-7.00248535822977,
130.745711989165));
#272975=CARTESIAN_POINT('Ctrl Pts',(37.6626253357672,-3.83435713342598,
136.664048853912));
#272976=CARTESIAN_POINT('Ctrl Pts',(37.3841777119543,2.8573579782368,137.197618491141));
#272977=CARTESIAN_POINT('Ctrl Pts',(37.1057300881414,6.92330069759731,131.856096470565));
#272978=CARTESIAN_POINT('Ctrl Pts',(36.8272824643285,4.62706829790778,125.548080581235));
#272979=CARTESIAN_POINT('Ctrl Pts',(36.5488348405156,-1.92121382270608,
124.070329261737));
#272980=CARTESIAN_POINT('Ctrl Pts',(36.2703872167028,-6.70399429676593,
128.780823782526));
#272981=CARTESIAN_POINT('Ctrl Pts',(35.9919395928899,-5.32613152042688,
135.350849799446));
#272982=CARTESIAN_POINT('Ctrl Pts',(35.7134919690769,0.946185927194629,
137.742874366562));
#272983=CARTESIAN_POINT('Ctrl Pts',(35.4350443452641,6.34900473147662,133.758743763591));
#272984=CARTESIAN_POINT('Ctrl Pts',(35.1565967214512,5.91739835365575,127.059679379064));
#272985=CARTESIAN_POINT('Ctrl Pts',(34.8781490976383,0.0479919698059151,
123.80179411487));
#272986=CARTESIAN_POINT('Ctrl Pts',(34.5997014738253,-5.8655166897575,126.978925372262));
#272987=CARTESIAN_POINT('Ctrl Pts',(34.3212538500126,-6.38890205785425,
133.671444737187));
#272988=CARTESIAN_POINT('Ctrl Pts',(34.0428062261996,-1.04119854999986,
137.729253861025));
#272989=CARTESIAN_POINT('Ctrl Pts',(33.7643586023867,5.26331555992738,135.423424393967));
#272990=CARTESIAN_POINT('Ctrl Pts',(33.4859109785738,6.73109979754094,128.872900970206));
#272991=CARTESIAN_POINT('Ctrl Pts',(33.207463354761,2.01333215372067,124.097294605319));
#272992=CARTESIAN_POINT('Ctrl Pts',(32.9290157309481,-4.55458938262534,
125.485154247296));
#272993=CARTESIAN_POINT('Ctrl Pts',(32.6505681071352,-6.93706578039975,
131.761104685873));
#272994=CARTESIAN_POINT('Ctrl Pts',(32.3721204833222,-2.94471762049033,
137.157854065221));
#272995=CARTESIAN_POINT('Ctrl Pts',(32.0936728595094,3.75368217519627,136.716053351584));
#272996=CARTESIAN_POINT('Ctrl Pts',(31.8152252356965,7.00263142944649,130.84169581763));
#272997=CARTESIAN_POINT('Ctrl Pts',(31.5367776118836,3.8165044975991,124.933029058741));
#272998=CARTESIAN_POINT('Ctrl Pts',(31.2583299880707,-2.87680362093211,
124.41982917192));
#272999=CARTESIAN_POINT('Ctrl Pts',(30.9798823642578,-6.92646975149653,
129.773701781947));
#273000=CARTESIAN_POINT('Ctrl Pts',(30.7014347404449,-4.6110485572945,136.074699511423));
#273001=CARTESIAN_POINT('Ctrl Pts',(30.422987116632,1.94170099881587,137.532513267813));
#273002=CARTESIAN_POINT('Ctrl Pts',(30.1445394928192,6.71012219438185,132.807483427156));
#273003=CARTESIAN_POINT('Ctrl Pts',(29.8660918690062,5.31226890100394,126.241681582474));
#273004=CARTESIAN_POINT('Ctrl Pts',(29.5876442451933,-0.967299993633269,
123.868758871779));
#273005=CARTESIAN_POINT('Ctrl Pts',(29.3091966213805,-6.35796744935336,
127.869315342481));
#273006=CARTESIAN_POINT('Ctrl Pts',(29.0307489975676,-5.90597342309497,
134.567035036052));
#273007=CARTESIAN_POINT('Ctrl Pts',(28.7523013737546,-0.026678343854083,
137.807040755898));
#273008=CARTESIAN_POINT('Ctrl Pts',(28.4738537499418,5.87713283007914,134.611925528561));
#273009=CARTESIAN_POINT('Ctrl Pts',(28.1954061261289,6.38014604707014,127.917844157905));
#273010=CARTESIAN_POINT('Ctrl Pts',(27.916958502316,1.02011673426565,123.876330399509));
#273011=CARTESIAN_POINT('Ctrl Pts',(27.6385108785031,-5.27735002185588,
126.201337958415));
#273012=CARTESIAN_POINT('Ctrl Pts',(27.3600632546902,-6.72518992077305,
132.756298470923));
#273013=CARTESIAN_POINT('Ctrl Pts',(27.0816156308773,-1.99290882629253,
137.51752345366));
#273014=CARTESIAN_POINT('Ctrl Pts',(26.8031680070644,4.57075812054227,136.109679746264));
#273015=CARTESIAN_POINT('Ctrl Pts',(26.5247203832516,6.93412164854658,129.826506938842));
#273016=CARTESIAN_POINT('Ctrl Pts',(26.2462727594386,2.92536613221128,124.441933891359));
#273017=CARTESIAN_POINT('Ctrl Pts',(25.9678251356258,-3.7716579475455,124.904120183435));
#273018=CARTESIAN_POINT('Ctrl Pts',(25.6893775118128,-7.00271262924226,
130.788339191706));
#273019=CARTESIAN_POINT('Ctrl Pts',(25.410929888,-3.79861650619593,136.687281107654));
#273020=CARTESIAN_POINT('Ctrl Pts',(25.1324822641871,2.89622261331168,137.180106489852));
#273021=CARTESIAN_POINT('Ctrl Pts',(24.8540346403742,6.92957463952618,131.813932887921));
#273022=CARTESIAN_POINT('Ctrl Pts',(24.5755870165613,4.59498610055721,125.520011689881));
#273023=CARTESIAN_POINT('Ctrl Pts',(24.2971393927484,-1.96217018727317,
124.082149001586));
#273024=CARTESIAN_POINT('Ctrl Pts',(24.0186917689355,-6.71618793034234,
128.821670390082));
#273025=CARTESIAN_POINT('Ctrl Pts',(23.7402441451226,-5.29835706944761,
135.383187237832));
#273026=CARTESIAN_POINT('Ctrl Pts',(23.4617965213097,0.988405099136929,
137.736986109674));
#273027=CARTESIAN_POINT('Ctrl Pts',(23.1833488974968,6.36687126788796,133.720040831851));
#273028=CARTESIAN_POINT('Ctrl Pts',(22.9049012736839,5.89449378040337,127.023727875996));
#273029=CARTESIAN_POINT('Ctrl Pts',(22.6264536498711,0.00536447075796404,
123.801631715467));
#273030=CARTESIAN_POINT('Ctrl Pts',(22.3480060260581,-5.88869452544514,
127.01470131364));
#273031=CARTESIAN_POINT('Ctrl Pts',(22.0695584022453,-6.3713309314846,133.710282676972));
#273032=CARTESIAN_POINT('Ctrl Pts',(21.7911107784324,-0.999025468309402,
137.735463629893));
#273033=CARTESIAN_POINT('Ctrl Pts',(21.5126631546195,5.29133559513472,135.391299517692));
#273034=CARTESIAN_POINT('Ctrl Pts',(21.2342155308066,6.71921774276442,128.831962640697));
#273035=CARTESIAN_POINT('Ctrl Pts',(20.9557679069937,1.97246703682929,124.085163147446));
#273036=CARTESIAN_POINT('Ctrl Pts',(20.6773202831809,-4.58688451558038,
125.51297787819));
#273037=CARTESIAN_POINT('Ctrl Pts',(20.3988726593679,-6.93111327993769,
131.803314848003));
#273038=CARTESIAN_POINT('Ctrl Pts',(20.120425035555,-2.90598754374001,137.175661681671));
#273039=CARTESIAN_POINT('Ctrl Pts',(19.8419774117421,3.78959877977074,136.693094092787));
#273040=CARTESIAN_POINT('Ctrl Pts',(19.5635297879293,7.00272895686486,130.799068120799));
#273041=CARTESIAN_POINT('Ctrl Pts',(19.2850821641163,3.78069332492835,124.909905694786));
#273042=CARTESIAN_POINT('Ctrl Pts',(19.0066345403035,-2.91561477548059,
124.437459382677));
#273043=CARTESIAN_POINT('Ctrl Pts',(18.7281869164906,-6.932615332923,129.815884265012));
#273044=CARTESIAN_POINT('Ctrl Pts',(18.4497392926777,-4.57888107649638,
136.102670625591));
#273045=CARTESIAN_POINT('Ctrl Pts',(18.1712916688647,1.98262119845391,137.520568925627));
#273046=CARTESIAN_POINT('Ctrl Pts',(17.892844045052,6.72219144845534,132.766599895572));
#273047=CARTESIAN_POINT('Ctrl Pts',(17.614396421239,5.28439615463518,126.209428829746));
#273048=CARTESIAN_POINT('Ctrl Pts',(17.3359487974261,-1.00950104819076,
123.87477560203));
#273049=CARTESIAN_POINT('Ctrl Pts',(17.0575011736132,-6.37571610459714,
127.908072474542));
#273050=CARTESIAN_POINT('Ctrl Pts',(16.7790535498004,-5.88295953192644,
134.602916658952));
#273051=CARTESIAN_POINT('Ctrl Pts',(16.5006059259874,0.0159494520341194,
137.807073411106));
#273052=CARTESIAN_POINT('Ctrl Pts',(16.2221583021745,5.90020166874948,134.576079207535));
#273053=CARTESIAN_POINT('Ctrl Pts',(15.9437106783617,6.3624567927597,127.879059878479));
#273054=CARTESIAN_POINT('Ctrl Pts',(15.6652630545488,0.977924947517885,
123.870249019757));
#273055=CARTESIAN_POINT('Ctrl Pts',(15.3868154307359,-5.3052721502032,126.233547969238));
#273056=CARTESIAN_POINT('Ctrl Pts',(15.108367806923,-6.71318331884074,132.797200445919));
#273057=CARTESIAN_POINT('Ctrl Pts',(14.8299201831101,-1.95200697470083,
137.529530475982));
#273058=CARTESIAN_POINT('Ctrl Pts',(14.5514725592972,4.6029684183469,136.081757948972));
#273059=CARTESIAN_POINT('Ctrl Pts',(14.2730249354843,6.92804070244224,129.784315089592));
#273060=CARTESIAN_POINT('Ctrl Pts',(13.9945773116714,2.88658203459712,124.424244238425));
#273061=CARTESIAN_POINT('Ctrl Pts',(13.7161296878585,-3.80750450567058,
124.927188653676));
#273062=CARTESIAN_POINT('Ctrl Pts',(13.4376820640456,-7.00268041216303,
130.830966987928));
#273063=CARTESIAN_POINT('Ctrl Pts',(13.1592344402328,-3.7627351198343,136.710295367612));
#273064=CARTESIAN_POINT('Ctrl Pts',(12.8807868164199,2.93497992779253,137.162358232954));
#273065=CARTESIAN_POINT('Ctrl Pts',(12.602339192607,6.93559180351842,131.771731895206));
#273066=CARTESIAN_POINT('Ctrl Pts',(12.323891568794,4.56273363430679,125.49213861202));
#273067=CARTESIAN_POINT('Ctrl Pts',(12.0454439449812,-2.00305384290271,
124.094217835458));
#273068=CARTESIAN_POINT('Ctrl Pts',(11.7669963211683,-6.72813269310505,
128.862590466954));
#273069=CARTESIAN_POINT('Ctrl Pts',(11.4885486973554,-5.27038628589867,
135.415355006116));
#273070=CARTESIAN_POINT('Ctrl Pts',(11.2101010735425,1.03058764536478,137.730840961799));
#273071=CARTESIAN_POINT('Ctrl Pts',(10.9316534497296,6.38450187754329,133.681229858508));
#273072=CARTESIAN_POINT('Ctrl Pts',(10.6532058259167,5.87137078451608,126.987916465666));
#273073=CARTESIAN_POINT('Ctrl Pts',(10.3747582021038,-0.0372632270726686,
123.801728804758));
#273074=CARTESIAN_POINT('Ctrl Pts',(10.0963105782909,-5.91165415339157,
127.050617682238));
#273075=CARTESIAN_POINT('Ctrl Pts',(9.81786295447806,-6.35352371310424,
133.749012936746));
#273076=CARTESIAN_POINT('Ctrl Pts',(9.53941533066515,-0.956815367363035,
137.741416564191));
#273077=CARTESIAN_POINT('Ctrl Pts',(9.26096770685226,5.31915955795546,135.35900467071));
#273078=CARTESIAN_POINT('Ctrl Pts',(8.98252008303941,6.70708670490366,128.791097399121));
#273079=CARTESIAN_POINT('Ctrl Pts',(8.70407245922646,1.93152882944647,124.073280671906));
#273080=CARTESIAN_POINT('Ctrl Pts',(8.42562483541358,-4.61900967984285,
125.540997583217));
#273081=CARTESIAN_POINT('Ctrl Pts',(8.14717721160073,-6.92490394452403,
131.845487993513));
#273082=CARTESIAN_POINT('Ctrl Pts',(7.86872958778781,-2.86714978455288,
137.193233207215));
#273083=CARTESIAN_POINT('Ctrl Pts',(7.59028196397491,3.82537495936868,136.669916624805));
#273084=CARTESIAN_POINT('Ctrl Pts',(7.31183434016203,7.00256699558648,130.756440620084));
#273085=CARTESIAN_POINT('Ctrl Pts',(7.03338671634916,3.7447420572761,124.887000752025));
#273086=CARTESIAN_POINT('Ctrl Pts',(6.75493909253623,-2.95431789085107,
124.455325521299));
#273087=CARTESIAN_POINT('Ctrl Pts',(6.47649146872337,-6.9385040237388,129.858103376433));
#273088=CARTESIAN_POINT('Ctrl Pts',(6.19804384491048,-4.54654392357636,
136.130445408932));
#273089=CARTESIAN_POINT('Ctrl Pts',(5.91959622109758,2.02346793133434,137.508375711873));
#273090=CARTESIAN_POINT('Ctrl Pts',(5.64114859728465,6.73401160925262,132.725643652489));
#273091=CARTESIAN_POINT('Ctrl Pts',(5.36270097347181,5.25632759302358,126.177346343905));
#273092=CARTESIAN_POINT('Ctrl Pts',(5.08425334965889,-1.05166469531565,
123.881049110601));
#273093=CARTESIAN_POINT('Ctrl Pts',(4.80580572584599,-6.39322850533622,
127.946936929627));
#273094=CARTESIAN_POINT('Ctrl Pts',(4.5273581020331,-5.85972764552883,134.638657524961));
#273095=CARTESIAN_POINT('Ctrl Pts',(4.24891047822024,0.0585766569097649,
137.806846578216));
#273096=CARTESIAN_POINT('Ctrl Pts',(3.97046285440732,5.92305187327717,134.54009312409));
#273097=CARTESIAN_POINT('Ctrl Pts',(3.69201523059441,6.34453177527304,127.840383997147));
#273098=CARTESIAN_POINT('Ctrl Pts',(3.41356760678156,0.935696923401329,
123.864424586062));
#273099=CARTESIAN_POINT('Ctrl Pts',(3.13511998296867,-5.33299768974021,
126.265927353204));
#273100=CARTESIAN_POINT('Ctrl Pts',(2.85667235915575,-6.70092795743158,
132.838028575505));
#273101=CARTESIAN_POINT('Ctrl Pts',(2.57822473534285,-1.91103279077285,
137.541288294661));
#273102=CARTESIAN_POINT('Ctrl Pts',(2.29977711153,4.63500815146407,136.053640595781));
#273103=CARTESIAN_POINT('Ctrl Pts',(2.02132948771708,6.92170303524179,129.742161038504));
#273104=CARTESIAN_POINT('Ctrl Pts',(1.74288186390418,2.84769097362441,124.40679100305));
#273105=CARTESIAN_POINT('Ctrl Pts',(1.46443424009131,-3.84320997531586,
124.950474904685));
#273106=CARTESIAN_POINT('Ctrl Pts',(1.18598661627842,-7.00238870818588,
130.873593798241));
#273107=CARTESIAN_POINT('Ctrl Pts',(0.907538992465495,-3.72671430393905,
136.733090780986));
#273108=CARTESIAN_POINT('Ctrl Pts',(0.629091368652655,2.97362848551254,
137.144374378117));
#273109=CARTESIAN_POINT('Ctrl Pts',(0.350643744839755,6.94135196660579,
131.729495056193));
#273110=CARTESIAN_POINT('Ctrl Pts',(0.0721961210268491,4.53031209428387,
125.4644623805));
#273111=CARTESIAN_POINT('Ctrl Pts',(-0.206251502786054,-2.04386327463549,
124.106535316138));
#273112=CARTESIAN_POINT('Ctrl Pts',(-0.484699126598912,-6.73982814243653,
128.903582496833));
#273113=CARTESIAN_POINT('Ctrl Pts',(-0.763146750411823,-5.24222020624778,
135.447351912307));
#273114=CARTESIAN_POINT('Ctrl Pts',(-1.04159437422473,1.07273200278813,
137.724439150648));
#273115=CARTESIAN_POINT('Ctrl Pts',(-1.32004199803759,6.40189590713365,
133.642312281717));
#273116=CARTESIAN_POINT('Ctrl Pts',(-1.59848962185049,5.84803022282516,
126.952246475077));
#273117=CARTESIAN_POINT('Ctrl Pts',(-1.87693724566341,-0.0798895441007186,
123.802085379146));
#273118=CARTESIAN_POINT('Ctrl Pts',(-2.1553848694763,-5.93439472281934,
127.08667314716));
#273119=CARTESIAN_POINT('Ctrl Pts',(-2.43383249328916,-6.33548106256618,
133.787634081347));
#273120=CARTESIAN_POINT('Ctrl Pts',(-2.71228011710207,-0.914569811271147,
137.747112443329));
#273121=CARTESIAN_POINT('Ctrl Pts',(-2.99072774091498,5.34678641736288,
135.326541049718));
#273122=CARTESIAN_POINT('Ctrl Pts',(-3.26917536472784,6.6947071334783,128.750306759754));
#273123=CARTESIAN_POINT('Ctrl Pts',(-3.54762298854074,1.89051904855254,
124.061647619009));
#273124=CARTESIAN_POINT('Ctrl Pts',(-3.82607061235365,-4.65096368500298,
125.569212324096));
#273125=CARTESIAN_POINT('Ctrl Pts',(-4.10451823616654,-6.91843800424817,
131.887622559669));
#273126=CARTESIAN_POINT('Ctrl Pts',(-4.38296585997939,-2.82820578207579,
137.210567990736));
#273127=CARTESIAN_POINT('Ctrl Pts',(-4.66141348379231,3.86100938829084,
136.646521806489));
#273128=CARTESIAN_POINT('Ctrl Pts',(-4.93986110760522,7.00214555161287,
130.713814895061));
#273129=CARTESIAN_POINT('Ctrl Pts',(-5.21830873141809,3.70865202682979,
124.864315079211));
#273130=CARTESIAN_POINT('Ctrl Pts',(-5.49675635523098,-2.99291153288594,
124.473426925751));
#273131=CARTESIAN_POINT('Ctrl Pts',(-5.77520397904388,-6.9441356057364,
129.900357551763));
#273132=CARTESIAN_POINT('Ctrl Pts',(-6.05365160285679,-4.51403829679898,
136.158022832244));
#273133=CARTESIAN_POINT('Ctrl Pts',(-6.33209922666964,2.06423968386644,
137.495934078373));
#273134=CARTESIAN_POINT('Ctrl Pts',(-6.61054685048256,6.74558223877327,
132.684616215558));
#273135=CARTESIAN_POINT('Ctrl Pts',(-6.88899447429547,5.22806425626005,
126.145435313781));
#273136=CARTESIAN_POINT('Ctrl Pts',(-7.16744209810832,-1.09378937261818,
123.887579165027));
#273137=CARTESIAN_POINT('Ctrl Pts',(-7.44588972192122,-6.41050400264194,
127.985907267597));
#273138=CARTESIAN_POINT('Ctrl Pts',(-7.72433734573414,-5.8362786247684,
134.674256309687));
#273139=CARTESIAN_POINT('Ctrl Pts',(-8.002784969547,0.101201691205851,137.806360265633));
#273140=CARTESIAN_POINT('Ctrl Pts',(-8.28123259335988,5.94568259693924,
134.503968611703));
#273141=CARTESIAN_POINT('Ctrl Pts',(-8.55968021717279,6.32637165882838,
127.80181794706));
#273142=CARTESIAN_POINT('Ctrl Pts',(-8.8381278409857,0.893434226691435,
123.858857314246));
#273143=CARTESIAN_POINT('Ctrl Pts',(-9.11657546479855,-5.3605256130866,
126.298474910485));
#273144=CARTESIAN_POINT('Ctrl Pts',(-9.39502308861147,-6.68842429067269,
132.878781346775));
#273145=CARTESIAN_POINT('Ctrl Pts',(-9.67347071242438,-1.86998779282204,
137.552796474009));
#273146=CARTESIAN_POINT('Ctrl Pts',(-9.95191833623725,4.66687613264966,
136.025328728591));
#273147=CARTESIAN_POINT('Ctrl Pts',(-10.2303659600501,6.91510888178999,
129.700046347612));
#273148=CARTESIAN_POINT('Ctrl Pts',(-10.508813583863,2.80869439041515,124.389574831969));
#273149=CARTESIAN_POINT('Ctrl Pts',(-10.787261207676,-3.87877303340228,
124.973978073582));
#273150=CARTESIAN_POINT('Ctrl Pts',(-11.0657088314888,-7.00183752812002,
130.916218043094));
#273151=CARTESIAN_POINT('Ctrl Pts',(-11.3441564553017,-3.69055539327479,
136.755666503084));
#273152=CARTESIAN_POINT('Ctrl Pts',(-11.6226040791146,3.01216685433575,
137.126155591738));
#273153=CARTESIAN_POINT('Ctrl Pts',(-11.9010517029275,6.94685491534338,
131.687223935982));
#273154=CARTESIAN_POINT('Ctrl Pts',(-12.1794993267404,4.49772268187999,
125.436984020872));
#273155=CARTESIAN_POINT('Ctrl Pts',(-12.4579469505533,-2.08459697026297,
124.119100987199));
#273156=CARTESIAN_POINT('Ctrl Pts',(-12.7363945743662,-6.75127384495765,
128.944644960744));
#273157=CARTESIAN_POINT('Ctrl Pts',(-13.0148421981791,-5.21385987419926,
135.479176770748));
#273158=CARTESIAN_POINT('Ctrl Pts',(-13.2932898219919,1.11483660973293,
137.717780913442));
#273159=CARTESIAN_POINT('Ctrl Pts',(-13.5717374458049,6.41905271211686,
133.603289543584));
#273160=CARTESIAN_POINT('Ctrl Pts',(-13.8501850696177,5.82447296022373,
126.916719225995));
#273161=CARTESIAN_POINT('Ctrl Pts',(-14.1286326934306,-0.122512900792341,
123.802701425419));
#273162=CARTESIAN_POINT('Ctrl Pts',(-14.4070803172435,-5.95691539106803,
127.122866372359));
#273163=CARTESIAN_POINT('Ctrl Pts',(-14.6855279410564,-6.31720364844761,
133.826144679651));
#273164=CARTESIAN_POINT('Ctrl Pts',(-14.9639755648693,-0.872290365458834,
137.752551056246));
#273165=CARTESIAN_POINT('Ctrl Pts',(-15.2424231886822,5.37421514963333,
135.293909857666));
#273166=CARTESIAN_POINT('Ctrl Pts',(-15.5208708124951,6.68207948721813,
128.709592234107));
#273167=CARTESIAN_POINT('Ctrl Pts',(-15.799318436308,1.84943921378025,124.050264419823));
#273168=CARTESIAN_POINT('Ctrl Pts',(-16.0777660601209,-4.68274534699314,
125.59762105532));
#273169=CARTESIAN_POINT('Ctrl Pts',(-16.3562136839338,-6.91171569870797,
131.929716985153));
#273170=CARTESIAN_POINT('Ctrl Pts',(-16.6346613077467,-2.78915697939336,
137.227665389888));
#273171=CARTESIAN_POINT('Ctrl Pts',(-16.9131089315595,3.89650074609022,
136.622910504741));
#273172=CARTESIAN_POINT('Ctrl Pts',(-17.1915565553724,7.00146464056082,
130.671192525245));
#273173=CARTESIAN_POINT('Ctrl Pts',(-17.4700041791854,3.67242457091876,
124.841849516969));
#273174=CARTESIAN_POINT('Ctrl Pts',(-17.7484518029982,-3.0313942714833,
124.491762925279));
#273175=CARTESIAN_POINT('Ctrl Pts',(-18.0268994268111,-6.94950987023543,
129.942645225261));
#273176=CARTESIAN_POINT('Ctrl Pts',(-18.305347050624,-4.48136540067248,
136.185401873632));
#273177=CARTESIAN_POINT('Ctrl Pts',(-18.5837946744369,2.10493494523792,
137.483244486159));
#273178=CARTESIAN_POINT('Ctrl Pts',(-18.8622422982498,6.75690290826339,
132.643519105064));
#273179=CARTESIAN_POINT('Ctrl Pts',(-19.1406899220627,5.19960719165284,
126.113696921846));
#273180=CARTESIAN_POINT('Ctrl Pts',(-19.4191375458756,-1.1358735191536,
123.894365523333));
#273181=CARTESIAN_POINT('Ctrl Pts',(-19.6975851696885,-6.42754195636435,
128.024982044393));
#273182=CARTESIAN_POINT('Ctrl Pts',(-19.9760327935014,-5.81261333855723,
134.709711694007));
#273183=CARTESIAN_POINT('Ctrl Pts',(-20.2544804173143,0.143822975436045,
137.805614491377));
#273184=CARTESIAN_POINT('Ctrl Pts',(-20.5329280411272,5.96809300114641,
134.467707008981));
#273185=CARTESIAN_POINT('Ctrl Pts',(-20.81137566494,6.30797711635522,127.763363157294));
#273186=CARTESIAN_POINT('Ctrl Pts',(-21.089823288753,0.851138423447451,
123.853547410611));
#273187=CARTESIAN_POINT('Ctrl Pts',(-21.3682709125658,-5.38785490018508,
126.331189435016));
#273188=CARTESIAN_POINT('Ctrl Pts',(-21.6467185363787,-6.67567278189203,
132.919457249623));
#273189=CARTESIAN_POINT('Ctrl Pts',(-21.9251661601916,-1.82887350178604,
137.564054587584));
#273190=CARTESIAN_POINT('Ctrl Pts',(-22.2036137840045,4.69857118102365,
135.996823396506));
#273191=CARTESIAN_POINT('Ctrl Pts',(-22.4820614078173,6.90825848643574,
129.657972577492));
#273192=CARTESIAN_POINT('Ctrl Pts',(-22.7605090316303,2.76959373000234,
124.372596363135));
#273193=CARTESIAN_POINT('Ctrl Pts',(-23.0389566554432,-3.91419236212754,
124.997697289448));
#273194=CARTESIAN_POINT('Ctrl Pts',(-23.3174042792561,-7.0010268923895,
130.958838143028));
#273195=CARTESIAN_POINT('Ctrl Pts',(-23.5958519030689,-3.65425972772349,
136.778021697354));
#273196=CARTESIAN_POINT('Ctrl Pts',(-23.8742995268818,3.05059360620828,
137.107702548922));
#273197=CARTESIAN_POINT('Ctrl Pts',(-24.1527471506948,6.95210044581739,
131.644920100946));
#273198=CARTESIAN_POINT('Ctrl Pts',(-24.4311947745076,4.4649666047081,125.409704551357));
#273199=CARTESIAN_POINT('Ctrl Pts',(-24.7096423983205,-2.12525342038311,
124.131914383013));
#273200=CARTESIAN_POINT('Ctrl Pts',(-24.9880900221334,-6.76246937654364,
128.985776337104));
#273201=CARTESIAN_POINT('Ctrl Pts',(-25.2665376459463,-5.18530634065569,
135.510828402156));
#273202=CARTESIAN_POINT('Ctrl Pts',(-25.5449852697592,1.15689990599717,
137.710866496904));
#273203=CARTESIAN_POINT('Ctrl Pts',(-25.8234328935721,6.43597165674122,
133.564163090109));
#273204=CARTESIAN_POINT('Ctrl Pts',(-26.101880517385,5.8006998696348,126.881336034893));
#273205=CARTESIAN_POINT('Ctrl Pts',(-26.3803281411979,-0.165131717723356,
123.803576920747));
#273206=CARTESIAN_POINT('Ctrl Pts',(-26.6587757650107,-5.9792153236265,
127.15919601668));
#273207=CARTESIAN_POINT('Ctrl Pts',(-26.9372233888237,-6.29869214802456,
133.864543304637));
#273208=CARTESIAN_POINT('Ctrl Pts',(-27.2156710126366,-0.829978596605981,
137.75773220141));
#273209=CARTESIAN_POINT('Ctrl Pts',(-27.4941186364494,5.40144473838504,
135.261112303716));
#273210=CARTESIAN_POINT('Ctrl Pts',(-27.7725662602623,6.66920423404522,
128.668955330874));
#273211=CARTESIAN_POINT('Ctrl Pts',(-28.0510138840753,1.80829084735756,
124.039131496154));
#273212=CARTESIAN_POINT('Ctrl Pts',(-28.3294615078881,-4.71435348813263,
125.626222724194));
#273213=CARTESIAN_POINT('Ctrl Pts',(-28.607909131701,-6.9047372770006,131.971769710144));
#273214=CARTESIAN_POINT('Ctrl Pts',(-28.8863567555139,-2.75000482347336,
137.244524771118));
#273215=CARTESIAN_POINT('Ctrl Pts',(-29.1648043793268,3.93184771762154,
136.599083594488));
#273216=CARTESIAN_POINT('Ctrl Pts',(-29.4432520031397,7.00052428766157,
130.628575090021));
#273217=CARTESIAN_POINT('Ctrl Pts',(-29.7216996269525,3.63606103196502,
124.819604897767));
#273218=CARTESIAN_POINT('Ctrl Pts',(-30.0001472507655,-3.06976468065099,
124.510332840438));
#273219=CARTESIAN_POINT('Ctrl Pts',(-30.2785948745783,-6.95462661809053,
129.984964829937));
#273220=CARTESIAN_POINT('Ctrl Pts',(-30.5570424983912,-4.44852644590303,
136.212581518559));
#273221=CARTESIAN_POINT('Ctrl Pts',(-30.8354901222041,2.14555220747066,
137.470307405446));
#273222=CARTESIAN_POINT('Ctrl Pts',(-31.113937746017,6.7679731982313,132.602353843876));
#273223=CARTESIAN_POINT('Ctrl Pts',(-31.3923853698299,5.17095745368924,
126.082132344179));
#273224=CARTESIAN_POINT('Ctrl Pts',(-31.6708329936428,-1.17791557547805,
123.901407934047));
#273225=CARTESIAN_POINT('Ctrl Pts',(-31.9492806174558,-6.44434173515584,
128.064159812084));
#273226=CARTESIAN_POINT('Ctrl Pts',(-32.2277282412685,-5.78873266382121,
134.745022364106));
#273227=CARTESIAN_POINT('Ctrl Pts',(-32.5061758650815,0.186438930252996,
137.804609283086));
#273228=CARTESIAN_POINT('Ctrl Pts',(-32.7846234888944,5.99028225547263,
134.431309659613));
#273229=CARTESIAN_POINT('Ctrl Pts',(-33.0630711127073,6.28934882947028,
127.725021052809));
#273230=CARTESIAN_POINT('Ctrl Pts',(-33.3415187365202,0.808811080956172,
123.848495071916));
#273231=CARTESIAN_POINT('Ctrl Pts',(-33.619966360333,-5.41498453833882,
126.364069714552));
#273232=CARTESIAN_POINT('Ctrl Pts',(-33.898413984146,-6.66267390360147,
132.960054776787));
#273233=CARTESIAN_POINT('Ctrl Pts',(-34.1768616079588,-1.78769144116968,
137.575062218212));
#273234=CARTESIAN_POINT('Ctrl Pts',(-34.4553092317717,4.73009212211488,
135.968125655805));
#273235=CARTESIAN_POINT('Ctrl Pts',(-34.7337568555846,6.90115210302259,
129.615941287202));
#273236=CARTESIAN_POINT('Ctrl Pts',(-35.0122044793975,2.73039044127535,
124.355856225691));
#273237=CARTESIAN_POINT('Ctrl Pts',(-35.2906521032104,-3.94946664901538,
125.02163167336));
#273238=CARTESIAN_POINT('Ctrl Pts',(-35.5690997270233,-6.99995683103299,
131.00145251874));
#273239=CARTESIAN_POINT('Ctrl Pts',(-35.8475473508362,-3.61782865223385,
136.800155535415));
#273240=CARTESIAN_POINT('Ctrl Pts',(-36.125994974649,3.08890731721304,137.089015933453));
#273241=CARTESIAN_POINT('Ctrl Pts',(-36.404442598462,6.95708836365274,131.60258511867));
#273242=CARTESIAN_POINT('Ctrl Pts',(-36.6828902222748,4.43204507655667,
125.382624982808));
#273243=CARTESIAN_POINT('Ctrl Pts',(-36.9613378460878,-2.16583111845593,
124.144975028777));
#273244=CARTESIAN_POINT('Ctrl Pts',(-37.2397854699006,-6.7734143223399,
129.026975101771));
#273245=CARTESIAN_POINT('Ctrl Pts',(-37.5182330937135,-5.15656066367905,
135.54230563367));
#273246=CARTESIAN_POINT('Ctrl Pts',(-37.7966807175264,1.19892033290996,
137.703696157251));
#273247=CARTESIAN_POINT('Ctrl Pts',(-38.0751283413393,6.45265211406898,
133.524934371139));
#273248=CARTESIAN_POINT('Ctrl Pts',(-38.3535759651522,5.77671183197903,
126.846098212911));
#273249=CARTESIAN_POINT('Ctrl Pts',(-38.6320235889651,-0.207744415637528,
123.80471183269));
#273250=CARTESIAN_POINT('Ctrl Pts',(-38.910471212778,-6.00129369416227,
127.195660733917));
#273251=CARTESIAN_POINT('Ctrl Pts',(-39.1889188365908,-6.27994724724761,
133.902828533427));
#273252=CARTESIAN_POINT('Ctrl Pts',(-39.4673664604039,-0.787636072591,137.762655686833));
#273253=CARTESIAN_POINT('Ctrl Pts',(-39.7458140842166,5.42847417461558,
135.228149603194));
#273254=CARTESIAN_POINT('Ctrl Pts',(-40.0242617080296,6.65608185105682,
128.628397555869));
#273255=CARTESIAN_POINT('Ctrl Pts',(-40.3027093318424,1.76707547405252,
124.028249260538));
#273256=CARTESIAN_POINT('Ctrl Pts',(-40.5811569556554,-4.7457869371699,
125.655016270872));
#273257=CARTESIAN_POINT('Ctrl Pts',(-40.8596045794682,-6.89750299771422,
132.013779176361));
#273258=CARTESIAN_POINT('Ctrl Pts',(-41.1380522032811,-2.7107507651133,
137.261145509698));
#273259=CARTESIAN_POINT('Ctrl Pts',(-41.416499827094,3.96704899308973,136.575041958643));
#273260=CARTESIAN_POINT('Ctrl Pts',(-41.694947450907,6.99932452776054,130.585964168594));
#273261=CARTESIAN_POINT('Ctrl Pts',(-41.9733950747197,3.59956275743227,
124.79758204589));
#273262=CARTESIAN_POINT('Ctrl Pts',(-42.2518426985328,-3.10802133855968,
124.529135983109));
#273263=CARTESIAN_POINT('Ctrl Pts',(-42.5302903223456,-6.95948565969872,
130.027314797628));
#273264=CARTESIAN_POINT('Ctrl Pts',(-42.8087379461585,-4.41552264935019,
136.23956075987));
#273265=CARTESIAN_POINT('Ctrl Pts',(-43.0871855699714,2.18608996547759,
137.457123315624));
#273266=CARTESIAN_POINT('Ctrl Pts',(-43.3656331937842,6.77879269846351,
132.561121957388));
#273267=CARTESIAN_POINT('Ctrl Pts',(-43.6440808175972,5.14211610399531,
126.050742750417));
#273268=CARTESIAN_POINT('Ctrl Pts',(-43.92252844141,-1.21991398370768,123.908706136214));
#273269=CARTESIAN_POINT('Ctrl Pts',(-44.200976065223,-6.46090271649442,
128.103439118922));
#273270=CARTESIAN_POINT('Ctrl Pts',(-44.4794236890358,-5.76463748546755,
134.780187011534));
#273271=CARTESIAN_POINT('Ctrl Pts',(-44.7578713128487,0.229047976506494,
137.803344678006));
#273272=CARTESIAN_POINT('Ctrl Pts',(-45.0363189366615,6.01224953768695,
134.394777912313));
#273273=CARTESIAN_POINT('Ctrl Pts',(-45.3147665604746,6.27048748845154,
127.686793054383));
#273274=CARTESIAN_POINT('Ctrl Pts',(-45.5932141842873,0.766453767672844,
123.843700485376));
#273275=CARTESIAN_POINT('Ctrl Pts',(-45.8716618081003,-5.44191352224889,
126.397114530699));
#273276=CARTESIAN_POINT('Ctrl Pts',(-46.1501094319132,-6.6494281374793,
133.000572423912));
#273277=CARTESIAN_POINT('Ctrl Pts',(-46.4285570557261,-1.74644313698983,
137.585818958004));
#273278=CARTESIAN_POINT('Ctrl Pts',(-46.7070046795389,4.76143778790304,
135.93923656989));
#273279=CARTESIAN_POINT('Ctrl Pts',(-46.9854523033519,6.89378999488032,
129.573954034227));
#273280=CARTESIAN_POINT('Ctrl Pts',(-47.2638999271647,2.69108597692664,
124.339355039948));
#273281=CARTESIAN_POINT('Ctrl Pts',(-47.5423475509777,-3.98459458696386,
125.045780338419));
#273282=CARTESIAN_POINT('Ctrl Pts',(-47.8207951747905,-6.998627383702,131.044059591139));
#273283=CARTESIAN_POINT('Ctrl Pts',(-48.0992427986034,-3.58126351677304,
136.822067197091));
#273284=CARTESIAN_POINT('Ctrl Pts',(-48.3776904224163,3.1271065676212,137.070096437769));
#273285=CARTESIAN_POINT('Ctrl Pts',(-48.6561380462292,6.9618184840203,131.560220557891));
#273286=CARTESIAN_POINT('Ctrl Pts',(-48.9345856700421,4.39895931734504,
125.355746318666));
#273287=CARTESIAN_POINT('Ctrl Pts',(-49.213033293855,-2.20632856086043,
124.158282440523));
#273288=CARTESIAN_POINT('Ctrl Pts',(-49.4914809176678,-6.78410827677761,
129.068239728113));
#273289=CARTESIAN_POINT('Ctrl Pts',(-49.7699285414808,-5.12762390845042,
135.573607298891));
#273290=CARTESIAN_POINT('Ctrl Pts',(-50.0483761652936,1.2408963333889,137.696270160183));
#273291=CARTESIAN_POINT('Ctrl Pts',(-50.3268237891066,6.46909346599971,
133.485604840309));
#273292=CARTESIAN_POINT('Ctrl Pts',(-50.6052714129194,5.7525097361419,126.811007065796));
#273293=CARTESIAN_POINT('Ctrl Pts',(-50.8837190367324,-0.250349415506305,
123.806106119193));
#273294=CARTESIAN_POINT('Ctrl Pts',(-51.1621666605453,-6.02314968455324,
127.232259172855));
#273295=CARTESIAN_POINT('Ctrl Pts',(-51.4406142843581,-6.26096964071598,
133.94099894735));
#273296=CARTESIAN_POINT('Ctrl Pts',(-51.719061908171,-0.745264362431691,
137.767321330073));
#273297=CARTESIAN_POINT('Ctrl Pts',(-51.997509531984,5.45530245673899,135.195022977544));
#273298=CARTESIAN_POINT('Ctrl Pts',(-52.2759571557968,6.64271282450778,
128.587920411975));
#273299=CARTESIAN_POINT('Ctrl Pts',(-52.5544047796097,1.72579462111621,
124.01761811622));
#273300=CARTESIAN_POINT('Ctrl Pts',(-52.8328524034226,-4.77704452932697,
125.684000628399));
#273301=CARTESIAN_POINT('Ctrl Pts',(-53.1113000272355,-6.89001312891767,
132.05574382713));
#273302=CARTESIAN_POINT('Ctrl Pts',(-53.3897476510484,-2.67139625888694,
137.277526989739));
#273303=CARTESIAN_POINT('Ctrl Pts',(-53.6681952748612,4.00210326809833,
136.550786488079));
#273304=CARTESIAN_POINT('Ctrl Pts',(-53.9466428986742,6.99786540531528,
130.543361339928));
#273305=CARTESIAN_POINT('Ctrl Pts',(-54.225090522487,3.56293109977782,124.775781777402));
#273306=CARTESIAN_POINT('Ctrl Pts',(-54.5035381462999,-3.14616282759469,
124.548171656537));
#273307=CARTESIAN_POINT('Ctrl Pts',(-54.7819857701128,-6.9640868150063,
130.069693559035));
#273308=CARTESIAN_POINT('Ctrl Pts',(-55.0604333939257,-4.382355233982,136.266338597842));
#273309=CARTESIAN_POINT('Ctrl Pts',(-55.3388810177386,2.22654671711671,
137.443692705233));
#273310=CARTESIAN_POINT('Ctrl Pts',(-55.6173286415515,6.78936100803939,
132.519824973462));
#273311=CARTESIAN_POINT('Ctrl Pts',(-55.8957762653644,5.11308421129812,
126.019529303714));
#273312=CARTESIAN_POINT('Ctrl Pts',(-56.1742238891773,-1.26186718757599,
123.916259859391));
#273313=CARTESIAN_POINT('Ctrl Pts',(-56.4526715129901,-6.47722428670686,
128.142818509401));
#273314=CARTESIAN_POINT('Ctrl Pts',(-56.7311191368031,-5.74032869635189,
134.815204333253));
#273315=CARTESIAN_POINT('Ctrl Pts',(-57.0095667606159,0.271648535303317,
137.801820722997));
#273316=CARTESIAN_POINT('Ctrl Pts',(-57.2880143844289,6.03399403378365,
134.358113120779));
#273317=CARTESIAN_POINT('Ctrl Pts',(-57.5664620082417,6.25139379221294,
127.64868057857));
#273318=CARTESIAN_POINT('Ctrl Pts',(-57.8449096320546,0.724068053163303,
123.839163828657));
#273319=CARTESIAN_POINT('Ctrl Pts',(-58.1233572558676,-5.46864085405239,
126.430322658971));
#273320=CARTESIAN_POINT('Ctrl Pts',(-58.4018048796803,-6.63593597435208,
133.0410086896));
#273321=CARTESIAN_POINT('Ctrl Pts',(-58.6802525034934,-1.705130117717,137.596324408362));
#273322=CARTESIAN_POINT('Ctrl Pts',(-58.9587001273061,4.79260701686295,
135.910157209259));
#273323=CARTESIAN_POINT('Ctrl Pts',(-59.2371477511191,6.88617243481463,
129.532012374421));
#273324=CARTESIAN_POINT('Ctrl Pts',(-59.515595374932,2.65168179339722,124.323093417365));
#273325=CARTESIAN_POINT('Ctrl Pts',(-59.7940429987449,-4.01957487429483,
125.070142389788));
#273326=CARTESIAN_POINT('Ctrl Pts',(-60.0724906225578,-6.99703859965941,
131.086657781405));
#273327=CARTESIAN_POINT('Ctrl Pts',(-60.3509382463707,-3.5445656762756,
136.843755870437));
#273328=CARTESIAN_POINT('Ctrl Pts',(-60.6293858701835,3.16518994194552,
137.050944762941));
#273329=CARTESIAN_POINT('Ctrl Pts',(-60.9078334939965,6.96629063164357,
131.517827988445));
#273330=CARTESIAN_POINT('Ctrl Pts',(-61.1862811178092,4.36571055307847,
125.32906955493));
#273331=CARTESIAN_POINT('Ctrl Pts',(-61.4647287416223,-2.24674424694855,
124.171836125139));
#273332=CARTESIAN_POINT('Ctrl Pts',(-61.743176365435,-6.79455084358828,
129.109568687053));
#273333=CARTESIAN_POINT('Ctrl Pts',(-62.0216239892481,-5.09849714723216,
135.60473223792));
#273334=CARTESIAN_POINT('Ctrl Pts',(-62.3000716130609,1.2828263519976,137.688588780872));
#273335=CARTESIAN_POINT('Ctrl Pts',(-62.5785192368738,6.48529510329292,
133.446175954988));
#273336=CARTESIAN_POINT('Ctrl Pts',(-62.8569668606868,5.72809447894126,
126.776063893867));
#273337=CARTESIAN_POINT('Ctrl Pts',(-63.1354144844995,-0.292945138585431,
123.80775972859));
#273338=CARTESIAN_POINT('Ctrl Pts',(-63.4138621083125,-6.04478248491762,
127.268989977326));
#273339=CARTESIAN_POINT('Ctrl Pts',(-63.6923097321254,-6.24176003165182,
133.979053131985));
#273340=CARTESIAN_POINT('Ctrl Pts',(-63.9707573559382,-0.702865036227365,
137.771728958244));
#273341=CARTESIAN_POINT('Ctrl Pts',(-64.2492049797512,5.48192859062395,
135.161733654286));
#273342=CARTESIAN_POINT('Ctrl Pts',(-64.527652603564,6.62909764979204,128.547525399088));
#273343=CARTESIAN_POINT('Ctrl Pts',(-64.806100227377,1.68444981822529,124.007238457143));
#273344=CARTESIAN_POINT('Ctrl Pts',(-65.0845478511898,-4.80812510634223,
125.713174722747));
#273345=CARTESIAN_POINT('Ctrl Pts',(-65.3629954750027,-6.88226794815085,
132.097662107432));
#273346=CARTESIAN_POINT('Ctrl Pts',(-65.6414430988157,-2.63194276308962,
137.29366860422));
#273347=CARTESIAN_POINT('Ctrl Pts',(-65.9198907226284,4.03700924369883,
136.526318081592));
#273348=CARTESIAN_POINT('Ctrl Pts',(-66.1983383464414,6.99614697439381,
130.500768182686));
#273349=CARTESIAN_POINT('Ctrl Pts',(-66.4767859702543,3.5261674164012,124.75420490012));
#273350=CARTESIAN_POINT('Ctrl Pts',(-66.7552335940671,-3.18418773440913,
124.567439155348));
#273351=CARTESIAN_POINT('Ctrl Pts',(-67.0336812178801,-6.96842991351606,
130.112099543802));
#273352=CARTESIAN_POINT('Ctrl Pts',(-67.3121288416929,-4.34902542882876,
136.292914040211));
#273353=CARTESIAN_POINT('Ctrl Pts',(-67.5905764655059,2.26692096324861,
137.43001607195));
#273354=CARTESIAN_POINT('Ctrl Pts',(-67.8690240893187,6.79967773534632,
132.478464422373));
#273355=CARTESIAN_POINT('Ctrl Pts',(-68.1474717131316,5.08386285138514,
125.988493160695));
#273356=CARTESIAN_POINT('Ctrl Pts',(-68.4259193369445,-1.30377363249137,
123.924068823677));
#273357=CARTESIAN_POINT('Ctrl Pts',(-68.7043669607574,-6.49330584099122,
128.182296524302));
#273358=CARTESIAN_POINT('Ctrl Pts',(-68.9828145845703,-5.71580719724563,
134.850073031684));
#273359=CARTESIAN_POINT('Ctrl Pts',(-69.2612622083832,0.314239028063776,
137.800037474531));
#273360=CARTESIAN_POINT('Ctrl Pts',(-69.5397098321961,6.05551493801243,
134.32131664364));
#273361=CARTESIAN_POINT('Ctrl Pts',(-69.818157456009,6.23206844827842,127.610685037641));
#273362=CARTESIAN_POINT('Ctrl Pts',(-70.0966050798218,0.681655508046095,
123.834885269867));
#273363=CARTESIAN_POINT('Ctrl Pts',(-70.3750527036349,-5.49516554335789,
126.463692868828));
#273364=CARTESIAN_POINT('Ctrl Pts',(-70.6535003274475,-6.62219791417695,
133.081362075471));
#273365=CARTESIAN_POINT('Ctrl Pts',(-70.9319479512606,-1.66375391422059,
137.606578180005));
#273366=CARTESIAN_POINT('Ctrl Pts',(-71.2103955750734,4.82359865400735,
135.880888651457));
#273367=CARTESIAN_POINT('Ctrl Pts',(-71.4888431988863,6.87829970509706,
129.490117861946));
#273368=CARTESIAN_POINT('Ctrl Pts',(-71.7672908226993,2.6121793508235,124.307071960521));
#273369=CARTESIAN_POINT('Ctrl Pts',(-72.045738446512,-4.05440621480077,
125.094716924722));
#273370=CARTESIAN_POINT('Ctrl Pts',(-72.3241860703251,-6.99519053777849,
131.129245511046));
#273371=CARTESIAN_POINT('Ctrl Pts',(-72.6026336941378,-3.5077364905931,
136.865220751771));
#273372=CARTESIAN_POINT('Ctrl Pts',(-72.8810813179508,3.20315602899298,
137.031561618638));
#273373=CARTESIAN_POINT('Ctrl Pts',(-73.1595289417638,6.97050464080582,
131.475408981201));
#273374=CARTESIAN_POINT('Ctrl Pts',(-73.4379765655765,4.33230001580124,
125.302595680118));
#273375=CARTESIAN_POINT('Ctrl Pts',(-73.7164241893894,-2.28707667910305,
124.18563558039));
#273376=CARTESIAN_POINT('Ctrl Pts',(-73.9948718132024,-6.80474163581863,
129.150960447132));
#273377=CARTESIAN_POINT('Ctrl Pts',(-74.2733194370152,-5.0691814593271,
135.635679297414));
#273378=CARTESIAN_POINT('Ctrl Pts',(-74.5517670608282,1.32470883500465,
137.680652303954));
#273379=CARTESIAN_POINT('Ctrl Pts',(-74.830214684641,6.5012564255912,133.406649176227));
#273380=CARTESIAN_POINT('Ctrl Pts',(-75.108662308454,5.70346696509291,126.741269991954));
#273381=CARTESIAN_POINT('Ctrl Pts',(-75.3871099322667,-0.335530006474783,
123.809672599606));
#273382=CARTESIAN_POINT('Ctrl Pts',(-75.6655575560798,-6.06619129364391,
127.305851786256));
#273383=CARTESIAN_POINT('Ctrl Pts',(-75.9440051798925,-6.22231913187452,
134.016989677222));
#273384=CARTESIAN_POINT('Ctrl Pts',(-76.2224528037055,-0.66043966510086,
137.775878408018));
#273385=CARTESIAN_POINT('Ctrl Pts',(-76.5009004275184,5.50835158962877,
135.128282866967));
#273386=CARTESIAN_POINT('Ctrl Pts',(-76.7793480513312,6.61523683142527,
128.507214014061));
#273387=CARTESIAN_POINT('Ctrl Pts',(-77.0577956751442,1.64304259742666,
123.997110667925));
#273388=CARTESIAN_POINT('Ctrl Pts',(-77.336243298957,-4.83902751651344,
125.742537472861));
#273389=CARTESIAN_POINT('Ctrl Pts',(-77.6146909227699,-6.87426774241415,
132.139532463972));
#273390=CARTESIAN_POINT('Ctrl Pts',(-77.8931385465828,-2.59239173968542,
137.309569755007));
#273391=CARTESIAN_POINT('Ctrl Pts',(-78.1715861703958,4.07176562643718,
136.501637645866));
#273392=CARTESIAN_POINT('Ctrl Pts',(-78.4500337942086,6.99416929867323,
130.458186275174));
#273393=CARTESIAN_POINT('Ctrl Pts',(-78.7284814180215,3.48927306959449,
124.732852213582));
#273394=CARTESIAN_POINT('Ctrl Pts',(-79.0069290418344,-3.22209464997582,
124.586937765577));
#273395=CARTESIAN_POINT('Ctrl Pts',(-79.2853766656473,-6.97251479429268,
130.154531180556));
#273396=CARTESIAN_POINT('Ctrl Pts',(-79.5638242894601,-4.3155344689392,
136.319286102215));
#273397=CARTESIAN_POINT('Ctrl Pts',(-79.8422719132732,2.30721120779087,
137.416093922569));
#273398=CARTESIAN_POINT('Ctrl Pts',(-80.1207195370859,6.80974249809405,
132.437041836753));
#273399=CARTESIAN_POINT('Ctrl Pts',(-80.3991671608989,5.0544531070646,125.957635471416));
#273400=CARTESIAN_POINT('Ctrl Pts',(-80.6776147847117,-1.34563176559565,
123.932132739704));
#273401=CARTESIAN_POINT('Ctrl Pts',(-80.9560624085247,-6.50914678343976,
128.221871700751));
#273402=CARTESIAN_POINT('Ctrl Pts',(-81.2345100323374,-5.69107389680138,
134.884791814753));
#273403=CARTESIAN_POINT('Ctrl Pts',(-81.5129576561506,0.356817876581242,
137.797994998686));
#273404=CARTESIAN_POINT('Ctrl Pts',(-81.7914052799631,6.07681145290804,
134.284389844403));
#273405=CARTESIAN_POINT('Ctrl Pts',(-82.0698529037763,6.21251217275584,
127.572807839535));
#273406=CARTESIAN_POINT('Ctrl Pts',(-82.348300527589,0.639217703933302,
123.830864967548));
#273407=CARTESIAN_POINT('Ctrl Pts',(-82.626748151402,-5.52148660728364,
126.497223923725));
#273408=CARTESIAN_POINT('Ctrl Pts',(-82.9051957752149,-6.60821446602265,
133.121631086217));
#273409=CARTESIAN_POINT('Ctrl Pts',(-83.1836433990278,-1.62231605971109,
137.616579892973));
#273410=CARTESIAN_POINT('Ctrl Pts',(-83.4620910228406,4.85441155092967,
135.851431981043));
#273411=CARTESIAN_POINT('Ctrl Pts',(-83.7405386466535,6.87017209745416,
129.448272049221));
#273412=CARTESIAN_POINT('Ctrl Pts',(-84.0189862704665,2.57258011298421,
124.291291263097));
#273413=CARTESIAN_POINT('Ctrl Pts',(-84.2974338942792,-4.08908731779306,
125.119503032603));
#273414=CARTESIAN_POINT('Ctrl Pts',(-84.5758815180923,-6.99308326653956,
131.171821201958));
#273415=CARTESIAN_POINT('Ctrl Pts',(-84.8543291419051,-3.47077732444568,
136.886461045702));
#273416=CARTESIAN_POINT('Ctrl Pts',(-85.132776765718,3.2410034219148,137.011947723114));
#273417=CARTESIAN_POINT('Ctrl Pts',(-85.4112243895309,6.97446035535538,
131.432965108015));
#273418=CARTESIAN_POINT('Ctrl Pts',(-85.6896720133437,4.29872894355427,
125.27632567523));
#273419=CARTESIAN_POINT('Ctrl Pts',(-85.9681196371569,-2.327324362789,124.19968029493));
#273420=CARTESIAN_POINT('Ctrl Pts',(-86.2465672609694,-6.81468027584547,
129.192413474561));
#273421=CARTESIAN_POINT('Ctrl Pts',(-86.5250148847825,-5.03967793103904,
135.666447330617));
#273422=CARTESIAN_POINT('Ctrl Pts',(-86.8034625085954,1.36654223043768,
137.672461023519));
#273423=CARTESIAN_POINT('Ctrl Pts',(-87.0819101324082,6.51697684144191,
133.367025968708));
#273424=CARTESIAN_POINT('Ctrl Pts',(-87.3603577562212,5.67862810717874,
126.706626649358));
#273425=CARTESIAN_POINT('Ctrl Pts',(-87.638805380034,-0.378102441176264,
123.811844661359));
#273426=CARTESIAN_POINT('Ctrl Pts',(-87.917253003847,-6.08737531742114,
127.342843233717));
#273427=CARTESIAN_POINT('Ctrl Pts',(-88.1957006276599,-6.20264766177327,
134.054807177307));
#273428=CARTESIAN_POINT('Ctrl Pts',(-88.4741482514726,-0.617989821139493,
137.779769525637));
#273429=CARTESIAN_POINT('Ctrl Pts',(-88.7525958752857,5.53457047463998,
135.094671855119));
#273430=CARTESIAN_POINT('Ctrl Pts',(-89.0310434990984,6.6011308830247,128.466987750645));
#273431=CARTESIAN_POINT('Ctrl Pts',(-89.3094911229114,1.60157449308101,
123.987235123859));
#273432=CARTESIAN_POINT('Ctrl Pts',(-89.5879387467241,-4.86975061474005,
125.772087790693));
#273433=CARTESIAN_POINT('Ctrl Pts',(-89.8663863705374,-6.8660128081587,
132.181353345229));
#273434=CARTESIAN_POINT('Ctrl Pts',(-90.1448339943499,-2.55274465425183,
137.325229852876));
#273435=CARTESIAN_POINT('Ctrl Pts',(-90.4232816181632,4.10637112840284,
136.476746095445));
#273436=CARTESIAN_POINT('Ctrl Pts',(-90.7017292419757,6.99193245143733,
130.415617195278));
#273437=CARTESIAN_POINT('Ctrl Pts',(-90.9801768657889,3.45224942649073,
124.711724509022));
#273438=CARTESIAN_POINT('Ctrl Pts',(-91.2586244896016,-3.2598821696406,
124.606666764696));
#273439=CARTESIAN_POINT('Ctrl Pts',(-91.5370721134145,-6.97634130596949,
130.196986896981));
#273440=CARTESIAN_POINT('Ctrl Pts',(-91.8155197372274,-4.28188359533257,
136.345453806627));
#273441=CARTESIAN_POINT('Ctrl Pts',(-92.0939673610402,2.34741595777304,
137.401926772977));
#273442=CARTESIAN_POINT('Ctrl Pts',(-92.3724149848533,6.81955492332935,
132.395558751529));
#273443=CARTESIAN_POINT('Ctrl Pts',(-92.650862608666,5.02485606812542,125.926957379319));
#273444=CARTESIAN_POINT('Ctrl Pts',(-92.929310232479,-1.38744003581995,
123.940451308663));
#273445=CARTESIAN_POINT('Ctrl Pts',(-93.2077578562919,-6.52474652706058,
128.261542572277));
#273446=CARTESIAN_POINT('Ctrl Pts',(-93.4862054801047,-5.66612971152105,
134.919359395943));
#273447=CARTESIAN_POINT('Ctrl Pts',(-93.7646531039176,0.39938350308132,
137.795693371147));
#273448=CARTESIAN_POINT('Ctrl Pts',(-94.0431007277306,6.09788278932073,
134.247334091402));
#273449=CARTESIAN_POINT('Ctrl Pts',(-94.3215483515434,6.19272569030992,
127.535050387806));
#273450=CARTESIAN_POINT('Ctrl Pts',(-94.5999959753563,0.596756213373149,
123.827103070676));
#273451=CARTESIAN_POINT('Ctrl Pts',(-94.8784435991693,-5.54760307049237,
126.530914581157));
#273452=CARTESIAN_POINT('Ctrl Pts',(-95.1568912229821,-6.59398614805128,
133.161814229653));
#273453=CARTESIAN_POINT('Ctrl Pts',(-95.4353388467949,-1.58081808968337,
137.626329176652));
#273454=CARTESIAN_POINT('Ctrl Pts',(-95.7137864706081,4.88504456584684,
135.821788289543));
#273455=CARTESIAN_POINT('Ctrl Pts',(-95.9922340944205,6.86178991305786,
129.406476486855));
#273456=CARTESIAN_POINT('Ctrl Pts',(-96.2706817182339,2.53288554724217,
124.275751909854));
#273457=CARTESIAN_POINT('Ctrl Pts',(-96.5491293420464,-4.12361689815126,
125.144499794972));
#273458=CARTESIAN_POINT('Ctrl Pts',(-96.8275769658595,-6.99071686402826,
131.214383276482));
#273459=CARTESIAN_POINT('Ctrl Pts',(-97.1060245896722,-3.4336895473684,
136.907475965166));
#273460=CARTESIAN_POINT('Ctrl Pts',(-97.3844722134854,3.27873071826322,
136.992103803166));
#273461=CARTESIAN_POINT('Ctrl Pts',(-97.6629198372979,6.9781576287114,131.390497941658));
#273462=CARTESIAN_POINT('Ctrl Pts',(-97.9413674611112,4.26499858032525,
125.250260513709));
#273463=CARTESIAN_POINT('Ctrl Pts',(-98.2198150849237,-2.36748580661544,
124.21396974833));
#273464=CARTESIAN_POINT('Ctrl Pts',(-98.498262708737,-6.82436639538843,
129.233926233285));
#273465=CARTESIAN_POINT('Ctrl Pts',(-98.7767103325495,-5.00998765563179,
135.69703519741));
#273466=CARTESIAN_POINT('Ctrl Pts',(-99.0551579563628,1.40832498814648,
137.664015243098));
#273467=CARTESIAN_POINT('Ctrl Pts',(-99.3336055801754,6.53245576831905,
133.327307800681));
#273468=CARTESIAN_POINT('Ctrl Pts',(-99.6120532039884,5.65357882561176,
126.672135149802));
#273469=CARTESIAN_POINT('Ctrl Pts',(-99.8905008278013,-0.420660865152761,
123.814275833361));
#273470=CARTESIAN_POINT('Ctrl Pts',(-100.168948451614,-6.10833377126732,
127.379962948978));
#273471=CARTESIAN_POINT('Ctrl Pts',(-100.447396075427,-6.18274635028192,
134.092504230901));
#273472=CARTESIAN_POINT('Ctrl Pts',(-100.72584369924,-0.575517077338011,
137.783402166914));
#273473=CARTESIAN_POINT('Ctrl Pts',(-101.004291323053,5.56058427410689,
135.060901864211));
#273474=CARTESIAN_POINT('Ctrl Pts',(-101.282738946866,6.58678032729173,
128.426848099441));
#273475=CARTESIAN_POINT('Ctrl Pts',(-101.561186570679,1.56004704180311,
123.977612190885));
#273476=CARTESIAN_POINT('Ctrl Pts',(-101.839634194492,-4.90029326256724,
125.801824581246));
#273477=CARTESIAN_POINT('Ctrl Pts',(-102.118081818304,-6.85750345127332,
132.223123201514));
#273478=CARTESIAN_POINT('Ctrl Pts',(-102.396529442117,-2.51300297592632,
137.340648317539));
#273479=CARTESIAN_POINT('Ctrl Pts',(-102.67497706593,4.14082446727623,136.451644352694));
#273480=CARTESIAN_POINT('Ctrl Pts',(-102.953424689743,6.98943651557314,
130.373062520413));
#273481=CARTESIAN_POINT('Ctrl Pts',(-103.231872313556,3.41509785901489,
124.690822569333));
#273482=CARTESIAN_POINT('Ctrl Pts',(-103.510319937369,-3.29754889317273,
124.626625421641));
#273483=CARTESIAN_POINT('Ctrl Pts',(-103.788767561182,-6.97990930675369,
130.239465119861));
#273484=CARTESIAN_POINT('Ctrl Pts',(-104.067215184995,-4.24807405495459,
136.371416183792));
#273485=CARTESIAN_POINT('Ctrl Pts',(-104.345662808808,2.38753372339306,
137.387515148146));
#273486=CARTESIAN_POINT('Ctrl Pts',(-104.62411043262,6.82911464744894,132.354016703874));
#273487=CARTESIAN_POINT('Ctrl Pts',(-104.902558056433,4.99507283129728,
125.896460021193));
#273488=CARTESIAN_POINT('Ctrl Pts',(-105.181005680246,-1.42919689394351,
123.949024222305));
#273489=CARTESIAN_POINT('Ctrl Pts',(-105.459453304059,-6.54010449379936,
128.301307668861));
#273490=CARTESIAN_POINT('Ctrl Pts',(-105.737900927872,-5.64097556572054,
134.953774494342));
#273491=CARTESIAN_POINT('Ctrl Pts',(-106.016348551685,0.441934330278796,
137.793132677202));
#273492=CARTESIAN_POINT('Ctrl Pts',(-106.294796175498,6.11872816644418,
134.210150757753));
#273493=CARTESIAN_POINT('Ctrl Pts',(-106.573243799311,6.17270973413615,
127.49741408157));
#273494=CARTESIAN_POINT('Ctrl Pts',(-106.851691423124,0.554272609792058,
123.823599718647));
#273495=CARTESIAN_POINT('Ctrl Pts',(-107.130139046936,-5.57351396522919,
126.564763592701));
#273496=CARTESIAN_POINT('Ctrl Pts',(-107.40858667075,-6.57951348749827,
133.201910016778));
#273497=CARTESIAN_POINT('Ctrl Pts',(-107.687034294562,-1.53926154185996,
137.635825669776));
#273498=CARTESIAN_POINT('Ctrl Pts',(-107.965481918375,4.91549656364115,
135.791958675416));
#273499=CARTESIAN_POINT('Ctrl Pts',(-108.243929542188,6.85315346251289,
129.364732723601));
#273500=CARTESIAN_POINT('Ctrl Pts',(-108.522377166001,2.49309712449469,
124.260454476607));
#273501=CARTESIAN_POINT('Ctrl Pts',(-108.800824789814,-4.15799367636883,
125.169706285567));
#273502=CARTESIAN_POINT('Ctrl Pts',(-109.079272413627,-6.98809141793296,
131.256930157466));
#273503=CARTESIAN_POINT('Ctrl Pts',(-109.35772003744,-3.39647453366164,
136.928264731447));
#273504=CARTESIAN_POINT('Ctrl Pts',(-109.636167661252,3.31633652003941,
136.97203059412));
#273505=CARTESIAN_POINT('Ctrl Pts',(-109.914615285065,6.98159632387027,
131.348009055767));
#273506=CARTESIAN_POINT('Ctrl Pts',(-110.193062908878,4.23111017600536,
125.22440116141));
#273507=CARTESIAN_POINT('Ctrl Pts',(-110.471510532691,-2.40755952238467,
124.228503411086));
#273508=CARTESIAN_POINT('Ctrl Pts',(-110.749958156504,-6.83379963552497,
129.275497185033));
#273509=CARTESIAN_POINT('Ctrl Pts',(-111.028405780317,-4.98011173328953,
135.727441764346));
#273510=CARTESIAN_POINT('Ctrl Pts',(-111.30685340413,1.45005555985492,137.655315275653));
#273511=CARTESIAN_POINT('Ctrl Pts',(-111.585301027943,6.54769263264538,
133.287496143919));
#273512=CARTESIAN_POINT('Ctrl Pts',(-111.863748651756,5.62832004860235,
126.63779677138));
#273513=CARTESIAN_POINT('Ctrl Pts',(-112.142196275568,-0.463203701385527,
123.816966025527));
#273514=CARTESIAN_POINT('Ctrl Pts',(-112.420643899382,-6.12906587855929,
127.417209556553));
#273515=CARTESIAN_POINT('Ctrl Pts',(-112.699091523194,-6.16261593485082,
134.130079441122));
#273516=CARTESIAN_POINT('Ctrl Pts',(-112.977539147007,-0.533023007539609,
137.786776197239));
#273517=CARTESIAN_POINT('Ctrl Pts',(-113.25598677082,5.58639202407863,135.026974145601));
#273518=CARTESIAN_POINT('Ctrl Pts',(-113.534434394633,6.57218569599142,
128.386796547837));
#273519=CARTESIAN_POINT('Ctrl Pts',(-113.812882018446,1.5184617824084,123.968242225583));
#273520=CARTESIAN_POINT('Ctrl Pts',(-114.091329642259,-4.93065432822552,
125.831746742611));
#273521=CARTESIAN_POINT('Ctrl Pts',(-114.369777266072,-6.84873998707567,
132.26484048503));
#273522=CARTESIAN_POINT('Ctrl Pts',(-114.648224889884,-2.4731681773514,
137.355824577657));
#273523=CARTESIAN_POINT('Ctrl Pts',(-114.926672513697,4.17512436637621,
136.426333347767));
#273524=CARTESIAN_POINT('Ctrl Pts',(-115.20512013751,6.98668158356849,130.330523827459));
#273525=CARTESIAN_POINT('Ctrl Pts',(-115.483567761323,3.377819743832,124.670147169045));
#273526=CARTESIAN_POINT('Ctrl Pts',(-115.762015385136,-3.33509342481799,
124.646812996834));
#273527=CARTESIAN_POINT('Ctrl Pts',(-116.040463008949,-6.98321866443162,
130.281964275151));
#273528=CARTESIAN_POINT('Ctrl Pts',(-116.318910632762,-4.21410710063033,
136.397172271667));
#273529=CARTESIAN_POINT('Ctrl Pts',(-116.597358256575,2.42756301807353,
137.372859582102));
#273530=CARTESIAN_POINT('Ctrl Pts',(-116.875805880388,6.83842131621399,
132.312417233142));
#273531=CARTESIAN_POINT('Ctrl Pts',(-117.154253504201,4.96510450020791,
125.866144527128));
#273532=CARTESIAN_POINT('Ctrl Pts',(-117.432701128013,-1.47090079265054,
123.957851162959));
#273533=CARTESIAN_POINT('Ctrl Pts',(-117.711148751826,-6.55522011456102,
128.341165516992));
#273534=CARTESIAN_POINT('Ctrl Pts',(-117.989596375639,-5.61561239149597,
134.988035834682));
#273535=CARTESIAN_POINT('Ctrl Pts',(-118.268043999452,0.484468781437156,
137.790313011739));
#273536=CARTESIAN_POINT('Ctrl Pts',(-118.546491623265,6.13934681184524,
134.172841221298));
#273537=CARTESIAN_POINT('Ctrl Pts',(-118.824939247078,6.15246504593319,
127.459900315453));
#273538=CARTESIAN_POINT('Ctrl Pts',(-119.103386870891,0.511768467435545,
123.820355041281));
#273539=CARTESIAN_POINT('Ctrl Pts',(-119.381834494704,-5.59921833135585,
126.598769704074));
#273540=CARTESIAN_POINT('Ctrl Pts',(-119.660282118516,-6.56479702065358,
133.241916961827));
#273541=CARTESIAN_POINT('Ctrl Pts',(-119.93872974233,-1.49764795613459,
137.645069020452));
#273542=CARTESIAN_POINT('Ctrl Pts',(-120.217177366142,4.94576641590264,
135.761944244007));
#273543=CARTESIAN_POINT('Ctrl Pts',(-120.495624989955,6.84426306584611,
129.323042306287));
#273544=CARTESIAN_POINT('Ctrl Pts',(-120.774072613768,2.45321631911644,
124.245399530209));
#273545=CARTESIAN_POINT('Ctrl Pts',(-121.052520237581,-4.19221637860163,
125.195121570349));
#273546=CARTESIAN_POINT('Ctrl Pts',(-121.330967861394,-6.98520702554029,
131.299460268319));
#273547=CARTESIAN_POINT('Ctrl Pts',(-121.609415485207,-3.35913366234199,
136.948826574209));
#273548=CARTESIAN_POINT('Ctrl Pts',(-121.88786310902,3.3538194337463,136.951728839794));
#273549=CARTESIAN_POINT('Ctrl Pts',(-122.166310732833,6.98477631340985,
131.305500024783));
#273550=CARTESIAN_POINT('Ctrl Pts',(-122.444758356646,4.19706498634193,
125.198748576561));
#273551=CARTESIAN_POINT('Ctrl Pts',(-122.723205980458,-2.44754402515043,
124.24328074465));
#273552=CARTESIAN_POINT('Ctrl Pts',(-123.001653604271,-6.84297964670285,
129.317124789377));
#273553=CARTESIAN_POINT('Ctrl Pts',(-123.280101228084,-4.95005127107555,
135.7576659047));
#273554=CARTESIAN_POINT('Ctrl Pts',(-123.558548851897,1.49173239922134,
137.646361443563));
#273555=CARTESIAN_POINT('Ctrl Pts',(-123.83699647571,6.5626868698133,133.247592473656));
#273556=CARTESIAN_POINT('Ctrl Pts',(-124.115444099523,5.60285271212367,
126.603612786514));
#273557=CARTESIAN_POINT('Ctrl Pts',(-124.393891723336,-0.505729373435472,
123.819915138168));
#273558=CARTESIAN_POINT('Ctrl Pts',(-124.672339347149,-6.14957087106115,
127.454581676257));
#273559=CARTESIAN_POINT('Ctrl Pts',(-124.950786970961,-6.14225716141998,
134.167531415611));
#273560=CARTESIAN_POINT('Ctrl Pts',(-125.229234594775,-0.490509186377616,
137.789891491587));
#273561=CARTESIAN_POINT('Ctrl Pts',(-125.507682218587,5.6119927682395,134.992889956494));
#273562=CARTESIAN_POINT('Ctrl Pts',(-125.786129842401,6.55734752993325,
128.346834579959));
#273563=CARTESIAN_POINT('Ctrl Pts',(-126.064577466213,1.47682025585389,
123.959125575163));
#273564=CARTESIAN_POINT('Ctrl Pts',(-126.343025090026,-4.9608326866744,
125.861853166013));
#273565=CARTESIAN_POINT('Ctrl Pts',(-126.621472713839,-6.8397227402992,
132.306503649927));
#273566=CARTESIAN_POINT('Ctrl Pts',(-126.899920337652,-2.43324173462049,
137.370758070868));
#273567=CARTESIAN_POINT('Ctrl Pts',(-127.178367961465,4.20926955470684,
136.400814018573));
#273568=CARTESIAN_POINT('Ctrl Pts',(-127.456815585278,6.98366775750873,
130.288002692701));
#273569=CARTESIAN_POINT('Ctrl Pts',(-127.73526320909,3.34041646229627,124.649699074291));
#273570=CARTESIAN_POINT('Ctrl Pts',(-128.013710832904,-3.37251437334987,
124.66722874222));
#273571=CARTESIAN_POINT('Ctrl Pts',(-128.292158456716,-6.9862692563739,
130.324482788031));
#273572=CARTESIAN_POINT('Ctrl Pts',(-128.570606080529,-4.17998399101771,
136.422721115849));
#273573=CARTESIAN_POINT('Ctrl Pts',(-128.849053704342,2.46750235851359,
137.357960617914));
#273574=CARTESIAN_POINT('Ctrl Pts',(-129.127501328155,6.84747458476236,
132.270761880817));
#273575=CARTESIAN_POINT('Ctrl Pts',(-129.405948951968,4.93495218534535,
125.836012020477));
#273576=CARTESIAN_POINT('Ctrl Pts',(-129.684396575781,-1.51255018658779,
123.966931803538));
#273577=CARTESIAN_POINT('Ctrl Pts',(-129.962844199593,-6.57009282923063,
128.381114639724));
#273578=CARTESIAN_POINT('Ctrl Pts',(-130.241291823406,-5.59004112868908,
135.022142147398));
#273579=CARTESIAN_POINT('Ctrl Pts',(-130.519739447219,0.52698528042665,
137.78723447924));
#273580=CARTESIAN_POINT('Ctrl Pts',(-130.798187071032,6.15973796149245,
134.135406864555));
#273581=CARTESIAN_POINT('Ctrl Pts',(-131.076634694845,6.13199237587537,
127.422510479544));
#273582=CARTESIAN_POINT('Ctrl Pts',(-131.355082318658,0.4692453613103,123.81736915881));
#273583=CARTESIAN_POINT('Ctrl Pts',(-131.633529942471,-5.62471521638866,
126.632931655165));
#273584=CARTESIAN_POINT('Ctrl Pts',(-131.911977566284,-6.54983729284086,
133.281833582332));
#273585=CARTESIAN_POINT('Ctrl Pts',(-132.190425190097,-1.45597887451291,
137.654058886162));
#273586=CARTESIAN_POINT('Ctrl Pts',(-132.46887281391,4.97585300097076,135.731746107516));
#273587=CARTESIAN_POINT('Ctrl Pts',(-132.747320437723,6.83511905249447,
129.281406779768));
#273588=CARTESIAN_POINT('Ctrl Pts',(-133.025768061535,2.4132446089053,124.230587628526));
#273589=CARTESIAN_POINT('Ctrl Pts',(-133.304215685348,-4.22628373671482,
125.220744707546));
#273590=CARTESIAN_POINT('Ctrl Pts',(-133.582663309161,-6.98206379373247,
131.341972033073));
#273591=CARTESIAN_POINT('Ctrl Pts',(-133.861110932974,-3.32166831708915,
136.969160731525));
#273592=CARTESIAN_POINT('Ctrl Pts',(-134.139558556787,3.39117807044069,
136.931199292478));
#273593=CARTESIAN_POINT('Ctrl Pts',(-134.4180061806,6.98769747949419,131.262972423894));
#273594=CARTESIAN_POINT('Ctrl Pts',(-134.696453804413,4.16286427289247,
125.173303709728));
#273595=CARTESIAN_POINT('Ctrl Pts',(-134.974901428226,-2.48743783327188,
124.25830120144));
#273596=CARTESIAN_POINT('Ctrl Pts',(-135.253349052039,-6.85190608875344,
129.358807503792));
#273597=CARTESIAN_POINT('Ctrl Pts',(-135.531796675851,-4.91980738289134,
135.787706498505));
#273598=CARTESIAN_POINT('Ctrl Pts',(-135.810244299665,1.53335396189511,
137.637154078616));
#273599=CARTESIAN_POINT('Ctrl Pts',(-136.088691923477,6.57743792420584,
133.207598268539));
#273600=CARTESIAN_POINT('Ctrl Pts',(-136.36713954729,5.57717775987727,126.569584461903));
#273601=CARTESIAN_POINT('Ctrl Pts',(-136.645587171103,-0.548236305497475,
123.823123062006));
#273602=CARTESIAN_POINT('Ctrl Pts',(-136.924034794916,-6.1698479889529,
127.492077923251));
#273603=CARTESIAN_POINT('Ctrl Pts',(-137.202482418729,-6.12167078439119,
134.204858766568));
#273604=CARTESIAN_POINT('Ctrl Pts',(-137.480930042542,-0.447977189217358,
137.792747934521));
#273605=CARTESIAN_POINT('Ctrl Pts',(-137.759377666354,5.63738555794455,
134.958650559891));
#273606=CARTESIAN_POINT('Ctrl Pts',(-138.037825290167,6.54226637895086,
128.306963676612));
#273607=CARTESIAN_POINT('Ctrl Pts',(-138.31627291398,1.43512400518173,123.950262577445));
#273608=CARTESIAN_POINT('Ctrl Pts',(-138.594720537793,-4.99082721964375,
125.892142735845));
#273609=CARTESIAN_POINT('Ctrl Pts',(-138.873168161606,-6.83045204508126,
132.348111152362));
#273610=CARTESIAN_POINT('Ctrl Pts',(-139.151615785419,-2.39322512722196,
137.385448243807));
#273611=CARTESIAN_POINT('Ctrl Pts',(-139.430063409232,4.24325876700673,
136.375087310741));
#273612=CARTESIAN_POINT('Ctrl Pts',(-139.708511033045,6.98039514907165,
130.245500691775));
#273613=CARTESIAN_POINT('Ctrl Pts',(-139.986958656858,3.30288940040013,
124.629479042785));
#273614=CARTESIAN_POINT('Ctrl Pts',(-140.26540628067,-3.40981035212143,
124.687871901284));
#273615=CARTESIAN_POINT('Ctrl Pts',(-140.543853904484,-6.98906096953965,
130.36701908296));
#273616=CARTESIAN_POINT('Ctrl Pts',(-140.822301528296,-4.1457059905611,
136.448061769617));
#273617=CARTESIAN_POINT('Ctrl Pts',(-141.100749152109,2.50735026474636,
137.342818807668));
#273618=CARTESIAN_POINT('Ctrl Pts',(-141.379196775922,6.85627411762182,
132.229052190456));
#273619=CARTESIAN_POINT('Ctrl Pts',(-141.657644399735,4.90461700401472,
125.80606361781));
#273620=CARTESIAN_POINT('Ctrl Pts',(-141.936092023548,-1.5541435324211,
123.976265807557));
#273621=CARTESIAN_POINT('Ctrl Pts',(-142.214539647361,-6.58472208669408,
128.421153556726));
#273622=CARTESIAN_POINT('Ctrl Pts',(-142.492987271174,-5.56426272485295,
135.056092168669));
#273623=CARTESIAN_POINT('Ctrl Pts',(-142.771434894987,0.569482251782813,
137.783897193782));
#273624=CARTESIAN_POINT('Ctrl Pts',(-143.0498825188,6.17990085978423,134.097849074668));
#273625=CARTESIAN_POINT('Ctrl Pts',(-143.328330142612,6.11129248258502,
127.385245959334));
#273626=CARTESIAN_POINT('Ctrl Pts',(-143.606777766425,0.426704867125613,
123.814642181877));
#273627=CARTESIAN_POINT('Ctrl Pts',(-143.885225390238,-5.65000367553061,
126.667248180088));
#273628=CARTESIAN_POINT('Ctrl Pts',(-144.163673014051,-6.53463485839856,
133.321658399163));
#273629=CARTESIAN_POINT('Ctrl Pts',(-144.442120637864,-1.4142558410586,
137.662794933783));
#273630=CARTESIAN_POINT('Ctrl Pts',(-144.720568261677,5.00575520397605,
135.701365384942));
#273631=CARTESIAN_POINT('Ctrl Pts',(-144.99901588549,6.82572176129271,129.239827686864));
#273632=CARTESIAN_POINT('Ctrl Pts',(-145.277463509303,2.37318347502772,
124.216019320419));
#273633=CARTESIAN_POINT('Ctrl Pts',(-145.555911133116,-4.26019448832994,
125.246574747685));
#273634=CARTESIAN_POINT('Ctrl Pts',(-145.834358756928,-6.97866183898313,
131.384463876438));
#273635=CARTESIAN_POINT('Ctrl Pts',(-146.112806380741,-3.28407988619528,
136.989266449907));
#273636=CARTESIAN_POINT('Ctrl Pts',(-146.391254004554,3.42841104578457,
136.910442712901));
#273637=CARTESIAN_POINT('Ctrl Pts',(-146.669701628367,6.99035971387901,
131.220427828976));
#273638=CARTESIAN_POINT('Ctrl Pts',(-146.94814925218,4.12850930297597,125.148067503779));
#273639=CARTESIAN_POINT('Ctrl Pts',(-147.226596875993,-2.52723946847004,
124.27356422487));
#273640=CARTESIAN_POINT('Ctrl Pts',(-147.505044499806,-6.86057863090408,
129.400543783708));
#273641=CARTESIAN_POINT('Ctrl Pts',(-147.783492123619,-4.88938118943532,
135.817562432597));
#273642=CARTESIAN_POINT('Ctrl Pts',(-148.061939747432,1.57491870557395,
137.627693521995));
#273643=CARTESIAN_POINT('Ctrl Pts',(-148.340387371245,6.5919452492172,133.167515010566));
#273644=CARTESIAN_POINT('Ctrl Pts',(-148.618834995057,5.55129614325799,
126.535713058481));
#273645=CARTESIAN_POINT('Ctrl Pts',(-148.89728261887,-0.590722922461593,
123.826589678167));
#273646=CARTESIAN_POINT('Ctrl Pts',(-149.175730242683,-6.18989648085842,
127.529696908099));
#273647=CARTESIAN_POINT('Ctrl Pts',(-149.454177866496,-6.10085756660025,
134.242060110815));
#273648=CARTESIAN_POINT('Ctrl Pts',(-149.732625490309,-0.405428592098244,
137.795345420191));
#273649=CARTESIAN_POINT('Ctrl Pts',(-150.011073114122,5.66256945225453,
134.924257224548));
#273650=CARTESIAN_POINT('Ctrl Pts',(-150.289520737935,6.52694280188189,
128.267185315226));
#273651=CARTESIAN_POINT('Ctrl Pts',(-150.567968361748,1.39337457546175,
123.94165356085));
#273652=CARTESIAN_POINT('Ctrl Pts',(-150.84641598556,-5.02063681567507,
125.922614329717));
#273653=CARTESIAN_POINT('Ctrl Pts',(-151.124863609373,-6.8209282449509,
132.389661450552));
#273654=CARTESIAN_POINT('Ctrl Pts',(-151.403311233186,-2.35311983798619,
137.399894552124));
#273655=CARTESIAN_POINT('Ctrl Pts',(-151.681758856999,4.2770907437925,136.349154177582));
#273656=CARTESIAN_POINT('Ctrl Pts',(-151.960206480812,6.97686387952531,
130.20301939961));
#273657=CARTESIAN_POINT('Ctrl Pts',(-152.238654104625,3.26523994872261,
124.609487823786));
#273658=CARTESIAN_POINT('Ctrl Pts',(-152.517101728438,-3.44697997911642,
124.708741709087));
#273659=CARTESIAN_POINT('Ctrl Pts',(-152.795549352251,-6.99159370048095,
130.40957158374));
#273660=CARTESIAN_POINT('Ctrl Pts',(-153.073996976064,-4.11127436944443,
136.473193293963));
#273661=CARTESIAN_POINT('Ctrl Pts',(-153.352444599876,2.54710526019297,
137.327434712448));
#273662=CARTESIAN_POINT('Ctrl Pts',(-153.63089222369,6.86481958872245,132.187289707623));
#273663=CARTESIAN_POINT('Ctrl Pts',(-153.909339847502,4.87410008029735,
125.776300428876));
#273664=CARTESIAN_POINT('Ctrl Pts',(-154.187787471315,-1.5956792888948,
123.98585282914));
#273665=CARTESIAN_POINT('Ctrl Pts',(-154.466235095128,-6.5991073448593,
128.461280784342));
#273666=CARTESIAN_POINT('Ctrl Pts',(-154.744682718941,-5.53827813521478,
135.089884640464));
#273667=CARTESIAN_POINT('Ctrl Pts',(-155.023130342754,0.611958120764675,
137.78030127903));
#273668=CARTESIAN_POINT('Ctrl Pts',(-155.301577966567,6.19983475957701,
134.060169243357));
#273669=CARTESIAN_POINT('Ctrl Pts',(-155.58002559038,6.0903661331043,127.348108135675));
#273670=CARTESIAN_POINT('Ctrl Pts',(-155.858473214192,0.38414856123516,
123.812174211531));
#273671=CARTESIAN_POINT('Ctrl Pts',(-156.136920838005,-5.67508277170857,
126.701718007236));
#273672=CARTESIAN_POINT('Ctrl Pts',(-156.415368461818,-6.51919028065846,
133.3613899366));
#273673=CARTESIAN_POINT('Ctrl Pts',(-156.693816085631,-1.37248040183399,
137.671276839599));
#273674=CARTESIAN_POINT('Ctrl Pts',(-156.972263709444,5.03547191688086,
135.670803202055));
#273675=CARTESIAN_POINT('Ctrl Pts',(-157.250711333257,6.81607154046107,
129.198306568304));
#273676=CARTESIAN_POINT('Ctrl Pts',(-157.52915895707,2.33303440196427,124.201695145721));
#273677=CARTESIAN_POINT('Ctrl Pts',(-157.807606580883,-4.29394737687161,
125.272610733624));
#273678=CARTESIAN_POINT('Ctrl Pts',(-158.086054204696,-6.97500128735293,
131.426934223863));
#273679=CARTESIAN_POINT('Ctrl Pts',(-158.364501828508,-3.2463697625135,
137.009142984327));
#273680=CARTESIAN_POINT('Ctrl Pts',(-158.642949452322,3.46551698009634,
136.889459870208));
#273681=CARTESIAN_POINT('Ctrl Pts',(-158.921397076134,6.99276291791392,
131.177867816534));
#273682=CARTESIAN_POINT('Ctrl Pts',(-159.199844699947,4.09400134962899,
125.123040893851));
#273683=CARTESIAN_POINT('Ctrl Pts',(-159.47829232376,-2.56694745588028,
124.289069249361));
#273684=CARTESIAN_POINT('Ctrl Pts',(-159.756739947573,-6.86899695179061,
129.442332082575));
#273685=CARTESIAN_POINT('Ctrl Pts',(-160.035187571386,-4.85877381816122,
135.84723260065));
#273686=CARTESIAN_POINT('Ctrl Pts',(-160.313635195198,1.61642509006095,
137.617980124263));
#273687=CARTESIAN_POINT('Ctrl Pts',(-160.592082819012,6.60620830727321,
133.12734418504));
#273688=CARTESIAN_POINT('Ctrl Pts',(-160.870530442824,5.52520882131862,
126.501999831362));
#273689=CARTESIAN_POINT('Ctrl Pts',(-161.148978066638,-0.633187649970563,
123.830314858198));
#273690=CARTESIAN_POINT('Ctrl Pts',(-161.42742569045,-6.20971560387352,
127.567437236815));
#273691=CARTESIAN_POINT('Ctrl Pts',(-161.705873314263,-6.07981827928859,
134.279134069845));
#273692=CARTESIAN_POINT('Ctrl Pts',(-161.984320938076,-0.362864971672915,
137.79768385235));
#273693=CARTESIAN_POINT('Ctrl Pts',(-162.262768561889,5.68754351797111,
134.889711224922));
#273694=CARTESIAN_POINT('Ctrl Pts',(-162.541216185702,6.5113773665471,128.227500969805));
#273695=CARTESIAN_POINT('Ctrl Pts',(-162.819663809515,1.35157351373451,
123.93329884439));
#273696=CARTESIAN_POINT('Ctrl Pts',(-163.098111433328,-5.05026037016286,
125.953266818493));
#273697=CARTESIAN_POINT('Ctrl Pts',(-163.376559057141,-6.81115169281603,
132.431153004838));
#273698=CARTESIAN_POINT('Ctrl Pts',(-163.655006680953,-2.31292735302948,
137.414096460505));
#273699=CARTESIAN_POINT('Ctrl Pts',(-163.933454304766,4.31076423140788,
136.323015580059));
#273700=CARTESIAN_POINT('Ctrl Pts',(-164.211901928579,6.97307407972212,
130.160560390364));
#273701=CARTESIAN_POINT('Ctrl Pts',(-164.490349552392,3.2274695023783,124.589726158078));
#273702=CARTESIAN_POINT('Ctrl Pts',(-164.768797176205,-3.4840218770001,
124.729837392289));
#273703=CARTESIAN_POINT('Ctrl Pts',(-165.047244800018,-6.99386735534677,
130.452138713572));
#273704=CARTESIAN_POINT('Ctrl Pts',(-165.325692423831,-4.07669040354407,
136.498114757629));
#273705=CARTESIAN_POINT('Ctrl Pts',(-165.604140047644,2.58676587171747,
137.31180890232));
#273706=CARTESIAN_POINT('Ctrl Pts',(-165.882587671457,6.87311068140868,
132.145475979844));
#273707=CARTESIAN_POINT('Ctrl Pts',(-166.161035295269,4.84340254500906,
125.746723556562));
#273708=CARTESIAN_POINT('Ctrl Pts',(-166.439482919082,-1.63715591688565,
123.995692513036));
#273709=CARTESIAN_POINT('Ctrl Pts',(-166.717930542895,-6.61324807067504,
128.501494835643));
#273710=CARTESIAN_POINT('Ctrl Pts',(-166.996378166708,-5.5120883226436,
135.12351831059));
#273711=CARTESIAN_POINT('Ctrl Pts',(-167.274825790521,0.654411313413328,
137.776446868231));
#273712=CARTESIAN_POINT('Ctrl Pts',(-167.553273414334,6.21953892221278,
134.022368766858));
#273713=CARTESIAN_POINT('Ctrl Pts',(-167.831721038147,6.06921410286677,
127.311098384725));
#273714=CARTESIAN_POINT('Ctrl Pts',(-168.11016866196,0.3415780205785,123.809965339223));
#273715=CARTESIAN_POINT('Ctrl Pts',(-168.388616285773,-5.69995157560742,
126.736339859314));
#273716=CARTESIAN_POINT('Ctrl Pts',(-168.667063909585,-6.50350413192509,
133.401026722375));
#273717=CARTESIAN_POINT('Ctrl Pts',(-168.945511533399,-1.33065410484337,
137.679504289309));
#273718=CARTESIAN_POINT('Ctrl Pts',(-169.223959157211,5.06500203852252,
135.640060691349));
#273719=CARTESIAN_POINT('Ctrl Pts',(-169.502406781024,6.80616874759175,
129.156844962666));
#273720=CARTESIAN_POINT('Ctrl Pts',(-169.780854404837,2.29279887745254,
124.18761563522));
#273721=CARTESIAN_POINT('Ctrl Pts',(-170.05930202865,-4.32754115161411,
125.298851700587));
#273722=CARTESIAN_POINT('Ctrl Pts',(-170.337749652463,-6.97108227448498,
131.469381501595));
#273723=CARTESIAN_POINT('Ctrl Pts',(-170.616197276276,-3.20853934340632,
137.028789598255));
#273724=CARTESIAN_POINT('Ctrl Pts',(-170.894644900089,3.50249449840198,
136.868251541923));
#273725=CARTESIAN_POINT('Ctrl Pts',(-171.173092523901,6.99490700254731,
131.135293963646));
#273726=CARTESIAN_POINT('Ctrl Pts',(-171.451540147715,4.05934169155642,
125.098224807315));
#273727=CARTESIAN_POINT('Ctrl Pts',(-171.729987771527,-2.60656032410858,
124.304815700371));
#273728=CARTESIAN_POINT('Ctrl Pts',(-172.00843539534,-6.87716073946864,
129.484170851909));
#273729=CARTESIAN_POINT('Ctrl Pts',(-172.286883019153,-4.82798640323697,
135.876715903229));
#273730=CARTESIAN_POINT('Ctrl Pts',(-172.565330642966,1.65787157732142,
137.608014245356));
#273731=CARTESIAN_POINT('Ctrl Pts',(-172.843778266779,6.62022656985093,
133.087087280501));
#273732=CARTESIAN_POINT('Ctrl Pts',(-173.122225890592,5.49891676073447,
126.468446029806));
#273733=CARTESIAN_POINT('Ctrl Pts',(-173.400673514405,-0.675628914478315,
123.834298464058));
#273734=CARTESIAN_POINT('Ctrl Pts',(-173.679121138218,-6.22930462359329,
127.605297510917));
#273735=CARTESIAN_POINT('Ctrl Pts',(-173.95756876203,-6.05855370207473,
134.316079269865));
#273736=CARTESIAN_POINT('Ctrl Pts',(-174.236016385844,-0.320287905152608,
137.799763144343));
#273737=CARTESIAN_POINT('Ctrl Pts',(-174.514464009656,5.71230682967103,
134.855013841124));
#273738=CARTESIAN_POINT('Ctrl Pts',(-174.792911633469,6.49557064972945,
128.187912110866));
#273739=CARTESIAN_POINT('Ctrl Pts',(-175.071359257282,1.30972236895365,
123.925198737649));
#273740=CARTESIAN_POINT('Ctrl Pts',(-175.349806881095,-5.07969678539539,
125.984099066334));
#273741=CARTESIAN_POINT('Ctrl Pts',(-175.628254504908,-6.80112275095037,
132.472584277733));
#273742=CARTESIAN_POINT('Ctrl Pts',(-175.906702128721,-2.27264916169912,
137.428053442694));
#273743=CARTESIAN_POINT('Ctrl Pts',(-176.185149752534,4.34427798206938,
136.296672486746));
#273744=CARTESIAN_POINT('Ctrl Pts',(-176.463597376347,6.96902589009458,
130.118125237372));
#273745=CARTESIAN_POINT('Ctrl Pts',(-176.742045000159,3.18957946096438,
124.570194777934));
#273746=CARTESIAN_POINT('Ctrl Pts',(-177.020492623972,-3.52093467317244,
124.751158169184));
#273747=CARTESIAN_POINT('Ctrl Pts',(-177.298940247785,-6.99588184988549,
130.494718895118));
#273748=CARTESIAN_POINT('Ctrl Pts',(-177.577387871598,-4.04195537438161,
136.522825237142));
#273749=CARTESIAN_POINT('Ctrl Pts',(-177.855835495411,2.62633062968132,
137.295941956302));
#273750=CARTESIAN_POINT('Ctrl Pts',(-178.134283119224,6.88114708845103,
132.103612556543));
#273751=CARTESIAN_POINT('Ctrl Pts',(-178.412730743037,4.81252553565828,
125.717334096849));
#273752=CARTESIAN_POINT('Ctrl Pts',(-178.69117836685,-1.67857187946192,
124.005784494632));
#273753=CARTESIAN_POINT('Ctrl Pts',(-178.969625990663,-6.62714374015151,
128.541794220484));
#273754=CARTESIAN_POINT('Ctrl Pts',(-179.248073614475,-5.48569425761253,
135.15699193274));
#273755=CARTESIAN_POINT('Ctrl Pts',(-179.526521238288,0.696840256609583,
137.772334104211));
#273756=CARTESIAN_POINT('Ctrl Pts',(-179.804968862101,6.23901261754625,
133.984449045885));
#273757=CARTESIAN_POINT('Ctrl Pts',(-180.083416485914,6.0478371756692,127.27421807789));
#273758=CARTESIAN_POINT('Ctrl Pts',(-180.361864109727,0.298994822622653,
123.808015646805));
#273759=CARTESIAN_POINT('Ctrl Pts',(-180.64031173354,-5.72460916570447,
126.771112453397));
#273760=CARTESIAN_POINT('Ctrl Pts',(-180.918759357353,-6.48757699345442,
133.440567287733));
#273761=CARTESIAN_POINT('Ctrl Pts',(-181.197206981166,-1.28877849997557,
137.687476978041));
#273762=CARTESIAN_POINT('Ctrl Pts',(-181.475654604978,5.094344474651,135.609138992));
#273763=CARTESIAN_POINT('Ctrl Pts',(-181.754102228792,6.79601374963652,
129.115444406326));
#273764=CARTESIAN_POINT('Ctrl Pts',(-182.032549852604,2.25247839243521,
124.173781310638));
#273765=CARTESIAN_POINT('Ctrl Pts',(-182.310997476417,-4.36097456772779,
125.32529667621));
#273766=CARTESIAN_POINT('Ctrl Pts',(-182.58944510023,-6.96690494559973,
131.511804136733));
#273767=CARTESIAN_POINT('Ctrl Pts',(-182.867892724043,-3.17059003069381,
137.048205563678));
#273768=CARTESIAN_POINT('Ctrl Pts',(-183.146340347856,3.53934223048593,
136.84681851393));
#273769=CARTESIAN_POINT('Ctrl Pts',(-183.424787971669,6.99679188832936,
131.092707847901));
#273770=CARTESIAN_POINT('Ctrl Pts',(-183.703235595482,4.02453161308464,
125.07362016374));
#273771=CARTESIAN_POINT('Ctrl Pts',(-183.981683219295,-2.64607660528548,
124.320802994409));
#273772=CARTESIAN_POINT('Ctrl Pts',(-184.260130843107,-6.88506969142675,
129.52605854136));
#273773=CARTESIAN_POINT('Ctrl Pts',(-184.53857846692,-4.79702008550057,
135.906011247817));
#273774=CARTESIAN_POINT('Ctrl Pts',(-184.817026090733,1.6992566315413,137.597796254561));
#273775=CARTESIAN_POINT('Ctrl Pts',(-185.095473714546,6.63399951749853,
133.046745788687));
#273776=CARTESIAN_POINT('Ctrl Pts',(-185.373921338359,5.47242093576752,
126.435052897159));
#273777=CARTESIAN_POINT('Ctrl Pts',(-185.652368962172,-0.718045143308166,
123.838540348135));
#273778=CARTESIAN_POINT('Ctrl Pts',(-185.930816585985,-6.24866281413942,
127.64327632748));
#273779=CARTESIAN_POINT('Ctrl Pts',(-186.209264209798,-6.03706462292539,
134.35289434186));
#273780=CARTESIAN_POINT('Ctrl Pts',(-186.487711833611,-0.277698970246197,
137.801583219124));
#273781=CARTESIAN_POINT('Ctrl Pts',(-186.766159457423,5.73685846974069,
134.820166358884));
#273782=CARTESIAN_POINT('Ctrl Pts',(-187.044607081237,6.47952323715255,
128.148420205389));
#273783=CARTESIAN_POINT('Ctrl Pts',(-187.323054705049,1.2678226919294,123.917353540782));
#273784=CARTESIAN_POINT('Ctrl Pts',(-187.601502328862,-5.10894497059535,
126.01510993074));
#273785=CARTESIAN_POINT('Ctrl Pts',(-187.879949952675,-6.79084179098006,
132.513953733987));
#273786=CARTESIAN_POINT('Ctrl Pts',(-188.158397576488,-2.23228675651833,
137.44176498151));
#273787=CARTESIAN_POINT('Ctrl Pts',(-188.436845200301,4.37763075391265,
136.270125873797));
#273788=CARTESIAN_POINT('Ctrl Pts',(-188.715292824114,6.96471946064982,
130.075715513085));
#273789=CARTESIAN_POINT('Ctrl Pts',(-188.993740447926,3.15157122851057,
124.550894407098));
#273790=CARTESIAN_POINT('Ctrl Pts',(-189.27218807174,-3.55771699981564,
124.772703249722));
#273791=CARTESIAN_POINT('Ctrl Pts',(-189.550635695553,-6.99763710944952,
130.53731055055));
#273792=CARTESIAN_POINT('Ctrl Pts',(-189.829083319365,-4.00707056907658,
136.547323816845));
#273793=CARTESIAN_POINT('Ctrl Pts',(-190.107530943179,2.66579806799723,
137.279834462351));
#273794=CARTESIAN_POINT('Ctrl Pts',(-190.385978566991,6.88892851205765,
132.061700988983));
#273795=CARTESIAN_POINT('Ctrl Pts',(-190.664426190804,4.78147019640398,
125.688133138775));
#273796=CARTESIAN_POINT('Ctrl Pts',(-190.942873814617,-1.71992564193992,
124.016128399968));
#273797=CARTESIAN_POINT('Ctrl Pts',(-191.22132143843,-6.64079383837953,
128.582177445553));
#273798=CARTESIAN_POINT('Ctrl Pts',(-191.499769062243,-5.45909691816341,
135.190304266535));
#273799=CARTESIAN_POINT('Ctrl Pts',(-191.778216686055,0.739243378134395,
137.767963139373));
#273800=CARTESIAN_POINT('Ctrl Pts',(-192.056664309869,6.25825512397307,
133.946411485565));
#273801=CARTESIAN_POINT('Ctrl Pts',(-192.335111933681,6.0262361436405,127.237468581785));
#273802=CARTESIAN_POINT('Ctrl Pts',(-192.613559557494,0.256400545303713,
123.806325206523));
#273803=CARTESIAN_POINT('Ctrl Pts',(-192.892007181307,-5.74905462830365,
126.806034500975));
#273804=CARTESIAN_POINT('Ctrl Pts',(-193.17045480512,-6.47140945543246,
133.480010167483));
#273805=CARTESIAN_POINT('Ctrl Pts',(-193.448902428933,-1.24685513894648,
137.695194610365));
#273806=CARTESIAN_POINT('Ctrl Pts',(-193.727350052746,5.12349813797151,
135.578039249819));
#273807=CARTESIAN_POINT('Ctrl Pts',(-194.005797676559,6.78560692289256,
129.074106433399));
#273808=CARTESIAN_POINT('Ctrl Pts',(-194.284245300372,2.2120744410027,124.160192684611));
#273809=CARTESIAN_POINT('Ctrl Pts',(-194.562692924184,-4.39424638632456,
125.35194468056));
#273810=CARTESIAN_POINT('Ctrl Pts',(-194.841140547997,-6.9624694554897,
131.554200557291));
#273811=CARTESIAN_POINT('Ctrl Pts',(-195.11958817181,-3.13252323060231,
137.067390161131));
#273812=CARTESIAN_POINT('Ctrl Pts',(-195.398035795623,3.57605881094196,
136.825161580438));
#273813=CARTESIAN_POINT('Ctrl Pts',(-195.676483419436,6.99841750541489,
131.050111047343));
#273814=CARTESIAN_POINT('Ctrl Pts',(-195.954931043249,3.98957240411393,
125.04922787486));
#273815=CARTESIAN_POINT('Ctrl Pts',(-196.233378667062,-2.68549483512068,
124.337030539057));
#273816=CARTESIAN_POINT('Ctrl Pts',(-196.511826290875,-6.89272351459547,
129.567993598765));
#273817=CARTESIAN_POINT('Ctrl Pts',(-196.790273914688,-4.76587601242081,
135.935117548864));
#273818=CARTESIAN_POINT('Ctrl Pts',(-197.0687215385,1.74057871918182,137.58732653051));
#273819=CARTESIAN_POINT('Ctrl Pts',(-197.347169162313,6.64752663985393,
133.006321204467));
#273820=CARTESIAN_POINT('Ctrl Pts',(-197.625616786126,5.44572232823074,
126.401821670817));
#273821=CARTESIAN_POINT('Ctrl Pts',(-197.904064409939,-0.760434764710735,
123.843040353244));
#273822=CARTESIAN_POINT('Ctrl Pts',(-198.182512033752,-6.26778945818702,
127.681372279183));
#273823=CARTESIAN_POINT('Ctrl Pts',(-198.460959657565,-6.01535183812634,
134.389577921633));
#273824=CARTESIAN_POINT('Ctrl Pts',(-198.739407281378,-0.235099745102313,
137.803144009248));
#273825=CARTESIAN_POINT('Ctrl Pts',(-199.017854905191,5.76119752841001,
134.785170069484));
#273826=CARTESIAN_POINT('Ctrl Pts',(-199.296302529004,6.46323572345932,
128.10902671676));
#273827=CARTESIAN_POINT('Ctrl Pts',(-199.574750152817,1.22587603526843,
123.909763544495));
#273828=CARTESIAN_POINT('Ctrl Pts',(-199.853197776629,-5.13800384196074,
126.04629826259));
#273829=CARTESIAN_POINT('Ctrl Pts',(-200.131645400443,-6.78030919386985,
132.555259840639));
#273830=CARTESIAN_POINT('Ctrl Pts',(-200.410093024255,-2.19184163313082,
137.455230568865));
#273831=CARTESIAN_POINT('Ctrl Pts',(-200.688540648069,4.41082131103843,
136.243376724908));
#273832=CARTESIAN_POINT('Ctrl Pts',(-200.96698827188,6.96015495096418,130.03333278901));
#273833=CARTESIAN_POINT('Ctrl Pts',(-201.245435895694,3.11344621342587,
124.531825760752));
#273834=CARTESIAN_POINT('Ctrl Pts',(-201.523883519507,-3.59436749394705,
124.794471835542));
#273835=CARTESIAN_POINT('Ctrl Pts',(-201.80233114332,-6.99913306899709,
130.579912101622));
#273836=CARTESIAN_POINT('Ctrl Pts',(-202.080778767133,-3.97203728029775,
136.571609588935));
#273837=CARTESIAN_POINT('Ctrl Pts',(-202.359226390945,2.705166724186,137.263487017335));
#273838=CARTESIAN_POINT('Ctrl Pts',(-202.637674014758,6.89645466388467,
132.019742830214));
#273839=CARTESIAN_POINT('Ctrl Pts',(-202.916121638571,4.75023767801316,
125.659121764391));
#273840=CARTESIAN_POINT('Ctrl Pts',(-203.194569262384,-1.76121567194074,
124.026723845744));
#273841=CARTESIAN_POINT('Ctrl Pts',(-203.473016886197,-6.65419785954973,
128.622643014438));
#273842=CARTESIAN_POINT('Ctrl Pts',(-203.75146451001,-5.43229728987039,
135.223454077576));
#273843=CARTESIAN_POINT('Ctrl Pts',(-204.029912133822,0.781619106723946,
137.763334135682));
#273844=CARTESIAN_POINT('Ctrl Pts',(-204.308359757636,6.27726572845484,
133.908257495395));
#273845=CARTESIAN_POINT('Ctrl Pts',(-204.586807381448,6.00441180721532,
127.200851258176));
#273846=CARTESIAN_POINT('Ctrl Pts',(-204.865255005262,0.213796766968775,
123.804894081017));
#273847=CARTESIAN_POINT('Ctrl Pts',(-205.143702629074,-5.77328705756903,
126.841104707996));
#273848=CARTESIAN_POINT('Ctrl Pts',(-205.422150252887,-6.4550021169537,
133.519353900054));
#273849=CARTESIAN_POINT('Ctrl Pts',(-205.7005978767,-1.20488557524167,137.702656900301));
#273850=CARTESIAN_POINT('Ctrl Pts',(-205.979045500513,5.15246194818434,
135.546762617222));
#273851=CARTESIAN_POINT('Ctrl Pts',(-206.257493124326,6.77494865298866,
129.032832575676));
#273852=CARTESIAN_POINT('Ctrl Pts',(-206.535940748139,2.17158852033829,
124.14685026067));
#273853=CARTESIAN_POINT('Ctrl Pts',(-206.814388371952,-4.42735537450605,
125.378794726189));
#273854=CARTESIAN_POINT('Ctrl Pts',(-207.092835995765,-6.9577759685135,
131.596569192254));
#273855=CARTESIAN_POINT('Ctrl Pts',(-207.371283619578,-3.09434035370993,
137.086342679721));
#273856=CARTESIAN_POINT('Ctrl Pts',(-207.64973124339,3.61264287922363,136.803281543952));
#273857=CARTESIAN_POINT('Ctrl Pts',(-207.928178867203,6.99978379356611,
131.007505140413));
#273858=CARTESIAN_POINT('Ctrl Pts',(-208.206626491016,3.95446536007061,
125.025048844539));
#273859=CARTESIAN_POINT('Ctrl Pts',(-208.485074114829,-2.72481355295718,
124.353497733001));
#273860=CARTESIAN_POINT('Ctrl Pts',(-208.763521738642,-6.90012192535954,
129.609974470206));
#273861=CARTESIAN_POINT('Ctrl Pts',(-209.041969362455,-4.73455533805275,
135.964033727826));
#273862=CARTESIAN_POINT('Ctrl Pts',(-209.320416986268,1.78183630903778,
137.576605461163));
#273863=CARTESIAN_POINT('Ctrl Pts',(-209.598864610081,6.66080743566547,
132.965815025787));
#273864=CARTESIAN_POINT('Ctrl Pts',(-209.877312233893,5.41882192745001,
126.368753582173));
#273865=CARTESIAN_POINT('Ctrl Pts',(-210.155759857706,-0.802796207923886,
123.847798312635));
#273866=CARTESIAN_POINT('Ctrl Pts',(-210.434207481519,-6.28668384699127,
127.719583954367));
#273867=CARTESIAN_POINT('Ctrl Pts',(-210.712655105332,-5.99341615225276,
134.42612864986));
#273868=CARTESIAN_POINT('Ctrl Pts',(-210.991102729145,-0.19249180825093,
137.804445456879));
#273869=CARTESIAN_POINT('Ctrl Pts',(-211.269550352958,5.78532310378624,
134.750026269725));
#273870=CARTESIAN_POINT('Ctrl Pts',(-211.547997976771,6.44670871218949,
128.069733104719));
#273871=CARTESIAN_POINT('Ctrl Pts',(-211.826445600584,1.18388395332015,
123.902429030038));
#273872=CARTESIAN_POINT('Ctrl Pts',(-212.104893224396,-5.16687232270428,
126.077662906191));
#273873=CARTESIAN_POINT('Ctrl Pts',(-212.38334084821,-6.76952534990887,
132.596501067076));
#273874=CARTESIAN_POINT('Ctrl Pts',(-212.661788472022,-2.15131529024619,
137.468449705789));
#273875=CARTESIAN_POINT('Ctrl Pts',(-212.940236095835,4.44384842355829,
136.216426031276));
#273876=CARTESIAN_POINT('Ctrl Pts',(-213.218683719648,6.95533253017721,
129.990978635656));
#273877=CARTESIAN_POINT('Ctrl Pts',(-213.497131343461,3.0752058284468,124.512989545492));
#273878=CARTESIAN_POINT('Ctrl Pts',(-213.775578967274,-3.63088479746918,
124.81646312));
#273879=CARTESIAN_POINT('Ctrl Pts',(-214.054026591087,-7.00036967309483,
130.622521969716));
#273880=CARTESIAN_POINT('Ctrl Pts',(-214.3324742149,-3.93685680621679,136.595681653493));
#273881=CARTESIAN_POINT('Ctrl Pts',(-214.610921838713,2.74443513942699,
137.246900227015));
#273882=CARTESIAN_POINT('Ctrl Pts',(-214.889369462525,6.90372526504794,
131.977739635008));
#273883=CARTESIAN_POINT('Ctrl Pts',(-215.167817086339,4.71882913781829,
125.630301048724));
#273884=CARTESIAN_POINT('Ctrl Pts',(-215.446264710151,-1.80244043944716,
124.037570439344));
#273885=CARTESIAN_POINT('Ctrl Pts',(-215.724712333964,-6.66735530697114,
128.66318942767));
#273886=CARTESIAN_POINT('Ctrl Pts',(-216.003159957777,-5.40529636580357,
135.256440137483));
#273887=CARTESIAN_POINT('Ctrl Pts',(-216.28160758159,0.823965872130078,
137.758447264668));
#273888=CARTESIAN_POINT('Ctrl Pts',(-216.560055205403,6.29604372654653,
133.869988489185));
#273889=CARTESIAN_POINT('Ctrl Pts',(-216.838502829216,5.98236497510254,
127.164367463932));
#273890=CARTESIAN_POINT('Ctrl Pts',(-217.116950453029,0.171185066315507,
123.803722323317));
#273891=CARTESIAN_POINT('Ctrl Pts',(-217.395398076842,-5.79730555555969,
126.876321774922));
#273892=CARTESIAN_POINT('Ctrl Pts',(-217.673845700654,-6.43835558599724,
133.558597027552));
#273893=CARTESIAN_POINT('Ctrl Pts',(-217.952293324468,-1.16287136405879,
137.709863571333));
#273894=CARTESIAN_POINT('Ctrl Pts',(-218.23074094828,5.18123483202488,135.515310253174));
#273895=CARTESIAN_POINT('Ctrl Pts',(-218.509188572093,6.76403933487094,
128.991624362576));
#273896=CARTESIAN_POINT('Ctrl Pts',(-218.787636195906,2.13102213066266,
124.133754533223));
#273897=CARTESIAN_POINT('Ctrl Pts',(-219.066083819719,-4.46030030540597,
125.405845818157));
#273898=CARTESIAN_POINT('Ctrl Pts',(-219.344531443532,-6.95282465859006,
131.638908471637));
#273899=CARTESIAN_POINT('Ctrl Pts',(-219.622979067345,-3.0560428148978,
137.105062417155));
#273900=CARTESIAN_POINT('Ctrl Pts',(-219.901426691158,3.6490930796943,136.781179215245));
#273901=CARTESIAN_POINT('Ctrl Pts',(-220.179874314971,7.00089070215466,
130.964891705888));
#273902=CARTESIAN_POINT('Ctrl Pts',(-220.458321938783,3.91921178185968,
125.001083968743));
#273903=CARTESIAN_POINT('Ctrl Pts',(-220.736769562596,-2.76403130182543,
124.370203966041));
#273904=CARTESIAN_POINT('Ctrl Pts',(-221.015217186409,-6.90726464956813,
129.651999600063));
#273905=CARTESIAN_POINT('Ctrl Pts',(-221.293664810222,-4.7030592229955,
135.992758713204));
#273906=CARTESIAN_POINT('Ctrl Pts',(-221.572112434035,1.82302787229404,
137.565633443793));
#273907=CARTESIAN_POINT('Ctrl Pts',(-221.850560057848,6.67384141280798,
132.925228753618));
#273908=CARTESIAN_POINT('Ctrl Pts',(-222.129007681661,5.39172073022998,
126.33584985658));
#273909=CARTESIAN_POINT('Ctrl Pts',(-222.407455305474,-0.845127903228338,
123.85281405));
#273910=CARTESIAN_POINT('Ctrl Pts',(-222.685902929286,-6.30534528041361,
127.757909937084));
#273911=CARTESIAN_POINT('Ctrl Pts',(-222.964350553099,-5.9712583781396,
134.462545172141));
#273912=CARTESIAN_POINT('Ctrl Pts',(-223.242798176912,-0.14987673854478,
137.805487513793));
#273913=CARTESIAN_POINT('Ctrl Pts',(-223.521245800725,5.80923430188729,
134.714736261875));
#273914=CARTESIAN_POINT('Ctrl Pts',(-223.799693424538,6.42994281575757,
128.030540825308));
#273915=CARTESIAN_POINT('Ctrl Pts',(-224.078141048351,1.1418480021166,123.895350269195));
#273916=CARTESIAN_POINT('Ctrl Pts',(-224.356588672164,-5.19554934309376,
126.109202699315));
#273917=CARTESIAN_POINT('Ctrl Pts',(-224.635036295977,-6.75849065869668,
132.637675885092));
#273918=CARTESIAN_POINT('Ctrl Pts',(-224.913483919789,-2.11070922958169,
137.481421902441));
#273919=CARTESIAN_POINT('Ctrl Pts',(-225.191931543603,4.47671086764076,
136.189274791569));
#273920=CARTESIAN_POINT('Ctrl Pts',(-225.470379167415,6.95025237698553,
129.948654622468));
#273921=CARTESIAN_POINT('Ctrl Pts',(-225.748826791228,3.03685149058481,
124.494386459301));
#273922=CARTESIAN_POINT('Ctrl Pts',(-226.027274415041,-3.66726755721984,
124.838676288203));
#273923=CARTESIAN_POINT('Ctrl Pts',(-226.305722038854,-7.00134687591997,
130.665138575908));
#273924=CARTESIAN_POINT('Ctrl Pts',(-226.584169662667,-3.9015304504591,
136.619539118521));
#273925=CARTESIAN_POINT('Ctrl Pts',(-226.86261728648,2.78360185861461,137.230074706019));
#273926=CARTESIAN_POINT('Ctrl Pts',(-227.141064910293,6.91074004613266,
131.935692959814));
#273927=CARTESIAN_POINT('Ctrl Pts',(-227.419512534106,4.68724573967455,
125.601672059739));
#273928=CARTESIAN_POINT('Ctrl Pts',(-227.697960157918,-1.8435984168596,
124.048667778841));
#273929=CARTESIAN_POINT('Ctrl Pts',(-227.976407781732,-6.68026569308986,
128.703815182788));
#273930=CARTESIAN_POINT('Ctrl Pts',(-228.254855405544,-5.37809514649209,
135.289261223946));
#273931=CARTESIAN_POINT('Ctrl Pts',(-228.533303029357,0.86628210517778,
137.753302707416));
#273932=CARTESIAN_POINT('Ctrl Pts',(-228.81175065317,6.31458842242258,133.831605885006));
#273933=CARTESIAN_POINT('Ctrl Pts',(-229.090198276983,5.96009646425557,
127.128018550972));
#273934=CARTESIAN_POINT('Ctrl Pts',(-229.368645900796,0.128567022336676,
123.802809976843));
#273935=CARTESIAN_POINT('Ctrl Pts',(-229.647093524609,-5.82110923226107,
126.911684396774));
#273936=CARTESIAN_POINT('Ctrl Pts',(-229.925541148421,-6.42147047940683,
133.597738095807));
#273937=CARTESIAN_POINT('Ctrl Pts',(-230.203988772235,-1.12081406224988,
137.716814356412));
#273938=CARTESIAN_POINT('Ctrl Pts',(-230.482436396047,5.20981572330331,
135.483683323156));
#273939=CARTESIAN_POINT('Ctrl Pts',(-230.76088401986,6.75287937278817,128.950483321085));
#273940=CARTESIAN_POINT('Ctrl Pts',(-231.039331643673,2.0903767751783,124.120905987538));
#273941=CARTESIAN_POINT('Ctrl Pts',(-231.317779267486,-4.49307995823781,
125.433096954076));
#273942=CARTESIAN_POINT('Ctrl Pts',(-231.596226891299,-6.94761570919197,
131.681216826544));
#273943=CARTESIAN_POINT('Ctrl Pts',(-231.874674515112,-3.01763203329532,
137.123548679767));
#273944=CARTESIAN_POINT('Ctrl Pts',(-232.153122138925,3.68540806167951,
136.758855413326));
#273945=CARTESIAN_POINT('Ctrl Pts',(-232.431569762738,7.00173819016367,
130.922272322824));
#273946=CARTESIAN_POINT('Ctrl Pts',(-232.71001738655,3.88381297581431,124.977334135496));
#273947=CARTESIAN_POINT('Ctrl Pts',(-232.988465010364,-2.80314662849731,
124.38714861912));
#273948=CARTESIAN_POINT('Ctrl Pts',(-233.266912634176,-6.914151422545,129.694067431082));
#273949=CARTESIAN_POINT('Ctrl Pts',(-233.545360257989,-4.67138883434919,
136.021291440583));
#273950=CARTESIAN_POINT('Ctrl Pts',(-233.823807881803,1.86415188258208,
137.554410884971));
#273951=CARTESIAN_POINT('Ctrl Pts',(-234.102255505615,6.68662808830262,
132.884563891901));
#273952=CARTESIAN_POINT('Ctrl Pts',(-234.380703129428,5.36441974081549,
126.303111713297));
#273953=CARTESIAN_POINT('Ctrl Pts',(-234.659150753241,-0.887428282007554,
123.858087379481));
#273954=CARTESIAN_POINT('Ctrl Pts',(-234.937598377053,-6.32377306694735,
127.796348807152));
#273955=CARTESIAN_POINT('Ctrl Pts',(-235.216046000867,-5.94887933685163,
134.498826139047));
#273956=CARTESIAN_POINT('Ctrl Pts',(-235.494493624679,-0.107256115101469,
137.806270141374));
#273957=CARTESIAN_POINT('Ctrl Pts',(-235.772941248493,5.83293023667497,
134.679301353618));
#273958=CARTESIAN_POINT('Ctrl Pts',(-236.051388872305,6.41293865542997,
127.991451330808));
#273959=CARTESIAN_POINT('Ctrl Pts',(-236.329836496118,1.09976973931543,
123.88852752427));
#273960=CARTESIAN_POINT('Ctrl Pts',(-236.608284119931,-5.22403384049169,
126.140916473241));
#273961=CARTESIAN_POINT('Ctrl Pts',(-236.886731743744,-6.7472055291277,
132.678782768935));
#273962=CARTESIAN_POINT('Ctrl Pts',(-237.165179367557,-2.07002495581049,
137.494146678133));
#273963=CARTESIAN_POINT('Ctrl Pts',(-237.44362699137,4.50940742555574,136.161924011888));
#273964=CARTESIAN_POINT('Ctrl Pts',(-237.722074615182,6.94491467963605,
129.906362317783));
#273965=CARTESIAN_POINT('Ctrl Pts',(-238.000522238996,2.99838462107406,
124.476017191522));
#273966=CARTESIAN_POINT('Ctrl Pts',(-238.278969862808,-3.70351442502255,
124.861110517033));
#273967=CARTESIAN_POINT('Ctrl Pts',(-238.557417486622,-7.00206464126185,
130.707760341024));
#273968=CARTESIAN_POINT('Ctrl Pts',(-238.835865110434,-3.86605952205578,
136.64318109997));
#273969=CARTESIAN_POINT('Ctrl Pts',(-239.114312734247,2.82266543041169,
137.213011077826));
#273970=CARTESIAN_POINT('Ctrl Pts',(-239.39276035806,6.91749874720356,131.893604362681));
#273971=CARTESIAN_POINT('Ctrl Pts',(-239.671207981873,4.655488653916,125.573235858291));
#273972=CARTESIAN_POINT('Ctrl Pts',(-239.949655605686,-1.88468807905538,
124.060015453022));
#273973=CARTESIAN_POINT('Ctrl Pts',(-240.228103229498,-6.69292853950653,
128.74451877439));
#273974=CARTESIAN_POINT('Ctrl Pts',(-240.506550853312,-5.35069463988719,
135.321916120768));
#273975=CARTESIAN_POINT('Ctrl Pts',(-240.784998477124,0.908566237823527,
137.747900654559));
#273976=CARTESIAN_POINT('Ctrl Pts',(-241.063446100938,6.33289912890243,
133.79311110514));
#273977=CARTESIAN_POINT('Ctrl Pts',(-241.34189372475,5.9376070998423,127.091805866219));
#273978=CARTESIAN_POINT('Ctrl Pts',(-241.620341348563,0.0859442142595387,
123.802157075403));
#273979=CARTESIAN_POINT('Ctrl Pts',(-241.898788972376,-5.84469720561911,
126.947191263173));
#273980=CARTESIAN_POINT('Ctrl Pts',(-242.177236596189,-6.40434742286629,
133.636775654432));
#273981=CARTESIAN_POINT('Ctrl Pts',(-242.455684220002,-1.07871522826414,
137.723508997977));
#273982=CARTESIAN_POINT('Ctrl Pts',(-242.734131843815,5.23820356294377,
135.451882999115));
#273983=CARTESIAN_POINT('Ctrl Pts',(-243.012579467628,6.74146918027728,
128.909410975699));
#273984=CARTESIAN_POINT('Ctrl Pts',(-243.29102709144,2.04965396001378,124.108305099723));
#273985=CARTESIAN_POINT('Ctrl Pts',(-243.569474715254,-4.52569311833944,
125.460547124147));
#273986=CARTESIAN_POINT('Ctrl Pts',(-243.847922339066,-6.94214931333881,
131.72349268922));
#273987=CARTESIAN_POINT('Ctrl Pts',(-244.12636996288,-2.9791094322281,137.141800782542));
#273988=CARTESIAN_POINT('Ctrl Pts',(-244.404817586691,3.72158647951367,
136.736310965414));
#273989=CARTESIAN_POINT('Ctrl Pts',(-244.683265210505,7.00232622618917,
130.879648570499));
#273990=CARTESIAN_POINT('Ctrl Pts',(-244.961712834317,3.84827025365086,
124.953800224859));
#273991=CARTESIAN_POINT('Ctrl Pts',(-245.240160458131,-2.84215808354001,
124.404331064352));
#273992=CARTESIAN_POINT('Ctrl Pts',(-245.518608081943,-6.92078198909823,
129.736176404423));
#273993=CARTESIAN_POINT('Ctrl Pts',(-245.797055705757,-4.63954534567172,
136.049630852671));
#273994=CARTESIAN_POINT('Ctrl Pts',(-246.075503329569,1.90520681603656,
137.542938200555));
#273995=CARTESIAN_POINT('Ctrl Pts',(-246.353950953382,6.69916698833444,
132.843821947487));
#273996=CARTESIAN_POINT('Ctrl Pts',(-246.632398577195,5.33691997085474,
126.270540365447));
#273997=CARTESIAN_POINT('Ctrl Pts',(-246.910846201008,-0.929695776805409,
123.86361810567));
#273998=CARTESIAN_POINT('Ctrl Pts',(-247.189293824821,-6.34196652374499,
127.834899140205));
#273999=CARTESIAN_POINT('Ctrl Pts',(-247.467741448634,-5.9262798576518,
134.534970206175));
#274000=CARTESIAN_POINT('Ctrl Pts',(-247.746189072447,-0.0646315172428821,
137.806793310625));
#274001=CARTESIAN_POINT('Ctrl Pts',(-248.024636696259,5.85641003008765,
134.643722858007));
#274002=CARTESIAN_POINT('Ctrl Pts',(-248.303084320073,6.39569686130214,
127.952466069697));
#274003=CARTESIAN_POINT('Ctrl Pts',(-248.581531943885,1.05765072414216,
123.881961048084));
#274004=CARTESIAN_POINT('Ctrl Pts',(-248.859979567699,-5.25232475939459,
126.172803052805));
#274005=CARTESIAN_POINT('Ctrl Pts',(-249.138427191511,-6.73567037937639,
132.719820195375));
#274006=CARTESIAN_POINT('Ctrl Pts',(-249.416874815324,-2.02926397650361,
137.506623561341));
#274007=CARTESIAN_POINT('Ctrl Pts',(-249.695322439137,4.54193688572079,
136.134374705723));
#274008=CARTESIAN_POINT('Ctrl Pts',(-249.97377006295,6.93931963591783,129.864103288757));
#274009=CARTESIAN_POINT('Ctrl Pts',(-250.252217686763,2.95980664532115,
124.457882422832));
#274010=CARTESIAN_POINT('Ctrl Pts',(-250.530665310576,-3.73962405773988,
124.883764975191));
#274011=CARTESIAN_POINT('Ctrl Pts',(-250.809112934388,-7.00252294251614,
130.750385685678));
#274012=CARTESIAN_POINT('Ctrl Pts',(-251.087560558202,-3.83044533540895,
136.666606721818));
#274013=CARTESIAN_POINT('Ctrl Pts',(-251.366008182014,2.86162440732935,
137.195709974661));
#274014=CARTESIAN_POINT('Ctrl Pts',(-251.644455805827,6.9240011177651,131.851475403357));
#274015=CARTESIAN_POINT('Ctrl Pts',(-251.92290342964,4.62355905740654,125.54499349784));
#274016=CARTESIAN_POINT('Ctrl Pts',(-252.201351053453,-1.92570790361727,
124.071613041873));
#274017=CARTESIAN_POINT('Ctrl Pts',(-252.479798677266,-6.70534337666252,
128.785298693283));
#274018=CARTESIAN_POINT('Ctrl Pts',(-252.758246301079,-5.3230958619522,
135.354403619622));
#274019=CARTESIAN_POINT('Ctrl Pts',(-253.036693924892,0.950816704398073,
137.74224130304));
#274020=CARTESIAN_POINT('Ctrl Pts',(-253.315141548704,6.35097516523885,
133.754505582129));
#274021=CARTESIAN_POINT('Ctrl Pts',(-253.593589172518,5.91489771943887,
127.055730740027));
#274022=CARTESIAN_POINT('Ctrl Pts',(-253.87203679633,0.0433182135112656,
123.801763664947));
#274023=CARTESIAN_POINT('Ctrl Pts',(-254.150484420143,-5.86806858651122,
126.982841017323));
#274024=CARTESIAN_POINT('Ctrl Pts',(-254.428932043956,-6.38698707931617,
133.675708334441));
#274025=CARTESIAN_POINT('Ctrl Pts',(-254.707379667769,-1.03657636838919,
137.729947101491));
#274026=CARTESIAN_POINT('Ctrl Pts',(-254.985827291582,5.26639719763008,
135.41991073597));
#274027=CARTESIAN_POINT('Ctrl Pts',(-255.264274915395,6.72980937160111,
128.868408326187));
#274028=CARTESIAN_POINT('Ctrl Pts',(-255.542722539208,2.00885483266244,
124.095953322692));
#274029=CARTESIAN_POINT('Ctrl Pts',(-255.821170163021,-4.5581378946222,
125.488193449449));
#274030=CARTESIAN_POINT('Ctrl Pts',(-256.099617786833,-6.93642696247006,
131.765738008466));
#274031=CARTESIAN_POINT('Ctrl Pts',(-256.378065410647,-2.94047400549736,
137.159811411449));
#274032=CARTESIAN_POINT('Ctrl Pts',(-256.656513034459,3.7576223973322,136.713559240208));
#274033=CARTESIAN_POINT('Ctrl Pts',(-256.934960658272,7.0026634652268,130.836998362911));
#274034=CARTESIAN_POINT('Ctrl Pts',(-257.213408282085,3.81256854888166,
124.930527794066));
#274035=CARTESIAN_POINT('Ctrl Pts',(-257.491855905898,-2.88103328591622,
124.421666290213));
#274036=CARTESIAN_POINT('Ctrl Pts',(-257.770303529711,-6.92721451599304,
129.778484277494));
#274037=CARTESIAN_POINT('Ctrl Pts',(-258.048751153524,-4.60741964202412,
136.077475067175));
#274038=CARTESIAN_POINT('Ctrl Pts',(-258.327198777336,1.94598288966397,
137.53178391186));
#274039=CARTESIAN_POINT('Ctrl Pts',(-258.60564640115,6.71185090883407,132.801931226644));
#274040=CARTESIAN_POINT('Ctrl Pts',(-258.884094024962,5.30847971878909,
126.240167716581));
#274041=CARTESIAN_POINT('Ctrl Pts',(-259.162541648776,-0.970525071554103,
123.86553674091));
#274042=CARTESIAN_POINT('Ctrl Pts',(-259.440989272588,-6.36258613651914,
127.881151058581));
#274043=CARTESIAN_POINT('Ctrl Pts',(-259.673028959099,-5.97575359986218,
133.442106215535));
#274044=CARTESIAN_POINT('Ctrl Pts',(-259.858689921174,-2.9628379271774,
136.206922793942));
#274045=CARTESIAN_POINT('Ctrl Pts',(-259.951535008647,-1.00384119663989,
136.721969923993));
#274046=CARTESIAN_POINT('Ctrl Pts',(-259.997972158816,-0.016740685831905,
136.724751058381));
#274047=CARTESIAN_POINT('Ctrl Pts',(210.384788400103,3.2437100417032,135.350446923363));
#274048=CARTESIAN_POINT('Ctrl Pts',(210.338370536501,4.00135710969089,134.809856772425));
#274049=CARTESIAN_POINT('Ctrl Pts',(210.245544735596,5.2274450014198,133.344996311945));
#274050=CARTESIAN_POINT('Ctrl Pts',(210.059903060087,6.03752477204218,129.574087134129));
#274051=CARTESIAN_POINT('Ctrl Pts',(209.827863373576,3.30140998082846,125.08375145776));
#274052=CARTESIAN_POINT('Ctrl Pts',(209.549415749763,-3.03864792542705,
124.935284604053));
#274053=CARTESIAN_POINT('Ctrl Pts',(209.27096812595,-6.57501826603042,130.18815040753));
#274054=CARTESIAN_POINT('Ctrl Pts',(208.992520502138,-4.0751627655632,136.003208990552));
#274055=CARTESIAN_POINT('Ctrl Pts',(208.714072878324,2.17267791003586,137.042921783734));
#274056=CARTESIAN_POINT('Ctrl Pts',(208.435625254512,6.42228832295553,132.348569225854));
#274057=CARTESIAN_POINT('Ctrl Pts',(208.157177630698,4.77100074356668,126.235763887068));
#274058=CARTESIAN_POINT('Ctrl Pts',(207.878730006886,-1.26506482749479,
124.320958291314));
#274059=CARTESIAN_POINT('Ctrl Pts',(207.600282383073,-6.13835327551471,
128.364250828182));
#274060=CARTESIAN_POINT('Ctrl Pts',(207.32183475926,-5.37092434612766,134.649796015418));
#274061=CARTESIAN_POINT('Ctrl Pts',(207.043387135447,0.332190207827403,
137.40162108792));
#274062=CARTESIAN_POINT('Ctrl Pts',(206.764939511634,5.73000189292936,134.090861108297));
#274063=CARTESIAN_POINT('Ctrl Pts',(206.486491887821,5.86224098722307,127.759980958474));
#274064=CARTESIAN_POINT('Ctrl Pts',(206.208044264008,0.607356820266201,
124.226729984437));
#274065=CARTESIAN_POINT('Ctrl Pts',(205.929596640195,-5.20565320191231,
126.738003936844));
#274066=CARTESIAN_POINT('Ctrl Pts',(205.651149016382,-6.23492509722864,
132.986059061584));
#274067=CARTESIAN_POINT('Ctrl Pts',(205.37270139257,-1.53460390898592,137.229240938669));
#274068=CARTESIAN_POINT('Ctrl Pts',(205.094253768756,4.57594250116295,135.568271122458));
#274069=CARTESIAN_POINT('Ctrl Pts',(204.815806144944,6.48142172411287,129.529500574057));
#274070=CARTESIAN_POINT('Ctrl Pts',(204.537358521131,2.43079079302514,124.662263970705));
#274071=CARTESIAN_POINT('Ctrl Pts',(204.258910897318,-3.85361800715474,
125.439314209572));
#274072=CARTESIAN_POINT('Ctrl Pts',(203.980463273505,-6.5967401814699,131.146579956944));
#274073=CARTESIAN_POINT('Ctrl Pts',(203.702015649692,-3.27778036432047,
136.539362872731));
#274074=CARTESIAN_POINT('Ctrl Pts',(203.42356802588,3.05329946149495,136.661958874297));
#274075=CARTESIAN_POINT('Ctrl Pts',(203.145120402066,6.5785462535266,131.40170824395));
#274076=CARTESIAN_POINT('Ctrl Pts',(202.866672778254,4.05843041346184,125.592524323598));
#274077=CARTESIAN_POINT('Ctrl Pts',(202.58822515444,-2.19118470860141,124.572763346851));
#274078=CARTESIAN_POINT('Ctrl Pts',(202.309777530628,-6.42720813017419,
129.279535830482));
#274079=CARTESIAN_POINT('Ctrl Pts',(202.031329906815,-4.75694126595338,
135.387547802118));
#274080=CARTESIAN_POINT('Ctrl Pts',(201.752882283002,1.28472223178851,137.283834652022));
#274081=CARTESIAN_POINT('Ctrl Pts',(201.474434659189,6.14578876089344,133.225801404307));
#274082=CARTESIAN_POINT('Ctrl Pts',(201.195987035376,5.35917565710019,126.94258236746));
#274083=CARTESIAN_POINT('Ctrl Pts',(200.917539411563,-0.352258065224466,
124.208148884143));
#274084=CARTESIAN_POINT('Ctrl Pts',(200.63909178775,-5.73998383440169,127.535311740963));
#274085=CARTESIAN_POINT('Ctrl Pts',(200.360644163938,-5.85294487354697,
133.866570813476));
#274086=CARTESIAN_POINT('Ctrl Pts',(200.082196540124,-0.587335506164227,
137.383808313225));
#274087=CARTESIAN_POINT('Ctrl Pts',(199.803748916312,5.2180064984534,134.854854804556));
#274088=CARTESIAN_POINT('Ctrl Pts',(199.525301292498,6.22825544477889,128.603695015683));
#274089=CARTESIAN_POINT('Ctrl Pts',(199.246853668687,1.51504190454761,124.374839406449));
#274090=CARTESIAN_POINT('Ctrl Pts',(198.968406044873,-4.5904211320519,126.054399690658));
#274091=CARTESIAN_POINT('Ctrl Pts',(198.689958421061,-6.47751140283473,
132.098942018204));
#274092=CARTESIAN_POINT('Ctrl Pts',(198.411510797247,-2.41208513843682,
136.95382728238));
#274093=CARTESIAN_POINT('Ctrl Pts',(198.133063173434,3.86992953127461,136.15765309974));
#274094=CARTESIAN_POINT('Ctrl Pts',(197.854615549622,6.59566801831256,130.442064648858));
#274095=CARTESIAN_POINT('Ctrl Pts',(197.576167925809,3.26030981281707,125.059408494076));
#274096=CARTESIAN_POINT('Ctrl Pts',(197.297720301996,-3.07111383566833,
124.956082684267));
#274097=CARTESIAN_POINT('Ctrl Pts',(197.019272678183,-6.58033390142619,
130.227038590899));
#274098=CARTESIAN_POINT('Ctrl Pts',(196.74082505437,-4.04254857895594,136.028525236289));
#274099=CARTESIAN_POINT('Ctrl Pts',(196.462377430557,2.21014139809766,137.029259811701));
#274100=CARTESIAN_POINT('Ctrl Pts',(196.183929806745,6.43181940170927,132.309616130935));
#274101=CARTESIAN_POINT('Ctrl Pts',(195.905482182931,4.74296958699597,126.206716169203));
#274102=CARTESIAN_POINT('Ctrl Pts',(195.627034559119,-1.30443757122094,
124.328826848098));
#274103=CARTESIAN_POINT('Ctrl Pts',(195.348586935305,-6.15313032680387,
128.401636713722));
#274104=CARTESIAN_POINT('Ctrl Pts',(195.070139311493,-5.34739690918169,
134.682432467391));
#274105=CARTESIAN_POINT('Ctrl Pts',(194.791691687679,0.372333033116476,
137.399469645412));
#274106=CARTESIAN_POINT('Ctrl Pts',(194.513244063867,5.74990710746052,134.055923815831));
#274107=CARTESIAN_POINT('Ctrl Pts',(194.234796440054,5.84359744862664,127.724350254736));
#274108=CARTESIAN_POINT('Ctrl Pts',(193.956348816241,0.567307210110782,
124.223155750211));
#274109=CARTESIAN_POINT('Ctrl Pts',(193.677901192428,-5.23031063999889,
126.769767009054));
#274110=CARTESIAN_POINT('Ctrl Pts',(193.399453568615,-6.22152852682933,
133.023972693263));
#274111=CARTESIAN_POINT('Ctrl Pts',(193.121005944802,-1.49546563606909,
137.238463313985));
#274112=CARTESIAN_POINT('Ctrl Pts',(192.84255832099,4.60485711668079,135.540327880088));
#274113=CARTESIAN_POINT('Ctrl Pts',(192.564110697177,6.47354113897745,129.490069896797));
#274114=CARTESIAN_POINT('Ctrl Pts',(192.285663073364,2.39335710461987,124.64758087922));
#274115=CARTESIAN_POINT('Ctrl Pts',(192.007215449551,-3.88620518688872,
125.462871665772));
#274116=CARTESIAN_POINT('Ctrl Pts',(191.728767825738,-6.59453476332446,
131.18672985278));
#274117=CARTESIAN_POINT('Ctrl Pts',(191.450320201925,-3.24280905319821,
136.559209392401));
#274118=CARTESIAN_POINT('Ctrl Pts',(191.171872578112,3.08889975678785,136.643264047941));
#274119=CARTESIAN_POINT('Ctrl Pts',(190.893424954299,6.58206059142805,131.361651697256));
#274120=CARTESIAN_POINT('Ctrl Pts',(190.614977330486,4.02662929408197,125.567916069518));
#274121=CARTESIAN_POINT('Ctrl Pts',(190.336529706674,-2.22907761274862,
124.586217166899));
#274122=CARTESIAN_POINT('Ctrl Pts',(190.05808208286,-6.43637108995848,129.318688322246));
#274123=CARTESIAN_POINT('Ctrl Pts',(189.779634459048,-4.72895396970476,
135.416419737866));
#274124=CARTESIAN_POINT('Ctrl Pts',(189.501186835235,1.32414082646293,137.275894133543));
#274125=CARTESIAN_POINT('Ctrl Pts',(189.222739211422,6.16041489098677,133.188345380025));
#274126=CARTESIAN_POINT('Ctrl Pts',(188.944291587609,5.33556862369218,126.910031093937));
#274127=CARTESIAN_POINT('Ctrl Pts',(188.665843963796,-0.392404551757433,
124.210415391489));
#274128=CARTESIAN_POINT('Ctrl Pts',(188.387396339983,-5.75977711417006,
127.570313219673));
#274129=CARTESIAN_POINT('Ctrl Pts',(188.10894871617,-5.83419588941534,133.902142614521));
#274130=CARTESIAN_POINT('Ctrl Pts',(187.830501092358,-0.547273658602122,
137.387261689231));
#274131=CARTESIAN_POINT('Ctrl Pts',(187.552053468544,5.24256632866185,134.823016271676));
#274132=CARTESIAN_POINT('Ctrl Pts',(187.273605844732,6.214743973489,128.565822630237));
#274133=CARTESIAN_POINT('Ctrl Pts',(186.995158220918,1.47587551380139,124.365736040492));
#274134=CARTESIAN_POINT('Ctrl Pts',(186.716710597106,-4.61925044254253,
126.082430892781));
#274135=CARTESIAN_POINT('Ctrl Pts',(186.438262973293,-6.46951090511933,
132.138348483055));
#274136=CARTESIAN_POINT('Ctrl Pts',(186.15981534948,-2.37460689906969,136.968396393875));
#274137=CARTESIAN_POINT('Ctrl Pts',(185.881367725667,3.90244484122886,136.133996556155));
#274138=CARTESIAN_POINT('Ctrl Pts',(185.602920101854,6.59334041746713,130.401921658061));
#274139=CARTESIAN_POINT('Ctrl Pts',(185.324472478041,3.22527825263932,125.039668503516));
#274140=CARTESIAN_POINT('Ctrl Pts',(185.046024854228,-3.10665706276191,
124.974885780916));
#274141=CARTESIAN_POINT('Ctrl Pts',(184.767577230416,-6.5837263061198,130.26710564752));
#274142=CARTESIAN_POINT('Ctrl Pts',(184.489129606603,-4.01067270706429,
136.05303658523));
#274143=CARTESIAN_POINT('Ctrl Pts',(184.21068198279,2.247993177529,137.015690720733));
#274144=CARTESIAN_POINT('Ctrl Pts',(183.932234358977,6.44086315254518,132.270435931769));
#274145=CARTESIAN_POINT('Ctrl Pts',(183.653786735164,4.71489454403,126.177929550814));
#274146=CARTESIAN_POINT('Ctrl Pts',(183.375339111351,-1.34383181504516,
124.33688730648));
#274147=CARTESIAN_POINT('Ctrl Pts',(183.096891487538,-6.16764238592767,
128.439137081397));
#274148=CARTESIAN_POINT('Ctrl Pts',(182.818443863726,-5.32369091022383,
134.71491173846));
#274149=CARTESIAN_POINT('Ctrl Pts',(182.539996239912,0.412472435216218,
137.397080956463));
#274150=CARTESIAN_POINT('Ctrl Pts',(182.2615486161,5.76959376309122,134.020862255314));
#274151=CARTESIAN_POINT('Ctrl Pts',(181.983100992287,5.82474028301032,127.688835683913));
#274152=CARTESIAN_POINT('Ctrl Pts',(181.704653368474,0.527235037225083,
124.219824324685));
#274153=CARTESIAN_POINT('Ctrl Pts',(181.426205744661,-5.25477345090652,
126.801680146133));
#274154=CARTESIAN_POINT('Ctrl Pts',(181.147758120848,-6.20790184760947,
133.061803779016));
#274155=CARTESIAN_POINT('Ctrl Pts',(180.869310497035,-1.45627171922457,
137.247447428754));
#274156=CARTESIAN_POINT('Ctrl Pts',(180.590862873222,4.63360097629919,135.5122090613));
#274157=CARTESIAN_POINT('Ctrl Pts',(180.31241524941,6.46542073859599,129.450687965235));
#274158=CARTESIAN_POINT('Ctrl Pts',(180.033967625596,2.35583469548556,124.633125906077));
#274159=CARTESIAN_POINT('Ctrl Pts',(179.755520001784,-3.91864834385308,
125.4866270652));
#274160=CARTESIAN_POINT('Ctrl Pts',(179.477072377971,-6.59208499180493,
131.226865573221));
#274161=CARTESIAN_POINT('Ctrl Pts',(179.198624754158,-3.20771757354326,
136.578842667508));
#274162=CARTESIAN_POINT('Ctrl Pts',(178.920177130345,3.12438558908937,136.62435285703));
#274163=CARTESIAN_POINT('Ctrl Pts',(178.641729506532,6.58533103007041,131.32157450091));
#274164=CARTESIAN_POINT('Ctrl Pts',(178.363281882719,3.99467896572256,125.5435018533));
#274165=CARTESIAN_POINT('Ctrl Pts',(178.084834258906,-2.26688791720775,
124.599901402811));
#274166=CARTESIAN_POINT('Ctrl Pts',(177.806386635093,-6.44529554785546,
129.357895865998));
#274167=CARTESIAN_POINT('Ctrl Pts',(177.527939011281,-4.70079144021631,
135.445120772143));
#274168=CARTESIAN_POINT('Ctrl Pts',(177.249491387467,1.36351035455298,137.26771380997));
#274169=CARTESIAN_POINT('Ctrl Pts',(176.971043763655,6.17481274467203,133.150801016333));
#274170=CARTESIAN_POINT('Ctrl Pts',(176.692596139842,5.31176387881016,126.877624126216));
#274171=CARTESIAN_POINT('Ctrl Pts',(176.414148516029,-0.432536497586617,
124.212926239906));
#274172=CARTESIAN_POINT('Ctrl Pts',(176.135700892216,-5.77935696328393,
127.605434537195));
#274173=CARTESIAN_POINT('Ctrl Pts',(175.857253268403,-5.81523071700703,
133.937599626117));
#274174=CARTESIAN_POINT('Ctrl Pts',(175.57880564459,-0.50719153161477,137.390471133416));
#274175=CARTESIAN_POINT('Ctrl Pts',(175.300358020777,5.2669318936477,134.791028826034));
#274176=CARTESIAN_POINT('Ctrl Pts',(175.021910396965,6.20100221257536,128.528033194638));
#274177=CARTESIAN_POINT('Ctrl Pts',(174.743462773151,1.43665443394553,124.356871260137));
#274178=CARTESIAN_POINT('Ctrl Pts',(174.465015149339,-4.64790858500931,
126.110637067746));
#274179=CARTESIAN_POINT('Ctrl Pts',(174.186567525525,-6.46127067729819,
132.177705516496));
#274180=CARTESIAN_POINT('Ctrl Pts',(173.908119901713,-2.33704066777073,
136.982737094758));
#274181=CARTESIAN_POINT('Ctrl Pts',(173.6296722779,3.93481554465429,136.11014252095));
#274182=CARTESIAN_POINT('Ctrl Pts',(173.351224654087,6.59076849796787,130.361793579788));
#274183=CARTESIAN_POINT('Ctrl Pts',(173.072777030274,3.1901271785899,125.020142125741));
#274184=CARTESIAN_POINT('Ctrl Pts',(172.794329406461,-3.14208517153551,
124.993904890899));
#274185=CARTESIAN_POINT('Ctrl Pts',(172.515881782648,-6.58687474841394,
130.30719261232));
#274186=CARTESIAN_POINT('Ctrl Pts',(172.237434158836,-3.97864821822065,
136.077353442554));
#274187=CARTESIAN_POINT('Ctrl Pts',(171.958986535022,2.28576165674636,137.001891466644));
#274188=CARTESIAN_POINT('Ctrl Pts',(171.68053891121,6.44966823482829,132.231201406644));
#274189=CARTESIAN_POINT('Ctrl Pts',(171.402091287397,4.68664478891289,126.149314366529));
#274190=CARTESIAN_POINT('Ctrl Pts',(171.123643663584,-1.38317626268716,
124.345187419464));
#274191=CARTESIAN_POINT('Ctrl Pts',(170.845196039771,-6.18192590079466,
128.476725093301));
#274192=CARTESIAN_POINT('Ctrl Pts',(170.566748415958,-5.29978763994156,
134.747246102621));
#274193=CARTESIAN_POINT('Ctrl Pts',(170.288300792145,0.452596552998033,
137.394447971839));
#274194=CARTESIAN_POINT('Ctrl Pts',(170.009853168332,5.78906662430322,133.985681506144));
#274195=CARTESIAN_POINT('Ctrl Pts',(169.73140554452,5.80566727950083,127.653436560012));
#274196=CARTESIAN_POINT('Ctrl Pts',(169.452957920706,0.487143327451347,
124.216736891574));
#274197=CARTESIAN_POINT('Ctrl Pts',(169.174510296894,-5.27904154425138,
126.833741604011));
#274198=CARTESIAN_POINT('Ctrl Pts',(168.896062673081,-6.19404513230377,
133.099551214382));
#274199=CARTESIAN_POINT('Ctrl Pts',(168.617615049268,-1.41702383969606,
137.256192792574));
#274200=CARTESIAN_POINT('Ctrl Pts',(168.339167425455,4.66217313612931,135.483915791456));
#274201=CARTESIAN_POINT('Ctrl Pts',(168.060719801642,6.45706075967145,129.411356194513));
#274202=CARTESIAN_POINT('Ctrl Pts',(167.782272177829,2.3182249900303,124.618899610305));
#274203=CARTESIAN_POINT('Ctrl Pts',(167.503824554016,-3.95094629386185,
125.510579515201));
#274204=CARTESIAN_POINT('Ctrl Pts',(167.225376930203,-6.58939094815179,
131.266985637585));
#274205=CARTESIAN_POINT('Ctrl Pts',(166.946929306391,-3.1725072307341,136.59826196706));
#274206=CARTESIAN_POINT('Ctrl Pts',(166.668481682578,3.15975564613386,136.605226004165));
#274207=CARTESIAN_POINT('Ctrl Pts',(166.390034058765,6.58835744684964,131.281478139015));
#274208=CARTESIAN_POINT('Ctrl Pts',(166.111586434952,3.96258061306513,125.519282580138));
#274209=CARTESIAN_POINT('Ctrl Pts',(165.833138811139,-2.30461422130139,
124.613815547242));
#274210=CARTESIAN_POINT('Ctrl Pts',(165.554691187326,-6.45398117295568,
129.397157009033));
#274211=CARTESIAN_POINT('Ctrl Pts',(165.276243563513,-4.67245472117232,
135.473649841348));
#274212=CARTESIAN_POINT('Ctrl Pts',(164.9977959397,1.40282935726546,137.259293984466));
#274213=CARTESIAN_POINT('Ctrl Pts',(164.719348315888,6.18898178840028,133.11316970443));
#274214=CARTESIAN_POINT('Ctrl Pts',(164.440900692075,5.2877623045642,126.845362665158));
#274215=CARTESIAN_POINT('Ctrl Pts',(164.162453068262,-0.472652415616787,
124.215681336348));
#274216=CARTESIAN_POINT('Ctrl Pts',(163.884005444449,-5.79872265620017,
127.640674392099));
#274217=CARTESIAN_POINT('Ctrl Pts',(163.605557820636,-5.79605005908598,
133.97294053439));
#274218=CARTESIAN_POINT('Ctrl Pts',(163.327110196823,-0.467090610458611,
137.393436526853));
#274219=CARTESIAN_POINT('Ctrl Pts',(163.04866257301,5.29110229053537,134.758893652935));
#274220=CARTESIAN_POINT('Ctrl Pts',(162.770214949197,6.18703067124424,128.49032810919));
#274221=CARTESIAN_POINT('Ctrl Pts',(162.491767325384,1.39738011833125,124.34824539387));
#274222=CARTESIAN_POINT('Ctrl Pts',(162.213319701571,-4.67639449751423,
126.139017170363));
#274223=CARTESIAN_POINT('Ctrl Pts',(161.934872077759,-6.45279102471594,
132.217011660137));
#274224=CARTESIAN_POINT('Ctrl Pts',(161.656424453946,-2.29938783657033,
136.996848853628));
#274225=CARTESIAN_POINT('Ctrl Pts',(161.377976830133,3.96704044204275,136.086091878046));
#274226=CARTESIAN_POINT('Ctrl Pts',(161.09952920632,6.58795235511813,130.321681900999));
#274227=CARTESIAN_POINT('Ctrl Pts',(160.821081582507,3.15485789320466,125.000830084311));
#274228=CARTESIAN_POINT('Ctrl Pts',(160.542633958694,-3.17739684918762,
125.013139309456));
#274229=CARTESIAN_POINT('Ctrl Pts',(160.264186334881,-6.58977911164196,
130.347297999864));
#274230=CARTESIAN_POINT('Ctrl Pts',(159.985738711068,-3.94647629910411,
136.10147490719));
#274231=CARTESIAN_POINT('Ctrl Pts',(159.707291087255,2.32344543622502,136.98786256077));
#274232=CARTESIAN_POINT('Ctrl Pts',(159.428843463442,6.45823432228318,132.191914009409));
#274233=CARTESIAN_POINT('Ctrl Pts',(159.15039583963,4.65822136844951,126.120871676696));
#274234=CARTESIAN_POINT('Ctrl Pts',(158.871948215817,-1.42246945622416,
124.353726879487));
#274235=CARTESIAN_POINT('Ctrl Pts',(158.593500592004,-6.19598034212407,
128.514399356595));
#274236=CARTESIAN_POINT('Ctrl Pts',(158.315052968191,-5.2756879840792,134.779434361708));
#274237=CARTESIAN_POINT('Ctrl Pts',(158.036605344378,0.49270389964821,137.391570789103));
#274238=CARTESIAN_POINT('Ctrl Pts',(157.758157720565,5.80832496952254,133.950382871961));
#274239=CARTESIAN_POINT('Ctrl Pts',(157.479710096752,5.78637914485521,127.618154194761));
#274240=CARTESIAN_POINT('Ctrl Pts',(157.201262472939,0.447033566402335,
124.213893565282));
#274241=CARTESIAN_POINT('Ctrl Pts',(156.922814849126,-5.3031140207705,126.865950194636));
#274242=CARTESIAN_POINT('Ctrl Pts',(156.644367225313,-6.17995889437779,
133.137213600617));
#274243=CARTESIAN_POINT('Ctrl Pts',(156.365919601501,-1.37772345182797,
137.264699081378));
#274244=CARTESIAN_POINT('Ctrl Pts',(156.087471977688,4.69057253741941,135.455449118975));
#274245=CARTESIAN_POINT('Ctrl Pts',(155.809024353875,6.44846151198586,129.372076042081));
#274246=CARTESIAN_POINT('Ctrl Pts',(155.530576730062,2.28052938189546,124.604902519066));
#274247=CARTESIAN_POINT('Ctrl Pts',(155.252129106249,-3.98309784010292,
125.534728128207));
#274248=CARTESIAN_POINT('Ctrl Pts',(154.973681482436,-6.58645273219382,
131.307088559209));
#274249=CARTESIAN_POINT('Ctrl Pts',(154.695233858623,-3.13717932950269,
136.617466571466));
#274250=CARTESIAN_POINT('Ctrl Pts',(154.41678623481,3.19500861727094,136.585884198101));
#274251=CARTESIAN_POINT('Ctrl Pts',(154.138338610998,6.59113972962085,131.241364097354));
#274252=CARTESIAN_POINT('Ctrl Pts',(153.859890987185,3.93033542552574,125.495259147487));
#274253=CARTESIAN_POINT('Ctrl Pts',(153.581443363372,-2.3422551270676,124.627959084596));
#274254=CARTESIAN_POINT('Ctrl Pts',(153.302995739559,-6.46242764341012,
129.436470296516));
#274255=CARTESIAN_POINT('Ctrl Pts',(153.024548115746,-4.64394486260028,
135.502005888322));
#274256=CARTESIAN_POINT('Ctrl Pts',(152.746100491933,1.44209637762021,137.250634969033));
#274257=CARTESIAN_POINT('Ctrl Pts',(152.46765286812,6.20292149713234,133.075452838754));
#274258=CARTESIAN_POINT('Ctrl Pts',(152.189205244307,5.26356479034146,126.813247906226));
#274259=CARTESIAN_POINT('Ctrl Pts',(151.910757620494,-0.512750819337957,
124.218680578724));
#274260=CARTESIAN_POINT('Ctrl Pts',(151.632309996682,-5.8178734753159,127.676031478561));
#274261=CARTESIAN_POINT('Ctrl Pts',(151.353862372869,-5.77665462639848,
134.008164029768));
#274262=CARTESIAN_POINT('Ctrl Pts',(151.075414749056,-0.4269723810881,137.39615775966));
#274263=CARTESIAN_POINT('Ctrl Pts',(150.796967125243,5.31507662368183,134.72661194316));
#274264=CARTESIAN_POINT('Ctrl Pts',(150.51851950143,6.17282986721635,128.452708771068));
#274265=CARTESIAN_POINT('Ctrl Pts',(150.240071877617,1.35805402228283,124.339858761329));
#274266=CARTESIAN_POINT('Ctrl Pts',(149.961624253804,-4.70470712450132,
126.167570148998));
#274267=CARTESIAN_POINT('Ctrl Pts',(149.683176629991,-6.44407226158927,
132.256265457474));
#274268=CARTESIAN_POINT('Ctrl Pts',(149.404729006178,-2.26164980070799,
137.010731147569));
#274269=CARTESIAN_POINT('Ctrl Pts',(149.126281382365,3.99911833928874,136.061845518646));
#274270=CARTESIAN_POINT('Ctrl Pts',(148.847833758553,6.58489209327119,130.281588108047));
#274271=CARTESIAN_POINT('Ctrl Pts',(148.56938613474,3.11947170339994,124.981733094838));
#274272=CARTESIAN_POINT('Ctrl Pts',(148.290938510927,-3.21259078723097,
125.032588323847));
#274273=CARTESIAN_POINT('Ctrl Pts',(148.012490887114,-6.59243928818165,
130.387420324031));
#274274=CARTESIAN_POINT('Ctrl Pts',(147.734043263301,-3.91415814185689,
136.125400085308));
#274275=CARTESIAN_POINT('Ctrl Pts',(147.455595639488,2.36104311957866,136.973604522958));
#274276=CARTESIAN_POINT('Ctrl Pts',(147.177148015675,6.46656109749016,132.152575195872));
#274277=CARTESIAN_POINT('Ctrl Pts',(146.898700391862,4.6296253358803,126.092602535266));
#274278=CARTESIAN_POINT('Ctrl Pts',(146.62025276805,-1.46170993963237,124.362505370115));
#274279=CARTESIAN_POINT('Ctrl Pts',(146.341805144237,-6.20980518912327,
128.552158475246));
#274280=CARTESIAN_POINT('Ctrl Pts',(146.063357520424,-5.2513928356585,134.811475322978));
#274281=CARTESIAN_POINT('Ctrl Pts',(145.784909896611,0.532792988974217,
137.388449514872));
#274282=CARTESIAN_POINT('Ctrl Pts',(145.506462272798,5.82736808512415,133.914967660766));
#274283=CARTESIAN_POINT('Ctrl Pts',(145.228014648985,5.76687659380242,127.582989895561));
#274284=CARTESIAN_POINT('Ctrl Pts',(144.949567025172,0.406907240360106,
124.211294451169));
#274285=CARTESIAN_POINT('Ctrl Pts',(144.671119401359,-5.32698998844935,
126.898304724507));
#274286=CARTESIAN_POINT('Ctrl Pts',(144.392671777546,-6.16564365580234,
133.174789542127));
#274287=CARTESIAN_POINT('Ctrl Pts',(144.114224153734,-1.33837201191069,
137.272965979966));
#274288=CARTESIAN_POINT('Ctrl Pts',(143.83577652992,4.71879812781917,135.426810098699));
#274289=CARTESIAN_POINT('Ctrl Pts',(143.557328906108,6.43962331418753,129.332848963481));
#274290=CARTESIAN_POINT('Ctrl Pts',(143.278881282295,2.24274926790569,124.591135151027));
#274291=CARTESIAN_POINT('Ctrl Pts',(143.000433658482,-4.01510179118866,
125.559072009383));
#274292=CARTESIAN_POINT('Ctrl Pts',(142.721986034669,-6.58327045280769,
131.347172852065));
#274293=CARTESIAN_POINT('Ctrl Pts',(142.443538410856,-3.10173517893752,
136.636455769093));
#274294=CARTESIAN_POINT('Ctrl Pts',(142.165090787043,3.23014319618891,136.566328155556));
#274295=CARTESIAN_POINT('Ctrl Pts',(141.886643163231,6.5936777752854,131.201233862367));
#274296=CARTESIAN_POINT('Ctrl Pts',(141.608195539417,3.89794459796173,125.471432445543));
#274297=CARTESIAN_POINT('Ctrl Pts',(141.329747915605,-2.37980923970876,
124.642331490782));
#274298=CARTESIAN_POINT('Ctrl Pts',(141.051300291792,-6.47063464623165,
129.475834271677));
#274299=CARTESIAN_POINT('Ctrl Pts',(140.772852667979,-4.61526292094352,
135.530187862324));
#274300=CARTESIAN_POINT('Ctrl Pts',(140.494405044166,1.48130996056343,137.241737084533));
#274301=CARTESIAN_POINT('Ctrl Pts',(140.215957420353,6.21663135432719,133.037651816923));
#274302=CARTESIAN_POINT('Ctrl Pts',(139.93750979654,5.23917223278974,126.781281039444));
#274303=CARTESIAN_POINT('Ctrl Pts',(139.659062172727,-0.552830222889001,
124.221923855894));
#274304=CARTESIAN_POINT('Ctrl Pts',(139.380614548914,-5.83680871099059,
127.711504486408));
#274305=CARTESIAN_POINT('Ctrl Pts',(139.102166925101,-5.75704513764935,
134.043268807033));
#274306=CARTESIAN_POINT('Ctrl Pts',(138.823719301288,-0.386838330098996,
137.398634730999));
#274307=CARTESIAN_POINT('Ctrl Pts',(138.545271677476,5.33885400470937,134.694184892919));
#274308=CARTESIAN_POINT('Ctrl Pts',(138.266824053663,6.15840032670771,128.41517657427));
#274309=CARTESIAN_POINT('Ctrl Pts',(137.98837642985,1.31867760304303,124.331711673279));
#274310=CARTESIAN_POINT('Ctrl Pts',(137.709928806037,-4.7328454168358,126.196294945608));
#274311=CARTESIAN_POINT('Ctrl Pts',(137.431481182224,-6.43511471099507,
132.295465453942));
#274312=CARTESIAN_POINT('Ctrl Pts',(137.153033558411,-2.22382795858067,
137.024383462168));
#274313=CARTESIAN_POINT('Ctrl Pts',(136.874585934598,4.03104804773404,136.037404341212));
#274314=CARTESIAN_POINT('Ctrl Pts',(136.596138310785,6.5815878258261,130.241513686623));
#274315=CARTESIAN_POINT('Ctrl Pts',(136.317690686972,3.08396992042408,124.96285186497));
#274316=CARTESIAN_POINT('Ctrl Pts',(136.03924306316,-3.24766568154122,125.052251213384));
#274317=CARTESIAN_POINT('Ctrl Pts',(135.760795439346,-6.5948551794591,130.427558098075));
#274318=CARTESIAN_POINT('Ctrl Pts',(135.482347815534,-3.88169494404043,
136.149128090351));
#274319=CARTESIAN_POINT('Ctrl Pts',(135.203900191721,2.3985533136112,136.959117881544));
#274320=CARTESIAN_POINT('Ctrl Pts',(134.925452567908,6.47464825189767,132.113186423748));
#274321=CARTESIAN_POINT('Ctrl Pts',(134.647004944095,4.60085775084163,126.064507989766));
#274322=CARTESIAN_POINT('Ctrl Pts',(134.368557320282,-1.50089625884118,
124.371522566057));
#274323=CARTESIAN_POINT('Ctrl Pts',(134.090109696469,-6.22339992950755,
128.590001050074));
#274324=CARTESIAN_POINT('Ctrl Pts',(133.811662072656,-5.22690309494509,
134.843367799137));
#274325=CARTESIAN_POINT('Ctrl Pts',(133.533214448844,0.572862335460145,
137.385084264805));
#274326=CARTESIAN_POINT('Ctrl Pts',(133.25476682503,5.84619526545829,133.879437184883));
#274327=CARTESIAN_POINT('Ctrl Pts',(132.976319201218,5.7471603490167,127.547944965438));
#274328=CARTESIAN_POINT('Ctrl Pts',(132.697871577405,0.366765836220533,
124.208939645549));
#274329=CARTESIAN_POINT('Ctrl Pts',(132.419423953592,-5.35066856255522,
126.930803994717));
#274330=CARTESIAN_POINT('Ctrl Pts',(132.140976329779,-6.15109994703373,
133.212277646521));
#274331=CARTESIAN_POINT('Ctrl Pts',(131.862528705966,-1.29897097812634,
137.280993182001));
#274332=CARTESIAN_POINT('Ctrl Pts',(131.584081082153,4.74684886141891,135.397999791857));
#274333=CARTESIAN_POINT('Ctrl Pts',(131.30563345834,6.43054649377913,129.293676412286));
#274334=CARTESIAN_POINT('Ctrl Pts',(131.027185834528,2.20488604801711,124.577598016342));
#274335=CARTESIAN_POINT('Ctrl Pts',(130.748738210715,-4.04695696120101,
125.583610256657));
#274336=CARTESIAN_POINT('Ctrl Pts',(130.470290586902,-6.57984422791396,
131.387237030814));
#274337=CARTESIAN_POINT('Ctrl Pts',(130.191842963089,-3.06617609243459,
136.65522885629));
#274338=CARTESIAN_POINT('Ctrl Pts',(129.913395339276,3.26515808096253,136.546558601182));
#274339=CARTESIAN_POINT('Ctrl Pts',(129.634947715463,6.59597148979528,131.161088921098));
#274340=CARTESIAN_POINT('Ctrl Pts',(129.35650009165,3.86540933062731,125.447803357213));
#274341=CARTESIAN_POINT('Ctrl Pts',(129.078052467837,-2.41727516764341,
124.656932233223));
#274342=CARTESIAN_POINT('Ctrl Pts',(128.799604844024,-6.47860187730669,
129.515247475871));
#274343=CARTESIAN_POINT('Ctrl Pts',(128.521157220212,-4.58640995902212,
135.558194719059));
#274344=CARTESIAN_POINT('Ctrl Pts',(128.242709596398,1.52046865302106,137.232600660681));
#274345=CARTESIAN_POINT('Ctrl Pts',(127.964261972586,6.23011085196111,132.999768039666));
#274346=CARTESIAN_POINT('Ctrl Pts',(127.685814348773,5.2145855357842,126.749463249355));
#274347=CARTESIAN_POINT('Ctrl Pts',(127.40736672496,-0.592889141112855,
124.225411047681));
#274348=CARTESIAN_POINT('Ctrl Pts',(127.128919101147,-5.85552766157182,
127.747092101177));
#274349=CARTESIAN_POINT('Ctrl Pts',(126.850471477334,-5.7372223194756,134.078253565364));
#274350=CARTESIAN_POINT('Ctrl Pts',(126.572023853521,-0.346689944673359,
137.400867349086));
#274351=CARTESIAN_POINT('Ctrl Pts',(126.293576229708,5.36243355253846,134.66161370381));
#274352=CARTESIAN_POINT('Ctrl Pts',(126.015128605896,6.14374258441013,128.377732909565));
#274353=CARTESIAN_POINT('Ctrl Pts',(125.736680982083,1.27925231971985,124.323804431618));
#274354=CARTESIAN_POINT('Ctrl Pts',(125.45823335827,-4.76080833184274,126.225190495787));
#274355=CARTESIAN_POINT('Ctrl Pts',(125.179785734457,-6.42591870485886,
132.334610196974));
#274356=CARTESIAN_POINT('Ctrl Pts',(124.901338110644,-2.1859237116904,137.037805291532));
#274357=CARTESIAN_POINT('Ctrl Pts',(124.622890486831,4.06282838421153,136.012769251418));
#274358=CARTESIAN_POINT('Ctrl Pts',(124.344442863018,6.5780396752237,130.201460121699));
#274359=CARTESIAN_POINT('Ctrl Pts',(124.065995239205,3.04835385980878,124.944187094356));
#274360=CARTESIAN_POINT('Ctrl Pts',(123.787547615392,-3.28262023240536,
125.07212724945));
#274361=CARTESIAN_POINT('Ctrl Pts',(123.509099991579,-6.59702669595264,
130.467709834674));
#274362=CARTESIAN_POINT('Ctrl Pts',(123.230652367767,-3.84908790859021,
136.17265804307));
#274363=CARTESIAN_POINT('Ctrl Pts',(122.952204743954,2.43597462836867,136.944403173336));
#274364=CARTESIAN_POINT('Ctrl Pts',(122.673757120141,6.48249548583303,132.073749152604));
#274365=CARTESIAN_POINT('Ctrl Pts',(122.395309496328,4.57191967932717,126.036589081248));
#274366=CARTESIAN_POINT('Ctrl Pts',(122.116861872515,-1.54002696178715,
124.380778133181));
#274367=CARTESIAN_POINT('Ctrl Pts',(121.838414248702,-6.23676405951882,
128.627925678811));
#274368=CARTESIAN_POINT('Ctrl Pts',(121.559966624889,-5.20221966941523,
134.8751106084));
#274369=CARTESIAN_POINT('Ctrl Pts',(121.281519001076,0.612910454321425,
137.381475163605));
#274370=CARTESIAN_POINT('Ctrl Pts',(121.003071377263,5.86480581287692,133.843792760907));
#274371=CARTESIAN_POINT('Ctrl Pts',(120.724623753451,5.72723114109079,127.513020702994));
#274372=CARTESIAN_POINT('Ctrl Pts',(120.446176129638,0.326610841437887,
124.206829235678));
#274373=CARTESIAN_POINT('Ctrl Pts',(120.167728505825,-5.3741488656698,126.963446800991));
#274374=CARTESIAN_POINT('Ctrl Pts',(119.889280882012,-6.13632830699453,
133.249676524665));
#274375=CARTESIAN_POINT('Ctrl Pts',(119.610833258199,-1.25952181049465,
137.288780390037));
#274376=CARTESIAN_POINT('Ctrl Pts',(119.332385634386,4.77472369878856,135.369019266025));
#274377=CARTESIAN_POINT('Ctrl Pts',(119.053938010573,6.42123138710552,129.254559840052));
#274378=CARTESIAN_POINT('Ctrl Pts',(118.77549038676,2.16694112526505,124.564291616636));
#274379=CARTESIAN_POINT('Ctrl Pts',(118.497042762948,-4.07866216973492,
125.608341960757));
#274380=CARTESIAN_POINT('Ctrl Pts',(118.218595139134,-6.57617418447253,
131.427279610862));
#274381=CARTESIAN_POINT('Ctrl Pts',(117.940147515322,-3.03050338764912,
136.673785137412));
#274382=CARTESIAN_POINT('Ctrl Pts',(117.661699891509,3.30005197410286,136.526576267552));
#274383=CARTESIAN_POINT('Ctrl Pts',(117.383252267696,6.59802078815589,131.120930761129));
#274384=CARTESIAN_POINT('Ctrl Pts',(117.104804643883,3.83273082912851,125.424372758082));
#274385=CARTESIAN_POINT('Ctrl Pts',(116.82635702007,-2.45465152255762,124.671760770883));
#274386=CARTESIAN_POINT('Ctrl Pts',(116.547909396257,-6.48632904140672,
129.554708448625));
#274387=CARTESIAN_POINT('Ctrl Pts',(116.269461772444,-4.55738704599302,
135.586025420722));
#274388=CARTESIAN_POINT('Ctrl Pts',(115.991014148631,1.55957100395386,137.223226036031));
#274389=CARTESIAN_POINT('Ctrl Pts',(115.712566524818,6.24335949054626,132.961802910777));
#274390=CARTESIAN_POINT('Ctrl Pts',(115.434118901006,5.18980561039392,126.717795714978));
#274391=CARTESIAN_POINT('Ctrl Pts',(115.155671277193,-0.632926089611396,
124.229142024863));
#274392=CARTESIAN_POINT('Ctrl Pts',(114.87722365338,-5.87402963342224,127.782793004156));
#274393=CARTESIAN_POINT('Ctrl Pts',(114.598776029567,-5.71718690641897,
134.113117008387));
#274394=CARTESIAN_POINT('Ctrl Pts',(114.320328405754,-0.306528712524212,
137.40285553119));
#274395=CARTESIAN_POINT('Ctrl Pts',(114.041880781941,5.38581439342023,134.628899582769));
#274396=CARTESIAN_POINT('Ctrl Pts',(113.763433158128,6.12885718347172,128.340379164441));
#274397=CARTESIAN_POINT('Ctrl Pts',(113.484985534315,1.23977963323159,124.316137329349));
#274398=CARTESIAN_POINT('Ctrl Pts',(113.206537910502,-4.78859483334625,
126.254255728798));
#274399=CARTESIAN_POINT('Ctrl Pts',(112.92809028669,-6.41648458394181,132.373698236044));
#274400=CARTESIAN_POINT('Ctrl Pts',(112.649642662877,-2.14793846459313,
137.050996138312));
#274401=CARTESIAN_POINT('Ctrl Pts',(112.371195039064,4.09445817108915,135.987941162125));
#274402=CARTESIAN_POINT('Ctrl Pts',(112.092747415251,6.57424777294209,130.161428897475));
#274403=CARTESIAN_POINT('Ctrl Pts',(111.814299791438,3.01262484132005,124.925739474628));
#274404=CARTESIAN_POINT('Ctrl Pts',(111.535852167625,-3.31745314456969,
125.092215695531));
#274405=CARTESIAN_POINT('Ctrl Pts',(111.257404543812,-6.59895375719588,
130.507874045991));
#274406=CARTESIAN_POINT('Ctrl Pts',(110.978956919999,-3.816338243772,136.195989071554));
#274407=CARTESIAN_POINT('Ctrl Pts',(110.700509296186,2.47330567719032,136.929460943594));
#274408=CARTESIAN_POINT('Ctrl Pts',(110.422061672374,6.49010250851429,132.0342648438));
#274409=CARTESIAN_POINT('Ctrl Pts',(110.143614048561,4.54281219364771,126.008846844259));
#274410=CARTESIAN_POINT('Ctrl Pts',(109.865166424748,-1.57910059846782,
124.390271728514));
#274411=CARTESIAN_POINT('Ctrl Pts',(109.586718800935,-6.24989708394428,
128.665930956147));
#274412=CARTESIAN_POINT('Ctrl Pts',(109.308271177122,-5.17734347372243,
134.906702574525));
#274413=CARTESIAN_POINT('Ctrl Pts',(109.029823553309,0.652935861560398,
137.377622345005));
#274414=CARTESIAN_POINT('Ctrl Pts',(108.751375929496,5.88319903775945,133.808035709655));
#274415=CARTESIAN_POINT('Ctrl Pts',(108.472928305683,5.70708970850866,127.478218402361));
#274416=CARTESIAN_POINT('Ctrl Pts',(108.19448068187,0.286443743970404,124.204963299759));
#274417=CARTESIAN_POINT('Ctrl Pts',(107.916033058058,-5.39743002772183,
126.996231933739));
#274418=CARTESIAN_POINT('Ctrl Pts',(107.637585434244,-6.12132928305326,
133.286984790727));
#274419=CARTESIAN_POINT('Ctrl Pts',(107.359137810432,-1.22002597081922,
137.296327315513));
#274420=CARTESIAN_POINT('Ctrl Pts',(107.080690186619,4.80242160701559,135.339869595089));
#274421=CARTESIAN_POINT('Ctrl Pts',(106.802242562806,6.41167833934146,129.215500696253));
#274422=CARTESIAN_POINT('Ctrl Pts',(106.523794938993,2.12891590571267,124.551216444981));
#274423=CARTESIAN_POINT('Ctrl Pts',(106.24534731518,-4.11021624194206,125.633266205238));
#274424=CARTESIAN_POINT('Ctrl Pts',(105.966899691367,-6.57226045847839,
131.467299108419));
#274425=CARTESIAN_POINT('Ctrl Pts',(105.688452067554,-2.99471838644612,
136.692123924851));
#274426=CARTESIAN_POINT('Ctrl Pts',(105.410004443742,3.33482358260376,136.506381895117));
#274427=CARTESIAN_POINT('Ctrl Pts',(105.131556819929,6.59982559442975,131.080760870538));
#274428=CARTESIAN_POINT('Ctrl Pts',(104.853109196116,3.79991030437941,125.401141516381));
#274429=CARTESIAN_POINT('Ctrl Pts',(104.574661572303,-2.49193691945696,
124.686816554284));
#274430=CARTESIAN_POINT('Ctrl Pts',(104.29621394849,-6.49381585219884,129.594215727701));
#274431=CARTESIAN_POINT('Ctrl Pts',(104.017766324677,-4.52819525731082,
135.613678936038));
#274432=CARTESIAN_POINT('Ctrl Pts',(103.739318700864,1.59861556440955,137.213613557961));
#274433=CARTESIAN_POINT('Ctrl Pts',(103.460871077051,6.25637677914949,132.923757837073));
#274434=CARTESIAN_POINT('Ctrl Pts',(103.182423453238,5.16483337484823,126.686279609768));
#274435=CARTESIAN_POINT('Ctrl Pts',(102.903975829425,-0.672939584800916,
124.233116649188));
#274436=CARTESIAN_POINT('Ctrl Pts',(102.625528205613,-5.89231394094447,
127.818605872432));
#274437=CARTESIAN_POINT('Ctrl Pts',(102.347080581799,-5.69693964089892,
134.147857844226));
#274438=CARTESIAN_POINT('Ctrl Pts',(102.068632957987,-0.266356121840884,
137.40459920364));
#274439=CARTESIAN_POINT('Ctrl Pts',(101.790185334174,5.40899566096888,134.59604374203));
#274440=CARTESIAN_POINT('Ctrl Pts',(101.511737710361,6.11374467547657,128.303116723058));
#274441=CARTESIAN_POINT('Ctrl Pts',(101.233290086548,1.20026100625305,124.308710650579));
#274442=CARTESIAN_POINT('Ctrl Pts',(100.954842462735,-4.81620389170723,
126.28348956762));
#274443=CARTESIAN_POINT('Ctrl Pts',(100.676394838922,-6.40681269782886,
132.412728122731));
#274444=CARTESIAN_POINT('Ctrl Pts',(100.397947215109,-2.10987362484612,
137.063955513716));
#274445=CARTESIAN_POINT('Ctrl Pts',(100.119499591297,4.12593623631335,135.962920993349));
#274446=CARTESIAN_POINT('Ctrl Pts',(99.8410519674839,6.5702122594916,130.121421497322));
#274447=CARTESIAN_POINT('Ctrl Pts',(99.5626043436712,2.97678418891005,124.907509689368));
#274448=CARTESIAN_POINT('Ctrl Pts',(99.2841567198582,-3.35216312728773,
125.112515807244));
#274449=CARTESIAN_POINT('Ctrl Pts',(99.0057090960455,-6.6006362917809,130.548049243728));
#274450=CARTESIAN_POINT('Ctrl Pts',(98.7272614722323,-3.78344716313679,
136.219120311263));
#274451=CARTESIAN_POINT('Ctrl Pts',(98.4488138484198,2.51054507676055,136.914291746006));
#274452=CARTESIAN_POINT('Ctrl Pts',(98.1703662246066,6.49746903806041,131.994734960442));
#274453=CARTESIAN_POINT('Ctrl Pts',(97.8919186007939,4.51353637239165,125.981282306795));
#274454=CARTESIAN_POINT('Ctrl Pts',(97.6134709769809,-1.61811572099509,
124.400003000271));
#274455=CARTESIAN_POINT('Ctrl Pts',(97.335023353168,-6.26279851613479,128.704015473778));
#274456=CARTESIAN_POINT('Ctrl Pts',(97.0565757293552,-5.15227542966332,
134.938142526861));
#274457=CARTESIAN_POINT('Ctrl Pts',(96.7781281055422,0.692937074020952,
137.373525951775));
#274458=CARTESIAN_POINT('Ctrl Pts',(96.4996804817294,5.90137425853808,133.772167356118));
#274459=CARTESIAN_POINT('Ctrl Pts',(96.2212328579164,5.6867367976186,127.443539353151));
#274460=CARTESIAN_POINT('Ctrl Pts',(95.9427852341037,0.246266032224636,
124.203341906934));
#274461=CARTESIAN_POINT('Ctrl Pts',(95.6643376102905,-5.42051118601915,
127.029158178097));
#274462=CARTESIAN_POINT('Ctrl Pts',(95.3858899864779,-6.10610343100435,
133.324201062238));
#274463=CARTESIAN_POINT('Ctrl Pts',(95.1074423626648,-1.18048492263276,
137.303633678775));
#274464=CARTESIAN_POINT('Ctrl Pts',(94.828994738852,4.82994155974394,135.3105518592));
#274465=CARTESIAN_POINT('Ctrl Pts',(94.5505471150391,6.40188770447863,129.176500428244));
#274466=CARTESIAN_POINT('Ctrl Pts',(94.2720994912261,2.09081179839861,124.538372985881));
#274467=CARTESIAN_POINT('Ctrl Pts',(93.9936518674133,-4.14161800857485,
125.658382066524));
#274468=CARTESIAN_POINT('Ctrl Pts',(93.7152042436005,-6.56810319495607,
131.507294040545));
#274469=CARTESIAN_POINT('Ctrl Pts',(93.4367566197874,-2.95882241485189,
136.710244539055));
#274470=CARTESIAN_POINT('Ctrl Pts',(93.1583089959747,3.36947161799043,136.485976232185));
#274471=CARTESIAN_POINT('Ctrl Pts',(92.8798613721617,6.60138584173913,131.040580737834));
#274472=CARTESIAN_POINT('Ctrl Pts',(92.6014137483489,3.76694897255651,125.37811049295));
#274473=CARTESIAN_POINT('Ctrl Pts',(92.3229661245359,-2.5291299767175,124.702099025532));
#274474=CARTESIAN_POINT('Ctrl Pts',(92.044518500723,-6.50106203225643,129.633767849141));
#274475=CARTESIAN_POINT('Ctrl Pts',(91.7660708769102,-4.49883567468812,
135.641154240296));
#274476=CARTESIAN_POINT('Ctrl Pts',(91.4876232530973,1.63760088757763,137.203763582666));
#274477=CARTESIAN_POINT('Ctrl Pts',(91.2091756292845,6.26916223541028,132.885634228324));
#274478=CARTESIAN_POINT('Ctrl Pts',(90.9307280054714,5.13966975450256,126.654916101563));
#274479=CARTESIAN_POINT('Ctrl Pts',(90.6522803816587,-0.71292814396669,
124.237334773374));
#274480=CARTESIAN_POINT('Ctrl Pts',(90.3738327578456,-5.91037990660673,
127.85452937895));
#274481=CARTESIAN_POINT('Ctrl Pts',(90.0953851340328,-5.67648127318543,
134.182474785545));
#274482=CARTESIAN_POINT('Ctrl Pts',(89.8169375102199,-0.226173661233629,
137.406098301819));
#274483=CARTESIAN_POINT('Ctrl Pts',(89.5384898864071,5.43197649619419,134.563047399079));
#274484=CARTESIAN_POINT('Ctrl Pts',(89.260042262594,6.09840562042418,128.265946966186));
#274485=CARTESIAN_POINT('Ctrl Pts',(88.9815946387814,1.1606979031614,124.301524670509));
#274486=CARTESIAN_POINT('Ctrl Pts',(88.7031470149683,-4.84363448386183,
126.312890928981));
#274487=CARTESIAN_POINT('Ctrl Pts',(88.4246993911556,-6.39690340491527,
132.45169841077));
#274488=CARTESIAN_POINT('Ctrl Pts',(88.1462517673426,-2.07173060295614,
137.076682937528));
#274489=CARTESIAN_POINT('Ctrl Pts',(87.8678041435297,4.15726141345302,135.937709672222));
#274490=CARTESIAN_POINT('Ctrl Pts',(87.5893565197169,6.5659332844097,130.081439403729));
#274491=CARTESIAN_POINT('Ctrl Pts',(87.3109088959039,2.94083323066708,124.889498414087));
#274492=CARTESIAN_POINT('Ctrl Pts',(87.032461272091,-3.38674889436835,125.133026832359));
#274493=CARTESIAN_POINT('Ctrl Pts',(86.7540136482781,-6.60207423736065,
130.588233939178));
#274494=CARTESIAN_POINT('Ctrl Pts',(86.4755660244652,-3.75041588547566,
136.242050905059));
#274495=CARTESIAN_POINT('Ctrl Pts',(86.1971184006524,2.54769144715974,136.898896142674));
#274496=CARTESIAN_POINT('Ctrl Pts',(85.9186707768394,6.50459480150186,131.955160967326));
#274497=CARTESIAN_POINT('Ctrl Pts',(85.6402231530266,4.48409330038545,125.953896490271));
#274498=CARTESIAN_POINT('Ctrl Pts',(85.3617755292137,-1.65707088364924,
124.409971587854));
#274499=CARTESIAN_POINT('Ctrl Pts',(85.0833279054008,-6.27546787802325,
128.742177820471));
#274500=CARTESIAN_POINT('Ctrl Pts',(84.8048802815879,-5.12701646614329,
134.969429300388));
#274501=CARTESIAN_POINT('Ctrl Pts',(84.526432657775,0.732912609443495,137.369186135708));
#274502=CARTESIAN_POINT('Ctrl Pts',(84.2479850339622,5.91933080172332,133.73618902941));
#274503=CARTESIAN_POINT('Ctrl Pts',(83.9695374101491,5.6661731626052,127.408984840408));
#274504=CARTESIAN_POINT('Ctrl Pts',(83.6910897863363,0.206079195000604,
124.201965117285));
#274505=CARTESIAN_POINT('Ctrl Pts',(83.4126421625234,-5.44339148528112,
127.062224313968));
#274506=CARTESIAN_POINT('Ctrl Pts',(83.1341945387106,-6.09065131504733,
133.361323960135));
#274507=CARTESIAN_POINT('Ctrl Pts',(82.8557469148977,-1.14090013114324,
137.310699209084));
#274508=CARTESIAN_POINT('Ctrl Pts',(82.5772992910847,4.85728253721157,135.281067144739));
#274509=CARTESIAN_POINT('Ctrl Pts',(82.2988516672719,6.39185984531258,129.137560481192));
#274510=CARTESIAN_POINT('Ctrl Pts',(82.0204040434589,2.05263021528453,124.52576171526));
#274511=CARTESIAN_POINT('Ctrl Pts',(81.7419564196462,-4.17286630602932,
125.683688613938));
#274512=CARTESIAN_POINT('Ctrl Pts',(81.4635087958331,-6.56370254795435,
131.547262925216));
#274513=CARTESIAN_POINT('Ctrl Pts',(81.1850611720204,-2.92281680300497,
136.728146308557));
#274514=CARTESIAN_POINT('Ctrl Pts',(80.9066135482074,3.40399479636718,136.465360034899));
#274515=CARTESIAN_POINT('Ctrl Pts',(80.6281659243945,6.60270147226842,131.000391851905));
#274516=CARTESIAN_POINT('Ctrl Pts',(80.3497183005816,3.73384805505426,125.355280541214));
#274517=CARTESIAN_POINT('Ctrl Pts',(80.0712706767688,-2.56622931613655,
124.717607618327));
#274518=CARTESIAN_POINT('Ctrl Pts',(79.7928230529558,-6.50806731306963,
129.673363347327));
#274519=CARTESIAN_POINT('Ctrl Pts',(79.514375429143,-4.46930938605503,135.668450315387));
#274520=CARTESIAN_POINT('Ctrl Pts',(79.23592780533,1.67652552884245,137.193676475141));
#274521=CARTESIAN_POINT('Ctrl Pts',(78.9574801815173,6.28171538555901,132.847433497217));
#274522=CARTESIAN_POINT('Ctrl Pts',(78.6790325577042,5.11431568180404,126.62370635255));
#274523=CARTESIAN_POINT('Ctrl Pts',(78.4005849338915,-0.752890285318027,
124.241796241119));
#274524=CARTESIAN_POINT('Ctrl Pts',(78.1221373100785,-5.92822686096799,
127.890562192549));
#274525=CARTESIAN_POINT('Ctrl Pts',(77.8436896862655,-5.65581256137084,
134.216966549603));
#274526=CARTESIAN_POINT('Ctrl Pts',(77.5652420624528,-0.185982819678218,
137.407352770183));
#274527=CARTESIAN_POINT('Ctrl Pts',(77.2867944386398,5.45475604753291,134.529911776607));
#274528=CARTESIAN_POINT('Ctrl Pts',(77.008346814827,6.08284058670873,128.228871271165));
#274529=CARTESIAN_POINT('Ctrl Pts',(76.729899191014,1.12109178998211,124.294579655415));
#274530=CARTESIAN_POINT('Ctrl Pts',(76.4514515672013,-4.8708855933594,126.342458723402));
#274531=CARTESIAN_POINT('Ctrl Pts',(76.1730039433881,-6.38675707239351,
132.4906076561));
#274532=CARTESIAN_POINT('Ctrl Pts',(75.8945563195755,-2.03351081232684,
137.089177938131));
#274533=CARTESIAN_POINT('Ctrl Pts',(75.6161086957625,4.18843254174224,135.912308132958));
#274534=CARTESIAN_POINT('Ctrl Pts',(75.3376610719495,6.56141100625526,130.041484098248));
#274535=CARTESIAN_POINT('Ctrl Pts',(75.0592134481368,2.90477329876725,124.871706316201));
#274536=CARTESIAN_POINT('Ctrl Pts',(74.7807658243238,-3.42120916422307,
125.153748010832));
#274537=CARTESIAN_POINT('Ctrl Pts',(74.5023182005109,-6.60326754065171,
130.628426643279));
#274538=CARTESIAN_POINT('Ctrl Pts',(74.223870576698,-3.71724563477466,136.264780003243));
#274539=CARTESIAN_POINT('Ctrl Pts',(73.9454229528852,2.58474341191554,136.883274704086));
#274540=CARTESIAN_POINT('Ctrl Pts',(73.6669753290721,6.51147953479087,131.915544330879));
#274541=CARTESIAN_POINT('Ctrl Pts',(73.3885277052595,4.45448406865298,125.926690409479));
#274542=CARTESIAN_POINT('Ctrl Pts',(73.1100800814464,-1.6959646429323,124.420177121874));
#274543=CARTESIAN_POINT('Ctrl Pts',(72.8316324576336,-6.28790470014163,
128.780416582107));
#274544=CARTESIAN_POINT('Ctrl Pts',(72.5531848338207,-5.1015675191428,135.000561735763));
#274545=CARTESIAN_POINT('Ctrl Pts',(72.2747372100078,0.772860986519783,
137.364603057617));
#274546=CARTESIAN_POINT('Ctrl Pts',(71.996289586195,5.93706800192887,133.700102062723));
#274547=CARTESIAN_POINT('Ctrl Pts',(71.7178419623819,5.64539956546153,127.374556144564));
#274548=CARTESIAN_POINT('Ctrl Pts',(71.4393943385692,0.165884721436248,
124.20083298183));
#274549=CARTESIAN_POINT('Ctrl Pts',(71.1609467147562,-5.46607007766984,
127.095429116077));
#274550=CARTESIAN_POINT('Ctrl Pts',(70.8824990909434,-6.07497350776591,
133.398352108815));
#274551=CARTESIAN_POINT('Ctrl Pts',(70.6040514671303,-1.10127306317963,
137.317523644624));
#274552=CARTESIAN_POINT('Ctrl Pts',(70.3256038433176,4.88444352628841,135.251416544269));
#274553=CARTESIAN_POINT('Ctrl Pts',(70.0471562195047,6.38159513342946,129.098682298033));
#274554=CARTESIAN_POINT('Ctrl Pts',(69.7687085956917,2.01437257120279,124.513383100429));
#274555=CARTESIAN_POINT('Ctrl Pts',(69.4902609718789,-4.20395997638847,
125.709184909736));
#274556=CARTESIAN_POINT('Ctrl Pts',(69.211813348066,-6.5590586805409,131.587204281367));
#274557=CARTESIAN_POINT('Ctrl Pts',(68.9333657242531,-2.88670288510633,
136.745828570004));
#274558=CARTESIAN_POINT('Ctrl Pts',(68.6549181004402,3.43839183846502,136.444534067195));
#274559=CARTESIAN_POINT('Ctrl Pts',(68.3764704766273,6.60377243726651,130.960195701968));
#274560=CARTESIAN_POINT('Ctrl Pts',(68.0980228528144,3.70060877843901,125.332652507142));
#274561=CARTESIAN_POINT('Ctrl Pts',(67.8195752290015,-2.6032335629848,124.733341757993));
#274562=CARTESIAN_POINT('Ctrl Pts',(67.5411276051886,-6.51483143505509,
129.713000755032));
#274563=CARTESIAN_POINT('Ctrl Pts',(67.2626799813758,-4.43961748551916,
135.695566149845));
#274564=CARTESIAN_POINT('Ctrl Pts',(66.9842323575627,1.71538804583728,137.183352609169));
#274565=CARTESIAN_POINT('Ctrl Pts',(66.7057847337499,6.29403576443417,132.809157059292));
#274566=CARTESIAN_POINT('Ctrl Pts',(66.4273371099371,5.08877209625689,126.592651519219));
#274567=CARTESIAN_POINT('Ctrl Pts',(66.1488894861241,-0.792824528042931,
124.246500887099));
#274568=CARTESIAN_POINT('Ctrl Pts',(65.8704418623113,-5.94585414270274,
127.92670297802));
#274569=CARTESIAN_POINT('Ctrl Pts',(65.5919942384984,-5.63493427134196,
134.251331858291));
#274570=CARTESIAN_POINT('Ctrl Pts',(65.3135466146855,-0.145785086460763,
137.408362562243));
#274571=CARTESIAN_POINT('Ctrl Pts',(65.0350989908726,5.47733347088038,134.496638102466));
#274572=CARTESIAN_POINT('Ctrl Pts',(64.7566513670597,6.06705015109826,128.191891011849));
#274573=CARTESIAN_POINT('Ctrl Pts',(64.4782037432468,1.0814441343344,124.28787586265));
#274574=CARTESIAN_POINT('Ctrl Pts',(64.199756119434,-4.89795621039988,126.37219185524));
#274575=CARTESIAN_POINT('Ctrl Pts',(63.921308495621,-6.37637407623982,132.529454416925));
#274576=CARTESIAN_POINT('Ctrl Pts',(63.6428608718081,-1.99521566920641,
137.101440052517));
#274577=CARTESIAN_POINT('Ctrl Pts',(63.3644132479953,4.21944846612332,135.886717316821));
#274578=CARTESIAN_POINT('Ctrl Pts',(63.0859656241823,6.556645592603,130.001557061437));
#274579=CARTESIAN_POINT('Ctrl Pts',(62.8075180003696,2.86860572942485,124.854134055001));
#274580=CARTESIAN_POINT('Ctrl Pts',(62.5290703765565,-3.4555426599142,125.174678574835));
#274581=CARTESIAN_POINT('Ctrl Pts',(62.2506227527437,-6.60421615743575,
130.66862586668));
#274582=CARTESIAN_POINT('Ctrl Pts',(61.9721751289308,-3.68393764016947,
136.287306763578));
#274583=CARTESIAN_POINT('Ctrl Pts',(61.6937275051179,2.62169959805353,136.867428009101));
#274584=CARTESIAN_POINT('Ctrl Pts',(61.415279881305,6.51812298281107,131.875886519111));
#274585=CARTESIAN_POINT('Ctrl Pts',(61.1368322574921,4.42470977437533,125.899665072552));
#274586=CARTESIAN_POINT('Ctrl Pts',(60.8583846336791,-1.73479555762186,
124.430619224162));
#274587=CARTESIAN_POINT('Ctrl Pts',(60.5799370098664,-6.30010852163892,
128.818730341733));
#274588=CARTESIAN_POINT('Ctrl Pts',(60.3014893860534,-5.07592953168175,
135.031538679362));
#274589=CARTESIAN_POINT('Ctrl Pts',(60.0230417622406,0.81278072494776,137.35977688733));
#274590=CARTESIAN_POINT('Ctrl Pts',(59.7445941384276,5.95458520189618,133.663907793273));
#274591=CARTESIAN_POINT('Ctrl Pts',(59.4661465146148,5.62441677596096,127.340254541386));
#274592=CARTESIAN_POINT('Ctrl Pts',(59.1876988908018,0.125684100952275,
124.199945542519));
#274593=CARTESIAN_POINT('Ctrl Pts',(58.909251266989,-5.48854612282181,127.128771354006));
#274594=CARTESIAN_POINT('Ctrl Pts',(58.6308036431761,-6.05907059010694,
133.435284136186));
#274595=CARTESIAN_POINT('Ctrl Pts',(58.3523560193632,-1.06160518713815,
137.324106732513));
#274596=CARTESIAN_POINT('Ctrl Pts',(58.0739083955504,4.91142352051418,135.221601156507));
#274597=CARTESIAN_POINT('Ctrl Pts',(57.7954607717374,6.37109394919177,129.059867319411));
#274598=CARTESIAN_POINT('Ctrl Pts',(57.5170131479246,1.97604028380464,124.501237600083));
#274599=CARTESIAN_POINT('Ctrl Pts',(57.2385655241116,-4.23489786746425,
125.734870009144));
#274600=CARTESIAN_POINT('Ctrl Pts',(56.9601179002987,-6.554171764796,131.627116628959));
#274601=CARTESIAN_POINT('Ctrl Pts',(56.6816702764859,-2.85048199937133,
136.76329066817));
#274602=CARTESIAN_POINT('Ctrl Pts',(56.4032226526729,3.47266146968847,136.423499100792));
#274603=CARTESIAN_POINT('Ctrl Pts',(56.1247750288601,6.60459869704857,130.919993777505));
#274604=CARTESIAN_POINT('Ctrl Pts',(55.8463274050471,3.66723237440476,125.310227229228));
#274605=CARTESIAN_POINT('Ctrl Pts',(55.5678797812343,-2.6401413460556,124.749300861495));
#274606=CARTESIAN_POINT('Ctrl Pts',(55.2894321574214,-6.5213541475661,129.752678603477));
#274607=CARTESIAN_POINT('Ctrl Pts',(55.0109845336085,-4.40976107332459,
135.722500738884));
#274608=CARTESIAN_POINT('Ctrl Pts',(54.7325369097956,1.75418699849736,137.172792367301));
#274609=CARTESIAN_POINT('Ctrl Pts',(54.4540892859827,6.30612291549916,132.770806332897));
#274610=CARTESIAN_POINT('Ctrl Pts',(54.1756416621698,5.06303994438864,126.561752752318));
#274611=CARTESIAN_POINT('Ctrl Pts',(53.897194038357,-0.832729392363195,
124.251448536985));
#274612=CARTESIAN_POINT('Ctrl Pts',(53.618746414544,-5.96326109862574,127.962950396153));
#274613=CARTESIAN_POINT('Ctrl Pts',(53.3402987907312,-5.61384717675129,
134.285569438194));
#274614=CARTESIAN_POINT('Ctrl Pts',(53.0618511669183,-0.105581951123662,
137.409127640582));
#274615=CARTESIAN_POINT('Ctrl Pts',(52.7834035431054,5.49970792962155,134.463227609627));
#274616=CARTESIAN_POINT('Ctrl Pts',(52.5049559192925,6.05103489871361,128.155007558556));
#274617=CARTESIAN_POINT('Ctrl Pts',(52.2265082954796,1.04175640537643,124.281413540623));
#274618=CARTESIAN_POINT('Ctrl Pts',(51.9480606716666,-4.9248453318719,126.402089222721));
#274619=CARTESIAN_POINT('Ctrl Pts',(51.6696130478539,-6.36575480119974,
132.568237253767));
#274620=CARTESIAN_POINT('Ctrl Pts',(51.3911654240409,-1.95684659263562,
137.113468826308));
#274621=CARTESIAN_POINT('Ctrl Pts',(51.112717800228,4.25030803728985,135.860938172086));
#274622=CARTESIAN_POINT('Ctrl Pts',(50.8342701764151,6.55163722003711,129.961659772806));
#274623=CARTESIAN_POINT('Ctrl Pts',(50.5558225526023,2.83233186284197,124.836782281636));
#274624=CARTESIAN_POINT('Ctrl Pts',(50.2773749287893,-3.48974810920128,
125.195817748775));
#274625=CARTESIAN_POINT('Ctrl Pts',(49.9989273049765,-6.60492005256131,
130.708830119782));
#274626=CARTESIAN_POINT('Ctrl Pts',(49.7204796811635,-3.65049313590031,
136.309630351328));
#274627=CARTESIAN_POINT('Ctrl Pts',(49.4420320573507,2.65855863614892,136.851356644924));
#274628=CARTESIAN_POINT('Ctrl Pts',(49.1635844335378,6.52452489938715,131.836189001557));
#274629=CARTESIAN_POINT('Ctrl Pts',(48.8851368097249,4.39477152084969,125.87282148092));
#274630=CARTESIAN_POINT('Ctrl Pts',(48.606689185912,-1.77356218882415,124.441297507781));
#274631=CARTESIAN_POINT('Ctrl Pts',(48.3282415620992,-6.31207889029818,
128.857117679619));
#274632=CARTESIAN_POINT('Ctrl Pts',(48.0497939382862,-5.05010345378512,
135.062358983324));
#274633=CARTESIAN_POINT('Ctrl Pts',(47.7713463144734,0.852670345487299,
137.354707803682));
#274634=CARTESIAN_POINT('Ctrl Pts',(47.4928986906604,5.97188175251911,133.627607562248));
#274635=CARTESIAN_POINT('Ctrl Pts',(47.2144510668476,5.60322557162828,127.306081301933));
#274636=CARTESIAN_POINT('Ctrl Pts',(46.9360034430346,0.0854788231980546,
124.199302832238));
#274637=CARTESIAN_POINT('Ctrl Pts',(46.6575558192218,-5.5108187878785,127.162249792247));
#274638=CARTESIAN_POINT('Ctrl Pts',(46.3791081954089,-6.04294315135938,
133.47211867372));
#274639=CARTESIAN_POINT('Ctrl Pts',(46.100660571596,-1.02189797292572,137.330448228811));
#274640=CARTESIAN_POINT('Ctrl Pts',(45.822212947783,4.93822152013526,135.191622086273));
#274641=CARTESIAN_POINT('Ctrl Pts',(45.5437653239702,6.36035668172477,129.02111698363));
#274642=CARTESIAN_POINT('Ctrl Pts',(45.2653177001572,1.9376347735074,124.489325664279));
#274643=CARTESIAN_POINT('Ctrl Pts',(44.9868700763445,-4.26567883284234,
125.76074296039));
#274644=CARTESIAN_POINT('Ctrl Pts',(44.7084224525315,-6.54904198180601,
131.666998489025));
#274645=CARTESIAN_POINT('Ctrl Pts',(44.4299748287186,-2.81415548797717,
136.780531955991));
#274646=CARTESIAN_POINT('Ctrl Pts',(44.1515272049057,3.50680242016433,136.402255915145));
#274647=CARTESIAN_POINT('Ctrl Pts',(43.8730795810928,6.60518022099696,130.879787568212));
#274648=CARTESIAN_POINT('Ctrl Pts',(43.59463195728,3.63372007972613,125.288005538446));
#274649=CARTESIAN_POINT('Ctrl Pts',(43.316184333467,-2.6769512977182,124.765484337463));
#274650=CARTESIAN_POINT('Ctrl Pts',(43.0377367096542,-6.52763520890084,
129.792395422388));
#274651=CARTESIAN_POINT('Ctrl Pts',(42.7592890858413,-4.37974125581177,
135.749253084432));
#274652=CARTESIAN_POINT('Ctrl Pts',(42.4808414620283,1.79292094911309,137.161996140853));
#274653=CARTESIAN_POINT('Ctrl Pts',(42.2023938382155,6.31797639086063,132.732382739134));
#274654=CARTESIAN_POINT('Ctrl Pts',(41.9239462144025,5.0371201797131,126.531011196811));
#274655=CARTESIAN_POINT('Ctrl Pts',(41.6454985905898,-0.872603399589798,
124.256639007436));
#274656=CARTESIAN_POINT('Ctrl Pts',(41.3670509667768,-5.98044708371573,
127.999303103786));
#274657=CARTESIAN_POINT('Ctrl Pts',(41.0886033429639,-5.592552058989,134.319678020622));
#274658=CARTESIAN_POINT('Ctrl Pts',(40.810155719151,-0.0653749034083074,
137.409647976851));
#274659=CARTESIAN_POINT('Ctrl Pts',(40.5317080953382,5.52187859466303,134.429681536124));
#274660=CARTESIAN_POINT('Ctrl Pts',(40.2532604715252,6.03479542300531,128.118222278014));
#274661=CARTESIAN_POINT('Ctrl Pts',(39.9748128477124,1.00203007375177,124.275192928799));
#274662=CARTESIAN_POINT('Ctrl Pts',(39.6963652238994,-4.95155196138904,
126.432149717987));
#274663=CARTESIAN_POINT('Ctrl Pts',(39.4179176000866,-6.35489964077443,
132.60695472951));
#274664=CARTESIAN_POINT('Ctrl Pts',(39.1394699762736,-1.91840500439501,
137.125263813774));
#274665=CARTESIAN_POINT('Ctrl Pts',(38.8610223524608,4.28101011172891,135.834971654011));
#274666=CARTESIAN_POINT('Ctrl Pts',(38.5825747286478,6.54638607414467,129.921793710766));
#274667=CARTESIAN_POINT('Ctrl Pts',(38.304127104835,2.79595304316033,124.819651639079));
#274668=CARTESIAN_POINT('Ctrl Pts',(38.0256794810221,-3.52382424458856,
125.217164749334));
#274669=CARTESIAN_POINT('Ctrl Pts',(37.7472318572093,-6.60537919994535,
130.749037912801));
#274670=CARTESIAN_POINT('Ctrl Pts',(37.4687842333963,-3.61691336126579,
136.331749939282));
#274671=CARTESIAN_POINT('Ctrl Pts',(37.1903366095834,2.69531916037638,136.835061207086));
#274672=CARTESIAN_POINT('Ctrl Pts',(36.9118889857706,6.53068504729366,131.796453249222));
#274673=CARTESIAN_POINT('Ctrl Pts',(36.6334413619576,4.36467041744916,125.846160629286));
#274674=CARTESIAN_POINT('Ctrl Pts',(36.3549937381448,-1.8122631000273,124.452211577043));
#274675=CARTESIAN_POINT('Ctrl Pts',(36.0765461143319,-6.32381536255287,
128.895577173308));
#274676=CARTESIAN_POINT('Ctrl Pts',(35.798098490519,-5.02409024244786,135.093021505591));
#274677=CARTESIAN_POINT('Ctrl Pts',(35.5196508667061,0.892528370013623,
137.34939599451));
#274678=CARTESIAN_POINT('Ctrl Pts',(35.2412032428932,5.98895701286753,133.591202714771));
#274679=CARTESIAN_POINT('Ctrl Pts',(34.9627556190803,5.58182673771145,127.272037692505));
#274680=CARTESIAN_POINT('Ctrl Pts',(34.6843079952674,0.0452703779943793,
124.198904874802));
#274681=CARTESIAN_POINT('Ctrl Pts',(34.4058603714545,-5.53288724751859,
127.195863190245));
#274682=CARTESIAN_POINT('Ctrl Pts',(34.1274127476417,-6.02659178913083,
133.508854356496));
#274683=CARTESIAN_POINT('Ctrl Pts',(33.8489651238287,-0.982152891908117,
137.336547898535));
#274684=CARTESIAN_POINT('Ctrl Pts',(33.5705175000158,4.96483653214189,135.161480444452));
#274685=CARTESIAN_POINT('Ctrl Pts',(33.292069876203,6.34938372890195,128.982432726597));
#274686=CARTESIAN_POINT('Ctrl Pts',(33.0136222523901,1.89915746344075,124.477647734417));
#274687=CARTESIAN_POINT('Ctrl Pts',(32.7351746285772,-4.29630173192265,
125.786802804744));
#274688=CARTESIAN_POINT('Ctrl Pts',(32.4567270047643,-6.543669521657,131.706848383727));
#274689=CARTESIAN_POINT('Ctrl Pts',(32.1782793809514,-2.77772469701646,
136.797551794587));
#274690=CARTESIAN_POINT('Ctrl Pts',(31.8998317571386,3.54081342478663,136.380805297429));
#274691=CARTESIAN_POINT('Ctrl Pts',(31.6213841333256,6.60551698756319,130.839578563946));
#274692=CARTESIAN_POINT('Ctrl Pts',(31.3429365095127,3.6000731362139,125.26598825823));
#274693=CARTESIAN_POINT('Ctrl Pts',(31.0644888856998,-2.71366205396602,
124.781891586214));
#274694=CARTESIAN_POINT('Ctrl Pts',(30.7860412618869,-6.53367438631237,
129.83214974004));
#274695=CARTESIAN_POINT('Ctrl Pts',(30.507593638074,-4.34955914537615,135.775822195171));
#274696=CARTESIAN_POINT('Ctrl Pts',(30.2291460142612,1.83158846238341,137.150964329883));
#274697=CARTESIAN_POINT('Ctrl Pts',(29.9506983904483,6.32959575128355,132.693887701803));
#274698=CARTESIAN_POINT('Ctrl Pts',(29.6722507666353,5.01101376269691,126.500427991838));
#274699=CARTESIAN_POINT('Ctrl Pts',(29.3938031428225,-0.912445072176531,
124.26207210612));
#274700=CARTESIAN_POINT('Ctrl Pts',(29.1153555190096,-5.99741146113971,
128.035759753857));
#274701=CARTESIAN_POINT('Ctrl Pts',(28.8369078951967,-5.57104970715349,
134.353656341672));
#274702=CARTESIAN_POINT('Ctrl Pts',(28.5584602713837,-0.0251654332018655,
137.409923551768));
#274703=CARTESIAN_POINT('Ctrl Pts',(28.280012647571,5.54384464446253,134.396001125022));
#274704=CARTESIAN_POINT('Ctrl Pts',(28.001565023758,6.0183323257333,128.081536533317));
#274705=CARTESIAN_POINT('Ctrl Pts',(27.7231173999451,0.962266611534229,
124.269214257685));
#274706=CARTESIAN_POINT('Ctrl Pts',(27.4446697761322,-4.97807510932732,
126.462372227135));
#274707=CARTESIAN_POINT('Ctrl Pts',(27.1662221523194,-6.34380899720599,
132.645605409466));
#274708=CARTESIAN_POINT('Ctrl Pts',(26.8877745285064,-1.87989232895117,
137.136824577849));
#274709=CARTESIAN_POINT('Ctrl Pts',(26.6093269046936,4.31155355176403,135.808818724794));
#274710=CARTESIAN_POINT('Ctrl Pts',(26.3308792808807,6.5408923495088,129.881960352566));
#274711=CARTESIAN_POINT('Ctrl Pts',(26.0524316570678,2.75947061841045,124.802742762115));
#274712=CARTESIAN_POINT('Ctrl Pts',(25.7739840332549,-3.55776980337282,
125.238718785491));
#274713=CARTESIAN_POINT('Ctrl Pts',(25.4955364094419,-6.60559358257403,
130.789247755823));
#274714=CARTESIAN_POINT('Ctrl Pts',(25.2170887856292,-3.58319956057628,
136.353664707793));
#274715=CARTESIAN_POINT('Ctrl Pts',(24.9386411618162,2.73197980856112,136.81854229942));
#274716=CARTESIAN_POINT('Ctrl Pts',(24.6601935380033,6.5366031982641,131.756680734531));
#274717=CARTESIAN_POINT('Ctrl Pts',(24.3817459141905,4.3344075795813,125.819683505575));
#274718=CARTESIAN_POINT('Ctrl Pts',(24.1032982903775,-1.85089685715453,
124.463361027524));
#274719=CARTESIAN_POINT('Ctrl Pts',(23.8248506665647,-6.33531750350378,
128.934107397669));
#274720=CARTESIAN_POINT('Ctrl Pts',(23.5464030427517,-4.99789086159903,
135.123525109951));
#274721=CARTESIAN_POINT('Ctrl Pts',(23.2679554189389,0.932353321572971,
137.343841656646));
#274722=CARTESIAN_POINT('Ctrl Pts',(22.9895077951259,6.00581035021119,133.554694599836));
#274723=CARTESIAN_POINT('Ctrl Pts',(22.7110601713131,5.56022106715229,127.238124974604));
#274724=CARTESIAN_POINT('Ctrl Pts',(22.4326125475002,0.00506025528043594,
124.198751684957));
#274725=CARTESIAN_POINT('Ctrl Pts',(22.1541649236873,-5.554750683987,127.229610302442));
#274726=CARTESIAN_POINT('Ctrl Pts',(21.8757172998744,-6.01001710932725,
133.545489823263));
#274727=CARTESIAN_POINT('Ctrl Pts',(21.5972696760615,-0.942371416853923,
137.342405515655));
#274728=CARTESIAN_POINT('Ctrl Pts',(21.3188220522486,4.99126757030501,135.131177347952));
#274729=CARTESIAN_POINT('Ctrl Pts',(21.0403744284357,6.33817549733007,128.943815981773));
#274730=CARTESIAN_POINT('Ctrl Pts',(20.7619268046228,1.86060977939589,124.466204243228));
#274731=CARTESIAN_POINT('Ctrl Pts',(20.48347918081,-4.32676542996233,125.813048576547));
#274732=CARTESIAN_POINT('Ctrl Pts',(20.205031556997,-6.5380545834274,131.746664836412));
#274733=CARTESIAN_POINT('Ctrl Pts',(19.9265839331841,-2.74119097644563,
136.814349553278));
#274734=CARTESIAN_POINT('Ctrl Pts',(19.6481363093713,3.57469322326559,136.359148042506));
#274735=CARTESIAN_POINT('Ctrl Pts',(19.3696886855584,6.60560898426828,130.799368254665));
#274736=CARTESIAN_POINT('Ctrl Pts',(19.0912410617455,3.56629279066743,125.244176204439));
#274737=CARTESIAN_POINT('Ctrl Pts',(18.8127934379326,-2.75027225446848,
124.798521999768));
#274738=CARTESIAN_POINT('Ctrl Pts',(18.5343458141197,-6.53947145601676,
129.871940083324));
#274739=CARTESIAN_POINT('Ctrl Pts',(18.2558981903068,-4.31921586042675,
135.802207086573));
#274740=CARTESIAN_POINT('Ctrl Pts',(17.9774505664939,1.87018810546999,137.139697343177));
#274741=CARTESIAN_POINT('Ctrl Pts',(17.6990029426811,6.34098056620813,132.65532264735));
#274742=CARTESIAN_POINT('Ctrl Pts',(17.4205553188681,4.98472166072295,126.470004270672));
#274743=CARTESIAN_POINT('Ctrl Pts',(17.1421076950552,-0.95225293377558,
124.26774763171));
#274744=CARTESIAN_POINT('Ctrl Pts',(16.8636600712423,-6.01415360227624,
128.072318995452));
#274745=CARTESIAN_POINT('Ctrl Pts',(16.5852124474295,-5.54934091802252,
134.387503142263));
#274746=CARTESIAN_POINT('Ctrl Pts',(16.3067648236166,0.0150449695187284,
137.409954355121));
#274747=CARTESIAN_POINT('Ctrl Pts',(16.0283171998036,5.56560526505998,134.362187624359));
#274748=CARTESIAN_POINT('Ctrl Pts',(15.7498695759908,6.00164621694371,128.044951683866));
#274749=CARTESIAN_POINT('Ctrl Pts',(15.4714219521779,0.922467492173741,
124.263477748823));
#274750=CARTESIAN_POINT('Ctrl Pts',(15.192974328365,-5.00441379286154,126.492755630261));
#274751=CARTESIAN_POINT('Ctrl Pts',(14.9145267045521,-6.33248328146239,
132.684187861418));
#274752=CARTESIAN_POINT('Ctrl Pts',(14.6360790807393,-1.84130999340576,
137.148150690142));
#274753=CARTESIAN_POINT('Ctrl Pts',(14.3576314569263,4.34193722559672,135.782480353541));
#274754=CARTESIAN_POINT('Ctrl Pts',(14.0791838331134,6.53515624970152,129.842161174248));
#274755=CARTESIAN_POINT('Ctrl Pts',(13.8007362093005,2.72288594046203,124.786056277307));
#274756=CARTESIAN_POINT('Ctrl Pts',(13.5222885854877,-3.59158352768866,
125.260479058552));
#274757=CARTESIAN_POINT('Ctrl Pts',(13.2438409616747,-6.60556319250329,
130.829458158858));
#274758=CARTESIAN_POINT('Ctrl Pts',(12.9653933378619,-3.54935298310934,
136.375373844801));
#274759=CARTESIAN_POINT('Ctrl Pts',(12.686945714049,2.76853922222938,136.801800534039));
#274760=CARTESIAN_POINT('Ctrl Pts',(12.4084980902361,6.5422791329992,131.716872931266));
#274761=CARTESIAN_POINT('Ctrl Pts',(12.1300504664232,4.30398412864651,125.793391090908));
#274762=CARTESIAN_POINT('Ctrl Pts',(11.8516028426103,-1.88946202861834,
124.474745446076));
#274763=CARTESIAN_POINT('Ctrl Pts',(11.5731552187974,-6.34658488693473,
128.972706924952));
#274764=CARTESIAN_POINT('Ctrl Pts',(11.2947075949845,-4.97150628206636,
135.153868666082));
#274765=CARTESIAN_POINT('Ctrl Pts',(11.0162599711716,0.972143724437105,
137.338044995907));
#274766=CARTESIAN_POINT('Ctrl Pts',(10.7378123473587,6.0224411400439,133.518084570262));
#274767=CARTESIAN_POINT('Ctrl Pts',(10.4593647235458,5.53840936055655,127.204344404875));
#274768=CARTESIAN_POINT('Ctrl Pts',(10.1809170997329,-0.0351500549433496,
124.198843268382));
#274769=CARTESIAN_POINT('Ctrl Pts',(9.90246947592002,-5.57640828712608,
127.263489878326));
#274770=CARTESIAN_POINT('Ctrl Pts',(9.62402185210712,-5.99321972612948,
133.582023716479));
#274771=CARTESIAN_POINT('Ctrl Pts',(9.34557422829421,-0.902555021880531,
137.348020863117));
#274772=CARTESIAN_POINT('Ctrl Pts',(9.06712660448133,5.01751365521256,135.100713919668));
#274773=CARTESIAN_POINT('Ctrl Pts',(8.78867898066847,6.32673240233446,128.905268180115));
#274774=CARTESIAN_POINT('Ctrl Pts',(8.51023135685555,1.82199314977141,124.454995614755));
#274775=CARTESIAN_POINT('Ctrl Pts',(8.23178373304265,-4.35706879811783,
125.839479303254));
#274776=CARTESIAN_POINT('Ctrl Pts',(7.9533361092298,-6.53219737518076,131.786446371669));
#274777=CARTESIAN_POINT('Ctrl Pts',(7.67488848541689,-2.70455568003535,
136.83092460962));
#274778=CARTESIAN_POINT('Ctrl Pts',(7.39644086160398,3.60844056017245,136.337284952891));
#274779=CARTESIAN_POINT('Ctrl Pts',(7.1179932377911,6.60545620770325,130.759158130379));
#274780=CARTESIAN_POINT('Ctrl Pts',(6.83954561397822,3.53238029483008,125.222570185327));
#274781=CARTESIAN_POINT('Ctrl Pts',(6.5610979901653,-2.78678054262086,124.815374961881));
#274782=CARTESIAN_POINT('Ctrl Pts',(6.28265036635242,-6.54502620320144,
129.911764977794));
#274783=CARTESIAN_POINT('Ctrl Pts',(6.00420274253956,-4.28871252534551,
135.828406780936));
#274784=CARTESIAN_POINT('Ctrl Pts',(5.72575511872663,1.90871844804856,137.128195598241));
#274785=CARTESIAN_POINT('Ctrl Pts',(5.44730749491374,6.35213041376593,132.616689004818));
#274786=CARTESIAN_POINT('Ctrl Pts',(5.16885987110085,4.95824484805471,126.439741160674));
#274787=CARTESIAN_POINT('Ctrl Pts',(4.89041224728798,-0.992025509291961,
124.273665373899));
#274788=CARTESIAN_POINT('Ctrl Pts',(4.61196462347505,-6.03067288673954,
128.108979473854));
#274789=CARTESIAN_POINT('Ctrl Pts',(4.33351699966218,-5.52742649602286,
134.421217168191));
#274790=CARTESIAN_POINT('Ctrl Pts',(4.05506937584931,0.0552548147426717,
137.409740385768));
#274791=CARTESIAN_POINT('Ctrl Pts',(3.77662175203639,5.58715965010757,134.328242287108));
#274792=CARTESIAN_POINT('Ctrl Pts',(3.49817412822347,5.98473771494644,128.008469085329));
#274793=CARTESIAN_POINT('Ctrl Pts',(3.21972650441063,0.882634190440881,
124.25798361478));
#274794=CARTESIAN_POINT('Ctrl Pts',(2.94127888059773,-5.03056703600248,
126.523298801495));
#274795=CARTESIAN_POINT('Ctrl Pts',(2.66283125678483,-6.32092291322184,
132.722700655682));
#274796=CARTESIAN_POINT('Ctrl Pts',(2.38438363297192,-1.80265942744139,
137.159241730961));
#274797=CARTESIAN_POINT('Ctrl Pts',(2.10593600915906,4.37216000734877,135.755957516231));
#274798=CARTESIAN_POINT('Ctrl Pts',(1.82748838534615,6.529177987276,129.802397650584));
#274799=CARTESIAN_POINT('Ctrl Pts',(1.54904076153325,2.68620036497402,124.769592802981));
#274800=CARTESIAN_POINT('Ctrl Pts',(1.27059313772038,-3.62526416455594,
125.282444762183));
#274801=CARTESIAN_POINT('Ctrl Pts',(0.992145513907496,-6.60528803085927,
130.869667631896));
#274802=CARTESIAN_POINT('Ctrl Pts',(0.713697890094564,-3.51537488306232,
136.396876545864));
#274803=CARTESIAN_POINT('Ctrl Pts',(0.435250266281723,2.80499604665836,
136.784836531317));
#274804=CARTESIAN_POINT('Ctrl Pts',(0.156802642468823,6.54771264117505,
131.677031314524));
#274805=CARTESIAN_POINT('Ctrl Pts',(-0.121644981344083,4.27340119199728,
125.767284359559));
#274806=CARTESIAN_POINT('Ctrl Pts',(-0.400092605156985,-1.92795718537184,
124.486364410847));
#274807=CARTESIAN_POINT('Ctrl Pts',(-0.678540228969845,-6.35761709532873,
129.011374324836));
#274808=CARTESIAN_POINT('Ctrl Pts',(-0.956987852782752,-4.94493748154019,
135.184051049593));
#274809=CARTESIAN_POINT('Ctrl Pts',(-1.23543547659566,1.01189810415772,
137.332006227089));
#274810=CARTESIAN_POINT('Ctrl Pts',(-1.51388310040852,6.03884876610542,
133.48137398265));
#274811=CARTESIAN_POINT('Ctrl Pts',(-1.79233072422142,5.51639242616521,
127.170697235071));
#274812=CARTESIAN_POINT('Ctrl Pts',(-2.07077834803434,-0.0753590626689394,
124.19917962168));
#274813=CARTESIAN_POINT('Ctrl Pts',(-2.34922597184723,-5.59785925440532,
127.297500662476));
#274814=CARTESIAN_POINT('Ctrl Pts',(-2.6276735956601,-5.97620026197078,
133.618454682368));
#274815=CARTESIAN_POINT('Ctrl Pts',(-2.906121219473,-0.862705182398668,
137.353393732843));
#274816=CARTESIAN_POINT('Ctrl Pts',(-3.18456884328591,5.04357381430661,
135.070091288433));
#274817=CARTESIAN_POINT('Ctrl Pts',(-3.46301646709877,6.31505486794284,
128.866790750024));
#274818=CARTESIAN_POINT('Ctrl Pts',(-3.74146409091167,1.78330900552073,
124.444022264336));
#274819=CARTESIAN_POINT('Ctrl Pts',(-4.01991171472458,-4.38721071348669,
125.866094005463));
#274820=CARTESIAN_POINT('Ctrl Pts',(-4.29835933853748,-6.52609811395827,
131.826191515377));
#274821=CARTESIAN_POINT('Ctrl Pts',(-4.57680696235032,-2.66782016531947,
136.847276349416));
#274822=CARTESIAN_POINT('Ctrl Pts',(-4.85525458616324,3.64205418498746,
136.31521683873));
#274823=CARTESIAN_POINT('Ctrl Pts',(-5.13370220997616,6.60505866352928,
130.718949681087));
#274824=CARTESIAN_POINT('Ctrl Pts',(-5.41214983378902,3.49833690534187,
125.201171001511));
#274825=CARTESIAN_POINT('Ctrl Pts',(-5.69059745760191,-2.82318556559566,
124.832449848059));
#274826=CARTESIAN_POINT('Ctrl Pts',(-5.96904508141481,-6.55033842203324,
129.951622947723));
#274827=CARTESIAN_POINT('Ctrl Pts',(-6.24749270522772,-4.2580502704442,
135.854420307421));
#274828=CARTESIAN_POINT('Ctrl Pts',(-6.52594032904057,1.9471780623631,137.116459521273));
#274829=CARTESIAN_POINT('Ctrl Pts',(-6.80438795285348,6.36304488079526,
132.577988205793));
#274830=CARTESIAN_POINT('Ctrl Pts',(-7.0828355766664,4.93158430580029,126.409639783256));
#274831=CARTESIAN_POINT('Ctrl Pts',(-7.36128320047925,-1.03176132493798,
124.279825113401));
#274832=CARTESIAN_POINT('Ctrl Pts',(-7.63973082429214,-6.04696870240127,
128.145739830595));
#274833=CARTESIAN_POINT('Ctrl Pts',(-7.91817844810507,-5.50530725320171,
134.454797170168));
#274834=CARTESIAN_POINT('Ctrl Pts',(-8.19662607191793,0.09546261247915,
137.40928165164));
#274835=CARTESIAN_POINT('Ctrl Pts',(-8.47507369573082,5.60850700089942,
134.294166371127));
#274836=CARTESIAN_POINT('Ctrl Pts',(-8.75352131954372,5.96760744629241,
127.972090089581));
#274837=CARTESIAN_POINT('Ctrl Pts',(-9.03196894335663,0.842768182373745,
124.252732059145));
#274838=CARTESIAN_POINT('Ctrl Pts',(-9.31041656716948,-5.05653386963193,
126.554000609049));
#274839=CARTESIAN_POINT('Ctrl Pts',(-9.5888641909824,-6.30912832085822,
132.76114236515));
#274840=CARTESIAN_POINT('Ctrl Pts',(-9.86731181479532,-1.76394206326903,
137.170097289323));
#274841=CARTESIAN_POINT('Ctrl Pts',(-10.1457594386081,4.40222077710389,
135.729251195677));
#274842=CARTESIAN_POINT('Ctrl Pts',(-10.424207062421,6.52295778375913,129.762671255026));
#274843=CARTESIAN_POINT('Ctrl Pts',(-10.7026546862339,2.64941525134336,
124.753352949195));
#274844=CARTESIAN_POINT('Ctrl Pts',(-10.9811023100469,-3.65881046592654,
125.304615082438));
#274845=CARTESIAN_POINT('Ctrl Pts',(-11.2595499338597,-6.60476810783814,
130.909874684957));
#274846=CARTESIAN_POINT('Ctrl Pts',(-11.5379975576726,-3.48126651950624,
136.418172014193));
#274847=CARTESIAN_POINT('Ctrl Pts',(-11.8164451814855,2.84134893092756,
136.767650919861));
#274848=CARTESIAN_POINT('Ctrl Pts',(-12.0948928052984,6.5529035214511,131.637157360647));
#274849=CARTESIAN_POINT('Ctrl Pts',(-12.3733404291112,4.2426599028951,125.741364278924));
#274850=CARTESIAN_POINT('Ctrl Pts',(-12.6517880529242,-1.96638090096281,
124.498217491291));
#274851=CARTESIAN_POINT('Ctrl Pts',(-12.9302356767371,-6.36841371988325,
129.050108164486));
#274852=CARTESIAN_POINT('Ctrl Pts',(-13.2086833005499,-4.91818544453708,
135.214071142064));
#274853=CARTESIAN_POINT('Ctrl Pts',(-13.4871309243628,1.05161498762227,
137.325725573964));
#274854=CARTESIAN_POINT('Ctrl Pts',(-13.7655785481758,6.05503262040511,
133.444564197323));
#274855=CARTESIAN_POINT('Ctrl Pts',(-14.0440261719886,5.49417107982388,
127.137184712));
#274856=CARTESIAN_POINT('Ctrl Pts',(-14.3224737958015,-0.115565277936756,
124.199760732389));
#274857=CARTESIAN_POINT('Ctrl Pts',(-14.6009214196144,-5.61910279095105,
127.331641394614));
#274858=CARTESIAN_POINT('Ctrl Pts',(-14.8793690434273,-5.95895934751375,
133.654781370965));
#274859=CARTESIAN_POINT('Ctrl Pts',(-15.1578166672402,-0.822823375059262,
137.358523925738));
#274860=CARTESIAN_POINT('Ctrl Pts',(-15.4362642910531,5.06944708191823,
135.039310588977));
#274861=CARTESIAN_POINT('Ctrl Pts',(-15.714711914866,6.3031433268707,128.828385117298));
#274862=CARTESIAN_POINT('Ctrl Pts',(-15.9931595386788,1.74455878009922,
124.433284598595));
#274863=CARTESIAN_POINT('Ctrl Pts',(-16.2716071624918,-4.41719005914895,
125.892891696959));
#274864=CARTESIAN_POINT('Ctrl Pts',(-16.5500547863046,-6.51975702577033,
131.865898794765));
#274865=CARTESIAN_POINT('Ctrl Pts',(-16.8285024101176,-2.63098579354628,
136.863404166748));
#274866=CARTESIAN_POINT('Ctrl Pts',(-17.1069500339304,3.67553285214529,
136.292944517765));
#274867=CARTESIAN_POINT('Ctrl Pts',(-17.3853976577434,6.60441636647752,
130.678744396729));
#274868=CARTESIAN_POINT('Ctrl Pts',(-17.6638452815562,3.46416388369313,
125.179979445948));
#274869=CARTESIAN_POINT('Ctrl Pts',(-17.9422929053691,-2.8594859743911,
124.849746025587));
#274870=CARTESIAN_POINT('Ctrl Pts',(-18.220740529182,-6.55540791566593,
129.991512516161));
#274871=CARTESIAN_POINT('Ctrl Pts',(-18.4991881529949,-4.22723023192423,
135.880246702087));
#274872=CARTESIAN_POINT('Ctrl Pts',(-18.7776357768078,1.98556552327847,
137.104489547159));
#274873=CARTESIAN_POINT('Ctrl Pts',(-19.0560834006207,6.37372356285652,
132.539221684343));
#274874=CARTESIAN_POINT('Ctrl Pts',(-19.3345310244336,4.90474102187576,
126.379701253833));
#274875=CARTESIAN_POINT('Ctrl Pts',(-19.6129786482465,-1.07145890828896,
124.286226621967));
#274876=CARTESIAN_POINT('Ctrl Pts',(-19.8914262720594,-6.06304044541393,
128.182598703507));
#274877=CARTESIAN_POINT('Ctrl Pts',(-20.1698738958722,-5.48298400919569,
134.488241903877));
#274878=CARTESIAN_POINT('Ctrl Pts',(-20.4483215196851,0.135666872813404,
137.408578169733));
#274879=CARTESIAN_POINT('Ctrl Pts',(-20.7267691434981,5.62964652640204,
134.25996113911));
#274880=CARTESIAN_POINT('Ctrl Pts',(-21.0052167673109,5.95025604574973,
127.935816044659));
#274881=CARTESIAN_POINT('Ctrl Pts',(-21.2836643911238,0.802870945221437,
124.247723276515));
#274882=CARTESIAN_POINT('Ctrl Pts',(-21.5621120149367,-5.08231333153929,
126.584859915257));
#274883=CARTESIAN_POINT('Ctrl Pts',(-21.8405596387496,-6.29709994142449,
132.79951156535));
#274884=CARTESIAN_POINT('Ctrl Pts',(-22.1190072625625,-1.725159335575,137.180716962973));
#274885=CARTESIAN_POINT('Ctrl Pts',(-22.3974548863754,4.43211842094896,
135.702362381491));
#274886=CARTESIAN_POINT('Ctrl Pts',(-22.6759025101882,6.51649586964294,
129.722983459651));
#274887=CARTESIAN_POINT('Ctrl Pts',(-22.9543501340012,2.61253196265622,
124.737337317723));
#274888=CARTESIAN_POINT('Ctrl Pts',(-23.232797757814,-3.6922211887298,125.326989197785));
#274889=CARTESIAN_POINT('Ctrl Pts',(-23.511245381627,-6.60400344270576,
130.950077828156));
#274890=CARTESIAN_POINT('Ctrl Pts',(-23.7896930054398,-3.4470291563393,
136.439259460675));
#274891=CARTESIAN_POINT('Ctrl Pts',(-24.0681406292527,2.87759652796706,
136.75024433649));
#274892=CARTESIAN_POINT('Ctrl Pts',(-24.3465882530656,6.55785158147733,
131.597252547181));
#274893=CARTESIAN_POINT('Ctrl Pts',(-24.6250358768785,4.21176140046998,
125.715631809479));
#274894=CARTESIAN_POINT('Ctrl Pts',(-24.9034835006914,-2.00473175158637,
124.510304248187));
#274895=CARTESIAN_POINT('Ctrl Pts',(-25.1819311245043,-6.3789743605254,
129.088907008606));
#274896=CARTESIAN_POINT('Ctrl Pts',(-25.4603787483172,-4.89125116236366,
135.24392783109));
#274897=CARTESIAN_POINT('Ctrl Pts',(-25.73882637213,1.09129290310671,137.319203269261));
#274898=CARTESIAN_POINT('Ctrl Pts',(-26.017273995943,6.07099210324431,133.407656578282));
#274899=CARTESIAN_POINT('Ctrl Pts',(-26.2957216197559,5.47174614495268,
127.103808077481));
#274900=CARTESIAN_POINT('Ctrl Pts',(-26.5741692435687,-0.155767210890682,
124.200586578976));
#274901=CARTESIAN_POINT('Ctrl Pts',(-26.8526168673816,-5.64013810957666,
127.365910809639));
#274902=CARTESIAN_POINT('Ctrl Pts',(-27.1310644911945,-5.94149762162655,
133.691002436174));
#274903=CARTESIAN_POINT('Ctrl Pts',(-27.4095121150075,-0.782911077696857,
137.363411251701));
#274904=CARTESIAN_POINT('Ctrl Pts',(-27.6879597388203,5.09513249930392,
135.008372961895));
#274905=CARTESIAN_POINT('Ctrl Pts',(-27.9664073626332,6.29099822050462,
128.79005270507));
#274906=CARTESIAN_POINT('Ctrl Pts',(-28.2448549864461,1.70574390941038,
124.422783015417));
#274907=CARTESIAN_POINT('Ctrl Pts',(-28.523302610259,-4.44700572420938,
125.919871384741));
#274908=CARTESIAN_POINT('Ctrl Pts',(-28.8017502340719,-6.51317434558802,
131.905566738465));
#274909=CARTESIAN_POINT('Ctrl Pts',(-29.0801978578848,-2.59405392962697,
136.879307463993));
#274910=CARTESIAN_POINT('Ctrl Pts',(-29.3586454816977,3.7088753210816,136.270468815306));
#274911=CARTESIAN_POINT('Ctrl Pts',(-29.6370931055106,6.6035293403484,130.638543767126));
#274912=CARTESIAN_POINT('Ctrl Pts',(-29.9155407293234,3.42986249617799,
125.158996303897));
#274913=CARTESIAN_POINT('Ctrl Pts',(-30.1939883531365,-2.89568042388203,
124.86726285355));
#274914=CARTESIAN_POINT('Ctrl Pts',(-30.4724359769491,-6.56023449624756,
130.031432204983));
#274915=CARTESIAN_POINT('Ctrl Pts',(-30.7508836007622,-4.19625355183344,
135.905885007927));
#274916=CARTESIAN_POINT('Ctrl Pts',(-31.029331224575,2.02387940833292,137.092286119451));
#274917=CARTESIAN_POINT('Ctrl Pts',(-31.3077788483879,6.38416606424714,
132.50039087698));
#274918=CARTESIAN_POINT('Ctrl Pts',(-31.5862264722008,4.8777159909692,126.349926681791));
#274919=CARTESIAN_POINT('Ctrl Pts',(-31.8646740960137,-1.11111678833609,
124.292869662384));
#274920=CARTESIAN_POINT('Ctrl Pts',(-32.1431217198266,-6.07888752023319,
128.219554726771));
#274921=CARTESIAN_POINT('Ctrl Pts',(-32.4215693436394,-5.46045759120085,
134.52155013001));
#274922=CARTESIAN_POINT('Ctrl Pts',(-32.7000169674524,0.175866105961793,
137.407629966116));
#274923=CARTESIAN_POINT('Ctrl Pts',(-32.9784645912652,5.65057744328232,
134.225627858545));
#274924=CARTESIAN_POINT('Ctrl Pts',(-33.2569122150782,5.93268415628106,
127.89964829471));
#274925=CARTESIAN_POINT('Ctrl Pts',(-33.535359838891,0.762943957391,124.242957452493));
#274926=CARTESIAN_POINT('Ctrl Pts',(-33.813807462704,-5.10790446645711,
126.615875576613));
#274927=CARTESIAN_POINT('Ctrl Pts',(-34.0922550865168,-6.28483822063666,
132.837806834499));
#274928=CARTESIAN_POINT('Ctrl Pts',(-34.3707027103298,-1.68631268146717,
137.191100358392));
#274929=CARTESIAN_POINT('Ctrl Pts',(-34.6491503341426,4.46185183101625,
135.675292070049));
#274930=CARTESIAN_POINT('Ctrl Pts',(-34.9275979579556,6.5097924843757,129.683335735103));
#274931=CARTESIAN_POINT('Ctrl Pts',(-35.2060455817684,2.57555186563646,
124.721546502031));
#274932=CARTESIAN_POINT('Ctrl Pts',(-35.4844932055813,-3.72549509491909,
125.349566279145));
#274933=CARTESIAN_POINT('Ctrl Pts',(-35.7629408293942,-6.60299406379731,
130.990275571749));
#274934=CARTESIAN_POINT('Ctrl Pts',(-36.0413884532071,-3.41266406223907,
136.460138103909));
#274935=CARTESIAN_POINT('Ctrl Pts',(-36.3198360770199,2.91373749460914,
136.73261742621));
#274936=CARTESIAN_POINT('Ctrl Pts',(-36.5982837008328,6.56255663790157,
131.557318352812));
#274937=CARTESIAN_POINT('Ctrl Pts',(-36.8767313246458,4.18070682967726,
125.690087904753));
#274938=CARTESIAN_POINT('Ctrl Pts',(-37.1551789484586,-2.04300831613737,
124.522624233657));
#274939=CARTESIAN_POINT('Ctrl Pts',(-37.4336265722715,-6.38929862592666,
129.12776941949));
#274940=CARTESIAN_POINT('Ctrl Pts',(-37.7120741960844,-4.86413563307991,
135.273620010322));
#274941=CARTESIAN_POINT('Ctrl Pts',(-37.9905218198973,1.13093038033133,
137.312439554669));
#274942=CARTESIAN_POINT('Ctrl Pts',(-38.2689694437102,6.0867266232385,133.370652493151));
#274943=CARTESIAN_POINT('Ctrl Pts',(-38.5474170675231,5.44911845251588,
127.070568568297));
#274944=CARTESIAN_POINT('Ctrl Pts',(-38.825864691336,-0.195963371833029,
124.201657130839));
#274945=CARTESIAN_POINT('Ctrl Pts',(-39.1043123151489,-5.66096443081045,
127.400307637685));
#274946=CARTESIAN_POINT('Ctrl Pts',(-39.3827599389617,-5.92381573136,133.727116535809));
#274947=CARTESIAN_POINT('Ctrl Pts',(-39.6612075627747,-0.742969769276543,
137.368055529631));
#274948=CARTESIAN_POINT('Ctrl Pts',(-39.9396551865875,5.12062911468111,
134.977279553588));
#274949=CARTESIAN_POINT('Ctrl Pts',(-40.2181028104005,6.27861999888597,
128.751794933764));
#274950=CARTESIAN_POINT('Ctrl Pts',(-40.4965504342133,1.66686583175366,
124.412517903944));
#274951=CARTESIAN_POINT('Ctrl Pts',(-40.7749980580263,-4.47665660383728,
125.947032069068));
#274952=CARTESIAN_POINT('Ctrl Pts',(-41.0534456818391,-6.5063503173351,
131.945193876568));
#274953=CARTESIAN_POINT('Ctrl Pts',(-41.3318933056519,-2.55702594208532,
136.894985651848));
#274954=CARTESIAN_POINT('Ctrl Pts',(-41.6103409294649,3.74208035627896,
136.247790564197));
#274955=CARTESIAN_POINT('Ctrl Pts',(-41.8887885532778,6.60239761801125,
130.598349281928));
#274956=CARTESIAN_POINT('Ctrl Pts',(-42.1672361770906,3.39543401384647,
125.138222352896));
#274957=CARTESIAN_POINT('Ctrl Pts',(-42.4456838009036,-2.93176757287012,
124.884999682853));
#274958=CARTESIAN_POINT('Ctrl Pts',(-42.7241314247165,-6.56481798492739,
130.071380534953));
#274959=CARTESIAN_POINT('Ctrl Pts',(-43.0025790485293,-4.16512137802412,
135.931334274905));
#274960=CARTESIAN_POINT('Ctrl Pts',(-43.2810266723423,2.06211829779186,
137.079849690351));
#274961=CARTESIAN_POINT('Ctrl Pts',(-43.5594742961552,6.39437199801655,
132.461497222591));
#274962=CARTESIAN_POINT('Ctrl Pts',(-43.837921919968,4.85051021450257,126.320317170437));
#274963=CARTESIAN_POINT('Ctrl Pts',(-44.116369543781,-1.150733495542,124.299753988494));
#274964=CARTESIAN_POINT('Ctrl Pts',(-44.3948171675938,-6.09450933963988,
128.256606530968));
#274965=CARTESIAN_POINT('Ctrl Pts',(-44.6732647914067,-5.43772883394191,
134.554720614319));
#274966=CARTESIAN_POINT('Ctrl Pts',(-44.9517124152196,0.216058822326645,
137.406437075925));
#274967=CARTESIAN_POINT('Ctrl Pts',(-45.2301600390324,5.67129897593744,
134.191167801664));
#274968=CARTESIAN_POINT('Ctrl Pts',(-45.5086076628454,5.91489242901924,
127.863588179946));
#274969=CARTESIAN_POINT('Ctrl Pts',(-45.7870552866582,0.722988698391639,
124.238434763679));
#274970=CARTESIAN_POINT('Ctrl Pts',(-46.0655029104712,-5.13330632609627,
126.647046443824));
#274971=CARTESIAN_POINT('Ctrl Pts',(-46.343950534284,-6.27234361285742,
132.876026753548));
#274972=CARTESIAN_POINT('Ctrl Pts',(-46.622398158097,-1.64740354042306,
137.201247090823));
#274973=CARTESIAN_POINT('Ctrl Pts',(-46.9008457819097,4.49141990552312,
135.64804126445));
#274974=CARTESIAN_POINT('Ctrl Pts',(-47.1792934057228,6.50284787635396,
129.643729550545));
#274975=CARTESIAN_POINT('Ctrl Pts',(-47.4577410295356,2.53847633059532,
124.705981087252));
#274976=CARTESIAN_POINT('Ctrl Pts',(-47.7361886533485,-3.75863095151733,
125.372345489915));
#274977=CARTESIAN_POINT('Ctrl Pts',(-48.0146362771614,-6.60174000851572,
131.030466426196));
#274978=CARTESIAN_POINT('Ctrl Pts',(-48.2930839009743,-3.37817251061699,
136.480807170229));
#274979=CARTESIAN_POINT('Ctrl Pts',(-48.5715315247872,2.94977049163681,
136.714770842195));
#274980=CARTESIAN_POINT('Ctrl Pts',(-48.8499791486,6.56701851637621,131.517356257317));
#274981=CARTESIAN_POINT('Ctrl Pts',(-49.128426772413,4.14949734125552,125.664733511282));
#274982=CARTESIAN_POINT('Ctrl Pts',(-49.4068743962258,-2.08120917626415,
124.535176991179));
#274983=CARTESIAN_POINT('Ctrl Pts',(-49.6853220200388,-6.39938613351776,
129.166693957078));
#274984=CARTESIAN_POINT('Ctrl Pts',(-49.9637696438516,-4.83683986146123,
135.303146579501));
#274985=CARTESIAN_POINT('Ctrl Pts',(-50.2422172676646,1.17052595051479,
137.305434680818));
#274986=CARTESIAN_POINT('Ctrl Pts',(-50.5206648914774,6.10223559733929,
133.333553313131));
#274987=CARTESIAN_POINT('Ctrl Pts',(-50.7991125152903,5.42628884099088,
127.03746741615));
#274988=CARTESIAN_POINT('Ctrl Pts',(-51.0775601391032,-0.236152271280866,
124.202972348307));
#274989=CARTESIAN_POINT('Ctrl Pts',(-51.3560077629162,-5.68158098292544,
127.434830604167));
#274990=CARTESIAN_POINT('Ctrl Pts',(-51.634455386729,-5.90591433192304,
133.763122331648));
#274991=CARTESIAN_POINT('Ctrl Pts',(-51.9129030105419,-0.703000929838195,
137.372456587432));
#274992=CARTESIAN_POINT('Ctrl Pts',(-52.1913506343548,5.14593598326309,
134.946031516236));
#274993=CARTESIAN_POINT('Ctrl Pts',(-52.4697982581677,6.26600912069438,
128.713613221033));
#274994=CARTESIAN_POINT('Ctrl Pts',(-52.7482458819806,1.62792598777083,
124.402489644555));
#274995=CARTESIAN_POINT('Ctrl Pts',(-53.0266935057934,-4.50614159930848,
125.97437274349));
#274996=CARTESIAN_POINT('Ctrl Pts',(-53.3051411296064,-6.49928519387843,
131.984778740675));
#274997=CARTESIAN_POINT('Ctrl Pts',(-53.5835887534191,-2.51990320300721,
136.910438149353));
#274998=CARTESIAN_POINT('Ctrl Pts',(-53.8620363772322,3.7751467273123,136.22491060479));
#274999=CARTESIAN_POINT('Ctrl Pts',(-54.140484001045,6.60102124140245,130.558162430556));
#275000=CARTESIAN_POINT('Ctrl Pts',(-54.418931624858,3.36087971245889,125.117658362733));
#275001=CARTESIAN_POINT('Ctrl Pts',(-54.6973792486707,-2.96774608413265,
124.902955856252));
#275002=CARTESIAN_POINT('Ctrl Pts',(-54.9758268724838,-6.56915821186243,
130.111356025769));
#275003=CARTESIAN_POINT('Ctrl Pts',(-55.2542744962966,-4.13383486411065,
135.956593559989));
#275004=CARTESIAN_POINT('Ctrl Pts',(-55.5327221201095,2.10028077469877,
137.067180720695));
#275005=CARTESIAN_POINT('Ctrl Pts',(-55.8111697439224,6.40434098598004,
132.422542162396));
#275006=CARTESIAN_POINT('Ctrl Pts',(-56.0896173677353,4.82312470059616,
126.29087381696));
#275007=CARTESIAN_POINT('Ctrl Pts',(-56.3680649915482,-1.19030756189505,
124.306879345194));
#275008=CARTESIAN_POINT('Ctrl Pts',(-56.646512615361,-6.10990532476174,
128.293752743129));
#275009=CARTESIAN_POINT('Ctrl Pts',(-56.924960239174,-5.41479857964128,
134.587752127659));
#275010=CARTESIAN_POINT('Ctrl Pts',(-57.2034078629868,0.256243532552689,
137.404999543363));
#275011=CARTESIAN_POINT('Ctrl Pts',(-57.4818554867998,5.69181035652338,
134.156582245398));
#275012=CARTESIAN_POINT('Ctrl Pts',(-57.7603031106126,5.89688152324325,
127.827637036585));
#275013=CARTESIAN_POINT('Ctrl Pts',(-58.0387507344255,0.683006648780185,
124.234155377662));
#275014=CARTESIAN_POINT('Ctrl Pts',(-58.3171983582384,-5.15851796918197,
126.67837136184));
#275015=CARTESIAN_POINT('Ctrl Pts',(-58.5956459820513,-6.25961658107885,
132.91416990625));
#275016=CARTESIAN_POINT('Ctrl Pts',(-58.8740936058642,-1.60843335423465,
137.211156784272));
#275017=CARTESIAN_POINT('Ctrl Pts',(-59.1525412296771,4.52082154881365,
135.620610974484));
#275018=CARTESIAN_POINT('Ctrl Pts',(-59.4309888534899,6.49566230291273,
129.604166373598));
#275019=CARTESIAN_POINT('Ctrl Pts',(-59.7094364773029,2.50130673138007,
124.69064165017));
#275020=CARTESIAN_POINT('Ctrl Pts',(-59.9878841011157,-3.79162753066369,
125.395325986002));
#275021=CARTESIAN_POINT('Ctrl Pts',(-60.2663317249287,-6.60024132333016,
131.070648902209));
#275022=CARTESIAN_POINT('Ctrl Pts',(-60.5447793487415,-3.34355577957023,
136.501265893734));
#275023=CARTESIAN_POINT('Ctrl Pts',(-60.8232269725544,2.98569418383416,
136.696705245755));
#275024=CARTESIAN_POINT('Ctrl Pts',(-61.1016745963673,6.57123705156454,
131.477367741508));
#275025=CARTESIAN_POINT('Ctrl Pts',(-61.3801222201802,4.11813409168408,
125.639569568584));
#275026=CARTESIAN_POINT('Ctrl Pts',(-61.6585698439931,-2.11933291641938,
124.547962055604));
#275027=CARTESIAN_POINT('Ctrl Pts',(-61.937017467806,-6.40923650950231,
129.205679179005));
#275028=CARTESIAN_POINT('Ctrl Pts',(-62.2154650916189,-4.80936485896274,
135.332506444514));
#275029=CARTESIAN_POINT('Ctrl Pts',(-62.4939127154318,1.21007814642843,
137.298188907278));
#275030=CARTESIAN_POINT('Ctrl Pts',(-62.7723603392447,6.1175184508558,133.296360412945));
#275031=CARTESIAN_POINT('Ctrl Pts',(-63.0508079630576,5.40325815633759,
127.004505847616));
#275032=CARTESIAN_POINT('Ctrl Pts',(-63.3292555868704,-0.276332420019459,
124.204532182646));
#275033=CARTESIAN_POINT('Ctrl Pts',(-63.6077032106833,-5.70198700196771,
127.469478429822));
#275034=CARTESIAN_POINT('Ctrl Pts',(-63.8861508344962,-5.8877940866586,
133.799018489484));
#275035=CARTESIAN_POINT('Ctrl Pts',(-64.1645984583092,-0.663006040441876,
137.376614262022));
#275036=CARTESIAN_POINT('Ctrl Pts',(-64.4430460821219,5.17105216729505,
134.914630007745));
#275037=CARTESIAN_POINT('Ctrl Pts',(-64.721493705935,6.25316605323042,128.675508981716));
#275038=CARTESIAN_POINT('Ctrl Pts',(-64.9999413297477,1.58892582039159,
124.392698608848));
#275039=CARTESIAN_POINT('Ctrl Pts',(-65.2783889535607,-4.53545961804555,
126.00189239489));
#275040=CARTESIAN_POINT('Ctrl Pts',(-65.5568365773735,-6.49197923701883,
132.024319863954));
#275041=CARTESIAN_POINT('Ctrl Pts',(-65.8352842011867,-2.48268708798906,
136.92566438391));
#275042=CARTESIAN_POINT('Ctrl Pts',(-66.1137318249993,3.80807320889562,
136.201829784909));
#275043=CARTESIAN_POINT('Ctrl Pts',(-66.3921794488124,6.59940026152389,
130.517984702147));
#275044=CARTESIAN_POINT('Ctrl Pts',(-66.6706270726251,3.3262008724376,125.097305095413));
#275045=CARTESIAN_POINT('Ctrl Pts',(-66.9490746964381,-3.00361462447264,
124.921130708376));
#275046=CARTESIAN_POINT('Ctrl Pts',(-67.227522320251,-6.57325501622426,
130.151357196124));
#275047=CARTESIAN_POINT('Ctrl Pts',(-67.5059699440638,-4.10239516942585,
135.981661927186));
#275048=CARTESIAN_POINT('Ctrl Pts',(-67.7844175678767,2.13836542492937,
137.054279679937));
#275049=CARTESIAN_POINT('Ctrl Pts',(-68.0628651916897,6.41407265873309,
132.383527139888));
#275050=CARTESIAN_POINT('Ctrl Pts',(-68.3413128155024,4.79556046403026,
126.261597712398));
#275051=CARTESIAN_POINT('Ctrl Pts',(-68.6197604393155,-1.22983752096341,
124.314245468451));
#275052=CARTESIAN_POINT('Ctrl Pts',(-68.8982080631282,-6.12507490509475,
128.330991986789));
#275053=CARTESIAN_POINT('Ctrl Pts',(-69.1766556869413,-5.39166767798822,
134.620643446035));
#275054=CARTESIAN_POINT('Ctrl Pts',(-69.455103310754,0.296418747580413,
137.403317421698));
#275055=CARTESIAN_POINT('Ctrl Pts',(-69.733550934567,5.7121108249834,134.121872471326));
#275056=CARTESIAN_POINT('Ctrl Pts',(-70.0119985583799,5.87865210635384,
127.791796196812));
#275057=CARTESIAN_POINT('Ctrl Pts',(-70.2904461821926,0.642999290106501,
124.230119453016));
#275058=CARTESIAN_POINT('Ctrl Pts',(-70.5688938060058,-5.18353846148724,
126.709849169906));
#275059=CARTESIAN_POINT('Ctrl Pts',(-70.8473414298183,-6.24665759690589,
132.95223487919));
#275060=CARTESIAN_POINT('Ctrl Pts',(-71.1257890536316,-1.56940356695681,
137.220829071533));
#275061=CARTESIAN_POINT('Ctrl Pts',(-71.4042366774442,4.55005567139915,
135.593002216589));
#275062=CARTESIAN_POINT('Ctrl Pts',(-71.6826843012574,6.48823603031619,
129.56464767029));
#275063=CARTESIAN_POINT('Ctrl Pts',(-71.9611319250699,2.46404444532374,
124.675528759193));
#275064=CARTESIAN_POINT('Ctrl Pts',(-72.2395795488831,-3.82448360965763,
125.418506915858));
#275065=CARTESIAN_POINT('Ctrl Pts',(-72.518027172696,-6.59849806377525,
131.110821510811));
#275066=CARTESIAN_POINT('Ctrl Pts',(-72.7964747965087,-3.30881515183405,
136.52151351632));
#275067=CARTESIAN_POINT('Ctrl Pts',(-73.0749224203217,3.02150724003593,
136.678421306317));
#275068=CARTESIAN_POINT('Ctrl Pts',(-73.3533700441346,6.57521208714753,
131.437354287172));
#275069=CARTESIAN_POINT('Ctrl Pts',(-73.6318176679474,4.08661824313884,
125.614597009117));
#275070=CARTESIAN_POINT('Ctrl Pts',(-73.9102652917603,-2.15737812391465,
124.56097895318));
#275071=CARTESIAN_POINT('Ctrl Pts',(-74.1887129155733,-6.41884938887091,
129.244723640663));
#275072=CARTESIAN_POINT('Ctrl Pts',(-74.4671605393861,-4.78171164368069,
135.361698517417));
#275073=CARTESIAN_POINT('Ctrl Pts',(-74.745608163199,1.24958550245192,137.290702502541));
#275074=CARTESIAN_POINT('Ctrl Pts',(-75.0240557870119,6.13257461747648,
133.25907517079));
#275075=CARTESIAN_POINT('Ctrl Pts',(-75.3025034108249,5.380027251966,126.971685084098));
#275076=CARTESIAN_POINT('Ctrl Pts',(-75.5809510346376,-0.31650232915867,
124.206336576053));
#275077=CARTESIAN_POINT('Ctrl Pts',(-75.8593986584506,-5.72218173178456,
127.504249830764));
#275078=CARTESIAN_POINT('Ctrl Pts',(-76.1378462822634,-5.86945566701928,
133.83480367917));
#275079=CARTESIAN_POINT('Ctrl Pts',(-76.4162939060764,-0.622986583113102,
137.380528399336));
#275080=CARTESIAN_POINT('Ctrl Pts',(-76.6947415298893,5.19597673608708,
134.88307619171));
#275081=CARTESIAN_POINT('Ctrl Pts',(-76.9731891537022,6.24009127239896,
128.637483627779));
#275082=CARTESIAN_POINT('Ctrl Pts',(-77.2516367775151,1.54986677478153,
124.383145159635));
#275083=CARTESIAN_POINT('Ctrl Pts',(-77.5300844013279,-4.56460957365852,
126.029590003516));
#275084=CARTESIAN_POINT('Ctrl Pts',(-77.8085320251407,-6.48443271748106,
132.063815781194));
#275085=CARTESIAN_POINT('Ctrl Pts',(-78.0869796489538,-2.44537897608793,
136.940663791305));
#275086=CARTESIAN_POINT('Ctrl Pts',(-78.3654272727665,3.84085858092573,
136.178548959823));
#275087=CARTESIAN_POINT('Ctrl Pts',(-78.6438748965796,6.5975347384416,130.477817585504));
#275088=CARTESIAN_POINT('Ctrl Pts',(-78.9223225203923,3.29139877882003,
125.077163305135));
#275089=CARTESIAN_POINT('Ctrl Pts',(-79.2007701442053,-3.03937186476788,
124.939523565746));
#275090=CARTESIAN_POINT('Ctrl Pts',(-79.4792177680182,-6.57710824620412,
130.191382563762));
#275091=CARTESIAN_POINT('Ctrl Pts',(-79.7576653918309,-4.07080345897965,
136.00653844758));
#275092=CARTESIAN_POINT('Ctrl Pts',(-80.036113015644,2.17637083724304,137.041147046131));
#275093=CARTESIAN_POINT('Ctrl Pts',(-80.314560639457,6.42356665566488,132.344453600785));
#275094=CARTESIAN_POINT('Ctrl Pts',(-80.5930082632696,4.76781852620778,
126.232489941585));
#275095=CARTESIAN_POINT('Ctrl Pts',(-80.8714558870828,-1.26932190795047,
124.321852085313));
#275096=CARTESIAN_POINT('Ctrl Pts',(-81.1499035108954,-6.14001751852468,
128.368322882032));
#275097=CARTESIAN_POINT('Ctrl Pts',(-81.4283511347085,-5.36833698610627,
134.653393350648));
#275098=CARTESIAN_POINT('Ctrl Pts',(-81.7067987585213,0.336582978702201,
137.401390773263));
#275099=CARTESIAN_POINT('Ctrl Pts',(-81.9852463823341,5.73219962907597,
134.087039765632));
#275100=CARTESIAN_POINT('Ctrl Pts',(-82.2636940061471,5.86020485384888,
127.756066988721));
#275101=CARTESIAN_POINT('Ctrl Pts',(-82.54214162996,0.602968104857597,124.226327139294));
#275102=CARTESIAN_POINT('Ctrl Pts',(-82.8205892537728,-5.20836687586887,
126.741478701599));
#275103=CARTESIAN_POINT('Ctrl Pts',(-83.0990368775859,-6.23346714053832,
132.990220261861));
#275104=CARTESIAN_POINT('Ctrl Pts',(-83.3774845013985,-1.53031562485268,
137.230263594196));
#275105=CARTESIAN_POINT('Ctrl Pts',(-83.6559321252116,4.57912118999838,
135.56521601382));
#275106=CARTESIAN_POINT('Ctrl Pts',(-83.9343797490243,6.48056933374724,
129.525174905002));
#275107=CARTESIAN_POINT('Ctrl Pts',(-84.2128273728376,2.42669085319518,
124.660642974335));
#275108=CARTESIAN_POINT('Ctrl Pts',(-84.4912749966499,-3.85719797100462,
125.441887420503));
#275109=CARTESIAN_POINT('Ctrl Pts',(-84.7697226204634,-6.59651029444787,
131.150982763393));
#275110=CARTESIAN_POINT('Ctrl Pts',(-85.0481702442759,-3.27395191473627,
136.541549287701));
#275111=CARTESIAN_POINT('Ctrl Pts',(-85.326617868089,3.05720833317481,136.659919701402));
#275112=CARTESIAN_POINT('Ctrl Pts',(-85.6050654919017,6.57894347582879,
131.397317377022));
#275113=CARTESIAN_POINT('Ctrl Pts',(-85.8835131157147,4.05495096345227,
125.58981675825));
#275114=CARTESIAN_POINT('Ctrl Pts',(-86.1619607395276,-2.19534338896908,
124.574227201559));
#275115=CARTESIAN_POINT('Ctrl Pts',(-86.4404083633404,-6.42822441541511,
129.283825895241));
#275116=CARTESIAN_POINT('Ctrl Pts',(-86.7188559871533,-4.75388124031539,
135.390721716488));
#275117=CARTESIAN_POINT('Ctrl Pts',(-86.9973036109663,1.28904655462414,
137.282975744021));
#275118=CARTESIAN_POINT('Ctrl Pts',(-87.2757512347791,6.14740353928957,
133.221698968287));
#275119=CARTESIAN_POINT('Ctrl Pts',(-87.554198858592,5.35659698870609,126.939006341782));
#275120=CARTESIAN_POINT('Ctrl Pts',(-87.8326464824051,-0.356660510187587,
124.208385461669));
#275121=CARTESIAN_POINT('Ctrl Pts',(-88.1110941062178,-5.74216442405318,
127.539143518524));
#275122=CARTESIAN_POINT('Ctrl Pts',(-88.3895417300309,-5.85089975254147,
133.870476574676));
#275123=CARTESIAN_POINT('Ctrl Pts',(-88.6679893538435,-0.582944040787213,
137.384198854334));
#275124=CARTESIAN_POINT('Ctrl Pts',(-88.9464369776566,5.22070876605056,
134.851371237371));
#275125=CARTESIAN_POINT('Ctrl Pts',(-89.2248846014694,6.22678526269035,
128.599538568266));
#275126=CARTESIAN_POINT('Ctrl Pts',(-89.5033322252823,1.51075029828878,
124.373829650922));
#275127=CARTESIAN_POINT('Ctrl Pts',(-89.7817798490951,-4.59359038598471,
126.057464543021));
#275128=CARTESIAN_POINT('Ctrl Pts',(-90.0602274729082,-6.47664591490472,
132.103265028861));
#275129=CARTESIAN_POINT('Ctrl Pts',(-90.338675096721,-2.40798024976945,
136.955435815729));
#275130=CARTESIAN_POINT('Ctrl Pts',(-90.6171227205338,3.87350162852866,
136.155068992212));
#275131=CARTESIAN_POINT('Ctrl Pts',(-90.8955703443469,6.59542474128344,
130.437662569033));
#275132=CARTESIAN_POINT('Ctrl Pts',(-91.1740179681596,3.25647472121003,
125.057233738258));
#275133=CARTESIAN_POINT('Ctrl Pts',(-91.4524655919725,-3.07501648002118,
124.958133746811));
#275134=CARTESIAN_POINT('Ctrl Pts',(-91.7309132157855,-6.58071775901922,
130.231430645527));
#275135=CARTESIAN_POINT('Ctrl Pts',(-92.0093608395982,-4.03906090341396,
136.031222199361));
#275136=CARTESIAN_POINT('Ctrl Pts',(-92.2878084634112,2.21429560333469,
137.027783305909));
#275137=CARTESIAN_POINT('Ctrl Pts',(-92.5662560872241,6.4328226249721,132.305322992969));
#275138=CARTESIAN_POINT('Ctrl Pts',(-92.844703711037,4.73989991511645,126.203551583122));
#275139=CARTESIAN_POINT('Ctrl Pts',(-93.1231513348499,-1.30875925974737,
124.329698913911));
#275140=CARTESIAN_POINT('Ctrl Pts',(-93.4015989586628,-6.15473261134757,
128.40574404555));
#275141=CARTESIAN_POINT('Ctrl Pts',(-93.6800465824757,-5.34480736852315,
134.686000627937));
#275142=CARTESIAN_POINT('Ctrl Pts',(-93.9584942062885,0.37673473761816,
137.399219669449));
#275143=CARTESIAN_POINT('Ctrl Pts',(-94.2369418301014,5.75207602440345,
134.052085419056));
#275144=CARTESIAN_POINT('Ctrl Pts',(-94.5153894539144,5.84154044929785,
127.720450736271));
#275145=CARTESIAN_POINT('Ctrl Pts',(-94.7938370777271,0.56291457640357,
124.222778577022));
#275146=CARTESIAN_POINT('Ctrl Pts',(-95.0722847015402,-5.23300229230026,
126.773258784876));
#275147=CARTESIAN_POINT('Ctrl Pts',(-95.350732325353,-6.22004570075364,
133.028124646699));
#275148=CARTESIAN_POINT('Ctrl Pts',(-95.6291799491659,-1.49117097634027,
137.239460002661));
#275149=CARTESIAN_POINT('Ctrl Pts',(-95.9076275729788,4.60801702757804,
135.537253395802));
#275150=CARTESIAN_POINT('Ctrl Pts',(-96.1860751967916,6.47266249729856,
129.48574954041));
#275151=CARTESIAN_POINT('Ctrl Pts',(-96.4645228206046,2.38924733914408,
124.645984847192));
#275152=CARTESIAN_POINT('Ctrl Pts',(-96.7429704444176,-3.88976940246256,
125.465466633565));
#275153=CARTESIAN_POINT('Ctrl Pts',(-97.0214180682302,-6.59427808900543,
131.191131171763));
#275154=CARTESIAN_POINT('Ctrl Pts',(-97.2998656920433,-3.23896736014657,
136.561372465446));
#275155=CARTESIAN_POINT('Ctrl Pts',(-97.5783133158561,3.09279614033489,
136.641201116591));
#275156=CARTESIAN_POINT('Ctrl Pts',(-97.856760939669,6.58243107933991,131.357258494642));
#275157=CARTESIAN_POINT('Ctrl Pts',(-98.135208563482,4.02313342606635,125.565229734223));
#275158=CARTESIAN_POINT('Ctrl Pts',(-98.4136561872948,-2.2332273047675,
124.587706309824));
#275159=CARTESIAN_POINT('Ctrl Pts',(-98.6921038111079,-6.43736124173946,
129.322984493793));
#275160=CARTESIAN_POINT('Ctrl Pts',(-98.9705514349205,-4.72587468013238,
135.419574966262));
#275161=CARTESIAN_POINT('Ctrl Pts',(-99.2489990587337,1.32845984070286,
137.275008918035));
#275162=CARTESIAN_POINT('Ctrl Pts',(-99.5274466825463,6.16200466680371,
133.184233190419));
#275163=CARTESIAN_POINT('Ctrl Pts',(-99.8058943063594,5.3329682347749,126.906470831589));
#275164=CARTESIAN_POINT('Ctrl Pts',(-100.084341930172,-0.396805475030165,
124.210678763569));
#275165=CARTESIAN_POINT('Ctrl Pts',(-100.362789553985,-5.76193433830736,
127.574158200105));
#275166=CARTESIAN_POINT('Ctrl Pts',(-100.641237177798,-5.83212703082168,
133.906035854126));
#275167=CARTESIAN_POINT('Ctrl Pts',(-100.919684801611,-0.542879897255484,
137.387625491007));
#275168=CARTESIAN_POINT('Ctrl Pts',(-101.198132425424,5.24524734073077,
134.819516319564));
#275169=CARTESIAN_POINT('Ctrl Pts',(-101.476580049237,6.21324851716398,
128.561675209245));
#275170=CARTESIAN_POINT('Ctrl Pts',(-101.75502767305,1.47157784038775,124.3647524279));
#275171=CARTESIAN_POINT('Ctrl Pts',(-102.033475296863,-4.62240098113028,
126.085514980508));
#275172=CARTESIAN_POINT('Ctrl Pts',(-102.311922920676,-6.4686191178319,
132.142666145147));
#275173=CARTESIAN_POINT('Ctrl Pts',(-102.590370544489,-2.3704922948573,
136.969979909799));
#275174=CARTESIAN_POINT('Ctrl Pts',(-102.868818168302,3.90600114210426,
136.131390752135));
#275175=CARTESIAN_POINT('Ctrl Pts',(-103.147265792114,6.59307034823604,
130.397521140692));
#275176=CARTESIAN_POINT('Ctrl Pts',(-103.425713415927,3.22142999373166,
125.037517133282));
#275177=CARTESIAN_POINT('Ctrl Pts',(-103.70416103974,-3.11054714940797,
124.976960561963));
#275178=CARTESIAN_POINT('Ctrl Pts',(-103.982608663553,-6.58408342091771,
130.271499957422));
#275179=CARTESIAN_POINT('Ctrl Pts',(-104.261056287366,-4.00716867896111,
136.055712267864));
#275180=CARTESIAN_POINT('Ctrl Pts',(-104.539503911179,2.25213831788793,
137.014188954471));
#275181=CARTESIAN_POINT('Ctrl Pts',(-104.817951534992,6.44184022367115,
132.266136766442));
#275182=CARTESIAN_POINT('Ctrl Pts',(-105.096399158805,4.71180566529118,
126.17478370933));
#275183=CARTESIAN_POINT('Ctrl Pts',(-105.374846782618,-1.34814811498862,
124.337785663482));
#275184=CARTESIAN_POINT('Ctrl Pts',(-105.65329440643,-6.16921963829011,
128.443254090687));
#275185=CARTESIAN_POINT('Ctrl Pts',(-105.931742030243,-5.32107969713743,
134.718464069627));
#275186=CARTESIAN_POINT('Ctrl Pts',(-106.210189654056,0.416872536489867,
137.396804190707));
#275187=CARTESIAN_POINT('Ctrl Pts',(-106.488637277869,5.77173927443855,
134.017010726842));
#275188=CARTESIAN_POINT('Ctrl Pts',(-106.767084901682,5.82265958431723,
127.684948759235));
#275189=CARTESIAN_POINT('Ctrl Pts',(-107.045532525495,0.52284018894291,
124.219473897692));
#275190=CARTESIAN_POINT('Ctrl Pts',(-107.323980149308,-5.25744379790729,
126.805188242113));
#275191=CARTESIAN_POINT('Ctrl Pts',(-107.602427773121,-6.20639377488812,
133.065946629143));
#275192=CARTESIAN_POINT('Ctrl Pts',(-107.880875396933,-1.45197107193893,
137.248417956151));
#275193=CARTESIAN_POINT('Ctrl Pts',(-108.159323020746,4.63674211339212,
135.509115398702));
#275194=CARTESIAN_POINT('Ctrl Pts',(-108.437770644559,6.46451581396073,
129.446373037437));
#275195=CARTESIAN_POINT('Ctrl Pts',(-108.716218268372,2.35171529065418,
124.631554920928));
#275196=CARTESIAN_POINT('Ctrl Pts',(-108.994665892185,-3.92219669708481,
125.489243681306));
#275197=CARTESIAN_POINT('Ctrl Pts',(-109.273113515998,-6.59180153016358,
131.231265248209));
#275198=CARTESIAN_POINT('Ctrl Pts',(-109.551561139811,-3.20386278442967,
136.580982315001));
#275199=CARTESIAN_POINT('Ctrl Pts',(-109.830008763624,3.12826934279688,
136.622266245509));
#275200=CARTESIAN_POINT('Ctrl Pts',(-110.108456387437,6.5856747684467,131.317179124427));
#275201=CARTESIAN_POINT('Ctrl Pts',(-110.38690401125,3.99116680999183,125.540836848117));
#275202=CARTESIAN_POINT('Ctrl Pts',(-110.665351635062,-2.27102846750687,
124.601415778499));
#275203=CARTESIAN_POINT('Ctrl Pts',(-110.943799258875,-6.44625952927566,
129.362197985281));
#275204=CARTESIAN_POINT('Ctrl Pts',(-111.222246882688,-4.69769300092514,
135.448257197571));
#275205=CARTESIAN_POINT('Ctrl Pts',(-111.500694506501,1.36782390021364,
137.266802319797));
#275206=CARTESIAN_POINT('Ctrl Pts',(-111.779142130314,6.17637745896884,
133.1466792255));
#275207=CARTESIAN_POINT('Ctrl Pts',(-112.057589754127,5.30914186574463,
126.874079759138));
#275208=CARTESIAN_POINT('Ctrl Pts',(-112.33603737794,-0.436935736099303,
124.213216396775));
#275209=CARTESIAN_POINT('Ctrl Pts',(-112.614485001753,-5.78149074196569,
127.609292578024));
#275210=CARTESIAN_POINT('Ctrl Pts',(-112.892932625565,-5.81313819748998,
133.94148019986));
#275211=CARTESIAN_POINT('Ctrl Pts',(-113.171380249379,-0.502795637109545,
137.390808182378));
#275212=CARTESIAN_POINT('Ctrl Pts',(-113.449827873191,5.26959155084185,
134.787512618686));
#275213=CARTESIAN_POINT('Ctrl Pts',(-113.728275497004,6.19948153742887,
128.523894953756));
#275214=CARTESIAN_POINT('Ctrl Pts',(-114.006723120817,1.43235085262869,
124.355913826926));
#275215=CARTESIAN_POINT('Ctrl Pts',(-114.28517074463,-4.65104029150761,
126.113740276555));
#275216=CARTESIAN_POINT('Ctrl Pts',(-114.563618368443,-6.46035262369882,
132.182017670029));
#275217=CARTESIAN_POINT('Ctrl Pts',(-114.842065992256,-2.33291650048142,
136.984295534578));
#275218=CARTESIAN_POINT('Ctrl Pts',(-115.120513616069,3.93835591737112,
136.107515116997));
#275219=CARTESIAN_POINT('Ctrl Pts',(-115.398961239881,6.59047164654225,
130.357394787938));
#275220=CARTESIAN_POINT('Ctrl Pts',(-115.677408863695,3.18626589498021,
125.018014220813));
#275221=CARTESIAN_POINT('Ctrl Pts',(-115.955856487507,-3.14596255632626,
124.996003313566));
#275222=CARTESIAN_POINT('Ctrl Pts',(-116.23430411132,-6.58720510718372,
130.311589014666));
#275223=CARTESIAN_POINT('Ctrl Pts',(-116.512751735133,-3.97512796739924,
136.0800077456));
#275224=CARTESIAN_POINT('Ctrl Pts',(-116.791199358946,2.28989757862811,
137.00036449556));
#275225=CARTESIAN_POINT('Ctrl Pts',(-117.069646982759,6.45061911761184,
132.226896373261));
#275226=CARTESIAN_POINT('Ctrl Pts',(-117.348094606572,4.68353681777373,
126.146187386213));
#275227=CARTESIAN_POINT('Ctrl Pts',(-117.626542230384,-1.38748701410568,
124.346112034364));
#275228=CARTESIAN_POINT('Ctrl Pts',(-117.904989854198,-6.18347806253024,
128.480851627495));
#275229=CARTESIAN_POINT('Ctrl Pts',(-118.18343747801,-5.29715485118671,
134.750782472776));
#275230=CARTESIAN_POINT('Ctrl Pts',(-118.461885101824,0.45699488799644,
137.394144426544));
#275231=CARTESIAN_POINT('Ctrl Pts',(-118.740332725636,5.79118865055225,
133.981816988697));
#275232=CARTESIAN_POINT('Ctrl Pts',(-119.018780349449,5.80356295854445,
127.649562373154));
#275233=CARTESIAN_POINT('Ctrl Pts',(-119.297227973262,0.482746427446748,
124.216413223762));
#275234=CARTESIAN_POINT('Ctrl Pts',(-119.575675597075,-5.28169048700048,
126.837265890154));
#275235=CARTESIAN_POINT('Ctrl Pts',(-119.854123220888,-6.19251186881905,
133.103684807684));
#275236=CARTESIAN_POINT('Ctrl Pts',(-120.132570844701,-1.41271736421608,
137.257137122728));
#275237=CARTESIAN_POINT('Ctrl Pts',(-120.411018468513,4.66529538302207,
135.480803065184));
#275238=CARTESIAN_POINT('Ctrl Pts',(-120.689466092327,6.45612958561205,
129.407046855192));
#275239=CARTESIAN_POINT('Ctrl Pts',(-120.967913716139,2.31409609848935,
124.61735373025));
#275240=CARTESIAN_POINT('Ctrl Pts',(-121.246361339953,-3.95447865326606,
125.51321768266));
#275241=CARTESIAN_POINT('Ctrl Pts',(-121.524808963765,-6.5890807096919,
131.271383505546));
#275242=CARTESIAN_POINT('Ctrl Pts',(-121.803256587578,-3.16863948839908,
136.600378109714));
#275243=CARTESIAN_POINT('Ctrl Pts',(-122.081704211391,3.16362662608795,
136.603115789794));
#275244=CARTESIAN_POINT('Ctrl Pts',(-122.360151835204,6.58867442295306,
131.277080751534));
#275245=CARTESIAN_POINT('Ctrl Pts',(-122.638599459017,3.9590522997634,125.51663900382));
#275246=CARTESIAN_POINT('Ctrl Pts',(-122.91704708283,-2.30874547645122,
124.615355099576));
#275247=CARTESIAN_POINT('Ctrl Pts',(-123.195494706643,-6.45491894829438,
129.401464916637));
#275248=CARTESIAN_POINT('Ctrl Pts',(-123.473942330455,-4.66933724697619,
135.476767347585));
#275249=CARTESIAN_POINT('Ctrl Pts',(-123.752389954268,1.40713727450679,
137.258356253404));
#275250=CARTESIAN_POINT('Ctrl Pts',(-124.030837578081,6.19052138319586,
133.109038465103));
#275251=CARTESIAN_POINT('Ctrl Pts',(-124.309285201894,5.28511876451003,
126.841834324687));
#275252=CARTESIAN_POINT('Ctrl Pts',(-124.587732825707,-0.477049806354697,
124.215998267256));
#275253=CARTESIAN_POINT('Ctrl Pts',(-124.86618044952,-5.80083291035842,
127.644545350364));
#275254=CARTESIAN_POINT('Ctrl Pts',(-125.144628073333,-5.79393395618462,
133.976808298475));
#275255=CARTESIAN_POINT('Ctrl Pts',(-125.423075697146,-0.462692745686338,
137.393746810514));
#275256=CARTESIAN_POINT('Ctrl Pts',(-125.701523320958,5.2937404943001,134.755361320645));
#275257=CARTESIAN_POINT('Ctrl Pts',(-125.979970944772,6.18548483362552,
128.486199201761));
#275258=CARTESIAN_POINT('Ctrl Pts',(-126.258418568584,1.39307078858202,
124.34731417552));
#275259=CARTESIAN_POINT('Ctrl Pts',(-126.536866192397,-4.67950725587653,
126.142139385264));
#275260=CARTESIAN_POINT('Ctrl Pts',(-126.81531381621,-6.45184673882346,
132.221318145323));
#275261=CARTESIAN_POINT('Ctrl Pts',(-127.093761440023,-2.29525425902701,
136.998382159598));
#275262=CARTESIAN_POINT('Ctrl Pts',(-127.372209063836,3.97056475541062,
136.083442971518));
#275263=CARTESIAN_POINT('Ctrl Pts',(-127.650656687649,6.58762873249828,
130.317284997668));
#275264=CARTESIAN_POINT('Ctrl Pts',(-127.929104311462,3.15098372797424,
124.998725723536));
#275265=CARTESIAN_POINT('Ctrl Pts',(-128.207551935275,-3.18126138844507,
125.015261295985));
#275266=CARTESIAN_POINT('Ctrl Pts',(-128.485999559087,-6.59008270214206,
130.351696331743));
#275267=CARTESIAN_POINT('Ctrl Pts',(-128.764447182901,-3.94293995600869,
136.104107732291));
#275268=CARTESIAN_POINT('Ctrl Pts',(-129.042894806713,2.32757198637139,
136.986310441447));
#275269=CARTESIAN_POINT('Ctrl Pts',(-129.321342430526,6.45915898148892,
132.187603267495));
#275270=CARTESIAN_POINT('Ctrl Pts',(-129.599790054339,4.6550944200771,126.117763673416));
#275271=CARTESIAN_POINT('Ctrl Pts',(-129.878237678152,-1.42677449938118,
124.354677718024));
#275272=CARTESIAN_POINT('Ctrl Pts',(-130.156685301965,-6.19750735571679,
128.518535262782));
#275273=CARTESIAN_POINT('Ctrl Pts',(-130.435132925778,-5.27303371721495,
134.782954639811));
#275274=CARTESIAN_POINT('Ctrl Pts',(-130.713580549591,0.497100305389368,
137.391240475519));
#275275=CARTESIAN_POINT('Ctrl Pts',(-130.992028173403,5.81042343204081,
133.946505508738));
#275276=CARTESIAN_POINT('Ctrl Pts',(-131.270475797217,5.78425127961196,
127.614292889281));
#275277=CARTESIAN_POINT('Ctrl Pts',(-131.548923421029,0.442634777604211,
124.213596668645));
#275278=CARTESIAN_POINT('Ctrl Pts',(-131.827371044842,-5.30574146111081,
126.869490540348));
#275279=CARTESIAN_POINT('Ctrl Pts',(-132.105818668655,-6.17840049694519,
133.141337783923));
#275280=CARTESIAN_POINT('Ctrl Pts',(-132.384266292468,-1.37341130773126,
137.265617179298));
#275281=CARTESIAN_POINT('Ctrl Pts',(-132.662713916281,4.69367577841589,
135.45231744437));
#275282=CARTESIAN_POINT('Ctrl Pts',(-132.941161540094,6.44750412300737,
129.367772450924));
#275283=CARTESIAN_POINT('Ctrl Pts',(-133.219609163907,2.27639115664257,
124.603381801387));
#275284=CARTESIAN_POINT('Ctrl Pts',(-133.49805678772,-3.98661407478655,
125.537387749261));
#275285=CARTESIAN_POINT('Ctrl Pts',(-133.776504411532,-6.58611572841139,
131.311484457178));
#275286=CARTESIAN_POINT('Ctrl Pts',(-134.054952035345,-3.13329877726696,
136.619559130867));
#275287=CARTESIAN_POINT('Ctrl Pts',(-134.333399659158,3.19886668003099,
136.583750459073));
#275288=CARTESIAN_POINT('Ctrl Pts',(-134.611847282971,6.59142993170542,
131.236964861823));
#275289=CARTESIAN_POINT('Ctrl Pts',(-134.890294906784,3.92679108539655,
125.492637097993));
#275290=CARTESIAN_POINT('Ctrl Pts',(-135.168742530597,-2.34637693398254,
124.629523756529));
#275291=CARTESIAN_POINT('Ctrl Pts',(-135.44719015441,-6.46333917791768,
129.440783832808));
#275292=CARTESIAN_POINT('Ctrl Pts',(-135.725637778223,-4.64080846901838,
135.505104359849));
#275293=CARTESIAN_POINT('Ctrl Pts',(-136.004085402036,1.44639850681073,
137.24967103183));
#275294=CARTESIAN_POINT('Ctrl Pts',(-136.282533025848,6.20443591537649,
133.07131230402));
#275295=CARTESIAN_POINT('Ctrl Pts',(-136.560980649661,5.26089982125598,
126.809735723105));
#275296=CARTESIAN_POINT('Ctrl Pts',(-136.839428273474,-0.517146199354053,
124.219024271924));
#275297=CARTESIAN_POINT('Ctrl Pts',(-137.117875897287,-5.81996012675442,
127.679915210822));
#275298=CARTESIAN_POINT('Ctrl Pts',(-137.3963235211,-5.77451501852576,134.012018840873));
#275299=CARTESIAN_POINT('Ctrl Pts',(-137.674771144913,-0.422572709013315,
137.396441266521));
#275300=CARTESIAN_POINT('Ctrl Pts',(-137.953218768726,5.31769327625758,
134.723063616821));
#275301=CARTESIAN_POINT('Ctrl Pts',(-138.231666392539,6.17125892440694,
128.448589350091));
#275302=CARTESIAN_POINT('Ctrl Pts',(-138.510114016352,1.35373910378499,
124.338953792345));
#275303=CARTESIAN_POINT('Ctrl Pts',(-138.788561640165,-4.70780081938319,
126.170711254294));
#275304=CARTESIAN_POINT('Ctrl Pts',(-139.067009263977,-6.44310177839452,
132.260566114734));
#275305=CARTESIAN_POINT('Ctrl Pts',(-139.34545688779,-2.25750696608163,
137.012239262869));
#275306=CARTESIAN_POINT('Ctrl Pts',(-139.623904511603,4.00262646271346,
136.059175207703));
#275307=CARTESIAN_POINT('Ctrl Pts',(-139.902352135416,6.5845417114487,130.277193256163));
#275308=CARTESIAN_POINT('Ctrl Pts',(-140.180799759229,3.11558480010749,
124.979652356196));
#275309=CARTESIAN_POINT('Ctrl Pts',(-140.459247383042,-3.21644233775325,
125.034733795609));
#275310=CARTESIAN_POINT('Ctrl Pts',(-140.737695006855,-6.59271609916233,
130.391820422461));
#275311=CARTESIAN_POINT('Ctrl Pts',(-141.016142630668,-3.91060583752806,
136.128011334905));
#275312=CARTESIAN_POINT('Ctrl Pts',(-141.294590254481,2.36516014507876,
136.97202731291));
#275313=CARTESIAN_POINT('Ctrl Pts',(-141.573037878293,6.46745949885459,
132.148258905163));
#275314=CARTESIAN_POINT('Ctrl Pts',(-141.851485502106,4.62647952614482,
126.089513624195));
#275315=CARTESIAN_POINT('Ctrl Pts',(-142.129933125919,-1.4660091150024,
124.363482397054));
#275316=CARTESIAN_POINT('Ctrl Pts',(-142.408380749732,-6.21130699798892,
128.556303600169));
#275317=CARTESIAN_POINT('Ctrl Pts',(-142.686828373545,-5.24871718904012,
134.814979378581));
#275318=CARTESIAN_POINT('Ctrl Pts',(-142.965275997358,0.537187302547703,
137.388092445238));
#275319=CARTESIAN_POINT('Ctrl Pts',(-143.243723621171,5.82944290615228,
133.911077595444));
#275320=CARTESIAN_POINT('Ctrl Pts',(-143.522171244983,5.76472526312116,
127.579141614542));
#275321=CARTESIAN_POINT('Ctrl Pts',(-143.800618868797,0.402506725767204,
124.21102433671));
#275322=CARTESIAN_POINT('Ctrl Pts',(-144.079066492609,-5.32959582902011,
126.901860998601));
#275323=CARTESIAN_POINT('Ctrl Pts',(-144.357514116423,-6.1640601821688,
133.178904162615));
#275324=CARTESIAN_POINT('Ctrl Pts',(-144.635961740235,-1.33405435898536,
137.27385781163));
#275325=CARTESIAN_POINT('Ctrl Pts',(-144.914409364048,4.72188224792766,
135.423659591808));
#275326=CARTESIAN_POINT('Ctrl Pts',(-145.192856987861,6.43863974576633,
129.328551279958));
#275327=CARTESIAN_POINT('Ctrl Pts',(-145.471304611674,2.23860186228433,
124.589639652074));
#275328=CARTESIAN_POINT('Ctrl Pts',(-145.749752235487,-4.01860177085642,
125.56175298548));
#275329=CARTESIAN_POINT('Ctrl Pts',(-146.0281998593,-6.58290669619051,131.35156661715));
#275330=CARTESIAN_POINT('Ctrl Pts',(-146.306647483113,-3.09784196059638,
136.638524667701));
#275331=CARTESIAN_POINT('Ctrl Pts',(-146.585095106925,3.2339881987928,136.564170970937));
#275332=CARTESIAN_POINT('Ctrl Pts',(-146.863542730738,6.59394119259793,
131.196832941802));
#275333=CARTESIAN_POINT('Ctrl Pts',(-147.141990354551,3.89438436234147,
125.468832020033));
#275334=CARTESIAN_POINT('Ctrl Pts',(-147.420437978364,-2.38392144565404,
124.643921224334));
#275335=CARTESIAN_POINT('Ctrl Pts',(-147.698885602177,-6.47151990613084,
129.480153276819));
#275336=CARTESIAN_POINT('Ctrl Pts',(-147.97733322599,-4.61210772419611,
135.533267184325));
#275337=CARTESIAN_POINT('Ctrl Pts',(-148.255780849803,1.48560614228611,
137.240746976909));
#275338=CARTESIAN_POINT('Ctrl Pts',(-148.534228473616,6.21812053990256,
133.033502140209));
#275339=CARTESIAN_POINT('Ctrl Pts',(-148.812676097428,5.23648593342438,
126.777785143819));
#275340=CARTESIAN_POINT('Ctrl Pts',(-149.091123721242,-0.557223429310831,
124.222294298654));
#275341=CARTESIAN_POINT('Ctrl Pts',(-149.369571345054,-5.83887168238761,
127.715400848752));
#275342=CARTESIAN_POINT('Ctrl Pts',(-149.648018968867,-5.75488210408933,
134.047110522317));
#275343=CARTESIAN_POINT('Ctrl Pts',(-149.92646659268,-0.382437013753756,
137.398891450554));
#275344=CARTESIAN_POINT('Ctrl Pts',(-150.204914216493,5.34144900913504,
134.690620704017));
#275345=CARTESIAN_POINT('Ctrl Pts',(-150.483361840306,6.15680433691945,
128.411066792389));
#275346=CARTESIAN_POINT('Ctrl Pts',(-150.761809464119,1.31435725568762,
124.330832987197));
#275347=CARTESIAN_POINT('Ctrl Pts',(-151.040257087932,-4.73591993359918,
126.199454824906));
#275348=CARTESIAN_POINT('Ctrl Pts',(-151.318704711745,-6.43411806645975,
132.299760123916));
#275349=CARTESIAN_POINT('Ctrl Pts',(-151.597152335558,-2.21967602038541,
137.025866330917));
#275350=CARTESIAN_POINT('Ctrl Pts',(-151.87559995937,4.03453985122072,136.034712724799));
#275351=CARTESIAN_POINT('Ctrl Pts',(-152.154047583183,6.58121069778455,
130.237121049039));
#275352=CARTESIAN_POINT('Ctrl Pts',(-152.432495206996,3.08007042310019,
124.960794825562));
#275353=CARTESIAN_POINT('Ctrl Pts',(-152.710942830809,-3.25150410060774,
125.054420090877));
#275354=CARTESIAN_POINT('Ctrl Pts',(-152.989390454622,-6.59510520066311,
130.431959800007));
#275355=CARTESIAN_POINT('Ctrl Pts',(-153.267838078435,-3.87812681010997,
136.151717667683));
#275356=CARTESIAN_POINT('Ctrl Pts',(-153.546285702248,2.40266066190714,
136.957515639215));
#275357=CARTESIAN_POINT('Ctrl Pts',(-153.824733326061,6.47552036213011,
132.108864744186));
#275358=CARTESIAN_POINT('Ctrl Pts',(-154.103180949873,4.59769319631231,
126.061438285362));
#275359=CARTESIAN_POINT('Ctrl Pts',(-154.381628573686,-1.50518940711724,
124.372525745196));
#275360=CARTESIAN_POINT('Ctrl Pts',(-154.660076197499,-6.22487647799626,
128.594155240135));
#275361=CARTESIAN_POINT('Ctrl Pts',(-154.938523821312,-5.22420616771914,
134.846855502398));
#275362=CARTESIAN_POINT('Ctrl Pts',(-155.216971445125,0.577254394032953,
137.384700452354));
#275363=CARTESIAN_POINT('Ctrl Pts',(-155.495419068938,5.84824636811312,
133.87553456161));
#275364=CARTESIAN_POINT('Ctrl Pts',(-155.773866692751,5.74498563261573,
127.544109851479));
#275365=CARTESIAN_POINT('Ctrl Pts',(-156.052314316564,0.362363758895462,
124.208696323275));
#275366=CARTESIAN_POINT('Ctrl Pts',(-156.330761940377,-5.353252706796,126.934376065411));
#275367=CARTESIAN_POINT('Ctrl Pts',(-156.60920956419,-6.14949145587554,
133.216382551721));
#275368=CARTESIAN_POINT('Ctrl Pts',(-156.887657188002,-1.29464797636456,
137.281858714364));
#275369=CARTESIAN_POINT('Ctrl Pts',(-157.166104811815,4.74991374635575,
135.394830569423));
#275370=CARTESIAN_POINT('Ctrl Pts',(-157.444552435628,6.42953678236183,
129.28938479565));
#275371=CARTESIAN_POINT('Ctrl Pts',(-157.723000059441,2.20072961571137,
124.576127791533));
#275372=CARTESIAN_POINT('Ctrl Pts',(-158.001447683254,-4.05044055615985,
125.586312488451));
#275373=CARTESIAN_POINT('Ctrl Pts',(-158.279895307067,-6.57945373194114,
131.391628500203));
#275374=CARTESIAN_POINT('Ctrl Pts',(-158.55834293088,-3.06227035225273,
136.657274017441));
#275375=CARTESIAN_POINT('Ctrl Pts',(-158.836790554693,3.2689898809326,136.54437805091));
#275376=CARTESIAN_POINT('Ctrl Pts',(-159.115238178505,6.59620811257463,
131.156686478575));
#275377=CARTESIAN_POINT('Ctrl Pts',(-159.393685802319,3.86183333144169,
125.445224652049));
#275378=CARTESIAN_POINT('Ctrl Pts',(-159.672133426131,-2.42137762023968,
124.658546969484));
#275379=CARTESIAN_POINT('Ctrl Pts',(-159.950581049944,-6.47946082979399,
129.519571789819));
#275380=CARTESIAN_POINT('Ctrl Pts',(-160.229028673757,-4.58323607602601,
135.56125477743));
#275381=CARTESIAN_POINT('Ctrl Pts',(-160.50747629757,1.52475872807955,137.231584419323));
#275382=CARTESIAN_POINT('Ctrl Pts',(-160.785923921383,6.23157474968534,
132.99560937474));
#275383=CARTESIAN_POINT('Ctrl Pts',(-161.064371545196,5.2118780056808,126.745983770767));
#275384=CARTESIAN_POINT('Ctrl Pts',(-161.342819169009,-0.597280011148509,
124.225808226271));
#275385=CARTESIAN_POINT('Ctrl Pts',(-161.621266792821,-5.85756687648338,
127.751000949223));
#275386=CARTESIAN_POINT('Ctrl Pts',(-161.899714416635,-5.73503594038016,
134.08208204247));
#275387=CARTESIAN_POINT('Ctrl Pts',(-162.178162040447,-0.342287147149402,
137.401097271823));
#275388=CARTESIAN_POINT('Ctrl Pts',(-162.45660966426,5.36500681265522,134.658033784415));
#275389=CARTESIAN_POINT('Ctrl Pts',(-162.735057288073,6.14212160678308,
128.373632919072));
#275390=CARTESIAN_POINT('Ctrl Pts',(-163.013504911886,1.27492670359879,
124.322952060995));
#275391=CARTESIAN_POINT('Ctrl Pts',(-163.291952535699,-4.76386355656041,
126.228369031995));
#275392=CARTESIAN_POINT('Ctrl Pts',(-163.570400159512,-6.42489593591386,
132.338898720518));
#275393=CARTESIAN_POINT('Ctrl Pts',(-163.848847783325,-2.18176282377798,
137.039262858781));
#275394=CARTESIAN_POINT('Ctrl Pts',(-164.127295407138,4.06630373837012,
136.010056429275));
#275395=CARTESIAN_POINT('Ctrl Pts',(-164.405743030951,6.57763581493773,
130.197069861187));
#275396=CARTESIAN_POINT('Ctrl Pts',(-164.684190654763,3.04444191295097,
124.942153830408));
#275397=CARTESIAN_POINT('Ctrl Pts',(-164.962638278576,-3.28644537778151,
125.074319452304));
#275398=CARTESIAN_POINT('Ctrl Pts',(-165.241085902389,-6.59724991811553,
130.472112977002));
#275399=CARTESIAN_POINT('Ctrl Pts',(-165.519533526202,-3.84550407727676,
136.175225852179));
#275400=CARTESIAN_POINT('Ctrl Pts',(-165.797981150015,2.44007214726114,
136.942775958099));
#275401=CARTESIAN_POINT('Ctrl Pts',(-166.076428773828,6.48334127261722,
132.069422244329));
#275402=CARTESIAN_POINT('Ctrl Pts',(-166.354876397641,4.56873649726763,
126.03353869726));
#275403=CARTESIAN_POINT('Ctrl Pts',(-166.633324021454,-1.54431392388507,
124.381807427344));
#275404=CARTESIAN_POINT('Ctrl Pts',(-166.911771645267,-6.23821529291649,
128.632088780075));
#275405=CARTESIAN_POINT('Ctrl Pts',(-167.19021926908,-5.19950156151742,
134.878581830081));
#275406=CARTESIAN_POINT('Ctrl Pts',(-167.468666892892,0.617300095144361,
137.381064622557));
#275407=CARTESIAN_POINT('Ctrl Pts',(-167.747114516705,5.86683312115408,
133.839877724298));
#275408=CARTESIAN_POINT('Ctrl Pts',(-168.025562140518,5.72503311955499,
127.509198898206));
#275409=CARTESIAN_POINT('Ctrl Pts',(-168.304009764331,0.32220736450136,
124.206612714607));
#275410=CARTESIAN_POINT('Ctrl Pts',(-168.582457388144,-5.37671121782417,
126.967034535923));
#275411=CARTESIAN_POINT('Ctrl Pts',(-168.860905011957,-6.1346948579149,
133.253771562468));
#275412=CARTESIAN_POINT('Ctrl Pts',(-169.13935263577,-1.25519362008691,
137.289619591024));
#275413=CARTESIAN_POINT('Ctrl Pts',(-169.417800259582,4.77776923498369,
135.365831445486));
#275414=CARTESIAN_POINT('Ctrl Pts',(-169.696247883396,6.42019557010726,
129.250274449328));
#275415=CARTESIAN_POINT('Ctrl Pts',(-169.974695507208,2.16277582029264,
124.562846720449));
#275416=CARTESIAN_POINT('Ctrl Pts',(-170.253143131021,-4.08212925089891,
125.611065348116));
#275417=CARTESIAN_POINT('Ctrl Pts',(-170.531590754834,-6.57575696361412,
131.431668621828));
#275418=CARTESIAN_POINT('Ctrl Pts',(-170.810038378647,-3.02658527035502,
136.675806485322));
#275419=CARTESIAN_POINT('Ctrl Pts',(-171.08848600246,3.30387042945021,136.524372432426));
#275420=CARTESIAN_POINT('Ctrl Pts',(-171.366933626273,6.59823060763395,
131.116526959784));
#275421=CARTESIAN_POINT('Ctrl Pts',(-171.645381250086,3.82913919888762,
125.421815868818));
#275422=CARTESIAN_POINT('Ctrl Pts',(-171.923828873899,-2.45874406978715,
124.673400450021));
#275423=CARTESIAN_POINT('Ctrl Pts',(-172.202276497711,-6.48716165465291,
129.559037911142));
#275424=CARTESIAN_POINT('Ctrl Pts',(-172.480724121525,-4.55419459435809,
135.589066102071));
#275425=CARTESIAN_POINT('Ctrl Pts',(-172.759171745337,1.5638548133772,137.222183698596));
#275426=CARTESIAN_POINT('Ctrl Pts',(-173.03761936915,6.24479804617409,132.957635411742));
#275427=CARTESIAN_POINT('Ctrl Pts',(-173.316066992963,5.18707694988104,
126.714332782362));
#275428=CARTESIAN_POINT('Ctrl Pts',(-173.594514616776,-0.637314460555731,
124.229565924566));
#275429=CARTESIAN_POINT('Ctrl Pts',(-173.872962240589,-5.8760450162844,
127.786714193059));
#275430=CARTESIAN_POINT('Ctrl Pts',(-174.151409864401,-5.71497726280517,
134.11693210545));
#275431=CARTESIAN_POINT('Ctrl Pts',(-174.429857488215,-0.302124596968923,
137.403058648589));
#275432=CARTESIAN_POINT('Ctrl Pts',(-174.708305112027,5.38836581387496,
134.625304065538));
#275433=CARTESIAN_POINT('Ctrl Pts',(-174.98675273584,6.1272112780718,128.336289117263));
#275434=CARTESIAN_POINT('Ctrl Pts',(-175.265200359654,1.2354489086321,124.315311305772));
#275435=CARTESIAN_POINT('Ctrl Pts',(-175.543647983466,-4.79163065280562,
126.257452804136));
#275436=CARTESIAN_POINT('Ctrl Pts',(-175.822095607279,-6.41543572848632,
132.377980454247));
#275437=CARTESIAN_POINT('Ctrl Pts',(-176.100543231092,-2.14376878114676,
137.05242835005));
#275438=CARTESIAN_POINT('Ctrl Pts',(-176.378990854905,4.09791694713909,
135.985207234778));
#275439=CARTESIAN_POINT('Ctrl Pts',(-176.657438478718,6.57381719537689,
130.157041176716));
#275440=CARTESIAN_POINT('Ctrl Pts',(-176.93588610253,3.00870058988678,124.923730061481));
#275441=CARTESIAN_POINT('Ctrl Pts',(-177.214333726344,-3.32126487451375,
125.094431142515));
#275442=CARTESIAN_POINT('Ctrl Pts',(-177.492781350156,-6.59915017204588,
130.512278465557));
#275443=CARTESIAN_POINT('Ctrl Pts',(-177.771228973969,-3.81273884787578,
136.198535017289));
#275444=CARTESIAN_POINT('Ctrl Pts',(-178.049676597782,2.47739321484437,
136.927808815745));
#275445=CARTESIAN_POINT('Ctrl Pts',(-178.328124221595,6.49092194050925,
132.029932867148));
#275446=CARTESIAN_POINT('Ctrl Pts',(-178.606571845408,4.53961050201187,
126.005815893719));
#275447=CARTESIAN_POINT('Ctrl Pts',(-178.885019469221,-1.58338121553252,
124.391327099562));
#275448=CARTESIAN_POINT('Ctrl Pts',(-179.163467093034,-6.25132294847495,
128.670102814346));
#275449=CARTESIAN_POINT('Ctrl Pts',(-179.441914716847,-5.1746042858732,
134.910157185999));
#275450=CARTESIAN_POINT('Ctrl Pts',(-179.72036234066,0.657322921973241,
137.377185090575));
#275451=CARTESIAN_POINT('Ctrl Pts',(-179.998809964472,5.88520247653593,
133.804108404782));
#275452=CARTESIAN_POINT('Ctrl Pts',(-180.277257588285,5.70486846328706,
127.474410048364));
#275453=CARTESIAN_POINT('Ctrl Pts',(-180.555705212098,0.282039030594865,
124.204773587913));
#275454=CARTESIAN_POINT('Ctrl Pts',(-180.834152835911,-5.39997049284089,
126.999835199963));
#275455=CARTESIAN_POINT('Ctrl Pts',(-181.112600459724,-6.11967093658025,
133.291069809391));
#275456=CARTESIAN_POINT('Ctrl Pts',(-181.391048083537,-1.21569275214809,
137.297140154028));
#275457=CARTESIAN_POINT('Ctrl Pts',(-181.669495707349,4.8054476816156,135.336663294571));
#275458=CARTESIAN_POINT('Ctrl Pts',(-181.947943331163,6.41061645514481,
129.21122169024));
#275459=CARTESIAN_POINT('Ctrl Pts',(-182.226390954976,2.12474188242055,
124.549796930959));
#275460=CARTESIAN_POINT('Ctrl Pts',(-182.504838578788,-4.11366668083735,
125.636010647245));
#275461=CARTESIAN_POINT('Ctrl Pts',(-182.783286202602,-6.5718165281946,
131.471685498325));
#275462=CARTESIAN_POINT('Ctrl Pts',(-183.061733826414,-2.99078803722709,
136.694121384618));
#275463=CARTESIAN_POINT('Ctrl Pts',(-183.340181450227,3.33862855183402,
136.5041548568));
#275464=CARTESIAN_POINT('Ctrl Pts',(-183.61862907404,6.60000860283161,131.076355873553));
#275465=CARTESIAN_POINT('Ctrl Pts',(-183.897076697853,3.79630317617236,
125.398606537762));
#275466=CARTESIAN_POINT('Ctrl Pts',(-184.175524321666,-2.49601940966891,
124.68848111554));
#275467=CARTESIAN_POINT('Ctrl Pts',(-184.453971945479,-6.49462209535141,
129.598550178357));
#275468=CARTESIAN_POINT('Ctrl Pts',(-184.732419569291,-4.52498435533419,
135.616700127691));
#275469=CARTESIAN_POINT('Ctrl Pts',(-185.010867193105,1.60289294946002,
137.212545163075));
#275470=CARTESIAN_POINT('Ctrl Pts',(-185.289314816917,6.25778993937471,
132.919581658354));
#275471=CARTESIAN_POINT('Ctrl Pts',(-185.56776244073,5.16208368503734,126.682833351442));
#275472=CARTESIAN_POINT('Ctrl Pts',(-185.846210064543,-0.677325294041226,
124.233567254297));
#275473=CARTESIAN_POINT('Ctrl Pts',(-186.124657688356,-5.89430541707644,
127.822539256894));
#275474=CARTESIAN_POINT('Ctrl Pts',(-186.403105312169,-5.69470681464601,
134.151659419877));
#275475=CARTESIAN_POINT('Ctrl Pts',(-186.681552935982,-0.261950851450417,
137.404775508174));
#275476=CARTESIAN_POINT('Ctrl Pts',(-186.960000559794,5.41152514721792,
134.592432760195));
#275477=CARTESIAN_POINT('Ctrl Pts',(-187.238448183608,6.11207390329327,
128.299036770752));
#275478=CARTESIAN_POINT('Ctrl Pts',(-187.51689580742,1.19592533365239,124.307911004657));
#275479=CARTESIAN_POINT('Ctrl Pts',(-187.795343431234,-4.81922019341476,
126.286705063617));
#275480=CARTESIAN_POINT('Ctrl Pts',(-188.073791055046,-6.40573779472858,
132.417003876913));
#275481=CARTESIAN_POINT('Ctrl Pts',(-188.352238678859,-2.10569530037498,
137.065362316871));
#275482=CARTESIAN_POINT('Ctrl Pts',(-188.630686302672,4.12937830608858,
135.960166062105));
#275483=CARTESIAN_POINT('Ctrl Pts',(-188.909133926485,6.56975498060235,
130.117036478904));
#275484=CARTESIAN_POINT('Ctrl Pts',(-189.187581550298,2.97284777831579,
124.905524201484));
#275485=CARTESIAN_POINT('Ctrl Pts',(-189.466029174111,-3.35596130055467,
125.114754416262));
#275486=CARTESIAN_POINT('Ctrl Pts',(-189.744476797923,-6.60080589203976,
130.552454777323));
#275487=CARTESIAN_POINT('Ctrl Pts',(-190.022924421737,-3.77983233603489,
136.221644299282));
#275488=CARTESIAN_POINT('Ctrl Pts',(-190.301372045549,2.5146224817104,136.912614766765));
#275489=CARTESIAN_POINT('Ctrl Pts',(-190.579819669362,6.49826208490189,
131.990398075938));
#275490=CARTESIAN_POINT('Ctrl Pts',(-190.858267293175,4.51031628981952,
125.978270902017));
#275491=CARTESIAN_POINT('Ctrl Pts',(-191.136714916988,-1.62238983440674,
124.401084409096));
#275492=CARTESIAN_POINT('Ctrl Pts',(-191.415162540801,-6.26419895896261,
128.708195934325));
#275493=CARTESIAN_POINT('Ctrl Pts',(-191.693610164614,-5.14951526336424,
134.941580400114));
#275494=CARTESIAN_POINT('Ctrl Pts',(-191.972057788427,0.697321391460013,
137.373062000163));
#275495=CARTESIAN_POINT('Ctrl Pts',(-192.25050541224,5.90335375357599,133.768227928508));
#275496=CARTESIAN_POINT('Ctrl Pts',(-192.528953036052,5.68449241101982,
127.439744591064));
#275497=CARTESIAN_POINT('Ctrl Pts',(-192.807400659866,0.241860245628379,
124.203179011344));
#275498=CARTESIAN_POINT('Ctrl Pts',(-193.085848283678,-5.42302966996514,
127.032776842093));
#275499=CARTESIAN_POINT('Ctrl Pts',(-193.364295907491,-6.10442024858855,
133.32827591039));
#275500=CARTESIAN_POINT('Ctrl Pts',(-193.642743531304,-1.17614683626724,
137.304420124699));
#275501=CARTESIAN_POINT('Ctrl Pts',(-193.921191155117,4.83294806061645,
135.307327197512));
#275502=CARTESIAN_POINT('Ctrl Pts',(-194.19963877893,6.40079979243214,129.172227965502));
#275503=CARTESIAN_POINT('Ctrl Pts',(-194.478086402743,2.08662921145659,
124.536978906625));
#275504=CARTESIAN_POINT('Ctrl Pts',(-194.756534026555,-4.14505167734362,
125.661147461485));
#275505=CARTESIAN_POINT('Ctrl Pts',(-195.034981650369,-6.5676325716969,
131.511677646851));
#275506=CARTESIAN_POINT('Ctrl Pts',(-195.313429274181,-2.95487997934909,
136.712218036662));
#275507=CARTESIAN_POINT('Ctrl Pts',(-195.591876897994,3.3732629601091,136.483726073203));
#275508=CARTESIAN_POINT('Ctrl Pts',(-195.870324521807,6.60154203228333,
131.03617470844));
#275509=CARTESIAN_POINT('Ctrl Pts',(-196.14877214562,3.76332648004682,125.375597518911));
#275510=CARTESIAN_POINT('Ctrl Pts',(-196.427219769433,-2.53320225863353,
124.703788407225));
#275511=CARTESIAN_POINT('Ctrl Pts',(-196.705667393246,-6.50184187543975,
129.63810712732));
#275512=CARTESIAN_POINT('Ctrl Pts',(-196.984115017059,-4.49560644135098,
135.644155830301));
#275513=CARTESIAN_POINT('Ctrl Pts',(-197.262562640871,1.64187168975517,
137.202669169918));
#275514=CARTESIAN_POINT('Ctrl Pts',(-197.541010264685,6.27054994786743,
132.881449524674));
#275515=CARTESIAN_POINT('Ctrl Pts',(-197.819457888497,5.13689913728475,
126.651486645231));
#275516=CARTESIAN_POINT('Ctrl Pts',(-198.097905512311,-0.717311028988463,
124.237812067191));
#275517=CARTESIAN_POINT('Ctrl Pts',(-198.376353136123,-5.91234740221361,
127.858474813215));
#275518=CARTESIAN_POINT('Ctrl Pts',(-198.654800759936,-5.67422534703162,
134.186262698915));
#275519=CARTESIAN_POINT('Ctrl Pts',(-198.933248383749,-0.221767399246752,
137.406247786956));
#275520=CARTESIAN_POINT('Ctrl Pts',(-199.211696007562,5.43448395450644,
134.559421086446));
#275521=CARTESIAN_POINT('Ctrl Pts',(-199.490143631375,6.09671004336861,
128.261877259937));
#275522=CARTESIAN_POINT('Ctrl Pts',(-199.768591255188,1.15635744321901,
124.300751431872));
#275523=CARTESIAN_POINT('Ctrl Pts',(-200.047038879001,-4.84663115604747,
126.316124726487));
#275524=CARTESIAN_POINT('Ctrl Pts',(-200.325486502814,-6.39580249400115,
132.455967542492));
#275525=CARTESIAN_POINT('Ctrl Pts',(-200.603934126626,-2.06754379228947,
137.078064279972));
#275526=CARTESIAN_POINT('Ctrl Pts',(-200.882381750439,4.16068664940635,
135.934933839164));
#275527=CARTESIAN_POINT('Ctrl Pts',(-201.160829374253,6.56544932114097,
130.077057250143));
#275528=CARTESIAN_POINT('Ctrl Pts',(-201.439276998065,2.9368848067771,124.887536925038));
#275529=CARTESIAN_POINT('Ctrl Pts',(-201.717724621878,-3.39053337021544,
125.13528852046));
#275530=CARTESIAN_POINT('Ctrl Pts',(-201.996172245691,-6.60221701674386,
130.592640423553));
#275531=CARTESIAN_POINT('Ctrl Pts',(-202.274619869504,-3.74678576111652,
136.244552841837));
#275532=CARTESIAN_POINT('Ctrl Pts',(-202.553067493317,2.55175856831618,
136.897194374181));
#275533=CARTESIAN_POINT('Ctrl Pts',(-202.83151511713,6.50536143380309,131.950819335672));
#275534=CARTESIAN_POINT('Ctrl Pts',(-203.109962740942,4.48085494619837,
125.950904742844));
#275535=CARTESIAN_POINT('Ctrl Pts',(-203.388410364755,-1.66133833502902,
124.411078994385));
#275536=CARTESIAN_POINT('Ctrl Pts',(-203.666857988568,-6.27684284725421,
128.746366728457));
#275537=CARTESIAN_POINT('Ctrl Pts',(-203.945305612381,-5.12423542367342,
134.97285030803));
#275538=CARTESIAN_POINT('Ctrl Pts',(-204.223753236194,0.737294021446153,
137.368695504108));
#275539=CARTESIAN_POINT('Ctrl Pts',(-204.502200860007,5.9212862796718,133.732237625041));
#275540=CARTESIAN_POINT('Ctrl Pts',(-204.78064848382,5.66390571779574,127.405203810847));
#275541=CARTESIAN_POINT('Ctrl Pts',(-205.059096107633,0.20167249844203,
124.201829043986));
#275542=CARTESIAN_POINT('Ctrl Pts',(-205.337543731446,-5.44588789473034,
127.065858241646));
#275543=CARTESIAN_POINT('Ctrl Pts',(-205.615991355258,-6.08894335906002,
133.36538848678));
#275544=CARTESIAN_POINT('Ctrl Pts',(-205.894438979071,-1.13655733783284,
137.311459233274));
#275545=CARTESIAN_POINT('Ctrl Pts',(-206.172886602884,4.86026935294961,
135.277824241371));
#275546=CARTESIAN_POINT('Ctrl Pts',(-206.451334226697,6.39074594572923,
129.133294720038));
#275547=CARTESIAN_POINT('Ctrl Pts',(-206.72978185051,2.04843921967989,124.524393122426));
#275548=CARTESIAN_POINT('Ctrl Pts',(-207.008229474323,-4.17628307743617,
125.686474859378));
#275549=CARTESIAN_POINT('Ctrl Pts',(-207.286677098136,-6.56320524915893,
131.551643585487));
#275550=CARTESIAN_POINT('Ctrl Pts',(-207.565124721949,-2.9188624273063,
136.730095770877));
#275551=CARTESIAN_POINT('Ctrl Pts',(-207.843572345762,3.40777237088467,
136.463086838631));
#275552=CARTESIAN_POINT('Ctrl Pts',(-208.122019969575,6.60283083916734,
130.995984953369));
#275553=CARTESIAN_POINT('Ctrl Pts',(-208.400467593387,3.73021033247459,
125.352789664874));
#275554=CARTESIAN_POINT('Ctrl Pts',(-208.678915217201,-2.57029123885685,
124.719321757855));
#275555=CARTESIAN_POINT('Ctrl Pts',(-208.957362841013,-6.50882072738636,
129.677707292235));
#275556=CARTESIAN_POINT('Ctrl Pts',(-209.235810464827,-4.4660619410178,
135.671432192519));
#275557=CARTESIAN_POINT('Ctrl Pts',(-209.514258088639,1.68078958989102,
137.192556085085));
#275558=CARTESIAN_POINT('Ctrl Pts',(-209.792705712452,6.28307759882623,
132.8432404237));
#275559=CARTESIAN_POINT('Ctrl Pts',(-210.071153336265,5.11152423984512,
126.620293825292));
#275560=CARTESIAN_POINT('Ctrl Pts',(-210.349600960078,-0.757270183712145,
124.242300205957));
#275561=CARTESIAN_POINT('Ctrl Pts',(-210.62804858389,-5.93017030314353,
127.894519530418));
#275562=CARTESIAN_POINT('Ctrl Pts',(-210.906496207704,-5.65353361891029,
134.220740660327));
#275563=CARTESIAN_POINT('Ctrl Pts',(-211.184943831516,-0.181575729370575,
137.407475430382));
#275564=CARTESIAN_POINT('Ctrl Pts',(-211.463391455329,5.4572413849935,134.52627026755));
#275565=CARTESIAN_POINT('Ctrl Pts',(-211.741839079142,6.08112026761121,
128.224811961777));
#275566=CARTESIAN_POINT('Ctrl Pts',(-212.020286702955,1.11674670353533,
124.293832852717));
#275567=CARTESIAN_POINT('Ctrl Pts',(-212.298734326768,-4.87386252498038,
126.345710702588));
#275568=CARTESIAN_POINT('Ctrl Pts',(-212.577181950581,-6.38563019446009,
132.494870007167));
#275569=CARTESIAN_POINT('Ctrl Pts',(-212.855629574394,-2.02931567060901,
137.090533768676));
#275570=CARTESIAN_POINT('Ctrl Pts',(-213.134077198207,4.19184081695006,
135.909511500946));
#275571=CARTESIAN_POINT('Ctrl Pts',(-213.412524822019,6.56090037654053,
130.037104971874));
#275572=CARTESIAN_POINT('Ctrl Pts',(-213.690972445832,2.90081300789186,
124.869768898671));
#275573=CARTESIAN_POINT('Ctrl Pts',(-213.969420069645,-3.42497980241531,
125.156032694208));
#275574=CARTESIAN_POINT('Ctrl Pts',(-214.247867693459,-6.60338349386843,
130.632833915152));
#275575=CARTESIAN_POINT('Ctrl Pts',(-214.52631531727,-3.71360034767391,
136.267259796069));
#275576=CARTESIAN_POINT('Ctrl Pts',(-214.804762941084,2.58880009856982,
136.881548209402));
#275577=CARTESIAN_POINT('Ctrl Pts',(-215.083210564897,6.51221972414398,
131.911198112957));
#275578=CARTESIAN_POINT('Ctrl Pts',(-215.36165818871,4.45122756284936,125.923718430264));
#275579=CARTESIAN_POINT('Ctrl Pts',(-215.640105812523,-1.70022527414834,
124.421310485075));
#275580=CARTESIAN_POINT('Ctrl Pts',(-215.918553436335,-6.28925414482577,
128.784613782311));
#275581=CARTESIAN_POINT('Ctrl Pts',(-216.197001060149,-5.09876570355457,
135.003965751026));
#275582=CARTESIAN_POINT('Ctrl Pts',(-216.475448683961,0.77723933073121,
137.364085764208));
#275583=CARTESIAN_POINT('Ctrl Pts',(-216.753896307774,5.93899939032692,
133.696138828015));
#275584=CARTESIAN_POINT('Ctrl Pts',(-217.032343931587,5.64310914646246,
127.370788987637));
#275585=CARTESIAN_POINT('Ctrl Pts',(-217.3107915554,0.161477278206604,124.200723735865));
#275586=CARTESIAN_POINT('Ctrl Pts',(-217.589239179213,-5.46854432011718,
127.099078172778));
#275587=CARTESIAN_POINT('Ctrl Pts',(-217.867686803026,-6.07324084149572,
133.402406163341));
#275588=CARTESIAN_POINT('Ctrl Pts',(-218.146134426838,-1.09692572384833,
137.318257218917));
#275589=CARTESIAN_POINT('Ctrl Pts',(-218.424582050652,4.88741054621452,
135.24815551939));
#275590=CARTESIAN_POINT('Ctrl Pts',(-218.703029674464,6.38045528758512,
129.094423396537));
#275591=CARTESIAN_POINT('Ctrl Pts',(-218.981477298277,2.01017332223456,
124.512040044732));
#275592=CARTESIAN_POINT('Ctrl Pts',(-219.25992492209,-4.20735972382344,
125.711991902411));
#275593=CARTESIAN_POINT('Ctrl Pts',(-219.538372545903,-6.55853472463687,
131.591581833275));
#275594=CARTESIAN_POINT('Ctrl Pts',(-219.816820169716,-2.8827367157428,
136.747753924796));
#275595=CARTESIAN_POINT('Ctrl Pts',(-220.095267793529,3.44215550540127,
136.442237917877));
#275596=CARTESIAN_POINT('Ctrl Pts',(-220.373715417342,6.60387497572639,
130.955788097589));
#275597=CARTESIAN_POINT('Ctrl Pts',(-220.652163041155,3.69695596058723,
125.330183820803));
#275598=CARTESIAN_POINT('Ctrl Pts',(-220.930610664968,-2.60728497599312,
124.735080591838));
#275599=CARTESIAN_POINT('Ctrl Pts',(-221.20905828878,-6.51555839258729,
129.717349205704));
#275600=CARTESIAN_POINT('Ctrl Pts',(-221.487505912593,-4.43635194911701,
135.698528203611));
#275601=CARTESIAN_POINT('Ctrl Pts',(-221.765953536406,1.71964520775051,
137.182206283321));
#275602=CARTESIAN_POINT('Ctrl Pts',(-222.044401160219,6.295372428034,132.804955771283));
#275603=CARTESIAN_POINT('Ctrl Pts',(-222.322848784032,5.08595993299503,
126.589256047487));
#275604=CARTESIAN_POINT('Ctrl Pts',(-222.601296407845,-0.797201277510683,
124.247031504286));
#275605=CARTESIAN_POINT('Ctrl Pts',(-222.879744031658,-5.94777345943203,
127.930672072853));
#275606=CARTESIAN_POINT('Ctrl Pts',(-223.158191655471,-5.63263239702162,
134.255092026522));
#275607=CARTESIAN_POINT('Ctrl Pts',(-223.436639279283,-0.141377331138957,
137.40845839296));
#275608=CARTESIAN_POINT('Ctrl Pts',(-223.715086903097,5.47979659539413,
134.492981531924));
#275609=CARTESIAN_POINT('Ctrl Pts',(-223.993534526909,6.06530515370598,
128.187842249741));
#275610=CARTESIAN_POINT('Ctrl Pts',(-224.271982150722,1.07709458239186,
124.287155523561));
#275611=CARTESIAN_POINT('Ctrl Pts',(-224.550429774535,-4.90091329114502,
126.375461895601));
#275612=CARTESIAN_POINT('Ctrl Pts',(-224.828877398348,-6.37522127304402,
132.533709829396));
#275613=CARTESIAN_POINT('Ctrl Pts',(-225.107325022161,-1.99101235188949,
137.102770320923));
#275614=CARTESIAN_POINT('Ctrl Pts',(-225.385772645974,4.22283965429091,
135.883899989486));
#275615=CARTESIAN_POINT('Ctrl Pts',(-225.664220269787,6.55610831536389,
129.997181124546));
#275616=CARTESIAN_POINT('Ctrl Pts',(-225.9426678936,2.86463371831382,124.852220780782));
#275617=CARTESIAN_POINT('Ctrl Pts',(-226.221115517412,-3.45929932072906,
125.176986168825));
#275618=CARTESIAN_POINT('Ctrl Pts',(-226.499563141226,-6.60430528018926,
130.673033762736));
#275619=CARTESIAN_POINT('Ctrl Pts',(-226.778010765038,-3.68027732540471,
136.289764320562));
#275620=CARTESIAN_POINT('Ctrl Pts',(-227.056458388851,2.62574569988376,
136.865676852203));
#275621=CARTESIAN_POINT('Ctrl Pts',(-227.334906012664,6.51883670178814,
131.871535875972));
#275622=CARTESIAN_POINT('Ctrl Pts',(-227.613353636477,4.42143523762624,
125.896712971676));
#275623=CARTESIAN_POINT('Ctrl Pts',(-227.89180126029,-1.73904921079426,
124.431778502036));
#275624=CARTESIAN_POINT('Ctrl Pts',(-228.170248884103,-6.30143239177224,
128.822935678624));
#275625=CARTESIAN_POINT('Ctrl Pts',(-228.448696507916,-5.07310704679746,
135.034925576111));
#275626=CARTESIAN_POINT('Ctrl Pts',(-228.727144131728,0.81715583912702,
137.359232951281));
#275627=CARTESIAN_POINT('Ctrl Pts',(-229.005591755541,5.95649242917557,
133.659932875084));
#275628=CARTESIAN_POINT('Ctrl Pts',(-229.284039379354,5.62210346764449,
127.336501396687));
#275629=CARTESIAN_POINT('Ctrl Pts',(-229.562487003167,0.121276074371264,
124.199863127936));
#275630=CARTESIAN_POINT('Ctrl Pts',(-229.84093462698,-5.4909981065832,127.132435404515));
#275631=CARTESIAN_POINT('Ctrl Pts',(-230.119382250793,-6.0573132777586,
133.439327568368));
#275632=CARTESIAN_POINT('Ctrl Pts',(-230.397829874606,-1.05725346287773,
137.324813829725));
#275633=CARTESIAN_POINT('Ctrl Pts',(-230.676277498418,4.91437063468431,
135.218322130955));
#275634=CARTESIAN_POINT('Ctrl Pts',(-230.954725122232,6.3699281993239,129.055615435388));
#275635=CARTESIAN_POINT('Ctrl Pts',(-231.233172746044,1.97183293707754,
124.49992013129));
#275636=CARTESIAN_POINT('Ctrl Pts',(-231.511620369858,-4.23828046494889,
125.73769764504));
#275637=CARTESIAN_POINT('Ctrl Pts',(-231.79006799367,-6.55362117119865,
131.631490910294));
#275638=CARTESIAN_POINT('Ctrl Pts',(-232.068515617483,-2.84650418331021,
136.765191844092));
#275639=CARTESIAN_POINT('Ctrl Pts',(-232.346963241296,3.47641108958031,
136.421180083507));
#275640=CARTESIAN_POINT('Ctrl Pts',(-232.625410865109,6.60467440326965,
130.915585630608));
#275641=CARTESIAN_POINT('Ctrl Pts',(-232.903858488922,3.66356459663667,
125.307780824367));
#275642=CARTESIAN_POINT('Ctrl Pts',(-233.182306112735,-2.64418209922576,
124.751064325225));
#275643=CARTESIAN_POINT('Ctrl Pts',(-233.460753736548,-6.52205462137589,
129.75703139878));
#275644=CARTESIAN_POINT('Ctrl Pts',(-233.73920136036,-4.40647756656326,
135.725442859523));
#275645=CARTESIAN_POINT('Ctrl Pts',(-234.017648984174,1.75843710352442,
137.17162014814));
#275646=CARTESIAN_POINT('Ctrl Pts',(-234.296096607986,6.30743397990132,
132.766596986079));
#275647=CARTESIAN_POINT('Ctrl Pts',(-234.574544231799,5.06020716402928,
126.558374461932));
#275648=CARTESIAN_POINT('Ctrl Pts',(-234.852991855612,-0.837102830722735,
124.252005786856));
#275649=CARTESIAN_POINT('Ctrl Pts',(-235.131439479425,-5.96515621878728,
127.966931100874));
#275650=CARTESIAN_POINT('Ctrl Pts',(-235.409887103238,-5.6115224558684,
134.289315524594));
#275651=CARTESIAN_POINT('Ctrl Pts',(-235.688334727051,-0.101173694118813,
137.409196638266));
#275652=CARTESIAN_POINT('Ctrl Pts',(-235.966782350864,5.50214874991674,
134.459556113093));
#275653=CARTESIAN_POINT('Ctrl Pts',(-236.245229974676,6.04926528768773,
128.150969493757));
#275654=CARTESIAN_POINT('Ctrl Pts',(-236.52367759849,1.03740254911254,124.280719691838));
#275655=CARTESIAN_POINT('Ctrl Pts',(-236.802125222302,-4.92778245216537,
126.405377203086));
#275656=CARTESIAN_POINT('Ctrl Pts',(-237.080572846115,-6.36457611545918,
132.572485569954));
#275657=CARTESIAN_POINT('Ctrl Pts',(-237.359020469928,-1.95263525547508,
137.114773483282));
#275658=CARTESIAN_POINT('Ctrl Pts',(-237.637468093741,4.25368201275546,
135.858100253825));
#275659=CARTESIAN_POINT('Ctrl Pts',(-237.915915717553,6.55107331518259,
129.957287187551));
#275660=CARTESIAN_POINT('Ctrl Pts',(-238.194363341367,2.8283482786799,124.834893221623));
#275661=CARTESIAN_POINT('Ctrl Pts',(-238.47281096518,-3.49349065343433,
125.198148167872));
#275662=CARTESIAN_POINT('Ctrl Pts',(-238.751258588993,-6.60498234154917,
130.713238476685));
#275663=CARTESIAN_POINT('Ctrl Pts',(-239.029706212805,-3.64681792910581,
136.312065581403));
#275664=CARTESIAN_POINT('Ctrl Pts',(-239.308153836619,2.66259400322518,
136.8495808907));
#275665=CARTESIAN_POINT('Ctrl Pts',(-239.586601460431,6.52521212154101,
131.831834094415));
#275666=CARTESIAN_POINT('Ctrl Pts',(-239.865049084244,4.39147907449425,
125.869889367774));
#275667=CARTESIAN_POINT('Ctrl Pts',(-240.143496708057,-1.77780870633274,
124.44248265737));
#275668=CARTESIAN_POINT('Ctrl Pts',(-240.42194433187,-6.31337713682396,
128.861330997368));
#275669=CARTESIAN_POINT('Ctrl Pts',(-240.700391955683,-5.04726040419313,
135.065728636055));
#275670=CARTESIAN_POINT('Ctrl Pts',(-240.978839579496,0.857042067512721,
137.354137245149));
#275671=CARTESIAN_POINT('Ctrl Pts',(-241.257287203309,5.97376474800676,
133.623621107872));
#275672=CARTESIAN_POINT('Ctrl Pts',(-241.535734827122,5.60088945971499,
127.302342308534));
#275673=CARTESIAN_POINT('Ctrl Pts',(-241.814182450934,0.0810703766063902,
124.199247252091));
#275674=CARTESIAN_POINT('Ctrl Pts',(-242.092630074747,-5.51324842209508,
127.165928700792));
#275675=CARTESIAN_POINT('Ctrl Pts',(-242.37107769856,-6.04116125805038,
133.476151333726));
#275676=CARTESIAN_POINT('Ctrl Pts',(-242.649525322373,-1.01754202499167,
137.331128822742));
#275677=CARTESIAN_POINT('Ctrl Pts',(-242.927972946186,4.94114861934255,
135.188325181553));
#275678=CARTESIAN_POINT('Ctrl Pts',(-243.206420569999,6.35916507103108,
129.016872274634));
#275679=CARTESIAN_POINT('Ctrl Pts',(-243.484868193812,1.93341948492588,
124.488033831209));
#275680=CARTESIAN_POINT('Ctrl Pts',(-243.763315817625,-4.26904415503308,
125.763591134728));
#275681=CARTESIAN_POINT('Ctrl Pts',(-244.041763441437,-6.54846477091785,
131.671369337695));
#275682=CARTESIAN_POINT('Ctrl Pts',(-244.320211065251,-2.8101661726183,
136.782408882594));
#275683=CARTESIAN_POINT('Ctrl Pts',(-244.598658689063,3.51053785406796,
136.399914115825));
#275684=CARTESIAN_POINT('Ctrl Pts',(-244.877106312876,6.60522909217403,
130.875379042142));
#275685=CARTESIAN_POINT('Ctrl Pts',(-245.155553936689,3.6300374779527,125.285581505715));
#275686=CARTESIAN_POINT('Ctrl Pts',(-245.434001560502,-2.68098124131831,
124.767272365732));
#275687=CARTESIAN_POINT('Ctrl Pts',(-245.712449184315,-6.528309173032,129.796752401026));
#275688=CARTESIAN_POINT('Ctrl Pts',(-245.990896808128,-4.37643990036281,
135.752175162922));
#275689=CARTESIAN_POINT('Ctrl Pts',(-246.269344431941,1.79716383976481,
137.160798071814));
#275690=CARTESIAN_POINT('Ctrl Pts',(-246.547792055753,6.31926180748295,
132.728165489484));
#275691=CARTESIAN_POINT('Ctrl Pts',(-246.826239679567,5.03426688722615,
126.527650212955));
#275692=CARTESIAN_POINT('Ctrl Pts',(-247.104687303379,-0.876973364781528,
124.257222869343));
#275693=CARTESIAN_POINT('Ctrl Pts',(-247.383134927193,-5.98231793708558,
128.003295270889));
#275694=CARTESIAN_POINT('Ctrl Pts',(-247.661582551005,-5.59020457768662,
134.32340988638));
#275695=CARTESIAN_POINT('Ctrl Pts',(-247.940030174818,-0.0609663080697638,
137.409690138946));
#275696=CARTESIAN_POINT('Ctrl Pts',(-248.218477798631,5.524297020294,134.425995249648));
#275697=CARTESIAN_POINT('Ctrl Pts',(-248.496925422444,6.03300126391963,
128.114195060156));
#275698=CARTESIAN_POINT('Ctrl Pts',(-248.775373046256,0.997672074500306,
124.274525596028));
#275699=CARTESIAN_POINT('Ctrl Pts',(-249.05382067007,-4.95446901239483,
126.435455516518));
#275700=CARTESIAN_POINT('Ctrl Pts',(-249.332268293882,-6.35369511616563,
132.611195791991));
#275701=CARTESIAN_POINT('Ctrl Pts',(-249.610715917695,-1.91418580344349,
137.126542810973));
#275702=CARTESIAN_POINT('Ctrl Pts',(-249.889163541508,4.28436674946925,
135.832113249982));
#275703=CARTESIAN_POINT('Ctrl Pts',(-250.167611165321,6.54579556256923,
129.917424639176));
#275704=CARTESIAN_POINT('Ctrl Pts',(-250.446058789134,2.79195803356287,
124.817786863269));
#275705=CARTESIAN_POINT('Ctrl Pts',(-250.724506412947,-3.52755253356211,
125.219517907192));
#275706=CARTESIAN_POINT('Ctrl Pts',(-251.00295403676,-6.60541465285253,
130.75344656718));
#275707=CARTESIAN_POINT('Ctrl Pts',(-251.281401660573,-3.61322339864049,
136.334162752248));
#275708=CARTESIAN_POINT('Ctrl Pts',(-251.559849284386,2.6993436431913,136.83326092127));
#275709=CARTESIAN_POINT('Ctrl Pts',(-251.838296908198,6.53134574711249,
131.792094239578));
#275710=CARTESIAN_POINT('Ctrl Pts',(-252.116744532012,4.3613601835781,125.843248612281));
#275711=CARTESIAN_POINT('Ctrl Pts',(-252.395192155824,-1.81650232468185,
124.453422554885));
#275712=CARTESIAN_POINT('Ctrl Pts',(-252.673639779637,-6.32508793705065,
128.899798314935));
#275713=CARTESIAN_POINT('Ctrl Pts',(-252.95208740345,-5.02122673409033,
135.096373791053));
#275714=CARTESIAN_POINT('Ctrl Pts',(-253.230535027263,0.896896539007115,
137.348798831588));
#275715=CARTESIAN_POINT('Ctrl Pts',(-253.508982651076,5.99081570467794,
133.587204877683));
#275716=CARTESIAN_POINT('Ctrl Pts',(-253.787430274889,5.57946791275175,
127.26831297809));
#275717=CARTESIAN_POINT('Ctrl Pts',(-254.065877898701,0.0408616672245685,
124.198876151673));
#275718=CARTESIAN_POINT('Ctrl Pts',(-254.344325522515,-5.53529442795169,
127.199556781751));
#275719=CARTESIAN_POINT('Ctrl Pts',(-254.622773146327,-6.0247854077167,
133.512876168065));
#275720=CARTESIAN_POINT('Ctrl Pts',(-254.90122077014,-0.977792831057213,
137.337201825807));
#275721=CARTESIAN_POINT('Ctrl Pts',(-255.179668393953,4.96774341227684,
135.158166043599));
#275722=CARTESIAN_POINT('Ctrl Pts',(-255.458116017766,6.34816648213513,
128.97819485735));
#275723=CARTESIAN_POINT('Ctrl Pts',(-255.736563641579,1.89493404819936,
124.476382515012));
#275724=CARTESIAN_POINT('Ctrl Pts',(-256.015011265392,-4.29964901022966,
125.789669655819));
#275725=CARTESIAN_POINT('Ctrl Pts',(-256.293458889205,-6.54306693065544,
131.711218953762));
#275726=CARTESIAN_POINT('Ctrl Pts',(-256.571906513018,-2.77372173452912,
136.799398141047));
#275727=CARTESIAN_POINT('Ctrl Pts',(-256.85035413683,3.54453019961847,136.378452625405));
#275728=CARTESIAN_POINT('Ctrl Pts',(-257.128801760644,6.60554720661629,
130.835147498674));
#275729=CARTESIAN_POINT('Ctrl Pts',(-257.407249384456,3.5963603924579,125.263628838565));
#275730=CARTESIAN_POINT('Ctrl Pts',(-257.685697008269,-2.71765185753996,
124.783624522784));
#275731=CARTESIAN_POINT('Ctrl Pts',(-257.964144632082,-6.53437691572335,
129.836661023534));
#275732=CARTESIAN_POINT('Ctrl Pts',(-258.242592255895,-4.34613602341029,
135.778440351053));
#275733=CARTESIAN_POINT('Ctrl Pts',(-258.521039879708,1.83562753012831,
137.150276335207));
#275734=CARTESIAN_POINT('Ctrl Pts',(-258.799487503521,6.33122643152078,
132.688650362788));
#275735=CARTESIAN_POINT('Ctrl Pts',(-259.077935127334,5.00743946241547,
126.498999976245));
#275736=CARTESIAN_POINT('Ctrl Pts',(-259.356382751147,-0.915487258132909,
124.259032700089));
#275737=CARTESIAN_POINT('Ctrl Pts',(-259.634830374959,-6.00176822571329,
128.046924274587));
#275738=CARTESIAN_POINT('Ctrl Pts',(-259.86687006147,-5.63687269779404,
133.292521465648));
#275739=CARTESIAN_POINT('Ctrl Pts',(-260.052531023546,-2.79481741349804,
135.900547185714));
#275740=CARTESIAN_POINT('Ctrl Pts',(-260.145376111017,-0.946914048523564,
136.386386345067));
#275741=CARTESIAN_POINT('Ctrl Pts',(-260.191813261187,-0.0157913329746497,
136.389009763222));
#275742=CARTESIAN_POINT('Ctrl Pts',(210.190947297731,3.04870273111253,135.077142573452));
#275743=CARTESIAN_POINT('Ctrl Pts',(210.144529434129,3.76080111712433,134.569051946243));
#275744=CARTESIAN_POINT('Ctrl Pts',(210.051703633225,4.91317831978039,133.192256847685));
#275745=CARTESIAN_POINT('Ctrl Pts',(209.866061957716,5.67455722768035,129.648049455111));
#275746=CARTESIAN_POINT('Ctrl Pts',(209.634022271206,3.10293383059235,125.427666478792));
#275747=CARTESIAN_POINT('Ctrl Pts',(209.355574647392,-2.85596866243967,
125.28812524467));
#275748=CARTESIAN_POINT('Ctrl Pts',(209.07712702358,-6.17973736462657,130.225196103446));
#275749=CARTESIAN_POINT('Ctrl Pts',(208.798679399767,-3.83016968018938,
135.690661498217));
#275750=CARTESIAN_POINT('Ctrl Pts',(208.520231775954,2.04205955310628,136.667868212554));
#275751=CARTESIAN_POINT('Ctrl Pts',(208.241784152142,6.03618933210081,132.255733564264));
#275752=CARTESIAN_POINT('Ctrl Pts',(207.963336528328,4.48417485225333,126.510421532214));
#275753=CARTESIAN_POINT('Ctrl Pts',(207.684888904515,-1.18901089957204,
124.710731370568));
#275754=CARTESIAN_POINT('Ctrl Pts',(207.406441280703,-5.76932406256156,
128.510946815645));
#275755=CARTESIAN_POINT('Ctrl Pts',(207.12799365689,-5.04803188696711,134.418613818075));
#275756=CARTESIAN_POINT('Ctrl Pts',(206.849546033077,0.312219397189005,
137.005003016302));
#275757=CARTESIAN_POINT('Ctrl Pts',(206.571098409264,5.38552219392035,133.893281295751));
#275758=CARTESIAN_POINT('Ctrl Pts',(206.292650785451,5.50981125882569,127.943004805273));
#275759=CARTESIAN_POINT('Ctrl Pts',(206.014203161638,0.570843377758803,
124.622167937696));
#275760=CARTESIAN_POINT('Ctrl Pts',(205.735755537825,-4.89269661278007,
126.982467612715));
#275761=CARTESIAN_POINT('Ctrl Pts',(205.457307914013,-5.86009012142741,
132.854898402769));
#275762=CARTESIAN_POINT('Ctrl Pts',(205.178860290199,-1.44234566848361,
136.842986120511));
#275763=CARTESIAN_POINT('Ctrl Pts',(204.900412666387,4.30084323855829,135.281871486376));
#275764=CARTESIAN_POINT('Ctrl Pts',(204.621965042573,6.09176771588946,129.606143376667));
#275765=CARTESIAN_POINT('Ctrl Pts',(204.343517418761,2.28465505058828,125.031518229909));
#275766=CARTESIAN_POINT('Ctrl Pts',(204.065069794948,-3.62194388278553,
125.761853295313));
#275767=CARTESIAN_POINT('Ctrl Pts',(203.786622171135,-6.20015338889199,
131.126006208945));
#275768=CARTESIAN_POINT('Ctrl Pts',(203.508174547322,-3.08072479357708,
136.194582558939));
#275769=CARTESIAN_POINT('Ctrl Pts',(203.229726923509,2.86973936865286,136.309808260363));
#275770=CARTESIAN_POINT('Ctrl Pts',(202.951279299696,6.1830532544492,131.365796540178));
#275771=CARTESIAN_POINT('Ctrl Pts',(202.672831675884,3.81444325369211,125.905852631576));
#275772=CARTESIAN_POINT('Ctrl Pts',(202.39438405207,-2.05945374882828,124.947398258377));
#275773=CARTESIAN_POINT('Ctrl Pts',(202.115936428258,-6.04081336739099,
129.371206163854));
#275774=CARTESIAN_POINT('Ctrl Pts',(201.837488804444,-4.47096061076856,
135.112012999282));
#275775=CARTESIAN_POINT('Ctrl Pts',(201.559041180632,1.20748652821524,136.894297736177));
#275776=CARTESIAN_POINT('Ctrl Pts',(201.280593556819,5.77631253695961,133.08022777117));
#275777=CARTESIAN_POINT('Ctrl Pts',(201.002145933006,5.03698951269057,127.174747074221));
#275778=CARTESIAN_POINT('Ctrl Pts',(200.723698309193,-0.331080803069094,
124.604703907164));
#275779=CARTESIAN_POINT('Ctrl Pts',(200.44525068538,-5.39490403503349,127.731842386878));
#275780=CARTESIAN_POINT('Ctrl Pts',(200.166803061567,-5.50107401450091,
133.682475019745));
#275781=CARTESIAN_POINT('Ctrl Pts',(199.888355437754,-0.552025717056,136.988261120707));
#275782=CARTESIAN_POINT('Ctrl Pts',(199.609907813942,4.90430724641216,134.611344759621));
#275783=CARTESIAN_POINT('Ctrl Pts',(199.331460190128,5.85382143915379,128.735995953499));
#275784=CARTESIAN_POINT('Ctrl Pts',(199.053012566316,1.42395970438994,124.761373228423));
#275785=CARTESIAN_POINT('Ctrl Pts',(198.774564942502,-4.31445143441004,
126.339960697623));
#275786=CARTESIAN_POINT('Ctrl Pts',(198.49611731869,-6.088092477657,132.02111359519));
#275787=CARTESIAN_POINT('Ctrl Pts',(198.217669694877,-2.26707395378944,
136.584129948007));
#275788=CARTESIAN_POINT('Ctrl Pts',(197.939222071064,3.6372747808909,135.835820643578));
#275789=CARTESIAN_POINT('Ctrl Pts',(197.660774447251,6.19914568268399,130.46384537573));
#275790=CARTESIAN_POINT('Ctrl Pts',(197.382326823438,3.06430454719326,125.404786980035));
#275791=CARTESIAN_POINT('Ctrl Pts',(197.103879199626,-2.88648276756863,
125.307672973393));
#275792=CARTESIAN_POINT('Ctrl Pts',(196.825431575812,-6.1847334314575,130.261746383626));
#275793=CARTESIAN_POINT('Ctrl Pts',(196.546983952,-3.79951621286212,135.71445576667));
#275794=CARTESIAN_POINT('Ctrl Pts',(196.268536328187,2.07727078866752,136.65502757917));
#275795=CARTESIAN_POINT('Ctrl Pts',(195.990088704374,6.04514741573133,132.219122274927));
#275796=CARTESIAN_POINT('Ctrl Pts',(195.711641080561,4.45782888960729,126.483120122517));
#275797=CARTESIAN_POINT('Ctrl Pts',(195.433193456748,-1.22601660901765,
124.718126880723));
#275798=CARTESIAN_POINT('Ctrl Pts',(195.154745832935,-5.78321273819644,
128.54608511404));
#275799=CARTESIAN_POINT('Ctrl Pts',(194.876298209123,-5.02591888662151,
134.449288212205));
#275800=CARTESIAN_POINT('Ctrl Pts',(194.597850585309,0.349948891971121,
137.002980915508));
#275801=CARTESIAN_POINT('Ctrl Pts',(194.319402961497,5.40423073479611,133.860444384439));
#275802=CARTESIAN_POINT('Ctrl Pts',(194.040955337684,5.49228854369214,127.909516169605));
#275803=CARTESIAN_POINT('Ctrl Pts',(193.762507713871,0.533201494146887,
124.618808581434));
#275804=CARTESIAN_POINT('Ctrl Pts',(193.484060090058,-4.91587168017823,
127.012321133451));
#275805=CARTESIAN_POINT('Ctrl Pts',(193.205612466245,-5.84749893410212,
132.890532719942));
#275806=CARTESIAN_POINT('Ctrl Pts',(192.927164842432,-1.40556033379022,
136.851654059523));
#275807=CARTESIAN_POINT('Ctrl Pts',(192.648717218619,4.32801954783523,135.255608152653));
#275808=CARTESIAN_POINT('Ctrl Pts',(192.370269594806,6.08436090050943,129.569083216569));
#275809=CARTESIAN_POINT('Ctrl Pts',(192.091821970994,2.24947182316989,125.017717865345));
#275810=CARTESIAN_POINT('Ctrl Pts',(191.81337434718,-3.65257196685492,125.783994510198));
#275811=CARTESIAN_POINT('Ctrl Pts',(191.534926723368,-6.19808055740059,
131.163742349203));
#275812=CARTESIAN_POINT('Ctrl Pts',(191.256479099555,-3.04785590876364,
136.213235933607));
#275813=CARTESIAN_POINT('Ctrl Pts',(190.978031475742,2.90319942398833,136.292237340818));
#275814=CARTESIAN_POINT('Ctrl Pts',(190.699583851929,6.18635631527163,131.328148137043));
#275815=CARTESIAN_POINT('Ctrl Pts',(190.421136228116,3.7845539731278,125.882723791311));
#275816=CARTESIAN_POINT('Ctrl Pts',(190.142688604304,-2.09506858458051,
124.960043253581));
#275817=CARTESIAN_POINT('Ctrl Pts',(189.86424098049,-6.04942546284962,129.408004862578));
#275818=CARTESIAN_POINT('Ctrl Pts',(189.585793356678,-4.44465587162338,
135.139149194637));
#275819=CARTESIAN_POINT('Ctrl Pts',(189.307345732864,1.24453533211424,136.886834590562));
#275820=CARTESIAN_POINT('Ctrl Pts',(189.028898109051,5.79005936456987,133.045023550676));
#275821=CARTESIAN_POINT('Ctrl Pts',(188.750450485239,5.01480170111087,127.144152737732));
#275822=CARTESIAN_POINT('Ctrl Pts',(188.472002861426,-0.368813738986236,
124.606834155258));
#275823=CARTESIAN_POINT('Ctrl Pts',(188.193555237613,-5.41350737050784,
127.764739625646));
#275824=CARTESIAN_POINT('Ctrl Pts',(187.9151076138,-5.48345219307025,133.715908293866));
#275825=CARTESIAN_POINT('Ctrl Pts',(187.636659989987,-0.51437233173317,
136.991506884579));
#275826=CARTESIAN_POINT('Ctrl Pts',(187.358212366174,4.92739057398128,134.581420314804));
#275827=CARTESIAN_POINT('Ctrl Pts',(187.079764742362,5.84112225861874,128.700400402891));
#275828=CARTESIAN_POINT('Ctrl Pts',(186.801317118548,1.38714794227173,124.752817144095));
#275829=CARTESIAN_POINT('Ctrl Pts',(186.522869494736,-4.34154756707868,
126.366306703083));
#275830=CARTESIAN_POINT('Ctrl Pts',(186.244421870923,-6.08057295867359,
132.058150998494));
#275831=CARTESIAN_POINT('Ctrl Pts',(185.96597424711,-2.23184885375068,136.597823184897));
#275832=CARTESIAN_POINT('Ctrl Pts',(185.687526623297,3.66783531589119,135.813586298303));
#275833=CARTESIAN_POINT('Ctrl Pts',(185.409078999484,6.19695801394562,130.42611572539));
#275834=CARTESIAN_POINT('Ctrl Pts',(185.130631375671,3.03137903541329,125.386233730096));
#275835=CARTESIAN_POINT('Ctrl Pts',(184.852183751858,-2.9198891855651,125.325345654173));
#275836=CARTESIAN_POINT('Ctrl Pts',(184.573736128045,-6.18792188952598,
130.299404664846));
#275837=CARTESIAN_POINT('Ctrl Pts',(184.295288504232,-3.76955667380246,
135.737493527599));
#275838=CARTESIAN_POINT('Ctrl Pts',(184.01684088042,2.11284697206427,136.642274242971));
#275839=CARTESIAN_POINT('Ctrl Pts',(183.738393256607,6.05364746891681,132.182297534532));
#275840=CARTESIAN_POINT('Ctrl Pts',(183.459945632794,4.43144167895468,126.456064115361));
#275841=CARTESIAN_POINT('Ctrl Pts',(183.181498008981,-1.2630425260055,124.725702755623));
#275842=CARTESIAN_POINT('Ctrl Pts',(182.903050385168,-5.79685235262429,
128.581331012064));
#275843=CARTESIAN_POINT('Ctrl Pts',(182.624602761355,-5.00363805916239,
134.479814874928));
#275844=CARTESIAN_POINT('Ctrl Pts',(182.346155137542,0.387675169361259,
137.000735831198));
#275845=CARTESIAN_POINT('Ctrl Pts',(182.06770751373,5.42273385622678,133.827490675898));
#275846=CARTESIAN_POINT('Ctrl Pts',(181.789259889916,5.47456504449634,127.876136685104));
#275847=CARTESIAN_POINT('Ctrl Pts',(181.510812266103,0.495538404244469,
124.615677436551));
#275848=CARTESIAN_POINT('Ctrl Pts',(181.232364642291,-4.93886382111119,
127.042315697369));
#275849=CARTESIAN_POINT('Ctrl Pts',(180.953917018477,-5.83469147177671,
132.926089453735));
#275850=CARTESIAN_POINT('Ctrl Pts',(180.675469394665,-1.36872270040423,
136.860098061879));
#275851=CARTESIAN_POINT('Ctrl Pts',(180.397021770852,4.35503536681857,135.229179797918));
#275852=CARTESIAN_POINT('Ctrl Pts',(180.118574147039,6.07672868724052,129.532068871648));
#275853=CARTESIAN_POINT('Ctrl Pts',(179.840126523226,2.21420520878857,125.004131904969));
#275854=CARTESIAN_POINT('Ctrl Pts',(179.561678899413,-3.68306468660213,
125.80632176824));
#275855=CARTESIAN_POINT('Ctrl Pts',(179.2832312756,-6.19577806271818,131.20146516627));
#275856=CARTESIAN_POINT('Ctrl Pts',(179.004783651788,-3.01487407978163,
136.231688883676));
#275857=CARTESIAN_POINT('Ctrl Pts',(178.726336027974,2.93655189768736,136.274463064253));
#275858=CARTESIAN_POINT('Ctrl Pts',(178.447888404162,6.18943013971724,131.290480325685));
#275859=CARTESIAN_POINT('Ctrl Pts',(178.169440780348,3.75452445381909,125.859777323623));
#275860=CARTESIAN_POINT('Ctrl Pts',(177.890993156536,-2.13060578642238,
124.972904812372));
#275861=CARTESIAN_POINT('Ctrl Pts',(177.612545532723,-6.05781339482078,
129.44485530364));
#275862=CARTESIAN_POINT('Ctrl Pts',(177.33409790891,-4.41818643401566,135.166124762878));
#275863=CARTESIAN_POINT('Ctrl Pts',(177.055650285097,1.28153801924328,136.879146056599));
#275864=CARTESIAN_POINT('Ctrl Pts',(176.777202661284,5.80359163943039,133.009736301615));
#275865=CARTESIAN_POINT('Ctrl Pts',(176.498755037472,4.99242806419446,127.113694031581));
#275866=CARTESIAN_POINT('Ctrl Pts',(176.220307413658,-0.406533008366379,
124.60919405498));
#275867=CARTESIAN_POINT('Ctrl Pts',(175.941859789846,-5.43191010648008,
127.797749498684));
#275868=CARTESIAN_POINT('Ctrl Pts',(175.663412166033,-5.46562718029972,
133.749233679521));
#275869=CARTESIAN_POINT('Ctrl Pts',(175.38496454222,-0.476699886155768,
136.994523381468));
#275870=CARTESIAN_POINT('Ctrl Pts',(175.106516918407,4.95029131528126,134.551355909651));
#275871=CARTESIAN_POINT('Ctrl Pts',(174.828069294595,5.82820663315002,128.664882815304));
#275872=CARTESIAN_POINT('Ctrl Pts',(174.549621670781,1.35028477887665,124.744485301934));
#275873=CARTESIAN_POINT('Ctrl Pts',(174.271174046969,-4.36848282210566,
126.392817162263));
#275874=CARTESIAN_POINT('Ctrl Pts',(173.992726423155,-6.07282812182305,
132.095141942134));
#275875=CARTESIAN_POINT('Ctrl Pts',(173.714278799343,-2.19654105173196,
136.611301742902));
#275876=CARTESIAN_POINT('Ctrl Pts',(173.435831175529,3.69825993790488,135.791166334329));
#275877=CARTESIAN_POINT('Ctrl Pts',(173.157383551717,6.19454071464915,130.388400091055));
#275878=CARTESIAN_POINT('Ctrl Pts',(172.878935927904,2.99834119476844,125.367881250842));
#275879=CARTESIAN_POINT('Ctrl Pts',(172.600488304091,-2.95318740599396,
125.343221361866));
#275880=CARTESIAN_POINT('Ctrl Pts',(172.322040680278,-6.1908810518732,130.337081657394));
#275881=CARTESIAN_POINT('Ctrl Pts',(172.043593056465,-3.7394574524341,135.760348489473));
#275882=CARTESIAN_POINT('Ctrl Pts',(171.765145432652,2.14834486313941,136.629304580736));
#275883=CARTESIAN_POINT('Ctrl Pts',(171.486697808839,6.06192320196904,132.145421734178));
#275884=CARTESIAN_POINT('Ctrl Pts',(171.208250185027,4.40489025960108,126.42916923593));
#275885=CARTESIAN_POINT('Ctrl Pts',(170.929802561213,-1.30002164048796,
124.733503877423));
#275886=CARTESIAN_POINT('Ctrl Pts',(170.651354937401,-5.81027716255637,
128.616659285268));
#275887=CARTESIAN_POINT('Ctrl Pts',(170.372907313588,-4.98117182005496,
134.510205342342));
#275888=CARTESIAN_POINT('Ctrl Pts',(170.094459689775,0.42538708130529,136.998261137926));
#275889=CARTESIAN_POINT('Ctrl Pts',(169.816012065962,5.44103603626017,133.794424944161));
#275890=CARTESIAN_POINT('Ctrl Pts',(169.537564442149,5.45663868327959,127.842865707018));
#275891=CARTESIAN_POINT('Ctrl Pts',(169.259116818336,0.457856951984399,
124.612775615598));
#275892=CARTESIAN_POINT('Ctrl Pts',(168.980669194523,-4.9616729506289,127.072449665244));
#275893=CARTESIAN_POINT('Ctrl Pts',(168.702221570711,-5.82166780281318,
132.961567566087));
#275894=CARTESIAN_POINT('Ctrl Pts',(168.423773946897,-1.33183434849535,
136.868317666657));
#275895=CARTESIAN_POINT('Ctrl Pts',(168.145326323085,4.38188980836473,135.202587479883));
#275896=CARTESIAN_POINT('Ctrl Pts',(167.866878699272,6.06887129855542,129.495101671966));
#275897=CARTESIAN_POINT('Ctrl Pts',(167.588431075459,2.17885654621902,124.9907608742));
#275898=CARTESIAN_POINT('Ctrl Pts',(167.309983451646,-3.71342092903282,
125.82883423045));
#275899=CARTESIAN_POINT('Ctrl Pts',(167.031535827833,-6.19324598120115,
131.239173268482));
#275900=CARTESIAN_POINT('Ctrl Pts',(166.75308820402,-2.98178053353198,136.249940722101));
#275901=CARTESIAN_POINT('Ctrl Pts',(166.474640580207,2.96979555637586,136.25648609103));
#275902=CARTESIAN_POINT('Ctrl Pts',(166.196192956395,6.19227461255283,131.252794500981));
#275903=CARTESIAN_POINT('Ctrl Pts',(165.917745332582,3.7243558092261,125.837014079288));
#275904=CARTESIAN_POINT('Ctrl Pts',(165.639297708769,-2.16606403788322,
124.985982457902));
#275905=CARTESIAN_POINT('Ctrl Pts',(165.360850084956,-6.06597685228888,
129.481756121673));
#275906=CARTESIAN_POINT('Ctrl Pts',(165.082402461143,-4.39155327888481,
135.192938704347));
#275907=CARTESIAN_POINT('Ctrl Pts',(164.80395483733,1.31849321850979,136.871232419228));
#275908=CARTESIAN_POINT('Ctrl Pts',(164.525507213517,5.81690886006848,132.974367331546));
#275909=CARTESIAN_POINT('Ctrl Pts',(164.247059589704,4.96986943102014,127.083372084437));
#275910=CARTESIAN_POINT('Ctrl Pts',(163.968611965891,-0.444237213516358,
124.611783518878));
#275911=CARTESIAN_POINT('Ctrl Pts',(163.690164342078,-5.45011156102575,
127.830870782803));
#275912=CARTESIAN_POINT('Ctrl Pts',(163.411716718265,-5.44759963670407,
133.782449941821));
#275913=CARTESIAN_POINT('Ctrl Pts',(163.133269094453,-0.439009776288703,
136.9973104996));
#275914=CARTESIAN_POINT('Ctrl Pts',(162.85482147064,4.97300862171615,134.52115265821));
#275915=CARTESIAN_POINT('Ctrl Pts',(162.576373846827,5.81507504134112,128.629444506854));
#275916=CARTESIAN_POINT('Ctrl Pts',(162.297926223014,1.31337158018249,124.736378010682));
#275917=CARTESIAN_POINT('Ctrl Pts',(162.019478599201,-4.39525620139515,
126.419491092807));
#275918=CARTESIAN_POINT('Ctrl Pts',(161.741030975388,-6.06485825409316,
132.132085055398));
#275919=CARTESIAN_POINT('Ctrl Pts',(161.462583351575,-2.16115185607673,
136.624565122567));
#275920=CARTESIAN_POINT('Ctrl Pts',(161.184135727762,3.72854751953661,135.768561582436));
#275921=CARTESIAN_POINT('Ctrl Pts',(160.905688103949,6.19189387436843,130.350699870288));
#275922=CARTESIAN_POINT('Ctrl Pts',(160.627240480137,2.96519224948793,125.349730222329));
#275923=CARTESIAN_POINT('Ctrl Pts',(160.348792856324,-2.9863761949775,125.361299434083));
#275924=CARTESIAN_POINT('Ctrl Pts',(160.070345232511,-6.19361080884636,
130.374775965136));
#275925=CARTESIAN_POINT('Ctrl Pts',(159.791897608698,-3.70921966409463,
135.783019805394));
#275926=CARTESIAN_POINT('Ctrl Pts',(159.513449984885,2.18376314650564,136.616119073061));
#275927=CARTESIAN_POINT('Ctrl Pts',(159.235002361072,6.06997430822783,132.108496240312));
#275928=CARTESIAN_POINT('Ctrl Pts',(158.956554737259,4.37817561541891,126.402436480826));
#275929=CARTESIAN_POINT('Ctrl Pts',(158.678107113446,-1.3369525821905,124.741529957054));
#275930=CARTESIAN_POINT('Ctrl Pts',(158.399659489633,-5.82348667053154,
128.652068624549));
#275931=CARTESIAN_POINT('Ctrl Pts',(158.121211865821,-4.95852100179383,
134.540458488317));
#275932=CARTESIAN_POINT('Ctrl Pts',(157.842764242008,0.463083230374652,
136.995556927392));
#275933=CARTESIAN_POINT('Ctrl Pts',(157.564316618195,5.45913659670229,133.761248414491));
#275934=CARTESIAN_POINT('Ctrl Pts',(157.285868994382,5.43851012430973,127.809704468215));
#275935=CARTESIAN_POINT('Ctrl Pts',(157.007421370569,0.420158533666468,
124.610103226106));
#275936=CARTESIAN_POINT('Ctrl Pts',(156.728973746756,-4.98429822353081,
127.102721920452));
#275937=CARTESIAN_POINT('Ctrl Pts',(156.450526122943,-5.80842840980828,
132.996965742341));
#275938=CARTESIAN_POINT('Ctrl Pts',(156.172078499131,-1.2948966449748,136.876312569277));
#275939=CARTESIAN_POINT('Ctrl Pts',(155.893630875317,4.40858187737264,135.175832183934));
#275940=CARTESIAN_POINT('Ctrl Pts',(155.615183251505,6.06078902561252,129.458182987356));
#275941=CARTESIAN_POINT('Ctrl Pts',(155.336735627692,2.14342714531882,124.977605268507));
#275942=CARTESIAN_POINT('Ctrl Pts',(155.058288003879,-3.74363956928552,
125.85153106262));
#275943=CARTESIAN_POINT('Ctrl Pts',(154.779840380066,-6.19048440667673,
131.276865258552));
#275944=CARTESIAN_POINT('Ctrl Pts',(154.501392756253,-2.94857649630798,
136.267990772552));
#275945=CARTESIAN_POINT('Ctrl Pts',(154.22294513244,3.00292916819795,136.238307087292));
#275946=CARTESIAN_POINT('Ctrl Pts',(153.944497508627,6.19488962837548,131.215092059396));
#275947=CARTESIAN_POINT('Ctrl Pts',(153.666049884815,3.69404915725887,125.814434901805));
#275948=CARTESIAN_POINT('Ctrl Pts',(153.387602261001,-2.20144202504465,
124.999275705575));
#275949=CARTESIAN_POINT('Ctrl Pts',(153.109154637189,-6.07391553275397,
129.518705949301));
#275950=CARTESIAN_POINT('Ctrl Pts',(152.830707013376,-4.36475739313218,
135.219590025439));
#275951=CARTESIAN_POINT('Ctrl Pts',(152.552259389563,1.3553995605252,136.863093971691));
#275952=CARTESIAN_POINT('Ctrl Pts',(152.27381176575,5.83001053300956,132.93891795108));
#275953=CARTESIAN_POINT('Ctrl Pts',(151.995364141937,4.94712663750637,127.053188019893));
#275954=CARTESIAN_POINT('Ctrl Pts',(151.716916518124,-0.481924957293099,
124.614602450997));
#275955=CARTESIAN_POINT('Ctrl Pts',(151.438468894311,-5.46811105968323,
127.864102250682));
#275956=CARTESIAN_POINT('Ctrl Pts',(151.160021270498,-5.4293702303005,133.815555849925));
#275957=CARTESIAN_POINT('Ctrl Pts',(150.881573646685,-0.40130339875292,
136.999868135696));
#275958=CARTESIAN_POINT('Ctrl Pts',(150.603126022873,4.99554165148768,134.490811679673));
#275959=CARTESIAN_POINT('Ctrl Pts',(150.324678399059,5.80172796978809,128.59408679072));
#275960=CARTESIAN_POINT('Ctrl Pts',(150.046230775247,1.27640971402146,124.728495570759));
#275961=CARTESIAN_POINT('Ctrl Pts',(149.767783151434,-4.42186671284978,
126.446327506304));
#275962=CARTESIAN_POINT('Ctrl Pts',(149.489335527621,-6.05666365081033,
132.168978969345));
#275963=CARTESIAN_POINT('Ctrl Pts',(149.210887903808,-2.12568257814469,
136.637612832414));
#275964=CARTESIAN_POINT('Ctrl Pts',(148.932440279995,3.75869693846883,135.74577288025));
#275965=CARTESIAN_POINT('Ctrl Pts',(148.653992656183,6.18901759118317,130.313016460088));
#275966=CARTESIAN_POINT('Ctrl Pts',(148.375545032369,2.93193342791814,125.331781317152));
#275967=CARTESIAN_POINT('Ctrl Pts',(148.097097408557,-3.01945432269288,
125.379579200934));
#275968=CARTESIAN_POINT('Ctrl Pts',(147.818649784743,-6.19611105929333,
130.412486191295));
#275969=CARTESIAN_POINT('Ctrl Pts',(147.540202160931,-3.67884442925635,
135.805506635269));
#275970=CARTESIAN_POINT('Ctrl Pts',(147.261754537118,2.21910050972548,136.602718208539));
#275971=CARTESIAN_POINT('Ctrl Pts',(146.983306913305,6.07780048935632,132.071522421221));
#275972=CARTESIAN_POINT('Ctrl Pts',(146.704859289492,4.35129873632927,126.375866840638));
#275973=CARTESIAN_POINT('Ctrl Pts',(146.426411665679,-1.37383398262348,
124.749780697104));
#275974=CARTESIAN_POINT('Ctrl Pts',(146.147964041867,-5.83648038706648,
128.687557717801));
#275975=CARTESIAN_POINT('Ctrl Pts',(145.869516418053,-4.93568644371351,
134.570573191811));
#275976=CARTESIAN_POINT('Ctrl Pts',(145.591068794241,0.500762219724632,
136.992623299802));
#275977=CARTESIAN_POINT('Ctrl Pts',(145.312621170428,5.47703486683029,133.727962316256));
#275978=CARTESIAN_POINT('Ctrl Pts',(145.034173546615,5.42018003934715,127.776654197497));
#275979=CARTESIAN_POINT('Ctrl Pts',(144.755725922802,0.382444546219556,
124.607660367099));
#275980=CARTESIAN_POINT('Ctrl Pts',(144.477278298989,-5.00673880142907,
127.133131341243));
#275981=CARTESIAN_POINT('Ctrl Pts',(144.198830675176,-5.79497378335261,
133.032282670807));
#275982=CARTESIAN_POINT('Ctrl Pts',(143.920383051363,-1.25791095858285,
136.884082473484));
#275983=CARTESIAN_POINT('Ctrl Pts',(143.64193542755,4.43511058475782,135.148914901497));
#275984=CARTESIAN_POINT('Ctrl Pts',(143.363487803737,6.05248216790344,129.421314185853));
#275985=CARTESIAN_POINT('Ctrl Pts',(143.085040179924,2.10791831893749,124.964665575378));
#275986=CARTESIAN_POINT('Ctrl Pts',(142.806592556112,-3.77371948759721,
125.87441142371));
#275987=CARTESIAN_POINT('Ctrl Pts',(142.528144932299,-6.18749344147606,
131.314539739788));
#275988=CARTESIAN_POINT('Ctrl Pts',(142.249697308486,-2.91526319849757,
136.285838366179));
#275989=CARTESIAN_POINT('Ctrl Pts',(141.971249684673,3.03595150537554,136.219926726669));
#275990=CARTESIAN_POINT('Ctrl Pts',(141.69280206086,6.19727509028471,131.177374398005));
#275991=CARTESIAN_POINT('Ctrl Pts',(141.414354437047,3.6636056209416,125.792040627854));
#275992=CARTESIAN_POINT('Ctrl Pts',(141.135906813234,-2.23673843696229,
125.012784062803));
#275993=CARTESIAN_POINT('Ctrl Pts',(140.857459189421,-6.0816291420453,129.555703417335));
#275994=CARTESIAN_POINT('Ctrl Pts',(140.579011565609,-4.33779976968917,
135.246077738584));
#275995=CARTESIAN_POINT('Ctrl Pts',(140.300563941795,1.39225567771152,136.854731015561));
#275996=CARTESIAN_POINT('Ctrl Pts',(140.022116317983,5.84289617276637,132.903389473806));
#275997=CARTESIAN_POINT('Ctrl Pts',(139.74366869417,4.92420052639575,127.023142956427));
#275998=CARTESIAN_POINT('Ctrl Pts',(139.465221070357,-0.519594843163371,
124.617650746882));
#275999=CARTESIAN_POINT('Ctrl Pts',(139.186773446544,-5.48590793547459,
127.897442670915));
#276000=CARTESIAN_POINT('Ctrl Pts',(138.908325822731,-5.41093963658633,
133.848550177083));
#276001=CARTESIAN_POINT('Ctrl Pts',(138.629878198918,-0.363582150772119,
137.002196194983));
#276002=CARTESIAN_POINT('Ctrl Pts',(138.351430575105,5.0178895696262,134.460334098336));
#276003=CARTESIAN_POINT('Ctrl Pts',(138.072982951292,5.78816591307159,128.558810977095));
#276004=CARTESIAN_POINT('Ctrl Pts',(137.79453532748,1.23940055002892,124.720838274248));
#276005=CARTESIAN_POINT('Ctrl Pts',(137.516087703667,-4.44831337040726,
126.473325408321));
#276006=CARTESIAN_POINT('Ctrl Pts',(137.237640079854,-6.0482446156285,132.205822316857));
#276007=CARTESIAN_POINT('Ctrl Pts',(136.959192456041,-2.09013453226308,
136.650444388955));
#276008=CARTESIAN_POINT('Ctrl Pts',(136.680744832228,3.78870707750376,135.722801072215));
#276009=CARTESIAN_POINT('Ctrl Pts',(136.402297208415,6.18591197167502,130.275351256826));
#276010=CARTESIAN_POINT('Ctrl Pts',(136.123849584602,2.89856596247695,125.314035200413));
#276011=CARTESIAN_POINT('Ctrl Pts',(135.845401960789,-3.05242056341787,
125.398059985055));
#276012=CARTESIAN_POINT('Ctrl Pts',(135.566954336976,-6.19838171056633,
130.450210938505));
#276013=CARTESIAN_POINT('Ctrl Pts',(135.288506713164,-3.64833287348497,
135.827808145838));
#276014=CARTESIAN_POINT('Ctrl Pts',(135.01005908935,2.25435564335981,136.589102483743));
#276015=CARTESIAN_POINT('Ctrl Pts',(134.731611465538,6.08540145535266,132.034501646982));
#276016=CARTESIAN_POINT('Ctrl Pts',(134.453163841725,4.32426061826468,126.349461299917));
#276017=CARTESIAN_POINT('Ctrl Pts',(134.174716217912,-1.41066447513297,
124.75825579184));
#276018=CARTESIAN_POINT('Ctrl Pts',(133.896268594099,-5.84925783067434,
128.723125249964));
#276019=CARTESIAN_POINT('Ctrl Pts',(133.617820970286,-4.91266899195694,
134.600548336913));
#276020=CARTESIAN_POINT('Ctrl Pts',(133.339373346473,0.538422653146471,
136.989460363863));
#276021=CARTESIAN_POINT('Ctrl Pts',(133.06092572266,5.49473018341705,133.694567882885));
#276022=CARTESIAN_POINT('Ctrl Pts',(132.782478098847,5.40164910761999,127.743716119554));
#276023=CARTESIAN_POINT('Ctrl Pts',(132.504030475035,0.344716387149417,
124.605447129098));
#276024=CARTESIAN_POINT('Ctrl Pts',(132.225582851222,-5.02899385277987,
127.163676800786));
#276025=CARTESIAN_POINT('Ctrl Pts',(131.947135227409,-5.78130442201224,
133.067517042801));
#276026=CARTESIAN_POINT('Ctrl Pts',(131.668687603596,-1.22087865983776,
136.891627091362));
#276027=CARTESIAN_POINT('Ctrl Pts',(131.390239979783,4.46147494748924,135.121836630005));
#276028=CARTESIAN_POINT('Ctrl Pts',(131.11179235597,6.04395103324181,129.384496633644));
#276029=CARTESIAN_POINT('Ctrl Pts',(130.833344732157,2.07233138286776,124.951942274296));
#276030=CARTESIAN_POINT('Ctrl Pts',(130.554897108344,-3.80365956934553,
125.897474465882));
#276031=CARTESIAN_POINT('Ctrl Pts',(130.276449484532,-6.18427319643048,
131.35219531615));
#276032=CARTESIAN_POINT('Ctrl Pts',(129.998001860718,-2.88184187453723,
136.303482841632));
#276033=CARTESIAN_POINT('Ctrl Pts',(129.719554236906,3.0688613442533,136.201345690253));
#276034=CARTESIAN_POINT('Ctrl Pts',(129.441106613093,6.1994309098865,131.139642914452));
#276035=CARTESIAN_POINT('Ctrl Pts',(129.16265898928,3.63302632837089,125.769832087263));
#276036=CARTESIAN_POINT('Ctrl Pts',(128.884211365467,-2.27195196571463,
125.026507029031));
#276037=CARTESIAN_POINT('Ctrl Pts',(128.605763741654,-6.08911739433215,
129.592747154821));
#276038=CARTESIAN_POINT('Ctrl Pts',(128.327316117841,-4.31068140748063,
135.272400862266));
#276039=CARTESIAN_POINT('Ctrl Pts',(128.048868494028,1.42906020435147,136.846143860731));
#276040=CARTESIAN_POINT('Ctrl Pts',(127.770420870216,5.85556530185681,132.867783216248));
#276041=CARTESIAN_POINT('Ctrl Pts',(127.491973246402,4.9010919472237,126.993238007373));
#276042=CARTESIAN_POINT('Ctrl Pts',(127.21352562259,-0.557245475255655,
124.620928293575));
#276043=CARTESIAN_POINT('Ctrl Pts',(126.935077998777,-5.50350152892981,
127.930890808061));
#276044=CARTESIAN_POINT('Ctrl Pts',(126.656630374964,-5.39230853851415,
133.881431700678));
#276045=CARTESIAN_POINT('Ctrl Pts',(126.378182751151,-0.325847430121078,
137.004294591193));
#276046=CARTESIAN_POINT('Ctrl Pts',(126.099735127338,5.04005154802147,134.429721043558));
#276047=CARTESIAN_POINT('Ctrl Pts',(125.821287503525,5.77438937373851,128.523618373138));
#276048=CARTESIAN_POINT('Ctrl Pts',(125.542839879712,1.20234545959337,124.713406404895));
#276049=CARTESIAN_POINT('Ctrl Pts',(125.264392255899,-4.47459519407686,
126.50048379844));
#276050=CARTESIAN_POINT('Ctrl Pts',(124.985944632086,-6.03960146051831,
132.24261373269));
#276051=CARTESIAN_POINT('Ctrl Pts',(124.707497008274,-2.05450903567761,
136.663059316712));
#276052=CARTESIAN_POINT('Ctrl Pts',(124.429049384461,3.81857682460466,135.69964700956));
#276053=CARTESIAN_POINT('Ctrl Pts',(124.150601760648,6.18257713092382,130.237705656202));
#276054=CARTESIAN_POINT('Ctrl Pts',(123.872154136835,2.86509108960817,125.296492529702));
#276055=CARTESIAN_POINT('Ctrl Pts',(123.593706513022,-3.08527369557641,
125.416741101634));
#276056=CARTESIAN_POINT('Ctrl Pts',(123.315258889209,-6.20042267852561,
130.487948808862));
#276057=CARTESIAN_POINT('Ctrl Pts',(123.036811265396,-3.61768612739718,
135.849923510712));
#276058=CARTESIAN_POINT('Ctrl Pts',(122.758363641583,2.28952724101679,136.575272403211));
#276059=CARTESIAN_POINT('Ctrl Pts',(122.47991601777,6.09277692456002,131.997435289415));
#276060=CARTESIAN_POINT('Ctrl Pts',(122.201468393958,4.29706226313277,126.323220837128));
#276061=CARTESIAN_POINT('Ctrl Pts',(121.923020770144,-1.44744269495155,
124.766954927214));
#276062=CARTESIAN_POINT('Ctrl Pts',(121.644573146332,-5.86181852788225,
128.758769903068));
#276063=CARTESIAN_POINT('Ctrl Pts',(121.366125522519,-4.88946949944416,
134.630382812884));
#276064=CARTESIAN_POINT('Ctrl Pts',(121.087677898706,0.576063135118759,
136.986068236777));
#276065=CARTESIAN_POINT('Ctrl Pts',(120.809230274893,5.51222189075617,133.661066351821));
#276066=CARTESIAN_POINT('Ctrl Pts',(120.53078265108,5.38291801579874,127.710891454918));
#276067=CARTESIAN_POINT('Ctrl Pts',(120.252335027267,0.306975454486648,
124.603463594118));
#276068=CARTESIAN_POINT('Ctrl Pts',(119.973887403454,-5.05106255291402,
127.194357167205));
#276069=CARTESIAN_POINT('Ctrl Pts',(119.695439779642,-5.76742083231046,
133.102667552701));
#276070=CARTESIAN_POINT('Ctrl Pts',(119.416992155829,-1.18380112098488,
136.898946143343));
#276071=CARTESIAN_POINT('Ctrl Pts',(119.138544532016,4.48767398862585,135.09459837285));
#276072=CARTESIAN_POINT('Ctrl Pts',(118.860096908203,6.03519593775195,129.347731695017));
#276073=CARTESIAN_POINT('Ctrl Pts',(118.58164928439,2.0366676557964,124.939435836727));
#276074=CARTESIAN_POINT('Ctrl Pts',(118.303201660577,-3.83345870508974,
125.920719334523));
#276075=CARTESIAN_POINT('Ctrl Pts',(118.024754036764,-6.18082379086727,
131.389830592295));
#276076=CARTESIAN_POINT('Ctrl Pts',(117.746306412951,-2.84831376286653,
136.320923545089));
#276077=CARTESIAN_POINT('Ctrl Pts',(117.467858789138,3.10165746534553,136.18256466657));
#276078=CARTESIAN_POINT('Ctrl Pts',(117.189411165326,6.20135700729606,131.101899006891));
#276079=CARTESIAN_POINT('Ctrl Pts',(116.910963541513,3.60231241267338,125.747810102979));
#276080=CARTESIAN_POINT('Ctrl Pts',(116.6325159177,-2.30708130645123,125.040444095748));
#276081=CARTESIAN_POINT('Ctrl Pts',(116.354068293887,-6.09638001213474,
129.62983578909));
#276082=CARTESIAN_POINT('Ctrl Pts',(116.075620670074,-4.28340331138726,
135.298558421074));
#276083=CARTESIAN_POINT('Ctrl Pts',(115.797173046261,1.46581177664024,136.837332825402));
#276084=CARTESIAN_POINT('Ctrl Pts',(115.518725422448,5.86801745082159,132.832100497806));
#276085=CARTESIAN_POINT('Ctrl Pts',(115.240277798635,4.87780175628715,126.963474280869));
#276086=CARTESIAN_POINT('Ctrl Pts',(114.961830174822,-0.594875458411799,
124.624434969628));
#276087=CARTESIAN_POINT('Ctrl Pts',(114.68338255101,-5.52089118811201,127.964445422689));
#276088=CARTESIAN_POINT('Ctrl Pts',(114.404934927196,-5.37347762646609,
133.914199202272));
#276089=CARTESIAN_POINT('Ctrl Pts',(114.126487303384,-0.288100635073559,
137.006163246571));
#276090=CARTESIAN_POINT('Ctrl Pts',(113.848039679571,5.06202676545313,134.398973649715));
#276091=CARTESIAN_POINT('Ctrl Pts',(113.569592055758,5.76039886228364,128.488510282924));
#276092=CARTESIAN_POINT('Ctrl Pts',(113.291144431945,1.16524581580469,124.706200238089));
#276093=CARTESIAN_POINT('Ctrl Pts',(113.012696808132,-4.50071120997606,
126.527801670297));
#276094=CARTESIAN_POINT('Ctrl Pts',(112.734249184319,-6.03073450575487,
132.279351853526));
#276095=CARTESIAN_POINT('Ctrl Pts',(112.455801560506,-2.01880740850426,
136.675457148234));
#276096=CARTESIAN_POINT('Ctrl Pts',(112.177353936694,3.84830507293705,135.676311550269));
#276097=CARTESIAN_POINT('Ctrl Pts',(111.898906312881,6.17901319250346,130.200081053184));
#276098=CARTESIAN_POINT('Ctrl Pts',(111.620458689068,2.8315100497353,125.279153955068));
#276099=CARTESIAN_POINT('Ctrl Pts',(111.342011065255,-3.11801250178361,
125.435621858436));
#276100=CARTESIAN_POINT('Ctrl Pts',(111.063563441442,-6.20223388754234,
130.525698403974));
#276101=CARTESIAN_POINT('Ctrl Pts',(110.785115817629,-3.58690532661952,
135.871851910398));
#276102=CARTESIAN_POINT('Ctrl Pts',(110.506668193816,2.32461399939974,136.56122847942));
#276103=CARTESIAN_POINT('Ctrl Pts',(110.228220570003,6.09992662367788,131.960324722029));
#276104=CARTESIAN_POINT('Ctrl Pts',(109.94977294619,4.26970467877848,126.297146424621));
#276105=CARTESIAN_POINT('Ctrl Pts',(109.671325322378,-1.48416727924886,
124.775877780875));
#276106=CARTESIAN_POINT('Ctrl Pts',(109.392877698565,-5.8741620132489,128.794490356288));
#276107=CARTESIAN_POINT('Ctrl Pts',(109.114430074752,-4.86608882584101,
134.660075514194));
#276108=CARTESIAN_POINT('Ctrl Pts',(108.835982450939,0.61368227085971,136.982447044243));
#276109=CARTESIAN_POINT('Ctrl Pts',(108.557534827126,5.52950934068608,133.627458964475));
#276110=CARTESIAN_POINT('Ctrl Pts',(108.279087203313,5.36398745797076,127.67818141992));
#276111=CARTESIAN_POINT('Ctrl Pts',(108.0006395795,0.269223146735527,124.601709835656));
#276112=CARTESIAN_POINT('Ctrl Pts',(107.722191955687,-5.07294408406776,
127.225171303631));
#276113=CARTESIAN_POINT('Ctrl Pts',(107.443744331874,-5.75332352870873,
133.137732897993));
#276114=CARTESIAN_POINT('Ctrl Pts',(107.165296708062,-1.14667971594628,
136.906039358215));
#276115=CARTESIAN_POINT('Ctrl Pts',(106.886849084249,4.51370673735246,135.067201139359));
#276116=CARTESIAN_POINT('Ctrl Pts',(106.608401460436,6.02621720585718,129.31102073231));
#276117=CARTESIAN_POINT('Ctrl Pts',(106.329953836623,2.00092845925606,124.927146726103));
#276118=CARTESIAN_POINT('Ctrl Pts',(106.05150621281,-3.86311579061174,125.944145168289));
#276119=CARTESIAN_POINT('Ctrl Pts',(105.773058588997,-6.17714535260555,
131.427444173636));
#276120=CARTESIAN_POINT('Ctrl Pts',(105.494610965184,-2.81468010588189,
136.338159830278));
#276121=CARTESIAN_POINT('Ctrl Pts',(105.216163341371,3.13433865337982,136.163584351558));
#276122=CARTESIAN_POINT('Ctrl Pts',(104.937715717558,6.20305331114115,131.064144073934));
#276123=CARTESIAN_POINT('Ctrl Pts',(104.659268093745,3.57146501196475,125.725975491034));
#276124=CARTESIAN_POINT('Ctrl Pts',(104.380820469933,-2.34212515744159,
125.054594746511));
#276125=CARTESIAN_POINT('Ctrl Pts',(104.10237284612,-6.10341672633411,129.666967945808));
#276126=CARTESIAN_POINT('Ctrl Pts',(103.823925222307,-4.25596649220884,
135.324549445729));
#276127=CARTESIAN_POINT('Ctrl Pts',(103.545477598494,1.50250903273456,136.828298236068));
#276128=CARTESIAN_POINT('Ctrl Pts',(103.267029974681,5.88025215824177,132.796342640716));
#276129=CARTESIAN_POINT('Ctrl Pts',(102.988582350868,4.85433081661274,126.933852879821));
#276130=CARTESIAN_POINT('Ctrl Pts',(102.710134727055,-0.63248339823904,
124.628170645098));
#276131=CARTESIAN_POINT('Ctrl Pts',(102.431687103242,-5.53807626864099,
127.998105271418));
#276132=CARTESIAN_POINT('Ctrl Pts',(102.153239479429,-5.35444759822839,
133.946851467654));
#276133=CARTESIAN_POINT('Ctrl Pts',(101.874791855617,-0.250343164351048,
137.00780209187));
#276134=CARTESIAN_POINT('Ctrl Pts',(101.596344231803,5.0838144076213,134.368093056165));
#276135=CARTESIAN_POINT('Ctrl Pts',(101.317896607991,5.74619489713063,128.453488007394));
#276136=CARTESIAN_POINT('Ctrl Pts',(101.039448984178,1.12810299340375,124.69922004086));
#276137=CARTESIAN_POINT('Ctrl Pts',(100.761001360365,-4.52666045036627,
126.55527801162));
#276138=CARTESIAN_POINT('Ctrl Pts',(100.482553736552,-6.0216440799065,132.316035318018));
#276139=CARTESIAN_POINT('Ctrl Pts',(100.204106112739,-1.98303097367997,
136.687637424115));
#276140=CARTESIAN_POINT('Ctrl Pts',(99.9256584889259,3.87789072090961,135.652795559044));
#276141=CARTESIAN_POINT('Ctrl Pts',(99.6472108651132,6.17522028847693,130.162478841968));
#276142=CARTESIAN_POINT('Ctrl Pts',(99.3687632413001,2.79782408721636,125.262020118999));
#276143=CARTESIAN_POINT('Ctrl Pts',(99.0903156174874,-3.15063576889091,
125.454701555827));
#276144=CARTESIAN_POINT('Ctrl Pts',(98.8118679936743,-6.20381527050148,
130.563458325018));
#276145=CARTESIAN_POINT('Ctrl Pts',(98.5334203698616,-3.55599161174595,
135.89359253233));
#276146=CARTESIAN_POINT('Ctrl Pts',(98.2549727460486,2.35961461835606,136.546971232774));
#276147=CARTESIAN_POINT('Ctrl Pts',(97.9765251222358,6.10685028777152,131.923171319966));
#276148=CARTESIAN_POINT('Ctrl Pts',(97.6980774984228,4.24218887894701,126.271239028595));
#276149=CARTESIAN_POINT('Ctrl Pts',(97.4196298746099,-1.52083686718185,
124.785024022185));
#276150=CARTESIAN_POINT('Ctrl Pts',(97.141182250797,-5.88628782938184,128.830285285991));
#276151=CARTESIAN_POINT('Ctrl Pts',(96.8627346269842,-4.842527837527,134.689625340572));
#276152=CARTESIAN_POINT('Ctrl Pts',(96.5842870031713,0.651278666378471,
136.978596920444));
#276153=CARTESIAN_POINT('Ctrl Pts',(96.3058393793584,5.54659189261388,133.593746966183));
#276154=CARTESIAN_POINT('Ctrl Pts',(96.0273917555454,5.34485813561491,127.645587226641));
#276155=CARTESIAN_POINT('Ctrl Pts',(95.7489441317327,0.231460862821695,
124.6001859187));
#276156=CARTESIAN_POINT('Ctrl Pts',(95.4704965079195,-5.09463763541278,
127.256118068232));
#276157=CARTESIAN_POINT('Ctrl Pts',(95.192048884107,-5.73901303358793,133.172711779316));
#276158=CARTESIAN_POINT('Ctrl Pts',(94.9136012602939,-1.10951582026908,
136.912906473138));
#276159=CARTESIAN_POINT('Ctrl Pts',(94.635153636481,4.53957222901603,135.039645944743));
#276160=CARTESIAN_POINT('Ctrl Pts',(94.3567060126683,6.01701517026768,129.274365105863));
#276161=CARTESIAN_POINT('Ctrl Pts',(94.0782583888551,1.96511511757592,124.915075397801));
#276162=CARTESIAN_POINT('Ctrl Pts',(93.7998107650425,-3.89262972695748,
125.967751099126));
#276163=CARTESIAN_POINT('Ctrl Pts',(93.5213631412293,-6.17323801795121,
131.465034666385));
#276164=CARTESIAN_POINT('Ctrl Pts',(93.2429155174167,-2.7809421498907,136.355191058501));
#276165=CARTESIAN_POINT('Ctrl Pts',(92.9644678936037,3.16690369734264,136.14440544854));
#276166=CARTESIAN_POINT('Ctrl Pts',(92.6860202697908,6.20451975856463,131.026379514606));
#276167=CARTESIAN_POINT('Ctrl Pts',(92.4075726459779,3.54048526930663,125.704329060518));
#276168=CARTESIAN_POINT('Ctrl Pts',(92.129125022165,-2.37708222012305,125.068958456964));
#276169=CARTESIAN_POINT('Ctrl Pts',(91.850677398352,-6.1102272761821,129.70414224903));
#276170=CARTESIAN_POINT('Ctrl Pts',(91.5722297745392,-4.22837196662692,
135.350372973126));
#276171=CARTESIAN_POINT('Ctrl Pts',(91.2937821507264,1.53915061280415,136.819040427511));
#276172=CARTESIAN_POINT('Ctrl Pts',(91.0153345269133,5.89226897075567,132.76051097));
#276173=CARTESIAN_POINT('Ctrl Pts',(90.7368869031008,4.8306799979248,126.90437490186));
#276174=CARTESIAN_POINT('Ctrl Pts',(90.4584392792875,-0.670067901161403,
124.632135181558));
#276175=CARTESIAN_POINT('Ctrl Pts',(90.1799916554748,-5.5550561337172,128.031869106972));
#276176=CARTESIAN_POINT('Ctrl Pts',(89.9015440316619,-5.3352191589658,133.979387286881));
#276177=CARTESIAN_POINT('Ctrl Pts',(89.6230964078489,-0.212576417070642,
137.009211066365));
#276178=CARTESIAN_POINT('Ctrl Pts',(89.3446487840362,5.10541366717708,134.337080407198));
#276179=CARTESIAN_POINT('Ctrl Pts',(89.0662011602232,5.73177800461257,128.418552844315));
#276180=CARTESIAN_POINT('Ctrl Pts',(88.7877535364103,1.09091836873142,124.69246607186));
#276181=CARTESIAN_POINT('Ctrl Pts',(88.5093059125973,-4.5524419536888,126.58291180426));
#276182=CARTESIAN_POINT('Ctrl Pts',(88.2308582887847,-6.0123305198223,132.352662766849));
#276183=CARTESIAN_POINT('Ctrl Pts',(87.9524106649715,-1.94718105691378,
136.69959969301));
#276184=CARTESIAN_POINT('Ctrl Pts',(87.6739630411587,3.90733267221543,135.629099907278));
#276185=CARTESIAN_POINT('Ctrl Pts',(87.395515417346,6.17119855939173,130.124900415918));
#276186=CARTESIAN_POINT('Ctrl Pts',(87.1170677935327,2.76403445029686,125.245091656395));
#276187=CARTESIAN_POINT('Ctrl Pts',(86.8386201697203,-3.18314228803115,
125.473979486801));
#276188=CARTESIAN_POINT('Ctrl Pts',(86.5601725459069,-6.20516676880425,
130.601227172784));
#276189=CARTESIAN_POINT('Ctrl Pts',(86.2817249220945,-3.52494612829556,
135.915144570902));
#276190=CARTESIAN_POINT('Ctrl Pts',(86.0032772982812,2.394527800925,136.532501191579));
#276191=CARTESIAN_POINT('Ctrl Pts',(85.7248296744686,6.11354766028192,131.885976459962));
#276192=CARTESIAN_POINT('Ctrl Pts',(85.4463820506556,4.21451588324655,126.245499609054));
#276193=CARTESIAN_POINT('Ctrl Pts',(85.1679344268427,-1.55745009994542,
124.794393312227));
#276194=CARTESIAN_POINT('Ctrl Pts',(84.8894868030298,-5.89819552695468,
128.86615336578));
#276195=CARTESIAN_POINT('Ctrl Pts',(84.611039179217,-4.81878740756302,134.719031197036));
#276196=CARTESIAN_POINT('Ctrl Pts',(84.332591555404,0.68885092852684,136.974518008049));
#276197=CARTESIAN_POINT('Ctrl Pts',(84.0541439315912,5.56346891353935,133.559931606153));
#276198=CARTESIAN_POINT('Ctrl Pts',(83.7756963077782,5.32553075757526,127.613110082872));
#276199=CARTESIAN_POINT('Ctrl Pts',(83.4972486839655,0.193690002040587,
124.598891899719));
#276200=CARTESIAN_POINT('Ctrl Pts',(83.2188010601524,-5.11614240308669,
127.287196314267));
#276201=CARTESIAN_POINT('Ctrl Pts',(82.9403534363397,-5.72448987722869,
133.207602900518));
#276202=CARTESIAN_POINT('Ctrl Pts',(82.6619058125266,-1.07231081107503,
136.919547233648));
#276203=CARTESIAN_POINT('Ctrl Pts',(82.3834581887138,4.56526950516122,135.011933810073));
#276204=CARTESIAN_POINT('Ctrl Pts',(82.1050105649009,6.00759017196827,129.237766173961));
#276205=CARTESIAN_POINT('Ctrl Pts',(81.826562941088,1.92922895783247,124.903222299129));
#276206=CARTESIAN_POINT('Ctrl Pts',(81.5481153172751,-3.92199942047723,
125.991536252305));
#276207=CARTESIAN_POINT('Ctrl Pts',(81.2696676934623,-6.16910193169181,
131.502600677615));
#276208=CARTESIAN_POINT('Ctrl Pts',(80.9912200696492,-2.74710114506546,
136.372016598662));
#276209=CARTESIAN_POINT('Ctrl Pts',(80.7127724458365,3.19935139052435,136.125028668197));
#276210=CARTESIAN_POINT('Ctrl Pts',(80.4343248220235,6.20575629522666,130.988606728286));
#276211=CARTESIAN_POINT('Ctrl Pts',(80.1558771982107,3.50937433266497,125.682871613546));
#276212=CARTESIAN_POINT('Ctrl Pts',(79.8774295743978,-2.41195119914859,
125.083534694853));
#276213=CARTESIAN_POINT('Ctrl Pts',(79.5989819505849,-6.11681140931136,
129.741357321249));
#276214=CARTESIAN_POINT('Ctrl Pts',(79.320534326772,-4.20062075716678,135.376028046362));
#276215=CARTESIAN_POINT('Ctrl Pts',(79.0420867029591,1.57573515908161,136.809559742781));
#276216=CARTESIAN_POINT('Ctrl Pts',(78.7636390791462,5.90406744307602,132.724606813414));
#276217=CARTESIAN_POINT('Ctrl Pts',(78.4851914553333,4.80685017661309,126.875041439303));
#276218=CARTESIAN_POINT('Ctrl Pts',(78.2067438315204,-0.707627574471386,
124.636328432103));
#276219=CARTESIAN_POINT('Ctrl Pts',(77.9282962077074,-5.57183015414549,
128.065735678218));
#276220=CARTESIAN_POINT('Ctrl Pts',(77.6498485838947,-5.31579302119528,
134.011805454327));
#276221=CARTESIAN_POINT('Ctrl Pts',(77.3714009600817,-0.174801792692954,
137.010390117845));
#276222=CARTESIAN_POINT('Ctrl Pts',(77.0929533362689,5.12682374375196,134.305936852001));
#276223=CARTESIAN_POINT('Ctrl Pts',(76.814505712456,5.7171487189526,128.38370608822));
#276224=CARTESIAN_POINT('Ctrl Pts',(76.536058088643,1.05369331967776,124.68593858136));
#276225=CARTESIAN_POINT('Ctrl Pts',(76.2576104648302,-4.57805476460059,
126.610702024239));
#276226=CARTESIAN_POINT('Ctrl Pts',(75.9791628410172,-6.00279417061961,
132.389232842773));
#276227=CARTESIAN_POINT('Ctrl Pts',(75.7007152172044,-1.91125898663751,
136.711343511654));
#276228=CARTESIAN_POINT('Ctrl Pts',(75.4222675933915,3.93662983587222,135.605225473025));
#276229=CARTESIAN_POINT('Ctrl Pts',(75.1438199695785,6.16694815427437,130.087347167514));
#276230=CARTESIAN_POINT('Ctrl Pts',(74.8653723457658,2.73014239106432,125.228369194547));
#276231=CARTESIAN_POINT('Ctrl Pts',(74.5869247219528,-3.21553085466319,
125.493454937009));
#276232=CARTESIAN_POINT('Ctrl Pts',(74.3084770981399,-6.20628833237051,
130.639003547736));
#276233=CARTESIAN_POINT('Ctrl Pts',(74.0300294743271,-3.49377002667009,
135.936507227495));
#276234=CARTESIAN_POINT('Ctrl Pts',(73.7515818505141,2.42935225338577,136.517818892029));
#276235=CARTESIAN_POINT('Ctrl Pts',(73.4731342267013,6.1200184930355,131.848741520285));
#276236=CARTESIAN_POINT('Ctrl Pts',(73.1946866028884,4.18668671711015,126.219929119786));
#276237=CARTESIAN_POINT('Ctrl Pts',(72.9162389790755,-1.59400562082267,
124.803985303816));
#276238=CARTESIAN_POINT('Ctrl Pts',(72.6377913552626,-5.90988466472314,
128.902093266552));
#276239=CARTESIAN_POINT('Ctrl Pts',(72.3593437314497,-4.79486841565966,
134.748291993943));
#276240=CARTESIAN_POINT('Ctrl Pts',(72.0808961076369,0.726397665050741,
136.970210458201));
#276241=CARTESIAN_POINT('Ctrl Pts',(71.8024484838239,5.58013977807825,133.526014137426));
#276242=CARTESIAN_POINT('Ctrl Pts',(71.524000860011,5.30600604003494,127.580751192065));
#276243=CARTESIAN_POINT('Ctrl Pts',(71.2455532361981,0.155911964005252,
124.597827826664));
#276244=CARTESIAN_POINT('Ctrl Pts',(70.9671056123853,-5.13745759022245,
127.318404890117));
#276245=CARTESIAN_POINT('Ctrl Pts',(70.6886579885723,-5.70975459779179,
133.242404968692));
#276246=CARTESIAN_POINT('Ctrl Pts',(70.4102103647595,-1.03506606700937,
136.925961393668));
#276247=CARTESIAN_POINT('Ctrl Pts',(70.1317627409465,4.59079761356593,134.98406576223));
#276248=CARTESIAN_POINT('Ctrl Pts',(69.8533151171337,5.99794256020584,129.201225292793));
#276249=CARTESIAN_POINT('Ctrl Pts',(69.5748674933208,1.89327130980037,124.891587869307));
#276250=CARTESIAN_POINT('Ctrl Pts',(69.2964198695077,-3.95122378286636,
126.015499746463));
#276251=CARTESIAN_POINT('Ctrl Pts',(69.0179722456952,-6.16473724709165,
131.540140815303));
#276252=CARTESIAN_POINT('Ctrl Pts',(68.7395246218819,-2.71315834539685,
136.388635827283));
#276253=CARTESIAN_POINT('Ctrl Pts',(68.4610769980694,3.23168053056381,136.105454728543));
#276254=CARTESIAN_POINT('Ctrl Pts',(68.1826293742561,6.20676287530703,130.950827114659));
#276255=CARTESIAN_POINT('Ctrl Pts',(67.9041817504435,3.47813335486666,125.661603945233));
#276256=CARTESIAN_POINT('Ctrl Pts',(67.6257341266304,-2.44673080243567,
125.09832292005));
#276257=CARTESIAN_POINT('Ctrl Pts',(67.3472865028177,-6.12316888174425,
129.778611783445));
#276258=CARTESIAN_POINT('Ctrl Pts',(67.0688388790048,-4.17271389215982,
135.401513714782));
#276259=CARTESIAN_POINT('Ctrl Pts',(66.7903912551918,1.61226131591331,136.799856533191));
#276260=CARTESIAN_POINT('Ctrl Pts',(66.511943631379,5.91564713800617,132.688631501398));
#276261=CARTESIAN_POINT('Ctrl Pts',(66.233496007566,4.78284223570014,126.845853579115));
#276262=CARTESIAN_POINT('Ctrl Pts',(65.9550483837533,-0.745161026381345,
124.640750241348));
#276263=CARTESIAN_POINT('Ctrl Pts',(65.6766007599402,-5.58839770835831,
128.099703730218));
#276264=CARTESIAN_POINT('Ctrl Pts',(65.3981531361275,-5.2961699047596,134.044104768727));
#276265=CARTESIAN_POINT('Ctrl Pts',(65.1197055123145,-0.137020690970298,
137.011339202618));
#276266=CARTESIAN_POINT('Ctrl Pts',(64.8412578885016,5.14804384398771,134.274663544608));
#276267=CARTESIAN_POINT('Ctrl Pts',(64.5628102646887,5.70230758224426,128.348949030369));
#276268=CARTESIAN_POINT('Ctrl Pts',(64.2843626408759,1.01642922563077,124.679637811238));
#276269=CARTESIAN_POINT('Ctrl Pts',(64.0059150170629,-4.60349793400934,
126.638647641779));
#276270=CARTESIAN_POINT('Ctrl Pts',(63.72746739325,-5.9930353856715,132.425744190676));
#276271=CARTESIAN_POINT('Ctrl Pts',(63.4490197694371,-1.87526609395646,
136.722868444874));
#276272=CARTESIAN_POINT('Ctrl Pts',(63.1705721456243,3.96578112626272,135.581173140958));
#276273=CARTESIAN_POINT('Ctrl Pts',(62.8921245218114,6.16246923062527,130.049820488308));
#276274=CARTESIAN_POINT('Ctrl Pts',(62.6136768979985,2.69614916540168,125.211853353112));
#276275=CARTESIAN_POINT('Ctrl Pts',(62.3352292741856,-3.24780026861702,
125.513127184779));
#276276=CARTESIAN_POINT('Ctrl Pts',(62.0567816503727,-6.20717991964031,
130.676786050054));
#276277=CARTESIAN_POINT('Ctrl Pts',(61.7783340265599,-3.46246446211126,
135.957679710507));
#276278=CARTESIAN_POINT('Ctrl Pts',(61.4998864027468,2.46408668530527,136.502924878181));
#276279=CARTESIAN_POINT('Ctrl Pts',(61.2214387789342,6.12626254625314,131.81146788069));
#276280=CARTESIAN_POINT('Ctrl Pts',(60.942991155121,4.15870241175792,126.194528508313));
#276281=CARTESIAN_POINT('Ctrl Pts',(60.6645435313083,-1.63050207523548,
124.813799641521));
#276282=CARTESIAN_POINT('Ctrl Pts',(60.3860959074953,-5.92135480954196,
128.938103656541));
#276283=CARTESIAN_POINT('Ctrl Pts',(60.1076482836825,-4.77077174814381,
134.777406647022));
#276284=CARTESIAN_POINT('Ctrl Pts',(59.8292006598696,0.763917484641806,
136.965674430521));
#276285=CARTESIAN_POINT('Ctrl Pts',(59.5507530360567,5.59660386848551,133.491995816827));
#276286=CARTESIAN_POINT('Ctrl Pts',(59.2723054122438,5.28628470648961,127.548511753291));
#276287=CARTESIAN_POINT('Ctrl Pts',(58.9938577884309,0.11812814859451,124.596993738963));
#276288=CARTESIAN_POINT('Ctrl Pts',(58.715410164618,-5.15858240697801,127.34974263934));
#276289=CARTESIAN_POINT('Ctrl Pts',(58.4369625408051,-5.69480774129836,
133.277116694236));
#276290=CARTESIAN_POINT('Ctrl Pts',(58.1585149169922,-0.997782968190397,
136.932148715521));
#276291=CARTESIAN_POINT('Ctrl Pts',(57.8800672931793,4.61615560827684,134.956042833877));
#276292=CARTESIAN_POINT('Ctrl Pts',(57.6016196693665,5.98807269247603,129.164743816393));
#276293=CARTESIAN_POINT('Ctrl Pts',(57.3231720455535,1.85724350590365,124.880172539454));
#276294=CARTESIAN_POINT('Ctrl Pts',(57.0447244217407,-3.98030173120474,
126.039640693622));
#276295=CARTESIAN_POINT('Ctrl Pts',(56.7662767979277,-6.16014412588574,
131.577653688385));
#276296=CARTESIAN_POINT('Ctrl Pts',(56.4878291741149,-2.67911500864857,
136.405048128532));
#276297=CARTESIAN_POINT('Ctrl Pts',(56.209381550302,3.26388991949243,136.085684354897));
#276298=CARTESIAN_POINT('Ctrl Pts',(55.9309339264891,6.20753946150667,130.913042073662));
#276299=CARTESIAN_POINT('Ctrl Pts',(55.6524863026762,3.44676349355797,125.640526843659));
#276300=CARTESIAN_POINT('Ctrl Pts',(55.3740386788633,-2.48141974121268,
125.113322584571));
#276301=CARTESIAN_POINT('Ctrl Pts',(55.0955910550504,-6.12929945790263,
129.815904255142));
#276302=CARTESIAN_POINT('Ctrl Pts',(54.8171434312375,-4.14465240570495,
135.426829034002));
#276303=CARTESIAN_POINT('Ctrl Pts',(54.5386958074246,1.64872772980914,136.789931158292));
#276304=CARTESIAN_POINT('Ctrl Pts',(54.2602481836117,5.92700762645589,132.652586367033));
#276305=CARTESIAN_POINT('Ctrl Pts',(53.9818005597989,4.75865706480954,126.81681240286));
#276306=CARTESIAN_POINT('Ctrl Pts',(53.703352935986,-0.78266686607524,124.645400445441));
#276307=CARTESIAN_POINT('Ctrl Pts',(53.4249053121731,-5.604758182439,128.133772004274));
#276308=CARTESIAN_POINT('Ctrl Pts',(53.1464576883601,-5.27635053680027,
134.076284033214));
#276309=CARTESIAN_POINT('Ctrl Pts',(52.8680100645473,-0.0992345118958833,
137.012058285519));
#276310=CARTESIAN_POINT('Ctrl Pts',(52.5895624407343,5.1690731815654,134.243261643865));
#276311=CARTESIAN_POINT('Ctrl Pts',(52.3111148169216,5.68725514443172,128.314282958697));
#276312=CARTESIAN_POINT('Ctrl Pts',(52.0326671931086,0.979127467424884,
124.673563994973));
#276313=CARTESIAN_POINT('Ctrl Pts',(51.7542195692957,-4.62877051910935,
126.666747621346));
#276314=CARTESIAN_POINT('Ctrl Pts',(51.4757719454828,-5.98305452659317,
132.462195457613));
#276315=CARTESIAN_POINT('Ctrl Pts',(51.1973243216699,-1.83920371260068,
136.734174065611));
#276316=CARTESIAN_POINT('Ctrl Pts',(50.9188766978571,3.99478546317524,135.556943802347));
#276317=CARTESIAN_POINT('Ctrl Pts',(50.6404290740441,6.15776195441257,130.012321768865));
#276318=CARTESIAN_POINT('Ctrl Pts',(50.3619814502312,2.66205603294,125.195544744091));
#276319=CARTESIAN_POINT('Ctrl Pts',(50.0835338264184,-3.27994933413751,
125.532995501151));
#276320=CARTESIAN_POINT('Ctrl Pts',(49.8050862026055,-6.20784149757545,
130.714573279694));
#276321=CARTESIAN_POINT('Ctrl Pts',(49.5266385787925,-3.43103059465853,
135.978661235386));
#276322=CARTESIAN_POINT('Ctrl Pts',(49.2481909549797,2.4987298095866,136.487819701939));
#276323=CARTESIAN_POINT('Ctrl Pts',(48.9697433311668,6.13227958855924,131.774156922365));
#276324=CARTESIAN_POINT('Ctrl Pts',(48.6912957073539,4.13056400415832,126.169298715863));
#276325=CARTESIAN_POINT('Ctrl Pts',(48.412848083541,-1.66693811079436,124.823835961664));
#276326=CARTESIAN_POINT('Ctrl Pts',(48.1344004597282,-5.93260553638082,
128.974183201367));
#276327=CARTESIAN_POINT('Ctrl Pts',(47.8559528359152,-4.7464982979263,134.806374077418));
#276328=CARTESIAN_POINT('Ctrl Pts',(47.5775052121024,0.801408996989757,
136.960910093092));
#276329=CARTESIAN_POINT('Ctrl Pts',(47.2990575882894,5.61286057467834,133.457877904919));
#276330=CARTESIAN_POINT('Ctrl Pts',(47.0206099644766,5.26636748772036,127.516392961194));
#276331=CARTESIAN_POINT('Ctrl Pts',(46.7421623406636,0.0803399559020909,
124.596389667526));
#276332=CARTESIAN_POINT('Ctrl Pts',(46.4637147168508,-5.17951607056515,
127.381208400702));
#276333=CARTESIAN_POINT('Ctrl Pts',(46.1852670930379,-5.67964986161014,
133.311736790894));
#276334=CARTESIAN_POINT('Ctrl Pts',(45.9068194692249,-0.960462896156299,
136.938108969933));
#276335=CARTESIAN_POINT('Ctrl Pts',(45.6283718454121,4.64134254964412,134.927866063412));
#276336=CARTESIAN_POINT('Ctrl Pts',(45.3499242215992,5.97798093451044,129.128323096598));
#276337=CARTESIAN_POINT('Ctrl Pts',(45.0714765977863,1.82114688116607,124.868976732569));
#276338=CARTESIAN_POINT('Ctrl Pts',(44.7930289739735,-4.00923218799886,
126.063958199228));
#276339=CARTESIAN_POINT('Ctrl Pts',(44.5145813501605,-6.15532273827383,
131.615137906808));
#276340=CARTESIAN_POINT('Ctrl Pts',(44.2361337263477,-2.644972396308,136.421252894246));
#276341=CARTESIAN_POINT('Ctrl Pts',(43.9576861025347,3.29597836378001,136.065718279858));
#276342=CARTESIAN_POINT('Ctrl Pts',(43.6792384787219,6.20808602504863,130.875253005433));
#276343=CARTESIAN_POINT('Ctrl Pts',(43.4007908549089,3.41526591116036,125.619641089845));
#276344=CARTESIAN_POINT('Ctrl Pts',(43.1223432310961,-2.5160167300689,125.128533132602));
#276345=CARTESIAN_POINT('Ctrl Pts',(42.8438956072832,-6.13520291061547,
129.853233354452));
#276346=CARTESIAN_POINT('Ctrl Pts',(42.5654479834703,-4.11643733763101,
135.451973065955));
#276347=CARTESIAN_POINT('Ctrl Pts',(42.2870003596574,1.68513304949262,136.779783985877));
#276348=CARTESIAN_POINT('Ctrl Pts',(42.0085527358444,5.93814848745852,132.616472745983));
#276349=CARTESIAN_POINT('Ctrl Pts',(41.7301051120316,4.73429556013123,126.787918986671));
#276350=CARTESIAN_POINT('Ctrl Pts',(41.4516574882187,-0.820143703760798,
124.65027887207));
#276351=CARTESIAN_POINT('Ctrl Pts',(41.1732098644058,-5.62091097014408,
128.167939237972));
#276352=CARTESIAN_POINT('Ctrl Pts',(40.8947622405929,-5.25633565173145,
134.108342055376));
#276353=CARTESIAN_POINT('Ctrl Pts',(40.61631461678,-0.0614446556499193,
137.012547339898));
#276354=CARTESIAN_POINT('Ctrl Pts',(40.3378669929672,5.18991097723558,134.211732313379));
#276355=CARTESIAN_POINT('Ctrl Pts',(40.0594193691542,5.67199196328813,128.279709157768));
#276356=CARTESIAN_POINT('Ctrl Pts',(39.7809717453414,0.941789427290636,
124.66771735763));
#276357=CARTESIAN_POINT('Ctrl Pts',(39.5025241215285,-4.65387158341555,
126.695000921683));
#276358=CARTESIAN_POINT('Ctrl Pts',(39.2240764977156,-5.97285196322902,
132.49858529287));
#276359=CARTESIAN_POINT('Ctrl Pts',(38.9456288739027,-1.80307317887526,
136.745259954929));
#276360=CARTESIAN_POINT('Ctrl Pts',(38.6671812500898,4.02364177184326,135.532538355018));
#276361=CARTESIAN_POINT('Ctrl Pts',(38.3887336262769,6.15282650006613,129.974852398711));
#276362=CARTESIAN_POINT('Ctrl Pts',(38.110286002464,2.62786425701304,125.179443971804));
#276363=CARTESIAN_POINT('Ctrl Pts',(37.8318383786511,-3.31197685992897,
125.553059149895));
#276364=CARTESIAN_POINT('Ctrl Pts',(37.5533907548383,-6.20827304166094,
130.752363836438));
#276365=CARTESIAN_POINT('Ctrl Pts',(37.2749431310254,-3.3994695891056,135.999451024653));
#276366=CARTESIAN_POINT('Ctrl Pts',(36.9964955072125,2.53328034251594,136.47250392303));
#276367=CARTESIAN_POINT('Ctrl Pts',(36.7180478833995,6.13806939699002,131.73681002788));
#276368=CARTESIAN_POINT('Ctrl Pts',(36.4396002595867,4.10227253699055,126.144240677337));
#276369=CARTESIAN_POINT('Ctrl Pts',(36.1611526357737,-1.70331237734853,
124.834093892349));
#276370=CARTESIAN_POINT('Ctrl Pts',(35.8827050119609,-5.94363642833981,
129.01033056409));
#276371=CARTESIAN_POINT('Ctrl Pts',(35.604257388148,-4.72204896446884,134.835193211735));
#276372=CARTESIAN_POINT('Ctrl Pts',(35.3258097643351,0.838870812832614,
136.955917622458));
#276373=CARTESIAN_POINT('Ctrl Pts',(35.0473621405222,5.62890929425843,133.423661665951));
#276374=CARTESIAN_POINT('Ctrl Pts',(34.7689145167094,5.24625512176713,127.484396005948));
#276375=CARTESIAN_POINT('Ctrl Pts',(34.4904668928964,0.0425487861828518,
124.596015634733));
#276376=CARTESIAN_POINT('Ctrl Pts',(34.2120192690835,-5.20025780527969,
127.412801008228));
#276377=CARTESIAN_POINT('Ctrl Pts',(33.9335716452707,-5.66428152040741,
133.346263975806));
#276378=CARTESIAN_POINT('Ctrl Pts',(33.6551240214578,-0.923107233816384,
136.943841936043));
#276379=CARTESIAN_POINT('Ctrl Pts',(33.3766763976448,4.66635750435639,134.899536494936));
#276380=CARTESIAN_POINT('Ctrl Pts',(33.098228773832,5.96766766026296,129.091964482989));
#276381=CARTESIAN_POINT('Ctrl Pts',(32.8197811500191,1.78498277316083,124.858000863516));
#276382=CARTESIAN_POINT('Ctrl Pts',(32.5413335262063,-4.03801408121996,
126.08845136219));
#276383=CARTESIAN_POINT('Ctrl Pts',(32.2628859023933,-6.15027326291425,
131.65259208158));
#276384=CARTESIAN_POINT('Ctrl Pts',(31.9844382785804,-2.6107317735426,136.437249523951));
#276385=CARTESIAN_POINT('Ctrl Pts',(31.7059906547675,3.32794467437699,136.045557243275));
#276386=CARTESIAN_POINT('Ctrl Pts',(31.4275430309546,6.20840254567991,130.837461310262));
#276387=CARTESIAN_POINT('Ctrl Pts',(31.1490954071417,3.3836417748287,125.598947457719));
#276388=CARTESIAN_POINT('Ctrl Pts',(30.8706477833288,-2.55052048699994,
125.143954000505));
#276389=CARTESIAN_POINT('Ctrl Pts',(30.5922001595159,-6.14087902112821,
129.890597698133));
#276390=CARTESIAN_POINT('Ctrl Pts',(30.3137525357031,-4.08806973345779,
135.476944878919));
#276391=CARTESIAN_POINT('Ctrl Pts',(30.0353049118902,1.72147592595096,136.769415391952));
#276392=CARTESIAN_POINT('Ctrl Pts',(29.7568572880773,5.94906930818524,132.58029197645));
#276393=CARTESIAN_POINT('Ctrl Pts',(29.4784096642643,4.70975862438989,126.759174401203));
#276394=CARTESIAN_POINT('Ctrl Pts',(29.1999620404515,-0.857590150719802,
124.65538534046));
#276395=CARTESIAN_POINT('Ctrl Pts',(28.9215144166386,-5.63685547292606,
128.202204165235));
#276396=CARTESIAN_POINT('Ctrl Pts',(28.6430667928257,-5.23612599121204,
134.140277647291));
#276397=CARTESIAN_POINT('Ctrl Pts',(28.3646191690128,-0.0236525225496446,
137.012806347637));
#276398=CARTESIAN_POINT('Ctrl Pts',(28.0861715451999,5.2105564588459,134.180076721482));
#276399=CARTESIAN_POINT('Ctrl Pts',(27.807723921387,5.65651860439647,128.245228908728));
#276400=CARTESIAN_POINT('Ctrl Pts',(27.5292762975741,0.904416488802812,
124.662098115861));
#276401=CARTESIAN_POINT('Ctrl Pts',(27.2508286737613,-4.67880019679877,
126.723406495856));
#276402=CARTESIAN_POINT('Ctrl Pts',(26.9723810499484,-5.96242807363892,
132.53491234801));
#276403=CARTESIAN_POINT('Ctrl Pts',(26.6939334261354,-1.76687583160983,
136.756125702037));
#276404=CARTESIAN_POINT('Ctrl Pts',(26.4154858023226,4.05234898298581,135.507957703324));
#276405=CARTESIAN_POINT('Ctrl Pts',(26.1370381785097,6.14766305047102,129.937413766291));
#276406=CARTESIAN_POINT('Ctrl Pts',(25.8585905546968,2.59357510460964,125.163551632871));
#276407=CARTESIAN_POINT('Ctrl Pts',(25.5801429308839,-3.34388165920016,
125.573317387547));
#276408=CARTESIAN_POINT('Ctrl Pts',(25.301695307071,-6.2084745359058,130.790156319941));
#276409=CARTESIAN_POINT('Ctrl Pts',(25.0232476832582,-3.36778261495664,
136.020048307934));
#276410=CARTESIAN_POINT('Ctrl Pts',(24.7448000594452,2.56773700381057,136.456978108987));
#276411=CARTESIAN_POINT('Ctrl Pts',(24.4663524356323,6.14363175700203,131.69942858114));
#276412=CARTESIAN_POINT('Ctrl Pts',(24.1879048118195,4.07382905860539,126.11935532127));
#276413=CARTESIAN_POINT('Ctrl Pts',(23.9094571880065,-1.73962352703587,
124.844573053462));
#276414=CARTESIAN_POINT('Ctrl Pts',(23.6310095641937,-5.95444707666522,
129.046544405257));
#276415=CARTESIAN_POINT('Ctrl Pts',(23.3525619403807,-4.69742465375045,
134.863862982068));
#276416=CARTESIAN_POINT('Ctrl Pts',(23.0741143165679,0.876301544009003,
136.950697203617));
#276417=CARTESIAN_POINT('Ctrl Pts',(22.795666692755,5.64474943253441,133.389348367819));
#276418=CARTESIAN_POINT('Ctrl Pts',(22.5172190689421,5.22594835390121,127.452522073212));
#276419=CARTESIAN_POINT('Ctrl Pts',(22.2387714451292,0.0047560398029127,
124.595871654449));
#276420=CARTESIAN_POINT('Ctrl Pts',(21.9603238213163,-5.22080684252888,
127.444519291243));
#276421=CARTESIAN_POINT('Ctrl Pts',(21.6818761975034,-5.64870328716988,
133.380696969555));
#276422=CARTESIAN_POINT('Ctrl Pts',(21.4034285736905,-0.885717365398449,
136.949347401415));
#276423=CARTESIAN_POINT('Ctrl Pts',(21.1249809498776,4.69119954547528,134.871055178212));
#276424=CARTESIAN_POINT('Ctrl Pts',(20.8465333260648,5.95713325189572,129.055669322849));
#276425=CARTESIAN_POINT('Ctrl Pts',(20.5680857022518,1.74875252196249,124.847245339011));
#276426=CARTESIAN_POINT('Ctrl Pts',(20.289638078439,-4.06664634434428,126.113119274905));
#276427=CARTESIAN_POINT('Ctrl Pts',(20.011190454626,-6.14499588691713,131.690014824823));
#276428=CARTESIAN_POINT('Ctrl Pts',(19.7327428308132,-2.57639440915122,
136.453037424885));
#276429=CARTESIAN_POINT('Ctrl Pts',(19.4542952070003,3.35978766676044,136.025201992224));
#276430=CARTESIAN_POINT('Ctrl Pts',(19.1758475831874,6.20848901167171,130.799668388532));
#276431=CARTESIAN_POINT('Ctrl Pts',(18.8973999593745,3.3518922564065,125.578446714094));
#276432=CARTESIAN_POINT('Ctrl Pts',(18.6189523355616,-2.58492973345636,
125.159584616859));
#276433=CARTESIAN_POINT('Ctrl Pts',(18.3405047117487,-6.14632757911053,
129.927995901635));
#276434=CARTESIAN_POINT('Ctrl Pts',(18.0620570879358,-4.05955064435711,
135.501743547556));
#276435=CARTESIAN_POINT('Ctrl Pts',(17.7836094641229,1.75775501248606,136.758825760728));
#276436=CARTESIAN_POINT('Ctrl Pts',(17.5051618403101,5.95976968396092,132.544045399129));
#276437=CARTESIAN_POINT('Ctrl Pts',(17.2267142164972,4.68504716681072,126.730579711598));
#276438=CARTESIAN_POINT('Ctrl Pts',(16.9482665926842,-0.8950048193604,124.660719661391));
#276439=CARTESIAN_POINT('Ctrl Pts',(16.6698189688713,-5.65259109995534,
128.236565516362));
#276440=CARTESIAN_POINT('Ctrl Pts',(16.3913713450585,-5.21572230411858,
134.172089625574));
#276441=CARTESIAN_POINT('Ctrl Pts',(16.1129237212456,0.0141404870033325,
137.012835299135));
#276442=CARTESIAN_POINT('Ctrl Pts',(15.8344760974327,5.23100886137047,134.148296041183));
#276443=CARTESIAN_POINT('Ctrl Pts',(15.5560284736198,5.64083564112771,128.210843489254));
#276444=CARTESIAN_POINT('Ctrl Pts',(15.2775808498069,0.8670100368296,124.656706477888));
#276445=CARTESIAN_POINT('Ctrl Pts',(14.999133225994,-4.70355543551987,126.751963291284));
#276446=CARTESIAN_POINT('Ctrl Pts',(14.7206856021811,-5.95178324408404,
132.571175276918));
#276447=CARTESIAN_POINT('Ctrl Pts',(14.4422379783683,-1.73061301211068,
136.766770904302));
#276448=CARTESIAN_POINT('Ctrl Pts',(14.1637903545553,4.08090603284655,135.48320275811));
#276449=CARTESIAN_POINT('Ctrl Pts',(13.8853427307424,6.14227179696077,129.900007258904));
#276450=CARTESIAN_POINT('Ctrl Pts',(13.6068951069296,2.55918984632695,125.147868316191));
#276451=CARTESIAN_POINT('Ctrl Pts',(13.3284474831167,-3.37566254970675,
125.593769463429));
#276452=CARTESIAN_POINT('Ctrl Pts',(13.0499998593037,-6.20844597284355,
130.827949329789));
#276453=CARTESIAN_POINT('Ctrl Pts',(12.7715522354909,-3.33597084638438,
136.04045232199));
#276454=CARTESIAN_POINT('Ctrl Pts',(12.493104611678,2.60209851666622,136.441242835124));
#276455=CARTESIAN_POINT('Ctrl Pts',(12.2146569878651,6.14896646247997,131.662013967328));
#276456=CARTESIAN_POINT('Ctrl Pts',(11.9362093640522,4.04523462298623,126.094643569795));
#276457=CARTESIAN_POINT('Ctrl Pts',(11.6577617402393,-1.77587021433397,
124.855273056695));
#276458=CARTESIAN_POINT('Ctrl Pts',(11.3793141164265,-5.96503708076441,
129.08282338295));
#276459=CARTESIAN_POINT('Ctrl Pts',(11.1008664926135,-4.67262627823404,
134.892382326048));
#276460=CARTESIAN_POINT('Ctrl Pts',(10.8224188688007,0.913699803509421,
136.945249030013));
#276461=CARTESIAN_POINT('Ctrl Pts',(10.5439712449878,5.6603804025445,133.354939282016));
#276462=CARTESIAN_POINT('Ctrl Pts',(10.2655236211749,5.20544793659703,127.420772344084));
#276463=CARTESIAN_POINT('Ctrl Pts',(9.98707599736195,-0.0330368828140487,
124.595957732005));
#276464=CARTESIAN_POINT('Ctrl Pts',(9.70862837354909,-5.24116242086055,
127.476362074414));
#276465=CARTESIAN_POINT('Ctrl Pts',(9.43018074973619,-5.63291573915475,
133.415034496211));
#276466=CARTESIAN_POINT('Ctrl Pts',(9.15173312592329,-0.848294676398009,
136.954625162043));
#276467=CARTESIAN_POINT('Ctrl Pts',(8.87328550211039,4.71586775246963,134.842423168626));
#276468=CARTESIAN_POINT('Ctrl Pts',(8.59483787829755,5.94637809976527,129.019438961107));
#276469=CARTESIAN_POINT('Ctrl Pts',(8.3163902544846,1.71245747009635,124.836710557603));
#276470=CARTESIAN_POINT('Ctrl Pts',(8.03794263067172,-4.09512791639282,
126.137961023291));
#276471=CARTESIAN_POINT('Ctrl Pts',(7.75949500685887,-6.1394908058375,131.727404749824));
#276472=CARTESIAN_POINT('Ctrl Pts',(7.48104738304595,-2.54196157551782,
136.468616012024));
#276473=CARTESIAN_POINT('Ctrl Pts',(7.20259975923305,3.39150616097622,136.004653280976));
#276474=CARTESIAN_POINT('Ctrl Pts',(6.92415213542018,6.20834541982004,130.761875640674));
#276475=CARTESIAN_POINT('Ctrl Pts',(6.64570451160728,3.32001853238404,125.558139618628));
#276476=CARTESIAN_POINT('Ctrl Pts',(6.36725688779438,-2.61924319439064,
125.175424402463));
#276477=CARTESIAN_POINT('Ctrl Pts',(6.08880926398148,-6.15154838266407,
129.965426579154));
#276478=CARTESIAN_POINT('Ctrl Pts',(5.81036164016863,-4.03088112711464,
135.52636815294));
#276479=CARTESIAN_POINT('Ctrl Pts',(5.53191401635571,1.79396896476278,136.748015484609));
#276480=CARTESIAN_POINT('Ctrl Pts',(5.2534663925428,5.97024921827925,132.507734357147));
#276481=CARTESIAN_POINT('Ctrl Pts',(4.97501876872993,4.66016210308585,126.702135977443));
#276482=CARTESIAN_POINT('Ctrl Pts',(4.69657114491704,-0.932386323268277,
124.666281637197));
#276483=CARTESIAN_POINT('Ctrl Pts',(4.41812352110413,-5.66811726814286,
128.27102201808));
#276484=CARTESIAN_POINT('Ctrl Pts',(4.13967589729124,-5.19512534651691,
134.203776811419));
#276485=CARTESIAN_POINT('Ctrl Pts',(3.86122827347838,0.051932972575587,
137.012634193321));
#276486=CARTESIAN_POINT('Ctrl Pts',(3.58278064966546,5.25126742693796,134.116391450127));
#276487=CARTESIAN_POINT('Ctrl Pts',(3.30433302585255,5.62494365461986,128.176554173511));
#276488=CARTESIAN_POINT('Ctrl Pts',(3.02588540203969,0.829571457480427,
124.651542643499));
#276489=CARTESIAN_POINT('Ctrl Pts',(2.74743777822681,-4.72813638226476,
126.780670249786));
#276490=CARTESIAN_POINT('Ctrl Pts',(2.46899015441389,-5.9409178690121,132.607372735859));
#276491=CARTESIAN_POINT('Ctrl Pts',(2.19054253060099,-1.69428606410994,
136.77719516726));
#276492=CARTESIAN_POINT('Ctrl Pts',(1.91209490678813,4.10931186323347,135.458274436681));
#276493=CARTESIAN_POINT('Ctrl Pts',(1.63364728297522,6.13665293931019,129.862634262664));
#276494=CARTESIAN_POINT('Ctrl Pts',(1.35519965916232,2.52470975632363,125.132394602912));
#276495=CARTESIAN_POINT('Ctrl Pts',(1.07675203534945,-3.40731835379603,
125.614414619682));
#276496=CARTESIAN_POINT('Ctrl Pts',(0.798304411536565,-6.20818735353264,
130.86574146555));
#276497=CARTESIAN_POINT('Ctrl Pts',(0.519856787723634,-3.30403546218559,
136.060662310741));
#276498=CARTESIAN_POINT('Ctrl Pts',(0.241409163910791,2.63636360780418,
136.425298684517));
#276499=CARTESIAN_POINT('Ctrl Pts',(-0.0370384599021062,6.15407331574431,
131.624567572855));
#276500=CARTESIAN_POINT('Ctrl Pts',(-0.315486083715014,4.01649028971072,
126.070106338619));
#276501=CARTESIAN_POINT('Ctrl Pts',(-0.593933707527915,-1.81205109610819,
124.866193505555));
#276502=CARTESIAN_POINT('Ctrl Pts',(-0.872381331340776,-5.97540604822092,
129.119166152838));
#276503=CARTESIAN_POINT('Ctrl Pts',(-1.15082895515369,-4.6476547568326,
134.920750186879));
#276504=CARTESIAN_POINT('Ctrl Pts',(-1.42927657896659,0.951064205527318,
136.939573303531));
#276505=CARTESIAN_POINT('Ctrl Pts',(-1.70772420277945,5.67580162507719,
133.320435683583));
#276506=CARTESIAN_POINT('Ctrl Pts',(-1.98617182659235,5.18475462950527,
127.389147995065));
#276507=CARTESIAN_POINT('Ctrl Pts',(-2.26461945040527,-0.0708285812371651,
124.596273864213));
#276508=CARTESIAN_POINT('Ctrl Pts',(-2.54306707421816,-5.26132378599129,
127.508328177794));
#276509=CARTESIAN_POINT('Ctrl Pts',(-2.82151469803103,-5.61691946137538,
133.449275283389));
#276510=CARTESIAN_POINT('Ctrl Pts',(-3.09996232184393,-0.810840553526189,
136.959675022356));
#276511=CARTESIAN_POINT('Ctrl Pts',(-3.37840994565684,4.74036121125036,
134.813641527147));
#276512=CARTESIAN_POINT('Ctrl Pts',(-3.6568575694697,5.93540260240737,128.983274740293));
#276513=CARTESIAN_POINT('Ctrl Pts',(-3.9353051932826,1.6760989624889,124.826396909662));
#276514=CARTESIAN_POINT('Ctrl Pts',(-4.21375281709551,-4.12345774197041,
126.162975686831));
#276515=CARTESIAN_POINT('Ctrl Pts',(-4.49220044090841,-6.13375822366836,
131.764760471086));
#276516=CARTESIAN_POINT('Ctrl Pts',(-4.77064806472125,-2.50743454856317,
136.483984708096));
#276517=CARTESIAN_POINT('Ctrl Pts',(-5.04909568853418,3.4230989816841,135.983911870971));
#276518=CARTESIAN_POINT('Ctrl Pts',(-5.32754331234708,6.20797177544568,
130.724084467112));
#276519=CARTESIAN_POINT('Ctrl Pts',(-5.60599093615995,3.28802178385396,
125.538026923812));
#276520=CARTESIAN_POINT('Ctrl Pts',(-5.88443855997284,-2.65345959830539,
125.191472770368));
#276521=CARTESIAN_POINT('Ctrl Pts',(-6.16288618378574,-6.15654123833006,
130.002888343683));
#276522=CARTESIAN_POINT('Ctrl Pts',(-6.44133380759864,-4.00206224408943,
135.550817782599));
#276523=CARTESIAN_POINT('Ctrl Pts',(-6.71978143141151,1.83011644085978,
136.736984964173));
#276524=CARTESIAN_POINT('Ctrl Pts',(-6.9982290552244,5.98050752281724,132.471360196026));
#276525=CARTESIAN_POINT('Ctrl Pts',(-7.27667667903734,4.63510435534053,
126.673844252731));
#276526=CARTESIAN_POINT('Ctrl Pts',(-7.55512430285017,-0.969733277257762,
124.672071061776));
#276527=CARTESIAN_POINT('Ctrl Pts',(-7.83357192666308,-5.68343340216059,
128.305572393592));
#276528=CARTESIAN_POINT('Ctrl Pts',(-8.112019550476,-5.17433588163501,134.235338030648));
#276529=CARTESIAN_POINT('Ctrl Pts',(-8.39046717428886,0.0897235337524442,
137.012203037646));
#276530=CARTESIAN_POINT('Ctrl Pts',(-8.66891479810176,5.27133140485959,
134.084364130551));
#276531=CARTESIAN_POINT('Ctrl Pts',(-8.94736242191464,5.60884323375645,
128.142362232103));
#276532=CARTESIAN_POINT('Ctrl Pts',(-9.22581004572757,0.792102138056052,
124.646606804043));
#276533=CARTESIAN_POINT('Ctrl Pts',(-9.50425766954039,-4.75254212617725,
126.809526307613));
#276534=CARTESIAN_POINT('Ctrl Pts',(-9.78270529335335,-5.92983235104376,
132.643503383524));
#276535=CARTESIAN_POINT('Ctrl Pts',(-10.0611529171662,-1.65789633371603,
136.787398104638));
#276536=CARTESIAN_POINT('Ctrl Pts',(-10.3396005409791,4.13756542155812,
135.433173662763));
#276537=CARTESIAN_POINT('Ctrl Pts',(-10.618048164792,6.13080668572826,129.82529616244));
#276538=CARTESIAN_POINT('Ctrl Pts',(-10.8964957886049,2.49013611227157,
125.11713106642));
#276539=CARTESIAN_POINT('Ctrl Pts',(-11.1749434124178,-3.4388478984508,
125.635252091294));
#276540=CARTESIAN_POINT('Ctrl Pts',(-11.4533910362307,-6.20769868755626,
130.90353132682));
#276541=CARTESIAN_POINT('Ctrl Pts',(-11.7318386600436,-3.2719776457377,
136.080677525301));
#276542=CARTESIAN_POINT('Ctrl Pts',(-12.0102862838565,2.67053100751937,
136.409146247984));
#276543=CARTESIAN_POINT('Ctrl Pts',(-12.2887339076694,6.15895212755882,
131.587090785312));
#276544=CARTESIAN_POINT('Ctrl Pts',(-12.5671815314823,3.98759712391021,
126.045744536976));
#276545=CARTESIAN_POINT('Ctrl Pts',(-12.8456291552951,-1.84816483166266,
124.877333995382));
#276546=CARTESIAN_POINT('Ctrl Pts',(-13.1240767791081,-5.98555359480885,
129.155571368227));
#276547=CARTESIAN_POINT('Ctrl Pts',(-13.4025244029209,-4.62251101487491,
134.948965513381));
#276548=CARTESIAN_POINT('Ctrl Pts',(-13.6809720267338,0.988393365511613,
136.933670234486));
#276549=CARTESIAN_POINT('Ctrl Pts',(-13.9594196505467,5.69101252869335,
133.285838851062));
#276550=CARTESIAN_POINT('Ctrl Pts',(-14.2378672743596,5.16386919942402,
127.357650198006));
#276551=CARTESIAN_POINT('Ctrl Pts',(-14.5163148981725,-0.108617655081171,
124.59682003936));
#276552=CARTESIAN_POINT('Ctrl Pts',(-14.7947625219854,-5.28129019083405,
127.540416416869));
#276553=CARTESIAN_POINT('Ctrl Pts',(-15.0732101457983,-5.60071504657988,
133.483418062279));
#276554=CARTESIAN_POINT('Ctrl Pts',(-15.3516577696111,-0.77335638465969,
136.96449679523));
#276555=CARTESIAN_POINT('Ctrl Pts',(-15.6301053934241,4.76467901420313,
134.784711320289));
#276556=CARTESIAN_POINT('Ctrl Pts',(-15.908553017237,5.92420716652329,128.947178000488));
#276557=CARTESIAN_POINT('Ctrl Pts',(-16.1870006410499,1.63967834641818,
124.816304777366));
#276558=CARTESIAN_POINT('Ctrl Pts',(-16.4654482648627,-4.15163477130477,
126.188162338596));
#276559=CARTESIAN_POINT('Ctrl Pts',(-16.7438958886757,-6.12779835283271,
131.802080604377));
#276560=CARTESIAN_POINT('Ctrl Pts',(-17.0223435124885,-2.4728146076992,
136.499142943608));
#276561=CARTESIAN_POINT('Ctrl Pts',(-17.3007911363014,3.45456495820035,
135.96297853079));
#276562=CARTESIAN_POINT('Ctrl Pts',(-17.5792387601143,6.20736809239421,
130.686296268213));
#276563=CARTESIAN_POINT('Ctrl Pts',(-17.8576863839272,3.25590319646751,
125.518109374927));
#276564=CARTESIAN_POINT('Ctrl Pts',(-18.13613400774,-2.6875776772989,125.207729125896));
#276565=CARTESIAN_POINT('Ctrl Pts',(-18.414581631553,-6.16130596109642,
130.040379807061));
#276566=CARTESIAN_POINT('Ctrl Pts',(-18.6930292553659,-3.97309506317598,
135.575091530542));
#276567=CARTESIAN_POINT('Ctrl Pts',(-18.9714768791788,1.86619610131902,
136.72573460816));
#276568=CARTESIAN_POINT('Ctrl Pts',(-19.2499245029916,5.99054421744964,
132.434924263623));
#276569=CARTESIAN_POINT('Ctrl Pts',(-19.5283721268046,4.6098748520987,126.645705585822));
#276570=CARTESIAN_POINT('Ctrl Pts',(-19.8068197506174,-1.00704429742433,
124.678087720601));
#276571=CARTESIAN_POINT('Ctrl Pts',(-20.0852673744304,-5.6985389344635,
128.340215362621));
#276572=CARTESIAN_POINT('Ctrl Pts',(-20.3637149982432,-5.15335467983417,
134.266772113748));
#276573=CARTESIAN_POINT('Ctrl Pts',(-20.6421626220562,0.127510770190762,
137.011541848088));
#276574=CARTESIAN_POINT('Ctrl Pts',(-20.920610245869,5.29120005165768,134.05221526924));
#276575=CARTESIAN_POINT('Ctrl Pts',(-21.1990578696819,5.59253497514422,
128.108268932023));
#276576=CARTESIAN_POINT('Ctrl Pts',(-21.4775054934948,0.754603466995427,
124.64189914242));
#276577=CARTESIAN_POINT('Ctrl Pts',(-21.7559531173077,-4.77677176289349,
126.838530395495));
#276578=CARTESIAN_POINT('Ctrl Pts',(-22.0344007411205,-5.91852710095694,
132.679565881077));
#276579=CARTESIAN_POINT('Ctrl Pts',(-22.3128483649335,-1.62144516936395,
136.797379338361));
#276580=CARTESIAN_POINT('Ctrl Pts',(-22.5912959887463,4.16566566087426,
135.407901366475));
#276581=CARTESIAN_POINT('Ctrl Pts',(-22.8697436125593,6.12473325285015,
129.787994341809));
#276582=CARTESIAN_POINT('Ctrl Pts',(-23.1481912363721,2.45547019531011,
125.102078272311));
#276583=CARTESIAN_POINT('Ctrl Pts',(-23.426638860185,-3.47025001533206,
125.656281106122));
#276584=CARTESIAN_POINT('Ctrl Pts',(-23.7050864839979,-6.20697999302203,
130.941317513284));
#276585=CARTESIAN_POINT('Ctrl Pts',(-23.9835341078108,-3.23979858495512,
136.100497223997));
#276586=CARTESIAN_POINT('Ctrl Pts',(-24.2619817316237,2.70459944972584,
136.392786124057));
#276587=CARTESIAN_POINT('Ctrl Pts',(-24.5404293554366,6.16360271713728,
131.549584993415));
#276588=CARTESIAN_POINT('Ctrl Pts',(-24.8188769792495,3.95855619623184,
126.021559067602));
#276589=CARTESIAN_POINT('Ctrl Pts',(-25.0973246030624,-1.88421008278963,
124.88869411336));
#276590=CARTESIAN_POINT('Ctrl Pts',(-25.3757722268753,-5.99547934450715,
129.192037680109));
#276591=CARTESIAN_POINT('Ctrl Pts',(-25.6542198506882,-4.59719598407162,
134.977027260026));
#276592=CARTESIAN_POINT('Ctrl Pts',(-25.932667474501,1.02568590021626,136.92754004162));
#276593=CARTESIAN_POINT('Ctrl Pts',(-26.211115098314,5.7060125497474,133.251150066453));
#276594=CARTESIAN_POINT('Ctrl Pts',(-26.4895627221268,5.14279242027056,
127.326280120068));
#276595=CARTESIAN_POINT('Ctrl Pts',(-26.7680103459397,-0.146402704058008,
124.597596237205));
#276596=CARTESIAN_POINT('Ctrl Pts',(-27.0464579697526,-5.30106089552683,
127.572625602596));
#276597=CARTESIAN_POINT('Ctrl Pts',(-27.3249055935655,-5.58430309522854,
133.517461567711));
#276598=CARTESIAN_POINT('Ctrl Pts',(-27.6033532173784,-0.735843558787732,
136.969090301993));
#276599=CARTESIAN_POINT('Ctrl Pts',(-27.8818008411913,4.78882026022281,
134.755633620073));
#276600=CARTESIAN_POINT('Ctrl Pts',(-28.1602484650042,5.91279220696403,
128.911150079267));
#276601=CARTESIAN_POINT('Ctrl Pts',(-28.4386960888171,1.60319697146318,
124.806434534681));
#276602=CARTESIAN_POINT('Ctrl Pts',(-28.7171437126299,-4.17965796028613,
126.213520045287));
#276603=CARTESIAN_POINT('Ctrl Pts',(-28.9955913364429,-6.12161141417542,
131.839363766787));
#276604=CARTESIAN_POINT('Ctrl Pts',(-29.2740389602557,-2.43810303578058,
136.514090156867));
#276605=CARTESIAN_POINT('Ctrl Pts',(-29.5524865840687,3.48590292454168,
135.941854036124));
#276606=CARTESIAN_POINT('Ctrl Pts',(-29.8309342078815,6.20653439303521,
130.648512444231));
#276607=CARTESIAN_POINT('Ctrl Pts',(-30.1093818316944,3.22366396039099,
125.498387710026));
#276608=CARTESIAN_POINT('Ctrl Pts',(-30.3878294555073,-2.72159616711309,
125.224192866663));
#276609=CARTESIAN_POINT('Ctrl Pts',(-30.6662770793202,-6.16584237440457,
130.077899580028));
#276610=CARTESIAN_POINT('Ctrl Pts',(-30.9447247031331,-3.94398065776386,
135.599188497297));
#276611=CARTESIAN_POINT('Ctrl Pts',(-31.2231723269461,1.90220660919519,
136.714264833456));
#276612=CARTESIAN_POINT('Ctrl Pts',(-31.5016199507588,6.00035893026297,
132.398427910084));
#276613=CARTESIAN_POINT('Ctrl Pts',(-31.7800675745718,4.58447452824918,
126.617721019404));
#276614=CARTESIAN_POINT('Ctrl Pts',(-32.0585151983846,-1.04431800119413,
124.68433139072));
#276615=CARTESIAN_POINT('Ctrl Pts',(-32.3369628221976,-5.71343330531054,
128.374949641459));
#276616=CARTESIAN_POINT('Ctrl Pts',(-32.6154104460104,-5.1321825185805,
134.298077895915));
#276617=CARTESIAN_POINT('Ctrl Pts',(-32.8938580698234,0.165293281670594,
137.010650649146));
#276618=CARTESIAN_POINT('Ctrl Pts',(-33.1723056936362,5.31087263109202,
134.019946057479));
#276619=CARTESIAN_POINT('Ctrl Pts',(-33.4507533174492,5.57601948309184,
128.074275536613));
#276620=CARTESIAN_POINT('Ctrl Pts',(-33.729200941262,0.717076833825826,
124.637419833072));
#276621=CARTESIAN_POINT('Ctrl Pts',(-34.0076485650749,-4.80082439457541,
126.867681438675));
#276622=CARTESIAN_POINT('Ctrl Pts',(-34.2860961888878,-5.90700253767186,
132.715558892209));
#276623=CARTESIAN_POINT('Ctrl Pts',(-34.5645438127007,-1.58493392176466,
136.807138498572));
#276624=CARTESIAN_POINT('Ctrl Pts',(-34.8429914365135,4.19361153991761,
135.382458484293));
#276625=CARTESIAN_POINT('Ctrl Pts',(-35.1214390603265,6.11843286572883,
129.750730183006));
#276626=CARTESIAN_POINT('Ctrl Pts',(-35.3998866841394,2.42071328999757,
125.087236778371));
#276627=CARTESIAN_POINT('Ctrl Pts',(-35.6783343079523,-3.50152354082281,
125.677500884929));
#276628=CARTESIAN_POINT('Ctrl Pts',(-35.9567819317651,-6.20603129656164,
130.979098624759));
#276629=CARTESIAN_POINT('Ctrl Pts',(-36.2352295555781,-3.2074994722443,
136.120120672404));
#276630=CARTESIAN_POINT('Ctrl Pts',(-36.5136771793909,2.73856767200523,
136.376218918968));
#276631=CARTESIAN_POINT('Ctrl Pts',(-36.7921248032039,6.1680249121504,131.512051586954));
#276632=CARTESIAN_POINT('Ctrl Pts',(-37.0705724270167,3.92936858279784,
125.997550826698));
#276633=CARTESIAN_POINT('Ctrl Pts',(-37.3490200508296,-1.92018551381882,
124.900273438536));
#276634=CARTESIAN_POINT('Ctrl Pts',(-37.6274676746425,-6.00518292951342,
129.228563737208));
#276635=CARTESIAN_POINT('Ctrl Pts',(-37.9059152984554,-4.57171060248077,
135.004934386972));
#276636=CARTESIAN_POINT('Ctrl Pts',(-38.1843629222683,1.0629404277527,136.921182952087));
#276637=CARTESIAN_POINT('Ctrl Pts',(-38.4628105460811,5.72080113240803,
133.216370615161));
#276638=CARTESIAN_POINT('Ctrl Pts',(-38.7412581698941,5.12152507305273,
127.295038923683));
#276639=CARTESIAN_POINT('Ctrl Pts',(-39.0197057937069,-0.184182328028525,
124.598602428988));
#276640=CARTESIAN_POINT('Ctrl Pts',(-39.2981534175199,-5.32063516745863,
127.604954541453));
#276641=CARTESIAN_POINT('Ctrl Pts',(-39.5766010413327,-5.56768421547239,
133.55140453819));
#276642=CARTESIAN_POINT('Ctrl Pts',(-39.8550486651457,-0.698303465962086,
136.973455372429));
#276643=CARTESIAN_POINT('Ctrl Pts',(-40.1334962889585,4.81278405474664,
134.726409503982));
#276644=CARTESIAN_POINT('Ctrl Pts',(-40.4119439127715,5.90115814671511,
128.875192311658));
#276645=CARTESIAN_POINT('Ctrl Pts',(-40.6903915365843,1.56665618945481,
124.796786547352));
#276646=CARTESIAN_POINT('Ctrl Pts',(-40.9688391603973,-4.20752627050468,
126.239047867263));
#276647=CARTESIAN_POINT('Ctrl Pts',(-41.2472867842101,-6.11519763695597,
131.876608576776));
#276648=CARTESIAN_POINT('Ctrl Pts',(-41.5257344080229,-2.40330111905734,
136.528825793999));
#276649=CARTESIAN_POINT('Ctrl Pts',(-41.8041820318359,3.51711171946819,
135.920539169751));
#276650=CARTESIAN_POINT('Ctrl Pts',(-42.0826296556488,6.20547070826194,
130.610734395262));
#276651=CARTESIAN_POINT('Ctrl Pts',(-42.3610772794617,3.19130527026066,
125.478862659902));
#276652=CARTESIAN_POINT('Ctrl Pts',(-42.6395249032745,-2.75551380718057,
125.240863382598));
#276653=CARTESIAN_POINT('Ctrl Pts',(-42.9179725270875,-6.17015031015604,
130.115446272278));
#276654=CARTESIAN_POINT('Ctrl Pts',(-43.1964201509003,-3.91472010669807,
135.623107789941));
#276655=CARTESIAN_POINT('Ctrl Pts',(-43.4748677747133,1.93814663010615,
136.702576065077));
#276656=CARTESIAN_POINT('Ctrl Pts',(-43.7533153985261,6.00995129756958,
132.361872487794));
#276657=CARTESIAN_POINT('Ctrl Pts',(-44.031763022339,4.55890432500984,126.589891590455));
#276658=CARTESIAN_POINT('Ctrl Pts',(-44.3102106461518,-1.08155300737633,
124.690801840773));
#276659=CARTESIAN_POINT('Ctrl Pts',(-44.5886582699649,-5.72811596278534,
128.409773943013));
#276660=CARTESIAN_POINT('Ctrl Pts',(-44.8671058937777,-5.11082018241628,
134.329254217104));
#276661=CARTESIAN_POINT('Ctrl Pts',(-45.1455535175906,0.2030696681468,137.009529473845));
#276662=CARTESIAN_POINT('Ctrl Pts',(-45.4240011414034,5.33034841418793,
133.987557691017));
#276663=CARTESIAN_POINT('Ctrl Pts',(-45.7024487652165,5.55929736958694,
128.040383305508));
#276664=CARTESIAN_POINT('Ctrl Pts',(-45.9808963890292,0.679523629110432,
124.633169041983));
#276665=CARTESIAN_POINT('Ctrl Pts',(-46.2593440128422,-4.82469912994364,
126.896978356949));
#276666=CARTESIAN_POINT('Ctrl Pts',(-46.537791636655,-5.89525908823553,
132.751481083186));
#276667=CARTESIAN_POINT('Ctrl Pts',(-46.816239260468,-1.54836394385628,
136.816675223641));
#276668=CARTESIAN_POINT('Ctrl Pts',(-47.0946868842807,4.22140202314317,
135.35684595901));
#276669=CARTESIAN_POINT('Ctrl Pts',(-47.3731345080937,6.11190575782758,
129.713505066864));
#276670=CARTESIAN_POINT('Ctrl Pts',(-47.6515821319066,2.38586668426401,
125.072607134557));
#276671=CARTESIAN_POINT('Ctrl Pts',(-47.9300297557195,-3.53266731607082,
125.69891064141));
#276672=CARTESIAN_POINT('Ctrl Pts',(-48.2084773795324,-6.20485263332943,
131.016873261253));
#276673=CARTESIAN_POINT('Ctrl Pts',(-48.4869250033452,-3.17508150446096,
136.139547143367));
#276674=CARTESIAN_POINT('Ctrl Pts',(-48.7653726271582,2.77243441565242,
136.359445246621));
#276675=CARTESIAN_POINT('Ctrl Pts',(-49.043820250971,6.1722185487321,131.474491956744));
#276676=CARTESIAN_POINT('Ctrl Pts',(-49.322267874784,3.900035365166,125.973720703898));
#276677=CARTESIAN_POINT('Ctrl Pts',(-49.6007154985968,-1.95608979166789,
124.912071541833));
#276678=CARTESIAN_POINT('Ctrl Pts',(-49.8791631224098,-6.0146639902579,
129.265148186042));
#276679=CARTESIAN_POINT('Ctrl Pts',(-50.1576107462225,-4.54605581447205,
135.032685860113));
#276680=CARTESIAN_POINT('Ctrl Pts',(-50.4360583700356,1.10015556764067,
136.914599201455));
#276681=CARTESIAN_POINT('Ctrl Pts',(-50.7145059938484,5.73537772867887,
133.181501785951));
#276682=CARTESIAN_POINT('Ctrl Pts',(-50.9929536176612,5.10006794583985,
127.263927766504));
#276683=CARTESIAN_POINT('Ctrl Pts',(-51.2714012414742,-0.221955127055423,
124.599838577421));
#276684=CARTESIAN_POINT('Ctrl Pts',(-51.5498488652871,-5.34001228129766,
127.637402035479));
#276685=CARTESIAN_POINT('Ctrl Pts',(-51.8282964891,-5.5508590231301,133.585245715947));
#276686=CARTESIAN_POINT('Ctrl Pts',(-52.1067441129128,-0.660737497244709,
136.977591844792));
#276687=CARTESIAN_POINT('Ctrl Pts',(-52.3851917367258,4.8365695097872,134.697040054928));
#276688=CARTESIAN_POINT('Ctrl Pts',(-52.6636393605386,5.889305416881,128.83930603009));
#276689=CARTESIAN_POINT('Ctrl Pts',(-52.9420869843516,1.53005735442545,
124.78736117289));
#276690=CARTESIAN_POINT('Ctrl Pts',(-53.2205346081644,-4.23523866929,126.264744858582));
#276691=CARTESIAN_POINT('Ctrl Pts',(-53.4989822319774,-6.1085572588392,
131.913813654221));
#276692=CARTESIAN_POINT('Ctrl Pts',(-53.7774298557902,-2.36841014712749,
136.543349308967));
#276693=CARTESIAN_POINT('Ctrl Pts',(-54.0558774796031,3.54819018652628,
135.8990347215));
#276694=CARTESIAN_POINT('Ctrl Pts',(-54.334325103416,6.20417707748961,130.572963521183));
#276695=CARTESIAN_POINT('Ctrl Pts',(-54.6127727272289,3.15882832513996,
125.459534948064));
#276696=CARTESIAN_POINT('Ctrl Pts',(-54.8912203510417,-2.7893293406706,
125.257740055968));
#276697=CARTESIAN_POINT('Ctrl Pts',(-55.1696679748547,-6.17422960871856,
130.153018492501));
#276698=CARTESIAN_POINT('Ctrl Pts',(-55.4481155986676,-3.88531449423931,
135.646848522136));
#276699=CARTESIAN_POINT('Ctrl Pts',(-55.7265632224805,1.97401483228084,
136.690668736158));
#276700=CARTESIAN_POINT('Ctrl Pts',(-56.0050108462934,6.01932096392068,
132.32525935133));
#276701=CARTESIAN_POINT('Ctrl Pts',(-56.2834584701062,4.53316518989421,
126.562218330207));
#276702=CARTESIAN_POINT('Ctrl Pts',(-56.5619060939192,-1.11874793621411,
124.697498830995));
#276703=CARTESIAN_POINT('Ctrl Pts',(-56.840353717732,-5.74258636281662,
128.444686976857));
#276704=CARTESIAN_POINT('Ctrl Pts',(-57.118801341545,-5.08926846293066,
134.360299922064));
#276705=CARTESIAN_POINT('Ctrl Pts',(-57.3972489653578,0.240838529802063,
137.00817836373));
#276706=CARTESIAN_POINT('Ctrl Pts',(-57.6756965891708,5.34962667926312,
133.955051370017));
#276707=CARTESIAN_POINT('Ctrl Pts',(-57.9541442129836,5.54236925427356,
128.0065934946));
#276708=CARTESIAN_POINT('Ctrl Pts',(-58.2325918367966,0.641945244397073,
124.629146926667));
#276709=CARTESIAN_POINT('Ctrl Pts',(-58.5110394606094,-4.84839508431156,
126.92642006471));
#276710=CARTESIAN_POINT('Ctrl Pts',(-58.7894870844223,-5.88329718780563,
132.787331122898));
#276711=CARTESIAN_POINT('Ctrl Pts',(-59.0679347082352,-1.5117365907523,
136.825989160181));
#276712=CARTESIAN_POINT('Ctrl Pts',(-59.3463823320481,4.24903608076433,
135.331064739709));
#276713=CARTESIAN_POINT('Ctrl Pts',(-59.624829955861,6.10515217101086,129.676320372777));
#276714=CARTESIAN_POINT('Ctrl Pts',(-59.9032775796738,2.3509316693629,125.058189882977));
#276715=CARTESIAN_POINT('Ctrl Pts',(-60.1817252034868,-3.56368018703254,
125.720509582217));
#276716=CARTESIAN_POINT('Ctrl Pts',(-60.4601728272995,-6.20344404700091,
131.054640023013));
#276717=CARTESIAN_POINT('Ctrl Pts',(-60.7386204511126,-3.14254588286485,
136.158775917031));
#276718=CARTESIAN_POINT('Ctrl Pts',(-61.0170680749254,2.80619842572279,
136.342465728569));
#276719=CARTESIAN_POINT('Ctrl Pts',(-61.2955156987383,6.17618347148551,
131.436907494571));
#276720=CARTESIAN_POINT('Ctrl Pts',(-61.5739633225512,3.87055763028967,
125.950069582238));
#276721=CARTESIAN_POINT('Ctrl Pts',(-61.8524109463641,-1.9919215858902,
124.924087986069));
#276722=CARTESIAN_POINT('Ctrl Pts',(-62.130858570177,-6.02392217541635,
129.301789670958));
#276723=CARTESIAN_POINT('Ctrl Pts',(-62.4093061939898,-4.5202325706933,
135.060280651108));
#276724=CARTESIAN_POINT('Ctrl Pts',(-62.6877538178028,1.13732994085927,
136.907789033684));
#276725=CARTESIAN_POINT('Ctrl Pts',(-62.9662014416156,5.74974179841868,
133.146544870902));
#276726=CARTESIAN_POINT('Ctrl Pts',(-63.2446490654287,5.0784218337339,127.232947801366));
#276727=CARTESIAN_POINT('Ctrl Pts',(-63.5230966892413,-0.25971970145348,
124.601304636701));
#276728=CARTESIAN_POINT('Ctrl Pts',(-63.8015443130544,-5.3591915190178,
127.669966882319));
#276729=CARTESIAN_POINT('Ctrl Pts',(-64.0799919368672,-5.53382814166538,
133.618983846983));
#276730=CARTESIAN_POINT('Ctrl Pts',(-64.3584395606801,-0.623147044656387,
136.9814995658));
#276731=CARTESIAN_POINT('Ctrl Pts',(-64.636887184493,4.86017574396616,134.667526361205));
#276732=CARTESIAN_POINT('Ctrl Pts',(-64.9153348083059,5.8772344566688,128.803492564343));
#276733=CARTESIAN_POINT('Ctrl Pts',(-65.1937824321189,1.4934018225579,124.778158760555));
#276734=CARTESIAN_POINT('Ctrl Pts',(-65.4722300559316,-4.26279412974889,
126.290610067033));
#276735=CARTESIAN_POINT('Ctrl Pts',(-65.7506776797446,-6.10169052588679,
131.950977620477));
#276736=CARTESIAN_POINT('Ctrl Pts',(-66.0291253035574,-2.33343141288849,
136.5576601636));
#276737=CARTESIAN_POINT('Ctrl Pts',(-66.3075729273703,3.57913717409239,
135.877341488227));
#276738=CARTESIAN_POINT('Ctrl Pts',(-66.5860205511832,6.20265354865397,
130.535201221608));
#276739=CARTESIAN_POINT('Ctrl Pts',(-66.8644681749961,3.126234328474,125.440405290707));
#276740=CARTESIAN_POINT('Ctrl Pts',(-67.142915798809,-2.82304151453613,
125.274822261403));
#276741=CARTESIAN_POINT('Ctrl Pts',(-67.421363422622,-6.17808011893247,
130.190614848446));
#276742=CARTESIAN_POINT('Ctrl Pts',(-67.6998110464348,-3.85576491002292,
135.670409814162));
#276743=CARTESIAN_POINT('Ctrl Pts',(-67.9782586702478,2.00980988661012,
136.678543287925));
#276744=CARTESIAN_POINT('Ctrl Pts',(-68.2567062940606,6.02846758211988,
132.288589857404));
#276745=CARTESIAN_POINT('Ctrl Pts',(-68.5351539178734,4.50725807667536,
126.534702264101));
#276746=CARTESIAN_POINT('Ctrl Pts',(-68.8136015416864,-1.15590140943545,
124.704422113226));
#276747=CARTESIAN_POINT('Ctrl Pts',(-69.0920491654993,-5.75684396919829,
128.479687449276));
#276748=CARTESIAN_POINT('Ctrl Pts',(-69.3704967893121,-5.0675281587308,
134.391213860386));
#276749=CARTESIAN_POINT('Ctrl Pts',(-69.648944413125,0.278598467097045,
137.006597368867));
#276750=CARTESIAN_POINT('Ctrl Pts',(-69.9273920369379,5.36870671195437,
133.922428299012));
#276751=CARTESIAN_POINT('Ctrl Pts',(-70.2058396607509,5.52523576442926,
127.972907355982));
#276752=CARTESIAN_POINT('Ctrl Pts',(-70.4842872845636,0.604343072166899,
124.625353636165));
#276753=CARTESIAN_POINT('Ctrl Pts',(-70.7627349083767,-4.87191137961658,
126.956005470983));
#276754=CARTESIAN_POINT('Ctrl Pts',(-71.0411825321895,-5.87111727963483,
132.823107682909));
#276755=CARTESIAN_POINT('Ctrl Pts',(-71.3196301560023,-1.47505321969301,
136.835079963061));
#276756=CARTESIAN_POINT('Ctrl Pts',(-71.5980777798154,4.27651268879093,
135.305115781721));
#276757=CARTESIAN_POINT('Ctrl Pts',(-71.8765254036282,6.09817235553532,
129.639177478635));
#276758=CARTESIAN_POINT('Ctrl Pts',(-72.1549730274411,2.31590953982396,
125.043985557866));
#276759=CARTESIAN_POINT('Ctrl Pts',(-72.433420651254,-3.5945610045145,125.742296906994));
#276760=CARTESIAN_POINT('Ctrl Pts',(-72.7118682750669,-6.20180558977201,
131.092397510578));
#276761=CARTESIAN_POINT('Ctrl Pts',(-72.9903158988798,-3.109893813075,136.177806280867));
#276762=CARTESIAN_POINT('Ctrl Pts',(-73.2687635226926,2.8398584510789,136.325280993997));
#276763=CARTESIAN_POINT('Ctrl Pts',(-73.5472111465057,6.17991953348924,
131.399299593141));
#276764=CARTESIAN_POINT('Ctrl Pts',(-73.8256587703184,3.84093647047644,
125.926598338115));
#276765=CARTESIAN_POINT('Ctrl Pts',(-74.1041063941314,-2.02767956872624,
124.93632232597));
#276766=CARTESIAN_POINT('Ctrl Pts',(-74.3825540179442,-6.0329571419232,
129.338486834193));
#276767=CARTESIAN_POINT('Ctrl Pts',(-74.6610016417573,-4.49424182803428,
135.08771773742));
#276768=CARTESIAN_POINT('Ctrl Pts',(-74.9394492655699,1.17446216989917,
136.900752701129));
#276769=CARTESIAN_POINT('Ctrl Pts',(-75.217896889383,5.76389280936176,133.111501165354));
#276770=CARTESIAN_POINT('Ctrl Pts',(-75.4963445131958,5.05658753883907,
127.202100176243));
#276771=CARTESIAN_POINT('Ctrl Pts',(-75.7747921370087,-0.297474651842549,
124.603000552501));
#276772=CARTESIAN_POINT('Ctrl Pts',(-76.0532397608216,-5.37817216992523,
127.702647875272));
#276773=CARTESIAN_POINT('Ctrl Pts',(-76.3316873846344,-5.51659220216403,
133.65261768112));
#276774=CARTESIAN_POINT('Ctrl Pts',(-76.6101350084474,-0.585533501125347,
136.985178390654));
#276775=CARTESIAN_POINT('Ctrl Pts',(-76.8885826322602,4.8836018825454,134.637869516455));
#276776=CARTESIAN_POINT('Ctrl Pts',(-77.1670302560731,5.86494571337264,
128.767753241497));
#276777=CARTESIAN_POINT('Ctrl Pts',(-77.4454778798861,1.4566909521364,124.769179651345));
#276778=CARTESIAN_POINT('Ctrl Pts',(-77.7239255036988,-4.29019163080361,
126.316642534169));
#276779=CARTESIAN_POINT('Ctrl Pts',(-78.0023731275119,-6.09459769254796,
131.988099098418));
#276780=CARTESIAN_POINT('Ctrl Pts',(-78.2808207513247,-2.29836621249045,
136.571757827603));
#276781=CARTESIAN_POINT('Ctrl Pts',(-78.5592683751376,3.60995153541429,
135.855460273781));
#276782=CARTESIAN_POINT('Ctrl Pts',(-78.8377159989505,6.20090017820995,
130.497448895834));
#276783=CARTESIAN_POINT('Ctrl Pts',(-79.1161636227633,3.09352448804556,
125.421474396687));
#276784=CARTESIAN_POINT('Ctrl Pts',(-79.3946112465763,-2.85664907955992,
125.292109365916));
#276785=CARTESIAN_POINT('Ctrl Pts',(-79.6730588703891,-6.18170169811556,
130.228233946967));
#276786=CARTESIAN_POINT('Ctrl Pts',(-79.9515064942021,-3.8260724490201,
135.693790792945));
#276787=CARTESIAN_POINT('Ctrl Pts',(-80.2299541180149,2.04553046669522,
136.666200169693));
#276788=CARTESIAN_POINT('Ctrl Pts',(-80.5084017418279,6.03739081323573,
132.251865364817));
#276789=CARTESIAN_POINT('Ctrl Pts',(-80.7868493656406,4.48118394535095,
126.507344411756));
#276790=CARTESIAN_POINT('Ctrl Pts',(-81.0652969894537,-1.19301205030527,
124.711571430921));
#276791=CARTESIAN_POINT('Ctrl Pts',(-81.3437446132665,-5.77088825360962,
128.514774063314));
#276792=CARTESIAN_POINT('Ctrl Pts',(-81.6221922370794,-5.04560007541116,
134.421994886542));
#276793=CARTESIAN_POINT('Ctrl Pts',(-81.9006398608923,0.316348080823153,
137.00478654784));
#276794=CARTESIAN_POINT('Ctrl Pts',(-82.179087484705,5.38758780524389,133.889689686862));
#276795=CARTESIAN_POINT('Ctrl Pts',(-82.4575351085182,5.50789753494193,
127.939326137905));
#276796=CARTESIAN_POINT('Ctrl Pts',(-82.7359827323308,0.566718505781886,
124.621789311041));
#276797=CARTESIAN_POINT('Ctrl Pts',(-83.0144303561439,-4.89524714445407,
126.985733479472));
#276798=CARTESIAN_POINT('Ctrl Pts',(-83.2928779799568,-5.858719815054,132.858809437506));
#276799=CARTESIAN_POINT('Ctrl Pts',(-83.5713256037696,-1.43831518999427,
136.843947295418));
#276800=CARTESIAN_POINT('Ctrl Pts',(-83.8497732275826,4.30383082906709,
135.279000046597));
#276801=CARTESIAN_POINT('Ctrl Pts',(-84.1282208513953,6.09096657004034,
129.602077760783));
#276802=CARTESIAN_POINT('Ctrl Pts',(-84.4066684752085,2.28080159340614,
125.029994685571));
#276803=CARTESIAN_POINT('Ctrl Pts',(-84.685116099021,-3.6253086242162,125.764271808403));
#276804=CARTESIAN_POINT('Ctrl Pts',(-84.9635637228342,-6.19993732235617,
131.130144324829));
#276805=CARTESIAN_POINT('Ctrl Pts',(-85.242011346647,-3.07712650502686,
136.196637529698));
#276806=CARTESIAN_POINT('Ctrl Pts',(-85.5204589704598,2.87341324443482,
136.307891679689));
#276807=CARTESIAN_POINT('Ctrl Pts',(-85.7989065942728,6.18342659630218,
131.361669646028));
#276808=CARTESIAN_POINT('Ctrl Pts',(-86.0773542180856,3.81117298335027,
125.903307841269));
#276809=CARTESIAN_POINT('Ctrl Pts',(-86.3558018418987,-2.06336241514917,
124.948774108188));
#276810=CARTESIAN_POINT('Ctrl Pts',(-86.6342494657113,-6.04176855498474,
129.375238315919));
#276811=CARTESIAN_POINT('Ctrl Pts',(-86.9126970895244,-4.46808454959173,
135.114996102359));
#276812=CARTESIAN_POINT('Ctrl Pts',(-87.1911447133372,1.2115508788106,136.893490464523));
#276813=CARTESIAN_POINT('Ctrl Pts',(-87.4695923371502,5.77783023713722,
133.076371967865));
#276814=CARTESIAN_POINT('Ctrl Pts',(-87.7480399609628,5.03456587023344,
127.171386034204));
#276815=CARTESIAN_POINT('Ctrl Pts',(-88.026487584776,-0.33521857919891,
124.60492626198));
#276816=CARTESIAN_POINT('Ctrl Pts',(-88.3049352085887,-5.39695353068522,
127.735443803332));
#276817=CARTESIAN_POINT('Ctrl Pts',(-88.5833828324018,-5.49915184330967,
133.686145972045));
#276818=CARTESIAN_POINT('Ctrl Pts',(-88.8618304562145,-0.547898260434929,
136.988628183031));
#276819=CARTESIAN_POINT('Ctrl Pts',(-89.1402780800275,4.90684705746115,
134.608070619623));
#276820=CARTESIAN_POINT('Ctrl Pts',(-89.4187257038403,5.85243964235601,
128.732089385887));
#276821=CARTESIAN_POINT('Ctrl Pts',(-89.6971733276532,1.41992610349655,
124.760424177987));
#276822=CARTESIAN_POINT('Ctrl Pts',(-89.9756209514662,-4.31743015722937,
126.342841295349));
#276823=CARTESIAN_POINT('Ctrl Pts',(-90.254068575279,-6.08727902165076,
132.025176712493));
#276824=CARTESIAN_POINT('Ctrl Pts',(-90.5325161990919,-2.26321584528708,
136.585641778581));
#276825=CARTESIAN_POINT('Ctrl Pts',(-90.8109638229048,3.64063212865448,
135.833391888981));
#276826=CARTESIAN_POINT('Ctrl Pts',(-91.0894114467178,6.19891703112955,
130.459707942787));
#276827=CARTESIAN_POINT('Ctrl Pts',(-91.3678590705306,3.06070001592934,
125.402742967496));
#276828=CARTESIAN_POINT('Ctrl Pts',(-91.6463066943433,-2.89015079040179,
125.309600728926));
#276829=CARTESIAN_POINT('Ctrl Pts',(-91.9247543181566,-6.18509421206894,
130.265874394073));
#276830=CARTESIAN_POINT('Ctrl Pts',(-92.2032019419691,-3.79623821149537,
135.716990592095));
#276831=CARTESIAN_POINT('Ctrl Pts',(-92.4816495657822,2.08117524889636,
136.653639838841));
#276832=CARTESIAN_POINT('Ctrl Pts',(-92.7600971895951,6.04609032661485,
132.21508723441));
#276833=CARTESIAN_POINT('Ctrl Pts',(-93.0385448134079,4.45494376210749,
126.480145786926));
#276834=CARTESIAN_POINT('Ctrl Pts',(-93.3169924372209,-1.23007848367479,
124.718946519161));
#276835=CARTESIAN_POINT('Ctrl Pts',(-93.5954400610337,-5.78471869563455,
128.549945518824));
#276836=CARTESIAN_POINT('Ctrl Pts',(-93.8738876848466,-5.02348502552524,
134.45264185993));
#276837=CARTESIAN_POINT('Ctrl Pts',(-94.1523353086595,0.354085972155003,
137.002745967751));
#276838=CARTESIAN_POINT('Ctrl Pts',(-94.4307829324724,5.40626925948619,
133.85683674671));
#276839=CARTESIAN_POINT('Ctrl Pts',(-94.7092305562852,5.49035520828578,
127.905851084735));
#276840=CARTESIAN_POINT('Ctrl Pts',(-94.9876781800983,0.529072939433998,
124.618454083368));
#276841=CARTESIAN_POINT('Ctrl Pts',(-95.2661258039109,-4.91840151410816,
127.015602988595));
#276842=CARTESIAN_POINT('Ctrl Pts',(-95.5445734277241,-5.84610525345601,
132.894435063746));
#276843=CARTESIAN_POINT('Ctrl Pts',(-95.8230210515366,-1.40152386299717,
136.85259082867));
#276844=CARTESIAN_POINT('Ctrl Pts',(-96.10146867535,4.33098948930923,135.252718502061));
#276845=CARTESIAN_POINT('Ctrl Pts',(-96.3799162991623,6.08353508153927,
129.565022593965));
#276846=CARTESIAN_POINT('Ctrl Pts',(-96.6583639229758,2.245609131046,125.01621778453));
#276847=CARTESIAN_POINT('Ctrl Pts',(-96.9368115467883,-3.65592190677386,
125.786433472156));
#276848=CARTESIAN_POINT('Ctrl Pts',(-97.2152591706015,-6.19783931398261,
131.167879067045));
#276849=CARTESIAN_POINT('Ctrl Pts',(-97.493706794414,-3.04424517292474,
136.215268965725));
#276850=CARTESIAN_POINT('Ctrl Pts',(-97.7721544182274,2.90686156240656,
136.290298430015));
#276851=CARTESIAN_POINT('Ctrl Pts',(-98.0506020420397,6.18670452996842,
131.324019047625));
#276852=CARTESIAN_POINT('Ctrl Pts',(-98.3290496658531,3.78126827180747,
125.880198954735));
#276853=CARTESIAN_POINT('Ctrl Pts',(-98.6074972896656,-2.09896880291958,
124.961442871316));
#276854=CARTESIAN_POINT('Ctrl Pts',(-98.8859449134787,-6.05035608809047,
129.412042754299));
#276855=CARTESIAN_POINT('Ctrl Pts',(-99.1643925372916,-4.44176170463296,
135.142114735114));
#276856=CARTESIAN_POINT('Ctrl Pts',(-99.4428401611044,1.24859469325925,
136.886002592972));
#276857=CARTESIAN_POINT('Ctrl Pts',(-99.7212877849174,5.79155356528836,
133.041158580159));
#276858=CARTESIAN_POINT('Ctrl Pts',(-99.9997354087301,5.01235764393804,
127.140806513377));
#276859=CARTESIAN_POINT('Ctrl Pts',(-100.278183032543,-0.37295008490757,
124.607081693777));
#276860=CARTESIAN_POINT('Ctrl Pts',(-100.556630656356,-5.41553490534739,
127.768353451233));
#276861=CARTESIAN_POINT('Ctrl Pts',(-100.835078280169,-5.48150771136145,
133.719567477352));
#276862=CARTESIAN_POINT('Ctrl Pts',(-101.113525903981,-0.510242717172956,
136.9918488151));
#276863=CARTESIAN_POINT('Ctrl Pts',(-101.391973527794,4.92991040735466,
134.578130774917));
#276864=CARTESIAN_POINT('Ctrl Pts',(-101.670421151607,5.83971670703623,
128.696502319049));
#276865=CARTESIAN_POINT('Ctrl Pts',(-101.94886877542,1.38310863897239,124.751892664915));
#276866=CARTESIAN_POINT('Ctrl Pts',(-102.227316399233,-4.34450869969331,
126.36920537977));
#276867=CARTESIAN_POINT('Ctrl Pts',(-102.505764023046,-6.07973478439049,
132.062209088779));
#276868=CARTESIAN_POINT('Ctrl Pts',(-102.784211646859,-2.22798161378826,
136.599311502058));
#276869=CARTESIAN_POINT('Ctrl Pts',(-103.062659270672,3.6711778169323,135.811137151577));
#276870=CARTESIAN_POINT('Ctrl Pts',(-103.341106894485,6.19670418089893,
130.42197976097));
#276871=CARTESIAN_POINT('Ctrl Pts',(-103.619554518298,3.02776212844844,
125.384211697232));
#276872=CARTESIAN_POINT('Ctrl Pts',(-103.89800214211,-2.92354540564323,
125.327295702285));
#276873=CARTESIAN_POINT('Ctrl Pts',(-104.176449765923,-6.18825753508174,
130.303534794984));
#276874=CARTESIAN_POINT('Ctrl Pts',(-104.454897389736,-3.76626330296762,
135.740008351935));
#276875=CARTESIAN_POINT('Ctrl Pts',(-104.733345013549,2.1167429123828,136.640862760796));
#276876=CARTESIAN_POINT('Ctrl Pts',(-105.011792637362,6.05456579989334,
132.17825682901));
#276877=CARTESIAN_POINT('Ctrl Pts',(-105.290240261175,4.42853849928509,
126.453107397468));
#276878=CARTESIAN_POINT('Ctrl Pts',(-105.568687884988,-1.26709933603374,
124.726547104658));
#276879=CARTESIAN_POINT('Ctrl Pts',(-105.847135508801,-5.79833478278087,
128.585200512514));
#276880=CARTESIAN_POINT('Ctrl Pts',(-106.125583132613,-5.00118382855433,
134.483153644914));
#276881=CARTESIAN_POINT('Ctrl Pts',(-106.404030756427,0.391810742700936,
137.000475704212));
#276882=CARTESIAN_POINT('Ctrl Pts',(-106.682478380239,5.42475038243292,
133.823870695931));
#276883=CARTESIAN_POINT('Ctrl Pts',(-106.960926004052,5.47260943449832,
127.872483436902));
#276884=CARTESIAN_POINT('Ctrl Pts',(-107.239373627865,0.491407768093767,
124.615348076738));
#276885=CARTESIAN_POINT('Ctrl Pts',(-107.517821251678,-4.94137363058539,
127.045612891524));
#276886=CARTESIAN_POINT('Ctrl Pts',(-107.796268875491,-5.83327406227795,
132.929983241508));
#276887=CARTESIAN_POINT('Ctrl Pts',(-108.074716499304,-1.36468060201792,
136.861010242526));
#276888=CARTESIAN_POINT('Ctrl Pts',(-108.353164123117,4.3579876631431,135.22627212199));
#276889=CARTESIAN_POINT('Ctrl Pts',(-108.631611746929,6.07587816540856,
129.528013351273));
#276890=CARTESIAN_POINT('Ctrl Pts',(-108.910059370743,2.21033345681367,
125.00265536525));
#276891=CARTESIAN_POINT('Ctrl Pts',(-109.188506994555,-3.68639971780079,
125.808781077045));
#276892=CARTESIAN_POINT('Ctrl Pts',(-109.466954618368,-6.19551164239422,
131.205600338952));
#276893=CARTESIAN_POINT('Ctrl Pts',(-109.745402242181,-3.01125103519769,
136.233699898554));
#276894=CARTESIAN_POINT('Ctrl Pts',(-110.023849865994,2.94020216555433,
136.272501896897));
#276895=CARTESIAN_POINT('Ctrl Pts',(-110.302297489807,6.18975321302316,
131.286349193086));
#276896=CARTESIAN_POINT('Ctrl Pts',(-110.58074511362,3.75122344397827,125.857272534824));
#276897=CARTESIAN_POINT('Ctrl Pts',(-110.859192737433,-2.13449741262907,
124.974328145912));
#276898=CARTESIAN_POINT('Ctrl Pts',(-111.137640361246,-6.05871942302636,
129.44889878553));
#276899=CARTESIAN_POINT('Ctrl Pts',(-111.416087985058,-4.41527426856075,
135.169072630797));
#276900=CARTESIAN_POINT('Ctrl Pts',(-111.694535608871,1.28559224057236,
136.878289363941));
#276901=CARTESIAN_POINT('Ctrl Pts',(-111.972983232684,5.8050622852923,133.005862307081));
#276902=CARTESIAN_POINT('Ctrl Pts',(-112.251430856497,4.9899636828869,127.110362746893));
#276903=CARTESIAN_POINT('Ctrl Pts',(-112.52987848031,-0.410667770813077,
124.609466768025));
#276904=CARTESIAN_POINT('Ctrl Pts',(-112.808326104123,-5.43391560537209,
127.801375599495));
#276905=CARTESIAN_POINT('Ctrl Pts',(-113.086773727936,-5.46366046012913,
133.752880958598));
#276906=CARTESIAN_POINT('Ctrl Pts',(-113.365221351749,-0.472568266679477,
136.994840167519));
#276907=CARTESIAN_POINT('Ctrl Pts',(-113.643668975562,4.95279107760506,
134.548051091771));
#276908=CARTESIAN_POINT('Ctrl Pts',(-113.922116599375,5.8267773788663,128.660993359675));
#276909=CARTESIAN_POINT('Ctrl Pts',(-114.200564223187,1.34623992284899,
124.74358542827));
#276910=CARTESIAN_POINT('Ctrl Pts',(-114.479011847001,-4.37142625478972,
126.395733810498));
#276911=CARTESIAN_POINT('Ctrl Pts',(-114.757459470813,-6.07196526032194,
132.099194855029));
#276912=CARTESIAN_POINT('Ctrl Pts',(-115.035907094626,-2.19266482361144,
136.612766491501));
#276913=CARTESIAN_POINT('Ctrl Pts',(-115.314354718439,3.70158746836604,
135.788696886227));
#276914=CARTESIAN_POINT('Ctrl Pts',(-115.592802342252,6.19426170951602,
130.384265748418));
#276915=CARTESIAN_POINT('Ctrl Pts',(-115.871249966065,2.99471204612843,
125.36588127258));
#276916=CARTESIAN_POINT('Ctrl Pts',(-116.149697589878,-2.95683168783455,
125.345193630298));
#276917=CARTESIAN_POINT('Ctrl Pts',(-116.428145213691,-6.19119154993583,
130.34121375418));
#276918=CARTESIAN_POINT('Ctrl Pts',(-116.706592837503,-3.73614883416816,
135.762843219532));
#276919=CARTESIAN_POINT('Ctrl Pts',(-116.985040461316,2.1522321391827,136.627869409019));
#276920=CARTESIAN_POINT('Ctrl Pts',(-117.263488085129,6.06281691900968,
132.14137551338));
#276921=CARTESIAN_POINT('Ctrl Pts',(-117.541935708942,4.40196913533955,
126.426230245297));
#276922=CARTESIAN_POINT('Ctrl Pts',(-117.820383332755,-1.30407323556081,
124.73437290577));
#276923=CARTESIAN_POINT('Ctrl Pts',(-118.098830956568,-5.81173601049948,
128.620537737998));
#276924=CARTESIAN_POINT('Ctrl Pts',(-118.377278580381,-4.97869731087745,
134.51352911087));
#276925=CARTESIAN_POINT('Ctrl Pts',(-118.655726204194,0.429520994555717,
136.997975841351));
#276926=CARTESIAN_POINT('Ctrl Pts',(-118.934173828006,5.44303048925927,
133.790792756097));
#276927=CARTESIAN_POINT('Ctrl Pts',(-119.21262145182,5.45466087115571,127.839224430854));
#276928=CARTESIAN_POINT('Ctrl Pts',(-119.491069075632,0.453724387457947,
124.612471406243));
#276929=CARTESIAN_POINT('Ctrl Pts',(-119.769516699445,-4.96416264264509,
127.075762076232));
#276930=CARTESIAN_POINT('Ctrl Pts',(-120.047964323258,-5.82022671698453,
132.965452653541));
#276931=CARTESIAN_POINT('Ctrl Pts',(-120.326411947071,-1.32778677229758,
136.869205225004));
#276932=CARTESIAN_POINT('Ctrl Pts',(-120.604859570884,4.38482435014149,
135.199661886361));
#276933=CARTESIAN_POINT('Ctrl Pts',(-120.883307194697,6.06799610537801,
129.491051404098));
#276934=CARTESIAN_POINT('Ctrl Pts',(-121.16175481851,2.17497587786225,124.989307930291));
#276935=CARTESIAN_POINT('Ctrl Pts',(-121.440202442323,-3.71674092793051,
125.831313794972));
#276936=CARTESIAN_POINT('Ctrl Pts',(-121.718650066136,-6.19295439384353,
131.243306742772));
#276937=CARTESIAN_POINT('Ctrl Pts',(-121.997097689948,-2.97814531445616,
136.251929645219));
#276938=CARTESIAN_POINT('Ctrl Pts',(-122.275545313761,2.97343381842962,
136.254502739794));
#276939=CARTESIAN_POINT('Ctrl Pts',(-122.553992937574,6.19257253249627,
131.248661478285));
#276940=CARTESIAN_POINT('Ctrl Pts',(-122.832440561387,3.72103961318487,
125.83452943108));
#276941=CARTESIAN_POINT('Ctrl Pts',(-123.1108881852,-2.16994692775201,124.987429454503));
#276942=CARTESIAN_POINT('Ctrl Pts',(-123.389335809013,-6.06685824988591,
129.485805043896));
#276943=CARTESIAN_POINT('Ctrl Pts',(-123.667783432826,-4.38862322287681,
135.19586879047));
#276944=CARTESIAN_POINT('Ctrl Pts',(-123.946231056639,1.32254214979223,
136.870351063246));
#276945=CARTESIAN_POINT('Ctrl Pts',(-124.224678680451,5.81835589657845,
132.97048445655));
#276946=CARTESIAN_POINT('Ctrl Pts',(-124.503126304264,4.96738481689638,
127.080055862859));
#276947=CARTESIAN_POINT('Ctrl Pts',(-124.781573928077,-0.448370239273912,
124.612081396343));
#276948=CARTESIAN_POINT('Ctrl Pts',(-125.06002155189,-5.4520949496557,127.834509024472));
#276949=CARTESIAN_POINT('Ctrl Pts',(-125.338469175703,-5.44561075094924,
133.786085181339));
#276950=CARTESIAN_POINT('Ctrl Pts',(-125.616916799516,-0.434876304995071,
136.997602129441));
#276951=CARTESIAN_POINT('Ctrl Pts',(-125.895364423329,4.97548822036069,
134.517832684797));
#276952=CARTESIAN_POINT('Ctrl Pts',(-126.173812047142,5.8136221373178,128.625563823564));
#276953=CARTESIAN_POINT('Ctrl Pts',(-126.452259670955,1.30932132131015,
124.735502775877));
#276954=CARTESIAN_POINT('Ctrl Pts',(-126.730707294768,-4.39818182507867,
126.422425604514));
#276955=CARTESIAN_POINT('Ctrl Pts',(-127.00915491858,-6.0639707373477,132.136132640718));
#276956=CARTESIAN_POINT('Ctrl Pts',(-127.287602542393,-2.15726678343353,
136.626006248326));
#276957=CARTESIAN_POINT('Ctrl Pts',(-127.566050166206,3.73185995611441,
135.766071924465));
#276958=CARTESIAN_POINT('Ctrl Pts',(-127.844497790019,6.19158970748781,
130.346567302635));
#276959=CARTESIAN_POINT('Ctrl Pts',(-128.122945413832,2.96155099365221,
125.34775237278));
#276960=CARTESIAN_POINT('Ctrl Pts',(-128.401393037645,-2.99000840354028,
125.363293849751));
#276961=CARTESIAN_POINT('Ctrl Pts',(-128.679840661458,-6.19389614791022,
130.378909875453));
#276962=CARTESIAN_POINT('Ctrl Pts',(-128.958288285271,-3.70589592099968,
135.785494348734));
#276963=CARTESIAN_POINT('Ctrl Pts',(-129.236735909083,2.18764161422919,
136.614660264981));
#276964=CARTESIAN_POINT('Ctrl Pts',(-129.515183532897,6.07084337821547,
132.104444654172));
#276965=CARTESIAN_POINT('Ctrl Pts',(-129.793631156709,4.37523665480886,
126.399515326358));
#276966=CARTESIAN_POINT('Ctrl Pts',(-130.072078780522,-1.34099881217456,
124.742423632508));
#276967=CARTESIAN_POINT('Ctrl Pts',(-130.350526404335,-5.82492188220296,
128.655955885842));
#276968=CARTESIAN_POINT('Ctrl Pts',(-130.628974028148,-4.95602630574081,
134.543767132223));
#276969=CARTESIAN_POINT('Ctrl Pts',(-130.907421651961,0.467215330352083,
136.995246471799));
#276970=CARTESIAN_POINT('Ctrl Pts',(-131.185869275774,5.46110890258918,
133.757604152921));
#276971=CARTESIAN_POINT('Ctrl Pts',(-131.464316899587,5.43651018334856,
127.80607529902));
#276972=CARTESIAN_POINT('Ctrl Pts',(-131.742764523399,0.416024193898128,
124.60982417848));
#276973=CARTESIAN_POINT('Ctrl Pts',(-132.021212147213,-4.98676770583297,
127.106049425532));
#276974=CARTESIAN_POINT('Ctrl Pts',(-132.299659771025,-5.80696370104951,
133.000841985516));
#276975=CARTESIAN_POINT('Ctrl Pts',(-132.578107394838,-1.2908437409496,
136.877175472434));
#276976=CARTESIAN_POINT('Ctrl Pts',(-132.856555018651,4.41149855586104,
135.172888781227));
#276977=CARTESIAN_POINT('Ctrl Pts',(-133.135002642464,6.05988919352027,
129.454138122079));
#276978=CARTESIAN_POINT('Ctrl Pts',(-133.413450266277,2.13953770437982,
124.976175974248));
#276979=CARTESIAN_POINT('Ctrl Pts',(-133.69189789009,-3.74694441285829,
125.854030790976));
#276980=CARTESIAN_POINT('Ctrl Pts',(-133.970345513903,-6.19016766309031,
131.280996881284));
#276981=CARTESIAN_POINT('Ctrl Pts',(-134.248793137716,-2.94492923744478,
136.269957530209));
#276982=CARTESIAN_POINT('Ctrl Pts',(-134.527240761528,3.00655528962129,
136.236301625668));
#276983=CARTESIAN_POINT('Ctrl Pts',(-134.805688385342,6.19516238391663,
131.210957299752));
#276984=CARTESIAN_POINT('Ctrl Pts',(-135.084136009154,3.69071789790064,
125.811970486258));
#276985=CARTESIAN_POINT('Ctrl Pts',(-135.362583632967,-2.2053160346932,
125.000746311619));
#276986=CARTESIAN_POINT('Ctrl Pts',(-135.64103125678,-6.07477226708194,
129.522760161825));
#276987=CARTESIAN_POINT('Ctrl Pts',(-135.919478880593,-4.36180955514542,
135.222502221193));
#276988=CARTESIAN_POINT('Ctrl Pts',(-136.197926504406,1.35944305172635,
136.862187985044));
#276989=CARTESIAN_POINT('Ctrl Pts',(-136.476374128219,5.83143390654715,
132.935026339502));
#276990=CARTESIAN_POINT('Ctrl Pts',(-136.754821752032,4.9446218826347,127.049886984307));
#276991=CARTESIAN_POINT('Ctrl Pts',(-137.033269375845,-0.486056093210629,
124.614925481843));
#276992=CARTESIAN_POINT('Ctrl Pts',(-137.311716999657,-5.47007226455594,
127.867752498391));
#276993=CARTESIAN_POINT('Ctrl Pts',(-137.59016462347,-5.42735925266033,
133.819178915179));
#276994=CARTESIAN_POINT('Ctrl Pts',(-137.868612247283,-0.397168228809268,
137.000134598521));
#276995=CARTESIAN_POINT('Ctrl Pts',(-138.147059871096,4.99800099457058,
134.487476673751));
#276996=CARTESIAN_POINT('Ctrl Pts',(-138.425507494909,5.80025146986304,
128.590215023569));
#276997=CARTESIAN_POINT('Ctrl Pts',(-138.703955118722,1.27235420238826,
124.727645007244));
#276998=CARTESIAN_POINT('Ctrl Pts',(-138.982402742535,-4.42477441912264,
126.449279772744));
#276999=CARTESIAN_POINT('Ctrl Pts',(-139.260850366348,-6.05575151170779,
132.173021077107));
#277000=CARTESIAN_POINT('Ctrl Pts',(-139.539297990161,-2.12178880494131,
136.639030281933));
#277001=CARTESIAN_POINT('Ctrl Pts',(-139.817745613973,3.76199415842019,
135.743263104665));
#277002=CARTESIAN_POINT('Ctrl Pts',(-140.096193237787,6.18868827382574,
130.308885820552));
#277003=CARTESIAN_POINT('Ctrl Pts',(-140.374640861599,2.92828019981485,
125.329825669606));
#277004=CARTESIAN_POINT('Ctrl Pts',(-140.653088485412,-3.02307432338508,
125.381595689934));
#277005=CARTESIAN_POINT('Ctrl Pts',(-140.931536109225,-6.19637122878504,
130.416621761961));
#277006=CARTESIAN_POINT('Ctrl Pts',(-141.209983733038,-3.675505684495,135.807960900193));
#277007=CARTESIAN_POINT('Ctrl Pts',(-141.488431356851,2.22297002541115,
136.601235818153));
#277008=CARTESIAN_POINT('Ctrl Pts',(-141.766878980664,6.07864488008735,
132.06746561987));
#277009=CARTESIAN_POINT('Ctrl Pts',(-142.045326604476,4.34834204827492,
126.372963630579));
#277010=CARTESIAN_POINT('Ctrl Pts',(-142.32377422829,-1.3778746975837,124.750698986551));
#277011=CARTESIAN_POINT('Ctrl Pts',(-142.602221852102,-5.83789190928377,
128.691453643612));
#277012=CARTESIAN_POINT('Ctrl Pts',(-142.880669475915,-4.93317165322728,
134.573866588494));
#277013=CARTESIAN_POINT('Ctrl Pts',(-143.159117099728,0.504892353312588,
136.992287696695));
#277014=CARTESIAN_POINT('Ctrl Pts',(-143.437564723541,5.47898495252035,
133.72430611622));
#277015=CARTESIAN_POINT('Ctrl Pts',(-143.716012347354,5.4181580436573,127.77303726975));
#277016=CARTESIAN_POINT('Ctrl Pts',(-143.994459971167,0.378308584408798,
124.607406491544));
#277017=CARTESIAN_POINT('Ctrl Pts',(-144.27290759498,-5.00918798250961,
127.136473817112));
#277018=CARTESIAN_POINT('Ctrl Pts',(-144.551355218793,-5.79348550593904,
133.036149926065));
#277019=CARTESIAN_POINT('Ctrl Pts',(-144.829802842605,-1.2538528769121,
136.884920689477));
#277020=CARTESIAN_POINT('Ctrl Pts',(-145.108250466418,4.43800929187927,
135.145953798675));
#277021=CARTESIAN_POINT('Ctrl Pts',(-145.386698090231,6.05155773023994,
129.417274873051));
#277022=CARTESIAN_POINT('Ctrl Pts',(-145.665145714044,2.10402024954095,
124.963259983731));
#277023=CARTESIAN_POINT('Ctrl Pts',(-145.943593337857,-3.77700905338292,
125.876931223274));
#277024=CARTESIAN_POINT('Ctrl Pts',(-146.22204096167,-6.18715155339789,
131.318669357863));
#277025=CARTESIAN_POINT('Ctrl Pts',(-146.500488585483,-2.9116040349975,
136.287782885497));
#277026=CARTESIAN_POINT('Ctrl Pts',(-146.778936209295,3.03956535180104,
136.217899228972));
#277027=CARTESIAN_POINT('Ctrl Pts',(-147.057383833109,6.19752267131684,
131.173238054629));
#277028=CARTESIAN_POINT('Ctrl Pts',(-147.335831456921,3.66025942170698,
125.789596536289));
#277029=CARTESIAN_POINT('Ctrl Pts',(-147.614279080735,-2.24060342283806,
125.014278223797));
#277030=CARTESIAN_POINT('Ctrl Pts',(-147.892726704547,-6.08246118135759,
129.559762769929));
#277031=CARTESIAN_POINT('Ctrl Pts',(-148.17117432836,-4.33483425895693,
135.248971936054));
#277032=CARTESIAN_POINT('Ctrl Pts',(-148.449621952173,1.39629357899829,
136.853800431821));
#277033=CARTESIAN_POINT('Ctrl Pts',(-148.728069575986,5.84429583058792,
132.899489269852));
#277034=CARTESIAN_POINT('Ctrl Pts',(-149.006517199799,4.9216757235908,127.019857229157));
#277035=CARTESIAN_POINT('Ctrl Pts',(-149.284964823612,-0.52372393616008,
124.617998919139));
#277036=CARTESIAN_POINT('Ctrl Pts',(-149.563412447425,-5.48784688391679,
127.901104789406));
#277037=CARTESIAN_POINT('Ctrl Pts',(-149.841860071237,-5.40890664157841,
133.852160933818));
#277038=CARTESIAN_POINT('Ctrl Pts',(-150.12030769505,-0.359445435409253,
137.002437480918));
#277039=CARTESIAN_POINT('Ctrl Pts',(-150.398755318863,5.02032856601553,
134.456984183485));
#277040=CARTESIAN_POINT('Ctrl Pts',(-150.677202942676,5.78666587195703,
128.554948269553));
#277041=CARTESIAN_POINT('Ctrl Pts',(-150.955650566489,1.23533993591347,
124.720012413542));
#277042=CARTESIAN_POINT('Ctrl Pts',(-151.234098190302,-4.45120305152329,
126.476295320094));
#277043=CARTESIAN_POINT('Ctrl Pts',(-151.512545814115,-6.0473078879686,
132.209858797279));
#277044=CARTESIAN_POINT('Ctrl Pts',(-151.790993437928,-2.08623220278462,
136.651838109709));
#277045=CARTESIAN_POINT('Ctrl Pts',(-152.069441061741,3.79198895864895,
135.720271272016));
#277046=CARTESIAN_POINT('Ctrl Pts',(-152.347888685554,6.18555751604382,
130.27122269847));
#277047=CARTESIAN_POINT('Ctrl Pts',(-152.626336309366,2.89490089747778,
125.312101827337));
#277048=CARTESIAN_POINT('Ctrl Pts',(-152.904783933179,-3.05602822209906,
125.400098472666));
#277049=CARTESIAN_POINT('Ctrl Pts',(-153.183231556992,-6.19861670084527,
130.454348016274));
#277050=CARTESIAN_POINT('Ctrl Pts',(-153.461679180805,-3.64497925077551,
135.830242041403));
#277051=CARTESIAN_POINT('Ctrl Pts',(-153.740126804618,2.25821606362131,
136.587596565983));
#277052=CARTESIAN_POINT('Ctrl Pts',(-154.018574428431,6.08622113553776,
132.030439780749));
#277053=CARTESIAN_POINT('Ctrl Pts',(-154.297022052244,4.32128631232727,
126.346576141847));
#277054=CARTESIAN_POINT('Ctrl Pts',(-154.575469676057,-1.41469952533967,
124.759198661251));
#277055=CARTESIAN_POINT('Ctrl Pts',(-154.85391729987,-5.85064561113321,
128.727029695929));
#277056=CARTESIAN_POINT('Ctrl Pts',(-155.132364923682,-4.9101342002235,
134.603826364333));
#277057=CARTESIAN_POINT('Ctrl Pts',(-155.410812547495,0.542550667301237,
136.989099625678));
#277058=CARTESIAN_POINT('Ctrl Pts',(-155.689260171308,5.49665797664923,
133.690899879866));
#277059=CARTESIAN_POINT('Ctrl Pts',(-155.967707795121,5.39960513212718,
127.740111567281));
#277060=CARTESIAN_POINT('Ctrl Pts',(-156.246155418934,0.340578956555753,
124.605218435021));
#277061=CARTESIAN_POINT('Ctrl Pts',(-156.524603042747,-5.03142264188343,
127.167034123586));
#277062=CARTESIAN_POINT('Ctrl Pts',(-156.80305066656,-5.77979263109261,
133.071375166841));
#277063=CARTESIAN_POINT('Ctrl Pts',(-157.081498290373,-1.21681555089514,
136.89244058913));
#277064=CARTESIAN_POINT('Ctrl Pts',(-157.359945914186,4.46435557583064,
135.118857936792));
#277065=CARTESIAN_POINT('Ctrl Pts',(-157.638393537999,6.04300202426259,
129.380463022997));
#277066=CARTESIAN_POINT('Ctrl Pts',(-157.916841161811,2.06842482945845,
124.950560437346));
#277067=CARTESIAN_POINT('Ctrl Pts',(-158.195288785624,-3.80693373544809,
125.900014243279));
#277068=CARTESIAN_POINT('Ctrl Pts',(-158.473736409437,-6.18390617652933,
131.356322776543));
#277069=CARTESIAN_POINT('Ctrl Pts',(-158.75218403325,-2.87817094199197,
136.305405050556));
#277070=CARTESIAN_POINT('Ctrl Pts',(-159.030631657063,3.07246278176887,
136.199296231612));
#277071=CARTESIAN_POINT('Ctrl Pts',(-159.309079280876,6.19965330723533,
131.135505140616));
#277072=CARTESIAN_POINT('Ctrl Pts',(-159.587526904689,3.62966531325439,
125.767408410247));
#277073=CARTESIAN_POINT('Ctrl Pts',(-159.865974528502,-2.27580778459908,
125.028024689608));
#277074=CARTESIAN_POINT('Ctrl Pts',(-160.144422152314,-6.08992470779737,
129.596811497064));
#277075=CARTESIAN_POINT('Ctrl Pts',(-160.422869776128,-4.3076983338908,
135.275276954208));
#277076=CARTESIAN_POINT('Ctrl Pts',(-160.70131739994,1.43309236609815,136.845188714382));
#277077=CARTESIAN_POINT('Ctrl Pts',(-160.979765023753,5.85694119209746,
132.863874564441));
#277078=CARTESIAN_POINT('Ctrl Pts',(-161.258212647566,4.89854719004298,
126.989967710171));
#277079=CARTESIAN_POINT('Ctrl Pts',(-161.536660271379,-0.561372372326459,
124.621301594343));
#277080=CARTESIAN_POINT('Ctrl Pts',(-161.815107895192,-5.50541814909322,
127.934564661631));
#277081=CARTESIAN_POINT('Ctrl Pts',(-162.093555519005,-5.39025360147175,
133.885030015096));
#277082=CARTESIAN_POINT('Ctrl Pts',(-162.372003142818,-0.32170932262588,
137.004510691297));
#277083=CARTESIAN_POINT('Ctrl Pts',(-162.650450766631,5.04247010733932,
134.426356343909));
#277084=CARTESIAN_POINT('Ctrl Pts',(-162.928898390443,5.77286584701905,
128.519764868338));
#277085=CARTESIAN_POINT('Ctrl Pts',(-163.207346014257,1.19827989346308,
124.712605277602));
#277086=CARTESIAN_POINT('Ctrl Pts',(-163.485793638069,-4.47746674295796,
126.503471245498));
#277087=CARTESIAN_POINT('Ctrl Pts',(-163.764241261882,-6.03864017901171,
132.246644436198));
#277088=CARTESIAN_POINT('Ctrl Pts',(-164.042688885695,-2.05059829452646,
136.664429257056));
#277089=CARTESIAN_POINT('Ctrl Pts',(-164.321136509508,3.82184324533235,
135.697097278492));
#277090=CARTESIAN_POINT('Ctrl Pts',(-164.599584133321,6.18219755015336,
130.23357933201));
#277091=CARTESIAN_POINT('Ctrl Pts',(-164.878031757134,2.86141432352365,
125.294581502737));
#277092=CARTESIAN_POINT('Ctrl Pts',(-165.156479380946,-3.08886887856293,
125.418801512319));
#277093=CARTESIAN_POINT('Ctrl Pts',(-165.43492700476,-6.20063248088431,
130.492087240433));
#277094=CARTESIAN_POINT('Ctrl Pts',(-165.713374628572,-3.61431775100944,
135.85233694673));
#277095=CARTESIAN_POINT('Ctrl Pts',(-165.991822252385,2.2933784228048,136.573743013877));
#277096=CARTESIAN_POINT('Ctrl Pts',(-166.270269876198,6.09357186382579,
131.993368508814));
#277097=CARTESIAN_POINT('Ctrl Pts',(-166.548717500011,4.2940704495262,126.320353837957));
#277098=CARTESIAN_POINT('Ctrl Pts',(-166.827165123824,-1.45147193088449,
124.767922341652));
#277099=CARTESIAN_POINT('Ctrl Pts',(-167.105612747637,-5.86318251515793,
128.762682724506));
#277100=CARTESIAN_POINT('Ctrl Pts',(-167.38406037145,-4.88691480039125,
134.633645349573));
#277101=CARTESIAN_POINT('Ctrl Pts',(-167.662507995262,0.580188876875391,
136.985682376883));
#277102=CARTESIAN_POINT('Ctrl Pts',(-167.940955619076,5.51412732009539,
133.657386681736));
#277103=CARTESIAN_POINT('Ctrl Pts',(-168.219403242888,5.38085213624319,
127.707299411689));
#277104=CARTESIAN_POINT('Ctrl Pts',(-168.497850866701,0.302836708424229,
124.60326008999));
#277105=CARTESIAN_POINT('Ctrl Pts',(-168.776298490514,-5.05347086004094,
127.197729212531));
#277106=CARTESIAN_POINT('Ctrl Pts',(-169.054746114327,-5.7658855839047,
133.106516402559));
#277107=CARTESIAN_POINT('Ctrl Pts',(-169.33319373814,-1.17973313533045,
136.899734892741));
#277108=CARTESIAN_POINT('Ctrl Pts',(-169.611641361953,4.49053643144484,
135.091602199623));
#277109=CARTESIAN_POINT('Ctrl Pts',(-169.890088985766,6.03422239262278,
129.34370393599));
#277110=CARTESIAN_POINT('Ctrl Pts',(-170.168536609579,2.03275276313275,
124.938077805679));
#277111=CARTESIAN_POINT('Ctrl Pts',(-170.446984233392,-3.83671735018369,
125.923278995643));
#277112=CARTESIAN_POINT('Ctrl Pts',(-170.725431857205,-6.18043165274327,
131.393955742061));
#277113=CARTESIAN_POINT('Ctrl Pts',(-171.003879481017,-2.84463119730373,
136.32282337239));
#277114=CARTESIAN_POINT('Ctrl Pts',(-171.282327104831,3.10524636049842,
136.180493322929));
#277115=CARTESIAN_POINT('Ctrl Pts',(-171.560774728643,6.20155421272058,
131.097759955922));
#277116=CARTESIAN_POINT('Ctrl Pts',(-171.839222352457,3.59893670621881,
125.745406930321));
#277117=CARTESIAN_POINT('Ctrl Pts',(-172.117669976268,-2.31092781546573,
125.04198519967));
#277118=CARTESIAN_POINT('Ctrl Pts',(-172.396117600082,-6.09716256983718,
129.633904970377));
#277119=CARTESIAN_POINT('Ctrl Pts',(-172.674565223895,-4.2804027854792,
135.301416300912));
#277120=CARTESIAN_POINT('Ctrl Pts',(-172.953012847708,1.469838049433,136.836353151837));
#277121=CARTESIAN_POINT('Ctrl Pts',(-173.23146047152,5.86936952249723,132.828183542982));
#277122=CARTESIAN_POINT('Ctrl Pts',(-173.509908095334,4.8752371390276,126.960219534917));
#277123=CARTESIAN_POINT('Ctrl Pts',(-173.788355719146,-0.599000006633149,
124.624833385073));
#277124=CARTESIAN_POINT('Ctrl Pts',(-174.06680334296,-5.5227854089755,127.968130875202));
#277125=CARTESIAN_POINT('Ctrl Pts',(-174.345250966772,-5.37140082353563,
133.917784941036));
#277126=CARTESIAN_POINT('Ctrl Pts',(-174.623698590585,-0.283961288785237,
137.006354152836));
#277127=CARTESIAN_POINT('Ctrl Pts',(-174.902146214398,5.06442479807889,
134.39559428995));
#277128=CARTESIAN_POINT('Ctrl Pts',(-175.18059383821,5.75885190641417,128.484666123661));
#277129=CARTESIAN_POINT('Ctrl Pts',(-175.459041462024,1.16117544831056,
124.705423873895));
#277130=CARTESIAN_POINT('Ctrl Pts',(-175.737489085836,-4.50356452021585,
126.530806541938));
#277131=CARTESIAN_POINT('Ctrl Pts',(-176.01593670965,-6.02974870602229,
132.28337663076));
#277132=CARTESIAN_POINT('Ctrl Pts',(-176.294384333462,-2.01488840059438,
136.676803257405));
#277133=CARTESIAN_POINT('Ctrl Pts',(-176.572831957276,3.85155591220881,
135.67374198281));
#277134=CARTESIAN_POINT('Ctrl Pts',(-176.851279581088,6.17860850065921,
130.195957116059));
#277135=CARTESIAN_POINT('Ctrl Pts',(-177.129727204901,2.82782171880919,
125.277265345029));
#277136=CARTESIAN_POINT('Ctrl Pts',(-177.408174828714,-3.12159507585506,
125.437704115845));
#277137=CARTESIAN_POINT('Ctrl Pts',(-177.686622452527,-6.20241849420629,
130.529838035997));
#277138=CARTESIAN_POINT('Ctrl Pts',(-177.965070076339,-3.58352232136993,
135.874244797437));
#277139=CARTESIAN_POINT('Ctrl Pts',(-178.243517700153,2.32845580000743,
136.559675675186));
#277140=CARTESIAN_POINT('Ctrl Pts',(-178.521965323965,6.10069679256748,
131.956253177754));
#277141=CARTESIAN_POINT('Ctrl Pts',(-178.800412947778,4.26669546836545,
126.294297690589));
#277142=CARTESIAN_POINT('Ctrl Pts',(-179.078860571591,-1.48819055160311,
124.776869704492));
#277143=CARTESIAN_POINT('Ctrl Pts',(-179.357308195404,-5.8755021567984,
128.798411408209));
#277144=CARTESIAN_POINT('Ctrl Pts',(-179.635755819217,-4.86351431413387,
134.663322439258));
#277145=CARTESIAN_POINT('Ctrl Pts',(-179.91420344303,0.617805587336893,
136.982036076937));
#277146=CARTESIAN_POINT('Ctrl Pts',(-180.192651066843,5.53139233552561,
133.623767763677));
#277147=CARTESIAN_POINT('Ctrl Pts',(-180.471098690656,5.36189975090491,
127.674602018838));
#277148=CARTESIAN_POINT('Ctrl Pts',(-180.749546314469,0.265083238567079,
124.601531529021));
#277149=CARTESIAN_POINT('Ctrl Pts',(-181.027993938281,-5.07533181997731,
127.22855794653));
#277150=CARTESIAN_POINT('Ctrl Pts',(-181.306441562095,-5.75176487970607,
133.141572331048));
#277151=CARTESIAN_POINT('Ctrl Pts',(-181.584889185907,-1.14260700432061,
136.906803330016));
#277152=CARTESIAN_POINT('Ctrl Pts',(-181.86333680972,4.5165508885802,135.064187597142));
#277153=CARTESIAN_POINT('Ctrl Pts',(-182.141784433533,6.02521916065313,
129.306998974155));
#277154=CARTESIAN_POINT('Ctrl Pts',(-182.420232057346,1.99700537240587,
124.925812551278));
#277155=CARTESIAN_POINT('Ctrl Pts',(-182.698679681159,-3.86635879394691,
125.946724618282));
#277156=CARTESIAN_POINT('Ctrl Pts',(-182.977127304972,-6.17672811078948,
131.431566859916));
#277157=CARTESIAN_POINT('Ctrl Pts',(-183.255574928785,-2.81098604376035,
136.340037205557));
#277158=CARTESIAN_POINT('Ctrl Pts',(-183.534022552597,3.13791487318212,
136.161491199671));
#277159=CARTESIAN_POINT('Ctrl Pts',(-183.81247017641,6.20322531733387,131.060003899207));
#277160=CARTESIAN_POINT('Ctrl Pts',(-184.090917800223,3.56807473926006,
125.723592911784));
#277161=CARTESIAN_POINT('Ctrl Pts',(-184.369365424036,-2.34596221405232,
125.056159236672));
#277162=CARTESIAN_POINT('Ctrl Pts',(-184.647813047849,-6.10417449927606,
129.671041815353));
#277163=CARTESIAN_POINT('Ctrl Pts',(-184.926260671662,-4.25294862516783,
135.327389007565));
#277164=CARTESIAN_POINT('Ctrl Pts',(-185.204708295475,1.50652926737877,
136.827294071589));
#277165=CARTESIAN_POINT('Ctrl Pts',(-185.483155919288,5.88158036125089,
132.792417528021));
#277166=CARTESIAN_POINT('Ctrl Pts',(-185.761603543101,4.85174643430717,
126.930613805724));
#277167=CARTESIAN_POINT('Ctrl Pts',(-186.040051166913,-0.6366054447743,
124.628594160457));
#277168=CARTESIAN_POINT('Ctrl Pts',(-186.318498790727,-5.53994802001346,
128.001802186308));
#277169=CARTESIAN_POINT('Ctrl Pts',(-186.596946414539,-5.35234900636664,
133.950424497894));
#277170=CARTESIAN_POINT('Ctrl Pts',(-186.875394038353,-0.246202732654624,
137.007967797222));
#277171=CARTESIAN_POINT('Ctrl Pts',(-187.153841662165,5.08619182469514,
134.364699161505));
#277172=CARTESIAN_POINT('Ctrl Pts',(-187.432289285978,5.744624569434,128.449653336115));
#277173=CARTESIAN_POINT('Ctrl Pts',(-187.71073690979,1.12402797537536,124.698468468532));
#277174=CARTESIAN_POINT('Ctrl Pts',(-187.989184533604,-4.52949541623416,
126.558300196495));
#277175=CARTESIAN_POINT('Ctrl Pts',(-188.267632157416,-6.0206337984771,
132.32005401984));
#277176=CARTESIAN_POINT('Ctrl Pts',(-188.54607978123,-1.97910384423165,
136.688959652232));
#277177=CARTESIAN_POINT('Ctrl Pts',(-188.824527405043,3.88112585826452,
135.650206250412));
#277178=CARTESIAN_POINT('Ctrl Pts',(-189.102975028855,6.17479050055486,
130.158357444724));
#277179=CARTESIAN_POINT('Ctrl Pts',(-189.381422652668,2.79412432812102,
125.260153995869));
#277180=CARTESIAN_POINT('Ctrl Pts',(-189.659870276481,-3.15420560129371,
125.456805582802));
#277181=CARTESIAN_POINT('Ctrl Pts',(-189.938317900294,-6.20397467462999,
130.567599004095));
#277182=CARTESIAN_POINT('Ctrl Pts',(-190.216765524107,-3.55259410299321,
135.89596478172));
#277183=CARTESIAN_POINT('Ctrl Pts',(-190.49521314792,2.36344689542356,136.545395071179));
#277184=CARTESIAN_POINT('Ctrl Pts',(-190.773660771733,6.10759565774615,
131.919095162891));
#277185=CARTESIAN_POINT('Ctrl Pts',(-191.052108395545,4.23916238323504,
126.26840866526));
#277186=CARTESIAN_POINT('Ctrl Pts',(-191.330556019359,-1.52485402687357,
124.786040418225));
#277187=CARTESIAN_POINT('Ctrl Pts',(-191.609003643171,-5.88760407954571,
128.834214423098));
#277188=CARTESIAN_POINT('Ctrl Pts',(-191.887451266984,-4.83993360856504,
134.692856533694));
#277189=CARTESIAN_POINT('Ctrl Pts',(-192.165898890797,0.655399404785621,
136.978160860955));
#277190=CARTESIAN_POINT('Ctrl Pts',(-192.44434651461,5.54845238317892,133.59004437145));
#277191=CARTESIAN_POINT('Ctrl Pts',(-192.722794138423,5.34274867839911,
127.642020600343));
#277192=CARTESIAN_POINT('Ctrl Pts',(-193.001241762236,0.227319945953055,
124.600032816164));
#277193=CARTESIAN_POINT('Ctrl Pts',(-193.279689386049,-5.09700471162664,
127.259519183211));
#277194=CARTESIAN_POINT('Ctrl Pts',(-193.558137009861,-5.73743104174462,
133.176541653297));
#277195=CARTESIAN_POINT('Ctrl Pts',(-193.836584633675,-1.105438533588,136.913645639033));
#277196=CARTESIAN_POINT('Ctrl Pts',(-194.115032257487,4.5423979832614,135.036615145204));
#277197=CARTESIAN_POINT('Ctrl Pts',(-194.3934798813,6.01599266197172,129.270349497605));
#277198=CARTESIAN_POINT('Ctrl Pts',(-194.671927505113,1.96118398191049,
124.913765128639));
#277199=CARTESIAN_POINT('Ctrl Pts',(-194.950375128926,-3.89585696836267,
125.970350242409));
#277200=CARTESIAN_POINT('Ctrl Pts',(-195.228822752739,-6.17279568790409,
131.469154736412));
#277201=CARTESIAN_POINT('Ctrl Pts',(-195.507270376552,-2.77723672809589,
136.357045912194));
#277202=CARTESIAN_POINT('Ctrl Pts',(-195.785718000365,3.17046710927626,
136.142290565968));
#277203=CARTESIAN_POINT('Ctrl Pts',(-196.064165624178,6.20466655915177,
131.022238369536));
#277204=CARTESIAN_POINT('Ctrl Pts',(-196.342613247991,3.5370805559797,125.701967162963));
#277205=CARTESIAN_POINT('Ctrl Pts',(-196.621060871803,-2.38090968214636,
125.070546275391));
#277206=CARTESIAN_POINT('Ctrl Pts',(-196.899508495616,-6.11096023628406,
129.708220655875));
#277207=CARTESIAN_POINT('Ctrl Pts',(-197.177956119429,-4.22533687028115,
135.353194111738));
#277208=CARTESIAN_POINT('Ctrl Pts',(-197.456403743242,1.54316466032852,
136.818011809327));
#277209=CARTESIAN_POINT('Ctrl Pts',(-197.734851367055,5.89357325588093,
132.75657784488));
#277210=CARTESIAN_POINT('Ctrl Pts',(-198.013298990868,4.82807594633875,
126.901151619645));
#277211=CARTESIAN_POINT('Ctrl Pts',(-198.291746614681,-0.674187293266194,
124.632583781138));
#277212=CARTESIAN_POINT('Ctrl Pts',(-198.570194238494,-5.55690534624021,
128.035577347248));
#277213=CARTESIAN_POINT('Ctrl Pts',(-198.848641862306,-5.33309885593691,
133.982947476197));
#277214=CARTESIAN_POINT('Ctrl Pts',(-199.12708948612,-0.2084350533912,137.009351564664));
#277215=CARTESIAN_POINT('Ctrl Pts',(-199.405537109932,5.10777038060287,
134.333672103408));
#277216=CARTESIAN_POINT('Ctrl Pts',(-199.683984733745,5.7301843632779,128.414727803113));
#277217=CARTESIAN_POINT('Ctrl Pts',(-199.962432357558,1.08683885116959,
124.691739319248));
#277218=CARTESIAN_POINT('Ctrl Pts',(-200.240879981371,-4.5552584701342,
126.585951190383));
#277219=CARTESIAN_POINT('Ctrl Pts',(-200.519327605184,-6.01129579413245,
132.356675244344));
#277220=CARTESIAN_POINT('Ctrl Pts',(-200.797775228997,-1.94324595144814,
136.700897991079));
#277221=CARTESIAN_POINT('Ctrl Pts',(-201.076222852809,3.91055198777426,
135.626490953421));
#277222=CARTESIAN_POINT('Ctrl Pts',(-201.354670476623,6.17074369131775,
130.120781711275));
#277223=CARTESIAN_POINT('Ctrl Pts',(-201.633118100435,2.76032340012831,
125.243248089324));
#277224=CARTESIAN_POINT('Ctrl Pts',(-201.911565724248,-3.18669924648382,
125.476105205376));
#277225=CARTESIAN_POINT('Ctrl Pts',(-202.190013348061,-6.20530096449064,
130.605368745483));
#277226=CARTESIAN_POINT('Ctrl Pts',(-202.468460971874,-3.52153424193529,
135.91749609474));
#277227=CARTESIAN_POINT('Ctrl Pts',(-202.746908595687,2.39835041244635,
136.530901731028));
#277228=CARTESIAN_POINT('Ctrl Pts',(-203.0253562195,6.11426820372151,131.881895841131));
#277229=CARTESIAN_POINT('Ctrl Pts',(-203.303803843313,4.21147221438356,
126.242687721299));
#277230=CARTESIAN_POINT('Ctrl Pts',(-203.582251467125,-1.56146099811728,
124.795434143027));
#277231=CARTESIAN_POINT('Ctrl Pts',(-203.860699090939,-5.89948783495869,
128.870090442477));
#277232=CARTESIAN_POINT('Ctrl Pts',(-204.139146714752,-4.81617355747646,
134.722246538484));
#277233=CARTESIAN_POINT('Ctrl Pts',(-204.417594338564,0.69296893616836,
136.974056872534));
#277234=CARTESIAN_POINT('Ctrl Pts',(-204.696041962377,5.56530683088876,
133.556217754686));
#277235=CARTESIAN_POINT('Ctrl Pts',(-204.97448958619,5.32339962837619,127.60955636352));
#277236=CARTESIAN_POINT('Ctrl Pts',(-205.252937210003,0.18954822991528,
124.598764006957));
#277237=CARTESIAN_POINT('Ctrl Pts',(-205.531384833816,-5.11848873189165,
127.290611775294));
#277238=CARTESIAN_POINT('Ctrl Pts',(-205.809832457629,-5.72288460116635,
133.211423073505));
#277239=CARTESIAN_POINT('Ctrl Pts',(-206.088280081441,-1.06822910042401,
136.920261566246));
#277240=CARTESIAN_POINT('Ctrl Pts',(-206.366727705255,4.56807675771487,
135.00888586552));
#277241=CARTESIAN_POINT('Ctrl Pts',(-206.645175329067,6.00654323846982,
129.233756864401));
#277242=CARTESIAN_POINT('Ctrl Pts',(-206.92362295288,1.92528991902147,124.901935984182));
#277243=CARTESIAN_POINT('Ctrl Pts',(-207.202070576693,-3.92521078036628,
125.994154992568));
#277244=CARTESIAN_POINT('Ctrl Pts',(-207.480518200506,-6.16863452980439,
131.506717978718));
#277245=CARTESIAN_POINT('Ctrl Pts',(-207.758965824319,-2.74338450090264,
136.373848862034));
#277246=CARTESIAN_POINT('Ctrl Pts',(-208.037413448132,3.20290186254569,
136.12289213331));
#277247=CARTESIAN_POINT('Ctrl Pts',(-208.315861071945,6.20587788476857,
130.984464766326));
#277248=CARTESIAN_POINT('Ctrl Pts',(-208.594308695758,3.50595530487857,
125.680530485208));
#277249=CARTESIAN_POINT('Ctrl Pts',(-208.872756319571,-2.41576892475653,
125.085145782709));
#277250=CARTESIAN_POINT('Ctrl Pts',(-209.151203943383,-6.11751952941318,
129.745440114266));
#277251=CARTESIAN_POINT('Ctrl Pts',(-209.429651567197,-4.19756854398286,
135.378830657213));
#277252=CARTESIAN_POINT('Ctrl Pts',(-209.708099191009,1.57974287074426,
136.808506709009));
#277253=CARTESIAN_POINT('Ctrl Pts',(-209.986546814822,5.90534776198698,
132.720665821612));
#277254=CARTESIAN_POINT('Ctrl Pts',(-210.264994438635,4.80422655224024,
126.87183406841));
#277255=CARTESIAN_POINT('Ctrl Pts',(-210.543442062448,-0.711744159500396,
124.63680209928));
#277256=CARTESIAN_POINT('Ctrl Pts',(-210.821889686261,-5.57365675929581,
128.06945510647));
#277257=CARTESIAN_POINT('Ctrl Pts',(-211.100337310074,-5.31365108556781,
134.015352670796));
#277258=CARTESIAN_POINT('Ctrl Pts',(-211.378784933887,-0.170659650490228,
137.010505403884));
#277259=CARTESIAN_POINT('Ctrl Pts',(-211.657232557699,5.12915966620077,
134.302514265376));
#277260=CARTESIAN_POINT('Ctrl Pts',(-211.935680181513,5.71553182303293,
128.379890818834));
#277261=CARTESIAN_POINT('Ctrl Pts',(-212.214127805325,1.04960945375051,
124.685236675394));
#277262=CARTESIAN_POINT('Ctrl Pts',(-212.492575429138,-4.58085272725645,
126.613758498985));
#277263=CARTESIAN_POINT('Ctrl Pts',(-212.771023052951,-6.00173503901134,
132.393238947258));
#277264=CARTESIAN_POINT('Ctrl Pts',(-213.049470676764,-1.90731605097184,
136.712617831564));
#277265=CARTESIAN_POINT('Ctrl Pts',(-213.327918300577,3.93983321034183,
135.602596970618));
#277266=CARTESIAN_POINT('Ctrl Pts',(-213.60636592439,6.16646822290386,130.083231308093));
#277267=CARTESIAN_POINT('Ctrl Pts',(-213.884813548203,2.72642018733693,
125.226548251849));
#277268=CARTESIAN_POINT('Ctrl Pts',(-214.163261172015,-3.21907480736146,
125.495602268416));
#277269=CARTESIAN_POINT('Ctrl Pts',(-214.441708795829,-6.20639731464204,
130.643145860587));
#277270=CARTESIAN_POINT('Ctrl Pts',(-214.720156419641,-3.49034388913101,
135.938837938644));
#277271=CARTESIAN_POINT('Ctrl Pts',(-214.998604043455,2.43316505771265,
136.516196191791));
#277272=CARTESIAN_POINT('Ctrl Pts',(-215.277051667267,6.12071418324004,
131.844656590906));
#277273=CARTESIAN_POINT('Ctrl Pts',(-215.55549929108,4.18362598788043,126.217135811804));
#277274=CARTESIAN_POINT('Ctrl Pts',(-215.833946914893,-1.59801010884951,
124.805050530808));
#277275=CARTESIAN_POINT('Ctrl Pts',(-216.112394538706,-5.91115298268039,
128.90603813695));
#277276=CARTESIAN_POINT('Ctrl Pts',(-216.390842162519,-4.79223504130557,
134.75149136457));
#277277=CARTESIAN_POINT('Ctrl Pts',(-216.669289786332,0.730512789332353,
136.969724263749));
#277278=CARTESIAN_POINT('Ctrl Pts',(-216.947737410145,5.5819550541073,133.522289166845));
#277279=CARTESIAN_POINT('Ctrl Pts',(-217.226185033957,5.3038533178224,127.577210511344));
#277280=CARTESIAN_POINT('Ctrl Pts',(-217.50463265777,0.151769490097695,
124.597725148413));
#277281=CARTESIAN_POINT('Ctrl Pts',(-217.783080281583,-5.13978308467467,
127.321834570635));
#277282=CARTESIAN_POINT('Ctrl Pts',(-218.061527905396,-5.70812609699421,
133.24621529913));
#277283=CARTESIAN_POINT('Ctrl Pts',(-218.339975529209,-1.03098008363786,
136.9266508665));
#277284=CARTESIAN_POINT('Ctrl Pts',(-218.618423153022,4.59358626040416,
134.981000785606));
#277285=CARTESIAN_POINT('Ctrl Pts',(-218.896870776835,5.99687124029931,
129.197222430498));
#277286=CARTESIAN_POINT('Ctrl Pts',(-219.175318400648,1.88932451380644,
124.890325556239));
#277287=CARTESIAN_POINT('Ctrl Pts',(-219.45376602446,-3.95441914224089,
126.018137986666));
#277288=CARTESIAN_POINT('Ctrl Pts',(-219.732213648274,-6.16424479068368,
131.544255194914));
#277289=CARTESIAN_POINT('Ctrl Pts',(-220.010661272086,-2.70943061658779,
136.390445432439));
#277290=CARTESIAN_POINT('Ctrl Pts',(-220.289108895899,3.23521793110825,
136.103296620509));
#277291=CARTESIAN_POINT('Ctrl Pts',(-220.567556519712,6.20685924929812,
130.94668448929));
#277292=CARTESIAN_POINT('Ctrl Pts',(-220.846004143525,3.47470013931478,
125.659283672863));
#277293=CARTESIAN_POINT('Ctrl Pts',(-221.124451767337,-2.45053865016082,
125.099957217636));
#277294=CARTESIAN_POINT('Ctrl Pts',(-221.402899391151,-6.12385213560643,
129.782698811345));
#277295=CARTESIAN_POINT('Ctrl Pts',(-221.681347014963,-4.16964467523852,
135.404297694017));
#277296=CARTESIAN_POINT('Ctrl Pts',(-221.959794638777,1.61626254320698,
136.79877912285));
#277297=CARTESIAN_POINT('Ctrl Pts',(-222.238242262589,5.91690344326002,
132.684682788949));
#277298=CARTESIAN_POINT('Ctrl Pts',(-222.516689886402,4.7801991357601,126.842662238393));
#277299=CARTESIAN_POINT('Ctrl Pts',(-222.795137510215,-0.749274651793031,
124.64124895857));
#277300=CARTESIAN_POINT('Ctrl Pts',(-223.073585134028,-5.59020163845046,
128.103434208622));
#277301=CARTESIAN_POINT('Ctrl Pts',(-223.352032757841,-5.29400641590365,
134.047638880903));
#277302=CARTESIAN_POINT('Ctrl Pts',(-223.630480381654,-0.132877923733138,
137.011429272127));
#277303=CARTESIAN_POINT('Ctrl Pts',(-223.908928005467,5.15035888890098,
134.271226801972));
#277304=CARTESIAN_POINT('Ctrl Pts',(-224.187375629279,5.70066749165438,
128.345143674176));
#277305=CARTESIAN_POINT('Ctrl Pts',(-224.465823253093,1.01234116266713,
124.678960777928));
#277306=CARTESIAN_POINT('Ctrl Pts',(-224.744270876905,-4.60627723919628,
126.641721091889));
#277307=CARTESIAN_POINT('Ctrl Pts',(-225.022718500718,-5.99195188739136,
132.4297437737));
#277308=CARTESIAN_POINT('Ctrl Pts',(-225.301166124531,-1.87131547419729,
136.724118739406));
#277309=CARTESIAN_POINT('Ctrl Pts',(-225.579613748344,3.96896844094108,
135.578525187401));
#277310=CARTESIAN_POINT('Ctrl Pts',(-225.858061372157,6.16196425374224,
130.045707626623));
#277311=CARTESIAN_POINT('Ctrl Pts',(-226.13650899597,2.69241594604283,125.210055102262));
#277312=CARTESIAN_POINT('Ctrl Pts',(-226.414956619783,-3.25133108423828,
125.515296049447));
#277313=CARTESIAN_POINT('Ctrl Pts',(-226.693404243596,-6.20726368445854,
130.680928949564));
#277314=CARTESIAN_POINT('Ctrl Pts',(-226.971851867408,-3.45902420035033,
135.959989522602));
#277315=CARTESIAN_POINT('Ctrl Pts',(-227.250299491222,2.46788954115291,
136.501278998386));
#277316=CARTESIAN_POINT('Ctrl Pts',(-227.528747115034,6.12693335744362,
131.80737879213));
#277317=CARTESIAN_POINT('Ctrl Pts',(-227.807194738847,4.15562473557794,
126.191753883612));
#277318=CARTESIAN_POINT('Ctrl Pts',(-228.08564236266,-1.63450000472891,
124.81488922523));
#277319=CARTESIAN_POINT('Ctrl Pts',(-228.364089986473,-5.9225990904546,
128.942056174461));
#277320=CARTESIAN_POINT('Ctrl Pts',(-228.642537610286,-4.76811894710285,
134.780589928275));
#277321=CARTESIAN_POINT('Ctrl Pts',(-228.920985234099,0.768029573076269,
136.965163195147));
#277322=CARTESIAN_POINT('Ctrl Pts',(-229.199432857912,5.59839643592858,
133.48825986516));
#277323=CARTESIAN_POINT('Ctrl Pts',(-229.477880481725,5.28411047103341,
127.544984242401));
#277324=CARTESIAN_POINT('Ctrl Pts',(-229.756328105537,0.11398512640586,
124.59691627903));
#277325=CARTESIAN_POINT('Ctrl Pts',(-230.03477572935,-5.16088698090536,
127.353186412258));
#277326=CARTESIAN_POINT('Ctrl Pts',(-230.313223353163,-5.69315607611037,
133.280917040931));
#277327=CARTESIAN_POINT('Ctrl Pts',(-230.591670976976,-0.993692863505588,
136.932813303039));
#277328=CARTESIAN_POINT('Ctrl Pts',(-230.870118600789,4.6189255460653,134.952960938754));
#277329=CARTESIAN_POINT('Ctrl Pts',(-231.148566224602,5.98697702585963,
129.160747549691));
#277330=CARTESIAN_POINT('Ctrl Pts',(-231.427013848415,1.85328909897679,
124.878934275042));
#277331=CARTESIAN_POINT('Ctrl Pts',(-231.705461472227,-3.98348097165998,
126.042298336002));
#277332=CARTESIAN_POINT('Ctrl Pts',(-231.983909096041,-6.15962663320533,
131.581764994044));
#277333=CARTESIAN_POINT('Ctrl Pts',(-232.262356719853,-2.6753763333251,
136.406835008417));
#277334=CARTESIAN_POINT('Ctrl Pts',(-232.540804343666,3.26741411748112,
136.083504753687));
#277335=CARTESIAN_POINT('Ctrl Pts',(-232.819251967479,6.20761061637562,
130.90889893839));
#277336=CARTESIAN_POINT('Ctrl Pts',(-233.097699591292,3.44331621745904,
125.638227513236));
#277337=CARTESIAN_POINT('Ctrl Pts',(-233.376147215105,-2.48521756995422,
125.114980031328));
#277338=CARTESIAN_POINT('Ctrl Pts',(-233.654594838918,-6.12995782020675,
129.819995366479));
#277339=CARTESIAN_POINT('Ctrl Pts',(-233.933042462731,-4.14156629877734,
135.429594278462));
#277340=CARTESIAN_POINT('Ctrl Pts',(-234.211490086544,1.65272232446679,
136.788829411307));
#277341=CARTESIAN_POINT('Ctrl Pts',(-234.489937710357,5.92823987150001,
132.648630080257));
#277342=CARTESIAN_POINT('Ctrl Pts',(-234.768385334169,4.75599458724306,
126.813637210565));
#277343=CARTESIAN_POINT('Ctrl Pts',(-235.046832957982,-0.786777379437916,
124.64592419423));
#277344=CARTESIAN_POINT('Ctrl Pts',(-235.325280581795,-5.6065393706272,
128.137513394595));
#277345=CARTESIAN_POINT('Ctrl Pts',(-235.603728205608,-5.27416557488518,
134.079804910139));
#277346=CARTESIAN_POINT('Ctrl Pts',(-235.882175829421,-0.0950912731361558,
137.012123135159));
#277347=CARTESIAN_POINT('Ctrl Pts',(-236.160623453234,5.17136726315852,
134.239810872567));
#277348=CARTESIAN_POINT('Ctrl Pts',(-236.439071077047,5.68559191994549,
128.310487656705));
#277349=CARTESIAN_POINT('Ctrl Pts',(-236.71751870086,0.975035358909668,
124.672911859406));
#277350=CARTESIAN_POINT('Ctrl Pts',(-236.995966324673,-4.63153106383903,
126.669837932931));
#277351=CARTESIAN_POINT('Ctrl Pts',(-237.274413948486,-5.98194670179065,
132.466188370973));
#277352=CARTESIAN_POINT('Ctrl Pts',(-237.552861572298,-1.83524555513966,
136.735400288432));
#277353=CARTESIAN_POINT('Ctrl Pts',(-237.831309196112,3.99795659995517,
135.554276495761));
#277354=CARTESIAN_POINT('Ctrl Pts',(-238.109756819924,6.15723195072914,
130.008212057319));
#277355=CARTESIAN_POINT('Ctrl Pts',(-238.388204443737,2.65831193628575,
125.193769251723));
#277356=CARTESIAN_POINT('Ctrl Pts',(-238.66665206755,-3.28346688184612,
125.535185818711));
#277357=CARTESIAN_POINT('Ctrl Pts',(-238.945099691363,-6.20790004183648,
130.718716612347));
#277358=CARTESIAN_POINT('Ctrl Pts',(-239.223547315176,-3.42757633615586,
135.980950062836));
#277359=CARTESIAN_POINT('Ctrl Pts',(-239.501994938989,2.50252257603867,
136.486150703575));
#277360=CARTESIAN_POINT('Ctrl Pts',(-239.780442562802,6.13292549587844,
131.770063826148));
#277361=CARTESIAN_POINT('Ctrl Pts',(-240.058890186614,4.12746949507249,
126.166542877259));
#277362=CARTESIAN_POINT('Ctrl Pts',(-240.337337810428,-1.67092933361012,
124.824949861719));
#277363=CARTESIAN_POINT('Ctrl Pts',(-240.61578543424,-5.93382573414137,
128.978143220346));
#277364=CARTESIAN_POINT('Ctrl Pts',(-240.894233058053,-4.74382616849909,
134.80954115134));
#277365=CARTESIAN_POINT('Ctrl Pts',(-241.172680681866,0.805517897201924,
136.960373835741));
#277366=CARTESIAN_POINT('Ctrl Pts',(-241.451128305679,5.6146303671111,133.454131110603));
#277367=CARTESIAN_POINT('Ctrl Pts',(-241.729575929492,5.26417181958768,
127.512878750849));
#277368=CARTESIAN_POINT('Ctrl Pts',(-242.008023553305,0.0761965389532375,
124.596337428779));
#277369=CARTESIAN_POINT('Ctrl Pts',(-242.286471177117,-5.18179963857104,
127.384666138411));
#277370=CARTESIAN_POINT('Ctrl Pts',(-242.564918800931,-5.67797509323448,
133.315527013022));
#277371=CARTESIAN_POINT('Ctrl Pts',(-242.843366424743,-0.956368821719198,
136.938748647509));
#277372=CARTESIAN_POINT('Ctrl Pts',(-243.121814048556,4.64409367574132,
134.924767363992));
#277373=CARTESIAN_POINT('Ctrl Pts',(-243.400261672369,5.9768609617849,129.124333573571));
#277374=CARTESIAN_POINT('Ctrl Pts',(-243.678709296182,1.81718500983798,
124.867762562695));
#277375=CARTESIAN_POINT('Ctrl Pts',(-243.957156919995,-4.01239519172672,
126.066635145309));
#277376=CARTESIAN_POINT('Ctrl Pts',(-244.235604543808,-6.15478022849689,
131.619245986169));
#277377=CARTESIAN_POINT('Ctrl Pts',(-244.514052167621,-2.64122291300849,
136.423016982646));
#277378=CARTESIAN_POINT('Ctrl Pts',(-244.792499791433,3.29948922862226,
136.063517266237));
#277379=CARTESIAN_POINT('Ctrl Pts',(-245.070947415247,6.20813195815889,
130.871109513785));
#277380=CARTESIAN_POINT('Ctrl Pts',(-245.349395039059,3.41180470225455,
125.617362786572));
#277381=CARTESIAN_POINT('Ctrl Pts',(-245.627842662872,-2.51980439909662,
125.13021366711));
#277382=CARTESIAN_POINT('Ctrl Pts',(-245.906290286685,-6.13583635696575,
129.857328397629));
#277383=CARTESIAN_POINT('Ctrl Pts',(-246.184737910498,-4.1133344550539,
135.454719473173));
#277384=CARTESIAN_POINT('Ctrl Pts',(-246.463185534311,1.68912086349306,
136.778657943074));
#277385=CARTESIAN_POINT('Ctrl Pts',(-246.741633158124,5.93935662663147,
132.612509031482));
#277386=CARTESIAN_POINT('Ctrl Pts',(-247.020080781937,4.73161380359756,
126.784760060463));
#277387=CARTESIAN_POINT('Ctrl Pts',(-247.29852840575,-0.824250952757648,
124.650827633015));
#277388=CARTESIAN_POINT('Ctrl Pts',(-247.576976029562,-5.62266935042617,
128.171691401572));
#277389=CARTESIAN_POINT('Ctrl Pts',(-247.855423653376,-5.25412929772145,
134.111849566585));
#277390=CARTESIAN_POINT('Ctrl Pts',(-248.133871277188,-0.0573010988966442,
137.012586967267));
#277391=CARTESIAN_POINT('Ctrl Pts',(-248.412318901001,5.19218401050035,
134.208267641291));
#277392=CARTESIAN_POINT('Ctrl Pts',(-248.690766524814,5.67030566653712,
128.275924050614));
#277393=CARTESIAN_POINT('Ctrl Pts',(-248.969214148627,0.937693424858449,
124.667090143972));
#277394=CARTESIAN_POINT('Ctrl Pts',(-249.24766177244,-4.65661326539506,
126.698107980232));
#277395=CARTESIAN_POINT('Ctrl Pts',(-249.526109396252,-5.97171985295489,
132.502571388608));
#277396=CARTESIAN_POINT('Ctrl Pts',(-249.804557020066,-1.79910763038337,
136.746462060605));
#277397=CARTESIAN_POINT('Ctrl Pts',(-250.083004643878,4.02679661321771,
135.52985179424));
#277398=CARTESIAN_POINT('Ctrl Pts',(-250.361452267692,6.15227148922063,
129.970745989595));
#277399=CARTESIAN_POINT('Ctrl Pts',(-250.639899891504,2.62410942180459,
125.177691303707));
#277400=CARTESIAN_POINT('Ctrl Pts',(-250.918347515317,-3.31548100938434,
125.555270839195));
#277401=CARTESIAN_POINT('Ctrl Pts',(-251.19679513913,-6.20830636318893,
130.756507448682));
#277402=CARTESIAN_POINT('Ctrl Pts',(-251.475242762943,-3.39600146187203,
136.001718782677));
#277403=CARTESIAN_POINT('Ctrl Pts',(-251.753690386756,2.53706287905323,
136.47081186788));
#277404=CARTESIAN_POINT('Ctrl Pts',(-252.032138010569,6.13869037645988,
131.732713075798));
#277405=CARTESIAN_POINT('Ctrl Pts',(-252.310585634382,4.09916130974965,
126.141503726722));
#277406=CARTESIAN_POINT('Ctrl Pts',(-252.589033258195,-1.70729674574642,
124.835232067896));
#277407=CARTESIAN_POINT('Ctrl Pts',(-252.867480882007,-5.94483249743877,
129.014297936587));
#277408=CARTESIAN_POINT('Ctrl Pts',(-253.14592850582,-4.71935760622846,
134.838343962485));
#277409=CARTESIAN_POINT('Ctrl Pts',(-253.424376129633,0.842976373616159,
136.955356360136));
#277410=CARTESIAN_POINT('Ctrl Pts',(-253.702823753446,5.63065624411703,
133.419904173236));
#277411=CARTESIAN_POINT('Ctrl Pts',(-253.981271377259,5.24403810606461,
127.480895216153));
#277412=CARTESIAN_POINT('Ctrl Pts',(-254.259719001072,0.0384051209378723,
124.595988638398));
#277413=CARTESIAN_POINT('Ctrl Pts',(-254.538166624885,-5.20252026939218,
127.416272546179));
#277414=CARTESIAN_POINT('Ctrl Pts',(-254.816614248698,-5.66258373611722,
133.350044001689));
#277415=CARTESIAN_POINT('Ctrl Pts',(-255.095061872511,-0.919009293725241,
136.944456550123));
#277416=CARTESIAN_POINT('Ctrl Pts',(-255.373509496324,4.6690896269236,134.896421351226));
#277417=CARTESIAN_POINT('Ctrl Pts',(-255.651957120136,5.96652359266914,
129.087981388513));
#277418=CARTESIAN_POINT('Ctrl Pts',(-255.93040474395,1.78101326373629,124.856811707331));
#277419=CARTESIAN_POINT('Ctrl Pts',(-256.208852367762,-4.04116012583712,
126.091145862189));
#277420=CARTESIAN_POINT('Ctrl Pts',(-256.487299991575,-6.14970689884083,
131.656699899059));
#277421=CARTESIAN_POINT('Ctrl Pts',(-256.765747615388,-2.60696946356087,
136.438984870644));
#277422=CARTESIAN_POINT('Ctrl Pts',(-257.044195239201,3.33143800190474,
136.043346010603));
#277423=CARTESIAN_POINT('Ctrl Pts',(-257.322642863014,6.2084309480058,130.833296634437));
#277424=CARTESIAN_POINT('Ctrl Pts',(-257.601090486826,3.38015223603414,
125.596729883064));
#277425=CARTESIAN_POINT('Ctrl Pts',(-257.87953811064,-2.5542704291637,125.145582755354));
#277426=CARTESIAN_POINT('Ctrl Pts',(-258.157985734452,-6.14153931545366,
129.894837769574));
#277427=CARTESIAN_POINT('Ctrl Pts',(-258.436433358265,-4.08485240479644,
135.479405634932));
#277428=CARTESIAN_POINT('Ctrl Pts',(-258.714880982078,1.72527217059264,
136.768768758555));
#277429=CARTESIAN_POINT('Ctrl Pts',(-258.993328605892,5.95060195420752,
132.575369498931));
#277430=CARTESIAN_POINT('Ctrl Pts',(-259.271776229703,4.70639920604184,
126.75783223591));
#277431=CARTESIAN_POINT('Ctrl Pts',(-259.550223853517,-0.860449444711704,
124.652528659269));
#277432=CARTESIAN_POINT('Ctrl Pts',(-259.82867147733,-5.64095031490746,
128.212697490595));
#277433=CARTESIAN_POINT('Ctrl Pts',(-260.060711163841,-5.29799179572588,
133.142936715762));
#277434=CARTESIAN_POINT('Ctrl Pts',(-260.246372125917,-2.62679689981868,
135.594171577488));
#277435=CARTESIAN_POINT('Ctrl Pts',(-260.339217213388,-0.889986900407246,
136.05080276614));
#277436=CARTESIAN_POINT('Ctrl Pts',(-260.385654363559,-0.0148419801173944,
136.053268468065));
#277437=CARTESIAN_POINT('Ctrl Pts',(209.997106195361,2.85369542052185,134.803838223542));
#277438=CARTESIAN_POINT('Ctrl Pts',(209.950688331758,3.52024512455777,134.328247120061));
#277439=CARTESIAN_POINT('Ctrl Pts',(209.857862530854,4.598911638141,133.039517383424));
#277440=CARTESIAN_POINT('Ctrl Pts',(209.672220855345,5.31158968331849,129.722011776094));
#277441=CARTESIAN_POINT('Ctrl Pts',(209.440181168834,2.90445768035623,125.771581499823));
#277442=CARTESIAN_POINT('Ctrl Pts',(209.161733545021,-2.67328939945229,
125.640965885288));
#277443=CARTESIAN_POINT('Ctrl Pts',(208.883285921209,-5.78445646322271,
130.262241799363));
#277444=CARTESIAN_POINT('Ctrl Pts',(208.604838297395,-3.58517659481558,
135.378114005881));
#277445=CARTESIAN_POINT('Ctrl Pts',(208.326390673583,1.91144119617671,136.292814641374));
#277446=CARTESIAN_POINT('Ctrl Pts',(208.04794304977,5.65009034124608,132.162897902674));
#277447=CARTESIAN_POINT('Ctrl Pts',(207.769495425957,4.19734896093999,126.785079177362));
#277448=CARTESIAN_POINT('Ctrl Pts',(207.491047802144,-1.1129569716493,125.100504449821));
#277449=CARTESIAN_POINT('Ctrl Pts',(207.212600178331,-5.4002948496084,128.657642803108));
#277450=CARTESIAN_POINT('Ctrl Pts',(206.934152554519,-4.72513942780656,
134.187431620732));
#277451=CARTESIAN_POINT('Ctrl Pts',(206.655704930705,0.292248586550605,
136.608384944684));
#277452=CARTESIAN_POINT('Ctrl Pts',(206.377257306892,5.04104249491135,133.695701483205));
#277453=CARTESIAN_POINT('Ctrl Pts',(206.09880968308,5.15738153042831,128.12602865207));
#277454=CARTESIAN_POINT('Ctrl Pts',(205.820362059267,0.534329935251406,
125.017605890956));
#277455=CARTESIAN_POINT('Ctrl Pts',(205.541914435454,-4.57974002364783,
127.226931288585));
#277456=CARTESIAN_POINT('Ctrl Pts',(205.263466811641,-5.48525514562618,
132.723737743954));
#277457=CARTESIAN_POINT('Ctrl Pts',(204.985019187828,-1.35008742798131,
136.456731302353));
#277458=CARTESIAN_POINT('Ctrl Pts',(204.706571564015,4.02574397595362,134.995471850294));
#277459=CARTESIAN_POINT('Ctrl Pts',(204.428123940202,5.70211370766606,129.682786179275));
#277460=CARTESIAN_POINT('Ctrl Pts',(204.149676316389,2.13851930815143,125.40077248911));
#277461=CARTESIAN_POINT('Ctrl Pts',(203.871228692576,-3.39026975841633,
126.084392381055));
#277462=CARTESIAN_POINT('Ctrl Pts',(203.592781068764,-5.8035665963141,131.105432460946));
#277463=CARTESIAN_POINT('Ctrl Pts',(203.314333444951,-2.88366922283368,
135.849802245147));
#277464=CARTESIAN_POINT('Ctrl Pts',(203.035885821138,2.68617927581077,135.957657646429));
#277465=CARTESIAN_POINT('Ctrl Pts',(202.757438197325,5.78756025537181,131.329884836407));
#277466=CARTESIAN_POINT('Ctrl Pts',(202.478990573512,3.57045609392238,126.219180939555));
#277467=CARTESIAN_POINT('Ctrl Pts',(202.200542949699,-1.92772278905516,
125.322033169903));
#277468=CARTESIAN_POINT('Ctrl Pts',(201.922095325886,-5.6544186046078,129.462876497226));
#277469=CARTESIAN_POINT('Ctrl Pts',(201.643647702073,-4.18497995558374,
134.836478196445));
#277470=CARTESIAN_POINT('Ctrl Pts',(201.36520007826,1.13025082464198,136.504760820331));
#277471=CARTESIAN_POINT('Ctrl Pts',(201.086752454448,5.4068363130258,132.934654138033));
#277472=CARTESIAN_POINT('Ctrl Pts',(200.808304830635,4.71480336828096,127.406911780982));
#277473=CARTESIAN_POINT('Ctrl Pts',(200.529857206822,-0.309903540913717,
125.001258930184));
#277474=CARTESIAN_POINT('Ctrl Pts',(200.251409583008,-5.04982423566531,
127.928373032793));
#277475=CARTESIAN_POINT('Ctrl Pts',(199.972961959197,-5.14920315545485,
133.498379226012));
#277476=CARTESIAN_POINT('Ctrl Pts',(199.694514335383,-0.516715927947778,
136.59271392819));
#277477=CARTESIAN_POINT('Ctrl Pts',(199.416066711571,4.59060799437092,134.367834714685));
#277478=CARTESIAN_POINT('Ctrl Pts',(199.137619087757,5.47938743352869,128.868296891315));
#277479=CARTESIAN_POINT('Ctrl Pts',(198.859171463945,1.33287750423228,125.147907050397));
#277480=CARTESIAN_POINT('Ctrl Pts',(198.580723840131,-4.03848173676817,
126.625521704588));
#277481=CARTESIAN_POINT('Ctrl Pts',(198.302276216319,-5.69867355247927,
131.943285172176));
#277482=CARTESIAN_POINT('Ctrl Pts',(198.023828592506,-2.12206276914206,
136.214432613634));
#277483=CARTESIAN_POINT('Ctrl Pts',(197.745380968693,3.4046200305072,135.513988187415));
#277484=CARTESIAN_POINT('Ctrl Pts',(197.46693334488,5.80262334705539,130.485626102603));
#277485=CARTESIAN_POINT('Ctrl Pts',(197.188485721067,2.86829928156946,125.750165465994));
#277486=CARTESIAN_POINT('Ctrl Pts',(196.910038097254,-2.70185169946893,
125.65926326252));
#277487=CARTESIAN_POINT('Ctrl Pts',(196.631590473441,-5.78913296148881,
130.296454176353));
#277488=CARTESIAN_POINT('Ctrl Pts',(196.353142849628,-3.5564838467683,135.400386297052));
#277489=CARTESIAN_POINT('Ctrl Pts',(196.074695225815,1.94440017923737,136.280795346639));
#277490=CARTESIAN_POINT('Ctrl Pts',(195.796247602003,5.6584754297534,132.128628418917));
#277491=CARTESIAN_POINT('Ctrl Pts',(195.51779997819,4.17268819221861,126.759524075833));
#277492=CARTESIAN_POINT('Ctrl Pts',(195.239352354377,-1.14759564681435,
125.107426913349));
#277493=CARTESIAN_POINT('Ctrl Pts',(194.960904730564,-5.41329514958902,
128.690533514357));
#277494=CARTESIAN_POINT('Ctrl Pts',(194.682457106751,-4.70444086406131,
134.216143957018));
#277495=CARTESIAN_POINT('Ctrl Pts',(194.404009482938,0.327564750825761,
136.606492185605));
#277496=CARTESIAN_POINT('Ctrl Pts',(194.125561859125,5.0585543621317,133.664964953048));
#277497=CARTESIAN_POINT('Ctrl Pts',(193.847114235312,5.14097963875765,128.094682084473));
#277498=CARTESIAN_POINT('Ctrl Pts',(193.568666611499,0.499095778182989,
125.014461412655));
#277499=CARTESIAN_POINT('Ctrl Pts',(193.290218987687,-4.60143272035756,
127.254875257849));
#277500=CARTESIAN_POINT('Ctrl Pts',(193.011771363874,-5.4734693413749,132.757092746623));
#277501=CARTESIAN_POINT('Ctrl Pts',(192.733323740061,-1.31565503151135,
136.464844805061));
#277502=CARTESIAN_POINT('Ctrl Pts',(192.454876116248,4.05118197898966,134.970888425217));
#277503=CARTESIAN_POINT('Ctrl Pts',(192.176428492435,5.69518066204141,129.648096536341));
#277504=CARTESIAN_POINT('Ctrl Pts',(191.897980868622,2.1055865417199,125.38785485147));
#277505=CARTESIAN_POINT('Ctrl Pts',(191.619533244809,-3.4189387468211,126.105117354624));
#277506=CARTESIAN_POINT('Ctrl Pts',(191.341085620997,-5.80162635147675,
131.140754845624));
#277507=CARTESIAN_POINT('Ctrl Pts',(191.062637997183,-2.85290276432908,
135.867262474811));
#277508=CARTESIAN_POINT('Ctrl Pts',(190.784190373371,2.71749909118881,135.941210633695));
#277509=CARTESIAN_POINT('Ctrl Pts',(190.505742749557,5.79065203911519,131.29464457683));
#277510=CARTESIAN_POINT('Ctrl Pts',(190.227295125745,3.54247865217362,126.197531513104));
#277511=CARTESIAN_POINT('Ctrl Pts',(189.948847501932,-1.96105955641241,
125.333869340265));
#277512=CARTESIAN_POINT('Ctrl Pts',(189.670399878119,-5.66247983574075,
129.497321402909));
#277513=CARTESIAN_POINT('Ctrl Pts',(189.391952254306,-4.160357773542,134.861878651407));
#277514=CARTESIAN_POINT('Ctrl Pts',(189.113504630493,1.16492983776554,136.497775047581));
#277515=CARTESIAN_POINT('Ctrl Pts',(188.83505700668,5.41970383815296,132.901701721328));
#277516=CARTESIAN_POINT('Ctrl Pts',(188.556609382867,4.69403477852959,127.378274381527));
#277517=CARTESIAN_POINT('Ctrl Pts',(188.278161759054,-0.345222926215044,
125.003252919028));
#277518=CARTESIAN_POINT('Ctrl Pts',(187.999714135242,-5.0672376268456,127.959166031618));
#277519=CARTESIAN_POINT('Ctrl Pts',(187.721266511429,-5.13270849672517,
133.529673973213));
#277520=CARTESIAN_POINT('Ctrl Pts',(187.442818887616,-0.48147100486422,
136.595752079925));
#277521=CARTESIAN_POINT('Ctrl Pts',(187.164371263803,4.61221481930072,134.339824357932));
#277522=CARTESIAN_POINT('Ctrl Pts',(186.88592363999,5.4675005437485,128.834978175547));
#277523=CARTESIAN_POINT('Ctrl Pts',(186.607476016177,1.29842037074208,125.139898247696));
#277524=CARTESIAN_POINT('Ctrl Pts',(186.329028392364,-4.06384469161484,
126.650182513385));
#277525=CARTESIAN_POINT('Ctrl Pts',(186.050580768551,-5.69163501222784,
131.977953513933));
#277526=CARTESIAN_POINT('Ctrl Pts',(185.772133144738,-2.08909080843167,
136.227249975919));
#277527=CARTESIAN_POINT('Ctrl Pts',(185.493685520926,3.4332257905535,135.493176040453));
#277528=CARTESIAN_POINT('Ctrl Pts',(185.215237897112,5.80057561042411,130.450309792719));
#277529=CARTESIAN_POINT('Ctrl Pts',(184.9367902733,2.83747981818726,125.732798956676));
#277530=CARTESIAN_POINT('Ctrl Pts',(184.658342649487,-2.73312130836828,
125.675805527429));
#277531=CARTESIAN_POINT('Ctrl Pts',(184.379895025674,-5.79211747293216,
130.331703682172));
#277532=CARTESIAN_POINT('Ctrl Pts',(184.101447401861,-3.52844064054064,
135.421950469967));
#277533=CARTESIAN_POINT('Ctrl Pts',(183.822999778048,1.97770076659953,136.26885776521));
#277534=CARTESIAN_POINT('Ctrl Pts',(183.544552154236,5.66643178528845,132.094159137294));
#277535=CARTESIAN_POINT('Ctrl Pts',(183.266104530422,4.14798881387936,126.734198679909));
#277536=CARTESIAN_POINT('Ctrl Pts',(182.98765690661,-1.18225323696583,125.114518204765));
#277537=CARTESIAN_POINT('Ctrl Pts',(182.709209282797,-5.42606231932092,
128.72352494273));
#277538=CARTESIAN_POINT('Ctrl Pts',(182.430761658984,-4.68358520810093,
134.244718011395));
#277539=CARTESIAN_POINT('Ctrl Pts',(182.152314035171,0.362877903506298,
136.604390705933));
#277540=CARTESIAN_POINT('Ctrl Pts',(181.873866411358,5.07587394936235,133.634119096483));
#277541=CARTESIAN_POINT('Ctrl Pts',(181.595418787545,5.12438980598236,128.063437686296));
#277542=CARTESIAN_POINT('Ctrl Pts',(181.316971163732,0.463841771263853,
125.011530548415));
#277543=CARTESIAN_POINT('Ctrl Pts',(181.038523539919,-4.62295419131585,
127.282951248603));
#277544=CARTESIAN_POINT('Ctrl Pts',(180.760075916106,-5.46148109594396,
132.790375128456));
#277545=CARTESIAN_POINT('Ctrl Pts',(180.481628292294,-1.2811736815839,136.472748695004));
#277546=CARTESIAN_POINT('Ctrl Pts',(180.203180668481,4.07646975733793,134.946150534538));
#277547=CARTESIAN_POINT('Ctrl Pts',(179.924733044668,5.68803663588505,129.61344977806));
#277548=CARTESIAN_POINT('Ctrl Pts',(179.646285420855,2.07257572209157,125.37513790386));
#277549=CARTESIAN_POINT('Ctrl Pts',(179.367837797042,-3.44748102935117,
126.12601647128));
#277550=CARTESIAN_POINT('Ctrl Pts',(179.089390173229,-5.79947113363144,
131.176064759319));
#277551=CARTESIAN_POINT('Ctrl Pts',(178.810942549416,-2.82203058602,135.884535099843));
#277552=CARTESIAN_POINT('Ctrl Pts',(178.532494925603,2.74871820628535,135.924573271475));
#277553=CARTESIAN_POINT('Ctrl Pts',(178.254047301791,5.79352924936408,131.259386150458));
#277554=CARTESIAN_POINT('Ctrl Pts',(177.975599677977,3.51436994191561,126.176052793945));
#277555=CARTESIAN_POINT('Ctrl Pts',(177.697152054165,-1.99432365563702,
125.345908221933));
#277556=CARTESIAN_POINT('Ctrl Pts',(177.418704430351,-5.6703312417861,129.531814741282));
#277557=CARTESIAN_POINT('Ctrl Pts',(177.140256806539,-4.135581427815,134.887128753614));
#277558=CARTESIAN_POINT('Ctrl Pts',(176.861809182726,1.19956568393359,136.490578303229));
#277559=CARTESIAN_POINT('Ctrl Pts',(176.583361558913,5.43237053418876,132.868671586896));
#277560=CARTESIAN_POINT('Ctrl Pts',(176.3049139351,4.67309224957875,127.349763936946));
#277561=CARTESIAN_POINT('Ctrl Pts',(176.026466311287,-0.380529519146142,
125.005461870054));
#277562=CARTESIAN_POINT('Ctrl Pts',(175.748018687475,-5.08446324967622,
127.990064460173));
#277563=CARTESIAN_POINT('Ctrl Pts',(175.469571063661,-5.11602364359241,
133.560867732924));
#277564=CARTESIAN_POINT('Ctrl Pts',(175.191123439849,-0.446208240696769,
136.59857562952));
#277565=CARTESIAN_POINT('Ctrl Pts',(174.912675816035,4.63365073691483,134.311682993269));
#277566=CARTESIAN_POINT('Ctrl Pts',(174.634228192223,5.45541105372469,128.801732435971));
#277567=CARTESIAN_POINT('Ctrl Pts',(174.35578056841,1.26391512380778,125.132099343732));
#277568=CARTESIAN_POINT('Ctrl Pts',(174.077332944597,-4.089057059202,126.674997256779));
#277569=CARTESIAN_POINT('Ctrl Pts',(173.798885320784,-5.68438556634791,
132.012578367773));
#277570=CARTESIAN_POINT('Ctrl Pts',(173.520437696972,-2.0560414356932,136.239866391045));
#277571=CARTESIAN_POINT('Ctrl Pts',(173.241990073158,3.46170433115548,135.472190147709));
#277572=CARTESIAN_POINT('Ctrl Pts',(172.963542449346,5.79831293133042,130.41500660232));
#277573=CARTESIAN_POINT('Ctrl Pts',(172.685094825533,2.80655521094699,125.715620375941));
#277574=CARTESIAN_POINT('Ctrl Pts',(172.40664720172,-2.76428964045241,125.692537832834));
#277575=CARTESIAN_POINT('Ctrl Pts',(172.128199577907,-5.79488735533246,
130.366970702468));
#277576=CARTESIAN_POINT('Ctrl Pts',(171.849751954094,-3.50026668664755,
135.443343536393));
#277577=CARTESIAN_POINT('Ctrl Pts',(171.571304330281,2.01092806953244,136.256717694829));
#277578=CARTESIAN_POINT('Ctrl Pts',(171.292856706468,5.6741781691098,132.059642061713));
#277579=CARTESIAN_POINT('Ctrl Pts',(171.014409082656,4.12313573028927,126.709024105332));
#277580=CARTESIAN_POINT('Ctrl Pts',(170.735961458842,-1.21686701828875,
125.121820335384));
#277581=CARTESIAN_POINT('Ctrl Pts',(170.45751383503,-5.43862842431808,128.756593477234));
#277582=CARTESIAN_POINT('Ctrl Pts',(170.179066211217,-4.66255600016836,
134.273164582064));
#277583=CARTESIAN_POINT('Ctrl Pts',(169.900618587404,0.398177609612544,
136.602074304013));
#277584=CARTESIAN_POINT('Ctrl Pts',(169.62217096359,5.09300544821711,133.603168382178));
#277585=CARTESIAN_POINT('Ctrl Pts',(169.343723339778,5.10761008705837,128.032294854024));
#277586=CARTESIAN_POINT('Ctrl Pts',(169.065275715965,0.428570576517446,
125.008814339624));
#277587=CARTESIAN_POINT('Ctrl Pts',(168.786828092152,-4.64430435700642,
127.311157726477));
#277588=CARTESIAN_POINT('Ctrl Pts',(168.508380468339,-5.4492904733226,132.823583917792));
#277589=CARTESIAN_POINT('Ctrl Pts',(168.229932844526,-1.24664485729461,
136.480442540741));
#277590=CARTESIAN_POINT('Ctrl Pts',(167.951485220714,4.10160648060013,134.92125916831));
#277591=CARTESIAN_POINT('Ctrl Pts',(167.673037596901,5.6806818374394,129.578847149419));
#277592=CARTESIAN_POINT('Ctrl Pts',(167.394589973088,2.03948810240773,125.362622138095));
#277593=CARTESIAN_POINT('Ctrl Pts',(167.116142349275,-3.47589556420378,
126.147088945699));
#277594=CARTESIAN_POINT('Ctrl Pts',(166.837694725462,-5.79710101425052,
131.21136089938));
#277595=CARTESIAN_POINT('Ctrl Pts',(166.559247101649,-2.79105383632985,
135.901619477142));
#277596=CARTESIAN_POINT('Ctrl Pts',(166.280799477836,2.77983546661788,135.907746177893));
#277597=CARTESIAN_POINT('Ctrl Pts',(166.002351854023,5.79619177825601,131.224110862948));
#277598=CARTESIAN_POINT('Ctrl Pts',(165.72390423021,3.48613100538707,126.154745578436));
#277599=CARTESIAN_POINT('Ctrl Pts',(165.445456606397,-2.02751385446508,
125.358149368562));
#277600=CARTESIAN_POINT('Ctrl Pts',(165.167008982585,-5.67797253162207,
129.566355234311));
#277601=CARTESIAN_POINT('Ctrl Pts',(164.888561358772,-4.11065183659732,
134.912227567346));
#277602=CARTESIAN_POINT('Ctrl Pts',(164.610113734959,1.23415707975413,136.483170853989));
#277603=CARTESIAN_POINT('Ctrl Pts',(164.331666111146,5.44483593173667,132.835564958663));
#277604=CARTESIAN_POINT('Ctrl Pts',(164.053218487333,4.65197655747607,127.321381503715));
#277605=CARTESIAN_POINT('Ctrl Pts',(163.77477086352,-0.415822011415935,
125.007885701408));
#277606=CARTESIAN_POINT('Ctrl Pts',(163.496323239708,-5.10150046585131,
128.021067173507));
#277607=CARTESIAN_POINT('Ctrl Pts',(163.217875615894,-5.09914921432216,
133.591959349252));
#277608=CARTESIAN_POINT('Ctrl Pts',(162.939427992082,-0.41092894211879,
136.601184472346));
#277609=CARTESIAN_POINT('Ctrl Pts',(162.660980368268,4.65491495289691,134.283411663486));
#277610=CARTESIAN_POINT('Ctrl Pts',(162.382532744456,5.443119411438,128.768560904517));
#277611=CARTESIAN_POINT('Ctrl Pts',(162.104085120643,1.22936304203373,125.124510627495));
#277612=CARTESIAN_POINT('Ctrl Pts',(161.82563749683,-4.11411790527609,126.69996501525));
#277613=CARTESIAN_POINT('Ctrl Pts',(161.547189873017,-5.67692548347038,
132.04715845066));
#277614=CARTESIAN_POINT('Ctrl Pts',(161.268742249204,-2.02291587558315,
136.252281391507));
#277615=CARTESIAN_POINT('Ctrl Pts',(160.990294625391,3.49005459703047,135.451031286826));
#277616=CARTESIAN_POINT('Ctrl Pts',(160.711847001578,5.79583539361873,130.379717839577));
#277617=CARTESIAN_POINT('Ctrl Pts',(160.433399377766,2.77552660577121,125.698630360346));
#277618=CARTESIAN_POINT('Ctrl Pts',(160.154951753952,-2.79535554076737,
125.70945955871));
#277619=CARTESIAN_POINT('Ctrl Pts',(159.87650413014,-5.79744250605075,130.402253930408));
#277620=CARTESIAN_POINT('Ctrl Pts',(159.598056506327,-3.47196302908515,
135.4645647036));
#277621=CARTESIAN_POINT('Ctrl Pts',(159.319608882514,2.04408085678626,136.244375585352));
#277622=CARTESIAN_POINT('Ctrl Pts',(159.041161258701,5.68171429417248,132.025078471215));
#277623=CARTESIAN_POINT('Ctrl Pts',(158.762713634888,4.09812986238831,126.684001284956));
#277624=CARTESIAN_POINT('Ctrl Pts',(158.484266011075,-1.25143570815684,
125.129333034622));
#277625=CARTESIAN_POINT('Ctrl Pts',(158.205818387262,-5.450992998939,128.789737892503));
#277626=CARTESIAN_POINT('Ctrl Pts',(157.927370763449,-4.64135401950845,
134.301482614925));
#277627=CARTESIAN_POINT('Ctrl Pts',(157.648923139637,0.43346256110109,136.59954306568));
#277628=CARTESIAN_POINT('Ctrl Pts',(157.370475515823,5.10994822388206,133.572113957021));
#277629=CARTESIAN_POINT('Ctrl Pts',(157.092027892011,5.09064110376424,128.001254741669));
#277630=CARTESIAN_POINT('Ctrl Pts',(156.813580268198,0.39328350093061,125.006312886931));
#277631=CARTESIAN_POINT('Ctrl Pts',(156.535132644385,-4.66548242629113,
127.339493646268));
#277632=CARTESIAN_POINT('Ctrl Pts',(156.256685020572,-5.43689792523874,
132.856717884066));
#277633=CARTESIAN_POINT('Ctrl Pts',(155.978237396759,-1.21206983812162,
136.487926057176));
#277634=CARTESIAN_POINT('Ctrl Pts',(155.699789772946,4.12659121732586,134.896215248893));
#277635=CARTESIAN_POINT('Ctrl Pts',(155.421342149133,5.67311653923917,129.544289932631));
#277636=CARTESIAN_POINT('Ctrl Pts',(155.142894525321,2.0063249087422,125.350308017949));
#277637=CARTESIAN_POINT('Ctrl Pts',(154.864446901507,-3.50418129846815,
126.168333997033));
#277638=CARTESIAN_POINT('Ctrl Pts',(154.585999277695,-5.79451608115961,
131.246641957895));
#277639=CARTESIAN_POINT('Ctrl Pts',(154.307551653882,-2.75997366311328,
135.918514973638));
#277640=CARTESIAN_POINT('Ctrl Pts',(154.029104030069,2.81084971912495,135.890729976482));
#277641=CARTESIAN_POINT('Ctrl Pts',(153.750656406256,5.79863952713012,131.188820021437));
#277642=CARTESIAN_POINT('Ctrl Pts',(153.472208782443,3.457762888992,126.133610656121));
#277643=CARTESIAN_POINT('Ctrl Pts',(153.19376115863,-2.0606289230217,125.370592326552));
#277644=CARTESIAN_POINT('Ctrl Pts',(152.915313534817,-5.68540342209783,
129.600941602086));
#277645=CARTESIAN_POINT('Ctrl Pts',(152.636865911004,-4.08556992366409,
134.937174162558));
#277646=CARTESIAN_POINT('Ctrl Pts',(152.358418287191,1.26870274343019,136.475552974349));
#277647=CARTESIAN_POINT('Ctrl Pts',(152.079970663379,5.45709956888678,132.802383063404));
#277648=CARTESIAN_POINT('Ctrl Pts',(151.801523039566,4.63068848467127,127.293128133558));
#277649=CARTESIAN_POINT('Ctrl Pts',(151.523075415753,-0.451099095248245,
125.010524323271));
#277650=CARTESIAN_POINT('Ctrl Pts',(151.24462779194,-5.11834864405056,128.052173022803));
#277651=CARTESIAN_POINT('Ctrl Pts',(150.966180168127,-5.08208583420252,
133.622947670083));
#277652=CARTESIAN_POINT('Ctrl Pts',(150.687732544314,-0.375634416417742,
136.603578511732));
#277653=CARTESIAN_POINT('Ctrl Pts',(150.409284920501,4.67600667929353,134.255011416186));
#277654=CARTESIAN_POINT('Ctrl Pts',(150.130837296688,5.43062607235983,128.735464810371));
#277655=CARTESIAN_POINT('Ctrl Pts',(149.852389672876,1.19476540576009,125.117132380189));
#277656=CARTESIAN_POINT('Ctrl Pts',(149.573942049063,-4.13902630119825,
126.725084863609));
#277657=CARTESIAN_POINT('Ctrl Pts',(149.29549442525,-5.66925504003138,132.081692481218));
#277658=CARTESIAN_POINT('Ctrl Pts',(149.017046801437,-1.98971535558138,
136.264494517259));
#277659=CARTESIAN_POINT('Ctrl Pts',(148.738599177624,3.5182755376489,135.429700241853));
#277660=CARTESIAN_POINT('Ctrl Pts',(148.460151553811,5.79314308909515,130.344444812129));
#277661=CARTESIAN_POINT('Ctrl Pts',(148.181703929998,2.74439515243632,125.681829539465));
#277662=CARTESIAN_POINT('Ctrl Pts',(147.903256306185,-2.82631785815477,
125.726570078021));
#277663=CARTESIAN_POINT('Ctrl Pts',(147.624808682372,-5.79978283040501,
130.437552058559));
#277664=CARTESIAN_POINT('Ctrl Pts',(147.346361058559,-3.4435307166558,135.48561318523));
#277665=CARTESIAN_POINT('Ctrl Pts',(147.067913434747,2.07715789987228,136.23183189412));
#277666=CARTESIAN_POINT('Ctrl Pts',(146.789465810933,5.68903988122249,131.990469646568));
#277667=CARTESIAN_POINT('Ctrl Pts',(146.511018187121,4.07297213677825,126.65913114601));
#277668=CARTESIAN_POINT('Ctrl Pts',(146.232570563308,-1.2859580256146,125.137056024094));
#277669=CARTESIAN_POINT('Ctrl Pts',(145.954122939495,-5.46315558500969,
128.822956960357));
#277670=CARTESIAN_POINT('Ctrl Pts',(145.675675315682,-4.61998005176852,
134.329671060644));
#277671=CARTESIAN_POINT('Ctrl Pts',(145.397227691869,0.468731450475054,
136.596797084732));
#277672=CARTESIAN_POINT('Ctrl Pts',(145.118780068056,5.12670164853643,133.540956971746));
#277673=CARTESIAN_POINT('Ctrl Pts',(144.840332444244,5.07348348489189,127.970318499433));
#277674=CARTESIAN_POINT('Ctrl Pts',(144.56188482043,0.357981852079004,125.004026283029));
#277675=CARTESIAN_POINT('Ctrl Pts',(144.283437196618,-4.6864876144088,127.367957957979));
#277676=CARTESIAN_POINT('Ctrl Pts',(144.004989572805,-5.42430391090288,
132.889775799486));
#277677=CARTESIAN_POINT('Ctrl Pts',(143.726541948992,-1.17744990525502,
136.495198967004));
#277678=CARTESIAN_POINT('Ctrl Pts',(143.448094325179,4.15142304169647,134.871019704297));
#277679=CARTESIAN_POINT('Ctrl Pts',(143.169646701366,5.66534102161933,129.509779408224));
#277680=CARTESIAN_POINT('Ctrl Pts',(142.891199077553,1.9730873699693,125.338195999729));
#277681=CARTESIAN_POINT('Ctrl Pts',(142.61275145374,-3.53233718400576,126.189750838038));
#277682=CARTESIAN_POINT('Ctrl Pts',(142.334303829928,-5.79171643014443,
131.281906627513));
#277683=CARTESIAN_POINT('Ctrl Pts',(142.055856206114,-2.72879121805762,
135.935220963265));
#277684=CARTESIAN_POINT('Ctrl Pts',(141.777408582302,2.84175981456215,135.873525297782));
#277685=CARTESIAN_POINT('Ctrl Pts',(141.498960958489,5.80087240528401,131.153514933643));
#277686=CARTESIAN_POINT('Ctrl Pts',(141.220513334676,3.42926664392146,126.112648810165));
#277687=CARTESIAN_POINT('Ctrl Pts',(140.942065710863,-2.09366763421581,
125.383236634823));
#277688=CARTESIAN_POINT('Ctrl Pts',(140.66361808705,-5.69262363785895,129.635572562993));
#277689=CARTESIAN_POINT('Ctrl Pts',(140.385170463237,-4.06033661843482,
134.961967614844));
#277690=CARTESIAN_POINT('Ctrl Pts',(140.106722839424,1.30320139485961,136.467724946589));
#277691=CARTESIAN_POINT('Ctrl Pts',(139.828275215611,5.46916099120554,132.769127130691));
#277692=CARTESIAN_POINT('Ctrl Pts',(139.549827591798,4.60922882000175,127.26500487341));
#277693=CARTESIAN_POINT('Ctrl Pts',(139.271379967986,-0.486359463437733,
125.013377637868));
#277694=CARTESIAN_POINT('Ctrl Pts',(138.992932344173,-5.13500715995863,
128.083380855422));
#277695=CARTESIAN_POINT('Ctrl Pts',(138.71448472036,-5.06483413552331,133.653831547135));
#277696=CARTESIAN_POINT('Ctrl Pts',(138.436037096547,-0.340325971445257,
136.605757658967));
#277697=CARTESIAN_POINT('Ctrl Pts',(138.157589472734,4.69692513454305,134.226483303753));
#277698=CARTESIAN_POINT('Ctrl Pts',(137.879141848921,5.41793149943546,128.70244537992));
#277699=CARTESIAN_POINT('Ctrl Pts',(137.600694225109,1.16012349701482,125.109964875215));
#277700=CARTESIAN_POINT('Ctrl Pts',(137.322246601295,-4.16378132397874,
126.750355871033));
#277701=CARTESIAN_POINT('Ctrl Pts',(137.043798977483,-5.66137452026194,
132.116179179772));
#277702=CARTESIAN_POINT('Ctrl Pts',(136.765351353669,-1.95644110594549,
136.276505315742));
#277703=CARTESIAN_POINT('Ctrl Pts',(136.486903729857,3.54636610727348,135.408197803219));
#277704=CARTESIAN_POINT('Ctrl Pts',(136.208456106044,5.79023611752392,130.309188827029));
#277705=CARTESIAN_POINT('Ctrl Pts',(135.930008482231,2.71316200452982,125.665218535856));
#277706=CARTESIAN_POINT('Ctrl Pts',(135.651560858418,-2.85717544529452,
125.743868756725));
#277707=CARTESIAN_POINT('Ctrl Pts',(135.373113234605,-5.80190824167357,
130.472863778936));
#277708=CARTESIAN_POINT('Ctrl Pts',(135.094665610792,-3.41497080292952,
135.506488201326));
#277709=CARTESIAN_POINT('Ctrl Pts',(134.816217986979,2.11015797310843,136.219087085943));
#277710=CARTESIAN_POINT('Ctrl Pts',(134.537770363167,5.69615465880763,131.955816870215));
#277711=CARTESIAN_POINT('Ctrl Pts',(134.259322739353,4.04766348568775,126.634414610068));
#277712=CARTESIAN_POINT('Ctrl Pts',(133.980875115541,-1.32043269142476,
125.144989017623));
#277713=CARTESIAN_POINT('Ctrl Pts',(133.702427491728,-5.47511573184112,
128.856249449853));
#277714=CARTESIAN_POINT('Ctrl Pts',(133.423979867915,-4.59843488896879,
134.357728874689));
#277715=CARTESIAN_POINT('Ctrl Pts',(133.145532244102,0.503982970832797,
136.59383646292));
#277716=CARTESIAN_POINT('Ctrl Pts',(132.867084620289,5.14326510137581,133.509698580887));
#277717=CARTESIAN_POINT('Ctrl Pts',(132.588636996476,5.05613786622328,127.93948727367));
#277718=CARTESIAN_POINT('Ctrl Pts',(132.310189372663,0.322666938078297,
125.001954612649));
#277719=CARTESIAN_POINT('Ctrl Pts',(132.03174174885,-4.70731914300451,127.396549606854));
#277720=CARTESIAN_POINT('Ctrl Pts',(131.753294125038,-5.41150889699075,
132.92275643908));
#277721=CARTESIAN_POINT('Ctrl Pts',(131.474846501225,-1.14278634154918,
136.502261000723));
#277722=CARTESIAN_POINT('Ctrl Pts',(131.196398877412,4.17610103355955,134.845673468154));
#277723=CARTESIAN_POINT('Ctrl Pts',(130.917951253599,5.65735557270449,129.475316855001));
#277724=CARTESIAN_POINT('Ctrl Pts',(130.639503629786,1.93977671771839,125.326286532249));
#277725=CARTESIAN_POINT('Ctrl Pts',(130.361056005973,-3.56036217749005,
126.211338675105));
#277726=CARTESIAN_POINT('Ctrl Pts',(130.08260838216,-5.788702164947,131.317153601487));
#277727=CARTESIAN_POINT('Ctrl Pts',(129.804160758347,-2.69750765663984,
135.951736826975));
#277728=CARTESIAN_POINT('Ctrl Pts',(129.525713134534,2.87256460754407,135.856132779323));
#277729=CARTESIAN_POINT('Ctrl Pts',(129.247265510721,5.80289032997773,131.118196907806));
#277730=CARTESIAN_POINT('Ctrl Pts',(128.968817886909,3.40064332611445,126.091860817314));
#277731=CARTESIAN_POINT('Ctrl Pts',(128.690370263096,-2.12662876378584,
125.396081824838));
#277732=CARTESIAN_POINT('Ctrl Pts',(128.411922639283,-5.69963291135762,
129.670246833772));
#277733=CARTESIAN_POINT('Ctrl Pts',(128.13347501547,-4.03495285593914,134.986607005474));
#277734=CARTESIAN_POINT('Ctrl Pts',(127.855027391657,1.33765175568188,136.459687060782));
#277735=CARTESIAN_POINT('Ctrl Pts',(127.576579767844,5.48101975175251,132.73579839283));
#277736=CARTESIAN_POINT('Ctrl Pts',(127.298132144031,4.5875983586632,127.237012765392));
#277737=CARTESIAN_POINT('Ctrl Pts',(127.019684520218,-0.521601809398458,
125.016445539469));
#277738=CARTESIAN_POINT('Ctrl Pts',(126.741236896406,-5.15147539628782,
128.114689514947));
#277739=CARTESIAN_POINT('Ctrl Pts',(126.462789272592,-5.0473947575527,133.684609835992));
#277740=CARTESIAN_POINT('Ctrl Pts',(126.18434164878,-0.305004915568794,
136.607721833301));
#277741=CARTESIAN_POINT('Ctrl Pts',(125.905894024967,4.71766954350447,134.197828383304));
#277742=CARTESIAN_POINT('Ctrl Pts',(125.627446401154,5.40503616306688,128.669503836711));
#277743=CARTESIAN_POINT('Ctrl Pts',(125.348998777341,1.12543859946687,125.10300837817));
#277744=CARTESIAN_POINT('Ctrl Pts',(125.070551153528,-4.18838205631096,
126.775777101093));
#277745=CARTESIAN_POINT('Ctrl Pts',(124.792103529715,-5.65328421617778,
132.150617268407));
#277746=CARTESIAN_POINT('Ctrl Pts',(124.513655905902,-1.9230943596648,136.288313341892));
#277747=CARTESIAN_POINT('Ctrl Pts',(124.23520828209,3.57432526499779,135.386524767704));
#277748=CARTESIAN_POINT('Ctrl Pts',(123.956760658277,5.78711458662396,130.273951190703));
#277749=CARTESIAN_POINT('Ctrl Pts',(123.678313034464,2.68182831940755,125.648797965047));
#277750=CARTESIAN_POINT('Ctrl Pts',(123.399865410651,-2.88792715874745,
125.761354953818));
#277751=CARTESIAN_POINT('Ctrl Pts',(123.121417786838,-5.8038186610986,130.50818778305));
#277752=CARTESIAN_POINT('Ctrl Pts',(122.842970163025,-3.38628434620416,
135.527188978355));
#277753=CARTESIAN_POINT('Ctrl Pts',(122.564522539212,2.1430798536649,136.206141633086));
#277754=CARTESIAN_POINT('Ctrl Pts',(122.286074915399,5.703058363287,131.921121426228));
#277755=CARTESIAN_POINT('Ctrl Pts',(122.007627291586,4.02220484693838,126.609852593007));
#277756=CARTESIAN_POINT('Ctrl Pts',(121.729179667773,-1.35485842811595,
125.153131721247));
#277757=CARTESIAN_POINT('Ctrl Pts',(121.450732043961,-5.48687299624567,
128.889614127324));
#277758=CARTESIAN_POINT('Ctrl Pts',(121.172284420148,-4.57671932947311,
134.385655017367));
#277759=CARTESIAN_POINT('Ctrl Pts',(120.893836796335,0.539215815916097,
136.59066130995));
#277760=CARTESIAN_POINT('Ctrl Pts',(120.615389172522,5.15963796863542,133.478339942736));
#277761=CARTESIAN_POINT('Ctrl Pts',(120.336941548709,5.0386048905067,127.908762206842));
#277762=CARTESIAN_POINT('Ctrl Pts',(120.058493924896,0.287340067535411,
125.000097952557));
#277763=CARTESIAN_POINT('Ctrl Pts',(119.780046301083,-4.72797624015824,
127.42526753342));
#277764=CARTESIAN_POINT('Ctrl Pts',(119.50159867727,-5.39851335762638,132.955658580739));
#277765=CARTESIAN_POINT('Ctrl Pts',(119.223151053457,-1.10808043147514,
136.509111896649));
#277766=CARTESIAN_POINT('Ctrl Pts',(118.944703429644,4.20062427846316,134.820177479675));
#277767=CARTESIAN_POINT('Ctrl Pts',(118.666255805832,5.64916048839838,129.440903549983));
#277768=CARTESIAN_POINT('Ctrl Pts',(118.387808182019,1.90639418632776,125.314580056818));
#277769=CARTESIAN_POINT('Ctrl Pts',(118.109360558206,-3.58825524044456,
126.23309670829));
#277770=CARTESIAN_POINT('Ctrl Pts',(117.830912934393,-5.785473397262,131.352381573729));
#277771=CARTESIAN_POINT('Ctrl Pts',(117.55246531058,-2.66612413808396,135.968061952766));
#277772=CARTESIAN_POINT('Ctrl Pts',(117.274017686767,2.9032629565882,135.838553065588));
#277773=CARTESIAN_POINT('Ctrl Pts',(116.995570062954,5.80469322643624,131.082867252651));
#277774=CARTESIAN_POINT('Ctrl Pts',(116.717122439142,3.37189399621826,126.071247447876));
#277775=CARTESIAN_POINT('Ctrl Pts',(116.438674815328,-2.15951109034483,
125.409127420613));
#277776=CARTESIAN_POINT('Ctrl Pts',(116.160227191516,-5.70643098286277,
129.704963129555));
#277777=CARTESIAN_POINT('Ctrl Pts',(115.881779567703,-4.00941957678149,
135.011091421425));
#277778=CARTESIAN_POINT('Ctrl Pts',(115.60333194389,1.37205254932662,136.451439614773));
#277779=CARTESIAN_POINT('Ctrl Pts',(115.324884320077,5.49267541109693,132.702398084833));
#277780=CARTESIAN_POINT('Ctrl Pts',(115.046436696264,4.56579790218037,127.20915284676));
#277781=CARTESIAN_POINT('Ctrl Pts',(114.767989072451,-0.556824827212187,
125.019727914392));
#277782=CARTESIAN_POINT('Ctrl Pts',(114.489541448638,-5.1677527428018,128.146097841224));
#277783=CARTESIAN_POINT('Ctrl Pts',(114.211093824825,-5.02976834651319,
133.715281396157));
#277784=CARTESIAN_POINT('Ctrl Pts',(113.932646201012,-0.269672557622912,
136.60947096195));
#277785=CARTESIAN_POINT('Ctrl Pts',(113.6541985772,4.73823913748602,134.169047716661));
#277786=CARTESIAN_POINT('Ctrl Pts',(113.375750953387,5.39194054109557,128.636641401405));
#277787=CARTESIAN_POINT('Ctrl Pts',(113.097303329574,1.09071199837779,125.09626314683));
#277788=CARTESIAN_POINT('Ctrl Pts',(112.818855705761,-4.21282758660586,
126.801347611796));
#277789=CARTESIAN_POINT('Ctrl Pts',(112.540408081948,-5.64498442756793,
132.185005471008));
#277790=CARTESIAN_POINT('Ctrl Pts',(112.261960458135,-1.8896763524154,136.299918158156));
#277791=CARTESIAN_POINT('Ctrl Pts',(111.983512834322,3.60215197478495,135.364681938413));
#277792=CARTESIAN_POINT('Ctrl Pts',(111.705065210509,5.78377861206482,130.238733208892));
#277793=CARTESIAN_POINT('Ctrl Pts',(111.426617586696,2.65039525815055,125.632568435507));
#277794=CARTESIAN_POINT('Ctrl Pts',(111.148169962883,-2.91857185899754,
125.77902802134));
#277795=CARTESIAN_POINT('Ctrl Pts',(110.869722339071,-5.80551401788879,
130.543522761958));
#277796=CARTESIAN_POINT('Ctrl Pts',(110.591274715258,-3.35747240946702,
135.547714749242));
#277797=CARTESIAN_POINT('Ctrl Pts',(110.312827091445,2.17592232160915,136.192996015246));
#277798=CARTESIAN_POINT('Ctrl Pts',(110.034379467632,5.70975073884148,131.886384600257));
#277799=CARTESIAN_POINT('Ctrl Pts',(109.755931843819,3.99659716390926,126.585446004984));
#277800=CARTESIAN_POINT('Ctrl Pts',(109.477484220006,-1.38923396002991,
125.161483833236));
#277801=CARTESIAN_POINT('Ctrl Pts',(109.199036596193,-5.49842694255352,
128.923049756431));
#277802=CARTESIAN_POINT('Ctrl Pts',(108.92058897238,-4.55483417795961,134.413448453863));
#277803=CARTESIAN_POINT('Ctrl Pts',(108.642141348568,0.57442868015902,136.58727174348));
#277804=CARTESIAN_POINT('Ctrl Pts',(108.363693724754,5.17581964361271,133.446882219296));
#277805=CARTESIAN_POINT('Ctrl Pts',(108.085246100942,5.02088520743284,127.878144437479));
#277806=CARTESIAN_POINT('Ctrl Pts',(107.806798477129,0.252002549500665,
124.998456371553));
#277807=CARTESIAN_POINT('Ctrl Pts',(107.528350853316,-4.74845814041369,
127.454110673523));
#277808=CARTESIAN_POINT('Ctrl Pts',(107.249903229503,-5.38531777436419,
132.988481005259));
#277809=CARTESIAN_POINT('Ctrl Pts',(106.97145560569,-1.07333346107335,136.515751400918));
#277810=CARTESIAN_POINT('Ctrl Pts',(106.693007981877,4.22499186768932,134.794532683627));
#277811=CARTESIAN_POINT('Ctrl Pts',(106.414560358064,5.64075607237289,129.406540768369));
#277812=CARTESIAN_POINT('Ctrl Pts',(106.136112734251,1.87294101279944,125.303077007226));
#277813=CARTESIAN_POINT('Ctrl Pts',(105.857665110439,-3.61601533928142,
126.25502413134));
#277814=CARTESIAN_POINT('Ctrl Pts',(105.579217486626,-5.78203024673271,
131.387589238853));
#277815=CARTESIAN_POINT('Ctrl Pts',(105.300769862813,-2.63464182531766,
135.984195735705));
#277816=CARTESIAN_POINT('Ctrl Pts',(105.022322239,2.93385372415587,135.820786808));
#277817=CARTESIAN_POINT('Ctrl Pts',(104.743874615187,5.80628102785255,131.047527277329));
#277818=CARTESIAN_POINT('Ctrl Pts',(104.465426991374,3.34301971955009,126.050809465687));
#277819=CARTESIAN_POINT('Ctrl Pts',(104.186979367561,-2.19231339542621,
125.422372938737));
#277820=CARTESIAN_POINT('Ctrl Pts',(103.908531743748,-5.71301760046937,
129.739720163916));
#277821=CARTESIAN_POINT('Ctrl Pts',(103.630084119935,-3.98373772710686,
135.03541995542));
#277822=CARTESIAN_POINT('Ctrl Pts',(103.351636496123,1.40640250105958,136.442982914176));
#277823=CARTESIAN_POINT('Ctrl Pts',(103.07318887231,5.50412753733405,132.66892744436));
#277824=CARTESIAN_POINT('Ctrl Pts',(102.794741248497,4.54382825837723,127.181426149873));
#277825=CARTESIAN_POINT('Ctrl Pts',(102.516293624684,-0.592027211677165,
125.023224641008));
#277826=CARTESIAN_POINT('Ctrl Pts',(102.237846000871,-5.18383859633749,
128.177604670405));
#277827=CARTESIAN_POINT('Ctrl Pts',(101.959398377058,-5.01195555555783,
133.745845091081));
#277828=CARTESIAN_POINT('Ctrl Pts',(101.680950753245,-0.234330206861215,
136.611004980102));
#277829=CARTESIAN_POINT('Ctrl Pts',(101.402503129432,4.75863315427373,134.140142370299));
#277830=CARTESIAN_POINT('Ctrl Pts',(101.124055505619,5.37864511878468,128.603859291732));
#277831=CARTESIAN_POINT('Ctrl Pts',(100.845607881807,1.05594498055446,125.089729431141));
#277832=CARTESIAN_POINT('Ctrl Pts',(100.567160257994,-4.23711700902531,
126.827066455619));
#277833=CARTESIAN_POINT('Ctrl Pts',(100.288712634181,-5.63647546198416,
132.219342513305));
#277834=CARTESIAN_POINT('Ctrl Pts',(100.010265010368,-1.85618832251382,
136.311319334515));
#277835=CARTESIAN_POINT('Ctrl Pts',(99.731817386555,3.62984520550588,135.342670124737));
#277836=CARTESIAN_POINT('Ctrl Pts',(99.4533697627421,5.78022831746224,130.203536186614));
#277837=CARTESIAN_POINT('Ctrl Pts',(99.1749221389292,2.61886398552269,125.616530548629));
#277838=CARTESIAN_POINT('Ctrl Pts',(98.8964745151164,-2.9491084104941,125.796887304409));
#277839=CARTESIAN_POINT('Ctrl Pts',(98.6180268913035,-5.80699424922206,
130.578867406308));
#277840=CARTESIAN_POINT('Ctrl Pts',(98.3395792674906,-3.32853606035512,
135.568064753397));
#277841=CARTESIAN_POINT('Ctrl Pts',(98.0611316436778,2.20868415995158,136.179650719541));
#277842=CARTESIAN_POINT('Ctrl Pts',(97.7826840198649,5.71623153748262,131.851607679491));
#277843=CARTESIAN_POINT('Ctrl Pts',(97.5042363960519,3.97084138550236,126.561195750394));
#277844=CARTESIAN_POINT('Ctrl Pts',(97.2257887722391,-1.42355801336861,
125.170045044101));
#277845=CARTESIAN_POINT('Ctrl Pts',(96.9473411484261,-5.50977714262889,
128.956555098203));
#277846=CARTESIAN_POINT('Ctrl Pts',(96.6688935246133,-4.53278024539068,
134.441108154283));
#277847=CARTESIAN_POINT('Ctrl Pts',(96.3904459008004,0.609620258735999,
136.583667889112));
#277848=CARTESIAN_POINT('Ctrl Pts',(96.1119982769875,5.19180952668969,133.415326576248));
#277849=CARTESIAN_POINT('Ctrl Pts',(95.8335506531746,5.00297947361121,127.847635100131));
#277850=CARTESIAN_POINT('Ctrl Pts',(95.5551030293618,0.216655693418756,
124.997029930466));
#277851=CARTESIAN_POINT('Ctrl Pts',(95.2766554055487,-4.7687640848064,127.483077958369));
#277852=CARTESIAN_POINT('Ctrl Pts',(94.9982077817361,-5.37192263617151,
133.021222496396));
#277853=CARTESIAN_POINT('Ctrl Pts',(94.7197601579228,-1.03854671790542,
136.522179267501));
#277854=CARTESIAN_POINT('Ctrl Pts',(94.4413125341102,4.24920289828813,134.768740030285));
#277855=CARTESIAN_POINT('Ctrl Pts',(94.1628649102971,5.63214263605674,129.372229783482));
#277856=CARTESIAN_POINT('Ctrl Pts',(93.8844172864844,1.83941843675322,125.29177780972));
#277857=CARTESIAN_POINT('Ctrl Pts',(93.6059696626714,-3.6436414453401,126.277120131727));
#277858=CARTESIAN_POINT('Ctrl Pts',(93.3275220388585,-5.77837284094635,
131.422775292226));
#277859=CARTESIAN_POINT('Ctrl Pts',(93.0490744150458,-2.60306188492951,
136.000137577949));
#277860=CARTESIAN_POINT('Ctrl Pts',(92.7706267912327,2.96433577669487,135.802834664895));
#277861=CARTESIAN_POINT('Ctrl Pts',(92.49217916742,5.80765367539012,131.012178291378));
#277862=CARTESIAN_POINT('Ctrl Pts',(92.213731543607,3.31402156605677,126.030547628085));
#277863=CARTESIAN_POINT('Ctrl Pts',(91.9352839197941,-2.22503446352861,
125.435817888395));
#277864=CARTESIAN_POINT('Ctrl Pts',(91.6568362959812,-5.71939252010779,
129.77451664892));
#277865=CARTESIAN_POINT('Ctrl Pts',(91.3783886721684,-3.95790825856573,
135.059591705955));
#277866=CARTESIAN_POINT('Ctrl Pts',(91.0999410483554,1.44070033803066,136.434317272356));
#277867=CARTESIAN_POINT('Ctrl Pts',(90.8214934245425,5.51537570610103,132.635387711677));
#277868=CARTESIAN_POINT('Ctrl Pts',(90.5430458007297,4.52169024134706,127.153833702157));
#277869=CARTESIAN_POINT('Ctrl Pts',(90.2645981769166,-0.627207658356129,
125.026935589742));
#277870=CARTESIAN_POINT('Ctrl Pts',(89.9861505531037,-5.19973236082766,
128.209208834995));
#277871=CARTESIAN_POINT('Ctrl Pts',(89.707702929291,-4.99395704474619,133.776299788217));
#277872=CARTESIAN_POINT('Ctrl Pts',(89.4292553054779,-0.198979172907652,
136.61232383091));
#277873=CARTESIAN_POINT('Ctrl Pts',(89.1508076816652,4.77885083815996,134.111113415317));
#277874=CARTESIAN_POINT('Ctrl Pts',(88.8723600578521,5.36515038880097,128.571158722445));
#277875=CARTESIAN_POINT('Ctrl Pts',(88.5939124340396,1.02113883430145,125.08340747321));
#277876=CARTESIAN_POINT('Ctrl Pts',(88.3154648102263,-4.26124942351577,
126.85293267954));
#277877=CARTESIAN_POINT('Ctrl Pts',(88.0370171864138,-5.62775763472933,
132.253627122929));
#277878=CARTESIAN_POINT('Ctrl Pts',(87.7585695626006,-1.82263151087143,
136.322516448493));
#277879=CARTESIAN_POINT('Ctrl Pts',(87.480121938788,3.65740393097785,135.320490142334));
#277880=CARTESIAN_POINT('Ctrl Pts',(87.2016743149749,5.77646383437373,130.168361428106));
#277881=CARTESIAN_POINT('Ctrl Pts',(86.9232266911622,2.58723566992664,125.600684898703));
#277882=CARTESIAN_POINT('Ctrl Pts',(86.6447790673492,-2.97953568169397,
125.814932141244));
#277883=CARTESIAN_POINT('Ctrl Pts',(86.3663314435363,-5.80825930024783,
130.614220406392));
#277884=CARTESIAN_POINT('Ctrl Pts',(86.0878838197235,-3.29947637111547,
135.588238236744));
#277885=CARTESIAN_POINT('Ctrl Pts',(85.8094361959104,2.24136415469026,136.166106240484));
#277886=CARTESIAN_POINT('Ctrl Pts',(85.5309885720977,5.72250051906197,131.816791952599));
#277887=CARTESIAN_POINT('Ctrl Pts',(85.2525409482847,3.94493846610766,126.537102727838));
#277888=CARTESIAN_POINT('Ctrl Pts',(84.9740933244718,-1.45782931624159,
125.178815036599));
#277889=CARTESIAN_POINT('Ctrl Pts',(84.6956457006588,-5.52092317588609,
128.990128911089));
#277890=CARTESIAN_POINT('Ctrl Pts',(84.417198076846,-4.51055834898274,134.468633093685));
#277891=CARTESIAN_POINT('Ctrl Pts',(84.138750453033,0.644789247610192,136.579849880389));
#277892=CARTESIAN_POINT('Ctrl Pts',(83.8603028292202,5.20760702535536,133.383674182895));
#277893=CARTESIAN_POINT('Ctrl Pts',(83.5818552054073,4.98488835254533,127.817235325336));
#277894=CARTESIAN_POINT('Ctrl Pts',(83.3034075815944,0.181300809080568,
124.995818682153));
#277895=CARTESIAN_POINT('Ctrl Pts',(83.0249599577814,-4.78889332089225,
127.512168314565));
#277896=CARTESIAN_POINT('Ctrl Pts',(82.7465123339688,-5.35832843941005,
133.053881840899));
#277897=CARTESIAN_POINT('Ctrl Pts',(82.4680647101557,-1.00372149100682,
136.528395258211));
#277898=CARTESIAN_POINT('Ctrl Pts',(82.1896170863428,4.27325647311088,134.742800475408));
#277899=CARTESIAN_POINT('Ctrl Pts',(81.91116946253,5.62332049862395,129.337971866731));
#277900=CARTESIAN_POINT('Ctrl Pts',(81.632721838717,1.80582770038043,125.280682882997));
#277901=CARTESIAN_POINT('Ctrl Pts',(81.3542742149043,-3.67113253492515,
126.299383890674));
#277902=CARTESIAN_POINT('Ctrl Pts',(81.0758265910913,-5.77450131542928,
131.457938430015));
#277903=CARTESIAN_POINT('Ctrl Pts',(80.7973789672785,-2.57138548712596,
136.015886888767));
#277904=CARTESIAN_POINT('Ctrl Pts',(80.5189313434656,2.99470798468153,135.784697301496));
#277905=CARTESIAN_POINT('Ctrl Pts',(80.2404837196526,5.80881111818491,130.976821604667));
#277906=CARTESIAN_POINT('Ctrl Pts',(79.9620360958398,3.2849006102757,126.010462685879));
#277907=CARTESIAN_POINT('Ctrl Pts',(79.6835884720269,-2.25767308216064,
125.449461771377));
#277908=CARTESIAN_POINT('Ctrl Pts',(79.4051408482139,-5.72555550555307,
129.809351295171));
#277909=CARTESIAN_POINT('Ctrl Pts',(79.1266932244012,-3.93193212827854,
135.083605777338));
#277910=CARTESIAN_POINT('Ctrl Pts',(78.8482456005881,1.47494478932078,136.425443010422));
#277911=CARTESIAN_POINT('Ctrl Pts',(78.5697979767754,5.526419500593,132.601780129612));
#277912=CARTESIAN_POINT('Ctrl Pts',(78.2913503529625,4.49938467142216,127.126376526057));
#277913=CARTESIAN_POINT('Ctrl Pts',(78.0129027291494,-0.662364863624755,
125.030860623086));
#277914=CARTESIAN_POINT('Ctrl Pts',(77.7344551053368,-5.21543344732299,
128.240909163888));
#277915=CARTESIAN_POINT('Ctrl Pts',(77.4560074815235,-4.97577348101974,
133.806644359053));
#277916=CARTESIAN_POINT('Ctrl Pts',(77.1775598577108,-0.163620765707691,
136.613427465507));
#277917=CARTESIAN_POINT('Ctrl Pts',(76.8991122338979,4.79889143997102,134.081961927395));
#277918=CARTESIAN_POINT('Ctrl Pts',(76.620664610085,5.35145685119646,128.538540905275));
#277919=CARTESIAN_POINT('Ctrl Pts',(76.3422169862721,0.986294849373407,
125.077297507303));
#277920=CARTESIAN_POINT('Ctrl Pts',(76.0637693624593,-4.28522393584178,
126.878945325076));
#277921=CARTESIAN_POINT('Ctrl Pts',(75.7853217386464,-5.61883126884571,
132.287858029448));
#277922=CARTESIAN_POINT('Ctrl Pts',(75.5068741148335,-1.78900716094817,
136.333509085178));
#277923=CARTESIAN_POINT('Ctrl Pts',(75.2284264910206,3.68482713000219,135.298142813091));
#277924=CARTESIAN_POINT('Ctrl Pts',(74.9499788672077,5.77248530229349,130.133210236781));
#277925=CARTESIAN_POINT('Ctrl Pts',(74.6715312433948,2.55551148336137,125.585032072894));
#277926=CARTESIAN_POINT('Ctrl Pts',(74.3930836195819,-3.0098525451033,125.833161863185));
#277927=CARTESIAN_POINT('Ctrl Pts',(74.1146359957691,-5.80930912408932,
130.649580452192));
#277928=CARTESIAN_POINT('Ctrl Pts',(73.8361883719562,-3.27029441856551,
135.608234451746));
#277929=CARTESIAN_POINT('Ctrl Pts',(73.5577407481433,2.273961094856,136.152363079971));
#277930=CARTESIAN_POINT('Ctrl Pts',(73.2792931243304,5.72855745128013,131.781938709691));
#277931=CARTESIAN_POINT('Ctrl Pts',(73.0008455005175,3.91888936556733,126.513167830092));
#277932=CARTESIAN_POINT('Ctrl Pts',(72.7223978767045,-1.49204659871303,
125.187793485758));
#277933=CARTESIAN_POINT('Ctrl Pts',(72.4439502528918,-5.53186462930466,
129.023769950998));
#277934=CARTESIAN_POINT('Ctrl Pts',(72.1655026290786,-4.48816931217651,
134.496022252122));
#277935=CARTESIAN_POINT('Ctrl Pts',(71.8870550052659,0.679934343581693,
136.575817858786));
#277936=CARTESIAN_POINT('Ctrl Pts',(71.6086073814528,5.22321155422762,133.351926212129));
#277937=CARTESIAN_POINT('Ctrl Pts',(71.3301597576401,4.96661251460835,127.786946239566));
#277938=CARTESIAN_POINT('Ctrl Pts',(71.0517121338272,0.145939206574258,
124.994822671498));
#277939=CARTESIAN_POINT('Ctrl Pts',(70.7732645100143,-4.80884510277506,
127.541380664158));
#277940=CARTESIAN_POINT('Ctrl Pts',(70.4948168862015,-5.34453568781766,
133.086457828568));
#277941=CARTESIAN_POINT('Ctrl Pts',(70.2163692623885,-0.968859070839113,
136.534399142713));
#277942=CARTESIAN_POINT('Ctrl Pts',(69.9379216385757,4.29715170084345,134.716714980192));
#277943=CARTESIAN_POINT('Ctrl Pts',(69.6594740147628,5.61428998698222,129.303768287553));
#277944=CARTESIAN_POINT('Ctrl Pts',(69.3810263909498,1.77217004839796,125.269792638185));
#277945=CARTESIAN_POINT('Ctrl Pts',(69.102578767137,-3.69848758934425,126.321814583191));
#277946=CARTESIAN_POINT('Ctrl Pts',(68.8241311433241,-5.77041581364239,
131.493077349239));
#277947=CARTESIAN_POINT('Ctrl Pts',(68.5456835195112,-2.53961380568736,
136.031443084562));
#277948=CARTESIAN_POINT('Ctrl Pts',(68.2672358956983,3.02496922266262,135.76637538989));
#277949=CARTESIAN_POINT('Ctrl Pts',(67.9887882718854,5.80975331334755,130.94145852735));
#277950=CARTESIAN_POINT('Ctrl Pts',(67.7103406480725,3.25565793129432,125.990555383323));
#277951=CARTESIAN_POINT('Ctrl Pts',(67.4318930242597,-2.29022804188655,
125.463304082106));
#277952=CARTESIAN_POINT('Ctrl Pts',(67.1534454004468,-5.73150632843341,
129.844222811859));
#277953=CARTESIAN_POINT('Ctrl Pts',(66.8749977766338,-3.90581029880048,
135.107461279717));
#277954=CARTESIAN_POINT('Ctrl Pts',(66.5965501528209,1.50913458598933,136.416360457212));
#277955=CARTESIAN_POINT('Ctrl Pts',(66.3181025290079,5.53725851157817,132.568105943505));
#277956=CARTESIAN_POINT('Ctrl Pts',(66.0396549051952,4.47691237514338,127.09905563901));
#277957=CARTESIAN_POINT('Ctrl Pts',(65.7612072813823,-0.69749752471975,
125.034999595595));
#277958=CARTESIAN_POINT('Ctrl Pts',(65.4827596575694,-5.23094127401388,
128.272704482416));
#277959=CARTESIAN_POINT('Ctrl Pts',(65.2043120337565,-4.95740553817722,
133.836877679162));
#277960=CARTESIAN_POINT('Ctrl Pts',(64.9258644099437,-0.128256295479839,
136.614315842995));
#277961=CARTESIAN_POINT('Ctrl Pts',(64.6474167861306,4.81875421709505,134.05268898675));
#277962=CARTESIAN_POINT('Ctrl Pts',(64.3689691623179,5.33756501339024,128.506007048888));
#277963=CARTESIAN_POINT('Ctrl Pts',(64.0905215385049,0.951414316927145,
125.071399759827));
#277964=CARTESIAN_POINT('Ctrl Pts',(63.8120739146922,-4.30903965761881,
126.905103428319));
#277965=CARTESIAN_POINT('Ctrl Pts',(63.5336262908791,-5.60969669510319,
132.322033964426));
#277966=CARTESIAN_POINT('Ctrl Pts',(63.2551786670663,-1.75531651870651,
136.344296837232));
#277967=CARTESIAN_POINT('Ctrl Pts',(62.9767310432534,3.71211378640213,135.275628965096));
#277968=CARTESIAN_POINT('Ctrl Pts',(62.6982834194405,5.76829286864752,130.098083915181));
#277969=CARTESIAN_POINT('Ctrl Pts',(62.4198357956276,2.52369260137852,125.569572651222));
#277970=CARTESIAN_POINT('Ctrl Pts',(62.1413881718147,-3.04005787731984,
125.851575794724));
#277971=CARTESIAN_POINT('Ctrl Pts',(61.8629405480017,-5.81014368184488,
130.684946233427));
#277972=CARTESIAN_POINT('Ctrl Pts',(61.5844929241889,-3.24099128405306,
135.628052657436));
#277973=CARTESIAN_POINT('Ctrl Pts',(61.3060453003759,2.306473772557,136.138421747261));
#277974=CARTESIAN_POINT('Ctrl Pts',(61.0275976765631,5.73440210969521,131.747049242268));
#277975=CARTESIAN_POINT('Ctrl Pts',(60.7491500527502,3.89269504914048,126.489391944074));
#277976=CARTESIAN_POINT('Ctrl Pts',(60.4707024289374,-1.5262085928491,125.196980058879));
#277977=CARTESIAN_POINT('Ctrl Pts',(60.1922548051244,-5.54260109744501,
129.057476971348));
#277978=CARTESIAN_POINT('Ctrl Pts',(59.9138071813117,-4.46561396460588,
134.52327461468));
#277979=CARTESIAN_POINT('Ctrl Pts',(59.6353595574987,0.715054244335847,
136.571571973714));
#277980=CARTESIAN_POINT('Ctrl Pts',(59.3569119336859,5.23862253507484,133.320083840384));
#277981=CARTESIAN_POINT('Ctrl Pts',(59.0784643098728,4.94815263701827,127.756768965196));
#277982=CARTESIAN_POINT('Ctrl Pts',(58.80001668606,0.110572196236736,124.994041935407));
#277983=CARTESIAN_POINT('Ctrl Pts',(58.5215690622471,-4.82861869113419,
127.570713924673));
#277984=CARTESIAN_POINT('Ctrl Pts',(58.2431214384343,-5.3305448924898,133.118949252284));
#277985=CARTESIAN_POINT('Ctrl Pts',(57.9646738146213,-0.933960749242644,
136.54019069853));
#277986=CARTESIAN_POINT('Ctrl Pts',(57.6862261908085,4.32088769603949,134.690484511247));
#277987=CARTESIAN_POINT('Ctrl Pts',(57.4077785669955,5.6050514357603,129.269620313377));
#277988=CARTESIAN_POINT('Ctrl Pts',(57.1293309431827,1.73844672800264,125.259107478825));
#277989=CARTESIAN_POINT('Ctrl Pts',(56.8508833193697,-3.72570559494523,
126.3444113781));
#277990=CARTESIAN_POINT('Ctrl Pts',(56.5724356955568,-5.76611648697549,
131.528190747811));
#277991=CARTESIAN_POINT('Ctrl Pts',(56.293988071744,-2.50774801792579,136.046805588895));
#277992=CARTESIAN_POINT('Ctrl Pts',(56.0155404479311,3.05511836929639,135.747869609001));
#277993=CARTESIAN_POINT('Ctrl Pts',(55.7370928241181,5.81048022596477,130.906090369819));
#277994=CARTESIAN_POINT('Ctrl Pts',(55.4586452003054,3.22629461271119,125.97082645809));
#277995=CARTESIAN_POINT('Ctrl Pts',(55.1801975764924,-2.32269813636975,
125.477344307648));
#277996=CARTESIAN_POINT('Ctrl Pts',(54.9017499526795,-5.73724476823917,
129.879129906805));
#277997=CARTESIAN_POINT('Ctrl Pts',(54.6233023288666,-3.87954373808533,
135.131157329118));
#277998=CARTESIAN_POINT('Ctrl Pts',(54.3448547050537,1.54326846112093,136.407069949284));
#277999=CARTESIAN_POINT('Ctrl Pts',(54.0664070812409,5.54789233741261,132.534366401168));
#278000=CARTESIAN_POINT('Ctrl Pts',(53.7879594574279,4.45427418523046,127.071872053402));
#278001=CARTESIAN_POINT('Ctrl Pts',(53.5095118336151,-0.732604339787292,
125.039352353899));
#278002=CARTESIAN_POINT('Ctrl Pts',(53.2310642098022,-5.24625526625226,
128.304593612394));
#278003=CARTESIAN_POINT('Ctrl Pts',(52.9526165859893,-4.93885389684926,
133.866998628235));
#278004=CARTESIAN_POINT('Ctrl Pts',(52.6741689621764,-0.0928870726681018,
136.614988930455));
#278005=CARTESIAN_POINT('Ctrl Pts',(52.3957213383635,4.83843843350925,134.023295678104));
#278006=CARTESIAN_POINT('Ctrl Pts',(52.1172737145507,5.32347539014984,128.473558358838));
#278007=CARTESIAN_POINT('Ctrl Pts',(51.8388260907377,0.91649852947334,125.065714449322));
#278008=CARTESIAN_POINT('Ctrl Pts',(51.5603784669247,-4.33269570634681,
126.931406019971));
#278009=CARTESIAN_POINT('Ctrl Pts',(51.2819308431118,-5.6003542519866,132.356153661459));
#278010=CARTESIAN_POINT('Ctrl Pts',(51.0034832192991,-1.72156083256576,
136.354879304913));
#278011=CARTESIAN_POINT('Ctrl Pts',(50.7250355954861,3.73926288906064,135.252949432607));
#278012=CARTESIAN_POINT('Ctrl Pts',(50.4465879716733,5.76388668878802,130.062983764924));
#278013=CARTESIAN_POINT('Ctrl Pts',(50.1681403478604,2.49178020303801,125.554307206545));
#278014=CARTESIAN_POINT('Ctrl Pts',(49.8896927240475,-3.07015055907373,
125.870173253527));
#278015=CARTESIAN_POINT('Ctrl Pts',(49.6112451002346,-5.81076294258959,
130.720316439607));
#278016=CARTESIAN_POINT('Ctrl Pts',(49.3327974764216,-3.21156805341676,
135.647692119444));
#278017=CARTESIAN_POINT('Ctrl Pts',(49.0543498526089,2.33890098302428,136.124282758954));
#278018=CARTESIAN_POINT('Ctrl Pts',(48.7759022287959,5.74003427773134,131.712124843171));
#278019=CARTESIAN_POINT('Ctrl Pts',(48.497454604983,3.86635648746696,126.465775950806));
#278020=CARTESIAN_POINT('Ctrl Pts',(48.2190069811701,-1.56031403276457,
125.206374415548));
#278021=CARTESIAN_POINT('Ctrl Pts',(47.9405593573573,-5.55313218246346,
129.091248723115));
#278022=CARTESIAN_POINT('Ctrl Pts',(47.6621117335443,-4.44289314206747,
134.550389171513));
#278023=CARTESIAN_POINT('Ctrl Pts',(47.3836641097315,0.750147648492217,
136.567112382502));
#278024=CARTESIAN_POINT('Ctrl Pts',(47.1052164859186,5.25383939683757,133.288148247589));
#278025=CARTESIAN_POINT('Ctrl Pts',(46.8267688621057,4.92950940381243,127.726704620456));
#278026=CARTESIAN_POINT('Ctrl Pts',(46.5483212382927,0.0752010886061242,
124.993476502813));
#278027=CARTESIAN_POINT('Ctrl Pts',(46.2698736144798,-4.84821335325179,
127.600167009156));
#278028=CARTESIAN_POINT('Ctrl Pts',(45.991425990667,-5.31635657186091,133.151354908068));
#278029=CARTESIAN_POINT('Ctrl Pts',(45.7129783668541,-0.899027819386881,
136.545769711054));
#278030=CARTESIAN_POINT('Ctrl Pts',(45.4345307430412,4.344463579153,134.664110040551));
#278031=CARTESIAN_POINT('Ctrl Pts',(45.1560831192283,5.5956051872961,129.235529209567));
#278032=CARTESIAN_POINT('Ctrl Pts',(44.8776354954154,1.70465898882477,125.248627800858));
#278033=CARTESIAN_POINT('Ctrl Pts',(44.5991878716026,-3.7527855431554,126.367173438067));
#278034=CARTESIAN_POINT('Ctrl Pts',(44.3207402477896,-5.76160349474165,
131.563277324591));
#278035=CARTESIAN_POINT('Ctrl Pts',(44.0422926239769,-2.47578930463884,
136.0619738325));
#278036=CARTESIAN_POINT('Ctrl Pts',(43.7638450001637,3.08515430739569,135.72918064457));
#278037=CARTESIAN_POINT('Ctrl Pts',(43.485397376351,5.8109918291003,130.870718442656));
#278038=CARTESIAN_POINT('Ctrl Pts',(43.206949752538,3.19681174259461,125.951276641244));
#278039=CARTESIAN_POINT('Ctrl Pts',(42.9285021287252,-2.3550821624196,125.491581927739));
#278040=CARTESIAN_POINT('Ctrl Pts',(42.6500545049123,-5.74277061233009,
129.914071286517));
#278041=CARTESIAN_POINT('Ctrl Pts',(42.3716068810994,-3.85313341945026,
135.154693047476));
#278042=CARTESIAN_POINT('Ctrl Pts',(42.0931592572865,1.57734514987214,136.397571830902));
#278043=CARTESIAN_POINT('Ctrl Pts',(41.8147116334736,5.5583205840564,132.50056275283));
#278044=CARTESIAN_POINT('Ctrl Pts',(41.5362640096606,4.43147094054935,127.04482677653));
#278045=CARTESIAN_POINT('Ctrl Pts',(41.2578163858478,-0.767684007931795,
125.043918736703));
#278046=CARTESIAN_POINT('Ctrl Pts',(40.9793687620349,-5.26137485657243,
128.336575372158));
#278047=CARTESIAN_POINT('Ctrl Pts',(40.700921138222,-4.9201192444739,133.897006090131));
#278048=CARTESIAN_POINT('Ctrl Pts',(40.4224735144091,-0.0575144078915333,
136.615446702946));
#278049=CARTESIAN_POINT('Ctrl Pts',(40.1440258905964,4.85794335980812,133.993783090635));
#278050=CARTESIAN_POINT('Ctrl Pts',(39.8655782667833,5.30918850357096,128.441196037522));
#278051=CARTESIAN_POINT('Ctrl Pts',(39.5871306429705,0.8815487808295,125.060241786462));
#278052=CARTESIAN_POINT('Ctrl Pts',(39.3086830191576,-4.35619120544207,
126.957852125381));
#278053=CARTESIAN_POINT('Ctrl Pts',(39.0302353953447,-5.59080428568363,
132.39021585623));
#278054=CARTESIAN_POINT('Ctrl Pts',(38.7517877715318,-1.6877413533555,136.365256096082));
#278055=CARTESIAN_POINT('Ctrl Pts',(38.4733401477189,3.76627343195761,135.230105056025));
#278056=CARTESIAN_POINT('Ctrl Pts',(38.194892523906,5.7592669259876,130.027911086658));
#278057=CARTESIAN_POINT('Ctrl Pts',(37.9164449000932,2.45977547086574,125.539236304527));
#278058=CARTESIAN_POINT('Ctrl Pts',(37.6379972762802,-3.10012947526937,
125.888953550457));
#278059=CARTESIAN_POINT('Ctrl Pts',(37.3595496524674,-5.81116688337655,
130.755689760074));
#278060=CARTESIAN_POINT('Ctrl Pts',(37.0811020286545,-3.18202581694541,
135.667152110023));
#278061=CARTESIAN_POINT('Ctrl Pts',(36.8026544048415,2.3712415246555,136.109946638975));
#278062=CARTESIAN_POINT('Ctrl Pts',(36.5242067810287,5.74545374668639,131.677166806538));
#278063=CARTESIAN_POINT('Ctrl Pts',(36.2457591572158,3.83987465653194,126.442320725389));
#278064=CARTESIAN_POINT('Ctrl Pts',(35.9673115334029,-1.59436165466975,
125.215976207654));
#278065=CARTESIAN_POINT('Ctrl Pts',(35.6888639095901,-5.56345749412674,
129.125083954872));
#278066=CARTESIAN_POINT('Ctrl Pts',(35.4104162857771,-4.42000768648982,
134.57736491788));
#278067=CARTESIAN_POINT('Ctrl Pts',(35.1319686619643,0.785213255651605,
136.562439250406));
#278068=CARTESIAN_POINT('Ctrl Pts',(34.8535210381513,5.26886157564935,133.25612061713));
#278069=CARTESIAN_POINT('Ctrl Pts',(34.5750734143385,4.91068350582282,127.69675431939));
#278070=CARTESIAN_POINT('Ctrl Pts',(34.2966257905255,0.0398271943713243,
124.993126394665));
#278071=CARTESIAN_POINT('Ctrl Pts',(34.0181781667127,-4.86762836304081,
127.629738826211));
#278072=CARTESIAN_POINT('Ctrl Pts',(33.7397305428998,-5.30197125168398,
133.183673595116));
#278073=CARTESIAN_POINT('Ctrl Pts',(33.4612829190869,-0.864061575724654,
136.551135973552));
#278074=CARTESIAN_POINT('Ctrl Pts',(33.182835295274,4.36787847657091,134.637592545421));
#278075=CARTESIAN_POINT('Ctrl Pts',(32.9043876714611,5.58595159162396,129.201496239381));
#278076=CARTESIAN_POINT('Ctrl Pts',(32.6259400476482,1.67080808288091,125.238353992614));
#278077=CARTESIAN_POINT('Ctrl Pts',(32.3474924238352,-3.77972643051725,
126.390099919638));
#278078=CARTESIAN_POINT('Ctrl Pts',(32.0690448000224,-5.75687700417149,
131.598335779433));
#278079=CARTESIAN_POINT('Ctrl Pts',(31.7905971762095,-2.44373885006871,
136.076947253315));
#278080=CARTESIAN_POINT('Ctrl Pts',(31.5121495523967,3.11507592396733,135.71030918912));
#278081=CARTESIAN_POINT('Ctrl Pts',(31.2337019285837,5.81128810379662,130.835344056578));
#278082=CARTESIAN_POINT('Ctrl Pts',(30.9552543047708,3.16721041344351,125.931906657209));
#278083=CARTESIAN_POINT('Ctrl Pts',(30.676806680958,-2.38737892003384,125.506016414799));
#278084=CARTESIAN_POINT('Ctrl Pts',(30.398359057145,-5.74808365594406,129.949045656226));
#278085=CARTESIAN_POINT('Ctrl Pts',(30.1199114333322,-3.82658032153943,
135.178067562667));
#278086=CARTESIAN_POINT('Ctrl Pts',(29.8414638095193,1.61136338951851,136.387866454021));
#278087=CARTESIAN_POINT('Ctrl Pts',(29.5630161857064,5.56854286508694,132.466696251098));
#278088=CARTESIAN_POINT('Ctrl Pts',(29.2845685618935,4.40850348608286,127.017920810568));
#278089=CARTESIAN_POINT('Ctrl Pts',(29.0061209380806,-0.802735229263066,
125.048698574801));
#278090=CARTESIAN_POINT('Ctrl Pts',(28.7276733142678,-5.27629948471241,
128.368648576612));
#278091=CARTESIAN_POINT('Ctrl Pts',(28.4492256904548,-4.90120227527057,
133.926898952911));
#278092=CARTESIAN_POINT('Ctrl Pts',(28.170778066642,-0.0221396118974229,
136.615689143506));
#278093=CARTESIAN_POINT('Ctrl Pts',(27.892330442829,4.87726827322928,133.964152317942));
#278094=CARTESIAN_POINT('Ctrl Pts',(27.6138828190162,5.29470488305963,128.408921284139));
#278095=CARTESIAN_POINT('Ctrl Pts',(27.3354351952032,0.846566366071392,
125.054981974037));
#278096=CARTESIAN_POINT('Ctrl Pts',(27.0569875713904,-4.37952528427021,
126.984440764576));
#278097=CARTESIAN_POINT('Ctrl Pts',(26.7785399475775,-5.58104715007188,
132.424219286554));
#278098=CARTESIAN_POINT('Ctrl Pts',(26.5000923237646,-1.65385933426847,
136.375426826225));
#278099=CARTESIAN_POINT('Ctrl Pts',(26.2216446999517,3.79314441420758,135.207096681855));
#278100=CARTESIAN_POINT('Ctrl Pts',(25.9431970761388,5.75443375143326,129.992867180015));
#278101=CARTESIAN_POINT('Ctrl Pts',(25.6647494523259,2.42767959080881,125.524360503627));
#278102=CARTESIAN_POINT('Ctrl Pts',(25.3863018285131,-3.12999351502748,
125.907915989602));
#278103=CARTESIAN_POINT('Ctrl Pts',(25.1078542047001,-5.81135548923757,
130.791064884058));
#278104=CARTESIAN_POINT('Ctrl Pts',(24.8294065808873,-3.152365669337,135.686431908074));
#278105=CARTESIAN_POINT('Ctrl Pts',(24.5509589570743,2.40349419906,136.095413918554));
#278106=CARTESIAN_POINT('Ctrl Pts',(24.2725113332615,5.75066031573997,131.64217642775));
#278107=CARTESIAN_POINT('Ctrl Pts',(23.9940637094486,3.81325053762949,126.419027136963));
#278108=CARTESIAN_POINT('Ctrl Pts',(23.7156160856357,-1.62835019691723,
125.2257850794));
#278109=CARTESIAN_POINT('Ctrl Pts',(23.4371684618228,-5.57357664982666,
129.158981412844));
#278110=CARTESIAN_POINT('Ctrl Pts',(23.1587208380098,-4.39695844590187,
134.604200854185));
#278111=CARTESIAN_POINT('Ctrl Pts',(22.880273214197,0.820249766445046,136.557552750588));
#278112=CARTESIAN_POINT('Ctrl Pts',(22.6018255903841,5.28368851485763,133.224002135804));
#278113=CARTESIAN_POINT('Ctrl Pts',(22.3233779665712,4.89167564065013,127.666919171818));
#278114=CARTESIAN_POINT('Ctrl Pts',(22.0449303427584,0.00445182432539013,
124.992991623939));
#278115=CARTESIAN_POINT('Ctrl Pts',(21.7664827189454,-4.88686300107076,
127.659428280044));
#278116=CARTESIAN_POINT('Ctrl Pts',(21.4880350951325,-5.28738946501251,
133.215904115845));
#278117=CARTESIAN_POINT('Ctrl Pts',(21.2095874713197,-0.829063313942982,
136.556289287176));
#278118=CARTESIAN_POINT('Ctrl Pts',(20.9311398475068,4.39113152064558,134.610933008472));
#278119=CARTESIAN_POINT('Ctrl Pts',(20.6526922236938,5.57609100646137,129.167522663925));
#278120=CARTESIAN_POINT('Ctrl Pts',(20.374244599881,1.6368952645291,125.228286434793));
#278121=CARTESIAN_POINT('Ctrl Pts',(20.0957969760681,-3.80652725872624,
126.413189973261));
#278122=CARTESIAN_POINT('Ctrl Pts',(19.8173493522552,-5.75193719040684,
131.633364813234));
#278123=CARTESIAN_POINT('Ctrl Pts',(19.5389017284423,-2.41159784185683,
136.091725296493));
#278124=CARTESIAN_POINT('Ctrl Pts',(19.2604541046294,3.14488211025528,135.691255941942));
#278125=CARTESIAN_POINT('Ctrl Pts',(18.9820064808165,5.81136903907515,130.799968522399));
#278126=CARTESIAN_POINT('Ctrl Pts',(18.7035588570036,3.13749172214556,125.912717223747));
#278127=CARTESIAN_POINT('Ctrl Pts',(18.4251112331907,-2.41958721244422,
125.52064723395));
#278128=CARTESIAN_POINT('Ctrl Pts',(18.1466636093778,-5.75318370220431,
129.984051719947));
#278129=CARTESIAN_POINT('Ctrl Pts',(17.868215985565,-3.79988542828747,135.201280008538));
#278130=CARTESIAN_POINT('Ctrl Pts',(17.589768361752,1.64532191950215,136.377954178279));
#278131=CARTESIAN_POINT('Ctrl Pts',(17.3113207379392,5.57855880171371,132.432768150908));
#278132=CARTESIAN_POINT('Ctrl Pts',(17.0328731141263,4.38537267289848,126.991155152525));
#278133=CARTESIAN_POINT('Ctrl Pts',(16.7544254903134,-0.83775670494522,
125.053691691071));
#278134=CARTESIAN_POINT('Ctrl Pts',(16.4759778665005,-5.29102859763445,
128.400812037271));
#278135=CARTESIAN_POINT('Ctrl Pts',(16.1975302426876,-4.88210369021464,
133.956676108886));
#278136=CARTESIAN_POINT('Ctrl Pts',(15.9190826188747,0.013236004487936,
136.61571624315));
#278137=CARTESIAN_POINT('Ctrl Pts',(15.6406349950618,4.89641245768097,133.934404458007));
#278138=CARTESIAN_POINT('Ctrl Pts',(15.3621873712489,5.2800250653117,128.376735294641));
#278139=CARTESIAN_POINT('Ctrl Pts',(15.0837397474361,0.811552581485459,
125.049935206953));
#278140=CARTESIAN_POINT('Ctrl Pts',(14.8052921236231,-4.40269707817821,
127.011170952307));
#278141=CARTESIAN_POINT('Ctrl Pts',(14.5268444998103,-5.57108320670569,
132.458162692417));
#278142=CARTESIAN_POINT('Ctrl Pts',(14.2483968759974,-1.6199160308156,136.385391118461));
#278143=CARTESIAN_POINT('Ctrl Pts',(13.9699492521845,3.81987484009636,135.18392516268));
#278144=CARTESIAN_POINT('Ctrl Pts',(13.6915016283715,5.74938734422005,129.95785334356));
#278145=CARTESIAN_POINT('Ctrl Pts',(13.4130540045587,2.39549375219187,125.509680355073));
#278146=CARTESIAN_POINT('Ctrl Pts',(13.1346063807458,-3.15974157172482,
125.927059868305));
#278147=CARTESIAN_POINT('Ctrl Pts',(12.8561587569329,-5.81132875318382,
130.82644050072));
#278148=CARTESIAN_POINT('Ctrl Pts',(12.57771113312,-3.12258870965941,135.705530799178));
#278149=CARTESIAN_POINT('Ctrl Pts',(12.2992635093071,2.43565781110307,136.080685136208));
#278150=CARTESIAN_POINT('Ctrl Pts',(12.0208158854942,5.75565379196074,131.607155003388));
#278151=CARTESIAN_POINT('Ctrl Pts',(11.7423682616813,3.78648511732596,126.395896048684));
#278152=CARTESIAN_POINT('Ctrl Pts',(11.4639206378685,-1.66227840004959,
125.235800667314));
#278153=CARTESIAN_POINT('Ctrl Pts',(11.1854730140555,-5.58348927459409,
129.192939840948));
#278154=CARTESIAN_POINT('Ctrl Pts',(10.9070253902426,-4.37374627440173,
134.630895986013));
#278155=CARTESIAN_POINT('Ctrl Pts',(10.6285777664298,0.855255882581734,
136.552453064119));
#278156=CARTESIAN_POINT('Ctrl Pts',(10.3501301426169,5.29831966504511,133.19179399377));
#278157=CARTESIAN_POINT('Ctrl Pts',(10.071682518804,4.87248651263752,127.637200283293));
#278158=CARTESIAN_POINT('Ctrl Pts',(9.79323489499104,-0.0309237106847325,
124.993072195629));
#278159=CARTESIAN_POINT('Ctrl Pts',(9.51478727117816,-4.90591655459505,
127.689234270502));
#278160=CARTESIAN_POINT('Ctrl Pts',(9.23633964736526,-5.27261175218,133.248045275945));
#278161=CARTESIAN_POINT('Ctrl Pts',(8.95789202355236,-0.794034330915497,
136.561229460968));
#278162=CARTESIAN_POINT('Ctrl Pts',(8.67944439973947,4.41422184972672,134.584132417584));
#278163=CARTESIAN_POINT('Ctrl Pts',(8.40099677592661,5.56602379719609,129.1336097421));
#278164=CARTESIAN_POINT('Ctrl Pts',(8.12254915211368,1.60292179042129,125.218425500451));
#278165=CARTESIAN_POINT('Ctrl Pts',(7.84410152830078,-3.83318703466779,
126.436442743329));
#278166=CARTESIAN_POINT('Ctrl Pts',(7.56565390448795,-5.74678423649425,
131.668363127979));
#278167=CARTESIAN_POINT('Ctrl Pts',(7.28720628067502,-2.37936747100029,
136.106307414428));
#278168=CARTESIAN_POINT('Ctrl Pts',(7.00875865686212,3.17457176177998,135.672021609062));
#278169=CARTESIAN_POINT('Ctrl Pts',(6.73031103304925,5.81123463193681,130.764593150968));
#278170=CARTESIAN_POINT('Ctrl Pts',(6.45186340923634,3.10765676993803,125.89370905193));
#278171=CARTESIAN_POINT('Ctrl Pts',(6.17341578542346,-2.45170584616043,
125.535473843045));
#278172=CARTESIAN_POINT('Ctrl Pts',(5.89496816161054,-5.75807056212669,
130.019088180515));
#278173=CARTESIAN_POINT('Ctrl Pts',(5.61652053779771,-3.77304972888379,
135.224329524944));
#278174=CARTESIAN_POINT('Ctrl Pts',(5.33807291398477,1.67921948147701,136.367835370977));
#278175=CARTESIAN_POINT('Ctrl Pts',(5.05962529017187,5.58836802279258,132.398779709476));
#278176=CARTESIAN_POINT('Ctrl Pts',(4.781177666359,4.36207935811697,126.964530794212));
#278177=CARTESIAN_POINT('Ctrl Pts',(4.50273004254611,-0.872747137244579,
125.058897900495));
#278178=CARTESIAN_POINT('Ctrl Pts',(4.2242824187332,-5.30556164954619,128.433064562307));
#278179=CARTESIAN_POINT('Ctrl Pts',(3.94583479492031,-4.86282419701095,
133.986336454649));
#278180=CARTESIAN_POINT('Ctrl Pts',(3.66738717110745,0.0486111304084952,
136.615528000873));
#278181=CARTESIAN_POINT('Ctrl Pts',(3.38893954729453,4.91537520376836,133.904540613147));
#278182=CARTESIAN_POINT('Ctrl Pts',(3.11049192348162,5.26514959429328,128.344639261694));
#278183=CARTESIAN_POINT('Ctrl Pts',(2.83204429966877,0.776508724519974,
125.045101672218));
#278184=CARTESIAN_POINT('Ctrl Pts',(2.55359667585587,-4.42570572852705,
127.038041698076));
#278185=CARTESIAN_POINT('Ctrl Pts',(2.27514905204296,-5.56091282480238,
132.492044816037));
#278186=CARTESIAN_POINT('Ctrl Pts',(1.99670142823006,-1.58591270077849,
136.395148603559));
#278187=CARTESIAN_POINT('Ctrl Pts',(1.7182538044172,3.84646371911817,135.160591357131));
#278188=CARTESIAN_POINT('Ctrl Pts',(1.43980618060429,5.7441278913444,129.922870874744));
#278189=CARTESIAN_POINT('Ctrl Pts',(1.16135855679139,2.36321914767325,125.495196402842));
#278190=CARTESIAN_POINT('Ctrl Pts',(0.882910932978526,-3.18937254303613,
125.946384477181));
#278191=CARTESIAN_POINT('Ctrl Pts',(0.604463309165634,-5.81108667620601,
130.861815299204));
#278192=CARTESIAN_POINT('Ctrl Pts',(0.326015685352703,-3.09269604130886,
135.724448075619));
#278193=CARTESIAN_POINT('Ctrl Pts',(0.0475680615398608,2.46773116894999,
136.065760837718));
#278194=CARTESIAN_POINT('Ctrl Pts',(-0.230879562273037,5.76043399031358,
131.572103831187));
#278195=CARTESIAN_POINT('Ctrl Pts',(-0.509327186085944,3.75957938742415,
126.37292831768));
#278196=CARTESIAN_POINT('Ctrl Pts',(-0.787774809898847,-1.69614500684454,
125.246022600264));
#278197=CARTESIAN_POINT('Ctrl Pts',(-1.06622243371171,-5.59319500111311,
129.226957980841));
#278198=CARTESIAN_POINT('Ctrl Pts',(-1.34467005752462,-4.35037203212501,
134.657449324165));
#278199=CARTESIAN_POINT('Ctrl Pts',(-1.62311768133752,0.890230306896913,
136.547140379971));
#278200=CARTESIAN_POINT('Ctrl Pts',(-1.90156530515039,5.31275448404895,
133.159497384516));
#278201=CARTESIAN_POINT('Ctrl Pts',(-2.18001292896328,4.85311683284533,
127.607598755059));
#278202=CARTESIAN_POINT('Ctrl Pts',(-2.4584605527762,-0.0662980998053887,
124.993368106748));
#278203=CARTESIAN_POINT('Ctrl Pts',(-2.73690817658909,-4.92478831757726,
127.719155693111));
#278204=CARTESIAN_POINT('Ctrl Pts',(-3.01535580040196,-5.25763866077998,
133.280095884409));
#278205=CARTESIAN_POINT('Ctrl Pts',(-3.29380342421486,-0.758975924653704,
136.565956311869));
#278206=CARTESIAN_POINT('Ctrl Pts',(-3.57225104802777,4.43714860819409,
134.557191765862));
#278207=CARTESIAN_POINT('Ctrl Pts',(-3.85069867184063,5.55575033687191,
129.099758730564));
#278208=CARTESIAN_POINT('Ctrl Pts',(-4.12914629565353,1.56888891945708,
125.208771554989));
#278209=CARTESIAN_POINT('Ctrl Pts',(-4.40759391946644,-3.85970477045413,
126.459857368199));
#278210=CARTESIAN_POINT('Ctrl Pts',(-4.68604154327934,-5.74141833337845,
131.703329426794));
#278211=CARTESIAN_POINT('Ctrl Pts',(-4.96448916709218,-2.34704893180687,
136.120693066776));
#278212=CARTESIAN_POINT('Ctrl Pts',(-5.24293679090511,3.20414377838073,
135.652606903212));
#278213=CARTESIAN_POINT('Ctrl Pts',(-5.52138441471801,5.81088488736209,
130.729219253137));
#278214=CARTESIAN_POINT('Ctrl Pts',(-5.79983203853088,3.07770666236606,
125.874882846113));
#278215=CARTESIAN_POINT('Ctrl Pts',(-6.07827966234377,-2.48373363101511,
125.550495692676));
#278216=CARTESIAN_POINT('Ctrl Pts',(-6.35672728615668,-5.7627440546269,
130.054153739642));
#278217=CARTESIAN_POINT('Ctrl Pts',(-6.63517490996957,-3.74607421773465,
135.247215257776));
#278218=CARTESIAN_POINT('Ctrl Pts',(-6.91362253378244,1.71305481935644,
136.357510407073));
#278219=CARTESIAN_POINT('Ctrl Pts',(-7.19207015759534,5.59797016483923,
132.36473218626));
#278220=CARTESIAN_POINT('Ctrl Pts',(-7.47051778140826,4.33862440488076,
126.938048722207));
#278221=CARTESIAN_POINT('Ctrl Pts',(-7.74896540522111,-0.907705229577551,
125.064317010151));
#278222=CARTESIAN_POINT('Ctrl Pts',(-8.027413029034,-5.31989810191992,128.46540495659));
#278223=CARTESIAN_POINT('Ctrl Pts',(-8.30586065284694,-4.84336451006833,
134.015878891129));
#278224=CARTESIAN_POINT('Ctrl Pts',(-8.58430827665978,0.0839844550257475,
136.615124423653));
#278225=CARTESIAN_POINT('Ctrl Pts',(-8.86275590047269,4.93415580881975,
133.874561889976));
#278226=CARTESIAN_POINT('Ctrl Pts',(-9.14120352428557,5.25007902122049,
128.312634374625));
#278227=CARTESIAN_POINT('Ctrl Pts',(-9.4196511480985,0.741436093738357,
125.040481548942));
#278228=CARTESIAN_POINT('Ctrl Pts',(-9.69809877191133,-4.44855038272257,
127.065052006178));
#278229=CARTESIAN_POINT('Ctrl Pts',(-9.97654639572428,-5.5505363812293,
132.525864401898));
#278230=CARTESIAN_POINT('Ctrl Pts',(-10.2549940195371,-1.55185060416301,
136.404698919952));
#278231=CARTESIAN_POINT('Ctrl Pts',(-10.53344164335,3.87291006601234,135.137096129849));
#278232=CARTESIAN_POINT('Ctrl Pts',(-10.8118892671629,5.7386555876974,129.887921069854));
#278233=CARTESIAN_POINT('Ctrl Pts',(-11.0903368909758,2.33085697319978,
125.480909183646));
#278234=CARTESIAN_POINT('Ctrl Pts',(-11.3687845147887,-3.21888533097506,
125.965889100148));
#278235=CARTESIAN_POINT('Ctrl Pts',(-11.6472321386015,-5.81062926727439,
130.897187968684));
#278236=CARTESIAN_POINT('Ctrl Pts',(-11.9256797624145,-3.06268877196916,
135.743183036409));
#278237=CARTESIAN_POINT('Ctrl Pts',(-12.2041273862274,2.49971308411117,
136.050641576106));
#278238=CARTESIAN_POINT('Ctrl Pts',(-12.4825750100403,5.76500073366654,
131.537024209977));
#278239=CARTESIAN_POINT('Ctrl Pts',(-12.7610226338531,3.73253434492532,
126.350124795028));
#278240=CARTESIAN_POINT('Ctrl Pts',(-13.039470257666,-1.7299487623625,125.256450499474));
#278241=CARTESIAN_POINT('Ctrl Pts',(-13.3179178814789,-5.60269346973446,
129.261034571969));
#278242=CARTESIAN_POINT('Ctrl Pts',(-13.5963655052918,-4.32683658521273,
134.683859884699));
#278243=CARTESIAN_POINT('Ctrl Pts',(-13.8748131291047,0.925171743400955,
136.541614895008));
#278244=CARTESIAN_POINT('Ctrl Pts',(-14.1532607529176,5.3269924369816,133.127113504801));
#278245=CARTESIAN_POINT('Ctrl Pts',(-14.4317083767304,4.83356731902416,
127.578115684011));
#278246=CARTESIAN_POINT('Ctrl Pts',(-14.7101560005434,-0.101670032225581,
124.99387934633));
#278247=CARTESIAN_POINT('Ctrl Pts',(-14.9886036243562,-4.94347759071707,
127.749191439124));
#278248=CARTESIAN_POINT('Ctrl Pts',(-15.2670512481692,-5.24247074564602,
133.312054753593));
#278249=CARTESIAN_POINT('Ctrl Pts',(-15.545498871982,-0.723889394260118,
136.570469664722));
#278250=CARTESIAN_POINT('Ctrl Pts',(-15.823946495795,4.45991094648802,134.530112051601));
#278251=CARTESIAN_POINT('Ctrl Pts',(-16.1023941196078,5.54527100617588,
129.065970883678));
#278252=CARTESIAN_POINT('Ctrl Pts',(-16.3808417434207,1.53479791273714,
125.199324956138));
#278253=CARTESIAN_POINT('Ctrl Pts',(-16.6592893672336,-3.88607948346057,
126.483432980235));
#278254=CARTESIAN_POINT('Ctrl Pts',(-16.9377369910465,-5.73583967989507,
131.738262413989));
#278255=CARTESIAN_POINT('Ctrl Pts',(-17.2161846148594,-2.31464342185212,
136.134881720468));
#278256=CARTESIAN_POINT('Ctrl Pts',(-17.4946322386723,3.23359706425542,
135.633012543814));
#278257=CARTESIAN_POINT('Ctrl Pts',(-17.7730798624852,5.81031981831091,
130.693848139697));
#278258=CARTESIAN_POINT('Ctrl Pts',(-18.0515274862981,3.04764250924188,
125.856239303907));
#278259=CARTESIAN_POINT('Ctrl Pts',(-18.3299751101109,-2.51566938020671,
125.565712226204));
#278260=CARTESIAN_POINT('Ctrl Pts',(-18.6084227339239,-5.76720400652691,
130.089247097961));
#278261=CARTESIAN_POINT('Ctrl Pts',(-18.8868703577367,-3.71895989442774,
135.269936358996));
#278262=CARTESIAN_POINT('Ctrl Pts',(-19.1653179815497,1.74682667935956,
136.346979669161));
#278263=CARTESIAN_POINT('Ctrl Pts',(-19.4437656053625,5.60736487204277,
132.330626842902));
#278264=CARTESIAN_POINT('Ctrl Pts',(-19.7222132291754,4.31500868232164,
126.91170991781));
#278265=CARTESIAN_POINT('Ctrl Pts',(-20.0006608529883,-0.942629686559699,
125.069948819234));
#278266=CARTESIAN_POINT('Ctrl Pts',(-20.2791084768012,-5.33403742351306,
128.497832021735));
#278267=CARTESIAN_POINT('Ctrl Pts',(-20.5575561006141,-4.82372535047263,
134.045302323618));
#278268=CARTESIAN_POINT('Ctrl Pts',(-20.836003724427,0.119354667568119,
136.614505526443));
#278269=CARTESIAN_POINT('Ctrl Pts',(-21.1144513482399,4.95275357691331,
133.844469399368));
#278270=CARTESIAN_POINT('Ctrl Pts',(-21.3928989720528,5.23481390453873,
128.280721819388));
#278271=CARTESIAN_POINT('Ctrl Pts',(-21.6713465958657,0.706335988769417,
125.036075008324));
#278272=CARTESIAN_POINT('Ctrl Pts',(-21.9497942196786,-4.47123019424771,
127.092200875735));
#278273=CARTESIAN_POINT('Ctrl Pts',(-22.2282418434914,-5.53995426048939,
132.559620196804));
#278274=CARTESIAN_POINT('Ctrl Pts',(-22.5066894673044,-1.5177310031529,
136.41404171375));
#278275=CARTESIAN_POINT('Ctrl Pts',(-22.7851370911172,3.89921290079955,
135.11344035146));
#278276=CARTESIAN_POINT('Ctrl Pts',(-23.0635847149301,5.73297063605735,
129.853005223969));
#278277=CARTESIAN_POINT('Ctrl Pts',(-23.342032338743,2.298408427964,125.466819226899));
#278278=CARTESIAN_POINT('Ctrl Pts',(-23.6204799625559,-3.24827884193431,
125.985573014458));
#278279=CARTESIAN_POINT('Ctrl Pts',(-23.8989275863688,-5.80995654333829,
130.932557198412));
#278280=CARTESIAN_POINT('Ctrl Pts',(-24.1773752101816,-3.03256801357094,
135.761734987319));
#278281=CARTESIAN_POINT('Ctrl Pts',(-24.4558228339946,2.53160237148462,
136.035327911625));
#278282=CARTESIAN_POINT('Ctrl Pts',(-24.7342704578075,5.76935385279724,
131.501917439649));
#278283=CARTESIAN_POINT('Ctrl Pts',(-25.0127180816204,3.70535099199371,
126.327486325724));
#278284=CARTESIAN_POINT('Ctrl Pts',(-25.2911657054332,-1.76368841399288,
125.267083978533));
#278285=CARTESIAN_POINT('Ctrl Pts',(-25.5696133292462,-5.61198432848891,
129.295168351611));
#278286=CARTESIAN_POINT('Ctrl Pts',(-25.8480609530591,-4.30314080577957,
134.71012668896));
#278287=CARTESIAN_POINT('Ctrl Pts',(-26.1265085768719,0.960078897325804,
136.535876813977));
#278288=CARTESIAN_POINT('Ctrl Pts',(-26.4049562006848,5.3410329962505,133.094643554625));
#278289=CARTESIAN_POINT('Ctrl Pts',(-26.6834038244978,4.81383869558843,
127.548752162656));
#278290=CARTESIAN_POINT('Ctrl Pts',(-26.9618514483106,-0.137038197225328,
124.994605895435));
#278291=CARTESIAN_POINT('Ctrl Pts',(-27.2402990721235,-4.96198368147699,
127.779340395554));
#278292=CARTESIAN_POINT('Ctrl Pts',(-27.5187466959364,-5.22710856883054,
133.343920699249));
#278293=CARTESIAN_POINT('Ctrl Pts',(-27.7971943197493,-0.688776039878604,
136.574769352283));
#278294=CARTESIAN_POINT('Ctrl Pts',(-28.0756419435621,4.48250802114168,
134.502894278251));
#278295=CARTESIAN_POINT('Ctrl Pts',(-28.3540895673751,5.53458619342344,
129.032247453463));
#278296=CARTESIAN_POINT('Ctrl Pts',(-28.632537191188,1.50065003351598,125.190086053944));
#278297=CARTESIAN_POINT('Ctrl Pts',(-28.9109848150008,-3.91231019636288,
126.507168705834));
#278298=CARTESIAN_POINT('Ctrl Pts',(-29.1894324388138,-5.73004848276283,
131.773160795109));
#278299=CARTESIAN_POINT('Ctrl Pts',(-29.4678800626266,-2.28215214193419,
136.148872849742));
#278300=CARTESIAN_POINT('Ctrl Pts',(-29.7463276864396,3.26293052800175,
135.613239256942));
#278301=CARTESIAN_POINT('Ctrl Pts',(-30.0247753102524,5.80953944572202,
130.658481121338));
#278302=CARTESIAN_POINT('Ctrl Pts',(-30.3032229340653,3.01746542460398,
125.837779116156));
#278303=CARTESIAN_POINT('Ctrl Pts',(-30.5816705578782,-2.54751191034413,
125.581122879776));
#278304=CARTESIAN_POINT('Ctrl Pts',(-30.8601181816911,-5.77145025256159,
130.124366955075));
#278305=CARTESIAN_POINT('Ctrl Pts',(-31.138565805504,-3.69170776369427,
135.292491986665));
#278306=CARTESIAN_POINT('Ctrl Pts',(-31.4170134293169,1.78053381005746,
136.336243547461));
#278307=CARTESIAN_POINT('Ctrl Pts',(-31.6954610531298,5.6165517962788,132.296464943187));
#278308=CARTESIAN_POINT('Ctrl Pts',(-31.9739086769427,4.29123306552915,
126.885515357016));
#278309=CARTESIAN_POINT('Ctrl Pts',(-32.2523563007555,-0.977519214052166,
125.075793119056));
#278310=CARTESIAN_POINT('Ctrl Pts',(-32.5308039245685,-5.34797909038788,
128.530344556146));
#278311=CARTESIAN_POINT('Ctrl Pts',(-32.8092515483813,-4.80390744596015,
134.07460566182));
#278312=CARTESIAN_POINT('Ctrl Pts',(-33.0876991721943,0.154720457379397,
136.613671332177));
#278313=CARTESIAN_POINT('Ctrl Pts',(-33.3661467960071,4.9711678189017,133.814264256411));
#278314=CARTESIAN_POINT('Ctrl Pts',(-33.64459441982,5.21935480990263,128.248902778514));
#278315=CARTESIAN_POINT('Ctrl Pts',(-33.9230420436329,0.671209710260644,
125.031882213649));
#278316=CARTESIAN_POINT('Ctrl Pts',(-34.2014896674458,-4.49374432269368,
127.119487300736));
#278317=CARTESIAN_POINT('Ctrl Pts',(-34.4799372912587,-5.52916685470707,
132.59331094992));
#278318=CARTESIAN_POINT('Ctrl Pts',(-34.7583849150716,-1.48355516206214,
136.423176638752));
#278319=CARTESIAN_POINT('Ctrl Pts',(-35.0368325388844,3.92537124881898,
135.089624898536));
#278320=CARTESIAN_POINT('Ctrl Pts',(-35.3152801626974,5.72707324708195,
129.818124630907));
#278321=CARTESIAN_POINT('Ctrl Pts',(-35.5937277865103,2.26587471435868,
125.45292705471));
#278322=CARTESIAN_POINT('Ctrl Pts',(-35.8721754103231,-3.27755198672651,
126.005435490714));
#278323=CARTESIAN_POINT('Ctrl Pts',(-36.1506230341361,-5.80906852932597,
130.967921677768));
#278324=CARTESIAN_POINT('Ctrl Pts',(-36.4290706579489,-3.00233488224952,
135.780103240898));
#278325=CARTESIAN_POINT('Ctrl Pts',(-36.7075182817618,2.56339784940132,
136.019820411726));
#278326=CARTESIAN_POINT('Ctrl Pts',(-36.9859659055747,5.77349318639923,
131.466784821096));
#278327=CARTESIAN_POINT('Ctrl Pts',(-37.2644135293876,3.67803033591843,
126.305013748643));
#278328=CARTESIAN_POINT('Ctrl Pts',(-37.5428611532005,-1.79736271150026,
125.277922643415));
#278329=CARTESIAN_POINT('Ctrl Pts',(-37.8213087770133,-5.62106723310019,
129.329358054928));
#278330=CARTESIAN_POINT('Ctrl Pts',(-38.0997564008263,-4.27928557188161,
134.736248763623));
#278331=CARTESIAN_POINT('Ctrl Pts',(-38.3782040246392,0.994950475174061,
136.529926349506));
#278332=CARTESIAN_POINT('Ctrl Pts',(-38.656651648452,5.35487564157755,133.062088737171));
#278333=CARTESIAN_POINT('Ctrl Pts',(-38.9350992722649,4.79393169358958,
127.51950927907));
#278334=CARTESIAN_POINT('Ctrl Pts',(-39.2135468960779,-0.172401284224016,
124.995547727136));
#278335=CARTESIAN_POINT('Ctrl Pts',(-39.4919945198907,-4.98030590410683,
127.809601445221));
#278336=CARTESIAN_POINT('Ctrl Pts',(-39.7704421437036,-5.21155269958477,
133.375692540572));
#278337=CARTESIAN_POINT('Ctrl Pts',(-40.0488897675166,-0.65363716264763,
136.578855215227));
#278338=CARTESIAN_POINT('Ctrl Pts',(-40.3273373913294,4.50493899481217,
134.475539454375));
#278339=CARTESIAN_POINT('Ctrl Pts',(-40.6057850151423,5.52369629454426,
128.998589689552));
#278340=CARTESIAN_POINT('Ctrl Pts',(-40.8842326389552,1.46644654715595,
125.181055190758));
#278341=CARTESIAN_POINT('Ctrl Pts',(-41.1626802627681,-3.93839593717207,
126.531063665459));
#278342=CARTESIAN_POINT('Ctrl Pts',(-41.441127886581,-5.72404495657686,
131.808023276983));
#278343=CARTESIAN_POINT('Ctrl Pts',(-41.7195755103939,-2.24957629602936,
136.162665936149));
#278344=CARTESIAN_POINT('Ctrl Pts',(-41.9980231342068,3.29214308265742,
135.593287775304));
#278345=CARTESIAN_POINT('Ctrl Pts',(-42.2764707580197,5.80854379851262,
130.623119508596));
#278346=CARTESIAN_POINT('Ctrl Pts',(-42.5549183818325,2.98717652667487,
125.81950296691));
#278347=CARTESIAN_POINT('Ctrl Pts',(-42.8333660056454,-2.57926004149102,
125.596727082342));
#278348=CARTESIAN_POINT('Ctrl Pts',(-43.1118136294584,-5.7754826353847,
130.159512009603));
#278349=CARTESIAN_POINT('Ctrl Pts',(-43.3902612532712,-3.66431883537201,
135.314881304976));
#278350=CARTESIAN_POINT('Ctrl Pts',(-43.6687088770841,1.81417496242045,
136.325302439805));
#278351=CARTESIAN_POINT('Ctrl Pts',(-43.947156500897,5.62553059712261,132.262247752997));
#278352=CARTESIAN_POINT('Ctrl Pts',(-44.2256041247099,4.26729843551711,
126.859466010475));
#278353=CARTESIAN_POINT('Ctrl Pts',(-44.5040517485228,-1.01237251921066,
125.081849693053));
#278354=CARTESIAN_POINT('Ctrl Pts',(-44.7824993723357,-5.3617225859308,
128.562941355057));
#278355=CARTESIAN_POINT('Ctrl Pts',(-45.0609469961486,-4.78391153089065,
134.103787819889));
#278356=CARTESIAN_POINT('Ctrl Pts',(-45.3393946199614,0.190080513966956,
136.612621871764));
#278357=CARTESIAN_POINT('Ctrl Pts',(-45.6178422437743,4.98939785243841,
133.783947580368));
#278358=CARTESIAN_POINT('Ctrl Pts',(-45.8962898675873,5.20370231015464,
128.217178431071));
#278359=CARTESIAN_POINT('Ctrl Pts',(-46.1747374914001,0.636058559829223,
125.027903320286));
#278360=CARTESIAN_POINT('Ctrl Pts',(-46.453185115213,-4.51609193379101,
127.146910270074));
#278361=CARTESIAN_POINT('Ctrl Pts',(-46.7316327390259,-5.51817456361365,
132.626935412823));
#278362=CARTESIAN_POINT('Ctrl Pts',(-47.0100803628388,-1.4493243472895,
136.43210335646));
#278363=CARTESIAN_POINT('Ctrl Pts',(-47.2885279866517,3.95138414076325,
135.06565065357));
#278364=CARTESIAN_POINT('Ctrl Pts',(-47.5669756104645,5.72096363930122,
129.783280583183));
#278365=CARTESIAN_POINT('Ctrl Pts',(-47.8454232342775,2.23325703793269,
125.439233181862));
#278366=CARTESIAN_POINT('Ctrl Pts',(-48.1238708580903,-3.30670368062431,
126.025475792906));
#278367=CARTESIAN_POINT('Ctrl Pts',(-48.4023184819033,-5.80796525814313,
131.00328009631));
#278368=CARTESIAN_POINT('Ctrl Pts',(-48.6807661057162,-2.97199049830493,
135.798287116504));
#278369=CARTESIAN_POINT('Ctrl Pts',(-48.9592137295291,2.59509833966803,
136.004119651047));
#278370=CARTESIAN_POINT('Ctrl Pts',(-49.2376613533419,5.77741858108801,
131.431627656171));
#278371=CARTESIAN_POINT('Ctrl Pts',(-49.5161089771548,3.65057338907646,
126.282707896514));
#278372=CARTESIAN_POINT('Ctrl Pts',(-49.7945566009678,-1.8309704070716,
125.288966092489));
#278373=CARTESIAN_POINT('Ctrl Pts',(-50.0730042247805,-5.62994184699806,
129.363602415007));
#278374=CARTESIAN_POINT('Ctrl Pts',(-50.3514518485936,-4.25527176748286,
134.762225140725));
#278375=CARTESIAN_POINT('Ctrl Pts',(-50.6298994724063,1.02978518476655,
136.52376372209));
#278376=CARTESIAN_POINT('Ctrl Pts',(-50.9083470962193,5.36851986001845,
133.029450258773));
#278377=CARTESIAN_POINT('Ctrl Pts',(-51.1867947200322,4.77384705068883,
127.490388116857));
#278378=CARTESIAN_POINT('Ctrl Pts',(-51.465242343845,-0.207757982829986,
124.996704806535));
#278379=CARTESIAN_POINT('Ctrl Pts',(-51.743689967658,-4.99844357966987,
127.839973466791));
#278380=CARTESIAN_POINT('Ctrl Pts',(-52.0221375914708,-5.19580371433717,
133.407369100245));
#278381=CARTESIAN_POINT('Ctrl Pts',(-52.3005852152837,-0.618474064651215,
136.58272710215));
#278382=CARTESIAN_POINT('Ctrl Pts',(-52.5790328390967,4.52720303631132,
134.448048593619));
#278383=CARTESIAN_POINT('Ctrl Pts',(-52.8574804629095,5.51260171306762,
128.964998839148));
#278384=CARTESIAN_POINT('Ctrl Pts',(-53.1359280867224,1.43218872108006,
125.172232701224));
#278385=CARTESIAN_POINT('Ctrl Pts',(-53.4143757105353,-3.96433573927151,
126.555116973674));
#278386=CARTESIAN_POINT('Ctrl Pts',(-53.6928233343482,-5.71782932379997,
131.842848567767));
#278387=CARTESIAN_POINT('Ctrl Pts',(-53.9712709581611,-2.21691709124776,
136.176260468582));
#278388=CARTESIAN_POINT('Ctrl Pts',(-54.249718581974,3.32123364574025,135.573158838211));
#278389=CARTESIAN_POINT('Ctrl Pts',(-54.5281662057869,5.80733291357678,
130.58776461181));
#278390=CARTESIAN_POINT('Ctrl Pts',(-54.8066138295998,2.95677693782102,
125.801411533396));
#278391=CARTESIAN_POINT('Ctrl Pts',(-55.0850614534126,-2.61091259720856,
125.612524255684));
#278392=CARTESIAN_POINT('Ctrl Pts',(-55.3635090772256,-5.77930100557468,
130.194680959234));
#278393=CARTESIAN_POINT('Ctrl Pts',(-55.6419567010384,-3.63679412436797,
135.337103484283));
#278394=CARTESIAN_POINT('Ctrl Pts',(-55.9204043248514,1.8477488898629,136.314156751619));
#278395=CARTESIAN_POINT('Ctrl Pts',(-56.1988519486642,5.63430094186134,
132.227976540264));
#278396=CARTESIAN_POINT('Ctrl Pts',(-56.4772995724772,4.24320567919224,
126.833562843453));
#278397=CARTESIAN_POINT('Ctrl Pts',(-56.7557471962901,-1.04718831053316,
125.088118316796));
#278398=CARTESIAN_POINT('Ctrl Pts',(-57.0341948201028,-5.3752674008715,
128.595621210585));
#278399=CARTESIAN_POINT('Ctrl Pts',(-57.3126424439159,-4.76373834622006,
134.13284771647));
#278400=CARTESIAN_POINT('Ctrl Pts',(-57.5910900677287,0.225433527051438,
136.611357184097));
#278401=CARTESIAN_POINT('Ctrl Pts',(-57.8695376915416,5.00744300200284,
133.753520494635));
#278402=CARTESIAN_POINT('Ctrl Pts',(-58.1479853153544,5.18785698530388,
128.185549952615));
#278403=CARTESIAN_POINT('Ctrl Pts',(-58.4264329391674,0.600883840013963,
125.024138475672));
#278404=CARTESIAN_POINT('Ctrl Pts',(-58.7048805629802,-4.53827219944114,
127.174468767579));
#278405=CARTESIAN_POINT('Ctrl Pts',(-58.9833281867932,-5.5069777945324,
132.660492339548));
#278406=CARTESIAN_POINT('Ctrl Pts',(-59.261775810606,-1.41503982726995,
136.440821536091));
#278407=CARTESIAN_POINT('Ctrl Pts',(-59.540223434419,3.97725061271504,135.041518504932));
#278408=CARTESIAN_POINT('Ctrl Pts',(-59.8186710582318,5.71464203910897,
129.748474371954));
#278409=CARTESIAN_POINT('Ctrl Pts',(-60.0971186820448,2.20055660734573,
125.425738115783));
#278410=CARTESIAN_POINT('Ctrl Pts',(-60.3755663058576,-3.3357328434014,
126.045693178431));
#278411=CARTESIAN_POINT('Ctrl Pts',(-60.6540139296705,-5.80664677067165,
131.038631143817));
#278412=CARTESIAN_POINT('Ctrl Pts',(-60.9324615534834,-2.94153598615947,
135.816285940328));
#278413=CARTESIAN_POINT('Ctrl Pts',(-61.2109091772963,2.62670266761142,
135.988226211385));
#278414=CARTESIAN_POINT('Ctrl Pts',(-61.4893568011092,5.78112989140647,
131.396447247635));
#278415=CARTESIAN_POINT('Ctrl Pts',(-61.767804424922,3.62298116889529,126.260569595891));
#278416=CARTESIAN_POINT('Ctrl Pts',(-62.046252048735,-1.86451025536104,
125.300213916535));
#278417=CARTESIAN_POINT('Ctrl Pts',(-62.3246996725479,-5.63860784133039,
129.39790016291));
#278418=CARTESIAN_POINT('Ctrl Pts',(-62.6031472963608,-4.23110028242386,
134.788054857702));
#278419=CARTESIAN_POINT('Ctrl Pts',(-62.8815949201736,1.0645817352901,136.517389160091));
#278420=CARTESIAN_POINT('Ctrl Pts',(-63.1600425439866,5.38196514598156,
132.99672932886));
#278421=CARTESIAN_POINT('Ctrl Pts',(-63.4384901677994,4.75358551113023,
127.461389755115));
#278422=CARTESIAN_POINT('Ctrl Pts',(-63.7169377916123,-0.243106982887504,
124.998077090756));
#278423=CARTESIAN_POINT('Ctrl Pts',(-63.9953854154252,-5.0163960360679,
127.870455334816));
#278424=CARTESIAN_POINT('Ctrl Pts',(-64.2738330392381,-5.17986219667218,
133.438949204482));
#278425=CARTESIAN_POINT('Ctrl Pts',(-64.552280663051,-0.583288048870894,
136.586384869579));
#278426=CARTESIAN_POINT('Ctrl Pts',(-64.8307282868638,4.54929932063727,
134.420422714664));
#278427=CARTESIAN_POINT('Ctrl Pts',(-65.1091759106768,5.50130286010717,
128.93147614697));
#278428=CARTESIAN_POINT('Ctrl Pts',(-65.3876235344896,1.39787782472419,
125.16361891226));
#278429=CARTESIAN_POINT('Ctrl Pts',(-65.6660711583025,-3.99012864145221,
126.579327739175));
#278430=CARTESIAN_POINT('Ctrl Pts',(-65.9445187821156,-5.71140181475477,
131.877635376998));
#278431=CARTESIAN_POINT('Ctrl Pts',(-66.2229664059283,-2.18417573778792,
136.189655943291));
#278432=CARTESIAN_POINT('Ctrl Pts',(-66.5014140297413,3.35020113928917,
135.552853191544));
#278433=CARTESIAN_POINT('Ctrl Pts',(-66.7798616535541,5.80590683578406,
130.552417741069));
#278434=CARTESIAN_POINT('Ctrl Pts',(-67.0583092773671,2.92626778451039,
125.783505486001));
#278435=CARTESIAN_POINT('Ctrl Pts',(-67.3367569011799,-2.64246840459962,
125.628513814431));
#278436=CARTESIAN_POINT('Ctrl Pts',(-67.6152045249929,-5.78290522164069,
130.229872500769));
#278437=CARTESIAN_POINT('Ctrl Pts',(-67.8936521488056,-3.60913465062,135.359157701137));
#278438=CARTESIAN_POINT('Ctrl Pts',(-68.1720997726187,1.88125434829088,
136.302806895912));
#278439=CARTESIAN_POINT('Ctrl Pts',(-68.4505473964314,5.64286250550667,
132.193652574919));
#278440=CARTESIAN_POINT('Ctrl Pts',(-68.7289950202444,4.21895568932047,
126.807806815805));
#278441=CARTESIAN_POINT('Ctrl Pts',(-69.0074426440573,-1.08196529790749,
125.094598758));
#278442=CARTESIAN_POINT('Ctrl Pts',(-69.2858902678701,-5.38861303330182,
128.628382911763));
#278443=CARTESIAN_POINT('Ctrl Pts',(-69.564337891683,-4.74338863947339,
134.161784274737));
#278444=CARTESIAN_POINT('Ctrl Pts',(-69.8427855154959,0.260778186613682,
136.609877316035));
#278445=CARTESIAN_POINT('Ctrl Pts',(-70.1212331393089,5.02530259892534,
133.722984126697));
#278446=CARTESIAN_POINT('Ctrl Pts',(-70.3996807631217,5.17181942250469,
128.154018515153));
#278447=CARTESIAN_POINT('Ctrl Pts',(-70.6781283869345,0.5656868542273,125.020587819316));
#278448=CARTESIAN_POINT('Ctrl Pts',(-70.9565760107477,-4.56028429774593,
127.202161772061));
#278449=CARTESIAN_POINT('Ctrl Pts',(-71.2350236345604,-5.49557696236377,
132.693980486629));
#278450=CARTESIAN_POINT('Ctrl Pts',(-71.5134712583732,-1.38070287242923,
136.449330854589));
#278451=CARTESIAN_POINT('Ctrl Pts',(-71.7919188821862,4.00296970618273,
135.017229346852));
#278452=CARTESIAN_POINT('Ctrl Pts',(-72.0703665059991,5.70810868075446,
129.71370728698));
#278453=CARTESIAN_POINT('Ctrl Pts',(-72.348814129812,2.16777463432419,125.412442356538));
#278454=CARTESIAN_POINT('Ctrl Pts',(-72.6272617536249,-3.36463839937136,
126.06608689813));
#278455=CARTESIAN_POINT('Ctrl Pts',(-72.9057093774378,-5.80511311576878,
131.073973510343));
#278456=CARTESIAN_POINT('Ctrl Pts',(-73.1841570012506,-2.91097247431594,
135.834099045416));
#278457=CARTESIAN_POINT('Ctrl Pts',(-73.4626046250635,2.65820966212185,
135.972140681676));
#278458=CARTESIAN_POINT('Ctrl Pts',(-73.7410522488765,5.78462697983096,
131.361244899111));
#278459=CARTESIAN_POINT('Ctrl Pts',(-74.0194998726893,3.59525469781404,
126.238599667113));
#278460=CARTESIAN_POINT('Ctrl Pts',(-74.2979474965022,-1.89798101353784,
125.31166569876));
#278461=CARTESIAN_POINT('Ctrl Pts',(-74.5763951203151,-5.64706489497548,
129.432250027724));
#278462=CARTESIAN_POINT('Ctrl Pts',(-74.854842744128,-4.20677201238788,
134.813736957424));
#278463=CARTESIAN_POINT('Ctrl Pts',(-75.1332903679409,1.09933883734644,
136.510802899716));
#278464=CARTESIAN_POINT('Ctrl Pts',(-75.4117379917539,5.39521100124704,
132.963927159917));
#278465=CARTESIAN_POINT('Ctrl Pts',(-75.6901856155667,4.73314782571214,
127.432515268386));
#278466=CARTESIAN_POINT('Ctrl Pts',(-75.9686332393795,-0.278446974526432,
124.99966452895));
#278467=CARTESIAN_POINT('Ctrl Pts',(-76.2470808631926,-5.03416260806588,
127.901045919781));
#278468=CARTESIAN_POINT('Ctrl Pts',(-76.5255284870053,-5.16372873730878,
133.470431683069));
#278469=CARTESIAN_POINT('Ctrl Pts',(-76.8039761108183,-0.548080419137594,
136.589828381972));
#278470=CARTESIAN_POINT('Ctrl Pts',(-77.0824237346311,4.57122702900371,
134.392662841198));
#278471=CARTESIAN_POINT('Ctrl Pts',(-77.360871358444,5.48980015434633,128.898022855216));
#278472=CARTESIAN_POINT('Ctrl Pts',(-77.639318982257,1.36351512949127,125.155214143056));
#278473=CARTESIAN_POINT('Ctrl Pts',(-77.9177666060698,-4.0157736879487,
126.603695064822));
#278474=CARTESIAN_POINT('Ctrl Pts',(-78.1962142298826,-5.70476266761487,
131.91238241564));
#278475=CARTESIAN_POINT('Ctrl Pts',(-78.4746618536957,-2.15135344889296,
136.202851863901));
#278476=CARTESIAN_POINT('Ctrl Pts',(-78.7531094775085,3.37904448990285,
135.532371587738));
#278477=CARTESIAN_POINT('Ctrl Pts',(-79.0315571013213,5.8042656179783,130.517080206165));
#278478=CARTESIAN_POINT('Ctrl Pts',(-79.3100047251342,2.8956501972711,125.765785488239));
#278479=CARTESIAN_POINT('Ctrl Pts',(-79.5884523489472,-2.67392629435197,
125.644695166086));
#278480=CARTESIAN_POINT('Ctrl Pts',(-79.8668999727601,-5.78629515002701,
130.265085330171));
#278481=CARTESIAN_POINT('Ctrl Pts',(-80.1453475965729,-3.58134143906054,
135.38104313831));
#278482=CARTESIAN_POINT('Ctrl Pts',(-80.4237952203859,1.91469009614739,
136.291253293255));
#278483=CARTESIAN_POINT('Ctrl Pts',(-80.7022428441988,5.65121497080658,
132.15927712885));
#278484=CARTESIAN_POINT('Ctrl Pts',(-80.9806904680116,4.19454936449412,
126.782198881926));
#278485=CARTESIAN_POINT('Ctrl Pts',(-81.2591380918246,-1.11670219266007,
125.10129077653));
#278486=CARTESIAN_POINT('Ctrl Pts',(-81.5375857156372,-5.40175898869456,
128.661225244595));
#278487=CARTESIAN_POINT('Ctrl Pts',(-81.8160333394505,-4.72286316471603,
134.190596422436));
#278488=CARTESIAN_POINT('Ctrl Pts',(-82.0944809632629,0.296113182944105,
136.608182322418));
#278489=CARTESIAN_POINT('Ctrl Pts',(-82.3729285870762,5.04297598141181,
133.692339608092));
#278490=CARTESIAN_POINT('Ctrl Pts',(-82.6513762108889,5.15559021603496,
128.122585287091));
#278491=CARTESIAN_POINT('Ctrl Pts',(-82.9298238347018,0.530468906706182,
125.017251482786));
#278492=CARTESIAN_POINT('Ctrl Pts',(-83.2082714585147,-4.58212741303929,
127.229988257347));
#278493=CARTESIAN_POINT('Ctrl Pts',(-83.4867190823277,-5.48397248956967,
132.72739861315));
#278494=CARTESIAN_POINT('Ctrl Pts',(-83.7651667061405,-1.34631475513585,
136.45763099664));
#278495=CARTESIAN_POINT('Ctrl Pts',(-84.0436143299535,4.02854046813582,
134.992784079373));
#278496=CARTESIAN_POINT('Ctrl Pts',(-84.3220619537663,5.70136380633342,
129.678980616565));
#278497=CARTESIAN_POINT('Ctrl Pts',(-84.6005095775792,2.13491233361711,
125.399346396808));
#278498=CARTESIAN_POINT('Ctrl Pts',(-84.8789572013921,-3.39341927742779,
126.086656196302));
#278499=CARTESIAN_POINT('Ctrl Pts',(-85.1574048252049,-5.80336435026449,
131.109305886265));
#278500=CARTESIAN_POINT('Ctrl Pts',(-85.4358524490179,-2.88030109531746,
135.851725771696));
#278501=CARTESIAN_POINT('Ctrl Pts',(-85.7143000728307,2.68961815569484,
135.955863657977));
#278502=CARTESIAN_POINT('Ctrl Pts',(-85.9927476966438,5.78790971677558,
131.326021915035));
#278503=CARTESIAN_POINT('Ctrl Pts',(-86.2711953204564,3.56739500324825,
126.216798924288));
#278504=CARTESIAN_POINT('Ctrl Pts',(-86.5496429442695,-1.93138144132926,
125.323321014816));
#278505=CARTESIAN_POINT('Ctrl Pts',(-86.8280905680822,-5.65531269455438,
129.466650736599));
#278506=CARTESIAN_POINT('Ctrl Pts',(-87.1065381918953,-4.18228785886808,
134.83927048823));
#278507=CARTESIAN_POINT('Ctrl Pts',(-87.3849858157081,1.13405520299706,
136.504005185026));
#278508=CARTESIAN_POINT('Ctrl Pts',(-87.663433439521,5.40825693498488,132.931044967442));
#278509=CARTESIAN_POINT('Ctrl Pts',(-87.9418810633338,4.71253475176078,
127.403765726628));
#278510=CARTESIAN_POINT('Ctrl Pts',(-88.2203286871468,-0.313776648210234,
125.00146706229));
#278511=CARTESIAN_POINT('Ctrl Pts',(-88.4987763109598,-5.05174263731727,
127.931744088139));
#278512=CARTESIAN_POINT('Ctrl Pts',(-88.7772239347726,-5.14740393407785,
133.501815369412));
#278513=CARTESIAN_POINT('Ctrl Pts',(-89.0556715585855,-0.512852480082647,
136.593057511728));
#278514=CARTESIAN_POINT('Ctrl Pts',(-89.3341191823985,4.59298534887173,
134.364770001874));
#278515=CARTESIAN_POINT('Ctrl Pts',(-89.6125668062112,5.47809402202166,
128.864640203508));
#278516=CARTESIAN_POINT('Ctrl Pts',(-89.8910144300243,1.32910190870433,
125.147018705051));
#278517=CARTESIAN_POINT('Ctrl Pts',(-90.169462053837,-4.04126992847403,
126.628218047677));
#278518=CARTESIAN_POINT('Ctrl Pts',(-90.44790967765,-5.69791212839678,131.947088396125));
#278519=CARTESIAN_POINT('Ctrl Pts',(-90.7263573014627,-2.1184514408047,
136.215847741432));
#278520=CARTESIAN_POINT('Ctrl Pts',(-91.0048049252757,3.40776262878029,
135.511714785749));
#278521=CARTESIAN_POINT('Ctrl Pts',(-91.2832525490887,5.80240932097568,
130.48175331654));
#278522=CARTESIAN_POINT('Ctrl Pts',(-91.5617001729014,2.86492531064864,
125.748252196732));
#278523=CARTESIAN_POINT('Ctrl Pts',(-91.8401477967144,-2.70528510078237,
125.661067711041));
#278524=CARTESIAN_POINT('Ctrl Pts',(-92.1185954205271,-5.78947066511866,
130.30031814262));
#278525=CARTESIAN_POINT('Ctrl Pts',(-92.3970430443404,-3.55341551957677,
135.402758984829));
#278526=CARTESIAN_POINT('Ctrl Pts',(-92.6754906681528,1.94805489445803,
136.279496371773));
#278527=CARTESIAN_POINT('Ctrl Pts',(-92.9539382919661,5.6593580282576,132.124851475851));
#278528=CARTESIAN_POINT('Ctrl Pts',(-93.2323859157787,4.16998760909852,
126.75673999073));
#278529=CARTESIAN_POINT('Ctrl Pts',(-93.5108335395918,-1.15139770760221,
125.10819412441));
#278530=CARTESIAN_POINT('Ctrl Pts',(-93.7892811634045,-5.41470477992152,
128.694146992097));
#278531=CARTESIAN_POINT('Ctrl Pts',(-94.0677287872175,-4.70216268252734,
134.219283091922));
#278532=CARTESIAN_POINT('Ctrl Pts',(-94.3461764110305,0.331437206691851,
136.606272266052));
#278533=CARTESIAN_POINT('Ctrl Pts',(-94.6246240348431,5.0604624945689,133.661588074364));
#278534=CARTESIAN_POINT('Ctrl Pts',(-94.9030716586564,5.13916996727372,
128.0912514332));
#278535=CARTESIAN_POINT('Ctrl Pts',(-95.1815192824688,0.495231302464415,
125.014129589715));
#278536=CARTESIAN_POINT('Ctrl Pts',(-95.459966906282,-4.60380073591605,
127.257947192314));
#278537=CARTESIAN_POINT('Ctrl Pts',(-95.7384145300948,-5.47216480615837,
132.760745480792));
#278538=CARTESIAN_POINT('Ctrl Pts',(-96.0168621539077,-1.31187674965409,
136.465721654678));
#278539=CARTESIAN_POINT('Ctrl Pts',(-96.2953097777207,4.05396195104042,
134.96818360832));
#278540=CARTESIAN_POINT('Ctrl Pts',(-96.5737574015334,5.69440766577999,
129.64429564752));
#278541=CARTESIAN_POINT('Ctrl Pts',(-96.8522050253465,2.10197092294792,
125.386450721867));
#278542=CARTESIAN_POINT('Ctrl Pts',(-97.1306526491593,-3.42207441108517,
126.107400310748));
#278543=CARTESIAN_POINT('Ctrl Pts',(-97.4091002729722,-5.80140053895979,
131.144626962327));
#278544=CARTESIAN_POINT('Ctrl Pts',(-97.6875478967851,-2.8495229857029,
135.869165466005));
#278545=CARTESIAN_POINT('Ctrl Pts',(-97.965995520598,2.72092698447821,135.93939574344));
#278546=CARTESIAN_POINT('Ctrl Pts',(-98.2444431444108,5.79097798059694,
131.290779600608));
#278547=CARTESIAN_POINT('Ctrl Pts',(-98.5228907682237,3.53940311754856,
126.195168175249));
#278548=CARTESIAN_POINT('Ctrl Pts',(-98.8013383920368,-1.96471030107164,
125.33517943281));
#278549=CARTESIAN_POINT('Ctrl Pts',(-99.0797860158496,-5.6633509344415,
129.501101014807));
#278550=CARTESIAN_POINT('Ctrl Pts',(-99.3582336396624,-4.15764872913354,
134.864654503967));
#278551=CARTESIAN_POINT('Ctrl Pts',(-99.6366812634755,1.16872954581563,
136.496996267908));
#278552=CARTESIAN_POINT('Ctrl Pts',(-99.9151288872883,5.42110246377302,
132.898083969897));
#278553=CARTESIAN_POINT('Ctrl Pts',(-100.193576511101,4.69174705310118,
127.375142195163));
#278554=CARTESIAN_POINT('Ctrl Pts',(-100.472024134914,-0.34909469478497,
125.003484623986));
#278555=CARTESIAN_POINT('Ctrl Pts',(-100.750471758727,-5.06913547238742,
127.96254870236));
#278556=CARTESIAN_POINT('Ctrl Pts',(-101.02891938254,-5.13088839190121,
133.533099100579));
#278557=CARTESIAN_POINT('Ctrl Pts',(-101.307367006353,-0.47760553709043,
136.596072139193));
#278558=CARTESIAN_POINT('Ctrl Pts',(-101.585814630166,4.61457347397855,
134.33674523027));
#278559=CARTESIAN_POINT('Ctrl Pts',(-101.864262253979,5.46618489690847,
128.831329428852));
#278560=CARTESIAN_POINT('Ctrl Pts',(-102.142709877791,1.29463943755703,
125.139032901931));
#278561=CARTESIAN_POINT('Ctrl Pts',(-102.421157501604,-4.06661641825637,
126.652895779031));
#278562=CARTESIAN_POINT('Ctrl Pts',(-102.699605125417,-5.69085045094906,
131.981752032413));
#278563=CARTESIAN_POINT('Ctrl Pts',(-102.97805274923,-2.08547093271925,
136.228643094318));
#278564=CARTESIAN_POINT('Ctrl Pts',(-103.256500373043,3.43635449176034,
135.490883551018));
#278565=CARTESIAN_POINT('Ctrl Pts',(-103.534947996856,5.80033801356182,
130.446438381249));
#278566=CARTESIAN_POINT('Ctrl Pts',(-103.813395620669,2.83409426316523,
125.730906261181));
#278567=CARTESIAN_POINT('Ctrl Pts',(-104.091843244482,-2.73654366187847,
125.677630842606));
#278568=CARTESIAN_POINT('Ctrl Pts',(-104.370290868295,-5.79243164924577,
130.335569632546));
#278569=CARTESIAN_POINT('Ctrl Pts',(-104.648738492108,-3.52535792697413,
135.424304436005));
#278570=CARTESIAN_POINT('Ctrl Pts',(-104.92718611592,1.98134750687769,136.267536567122));
#278571=CARTESIAN_POINT('Ctrl Pts',(-105.205633739733,5.66729137611554,
132.090376891579));
#278572=CARTESIAN_POINT('Ctrl Pts',(-105.484081363546,4.14527133327901,
126.731431085605));
#278573=CARTESIAN_POINT('Ctrl Pts',(-105.762528987359,-1.18605055707886,
125.115308545834));
#278574=CARTESIAN_POINT('Ctrl Pts',(-106.040976611172,-5.42744992727162,
128.72714693434));
#278575=CARTESIAN_POINT('Ctrl Pts',(-106.319424234985,-4.68128795997122,
134.247843220201));
#278576=CARTESIAN_POINT('Ctrl Pts',(-106.597871858798,0.366748948912009,
136.604147217717));
#278577=CARTESIAN_POINT('Ctrl Pts',(-106.876319482611,5.07776149042729,
133.630730665021));
#278578=CARTESIAN_POINT('Ctrl Pts',(-107.154767106424,5.12255928467941,
128.060018114567));
#278579=CARTESIAN_POINT('Ctrl Pts',(-107.433214730236,0.45997534724462,
125.011222255784));
#278580=CARTESIAN_POINT('Ctrl Pts',(-107.711662354049,-4.62530346326349,
127.286037540936));
#278581=CARTESIAN_POINT('Ctrl Pts',(-107.990109977862,-5.46015434966779,
132.794019853873));
#278582=CARTESIAN_POINT('Ctrl Pts',(-108.268557601675,-1.2773901320969,
136.473602528901));
#278583=CARTESIAN_POINT('Ctrl Pts',(-108.547005225488,4.07923321289408,
134.943428845277));
#278584=CARTESIAN_POINT('Ctrl Pts',(-108.825452849301,5.6872405168564,129.609653665109));
#278585=CARTESIAN_POINT('Ctrl Pts',(-109.103900473114,2.06895162297316,
125.373755809571));
#278586=CARTESIAN_POINT('Ctrl Pts',(-109.382348096927,-3.45060273851677,
126.128318472786));
#278587=CARTESIAN_POINT('Ctrl Pts',(-109.66079572074,-5.79922175462486,
131.179935429694));
#278588=CARTESIAN_POINT('Ctrl Pts',(-109.939243344552,-2.81863928596571,
135.886417482107));
#278589=CARTESIAN_POINT('Ctrl Pts',(-110.217690968365,2.7521349883118,135.922737548286));
#278590=CARTESIAN_POINT('Ctrl Pts',(-110.496138592178,5.79383165759959,
131.255519261747));
#278591=CARTESIAN_POINT('Ctrl Pts',(-110.774586215991,3.51128007796473,
126.17370822153));
#278592=CARTESIAN_POINT('Ctrl Pts',(-111.053033839804,-1.99796635775128,
125.347240513325));
#278593=CARTESIAN_POINT('Ctrl Pts',(-111.331481463617,-5.67117931677705,
129.535599585778));
#278594=CARTESIAN_POINT('Ctrl Pts',(-111.60992908743,-4.13285553619637,
134.889888064022));
#278595=CARTESIAN_POINT('Ctrl Pts',(-111.888376711243,1.20336058093108,
136.489776408084));
#278596=CARTESIAN_POINT('Ctrl Pts',(-112.166824335056,5.43374711161577,
132.865045388662));
#278597=CARTESIAN_POINT('Ctrl Pts',(-112.445271958868,4.67078550002918,
127.34664573465));
#278598=CARTESIAN_POINT('Ctrl Pts',(-112.723719582681,-0.384399805526852,
125.005717139274));
#278599=CARTESIAN_POINT('Ctrl Pts',(-113.002167206494,-5.08634046877848,
127.993458620965));
#278600=CARTESIAN_POINT('Ctrl Pts',(-113.280614830307,-5.11418272276831,
133.564281717336));
#278601=CARTESIAN_POINT('Ctrl Pts',(-113.55906245412,-0.442340896249408,
136.598872152659));
#278602=CARTESIAN_POINT('Ctrl Pts',(-113.837510077933,4.63599060436829,
134.308589564856));
#278603=CARTESIAN_POINT('Ctrl Pts',(-114.115957701746,5.45407322030374,
128.798091765594));
#278604=CARTESIAN_POINT('Ctrl Pts',(-114.394405325558,1.26012899306928,
125.131257029612));
#278605=CARTESIAN_POINT('Ctrl Pts',(-114.672852949372,-4.09181221807183,
126.677727344441));
#278606=CARTESIAN_POINT('Ctrl Pts',(-114.951300573184,-5.68357789694507,
132.016372040028));
#278607=CARTESIAN_POINT('Ctrl Pts',(-115.229748196997,-2.05241314674147,
136.241237448422));
#278608=CARTESIAN_POINT('Ctrl Pts',(-115.50819582081,3.46481901936097,135.469878655457));
#278609=CARTESIAN_POINT('Ctrl Pts',(-115.786643444623,5.79805177248978,
130.411136708898));
#278610=CARTESIAN_POINT('Ctrl Pts',(-116.065091068436,2.80315819727665,
125.713748324348));
#278611=CARTESIAN_POINT('Ctrl Pts',(-116.343538692249,-2.76770081934284,
125.694383947029));
#278612=CARTESIAN_POINT('Ctrl Pts',(-116.621986316062,-5.79517799268792,
130.370838493694));
#278613=CARTESIAN_POINT('Ctrl Pts',(-116.900433939875,-3.49716970093708,
135.445678693465));
#278614=CARTESIAN_POINT('Ctrl Pts',(-117.178881563688,2.0145666997373,136.255374322477));
#278615=CARTESIAN_POINT('Ctrl Pts',(-117.4573291875,5.67501472040751,132.055854653499));
#278616=CARTESIAN_POINT('Ctrl Pts',(-117.735776811314,4.12040145290537,
126.706273104381));
#278617=CARTESIAN_POINT('Ctrl Pts',(-118.014224435126,-1.22065945701595,
125.122633777175));
#278618=CARTESIAN_POINT('Ctrl Pts',(-118.29267205894,-5.43999395846872,
128.760223848501));
#278619=CARTESIAN_POINT('Ctrl Pts',(-118.571119682752,-4.6602397705682,
134.276275748964));
#278620=CARTESIAN_POINT('Ctrl Pts',(-118.849567306565,0.402047101114997,
136.601807256156));
#278621=CARTESIAN_POINT('Ctrl Pts',(-119.128014930377,5.09487232796628,
133.599768523497));
#278622=CARTESIAN_POINT('Ctrl Pts',(-119.406462554191,5.10575878376697,
128.028886488555));
#278623=CARTESIAN_POINT('Ctrl Pts',(-119.684910178003,0.424702347469154,
125.008529588725));
#278624=CARTESIAN_POINT('Ctrl Pts',(-119.963357801817,-4.64663479828973,
127.314258262312));
#278625=CARTESIAN_POINT('Ctrl Pts',(-120.241805425629,-5.44794156515001,
132.827220499399));
#278626=CARTESIAN_POINT('Ctrl Pts',(-120.520253049442,-1.24285618037906,
136.48127332728));
#278627=CARTESIAN_POINT('Ctrl Pts',(-120.798700673255,4.10435331726091,
134.918520707537));
#278628=CARTESIAN_POINT('Ctrl Pts',(-121.077148297068,5.67986262514396,
129.575055953004));
#278629=CARTESIAN_POINT('Ctrl Pts',(-121.355595920881,2.03585565723516,
125.361262130332));
#278630=CARTESIAN_POINT('Ctrl Pts',(-121.634043544694,-3.47900320259493,
126.149409907283));
#278631=CARTESIAN_POINT('Ctrl Pts',(-121.912491168507,-5.79682807799514,
131.215229979999));
#278632=CARTESIAN_POINT('Ctrl Pts',(-122.19093879232,-2.78765114051323,
135.903481180724));
#278633=CARTESIAN_POINT('Ctrl Pts',(-122.469386416133,2.78324101077128,
135.905889689793));
#278634=CARTESIAN_POINT('Ctrl Pts',(-122.747834039945,5.79647064203949,
131.220242205036));
#278635=CARTESIAN_POINT('Ctrl Pts',(-123.026281663758,3.48302692660634,
126.152419858339));
#278636=CARTESIAN_POINT('Ctrl Pts',(-123.304729287571,-2.03114837905279,
125.359503809431));
#278637=CARTESIAN_POINT('Ctrl Pts',(-123.583176911384,-5.67879755147744,
129.570145171156));
#278638=CARTESIAN_POINT('Ctrl Pts',(-123.861624535197,-4.10790919877744,
134.914970233354));
#278639=CARTESIAN_POINT('Ctrl Pts',(-124.14007215901,1.23794702507767,136.482345873087));
#278640=CARTESIAN_POINT('Ctrl Pts',(-124.418519782823,5.44619040996103,
132.831930447996));
#278641=CARTESIAN_POINT('Ctrl Pts',(-124.696967406636,4.64965086928273,
127.318277401031));
#278642=CARTESIAN_POINT('Ctrl Pts',(-124.975415030448,-0.419690672193134,
125.00816452543));
#278643=CARTESIAN_POINT('Ctrl Pts',(-125.253862654262,-5.10335698895296,
128.024472698579));
#278644=CARTESIAN_POINT('Ctrl Pts',(-125.532310278074,-5.09728754571388,
133.595362064203));
#278645=CARTESIAN_POINT('Ctrl Pts',(-125.810757901887,-0.407059864303788,
136.601457448367));
#278646=CARTESIAN_POINT('Ctrl Pts',(-126.0892055257,4.65723594642128,134.280304048949));
#278647=CARTESIAN_POINT('Ctrl Pts',(-126.367653149513,5.44175944101008,
128.764928445366));
#278648=CARTESIAN_POINT('Ctrl Pts',(-126.646100773326,1.22557185403828,
125.123691376234));
#278649=CARTESIAN_POINT('Ctrl Pts',(-126.924548397139,-4.11685639428078,
126.702711823764));
#278650=CARTESIAN_POINT('Ctrl Pts',(-127.202996020952,-5.67609473587197,
132.050947136115));
#278651=CARTESIAN_POINT('Ctrl Pts',(-127.481443644765,-2.01927930784003,
136.253630337055));
#278652=CARTESIAN_POINT('Ctrl Pts',(-127.759891268577,3.4931551568182,135.44870087741));
#278653=CARTESIAN_POINT('Ctrl Pts',(-128.038338892391,5.79555068247735,
130.375849607603));
#278654=CARTESIAN_POINT('Ctrl Pts',(-128.316786516203,2.77211825933019,
125.696779022025));
#278655=CARTESIAN_POINT('Ctrl Pts',(-128.595234140016,-2.7987554186355,
125.711326403516));
#278656=CARTESIAN_POINT('Ctrl Pts',(-128.873681763829,-5.79770959367839,
130.406123419165));
#278657=CARTESIAN_POINT('Ctrl Pts',(-129.152129387642,-3.46885188599067,
135.466880965177));
#278658=CARTESIAN_POINT('Ctrl Pts',(-129.430577011455,2.04771124208698,
136.243010088514));
#278659=CARTESIAN_POINT('Ctrl Pts',(-129.709024635268,5.68252777494204,
132.021286040849));
#278660=CARTESIAN_POINT('Ctrl Pts',(-129.98747225908,4.09537888954061,126.681266979298));
#278661=CARTESIAN_POINT('Ctrl Pts',(-130.265919882893,-1.25522312496795,
125.130169546993));
#278662=CARTESIAN_POINT('Ctrl Pts',(-130.544367506706,-5.45233640868912,
128.793376508901));
#278663=CARTESIAN_POINT('Ctrl Pts',(-130.822815130519,-4.63901889426667,
134.304579624636));
#278664=CARTESIAN_POINT('Ctrl Pts',(-131.101262754332,0.437330355314798,
136.599252468079));
#278665=CARTESIAN_POINT('Ctrl Pts',(-131.379710378145,5.11179437313754,
133.568702797104));
#278666=CARTESIAN_POINT('Ctrl Pts',(-131.658158001958,5.08876908708517,
127.997857708758));
#278667=CARTESIAN_POINT('Ctrl Pts',(-131.936605625771,0.389413610192037,
125.006051688315));
#278668=CARTESIAN_POINT('Ctrl Pts',(-132.215053249584,-4.66779395055513,
127.342608310716));
#278669=CARTESIAN_POINT('Ctrl Pts',(-132.493500873397,-5.43552690515385,
132.860346187109));
#278670=CARTESIAN_POINT('Ctrl Pts',(-132.77194849721,-1.20827617416795,
136.488733765571));
#278671=CARTESIAN_POINT('Ctrl Pts',(-133.050396121022,4.12932133330617,
134.893460118082));
#278672=CARTESIAN_POINT('Ctrl Pts',(-133.328843744835,5.67227426403318,
129.540503793235));
#278673=CARTESIAN_POINT('Ctrl Pts',(-133.607291368648,2.00268425211708,
125.348970147109));
#278674=CARTESIAN_POINT('Ctrl Pts',(-133.885738992461,-3.50727475093002,
126.170673832692));
#278675=CARTESIAN_POINT('Ctrl Pts',(-134.164186616274,-5.79421959776922,
131.25050930539));
#278676=CARTESIAN_POINT('Ctrl Pts',(-134.442634240087,-2.75655969762259,
135.920355929551));
#278677=CARTESIAN_POINT('Ctrl Pts',(-134.7210818639,2.81424389921159,135.888852792264));
#278678=CARTESIAN_POINT('Ctrl Pts',(-134.999529487713,5.79889483612785,
131.18494973768));
#278679=CARTESIAN_POINT('Ctrl Pts',(-135.277977111526,3.45464471040472,
126.131303874523));
#278680=CARTESIAN_POINT('Ctrl Pts',(-135.556424735338,-2.06425513540386,
125.371968866708));
#278681=CARTESIAN_POINT('Ctrl Pts',(-135.834872359151,-5.68620535624619,
129.604736490841));
#278682=CARTESIAN_POINT('Ctrl Pts',(-136.113319982964,-4.08281064127246,
134.939900082537));
#278683=CARTESIAN_POINT('Ctrl Pts',(-136.391767606777,1.27248759664198,
136.474704938258));
#278684=CARTESIAN_POINT('Ctrl Pts',(-136.67021523059,5.45843189771781,132.798740374984));
#278685=CARTESIAN_POINT('Ctrl Pts',(-136.948662854403,4.62834394401342,
127.290038245509));
#278686=CARTESIAN_POINT('Ctrl Pts',(-137.227110478216,-0.454965987067202,
125.010826691762));
#278687=CARTESIAN_POINT('Ctrl Pts',(-137.505558102029,-5.12018440235748,
128.055589785961));
#278688=CARTESIAN_POINT('Ctrl Pts',(-137.784005725841,-5.0802034867949,
133.626338989485));
#278689=CARTESIAN_POINT('Ctrl Pts',(-138.062453349655,-0.371763748605222,
136.603827930521));
#278690=CARTESIAN_POINT('Ctrl Pts',(-138.340900973467,4.67830871288359,
134.251889730681));
#278691=CARTESIAN_POINT('Ctrl Pts',(-138.61934859728,5.42924401531914,128.731840697047));
#278692=CARTESIAN_POINT('Ctrl Pts',(-138.897796221093,1.19096930099152,
125.116336222143));
#278693=CARTESIAN_POINT('Ctrl Pts',(-139.176243844906,-4.14174801886209,
126.727848291193));
#278694=CARTESIAN_POINT('Ctrl Pts',(-139.454691468719,-5.66840124502105,
132.085476039479));
#278695=CARTESIAN_POINT('Ctrl Pts',(-139.733139092532,-1.98607064380098,
136.265821300996));
#278696=CARTESIAN_POINT('Ctrl Pts',(-140.011586716345,3.52136185412693,
135.427351001626));
#278697=CARTESIAN_POINT('Ctrl Pts',(-140.290034340158,5.79283483620279,
130.340578384942));
#278698=CARTESIAN_POINT('Ctrl Pts',(-140.56848196397,2.7409755995222,125.679998983016));
#278699=CARTESIAN_POINT('Ctrl Pts',(-140.846929587784,-2.82970630901691,
125.72845758426));
#278700=CARTESIAN_POINT('Ctrl Pts',(-141.125377211596,-5.80002635840773,
130.441423101462));
#278701=CARTESIAN_POINT('Ctrl Pts',(-141.403824835409,-3.44040553146196,
135.487910465481));
#278702=CARTESIAN_POINT('Ctrl Pts',(-141.682272459222,2.08077990574355,
136.230444323395));
#278703=CARTESIAN_POINT('Ctrl Pts',(-141.960720083035,5.68983026132012,
131.986672334579));
#278704=CARTESIAN_POINT('Ctrl Pts',(-142.239167706848,4.07020457040501,
126.656413636965));
#278705=CARTESIAN_POINT('Ctrl Pts',(-142.517615330661,-1.289740280165,125.137915576048));
#278706=CARTESIAN_POINT('Ctrl Pts',(-142.796062954474,-5.46447682057862,
128.826603687055));
#278707=CARTESIAN_POINT('Ctrl Pts',(-143.074510578287,-4.61762611741445,
134.332753798405));
#278708=CARTESIAN_POINT('Ctrl Pts',(-143.352958202099,0.472597404077474,
136.596482948152));
#278709=CARTESIAN_POINT('Ctrl Pts',(-143.631405825913,5.12852699888841,
133.537534636997));
#278710=CARTESIAN_POINT('Ctrl Pts',(-143.909853449725,5.07159082419343,
127.966932924958));
#278711=CARTESIAN_POINT('Ctrl Pts',(-144.188301073538,0.354110443050382,
125.003788646376));
#278712=CARTESIAN_POINT('Ctrl Pts',(-144.466748697351,-4.6887801359991,
127.371086635623));
#278713=CARTESIAN_POINT('Ctrl Pts',(-144.745196321164,-5.4229108297093,
132.893395689516));
#278714=CARTESIAN_POINT('Ctrl Pts',(-145.023643944977,-1.17365139483885,
136.495983567324));
#278715=CARTESIAN_POINT('Ctrl Pts',(-145.30209156879,4.15413633583088,134.868248005541));
#278716=CARTESIAN_POINT('Ctrl Pts',(-145.580539192603,5.66447571471356,
129.505998466145));
#278717=CARTESIAN_POINT('Ctrl Pts',(-145.858986816416,1.96943863679757,
125.336880315387));
#278718=CARTESIAN_POINT('Ctrl Pts',(-146.137434440228,-3.53541633590941,
126.192109461069));
#278719=CARTESIAN_POINT('Ctrl Pts',(-146.415882064041,-5.79139641060527,
131.285772098575));
#278720=CARTESIAN_POINT('Ctrl Pts',(-146.694329687854,-2.72536610939861,
135.937041103293));
#278721=CARTESIAN_POINT('Ctrl Pts',(-146.972777311667,2.84514250480927,
135.871627487008));
#278722=CARTESIAN_POINT('Ctrl Pts',(-147.25122493548,5.80110415003576,131.149643167454));
#278723=CARTESIAN_POINT('Ctrl Pts',(-147.529672559293,3.42613448107249,
126.110361052543));
#278724=CARTESIAN_POINT('Ctrl Pts',(-147.808120183106,-2.09728540002206,
125.38463522326));
#278725=CARTESIAN_POINT('Ctrl Pts',(-148.086567806919,-5.69340245658434,
129.639372263039));
#278726=CARTESIAN_POINT('Ctrl Pts',(-148.365015430732,-4.05756079371773,
134.964676687782));
#278727=CARTESIAN_POINT('Ctrl Pts',(-148.643463054544,1.30698101571045,
136.466853886735));
#278728=CARTESIAN_POINT('Ctrl Pts',(-148.921910678358,5.47047112127328,
132.765476399497));
#278729=CARTESIAN_POINT('Ctrl Pts',(-149.20035830217,4.60686551375719,127.261929314495));
#278730=CARTESIAN_POINT('Ctrl Pts',(-149.478805925983,-0.49022444300932,
125.013703539625));
#278731=CARTESIAN_POINT('Ctrl Pts',(-149.757253549796,-5.13682208544599,
128.086808730058));
#278732=CARTESIAN_POINT('Ctrl Pts',(-150.035701173609,-5.06293117906749,
133.657211345319));
#278733=CARTESIAN_POINT('Ctrl Pts',(-150.314148797422,-0.336453857064764,
136.605983511281));
#278734=CARTESIAN_POINT('Ctrl Pts',(-150.592596421235,4.69920812289605,
134.223347662954));
#278735=CARTESIAN_POINT('Ctrl Pts',(-150.871044045047,5.41652740699458,
128.698829746717));
#278736=CARTESIAN_POINT('Ctrl Pts',(-151.14949166886,1.15632261613933,125.109191839888));
#278737=CARTESIAN_POINT('Ctrl Pts',(-151.427939292673,-4.1664861694474,
126.753135815284));
#278738=CARTESIAN_POINT('Ctrl Pts',(-151.706386916486,-5.66049770947745,
132.119957470642));
#278739=CARTESIAN_POINT('Ctrl Pts',(-151.984834540299,-1.95278838518384,
136.277809888502));
#278740=CARTESIAN_POINT('Ctrl Pts',(-152.263282164112,3.54943806607717,
135.405829819234));
#278741=CARTESIAN_POINT('Ctrl Pts',(-152.541729787925,5.78990433430307,
130.3053243479));
#278742=CARTESIAN_POINT('Ctrl Pts',(-152.820177411738,2.70973137185537,
125.663408829112));
#278743=CARTESIAN_POINT('Ctrl Pts',(-153.09862503555,-2.86055234359039,
125.745776854456));
#278744=CARTESIAN_POINT('Ctrl Pts',(-153.377072659364,-5.80212820102742,
130.476736232542));
#278745=CARTESIAN_POINT('Ctrl Pts',(-153.655520283176,-3.41183169144105,
135.508766415124));
#278746=CARTESIAN_POINT('Ctrl Pts',(-153.933967906989,2.1137714653355,136.21767749275));
#278747=CARTESIAN_POINT('Ctrl Pts',(-154.212415530802,5.69692190894542,
131.952014817313));
#278748=CARTESIAN_POINT('Ctrl Pts',(-154.490863154615,4.04487942834225,
126.631713998332));
#278749=CARTESIAN_POINT('Ctrl Pts',(-154.769310778428,-1.32420964356211,
125.145871577308));
#278750=CARTESIAN_POINT('Ctrl Pts',(-155.047758402241,-5.47641474427016,
128.859904151722));
#278751=CARTESIAN_POINT('Ctrl Pts',(-155.326206026054,-4.59606223272787,
134.360797226267));
#278752=CARTESIAN_POINT('Ctrl Pts',(-155.604653649866,0.507846940569522,
136.593498799002));
#278753=CARTESIAN_POINT('Ctrl Pts',(-155.88310127368,5.14506958518534,133.50626519812));
#278754=CARTESIAN_POINT('Ctrl Pts',(-156.161548897493,5.05422463163864,
127.936113283085));
#278755=CARTESIAN_POINT('Ctrl Pts',(-156.439996521305,0.318794154216047,
125.001740546765));
#278756=CARTESIAN_POINT('Ctrl Pts',(-156.718444145118,-4.70959257697085,
127.399692181761));
#278757=CARTESIAN_POINT('Ctrl Pts',(-156.996891768931,-5.41009380630968,
132.926367781962));
#278758=CARTESIAN_POINT('Ctrl Pts',(-157.275339392744,-1.1389831254257,
136.503022463895));
#278759=CARTESIAN_POINT('Ctrl Pts',(-157.553787016557,4.17879740530553,
134.84288530416));
#278760=CARTESIAN_POINT('Ctrl Pts',(-157.83223464037,5.65646726616335,129.471541250343));
#278761=CARTESIAN_POINT('Ctrl Pts',(-158.110682264183,1.93612004320555,
125.324993083158));
#278762=CARTESIAN_POINT('Ctrl Pts',(-158.389129887996,-3.56342691473634,
126.213715998108));
#278763=CARTESIAN_POINT('Ctrl Pts',(-158.667577511808,-5.78835862111754,
131.321017052882));
#278764=CARTESIAN_POINT('Ctrl Pts',(-158.946025135621,-2.69407153173119,
135.95353608367));
#278765=CARTESIAN_POINT('Ctrl Pts',(-159.224472759434,2.87593568260513,
135.854214412314));
#278766=CARTESIAN_POINT('Ctrl Pts',(-159.502920383247,5.80309850189603,
131.114323802656));
#278767=CARTESIAN_POINT('Ctrl Pts',(-159.78136800706,3.39749729506709,126.089592168444));
#278768=CARTESIAN_POINT('Ctrl Pts',(-160.059815630873,-2.13023794895846,
125.39750240973));
#278769=CARTESIAN_POINT('Ctrl Pts',(-160.338263254686,-5.70038858580074,
129.674051204309));
#278770=CARTESIAN_POINT('Ctrl Pts',(-160.616710878499,-4.03216059175559,
134.989299130986));
#278771=CARTESIAN_POINT('Ctrl Pts',(-160.895158502312,1.34142600411673,
136.458793009441));
#278772=CARTESIAN_POINT('Ctrl Pts',(-161.173606126125,5.48230763450959,
132.732139754142));
#278773=CARTESIAN_POINT('Ctrl Pts',(-161.452053749937,4.58521637440516,
127.233951649575));
#278774=CARTESIAN_POINT('Ctrl Pts',(-161.730501373751,-0.525464733504406,
125.016794962416));
#278775=CARTESIAN_POINT('Ctrl Pts',(-162.008948997563,-5.15326942170307,
128.118128374039));
#278776=CARTESIAN_POINT('Ctrl Pts',(-162.287396621376,-5.04547126256333,
133.687977987722));
#278777=CARTESIAN_POINT('Ctrl Pts',(-162.565844245189,-0.301131498102361,
136.607924110772));
#278778=CARTESIAN_POINT('Ctrl Pts',(-162.844291869002,4.71993340202341,
134.194678903404));
#278779=CARTESIAN_POINT('Ctrl Pts',(-163.122739492814,5.40361008725504,
128.665896817606));
#278780=CARTESIAN_POINT('Ctrl Pts',(-163.401187116628,1.12163308332736,
125.102258494207));
#278781=CARTESIAN_POINT('Ctrl Pts',(-163.67963474044,-4.19106992935549,
126.778573459));
#278782=CARTESIAN_POINT('Ctrl Pts',(-163.958082364253,-5.65238442210956,
132.154390151878));
#278783=CARTESIAN_POINT('Ctrl Pts',(-164.236529988066,-1.91943376527495,
136.289595655332));
#278784=CARTESIAN_POINT('Ctrl Pts',(-164.514977611879,3.57738275229458,
135.384138127707));
#278785=CARTESIAN_POINT('Ctrl Pts',(-164.793425235692,5.78675928536899,
130.270088802833));
#278786=CARTESIAN_POINT('Ctrl Pts',(-165.071872859505,2.67838673409632,
125.647009175068));
#278787=CARTESIAN_POINT('Ctrl Pts',(-165.350320483318,-2.89129237934434,
125.763283572333));
#278788=CARTESIAN_POINT('Ctrl Pts',(-165.628768107131,-5.80401504365309,
130.512061503863));
#278789=CARTESIAN_POINT('Ctrl Pts',(-165.907215730944,-3.38313142474212,
135.52944804128));
#278790=CARTESIAN_POINT('Ctrl Pts',(-166.185663354757,2.14668469834846,
136.204710069657));
#278791=CARTESIAN_POINT('Ctrl Pts',(-166.464110978569,5.70380245503433,
131.917314773299));
#278792=CARTESIAN_POINT('Ctrl Pts',(-166.742558602383,4.01940440178476,
126.607168978656));
#278793=CARTESIAN_POINT('Ctrl Pts',(-167.021006226195,-1.3586299378839,
125.15403725596));
#278794=CARTESIAN_POINT('Ctrl Pts',(-167.299453850008,-5.48814973739939,
128.893276668938));
#278795=CARTESIAN_POINT('Ctrl Pts',(-167.577901473821,-4.57432803926507,
134.388708869063));
#278796=CARTESIAN_POINT('Ctrl Pts',(-167.856349097634,0.543077658606429,
136.590300131209));
#278797=CARTESIAN_POINT('Ctrl Pts',(-168.134796721447,5.16142151903669,
133.474895639175));
#278798=CARTESIAN_POINT('Ctrl Pts',(-168.413244345259,5.03667115293141,
127.905399925171));
#278799=CARTESIAN_POINT('Ctrl Pts',(-168.691691969073,0.283466052347084,
124.999907465374));
#278800=CARTESIAN_POINT('Ctrl Pts',(-168.970139592885,-4.7302305022577,
127.42842388914));
#278801=CARTESIAN_POINT('Ctrl Pts',(-169.248587216698,-5.39707630989451,
132.959261242652));
#278802=CARTESIAN_POINT('Ctrl Pts',(-169.527034840511,-1.10427265057399,
136.509850194457));
#278803=CARTESIAN_POINT('Ctrl Pts',(-169.805482464324,4.20330362790601,
134.81737295376));
#278804=CARTESIAN_POINT('Ctrl Pts',(-170.083930088137,5.6482492151383,129.437133422652));
#278805=CARTESIAN_POINT('Ctrl Pts',(-170.36237771195,1.90272970597286,125.313308890908));
#278806=CARTESIAN_POINT('Ctrl Pts',(-170.640825335763,-3.59130544946847,
126.235492643171));
#278807=CARTESIAN_POINT('Ctrl Pts',(-170.919272959575,-5.78510634187241,
131.356242862295));
#278808=CARTESIAN_POINT('Ctrl Pts',(-171.197720583389,-2.66267712425244,
135.969840259458));
#278809=CARTESIAN_POINT('Ctrl Pts',(-171.476168207202,2.90662229154664,
135.836614213432));
#278810=CARTESIAN_POINT('Ctrl Pts',(-171.754615831014,5.80487781780722,
131.07899295206));
#278811=CARTESIAN_POINT('Ctrl Pts',(-172.033063454828,3.36873421355001,
126.068997991823));
#278812=CARTESIAN_POINT('Ctrl Pts',(-172.31151107864,-2.16311156114431,
125.410569949319));
#278813=CARTESIAN_POINT('Ctrl Pts',(-172.589958702453,-5.70716348502144,
129.70877202961));
#278814=CARTESIAN_POINT('Ctrl Pts',(-172.868406326266,-4.00661097660031,
135.013766499754));
#278815=CARTESIAN_POINT('Ctrl Pts',(-173.146853950079,1.3758212854888,136.450522605077));
#278816=CARTESIAN_POINT('Ctrl Pts',(-173.425301573892,5.49394099882038,
132.698731674224));
#278817=CARTESIAN_POINT('Ctrl Pts',(-173.703749197705,4.56339732817417,
127.206106287473));
#278818=CARTESIAN_POINT('Ctrl Pts',(-173.982196821517,-0.560685552710569,
125.02010084558));
#278819=CARTESIAN_POINT('Ctrl Pts',(-174.260644445331,-5.1695258016666,
128.149547557344));
#278820=CARTESIAN_POINT('Ctrl Pts',(-174.539092069143,-5.02782438426607,
133.718637776622));
#278821=CARTESIAN_POINT('Ctrl Pts',(-174.817539692956,-0.265797980601551,
136.609649657082));
#278822=CARTESIAN_POINT('Ctrl Pts',(-175.095987316769,4.74048378228282,
134.165884514362));
#278823=CARTESIAN_POINT('Ctrl Pts',(-175.374434940582,5.39049253475655,
128.633043130058));
#278824=CARTESIAN_POINT('Ctrl Pts',(-175.652882564395,1.08690198798901,
125.095536442018));
#278825=CARTESIAN_POINT('Ctrl Pts',(-175.931330188208,-4.21549838762608,
126.80416027974));
#278826=CARTESIAN_POINT('Ctrl Pts',(-176.209777812021,-5.64406168355824,
132.188772807274));
#278827=CARTESIAN_POINT('Ctrl Pts',(-176.488225435833,-1.886008020042,136.301178164761));
#278828=CARTESIAN_POINT('Ctrl Pts',(-176.766673059646,3.60519487727851,
135.362276730843));
#278829=CARTESIAN_POINT('Ctrl Pts',(-177.045120683459,5.78339980594152,
130.234873055403));
#278830=CARTESIAN_POINT('Ctrl Pts',(-177.323568307272,2.64694284773159,
125.630800628577));
#278831=CARTESIAN_POINT('Ctrl Pts',(-177.602015931085,-2.92192527719638,
125.780977089175));
#278832=CARTESIAN_POINT('Ctrl Pts',(-177.880463554898,-5.80568681636668,
130.547397606436));
#278833=CARTESIAN_POINT('Ctrl Pts',(-178.158911178711,-3.35430579486411,
135.549954577584));
#278834=CARTESIAN_POINT('Ctrl Pts',(-178.437358802524,2.17951838517049,
136.191542534628));
#278835=CARTESIAN_POINT('Ctrl Pts',(-178.715806426336,5.71047164462571,
131.88257348836));
#278836=CARTESIAN_POINT('Ctrl Pts',(-178.99425405015,3.99378043471903,126.582779487459));
#278837=CARTESIAN_POINT('Ctrl Pts',(-179.272701673962,-1.39299988767372,
125.162412309422));
#278838=CARTESIAN_POINT('Ctrl Pts',(-179.551149297775,-5.49968136512185,
128.926720002072));
#278839=CARTESIAN_POINT('Ctrl Pts',(-179.829596921588,-4.55242434239454,
134.416487692516));
#278840=CARTESIAN_POINT('Ctrl Pts',(-180.108044545401,0.578288252700551,
136.5868870633));
#278841=CARTESIAN_POINT('Ctrl Pts',(-180.386492169214,5.17758219451528,
133.443427122574));
#278842=CARTESIAN_POINT('Ctrl Pts',(-180.664939793027,5.01893103852278,
127.874793989312));
#278843=CARTESIAN_POINT('Ctrl Pts',(-180.94338741684,0.248127446539293,
124.998289470128));
#278844=CARTESIAN_POINT('Ctrl Pts',(-181.221835040653,-4.75069314711374,
127.457280693096));
#278845=CARTESIAN_POINT('Ctrl Pts',(-181.500282664465,-5.38385882283189,
132.992074852706));
#278846=CARTESIAN_POINT('Ctrl Pts',(-181.778730288279,-1.06952125649312,
136.516466506004));
#278847=CARTESIAN_POINT('Ctrl Pts',(-182.057177912091,4.22765409554481,
134.791711899713));
#278848=CARTESIAN_POINT('Ctrl Pts',(-182.335625535904,5.63982186616143,
129.402776258069));
#278849=CARTESIAN_POINT('Ctrl Pts',(-182.614073159717,1.86926886239121,
125.301828171599));
#278850=CARTESIAN_POINT('Ctrl Pts',(-182.89252078353,-3.61905090705647,
126.257438589318));
#278851=CARTESIAN_POINT('Ctrl Pts',(-183.170968407343,-5.78163969338434,
131.391448221508));
#278852=CARTESIAN_POINT('Ctrl Pts',(-183.449416031155,-2.63118405029363,
135.985953026497));
#278853=CARTESIAN_POINT('Ctrl Pts',(-183.727863654969,2.93720119453022,
135.818827542541));
#278854=CARTESIAN_POINT('Ctrl Pts',(-184.006311278781,5.80644203183612,
131.04365192486));
#278855=CARTESIAN_POINT('Ctrl Pts',(-184.284758902595,3.33984630234777,
126.048579285806));
#278856=CARTESIAN_POINT('Ctrl Pts',(-184.563206526407,-2.19590501843575,
125.423837357804));
#278857=CARTESIAN_POINT('Ctrl Pts',(-184.84165415022,-5.71372690320071,
129.743533452349));
#278858=CARTESIAN_POINT('Ctrl Pts',(-185.120101774033,-3.98091289500146,
135.03807788744));
#278859=CARTESIAN_POINT('Ctrl Pts',(-185.398549397846,1.41016558529749,
136.442042980103));
#278860=CARTESIAN_POINT('Ctrl Pts',(-185.676997021659,5.50537078312707,
132.665253397689));
#278861=CARTESIAN_POINT('Ctrl Pts',(-185.955444645472,4.54140918357699,
127.178394260007));
#278862=CARTESIAN_POINT('Ctrl Pts',(-186.233892269285,-0.595885595507362,
125.023621066618));
#278863=CARTESIAN_POINT('Ctrl Pts',(-186.512339893098,-5.18559062295048,
128.181065115723));
#278864=CARTESIAN_POINT('Ctrl Pts',(-186.79078751691,-5.00999119808726,
133.749189575911));
#278865=CARTESIAN_POINT('Ctrl Pts',(-187.069235140724,-0.230454613858838,
136.611160086272));
#278866=CARTESIAN_POINT('Ctrl Pts',(-187.347682764536,4.76085850217237,
134.136965562817));
#278867=CARTESIAN_POINT('Ctrl Pts',(-187.626130388349,5.37717523557474,
128.600269901479));
#278868=CARTESIAN_POINT('Ctrl Pts',(-187.904578012162,1.05213061709833,
125.089025932407));
#278869=CARTESIAN_POINT('Ctrl Pts',(-188.183025635975,-4.23977063905356,
126.829895329374));
#278870=CARTESIAN_POINT('Ctrl Pts',(-188.461473259788,-5.63552980222562,
132.223104162766));
#278871=CARTESIAN_POINT('Ctrl Pts',(-188.739920883601,-1.85251238808831,
136.312556987595));
#278872=CARTESIAN_POINT('Ctrl Pts',(-189.018368507414,3.63287341044046,
135.340246438718));
#278873=CARTESIAN_POINT('Ctrl Pts',(-189.296816131227,5.77982602050738,
130.199678410544));
#278874=CARTESIAN_POINT('Ctrl Pts',(-189.575263755039,2.61540087792624,
125.614783790254));
#278875=CARTESIAN_POINT('Ctrl Pts',(-189.853711378852,-2.95244990203274,
125.798856749341));
#278876=CARTESIAN_POINT('Ctrl Pts',(-190.132159002665,-5.80714345722022,
130.582743230867));
#278877=CARTESIAN_POINT('Ctrl Pts',(-190.410606626478,-3.32535586995153,
135.570285264159));
#278878=CARTESIAN_POINT('Ctrl Pts',(-190.689054250291,2.21227130913674,
136.178175375592));
#278879=CARTESIAN_POINT('Ctrl Pts',(-190.967501874104,5.7169292305904,131.847792249846));
#278880=CARTESIAN_POINT('Ctrl Pts',(-191.245949497917,3.96800847665057,
126.558546428502));
#278881=CARTESIAN_POINT('Ctrl Pts',(-191.52439712173,-1.4273182193404,125.170996427354));
#278882=CARTESIAN_POINT('Ctrl Pts',(-191.802844745543,-5.51100920012879,
128.960232911869));
#278883=CARTESIAN_POINT('Ctrl Pts',(-192.081292369355,-4.53035195376586,
134.444132667273));
#278884=CARTESIAN_POINT('Ctrl Pts',(-192.359739993168,0.613477418111232,
136.583259721745));
#278885=CARTESIAN_POINT('Ctrl Pts',(-192.638187616981,5.19355101278185,
133.411860814392));
#278886=CARTESIAN_POINT('Ctrl Pts',(-192.916635240794,5.00100494577841,
127.844296609621));
#278887=CARTESIAN_POINT('Ctrl Pts',(-193.195082864607,0.21277964627773,
124.996886620986));
#278888=CARTESIAN_POINT('Ctrl Pts',(-193.47353048842,-4.77097975328813,
127.486261524329));
#278889=CARTESIAN_POINT('Ctrl Pts',(-193.751978112233,-5.3704418349007,
133.024807396204));
#278890=CARTESIAN_POINT('Ctrl Pts',(-194.030425736046,-1.03473023090876,
136.522871153366));
#278891=CARTESIAN_POINT('Ctrl Pts',(-194.308873359859,4.25184790590635,
134.765903092897));
#278892=CARTESIAN_POINT('Ctrl Pts',(-194.587320983671,5.63118553151129,
129.368471029708));
#278893=CARTESIAN_POINT('Ctrl Pts',(-194.865768607484,1.83573875236439,
125.290551350653));
#278894=CARTESIAN_POINT('Ctrl Pts',(-195.144216231297,-3.64666225938173,
126.279553023333));
#278895=CARTESIAN_POINT('Ctrl Pts',(-195.42266385511,-5.77795880411129,
131.426631825972));
#278896=CARTESIAN_POINT('Ctrl Pts',(-195.701111478923,-2.59959347684268,
136.001873787725));
#278897=CARTESIAN_POINT('Ctrl Pts',(-195.979559102736,2.96767125844341,
135.800855058734));
#278898=CARTESIAN_POINT('Ctrl Pts',(-196.258006726549,5.80779108602021,
131.008302030633));
#278899=CARTESIAN_POINT('Ctrl Pts',(-196.536454350362,3.31083463191258,
126.028336807015));
#278900=CARTESIAN_POINT('Ctrl Pts',(-196.814901974175,-2.22861710565919,
125.437304143558));
#278901=CARTESIAN_POINT('Ctrl Pts',(-197.093349597988,-5.72007859712835,
129.778334184429));
#278902=CARTESIAN_POINT('Ctrl Pts',(-197.3717972218,-3.95506729921131,135.062232393175));
#278903=CARTESIAN_POINT('Ctrl Pts',(-197.650244845613,1.44445763090186,
136.433354448736));
#278904=CARTESIAN_POINT('Ctrl Pts',(-197.928692469426,5.51659656389443,
132.631706165088));
#278905=CARTESIAN_POINT('Ctrl Pts',(-198.207140093239,4.51925275539276,
127.150816594059));
#278906=CARTESIAN_POINT('Ctrl Pts',(-198.485587717052,-0.631063557543924,
125.027355495085));
#278907=CARTESIAN_POINT('Ctrl Pts',(-198.764035340865,-5.2014632902668,
128.212679881281));
#278908=CARTESIAN_POINT('Ctrl Pts',(-199.042482964678,-4.99197236484219,
133.779632253479));
#278909=CARTESIAN_POINT('Ctrl Pts',(-199.320930588491,-0.19510270753564,
136.612455342372));
#278910=CARTESIAN_POINT('Ctrl Pts',(-199.599378212304,4.7810568066993,134.10792312037));
#278911=CARTESIAN_POINT('Ctrl Pts',(-199.877825836116,5.36365868318719,
128.56757834629));
#278912=CARTESIAN_POINT('Ctrl Pts',(-200.156273459929,1.01732025912016,
125.082727206624));
#278913=CARTESIAN_POINT('Ctrl Pts',(-200.434721083742,-4.26388578422093,
126.855777654281));
#278914=CARTESIAN_POINT('Ctrl Pts',(-200.713168707555,-5.62678909426374,
132.257382946195));
#278915=CARTESIAN_POINT('Ctrl Pts',(-200.991616331368,-1.8189481106068,
136.323731702186));
#278916=CARTESIAN_POINT('Ctrl Pts',(-201.270063955181,3.66041732614217,
135.318048067677));
#278917=CARTESIAN_POINT('Ctrl Pts',(-201.548511578994,5.77603806149454,
130.164506172408));
#278918=CARTESIAN_POINT('Ctrl Pts',(-201.826959202806,2.58376199347953,
125.59895925361));
#278919=CARTESIAN_POINT('Ctrl Pts',(-202.10540682662,-2.9828651227522,125.816921890294));
#278920=CARTESIAN_POINT('Ctrl Pts',(-202.383854450432,-5.80838491223743,
130.618097067413));
#278921=CARTESIAN_POINT('Ctrl Pts',(-202.662302074245,-3.29628272275406,
135.590439347642));
#278922=CARTESIAN_POINT('Ctrl Pts',(-202.940749698058,2.24494225657654,
136.164609087875));
#278923=CARTESIAN_POINT('Ctrl Pts',(-203.219197321871,5.72317497363993,
131.812972346589));
#278924=CARTESIAN_POINT('Ctrl Pts',(-203.497644945684,3.94208948256877,
126.534470699752));
#278925=CARTESIAN_POINT('Ctrl Pts',(-203.776092569497,-1.46158366120557,
125.179789291667));
#278926=CARTESIAN_POINT('Ctrl Pts',(-204.05454019331,-5.52213282266317,
128.993814156497));
#278927=CARTESIAN_POINT('Ctrl Pts',(-204.332987817123,-4.5081116912795,
134.471642768938));
#278928=CARTESIAN_POINT('Ctrl Pts',(-204.611435440935,0.648643850890564,
136.579418240959));
#278929=CARTESIAN_POINT('Ctrl Pts',(-204.889883064748,5.20932738210573,
133.380197884332));
#278930=CARTESIAN_POINT('Ctrl Pts',(-205.168330688562,4.98289353895661,
127.813908916192));
#278931=CARTESIAN_POINT('Ctrl Pts',(-205.446778312374,0.177423961388546,
124.995698969927));
#278932=CARTESIAN_POINT('Ctrl Pts',(-205.725225936187,-4.79108956905296,
127.515365308944));
#278933=CARTESIAN_POINT('Ctrl Pts',(-206.00367356,-5.35682584327266,133.057457660231));
#278934=CARTESIAN_POINT('Ctrl Pts',(-206.282121183813,-0.999900863015179,
136.529063899218));
#278935=CARTESIAN_POINT('Ctrl Pts',(-206.560568807626,4.27588416248015,
134.739947489669));
#278936=CARTESIAN_POINT('Ctrl Pts',(-206.839016431439,5.62234053121038,
129.334219008764));
#278937=CARTESIAN_POINT('Ctrl Pts',(-207.117464055252,1.80214061836306,
125.279478845937));
#278938=CARTESIAN_POINT('Ctrl Pts',(-207.395911679064,-3.67413848329639,
126.301835125757));
#278939=CARTESIAN_POINT('Ctrl Pts',(-207.674359302878,-5.77406381044983,
131.461792371951));
#278940=CARTESIAN_POINT('Ctrl Pts',(-207.95280692669,-2.56790657449899,
136.01760195319));
#278941=CARTESIAN_POINT('Ctrl Pts',(-208.231254550503,2.99803135420673,
135.782697427989));
#278942=CARTESIAN_POINT('Ctrl Pts',(-208.509702174316,5.8089249303698,130.972944579282));
#278943=CARTESIAN_POINT('Ctrl Pts',(-208.788149798129,3.28170027728254,
126.008271305542));
#278944=CARTESIAN_POINT('Ctrl Pts',(-209.066597421942,-2.2612466106562,
125.450969807563));
#278945=CARTESIAN_POINT('Ctrl Pts',(-209.345045045754,-5.72621833144002,
129.813172936296));
#278946=CARTESIAN_POINT('Ctrl Pts',(-209.623492669568,-3.92907514694791,
135.086229121905));
#278947=CARTESIAN_POINT('Ctrl Pts',(-209.90194029338,1.4786961515975,136.424457332932));
#278948=CARTESIAN_POINT('Ctrl Pts',(-210.180387917194,5.52761792514773,
132.598091219525));
#278949=CARTESIAN_POINT('Ctrl Pts',(-210.458835541006,4.49692886463537,
127.123374311529));
#278950=CARTESIAN_POINT('Ctrl Pts',(-210.73728316482,-0.666218135288655,
125.031303992602));
#278951=CARTESIAN_POINT('Ctrl Pts',(-211.015730788632,-5.21714321544808,
128.244390682522));
#278952=CARTESIAN_POINT('Ctrl Pts',(-211.294178412445,-4.97376855222533,
133.809964681263));
#278953=CARTESIAN_POINT('Ctrl Pts',(-211.572626036258,-0.159743571609885,
136.613535377387));
#278954=CARTESIAN_POINT('Ctrl Pts',(-211.851073660071,4.80107794740803,
134.0787582632));
#278955=CARTESIAN_POINT('Ctrl Pts',(-212.129521283884,5.34994337845465,
128.534969675892));
#278956=CARTESIAN_POINT('Ctrl Pts',(-212.407968907697,0.982472203965689,
125.076640498072));
#278957=CARTESIAN_POINT('Ctrl Pts',(-212.686416531509,-4.28784292953254,
126.881806295382));
#278958=CARTESIAN_POINT('Ctrl Pts',(-212.964864155322,-5.61783988356258,
132.291607887347));
#278959=CARTESIAN_POINT('Ctrl Pts',(-213.243311779135,-1.78531643133465,
136.334701894451));
#278960=CARTESIAN_POINT('Ctrl Pts',(-213.521759402948,3.68782560373359,
135.295682440288));
#278961=CARTESIAN_POINT('Ctrl Pts',(-213.800207026761,5.77203606926717,
130.129357644311));
#278962=CARTESIAN_POINT('Ctrl Pts',(-214.078654650574,2.55202736678199,
125.583327605028));
#278963=CARTESIAN_POINT('Ctrl Pts',(-214.357102274386,-3.0131698123076,
125.835171842623));
#278964=CARTESIAN_POINT('Ctrl Pts',(-214.6355498982,-5.80941113541564,130.653457806023));
#278965=CARTESIAN_POINT('Ctrl Pts',(-214.913997522012,-3.26708743058812,
135.610416081219));
#278966=CARTESIAN_POINT('Ctrl Pts',(-215.192445145826,2.27753001685547,
136.15084417418));
#278967=CARTESIAN_POINT('Ctrl Pts',(-215.470892769638,5.72920864233609,
131.778115068854));
#278968=CARTESIAN_POINT('Ctrl Pts',(-215.749340393451,3.9160244129115,126.510553193344));
#278969=CARTESIAN_POINT('Ctrl Pts',(-216.027788017264,-1.49579494355069,
125.18879057654));
#278970=CARTESIAN_POINT('Ctrl Pts',(-216.306235641077,-5.53305182053502,
129.02746249159));
#278971=CARTESIAN_POINT('Ctrl Pts',(-216.58468326489,-4.48570437905656,
134.499016978113));
#278972=CARTESIAN_POINT('Ctrl Pts',(-216.863130888703,0.683786247933482,
136.57536276329));
#278973=CARTESIAN_POINT('Ctrl Pts',(-217.141578512516,5.2249107178877,133.348439505674));
#278974=CARTESIAN_POINT('Ctrl Pts',(-217.420026136328,4.96459748918233,
127.78363203505));
#278975=CARTESIAN_POINT('Ctrl Pts',(-217.698473760142,0.142061701988793,
124.994726560962));
#278976=CARTESIAN_POINT('Ctrl Pts',(-217.976921383954,-4.81102184923216,
127.544590968491));
#278977=CARTESIAN_POINT('Ctrl Pts',(-218.255369007768,-5.34301135249269,
133.090024434919));
#278978=CARTESIAN_POINT('Ctrl Pts',(-218.53381663158,-0.965034443427401,
136.535044514085));
#278979=CARTESIAN_POINT('Ctrl Pts',(-218.812264255394,4.29976197459382,
134.713846051821));
#278980=CARTESIAN_POINT('Ctrl Pts',(-219.090711879206,5.61328719301349,
129.300021464458));
#278981=CARTESIAN_POINT('Ctrl Pts',(-219.369159503019,1.76847570537835,
125.268611067748));
#278982=CARTESIAN_POINT('Ctrl Pts',(-219.647607126831,-3.70147856065836,
126.324284070919));
#278983=CARTESIAN_POINT('Ctrl Pts',(-219.926054750645,-5.76995485673049,
131.496928556552));
#278984=CARTESIAN_POINT('Ctrl Pts',(-220.204502374457,-2.5361245174328,
136.033136940081));
#278985=CARTESIAN_POINT('Ctrl Pts',(-220.48294999827,3.02828035681523,135.764355323142));
#278986=CARTESIAN_POINT('Ctrl Pts',(-220.761397622083,5.80984352286985,
130.937580880991));
#278987=CARTESIAN_POINT('Ctrl Pts',(-221.039845245896,3.25244431804234,
125.988383524923));
#278988=CARTESIAN_POINT('Ctrl Pts',(-221.318292869709,-2.29379232432851,
125.464833843433));
#278989=CARTESIAN_POINT('Ctrl Pts',(-221.596740493522,-5.73214587862558,
129.848048416986));
#278990=CARTESIAN_POINT('Ctrl Pts',(-221.875188117335,-3.90293740136003,
135.110067184424));
#278991=CARTESIAN_POINT('Ctrl Pts',(-222.153635741148,1.51287987866345,
136.415351962378));
#278992=CARTESIAN_POINT('Ctrl Pts',(-222.432083364961,5.53843445848603,
132.564409806615));
#278993=CARTESIAN_POINT('Ctrl Pts',(-222.710530988774,4.47443833852516,
127.0960684293));
#278994=CARTESIAN_POINT('Ctrl Pts',(-222.988978612586,-0.701348026075381,
125.035466412855));
#278995=CARTESIAN_POINT('Ctrl Pts',(-223.267426236399,-5.23262981746888,
128.27619634439));
#278996=CARTESIAN_POINT('Ctrl Pts',(-223.545873860212,-4.95538043478568,
133.840185735283));
#278997=CARTESIAN_POINT('Ctrl Pts',(-223.824321484025,-0.124378516327312,
136.614400151295));
#278998=CARTESIAN_POINT('Ctrl Pts',(-224.102769107838,4.82092118240782,
134.049472072021));
#278999=CARTESIAN_POINT('Ctrl Pts',(-224.381216731651,5.33602982960279,
128.502445098609));
#279000=CARTESIAN_POINT('Ctrl Pts',(-224.659664355464,0.947587742942381,
125.070766032295));
#279001=CARTESIAN_POINT('Ctrl Pts',(-224.938111979277,-4.31164118724753,
126.907980288176));
#279002=CARTESIAN_POINT('Ctrl Pts',(-225.216559603089,-5.60868250173869,
132.325777718005));
#279003=CARTESIAN_POINT('Ctrl Pts',(-225.495007226903,-1.75161859650508,
136.345467157888));
#279004=CARTESIAN_POINT('Ctrl Pts',(-225.773454850715,3.71509722759125,
135.273150385318));
#279005=CARTESIAN_POINT('Ctrl Pts',(-226.051902474528,5.7678201921206,130.0942341287));
#279006=CARTESIAN_POINT('Ctrl Pts',(-226.330350098341,2.52019817377184,
125.567889423742));
#279007=CARTESIAN_POINT('Ctrl Pts',(-226.608797722154,-3.04336284774751,
125.853605930069));
#279008=CARTESIAN_POINT('Ctrl Pts',(-226.887245345967,-5.81022208872781,
130.688824136393));
#279009=CARTESIAN_POINT('Ctrl Pts',(-227.16569296978,-3.23777107529596,
135.630214724643));
#279010=CARTESIAN_POINT('Ctrl Pts',(-227.444140593593,2.31003338242206,
136.13688114457));
#279011=CARTESIAN_POINT('Ctrl Pts',(-227.722588217406,5.73503001309909,
131.74322170829));
#279012=CARTESIAN_POINT('Ctrl Pts',(-228.001035841218,3.88981423352964,
126.486794795549));
#279013=CARTESIAN_POINT('Ctrl Pts',(-228.279483465031,-1.52995079866356,
125.197999948425));
#279014=CARTESIAN_POINT('Ctrl Pts',(-228.557931088844,-5.54376578913698,
129.061176670297));
#279015=CARTESIAN_POINT('Ctrl Pts',(-228.836378712657,-4.46313084740822,
134.526254280438));
#279016=CARTESIAN_POINT('Ctrl Pts',(-229.11482633647,0.718903307025501,
136.571093439014));
#279017=CARTESIAN_POINT('Ctrl Pts',(-229.393273960283,5.24030044268158,
133.316586855238));
#279018=CARTESIAN_POINT('Ctrl Pts',(-229.671721584096,4.94611747442232,
127.753467088116));
#279019=CARTESIAN_POINT('Ctrl Pts',(-229.950169207909,0.106694178440453,
124.993969430123));
#279020=CARTESIAN_POINT('Ctrl Pts',(-230.228616831722,-4.83077585522751,
127.57393742));
#279021=CARTESIAN_POINT('Ctrl Pts',(-230.507064455534,-5.32899887446215,
133.122506513493));
#279022=CARTESIAN_POINT('Ctrl Pts',(-230.785512079348,-0.930132264133436,
136.540812776352));
#279023=CARTESIAN_POINT('Ctrl Pts',(-231.06395970316,4.3234804574463,134.687599746553));
#279024=CARTESIAN_POINT('Ctrl Pts',(-231.342407326973,5.60402585239536,
129.265879663993));
#279025=CARTESIAN_POINT('Ctrl Pts',(-231.620854950786,1.73474526087603,
125.257948418793));
#279026=CARTESIAN_POINT('Ctrl Pts',(-231.899302574599,-3.72868147837107,
126.346899026965));
#279027=CARTESIAN_POINT('Ctrl Pts',(-232.177750198412,-5.76563209521201,
131.532039077795));
#279028=CARTESIAN_POINT('Ctrl Pts',(-232.456197822225,-2.50424848333998,
136.048478172742));
#279029=CARTESIAN_POINT('Ctrl Pts',(-232.734645446038,3.05841714538193,
135.745829423867));
#279030=CARTESIAN_POINT('Ctrl Pts',(-233.01309306985,5.81054682948159,130.902212246173));
#279031=CARTESIAN_POINT('Ctrl Pts',(-233.291540693664,3.22306783828139,
125.968674202107));
#279032=CARTESIAN_POINT('Ctrl Pts',(-233.569988317476,-2.32625304068266,
125.478895737432));
#279033=CARTESIAN_POINT('Ctrl Pts',(-233.84843594129,-5.73786101903762,
129.882959334177));
#279034=CARTESIAN_POINT('Ctrl Pts',(-234.126883565102,-3.87665503099142,
135.133745697402));
#279035=CARTESIAN_POINT('Ctrl Pts',(-234.405331188915,1.54700754540913,
136.406038674476));
#279036=CARTESIAN_POINT('Ctrl Pts',(-234.683778812728,5.54904576309872,
132.530663174436));
#279037=CARTESIAN_POINT('Ctrl Pts',(-234.962226436541,4.45178201045685,
127.0688999592));
#279038=CARTESIAN_POINT('Ctrl Pts',(-235.240674060353,-0.736451928153096,
125.039842601604));
#279039=CARTESIAN_POINT('Ctrl Pts',(-235.519121684167,-5.24792252246713,
128.308095688315));
#279040=CARTESIAN_POINT('Ctrl Pts',(-235.797569307979,-4.93680869390195,
133.870294295687));
#279041=CARTESIAN_POINT('Ctrl Pts',(-236.076016931792,-0.0890088521534987,
136.61504963205));
#279042=CARTESIAN_POINT('Ctrl Pts',(-236.354464555605,4.8405857764003,134.020065632043));
#279043=CARTESIAN_POINT('Ctrl Pts',(-236.632912179418,5.32191855220324,
128.470005819654));
#279044=CARTESIAN_POINT('Ctrl Pts',(-236.911359803231,0.912668168706789,
125.065104026974));
#279045=CARTESIAN_POINT('Ctrl Pts',(-237.189807427044,-4.33527967551271,
126.934298662776));
#279046=CARTESIAN_POINT('Ctrl Pts',(-237.468255050857,-5.59931728812211,
132.359891171993));
#279047=CARTESIAN_POINT('Ctrl Pts',(-237.74670267467,-1.71785585480426,
136.356027093583));
#279048=CARTESIAN_POINT('Ctrl Pts',(-238.025150298482,3.7422311871549,135.250452737698));
#279049=CARTESIAN_POINT('Ctrl Pts',(-238.303597922296,5.76339058627568,
130.059136927086));
#279050=CARTESIAN_POINT('Ctrl Pts',(-238.582045546108,2.48827559389159,
125.552645281824));
#279051=CARTESIAN_POINT('Ctrl Pts',(-238.860493169922,-3.07344311025789,
125.87222346955));
#279052=CARTESIAN_POINT('Ctrl Pts',(-239.138940793734,-5.81081774212379,
130.724194748009));
#279053=CARTESIAN_POINT('Ctrl Pts',(-239.417388417547,-3.20833474320591,
135.649834544268));
#279054=CARTESIAN_POINT('Ctrl Pts',(-239.69583604136,2.34245114885216,136.12272051645));
#279055=CARTESIAN_POINT('Ctrl Pts',(-239.974283665173,5.7406388702159,131.708293557882));
#279056=CARTESIAN_POINT('Ctrl Pts',(-240.252731288985,3.86345991565072,
126.463196386742));
#279057=CARTESIAN_POINT('Ctrl Pts',(-240.531178912799,-1.56404996088748,
125.207417066067));
#279058=CARTESIAN_POINT('Ctrl Pts',(-240.809626536611,-5.5542743314588,
129.094955443325));
#279059=CARTESIAN_POINT('Ctrl Pts',(-241.088074160425,-4.44039193280503,
134.553353666625));
#279060=CARTESIAN_POINT('Ctrl Pts',(-241.366521784237,0.753993726891117,
136.566610426332));
#279061=CARTESIAN_POINT('Ctrl Pts',(-241.64496940805,5.25549598621542,133.284641113335));
#279062=CARTESIAN_POINT('Ctrl Pts',(-241.923417031863,4.92745417946037,
127.723415193164));
#279063=CARTESIAN_POINT('Ctrl Pts',(-242.201864655676,0.071322701300089,
124.993427605467));
#279064=CARTESIAN_POINT('Ctrl Pts',(-242.480312279489,-4.85035085504701,
127.603403576029));
#279065=CARTESIAN_POINT('Ctrl Pts',(-242.758759903302,-5.31478892841856,
133.154902692318));
#279066=CARTESIAN_POINT('Ctrl Pts',(-243.037207527115,-0.895195618446729,
136.546368472274));
#279067=CARTESIAN_POINT('Ctrl Pts',(-243.315655150928,4.34703873214009,
134.661209546432));
#279068=CARTESIAN_POINT('Ctrl Pts',(-243.59410277474,5.59455685253872,129.231794872506));
#279069=CARTESIAN_POINT('Ctrl Pts',(-243.872550398553,1.7009505347501,125.247491294183));
#279070=CARTESIAN_POINT('Ctrl Pts',(-244.150998022366,-3.75574622842035,
126.36967915589));
#279071=CARTESIAN_POINT('Ctrl Pts',(-244.429445646179,-5.76109568607594,
131.567122634643));
#279072=CARTESIAN_POINT('Ctrl Pts',(-244.707893269992,-2.47227965339868,
136.063625082699));
#279073=CARTESIAN_POINT('Ctrl Pts',(-244.986340893805,3.08844060317656,
135.727120416648));
#279074=CARTESIAN_POINT('Ctrl Pts',(-245.264788517618,5.81103482414375,
130.866839985428));
#279075=CARTESIAN_POINT('Ctrl Pts',(-245.543236141431,3.1935719265564,125.949144067427));
#279076=CARTESIAN_POINT('Ctrl Pts',(-245.821683765243,-2.35862755687492,
125.49315496849));
#279077=CARTESIAN_POINT('Ctrl Pts',(-246.100131389057,-5.74336354089951,
129.917904394232));
#279078=CARTESIAN_POINT('Ctrl Pts',(-246.378579012869,-3.85022900974501,
135.157263783424));
#279079=CARTESIAN_POINT('Ctrl Pts',(-246.657026636682,1.58107788722132,
136.396517814333));
#279080=CARTESIAN_POINT('Ctrl Pts',(-246.935474260495,5.55945144577998,
132.496852573479));
#279081=CARTESIAN_POINT('Ctrl Pts',(-247.213921884308,4.42896071996899,
127.04186990797));
#279082=CARTESIAN_POINT('Ctrl Pts',(-247.492369508121,-0.77152854073377,
125.044432396689));
#279083=CARTESIAN_POINT('Ctrl Pts',(-247.770817131934,-5.26302076376676,
128.340087532256));
#279084=CARTESIAN_POINT('Ctrl Pts',(-248.049264755747,-4.91805401775627,
133.90028924679));
#279085=CARTESIAN_POINT('Ctrl Pts',(-248.32771237956,-0.0536358897235281,
136.615483795589));
#279086=CARTESIAN_POINT('Ctrl Pts',(-248.606160003372,4.86007100070672,
133.990540032933));
#279087=CARTESIAN_POINT('Ctrl Pts',(-248.884607627186,5.30761006915461,
128.437653041073));
#279088=CARTESIAN_POINT('Ctrl Pts',(-249.163055250998,0.877714775216597,
125.059654691916));
#279089=CARTESIAN_POINT('Ctrl Pts',(-249.441502874812,-4.35875751839529,
126.960760443945));
#279090=CARTESIAN_POINT('Ctrl Pts',(-249.719950498624,-5.58974458974414,
132.393946985223));
#279091=CARTESIAN_POINT('Ctrl Pts',(-249.998398122437,-1.68402945732324,
136.366381310236));
#279092=CARTESIAN_POINT('Ctrl Pts',(-250.27684574625,3.76922647696617,135.227590338499));
#279093=CARTESIAN_POINT('Ctrl Pts',(-250.555293370063,5.75874741587205,
130.024067340013));
#279094=CARTESIAN_POINT('Ctrl Pts',(-250.833740993876,2.45626081004631,
125.537595744144));
#279095=CARTESIAN_POINT('Ctrl Pts',(-251.112188617689,-3.10340948520656,
125.891023771197));
#279096=CARTESIAN_POINT('Ctrl Pts',(-251.390636241501,-5.81119807352532,
130.759568330183));
#279097=CARTESIAN_POINT('Ctrl Pts',(-251.669083865314,-3.17877952510356,
135.669274813107));
#279098=CARTESIAN_POINT('Ctrl Pts',(-251.947531489127,2.37478211491517,
136.10836281449));
#279099=CARTESIAN_POINT('Ctrl Pts',(-252.22597911294,5.74603500580729,131.673331912019));
#279100=CARTESIAN_POINT('Ctrl Pts',(-252.504426736753,3.83696243592119,
126.439758841162));
#279101=CARTESIAN_POINT('Ctrl Pts',(-252.782874360566,-1.59809116681098,
125.217041580908));
#279102=CARTESIAN_POINT('Ctrl Pts',(-253.061321984379,-5.5645770578269,
129.128797558239));
#279103=CARTESIAN_POINT('Ctrl Pts',(-253.339769608192,-4.41748847836656,
134.580314133917));
#279104=CARTESIAN_POINT('Ctrl Pts',(-253.618217232004,0.789056208225191,
136.561913888683));
#279105=CARTESIAN_POINT('Ctrl Pts',(-253.896664855818,5.27049678355612,
133.252603468789));
#279106=CARTESIAN_POINT('Ctrl Pts',(-254.17511247963,4.90860829937749,127.693477454216));
#279107=CARTESIAN_POINT('Ctrl Pts',(-254.453560103444,0.0359485746511809,
124.993101125124));
#279108=CARTESIAN_POINT('Ctrl Pts',(-254.732007727256,-4.86974611083267,
127.632988310607));
#279109=CARTESIAN_POINT('Ctrl Pts',(-255.010455351069,-5.30038206451776,
133.187211835313));
#279110=CARTESIAN_POINT('Ctrl Pts',(-255.288902974882,-0.860225756393269,
136.55171127444));
#279111=CARTESIAN_POINT('Ctrl Pts',(-255.567350598695,4.37043584157037,
134.634676658854));
#279112=CARTESIAN_POINT('Ctrl Pts',(-255.845798222508,5.58488070320316,
129.197767919676));
#279113=CARTESIAN_POINT('Ctrl Pts',(-256.12424584632,1.66709247927321,125.23724089965));
#279114=CARTESIAN_POINT('Ctrl Pts',(-256.402693470134,-3.78267124144458,
126.39262206856));
#279115=CARTESIAN_POINT('Ctrl Pts',(-256.681141093946,-5.75634686702621,
131.602180844355));
#279116=CARTESIAN_POINT('Ctrl Pts',(-256.95958871776,-2.44021719259262,
136.078571600242));
#279117=CARTESIAN_POINT('Ctrl Pts',(-257.238036341572,3.118345804191,135.708239395799));
#279118=CARTESIAN_POINT('Ctrl Pts',(-257.516483965385,5.81131468939531,
130.8314457702));
#279119=CARTESIAN_POINT('Ctrl Pts',(-257.794931589198,3.16394407961038,
125.929830927563));
#279120=CARTESIAN_POINT('Ctrl Pts',(-258.073379213011,-2.39088900078744,
125.507540987923));
#279121=CARTESIAN_POINT('Ctrl Pts',(-258.351826836824,-5.74870171518396,
129.953014515613));
#279122=CARTESIAN_POINT('Ctrl Pts',(-258.630274460636,-3.82356878618261,
135.180370918811));
#279123=CARTESIAN_POINT('Ctrl Pts',(-258.908722084449,1.61491681105698,
136.387261181902));
#279124=CARTESIAN_POINT('Ctrl Pts',(-259.187169708263,5.56997747689423,
132.462088635074));
#279125=CARTESIAN_POINT('Ctrl Pts',(-259.465617332075,4.40535894966821,
127.016664495574));
#279126=CARTESIAN_POINT('Ctrl Pts',(-259.744064955888,-0.805411631290512,
125.046024618449));
#279127=CARTESIAN_POINT('Ctrl Pts',(-260.022512579701,-5.28013240410161,
128.378470706602));
#279128=CARTESIAN_POINT('Ctrl Pts',(-260.254552266212,-4.95911089365773,
132.993351965875));
#279129=CARTESIAN_POINT('Ctrl Pts',(-260.440213228287,-2.45877638613931,
135.28779596926));
#279130=CARTESIAN_POINT('Ctrl Pts',(-260.53305831576,-0.833059752290926,
135.715219187214));
#279131=CARTESIAN_POINT('Ctrl Pts',(-260.579495465929,-0.013892627260139,
135.717527172907));
#279132=CARTESIAN_POINT('Ctrl Pts',(-207.955946566515,5.91285886696315,
130.43400564734));
#279133=CARTESIAN_POINT('Ctrl Pts',(-207.96403085718,5.89480070884798,130.766618159613));
#279134=CARTESIAN_POINT('Ctrl Pts',(-207.961339644263,5.86589899174327,
131.093332415071));
#279135=CARTESIAN_POINT('Ctrl Pts',(-207.946271365849,5.81943915897531,
131.462598684382));
#279136=CARTESIAN_POINT('Ctrl Pts',(-207.944637644607,5.81466923197383,
131.499362911161));
#279137=CARTESIAN_POINT('Ctrl Pts',(-207.942857924687,5.80972272473499,
131.536391330104));
#279138=CARTESIAN_POINT('Ctrl Pts',(-207.942844083457,5.80968426884596,
131.536679137172));
#279139=CARTESIAN_POINT('Ctrl Pts',(-207.942816746832,5.80960834566923,
131.53724722448));
#279140=CARTESIAN_POINT('Ctrl Pts',(-207.942803251882,5.80957087889668,
131.537527504213));
#279141=CARTESIAN_POINT('Ctrl Pts',(-207.942782545224,5.80951341028276,
131.537957318521));
#279142=CARTESIAN_POINT('Ctrl Pts',(-207.942775338973,5.80949341406807,
131.538106854989));
#279143=CARTESIAN_POINT('Ctrl Pts',(-207.942762251891,5.80945710634709,
131.538378341032));
#279144=CARTESIAN_POINT('Ctrl Pts',(-207.94275637189,5.80944079587429,131.538500288738));
#279145=CARTESIAN_POINT('Ctrl Pts',(-207.942743776405,5.80940586278758,
131.538761446312));
#279146=CARTESIAN_POINT('Ctrl Pts',(-207.942737060443,5.80938723960864,
131.538900656877));
#279147=CARTESIAN_POINT('Ctrl Pts',(-207.942718928357,5.80933696868309,
131.539276397358));
#279148=CARTESIAN_POINT('Ctrl Pts',(-207.942707508596,5.80930531703825,
131.539512927819));
#279149=CARTESIAN_POINT('Ctrl Pts',(-207.942651664994,5.80915058405599,
131.540669022502));
#279150=CARTESIAN_POINT('Ctrl Pts',(-207.94260716388,5.80902742209205,131.541588572013));
#279151=CARTESIAN_POINT('Ctrl Pts',(-207.937191179903,5.79405539795786,
131.653292239375));
#279152=CARTESIAN_POINT('Ctrl Pts',(-207.930620303857,5.77795735485189,
131.763821827678));
#279153=CARTESIAN_POINT('Ctrl Pts',(-207.905019315672,5.72103221687411,
132.127689826094));
#279154=CARTESIAN_POINT('Ctrl Pts',(-207.880926532226,5.6753051964054,132.379606835433));
#279155=CARTESIAN_POINT('Ctrl Pts',(-207.850713743235,5.62477921028189,
132.630029653041));
#279156=CARTESIAN_POINT('Origin',(-192.718407221598,12.,130.804360617566));
#279157=CARTESIAN_POINT('',(-177.476367722507,12.,130.804360617566));
#279158=CARTESIAN_POINT('Origin',(-192.718407221598,12.,130.804360617566));
#279159=CARTESIAN_POINT('',(-177.476367722506,12.,130.804360617566));
#279160=CARTESIAN_POINT('',(-177.476367722507,-12.,130.804360617566));
#279161=CARTESIAN_POINT('',(-177.476367722506,12.,130.804360617566));
#279162=CARTESIAN_POINT('Origin',(-192.718407221598,-12.,130.804360617566));
#279163=CARTESIAN_POINT('Origin',(-192.718407221598,-12.,130.804360617566));
#279164=CARTESIAN_POINT('Origin',(-192.718407221598,12.,130.804360617566));
#279253=UNCERTAINTY_MEASURE_WITH_UNIT(LENGTH_MEASURE(0.01),#279267,
'DISTANCE_ACCURACY_VALUE',
'Maximum model space distance between geometric entities at asserted c
onnectivities');
#279255=UNCERTAINTY_MEASURE_WITH_UNIT(LENGTH_MEASURE(0.01),#279267,
'DISTANCE_ACCURACY_VALUE',
'Maximum model space distance between geometric entities at asserted c
onnectivities');
#279264=(
GEOMETRIC_REPRESENTATION_CONTEXT(3)
GLOBAL_UNCERTAINTY_ASSIGNED_CONTEXT((#279253))
GLOBAL_UNIT_ASSIGNED_CONTEXT((#279267,#279269,#279270))
REPRESENTATION_CONTEXT('','3D')
);
#279266=(
GEOMETRIC_REPRESENTATION_CONTEXT(3)
GLOBAL_UNCERTAINTY_ASSIGNED_CONTEXT((#279255))
GLOBAL_UNIT_ASSIGNED_CONTEXT((#279267,#279269,#279270))
REPRESENTATION_CONTEXT('','3D')
);
#279267=(
LENGTH_UNIT()
NAMED_UNIT(*)
SI_UNIT(.MILLI.,.METRE.)
);
#279269=(
NAMED_UNIT(*)
PLANE_ANGLE_UNIT()
SI_UNIT($,.RADIAN.)
);
#279270=(
NAMED_UNIT(*)
SI_UNIT($,.STERADIAN.)
SOLID_ANGLE_UNIT()
);
#279279=SHAPE_DEFINITION_REPRESENTATION(#279289,#279308);
#279289=PRODUCT_DEFINITION_SHAPE('',$,#279319);
#279308=SHAPE_REPRESENTATION('',(#15608),#279264);
#279310=PRODUCT_DEFINITION_CONTEXT('part definition',#279342,'design');
#279319=PRODUCT_DEFINITION('Shaft_02','Shaft_02',#279329,#279310);
#279329=PRODUCT_DEFINITION_FORMATION('',$,#279352);
#279342=APPLICATION_CONTEXT(
'Core Data for Automotive Mechanical Design Process');
#279343=PRODUCT_CONTEXT('part definition',#279342,'mechanical');
#279352=PRODUCT('Shaft_02','Shaft_02',$,(#279343));
#279355=PRESENTATION_STYLE_ASSIGNMENT((#279357));
#279357=SURFACE_STYLE_USAGE(.BOTH.,#279359);
#279359=SURFACE_SIDE_STYLE('',(#279361));
#279361=SURFACE_STYLE_FILL_AREA(#279363);
#279363=FILL_AREA_STYLE('Opaque(160,160,160)',(#279365));
#279365=FILL_AREA_STYLE_COLOUR('Opaque(160,160,160)',#279367);
#279367=COLOUR_RGB('Opaque(160,160,160)', 0.66274510, 0.83137255, 0.94901961);
ENDSEC;
END-ISO-10303-21;
